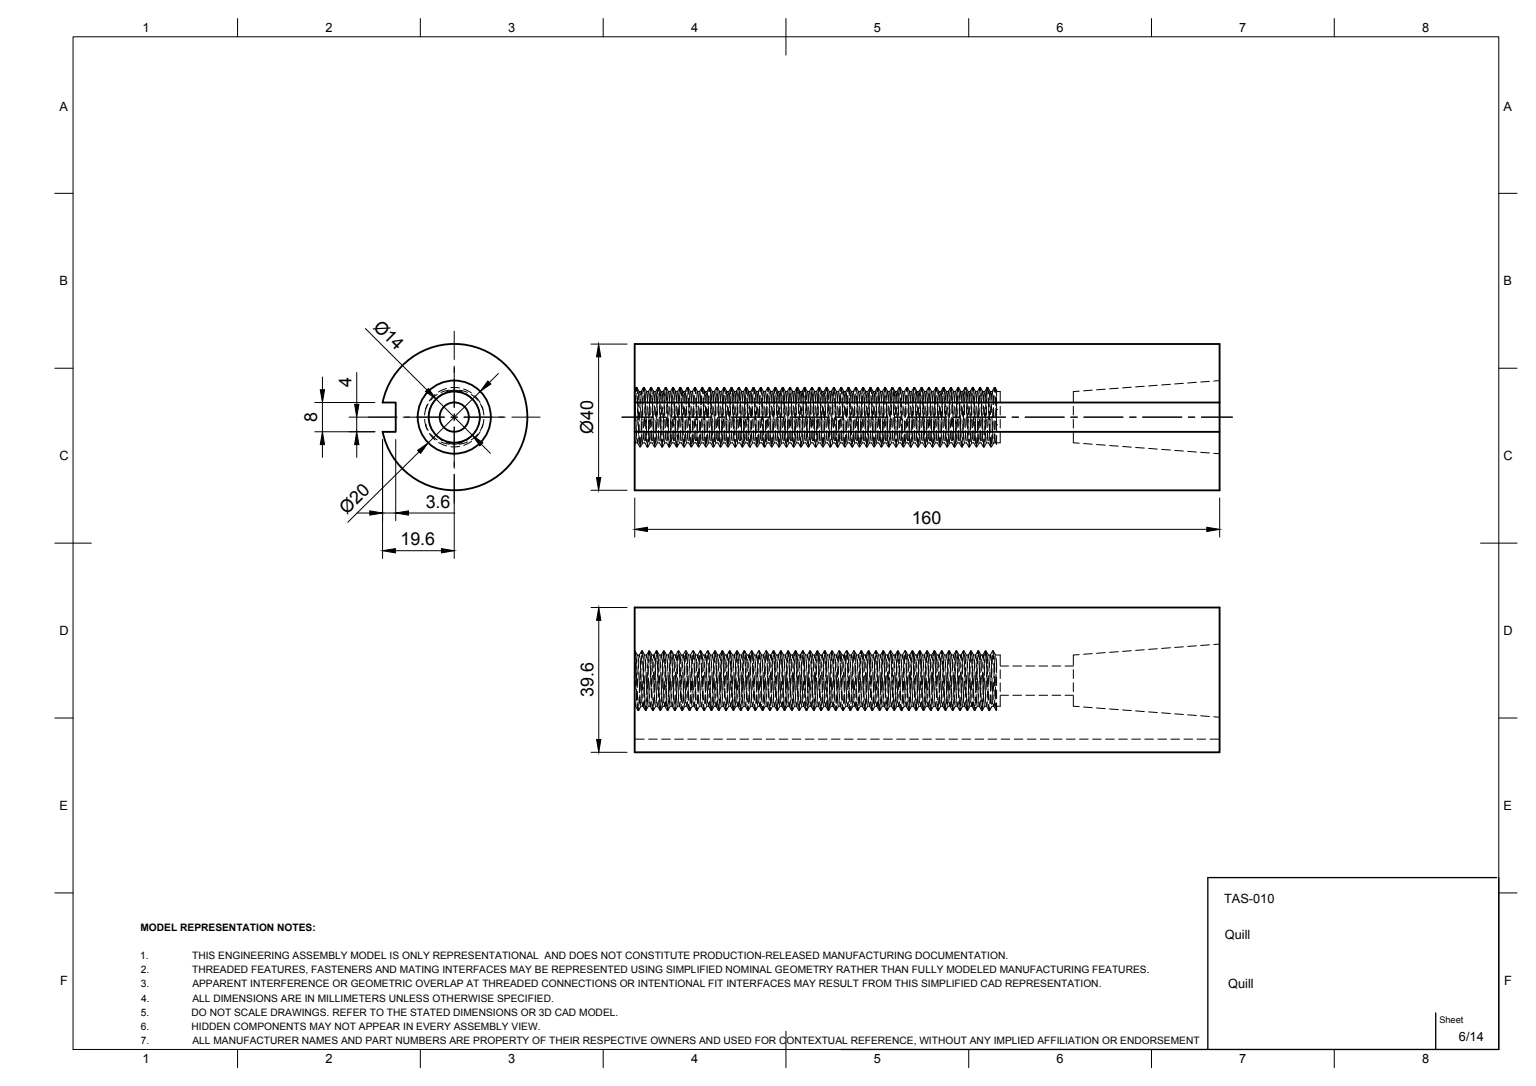
ISO-10303-21;
HEADER;
/* Generated by software containing ST-Developer
 * from STEP Tools, Inc. (www.steptools.com) 
 */

FILE_DESCRIPTION(
/* description */ (
'Independent keyed-quill tailstock, native coupled50mm slider andM16x2
 feed screw, conical dead center, bronze sleeves/thrust washers, cross
-pinned handwheel and bolted guide key. Custom center taper; no standa
rd taper compatibility, machine-bed compatibility or load rating assig
ned.'),
/* implementation_level */ '2;1');

FILE_NAME(
/* name */ 'Quill.step',
/* time_stamp */ '2026-11-14T07:17:36-08:00',
/* author */ (''),
/* organization */ (''),
/* preprocessor_version */ 'ST-DEVELOPER v20.2',
/* originating_system */ 'Autodesk Translation Framework v15.17.0.0',
/* authorisation */ '');

FILE_SCHEMA (('AUTOMOTIVE_DESIGN { 1 0 10303 214 3 1 1 }'));
ENDSEC;

DATA;
#10=MECHANICAL_DESIGN_GEOMETRIC_PRESENTATION_REPRESENTATION('',(#156),#289387);
#111=CONICAL_SURFACE('',#17511,8.5,0.0748598477107669);
#122=SHAPE_REPRESENTATION_RELATIONSHIP('SRR','None',#289457,#139);
#139=ADVANCED_BREP_SHAPE_REPRESENTATION('',(#173),#289373);
#156=STYLED_ITEM('',(#289551),#173);
#173=MANIFOLD_SOLID_BREP('Body1',#16844);
#218=FACE_BOUND('',#1502,.T.);
#219=FACE_BOUND('',#1508,.T.);
#220=FACE_BOUND('',#1513,.T.);
#221=FACE_BOUND('',#1517,.T.);
#293=B_SPLINE_SURFACE_WITH_KNOTS('',3,3,((#180613,#180614,#180615,#180616,
#180617,#180618,#180619,#180620,#180621,#180622,#180623,#180624,#180625,
#180626,#180627,#180628,#180629,#180630,#180631,#180632,#180633,#180634,
#180635,#180636,#180637,#180638,#180639,#180640,#180641,#180642,#180643,
#180644,#180645,#180646,#180647,#180648,#180649,#180650,#180651,#180652,
#180653,#180654,#180655,#180656,#180657,#180658,#180659,#180660,#180661,
#180662,#180663,#180664,#180665,#180666,#180667,#180668,#180669,#180670,
#180671,#180672,#180673,#180674,#180675,#180676,#180677,#180678,#180679,
#180680,#180681,#180682,#180683,#180684,#180685,#180686,#180687,#180688,
#180689,#180690,#180691,#180692,#180693,#180694,#180695,#180696,#180697,
#180698,#180699,#180700,#180701,#180702,#180703,#180704,#180705,#180706,
#180707,#180708,#180709,#180710,#180711,#180712,#180713,#180714,#180715,
#180716,#180717,#180718,#180719,#180720,#180721,#180722,#180723,#180724,
#180725,#180726,#180727,#180728,#180729,#180730,#180731,#180732,#180733,
#180734,#180735,#180736,#180737,#180738,#180739,#180740,#180741,#180742,
#180743,#180744,#180745,#180746,#180747,#180748,#180749,#180750,#180751,
#180752,#180753,#180754,#180755,#180756,#180757,#180758,#180759,#180760,
#180761,#180762,#180763,#180764,#180765,#180766,#180767,#180768,#180769,
#180770,#180771,#180772,#180773,#180774,#180775,#180776,#180777,#180778,
#180779,#180780,#180781,#180782,#180783,#180784,#180785,#180786,#180787,
#180788,#180789,#180790,#180791,#180792,#180793,#180794,#180795,#180796,
#180797,#180798,#180799,#180800,#180801,#180802,#180803,#180804,#180805,
#180806,#180807,#180808,#180809,#180810,#180811,#180812,#180813,#180814,
#180815,#180816,#180817,#180818,#180819,#180820,#180821,#180822,#180823,
#180824,#180825,#180826,#180827,#180828,#180829,#180830,#180831,#180832,
#180833,#180834,#180835,#180836,#180837,#180838,#180839,#180840,#180841,
#180842,#180843,#180844,#180845,#180846,#180847,#180848,#180849,#180850,
#180851,#180852,#180853,#180854,#180855,#180856,#180857,#180858,#180859,
#180860,#180861,#180862,#180863,#180864,#180865,#180866,#180867,#180868,
#180869,#180870,#180871,#180872,#180873,#180874,#180875,#180876,#180877,
#180878,#180879,#180880,#180881,#180882,#180883,#180884,#180885,#180886,
#180887,#180888,#180889,#180890,#180891,#180892,#180893,#180894,#180895,
#180896,#180897,#180898,#180899,#180900,#180901,#180902,#180903,#180904,
#180905,#180906,#180907,#180908,#180909,#180910,#180911,#180912,#180913,
#180914,#180915,#180916,#180917,#180918,#180919,#180920,#180921,#180922,
#180923,#180924,#180925,#180926,#180927,#180928,#180929,#180930,#180931,
#180932,#180933,#180934,#180935,#180936,#180937,#180938,#180939,#180940,
#180941,#180942,#180943,#180944,#180945,#180946,#180947,#180948,#180949,
#180950,#180951,#180952,#180953,#180954,#180955,#180956,#180957,#180958,
#180959,#180960,#180961,#180962,#180963,#180964,#180965,#180966,#180967,
#180968,#180969,#180970,#180971,#180972,#180973,#180974,#180975,#180976,
#180977,#180978,#180979,#180980,#180981,#180982,#180983,#180984,#180985,
#180986,#180987,#180988,#180989,#180990,#180991,#180992,#180993,#180994,
#180995,#180996,#180997,#180998,#180999,#181000,#181001,#181002,#181003,
#181004,#181005,#181006,#181007,#181008,#181009,#181010,#181011,#181012,
#181013,#181014,#181015,#181016,#181017,#181018,#181019,#181020,#181021,
#181022,#181023,#181024,#181025,#181026,#181027,#181028,#181029,#181030,
#181031,#181032,#181033,#181034,#181035,#181036,#181037,#181038,#181039,
#181040,#181041,#181042,#181043,#181044,#181045,#181046,#181047,#181048,
#181049,#181050,#181051,#181052,#181053,#181054,#181055,#181056,#181057,
#181058,#181059,#181060,#181061,#181062,#181063,#181064,#181065,#181066,
#181067,#181068,#181069,#181070,#181071,#181072,#181073,#181074,#181075,
#181076,#181077,#181078,#181079,#181080,#181081,#181082,#181083,#181084,
#181085,#181086,#181087,#181088,#181089,#181090,#181091,#181092,#181093,
#181094,#181095,#181096,#181097,#181098,#181099,#181100,#181101,#181102,
#181103,#181104,#181105,#181106,#181107,#181108,#181109,#181110,#181111,
#181112,#181113,#181114,#181115,#181116,#181117,#181118,#181119,#181120,
#181121,#181122,#181123,#181124,#181125,#181126,#181127,#181128,#181129,
#181130,#181131,#181132,#181133,#181134,#181135,#181136,#181137,#181138,
#181139,#181140,#181141,#181142,#181143,#181144,#181145,#181146,#181147,
#181148,#181149,#181150),(#181151,#181152,#181153,#181154,#181155,#181156,
#181157,#181158,#181159,#181160,#181161,#181162,#181163,#181164,#181165,
#181166,#181167,#181168,#181169,#181170,#181171,#181172,#181173,#181174,
#181175,#181176,#181177,#181178,#181179,#181180,#181181,#181182,#181183,
#181184,#181185,#181186,#181187,#181188,#181189,#181190,#181191,#181192,
#181193,#181194,#181195,#181196,#181197,#181198,#181199,#181200,#181201,
#181202,#181203,#181204,#181205,#181206,#181207,#181208,#181209,#181210,
#181211,#181212,#181213,#181214,#181215,#181216,#181217,#181218,#181219,
#181220,#181221,#181222,#181223,#181224,#181225,#181226,#181227,#181228,
#181229,#181230,#181231,#181232,#181233,#181234,#181235,#181236,#181237,
#181238,#181239,#181240,#181241,#181242,#181243,#181244,#181245,#181246,
#181247,#181248,#181249,#181250,#181251,#181252,#181253,#181254,#181255,
#181256,#181257,#181258,#181259,#181260,#181261,#181262,#181263,#181264,
#181265,#181266,#181267,#181268,#181269,#181270,#181271,#181272,#181273,
#181274,#181275,#181276,#181277,#181278,#181279,#181280,#181281,#181282,
#181283,#181284,#181285,#181286,#181287,#181288,#181289,#181290,#181291,
#181292,#181293,#181294,#181295,#181296,#181297,#181298,#181299,#181300,
#181301,#181302,#181303,#181304,#181305,#181306,#181307,#181308,#181309,
#181310,#181311,#181312,#181313,#181314,#181315,#181316,#181317,#181318,
#181319,#181320,#181321,#181322,#181323,#181324,#181325,#181326,#181327,
#181328,#181329,#181330,#181331,#181332,#181333,#181334,#181335,#181336,
#181337,#181338,#181339,#181340,#181341,#181342,#181343,#181344,#181345,
#181346,#181347,#181348,#181349,#181350,#181351,#181352,#181353,#181354,
#181355,#181356,#181357,#181358,#181359,#181360,#181361,#181362,#181363,
#181364,#181365,#181366,#181367,#181368,#181369,#181370,#181371,#181372,
#181373,#181374,#181375,#181376,#181377,#181378,#181379,#181380,#181381,
#181382,#181383,#181384,#181385,#181386,#181387,#181388,#181389,#181390,
#181391,#181392,#181393,#181394,#181395,#181396,#181397,#181398,#181399,
#181400,#181401,#181402,#181403,#181404,#181405,#181406,#181407,#181408,
#181409,#181410,#181411,#181412,#181413,#181414,#181415,#181416,#181417,
#181418,#181419,#181420,#181421,#181422,#181423,#181424,#181425,#181426,
#181427,#181428,#181429,#181430,#181431,#181432,#181433,#181434,#181435,
#181436,#181437,#181438,#181439,#181440,#181441,#181442,#181443,#181444,
#181445,#181446,#181447,#181448,#181449,#181450,#181451,#181452,#181453,
#181454,#181455,#181456,#181457,#181458,#181459,#181460,#181461,#181462,
#181463,#181464,#181465,#181466,#181467,#181468,#181469,#181470,#181471,
#181472,#181473,#181474,#181475,#181476,#181477,#181478,#181479,#181480,
#181481,#181482,#181483,#181484,#181485,#181486,#181487,#181488,#181489,
#181490,#181491,#181492,#181493,#181494,#181495,#181496,#181497,#181498,
#181499,#181500,#181501,#181502,#181503,#181504,#181505,#181506,#181507,
#181508,#181509,#181510,#181511,#181512,#181513,#181514,#181515,#181516,
#181517,#181518,#181519,#181520,#181521,#181522,#181523,#181524,#181525,
#181526,#181527,#181528,#181529,#181530,#181531,#181532,#181533,#181534,
#181535,#181536,#181537,#181538,#181539,#181540,#181541,#181542,#181543,
#181544,#181545,#181546,#181547,#181548,#181549,#181550,#181551,#181552,
#181553,#181554,#181555,#181556,#181557,#181558,#181559,#181560,#181561,
#181562,#181563,#181564,#181565,#181566,#181567,#181568,#181569,#181570,
#181571,#181572,#181573,#181574,#181575,#181576,#181577,#181578,#181579,
#181580,#181581,#181582,#181583,#181584,#181585,#181586,#181587,#181588,
#181589,#181590,#181591,#181592,#181593,#181594,#181595,#181596,#181597,
#181598,#181599,#181600,#181601,#181602,#181603,#181604,#181605,#181606,
#181607,#181608,#181609,#181610,#181611,#181612,#181613,#181614,#181615,
#181616,#181617,#181618,#181619,#181620,#181621,#181622,#181623,#181624,
#181625,#181626,#181627,#181628,#181629,#181630,#181631,#181632,#181633,
#181634,#181635,#181636,#181637,#181638,#181639,#181640,#181641,#181642,
#181643,#181644,#181645,#181646,#181647,#181648,#181649,#181650,#181651,
#181652,#181653,#181654,#181655,#181656,#181657,#181658,#181659,#181660,
#181661,#181662,#181663,#181664,#181665,#181666,#181667,#181668,#181669,
#181670,#181671,#181672,#181673,#181674,#181675,#181676,#181677,#181678,
#181679,#181680,#181681,#181682,#181683,#181684,#181685,#181686,#181687,
#181688),(#181689,#181690,#181691,#181692,#181693,#181694,#181695,#181696,
#181697,#181698,#181699,#181700,#181701,#181702,#181703,#181704,#181705,
#181706,#181707,#181708,#181709,#181710,#181711,#181712,#181713,#181714,
#181715,#181716,#181717,#181718,#181719,#181720,#181721,#181722,#181723,
#181724,#181725,#181726,#181727,#181728,#181729,#181730,#181731,#181732,
#181733,#181734,#181735,#181736,#181737,#181738,#181739,#181740,#181741,
#181742,#181743,#181744,#181745,#181746,#181747,#181748,#181749,#181750,
#181751,#181752,#181753,#181754,#181755,#181756,#181757,#181758,#181759,
#181760,#181761,#181762,#181763,#181764,#181765,#181766,#181767,#181768,
#181769,#181770,#181771,#181772,#181773,#181774,#181775,#181776,#181777,
#181778,#181779,#181780,#181781,#181782,#181783,#181784,#181785,#181786,
#181787,#181788,#181789,#181790,#181791,#181792,#181793,#181794,#181795,
#181796,#181797,#181798,#181799,#181800,#181801,#181802,#181803,#181804,
#181805,#181806,#181807,#181808,#181809,#181810,#181811,#181812,#181813,
#181814,#181815,#181816,#181817,#181818,#181819,#181820,#181821,#181822,
#181823,#181824,#181825,#181826,#181827,#181828,#181829,#181830,#181831,
#181832,#181833,#181834,#181835,#181836,#181837,#181838,#181839,#181840,
#181841,#181842,#181843,#181844,#181845,#181846,#181847,#181848,#181849,
#181850,#181851,#181852,#181853,#181854,#181855,#181856,#181857,#181858,
#181859,#181860,#181861,#181862,#181863,#181864,#181865,#181866,#181867,
#181868,#181869,#181870,#181871,#181872,#181873,#181874,#181875,#181876,
#181877,#181878,#181879,#181880,#181881,#181882,#181883,#181884,#181885,
#181886,#181887,#181888,#181889,#181890,#181891,#181892,#181893,#181894,
#181895,#181896,#181897,#181898,#181899,#181900,#181901,#181902,#181903,
#181904,#181905,#181906,#181907,#181908,#181909,#181910,#181911,#181912,
#181913,#181914,#181915,#181916,#181917,#181918,#181919,#181920,#181921,
#181922,#181923,#181924,#181925,#181926,#181927,#181928,#181929,#181930,
#181931,#181932,#181933,#181934,#181935,#181936,#181937,#181938,#181939,
#181940,#181941,#181942,#181943,#181944,#181945,#181946,#181947,#181948,
#181949,#181950,#181951,#181952,#181953,#181954,#181955,#181956,#181957,
#181958,#181959,#181960,#181961,#181962,#181963,#181964,#181965,#181966,
#181967,#181968,#181969,#181970,#181971,#181972,#181973,#181974,#181975,
#181976,#181977,#181978,#181979,#181980,#181981,#181982,#181983,#181984,
#181985,#181986,#181987,#181988,#181989,#181990,#181991,#181992,#181993,
#181994,#181995,#181996,#181997,#181998,#181999,#182000,#182001,#182002,
#182003,#182004,#182005,#182006,#182007,#182008,#182009,#182010,#182011,
#182012,#182013,#182014,#182015,#182016,#182017,#182018,#182019,#182020,
#182021,#182022,#182023,#182024,#182025,#182026,#182027,#182028,#182029,
#182030,#182031,#182032,#182033,#182034,#182035,#182036,#182037,#182038,
#182039,#182040,#182041,#182042,#182043,#182044,#182045,#182046,#182047,
#182048,#182049,#182050,#182051,#182052,#182053,#182054,#182055,#182056,
#182057,#182058,#182059,#182060,#182061,#182062,#182063,#182064,#182065,
#182066,#182067,#182068,#182069,#182070,#182071,#182072,#182073,#182074,
#182075,#182076,#182077,#182078,#182079,#182080,#182081,#182082,#182083,
#182084,#182085,#182086,#182087,#182088,#182089,#182090,#182091,#182092,
#182093,#182094,#182095,#182096,#182097,#182098,#182099,#182100,#182101,
#182102,#182103,#182104,#182105,#182106,#182107,#182108,#182109,#182110,
#182111,#182112,#182113,#182114,#182115,#182116,#182117,#182118,#182119,
#182120,#182121,#182122,#182123,#182124,#182125,#182126,#182127,#182128,
#182129,#182130,#182131,#182132,#182133,#182134,#182135,#182136,#182137,
#182138,#182139,#182140,#182141,#182142,#182143,#182144,#182145,#182146,
#182147,#182148,#182149,#182150,#182151,#182152,#182153,#182154,#182155,
#182156,#182157,#182158,#182159,#182160,#182161,#182162,#182163,#182164,
#182165,#182166,#182167,#182168,#182169,#182170,#182171,#182172,#182173,
#182174,#182175,#182176,#182177,#182178,#182179,#182180,#182181,#182182,
#182183,#182184,#182185,#182186,#182187,#182188,#182189,#182190,#182191,
#182192,#182193,#182194,#182195,#182196,#182197,#182198,#182199,#182200,
#182201,#182202,#182203,#182204,#182205,#182206,#182207,#182208,#182209,
#182210,#182211,#182212,#182213,#182214,#182215,#182216,#182217,#182218,
#182219,#182220,#182221,#182222,#182223,#182224,#182225,#182226),(#182227,
#182228,#182229,#182230,#182231,#182232,#182233,#182234,#182235,#182236,
#182237,#182238,#182239,#182240,#182241,#182242,#182243,#182244,#182245,
#182246,#182247,#182248,#182249,#182250,#182251,#182252,#182253,#182254,
#182255,#182256,#182257,#182258,#182259,#182260,#182261,#182262,#182263,
#182264,#182265,#182266,#182267,#182268,#182269,#182270,#182271,#182272,
#182273,#182274,#182275,#182276,#182277,#182278,#182279,#182280,#182281,
#182282,#182283,#182284,#182285,#182286,#182287,#182288,#182289,#182290,
#182291,#182292,#182293,#182294,#182295,#182296,#182297,#182298,#182299,
#182300,#182301,#182302,#182303,#182304,#182305,#182306,#182307,#182308,
#182309,#182310,#182311,#182312,#182313,#182314,#182315,#182316,#182317,
#182318,#182319,#182320,#182321,#182322,#182323,#182324,#182325,#182326,
#182327,#182328,#182329,#182330,#182331,#182332,#182333,#182334,#182335,
#182336,#182337,#182338,#182339,#182340,#182341,#182342,#182343,#182344,
#182345,#182346,#182347,#182348,#182349,#182350,#182351,#182352,#182353,
#182354,#182355,#182356,#182357,#182358,#182359,#182360,#182361,#182362,
#182363,#182364,#182365,#182366,#182367,#182368,#182369,#182370,#182371,
#182372,#182373,#182374,#182375,#182376,#182377,#182378,#182379,#182380,
#182381,#182382,#182383,#182384,#182385,#182386,#182387,#182388,#182389,
#182390,#182391,#182392,#182393,#182394,#182395,#182396,#182397,#182398,
#182399,#182400,#182401,#182402,#182403,#182404,#182405,#182406,#182407,
#182408,#182409,#182410,#182411,#182412,#182413,#182414,#182415,#182416,
#182417,#182418,#182419,#182420,#182421,#182422,#182423,#182424,#182425,
#182426,#182427,#182428,#182429,#182430,#182431,#182432,#182433,#182434,
#182435,#182436,#182437,#182438,#182439,#182440,#182441,#182442,#182443,
#182444,#182445,#182446,#182447,#182448,#182449,#182450,#182451,#182452,
#182453,#182454,#182455,#182456,#182457,#182458,#182459,#182460,#182461,
#182462,#182463,#182464,#182465,#182466,#182467,#182468,#182469,#182470,
#182471,#182472,#182473,#182474,#182475,#182476,#182477,#182478,#182479,
#182480,#182481,#182482,#182483,#182484,#182485,#182486,#182487,#182488,
#182489,#182490,#182491,#182492,#182493,#182494,#182495,#182496,#182497,
#182498,#182499,#182500,#182501,#182502,#182503,#182504,#182505,#182506,
#182507,#182508,#182509,#182510,#182511,#182512,#182513,#182514,#182515,
#182516,#182517,#182518,#182519,#182520,#182521,#182522,#182523,#182524,
#182525,#182526,#182527,#182528,#182529,#182530,#182531,#182532,#182533,
#182534,#182535,#182536,#182537,#182538,#182539,#182540,#182541,#182542,
#182543,#182544,#182545,#182546,#182547,#182548,#182549,#182550,#182551,
#182552,#182553,#182554,#182555,#182556,#182557,#182558,#182559,#182560,
#182561,#182562,#182563,#182564,#182565,#182566,#182567,#182568,#182569,
#182570,#182571,#182572,#182573,#182574,#182575,#182576,#182577,#182578,
#182579,#182580,#182581,#182582,#182583,#182584,#182585,#182586,#182587,
#182588,#182589,#182590,#182591,#182592,#182593,#182594,#182595,#182596,
#182597,#182598,#182599,#182600,#182601,#182602,#182603,#182604,#182605,
#182606,#182607,#182608,#182609,#182610,#182611,#182612,#182613,#182614,
#182615,#182616,#182617,#182618,#182619,#182620,#182621,#182622,#182623,
#182624,#182625,#182626,#182627,#182628,#182629,#182630,#182631,#182632,
#182633,#182634,#182635,#182636,#182637,#182638,#182639,#182640,#182641,
#182642,#182643,#182644,#182645,#182646,#182647,#182648,#182649,#182650,
#182651,#182652,#182653,#182654,#182655,#182656,#182657,#182658,#182659,
#182660,#182661,#182662,#182663,#182664,#182665,#182666,#182667,#182668,
#182669,#182670,#182671,#182672,#182673,#182674,#182675,#182676,#182677,
#182678,#182679,#182680,#182681,#182682,#182683,#182684,#182685,#182686,
#182687,#182688,#182689,#182690,#182691,#182692,#182693,#182694,#182695,
#182696,#182697,#182698,#182699,#182700,#182701,#182702,#182703,#182704,
#182705,#182706,#182707,#182708,#182709,#182710,#182711,#182712,#182713,
#182714,#182715,#182716,#182717,#182718,#182719,#182720,#182721,#182722,
#182723,#182724,#182725,#182726,#182727,#182728,#182729,#182730,#182731,
#182732,#182733,#182734,#182735,#182736,#182737,#182738,#182739,#182740,
#182741,#182742,#182743,#182744,#182745,#182746,#182747,#182748,#182749,
#182750,#182751,#182752,#182753,#182754,#182755,#182756,#182757,#182758,
#182759,#182760,#182761,#182762,#182763,#182764)),.UNSPECIFIED.,.F.,.F.,
 .F.,(4,4),(4,1,1,1,1,1,1,1,1,1,1,1,1,1,1,1,1,1,1,1,1,1,1,1,1,1,1,1,1,1,
1,1,1,1,1,1,1,1,1,1,1,1,1,1,1,1,1,1,1,1,1,1,1,1,1,1,1,1,1,1,1,1,1,1,1,1,
1,1,1,1,1,1,1,1,1,1,1,1,1,1,1,1,1,1,1,1,1,1,1,1,1,1,1,1,1,1,1,1,1,1,1,1,
1,1,1,1,1,1,1,1,1,1,1,1,1,1,1,1,1,1,1,1,1,1,1,1,1,1,1,1,1,1,1,1,1,1,1,1,
1,1,1,1,1,1,1,1,1,1,1,1,1,1,1,1,1,1,1,1,1,1,1,1,1,1,1,1,1,1,1,1,1,1,1,1,
1,1,1,1,1,1,1,1,1,1,1,1,1,1,1,1,1,1,1,1,1,1,1,1,1,1,1,1,1,1,1,1,1,1,1,1,
1,1,1,1,1,1,1,1,1,1,1,1,1,1,1,1,1,1,1,1,1,1,1,1,1,1,1,1,1,1,1,1,1,1,1,1,
1,1,1,1,1,1,1,1,1,1,1,1,1,1,1,1,1,1,1,1,1,1,1,1,1,1,1,1,1,1,1,1,1,1,1,1,
1,1,1,1,1,1,1,1,1,1,1,1,1,1,1,1,1,1,1,1,1,1,1,1,1,1,1,1,1,1,1,1,1,1,1,1,
1,1,1,1,1,1,1,1,1,1,1,1,1,1,1,1,1,1,1,1,1,1,1,1,1,1,1,1,1,1,1,1,1,1,1,1,
1,1,1,1,1,1,1,1,1,1,1,1,1,1,1,1,1,1,1,1,1,1,1,1,1,1,1,1,1,1,1,1,1,1,1,1,
1,1,1,1,1,1,1,1,1,1,1,1,1,1,1,1,1,1,1,1,1,1,1,1,1,1,1,1,1,1,1,1,1,1,1,1,
1,1,1,1,1,1,1,1,1,1,1,1,1,1,1,1,1,1,1,1,1,1,1,1,1,1,1,1,1,1,1,1,1,1,1,1,
1,1,1,1,1,1,1,1,1,1,1,1,1,1,1,1,1,1,1,1,1,1,1,1,1,1,1,1,1,1,1,1,1,1,1,1,
1,1,1,1,1,1,1,1,1,1,1,1,1,1,1,1,1,1,1,1,1,1,1,1,1,1,1,1,1,1,1,1,1,1,1,1,
1,4),(-0.000902833525214243,0.131480103365952),(11.8547611101884,12.3533763570464,
12.851844900354,13.3503134436615,13.8487819869691,14.3472505302766,14.8457190735842,
15.8426561601993,16.8395932468144,17.338061790122,17.8365303334295,18.3349988767371,
18.8334674200446,19.3319359633522,19.8304045066598,20.3288730499673,20.8273415932749,
21.82427867989,22.3227472231976,22.8212157665051,23.8181528531202,24.3166213964278,
24.8150899397353,25.3135584830429,25.8120270263505,26.310495569658,26.8089641129656,
27.3074326562731,27.8059011995807,28.8028382861958,29.3013068295034,29.7997753728109,
30.796712459426,31.2951810027336,31.7936495460412,32.2921180893487,32.7905866326563,
33.2890551759638,33.7875237192714,34.2859922625789,34.7844608058865,35.7813978925016,
36.2798664358092,36.7783349791167,37.7752720657319,38.2737406090394,38.772209152347,
39.2706776956545,39.7691462389621,40.2676147822696,40.7660833255772,41.2645518688848,
41.7630204121923,42.7599574988074,43.258426042115,43.7568945854225,44.7538316720377,
45.2523002153452,45.7507687586528,46.2492373019603,46.7477058452679,47.2461743885754,
47.744642931883,48.2431114751906,48.7415800184981,49.7385171051132,50.2369856484208,
50.7354541917284,51.7323912783435,52.230859821651,52.7293283649586,53.2277969082661,
53.7262654515737,54.2247339948813,54.7232025381888,55.2216710814964,55.7201396248039,
56.7170767114191,57.2155452547266,57.7140137980342,58.7109508846493,59.2094194279568,
59.7078879712644,60.206356514572,60.7048250578795,61.2032936011871,61.7017621444946,
62.2002306878022,62.6986992311097,63.6956363177249,64.1941048610324,64.69257340434,
65.6895104909551,66.1879790342627,66.6864475775702,67.1849161208778,67.6833846641853,
68.1818532074929,68.6803217508004,69.178790294108,69.6772588374156,70.6741959240307,
71.1726644673382,71.6711330106458,72.6680700972609,73.1665386405685,73.665007183876,
74.1634757271836,74.6619442704911,75.1604128137987,75.6588813571063,76.1573499004138,
76.6558184437214,77.6527555303365,78.151224073644,78.6496926169516,79.6466297035667,
80.1450982468743,80.6435667901818,81.1420353334894,81.6405038767969,82.1389724201045,
82.6374409634121,83.1359095067196,83.6343780500272,84.6313151366423,85.1297836799499,
85.6282522232574,86.6251893098725,87.1236578531801,87.6221263964876,88.1205949397952,
88.6190634831028,89.1175320264103,89.6160005697179,90.1144691130254,90.612937656333,
91.6098747429481,92.1083432862557,92.6068118295632,93.6037489161783,94.1022174594859,
94.6006860027935,95.099154546101,95.5976230894086,96.0960916327161,96.5945601760237,
97.0930287193312,97.5914972626388,98.5884343492539,99.0869028925615,99.585371435869,
100.582308522484,101.080777065792,101.579245609099,102.077714152407,102.576182695714,
103.074651239022,103.573119782329,104.071588325637,104.570056868945,105.56699395556,
106.065462498867,106.563931042175,107.56086812879,108.059336672098,108.557805215405,
109.056273758713,109.55474230202,110.053210845328,110.551679388635,111.050147931943,
111.54861647525,112.545553561866,113.044022105173,113.542490648481,114.539427735096,
115.037896278403,115.536364821711,116.034833365018,116.533301908326,117.031770451634,
117.530238994941,118.028707538249,118.527176081556,119.524113168171,120.022581711479,
120.521050254786,121.517987341402,122.016455884709,122.514924428017,123.013392971324,
123.511861514632,124.010330057939,124.508798601247,125.007267144555,125.505735687862,
126.502672774477,127.001141317785,127.499609861092,128.496546947707,128.995015491015,
129.493484034323,129.99195257763,130.490421120938,130.988889664245,131.487358207553,
131.98582675086,132.484295294168,133.481232380783,133.979700924091,134.478169467398,
135.475106554013,135.973575097321,136.472043640628,136.970512183936,137.468980727243,
137.967449270551,138.465917813859,138.964386357166,139.462854900474,140.459791987089,
140.958260530396,141.456729073704,142.453666160319,142.952134703627,143.450603246934,
143.949071790242,144.447540333549,144.946008876857,145.444477420164,145.942945963472,
146.441414506779,147.438351593395,147.936820136702,148.43528868001,149.432225766625,
149.930694309932,150.42916285324,150.927631396547,151.426099939855,151.924568483163,
152.42303702647,152.921505569778,153.419974113085,154.4169111997,154.915379743008,
155.413848286316,156.410785372931,156.909253916238,157.407722459546,157.906191002853,
158.404659546161,158.903128089468,159.401596632776,159.900065176084,160.398533719391,
161.395470806006,161.893939349314,162.392407892621,163.389344979236,163.887813522544,
164.386282065852,164.884750609159,165.383219152467,165.881687695774,166.380156239082,
167.377093325697,168.374030412312,169.370967498927,169.869436042235,170.367904585542,
170.86637312885,171.364841672157,172.361778758772,173.358715845388,174.355652932003,
174.85412147531,175.352590018618,176.349527105233,176.847995648541,177.346464191848,
177.844932735156,178.343401278463,178.841869821771,179.340338365078,179.838806908386,
180.337275451693,181.334212538309,181.832681081616,182.331149624924,183.328086711539,
183.826555254846,184.325023798154,184.823492341461,185.321960884769,185.820429428077,
186.318897971384,186.817366514692,187.315835057999,188.312772144614,188.811240687922,
189.309709231229,190.306646317845,190.805114861152,191.30358340446,191.802051947767,
192.300520491075,192.798989034382,193.29745757769,193.795926120997,194.294394664305,
195.29133175092,195.789800294228,196.288268837535,197.28520592415,197.783674467458,
198.282143010766,198.780611554073,199.279080097381,199.777548640688,200.276017183996,
200.774485727303,201.272954270611,202.269891357226,202.768359900534,203.266828443841,
204.263765530456,204.762234073764,205.260702617071,205.759171160379,206.257639703686,
206.756108246994,207.254576790302,207.753045333609,208.251513876917,209.248450963532,
209.746919506839,210.245388050147,211.242325136762,211.74079368007,212.239262223377,
212.737730766685,213.236199309992,213.7346678533,214.233136396607,214.731604939915,
215.230073483222,216.227010569838,216.725479113145,217.223947656453,218.220884743068,
218.719353286375,219.217821829683,219.71629037299,220.214758916298,220.713227459606,
221.211696002913,221.710164546221,222.208633089528,223.205570176143,223.704038719451,
224.202507262759,225.199444349374,225.697912892681,226.196381435989,226.694849979296,
227.193318522604,227.691787065911,228.190255609219,228.688724152527,229.187192695834,
230.184129782449,230.682598325757,231.181066869064,232.178003955679,232.676472498987,
233.174941042295,233.673409585602,234.17187812891,234.670346672217,235.168815215525,
235.667283758832,236.16575230214,237.162689388755,237.661157932063,238.15962647537,
239.156563561985,239.655032105293,240.1535006486,240.651969191908,241.150437735215,
241.648906278523,242.147374821831,242.645843365138,243.144311908446,244.141248995061,
244.639717538368,245.138186081676,246.135123168291,246.633591711599,247.132060254906,
247.630528798214,248.128997341521,248.627465884829,249.125934428136,249.624402971444,
250.122871514752,251.119808601367,251.618277144674,252.116745687982,253.113682774597,
253.612151317904,254.110619861212,254.60908840452,255.107556947827,255.606025491135,
256.104494034442,256.60296257775,257.101431121057,258.098368207672,258.59683675098,
259.095305294288,260.092242380903,260.59071092421,261.089179467518,261.587648010825,
262.086116554133,262.58458509744,263.083053640748,263.581522184056,264.079990727363,
265.076927813978,265.575396357286,266.073864900593,267.070801987209,267.569270530516,
268.067739073824,268.566207617131,269.064676160439,269.563144703746,270.061613247054,
270.560081790361,271.058550333669,272.055487420284,272.553955963592,273.052424506899,
274.049361593514,274.547830136822,275.046298680129,275.544767223437,276.043235766745,
276.541704310052,277.04017285336,277.538641396667,278.037109939975,279.03404702659,
279.532515569897,280.030984113205,281.02792119982,281.526389743128,282.024858286435,
282.523326829743,283.02179537305,283.520263916358,284.018732459666,284.517201002973,
285.015669546281,286.012606632896,286.511075176203,287.009543719511,288.006480806126,
288.504949349434,289.003417892741,289.501886436049,290.000354979356,290.498823522664,
290.997292065971,291.495760609279,291.994229152586,292.991166239202,293.489634782509,
293.988103325817,294.985040412432,295.483508955739,295.981977499047,296.480446042354,
296.978914585662,297.47738312897,297.975851672277,298.474320215585,298.972788758892,
299.969725845507,300.468194388815,300.966662932122,301.963600018738,302.462068562045,
302.960537105353,303.45900564866,303.957474191968,304.455942735275,304.954411278583,
305.452879821891,305.951348365198,306.948285451813,307.446753995121,307.945222538428,
308.942159625043,309.440628168351,309.939096711659,310.437565254966,310.936033798274,
311.434502341581,311.932970884889,312.431439428196,312.929907971504,313.926845058119,
314.425313601427,314.923782144734,315.920719231349,316.419187774657,316.917656317964,
317.416124861272,317.914593404579,318.413061947887,318.911530491195,319.409999034502,
319.90846757781,320.905404664425,321.90234175104,322.400810294347,322.899278837655,
323.397747380963,323.89621592427,324.394684467578,324.893207835215),
 .UNSPECIFIED.);
#294=B_SPLINE_SURFACE_WITH_KNOTS('',3,3,((#182877,#182878,#182879,#182880,
#182881,#182882,#182883,#182884,#182885,#182886,#182887,#182888,#182889,
#182890,#182891,#182892,#182893,#182894,#182895,#182896,#182897,#182898,
#182899,#182900,#182901,#182902,#182903,#182904,#182905,#182906,#182907,
#182908,#182909,#182910,#182911,#182912,#182913,#182914,#182915,#182916,
#182917,#182918,#182919,#182920,#182921,#182922,#182923,#182924,#182925,
#182926,#182927,#182928,#182929,#182930,#182931,#182932,#182933,#182934,
#182935,#182936,#182937,#182938,#182939,#182940,#182941,#182942,#182943,
#182944,#182945,#182946,#182947,#182948,#182949,#182950,#182951,#182952,
#182953,#182954,#182955,#182956,#182957,#182958,#182959,#182960,#182961,
#182962,#182963,#182964,#182965,#182966,#182967,#182968,#182969,#182970,
#182971,#182972,#182973,#182974,#182975,#182976,#182977,#182978,#182979,
#182980,#182981,#182982,#182983,#182984,#182985,#182986,#182987,#182988,
#182989,#182990,#182991,#182992,#182993,#182994,#182995,#182996,#182997,
#182998,#182999,#183000,#183001,#183002,#183003,#183004,#183005,#183006,
#183007,#183008,#183009,#183010,#183011,#183012,#183013,#183014,#183015,
#183016,#183017,#183018,#183019,#183020,#183021,#183022,#183023,#183024,
#183025,#183026,#183027,#183028,#183029,#183030,#183031,#183032,#183033,
#183034,#183035,#183036,#183037,#183038,#183039,#183040,#183041,#183042,
#183043,#183044,#183045,#183046,#183047,#183048,#183049,#183050,#183051,
#183052,#183053,#183054,#183055,#183056,#183057,#183058,#183059,#183060,
#183061,#183062,#183063,#183064,#183065,#183066,#183067,#183068,#183069,
#183070,#183071,#183072,#183073,#183074,#183075,#183076,#183077,#183078,
#183079,#183080,#183081,#183082,#183083,#183084,#183085,#183086,#183087,
#183088,#183089,#183090,#183091,#183092,#183093,#183094,#183095,#183096,
#183097,#183098,#183099,#183100,#183101,#183102,#183103,#183104,#183105,
#183106,#183107,#183108,#183109,#183110,#183111,#183112,#183113,#183114,
#183115,#183116,#183117,#183118,#183119,#183120,#183121,#183122,#183123,
#183124,#183125,#183126,#183127,#183128,#183129,#183130,#183131,#183132,
#183133,#183134,#183135,#183136,#183137,#183138,#183139,#183140,#183141,
#183142,#183143,#183144,#183145,#183146,#183147,#183148,#183149,#183150,
#183151,#183152,#183153,#183154,#183155,#183156,#183157,#183158,#183159,
#183160,#183161,#183162,#183163,#183164,#183165,#183166,#183167,#183168,
#183169,#183170,#183171,#183172,#183173,#183174,#183175,#183176,#183177,
#183178,#183179,#183180,#183181,#183182,#183183,#183184,#183185,#183186,
#183187,#183188,#183189,#183190,#183191,#183192,#183193,#183194,#183195,
#183196,#183197,#183198,#183199,#183200,#183201,#183202,#183203,#183204,
#183205,#183206,#183207,#183208,#183209,#183210,#183211,#183212,#183213,
#183214,#183215,#183216,#183217,#183218,#183219,#183220,#183221,#183222,
#183223,#183224,#183225,#183226,#183227,#183228,#183229,#183230,#183231,
#183232,#183233,#183234,#183235,#183236,#183237,#183238,#183239,#183240,
#183241,#183242,#183243,#183244,#183245,#183246,#183247,#183248,#183249,
#183250,#183251,#183252,#183253,#183254,#183255,#183256,#183257,#183258,
#183259,#183260,#183261,#183262,#183263,#183264,#183265,#183266,#183267,
#183268,#183269,#183270,#183271,#183272,#183273,#183274,#183275,#183276,
#183277,#183278,#183279,#183280,#183281,#183282,#183283,#183284,#183285,
#183286,#183287,#183288,#183289,#183290,#183291,#183292,#183293,#183294,
#183295,#183296,#183297,#183298,#183299,#183300,#183301,#183302,#183303,
#183304,#183305,#183306,#183307,#183308,#183309,#183310,#183311,#183312,
#183313,#183314,#183315,#183316,#183317,#183318,#183319,#183320,#183321,
#183322,#183323,#183324,#183325,#183326,#183327,#183328,#183329,#183330,
#183331,#183332,#183333,#183334,#183335,#183336,#183337,#183338,#183339,
#183340,#183341,#183342,#183343,#183344,#183345,#183346,#183347,#183348,
#183349,#183350,#183351,#183352,#183353,#183354,#183355,#183356,#183357,
#183358,#183359,#183360,#183361,#183362,#183363,#183364,#183365,#183366,
#183367,#183368,#183369,#183370,#183371,#183372,#183373,#183374,#183375,
#183376,#183377,#183378,#183379,#183380,#183381,#183382,#183383,#183384,
#183385,#183386,#183387,#183388,#183389,#183390,#183391,#183392,#183393,
#183394,#183395,#183396,#183397,#183398,#183399,#183400,#183401,#183402,
#183403,#183404,#183405,#183406,#183407,#183408,#183409,#183410,#183411,
#183412,#183413,#183414),(#183415,#183416,#183417,#183418,#183419,#183420,
#183421,#183422,#183423,#183424,#183425,#183426,#183427,#183428,#183429,
#183430,#183431,#183432,#183433,#183434,#183435,#183436,#183437,#183438,
#183439,#183440,#183441,#183442,#183443,#183444,#183445,#183446,#183447,
#183448,#183449,#183450,#183451,#183452,#183453,#183454,#183455,#183456,
#183457,#183458,#183459,#183460,#183461,#183462,#183463,#183464,#183465,
#183466,#183467,#183468,#183469,#183470,#183471,#183472,#183473,#183474,
#183475,#183476,#183477,#183478,#183479,#183480,#183481,#183482,#183483,
#183484,#183485,#183486,#183487,#183488,#183489,#183490,#183491,#183492,
#183493,#183494,#183495,#183496,#183497,#183498,#183499,#183500,#183501,
#183502,#183503,#183504,#183505,#183506,#183507,#183508,#183509,#183510,
#183511,#183512,#183513,#183514,#183515,#183516,#183517,#183518,#183519,
#183520,#183521,#183522,#183523,#183524,#183525,#183526,#183527,#183528,
#183529,#183530,#183531,#183532,#183533,#183534,#183535,#183536,#183537,
#183538,#183539,#183540,#183541,#183542,#183543,#183544,#183545,#183546,
#183547,#183548,#183549,#183550,#183551,#183552,#183553,#183554,#183555,
#183556,#183557,#183558,#183559,#183560,#183561,#183562,#183563,#183564,
#183565,#183566,#183567,#183568,#183569,#183570,#183571,#183572,#183573,
#183574,#183575,#183576,#183577,#183578,#183579,#183580,#183581,#183582,
#183583,#183584,#183585,#183586,#183587,#183588,#183589,#183590,#183591,
#183592,#183593,#183594,#183595,#183596,#183597,#183598,#183599,#183600,
#183601,#183602,#183603,#183604,#183605,#183606,#183607,#183608,#183609,
#183610,#183611,#183612,#183613,#183614,#183615,#183616,#183617,#183618,
#183619,#183620,#183621,#183622,#183623,#183624,#183625,#183626,#183627,
#183628,#183629,#183630,#183631,#183632,#183633,#183634,#183635,#183636,
#183637,#183638,#183639,#183640,#183641,#183642,#183643,#183644,#183645,
#183646,#183647,#183648,#183649,#183650,#183651,#183652,#183653,#183654,
#183655,#183656,#183657,#183658,#183659,#183660,#183661,#183662,#183663,
#183664,#183665,#183666,#183667,#183668,#183669,#183670,#183671,#183672,
#183673,#183674,#183675,#183676,#183677,#183678,#183679,#183680,#183681,
#183682,#183683,#183684,#183685,#183686,#183687,#183688,#183689,#183690,
#183691,#183692,#183693,#183694,#183695,#183696,#183697,#183698,#183699,
#183700,#183701,#183702,#183703,#183704,#183705,#183706,#183707,#183708,
#183709,#183710,#183711,#183712,#183713,#183714,#183715,#183716,#183717,
#183718,#183719,#183720,#183721,#183722,#183723,#183724,#183725,#183726,
#183727,#183728,#183729,#183730,#183731,#183732,#183733,#183734,#183735,
#183736,#183737,#183738,#183739,#183740,#183741,#183742,#183743,#183744,
#183745,#183746,#183747,#183748,#183749,#183750,#183751,#183752,#183753,
#183754,#183755,#183756,#183757,#183758,#183759,#183760,#183761,#183762,
#183763,#183764,#183765,#183766,#183767,#183768,#183769,#183770,#183771,
#183772,#183773,#183774,#183775,#183776,#183777,#183778,#183779,#183780,
#183781,#183782,#183783,#183784,#183785,#183786,#183787,#183788,#183789,
#183790,#183791,#183792,#183793,#183794,#183795,#183796,#183797,#183798,
#183799,#183800,#183801,#183802,#183803,#183804,#183805,#183806,#183807,
#183808,#183809,#183810,#183811,#183812,#183813,#183814,#183815,#183816,
#183817,#183818,#183819,#183820,#183821,#183822,#183823,#183824,#183825,
#183826,#183827,#183828,#183829,#183830,#183831,#183832,#183833,#183834,
#183835,#183836,#183837,#183838,#183839,#183840,#183841,#183842,#183843,
#183844,#183845,#183846,#183847,#183848,#183849,#183850,#183851,#183852,
#183853,#183854,#183855,#183856,#183857,#183858,#183859,#183860,#183861,
#183862,#183863,#183864,#183865,#183866,#183867,#183868,#183869,#183870,
#183871,#183872,#183873,#183874,#183875,#183876,#183877,#183878,#183879,
#183880,#183881,#183882,#183883,#183884,#183885,#183886,#183887,#183888,
#183889,#183890,#183891,#183892,#183893,#183894,#183895,#183896,#183897,
#183898,#183899,#183900,#183901,#183902,#183903,#183904,#183905,#183906,
#183907,#183908,#183909,#183910,#183911,#183912,#183913,#183914,#183915,
#183916,#183917,#183918,#183919,#183920,#183921,#183922,#183923,#183924,
#183925,#183926,#183927,#183928,#183929,#183930,#183931,#183932,#183933,
#183934,#183935,#183936,#183937,#183938,#183939,#183940,#183941,#183942,
#183943,#183944,#183945,#183946,#183947,#183948,#183949,#183950,#183951,
#183952),(#183953,#183954,#183955,#183956,#183957,#183958,#183959,#183960,
#183961,#183962,#183963,#183964,#183965,#183966,#183967,#183968,#183969,
#183970,#183971,#183972,#183973,#183974,#183975,#183976,#183977,#183978,
#183979,#183980,#183981,#183982,#183983,#183984,#183985,#183986,#183987,
#183988,#183989,#183990,#183991,#183992,#183993,#183994,#183995,#183996,
#183997,#183998,#183999,#184000,#184001,#184002,#184003,#184004,#184005,
#184006,#184007,#184008,#184009,#184010,#184011,#184012,#184013,#184014,
#184015,#184016,#184017,#184018,#184019,#184020,#184021,#184022,#184023,
#184024,#184025,#184026,#184027,#184028,#184029,#184030,#184031,#184032,
#184033,#184034,#184035,#184036,#184037,#184038,#184039,#184040,#184041,
#184042,#184043,#184044,#184045,#184046,#184047,#184048,#184049,#184050,
#184051,#184052,#184053,#184054,#184055,#184056,#184057,#184058,#184059,
#184060,#184061,#184062,#184063,#184064,#184065,#184066,#184067,#184068,
#184069,#184070,#184071,#184072,#184073,#184074,#184075,#184076,#184077,
#184078,#184079,#184080,#184081,#184082,#184083,#184084,#184085,#184086,
#184087,#184088,#184089,#184090,#184091,#184092,#184093,#184094,#184095,
#184096,#184097,#184098,#184099,#184100,#184101,#184102,#184103,#184104,
#184105,#184106,#184107,#184108,#184109,#184110,#184111,#184112,#184113,
#184114,#184115,#184116,#184117,#184118,#184119,#184120,#184121,#184122,
#184123,#184124,#184125,#184126,#184127,#184128,#184129,#184130,#184131,
#184132,#184133,#184134,#184135,#184136,#184137,#184138,#184139,#184140,
#184141,#184142,#184143,#184144,#184145,#184146,#184147,#184148,#184149,
#184150,#184151,#184152,#184153,#184154,#184155,#184156,#184157,#184158,
#184159,#184160,#184161,#184162,#184163,#184164,#184165,#184166,#184167,
#184168,#184169,#184170,#184171,#184172,#184173,#184174,#184175,#184176,
#184177,#184178,#184179,#184180,#184181,#184182,#184183,#184184,#184185,
#184186,#184187,#184188,#184189,#184190,#184191,#184192,#184193,#184194,
#184195,#184196,#184197,#184198,#184199,#184200,#184201,#184202,#184203,
#184204,#184205,#184206,#184207,#184208,#184209,#184210,#184211,#184212,
#184213,#184214,#184215,#184216,#184217,#184218,#184219,#184220,#184221,
#184222,#184223,#184224,#184225,#184226,#184227,#184228,#184229,#184230,
#184231,#184232,#184233,#184234,#184235,#184236,#184237,#184238,#184239,
#184240,#184241,#184242,#184243,#184244,#184245,#184246,#184247,#184248,
#184249,#184250,#184251,#184252,#184253,#184254,#184255,#184256,#184257,
#184258,#184259,#184260,#184261,#184262,#184263,#184264,#184265,#184266,
#184267,#184268,#184269,#184270,#184271,#184272,#184273,#184274,#184275,
#184276,#184277,#184278,#184279,#184280,#184281,#184282,#184283,#184284,
#184285,#184286,#184287,#184288,#184289,#184290,#184291,#184292,#184293,
#184294,#184295,#184296,#184297,#184298,#184299,#184300,#184301,#184302,
#184303,#184304,#184305,#184306,#184307,#184308,#184309,#184310,#184311,
#184312,#184313,#184314,#184315,#184316,#184317,#184318,#184319,#184320,
#184321,#184322,#184323,#184324,#184325,#184326,#184327,#184328,#184329,
#184330,#184331,#184332,#184333,#184334,#184335,#184336,#184337,#184338,
#184339,#184340,#184341,#184342,#184343,#184344,#184345,#184346,#184347,
#184348,#184349,#184350,#184351,#184352,#184353,#184354,#184355,#184356,
#184357,#184358,#184359,#184360,#184361,#184362,#184363,#184364,#184365,
#184366,#184367,#184368,#184369,#184370,#184371,#184372,#184373,#184374,
#184375,#184376,#184377,#184378,#184379,#184380,#184381,#184382,#184383,
#184384,#184385,#184386,#184387,#184388,#184389,#184390,#184391,#184392,
#184393,#184394,#184395,#184396,#184397,#184398,#184399,#184400,#184401,
#184402,#184403,#184404,#184405,#184406,#184407,#184408,#184409,#184410,
#184411,#184412,#184413,#184414,#184415,#184416,#184417,#184418,#184419,
#184420,#184421,#184422,#184423,#184424,#184425,#184426,#184427,#184428,
#184429,#184430,#184431,#184432,#184433,#184434,#184435,#184436,#184437,
#184438,#184439,#184440,#184441,#184442,#184443,#184444,#184445,#184446,
#184447,#184448,#184449,#184450,#184451,#184452,#184453,#184454,#184455,
#184456,#184457,#184458,#184459,#184460,#184461,#184462,#184463,#184464,
#184465,#184466,#184467,#184468,#184469,#184470,#184471,#184472,#184473,
#184474,#184475,#184476,#184477,#184478,#184479,#184480,#184481,#184482,
#184483,#184484,#184485,#184486,#184487,#184488,#184489,#184490),(#184491,
#184492,#184493,#184494,#184495,#184496,#184497,#184498,#184499,#184500,
#184501,#184502,#184503,#184504,#184505,#184506,#184507,#184508,#184509,
#184510,#184511,#184512,#184513,#184514,#184515,#184516,#184517,#184518,
#184519,#184520,#184521,#184522,#184523,#184524,#184525,#184526,#184527,
#184528,#184529,#184530,#184531,#184532,#184533,#184534,#184535,#184536,
#184537,#184538,#184539,#184540,#184541,#184542,#184543,#184544,#184545,
#184546,#184547,#184548,#184549,#184550,#184551,#184552,#184553,#184554,
#184555,#184556,#184557,#184558,#184559,#184560,#184561,#184562,#184563,
#184564,#184565,#184566,#184567,#184568,#184569,#184570,#184571,#184572,
#184573,#184574,#184575,#184576,#184577,#184578,#184579,#184580,#184581,
#184582,#184583,#184584,#184585,#184586,#184587,#184588,#184589,#184590,
#184591,#184592,#184593,#184594,#184595,#184596,#184597,#184598,#184599,
#184600,#184601,#184602,#184603,#184604,#184605,#184606,#184607,#184608,
#184609,#184610,#184611,#184612,#184613,#184614,#184615,#184616,#184617,
#184618,#184619,#184620,#184621,#184622,#184623,#184624,#184625,#184626,
#184627,#184628,#184629,#184630,#184631,#184632,#184633,#184634,#184635,
#184636,#184637,#184638,#184639,#184640,#184641,#184642,#184643,#184644,
#184645,#184646,#184647,#184648,#184649,#184650,#184651,#184652,#184653,
#184654,#184655,#184656,#184657,#184658,#184659,#184660,#184661,#184662,
#184663,#184664,#184665,#184666,#184667,#184668,#184669,#184670,#184671,
#184672,#184673,#184674,#184675,#184676,#184677,#184678,#184679,#184680,
#184681,#184682,#184683,#184684,#184685,#184686,#184687,#184688,#184689,
#184690,#184691,#184692,#184693,#184694,#184695,#184696,#184697,#184698,
#184699,#184700,#184701,#184702,#184703,#184704,#184705,#184706,#184707,
#184708,#184709,#184710,#184711,#184712,#184713,#184714,#184715,#184716,
#184717,#184718,#184719,#184720,#184721,#184722,#184723,#184724,#184725,
#184726,#184727,#184728,#184729,#184730,#184731,#184732,#184733,#184734,
#184735,#184736,#184737,#184738,#184739,#184740,#184741,#184742,#184743,
#184744,#184745,#184746,#184747,#184748,#184749,#184750,#184751,#184752,
#184753,#184754,#184755,#184756,#184757,#184758,#184759,#184760,#184761,
#184762,#184763,#184764,#184765,#184766,#184767,#184768,#184769,#184770,
#184771,#184772,#184773,#184774,#184775,#184776,#184777,#184778,#184779,
#184780,#184781,#184782,#184783,#184784,#184785,#184786,#184787,#184788,
#184789,#184790,#184791,#184792,#184793,#184794,#184795,#184796,#184797,
#184798,#184799,#184800,#184801,#184802,#184803,#184804,#184805,#184806,
#184807,#184808,#184809,#184810,#184811,#184812,#184813,#184814,#184815,
#184816,#184817,#184818,#184819,#184820,#184821,#184822,#184823,#184824,
#184825,#184826,#184827,#184828,#184829,#184830,#184831,#184832,#184833,
#184834,#184835,#184836,#184837,#184838,#184839,#184840,#184841,#184842,
#184843,#184844,#184845,#184846,#184847,#184848,#184849,#184850,#184851,
#184852,#184853,#184854,#184855,#184856,#184857,#184858,#184859,#184860,
#184861,#184862,#184863,#184864,#184865,#184866,#184867,#184868,#184869,
#184870,#184871,#184872,#184873,#184874,#184875,#184876,#184877,#184878,
#184879,#184880,#184881,#184882,#184883,#184884,#184885,#184886,#184887,
#184888,#184889,#184890,#184891,#184892,#184893,#184894,#184895,#184896,
#184897,#184898,#184899,#184900,#184901,#184902,#184903,#184904,#184905,
#184906,#184907,#184908,#184909,#184910,#184911,#184912,#184913,#184914,
#184915,#184916,#184917,#184918,#184919,#184920,#184921,#184922,#184923,
#184924,#184925,#184926,#184927,#184928,#184929,#184930,#184931,#184932,
#184933,#184934,#184935,#184936,#184937,#184938,#184939,#184940,#184941,
#184942,#184943,#184944,#184945,#184946,#184947,#184948,#184949,#184950,
#184951,#184952,#184953,#184954,#184955,#184956,#184957,#184958,#184959,
#184960,#184961,#184962,#184963,#184964,#184965,#184966,#184967,#184968,
#184969,#184970,#184971,#184972,#184973,#184974,#184975,#184976,#184977,
#184978,#184979,#184980,#184981,#184982,#184983,#184984,#184985,#184986,
#184987,#184988,#184989,#184990,#184991,#184992,#184993,#184994,#184995,
#184996,#184997,#184998,#184999,#185000,#185001,#185002,#185003,#185004,
#185005,#185006,#185007,#185008,#185009,#185010,#185011,#185012,#185013,
#185014,#185015,#185016,#185017,#185018,#185019,#185020,#185021,#185022,
#185023,#185024,#185025,#185026,#185027,#185028)),.UNSPECIFIED.,.F.,.F.,
 .F.,(4,4),(4,1,1,1,1,1,1,1,1,1,1,1,1,1,1,1,1,1,1,1,1,1,1,1,1,1,1,1,1,1,
1,1,1,1,1,1,1,1,1,1,1,1,1,1,1,1,1,1,1,1,1,1,1,1,1,1,1,1,1,1,1,1,1,1,1,1,
1,1,1,1,1,1,1,1,1,1,1,1,1,1,1,1,1,1,1,1,1,1,1,1,1,1,1,1,1,1,1,1,1,1,1,1,
1,1,1,1,1,1,1,1,1,1,1,1,1,1,1,1,1,1,1,1,1,1,1,1,1,1,1,1,1,1,1,1,1,1,1,1,
1,1,1,1,1,1,1,1,1,1,1,1,1,1,1,1,1,1,1,1,1,1,1,1,1,1,1,1,1,1,1,1,1,1,1,1,
1,1,1,1,1,1,1,1,1,1,1,1,1,1,1,1,1,1,1,1,1,1,1,1,1,1,1,1,1,1,1,1,1,1,1,1,
1,1,1,1,1,1,1,1,1,1,1,1,1,1,1,1,1,1,1,1,1,1,1,1,1,1,1,1,1,1,1,1,1,1,1,1,
1,1,1,1,1,1,1,1,1,1,1,1,1,1,1,1,1,1,1,1,1,1,1,1,1,1,1,1,1,1,1,1,1,1,1,1,
1,1,1,1,1,1,1,1,1,1,1,1,1,1,1,1,1,1,1,1,1,1,1,1,1,1,1,1,1,1,1,1,1,1,1,1,
1,1,1,1,1,1,1,1,1,1,1,1,1,1,1,1,1,1,1,1,1,1,1,1,1,1,1,1,1,1,1,1,1,1,1,1,
1,1,1,1,1,1,1,1,1,1,1,1,1,1,1,1,1,1,1,1,1,1,1,1,1,1,1,1,1,1,1,1,1,1,1,1,
1,1,1,1,1,1,1,1,1,1,1,1,1,1,1,1,1,1,1,1,1,1,1,1,1,1,1,1,1,1,1,1,1,1,1,1,
1,1,1,1,1,1,1,1,1,1,1,1,1,1,1,1,1,1,1,1,1,1,1,1,1,1,1,1,1,1,1,1,1,1,1,1,
1,1,1,1,1,1,1,1,1,1,1,1,1,1,1,1,1,1,1,1,1,1,1,1,1,1,1,1,1,1,1,1,1,1,1,1,
1,1,1,1,1,1,1,1,1,1,1,1,1,1,1,1,1,1,1,1,1,1,1,1,1,1,1,1,1,1,1,1,1,1,1,1,
1,4),(-0.00284646367232349,0.129536473500696),(14.3987987524829,14.897322120121,
15.3957906634286,15.8942592067361,16.3927277500437,16.8911962933512,17.3896648366588,
18.3866019232739,19.383539009889,19.8820075531966,20.3804760965041,20.8789446398117,
21.3774131831193,21.8758817264268,22.3743502697344,22.8728188130419,23.3712873563495,
24.3682244429646,24.8666929862722,25.3651615295797,26.3620986161948,26.8605671595024,
27.35903570281,27.8575042461175,28.3559727894251,28.8544413327326,29.3529098760402,
29.8513784193477,30.3498469626553,31.3467840492704,31.845252592578,32.3437211358855,
33.3406582225007,33.8391267658082,34.3375953091158,34.8360638524233,35.3345323957309,
35.8330009390384,36.331469482346,36.8299380256536,37.3284065689611,38.3253436555762,
38.8238121988838,39.3222807421914,40.3192178288065,40.817686372114,41.3161549154216,
41.8146234587291,42.3130920020367,42.8115605453443,43.3100290886518,43.8084976319594,
44.3069661752669,45.303903261882,45.8023718051896,46.3008403484972,47.2977774351123,
47.7962459784198,48.2947145217274,48.793183065035,49.2916516083425,49.7901201516501,
50.2885886949576,50.7870572382652,51.2855257815727,52.2824628681879,52.7809314114954,
53.279399954803,54.2763370414181,54.7748055847256,55.2732741280332,55.7717426713408,
56.2702112146483,56.7686797579559,57.2671483012634,57.765616844571,58.2640853878786,
59.2610224744937,59.7594910178012,60.2579595611088,61.2548966477239,61.7533651910315,
62.251833734339,62.7503022776466,63.2487708209541,63.7472393642617,64.2457079075693,
64.7441764508768,65.2426449941844,66.2395820807995,66.738050624107,67.2365191674146,
68.2334562540297,68.7319247973373,69.2303933406448,69.7288618839524,70.22733042726,
70.7257989705675,71.2242675138751,71.7227360571826,72.2212046004902,73.2181416871053,
73.7166102304129,74.2150787737204,75.2120158603355,75.7104844036431,76.2089529469506,
76.7074214902582,77.2058900335658,77.7043585768733,78.2028271201809,78.7012956634885,
79.199764206796,80.1967012934111,80.6951698367187,81.1936383800262,82.1905754666413,
82.6890440099489,83.1875125532565,83.685981096564,84.1844496398716,84.6829181831791,
85.1813867264867,85.6798552697942,86.1783238131018,87.1752608997169,87.6737294430245,
88.1721979863321,89.1691350729472,89.6676036162547,90.1660721595623,90.6645407028698,
91.1630092461774,91.661477789485,92.1599463327925,92.6584148761001,93.1568834194076,
94.1538205060227,94.6522890493303,95.1507575926379,96.147694679253,96.6461632225605,
97.1446317658681,97.6431003091757,98.1415688524832,98.6400373957908,99.1385059390983,
99.6369744824059,100.135443025713,101.132380112329,101.630848655636,102.129317198944,
103.126254285559,103.624722828866,104.123191372174,104.621659915481,105.120128458789,
105.618597002097,106.117065545404,106.615534088712,107.114002632019,108.110939718634,
108.609408261942,109.107876805249,110.104813891865,110.603282435172,111.10175097848,
111.600219521787,112.098688065095,112.597156608402,113.09562515171,113.594093695018,
114.092562238325,115.08949932494,115.587967868248,116.086436411555,117.08337349817,
117.581842041478,118.080310584786,118.578779128093,119.077247671401,119.575716214708,
120.074184758016,120.572653301323,121.071121844631,122.068058931246,122.566527474554,
123.064996017861,124.061933104476,124.560401647784,125.058870191091,125.557338734399,
126.055807277706,126.554275821014,127.052744364322,127.551212907629,128.049681450937,
129.046618537552,129.545087080859,130.043555624167,131.040492710782,131.53896125409,
132.037429797397,132.535898340705,133.034366884012,133.53283542732,134.031303970627,
134.529772513935,135.028241057242,136.025178143858,136.523646687165,137.022115230473,
138.019052317088,138.517520860395,139.015989403703,139.514457947011,140.012926490318,
140.511395033626,141.009863576933,141.508332120241,142.006800663548,143.003737750163,
143.502206293471,144.000674836779,144.997611923394,145.496080466701,145.994549010009,
146.493017553316,146.991486096624,147.489954639931,147.988423183239,148.486891726547,
148.985360269854,149.982297356469,150.480765899777,150.979234443084,151.976171529699,
152.474640073007,152.973108616315,153.471577159622,153.97004570293,154.468514246237,
154.966982789545,155.465451332852,155.96391987616,156.960856962775,157.459325506083,
157.95779404939,158.954731136005,159.453199679313,159.95166822262,160.450136765928,
160.948605309236,161.447073852543,161.945542395851,162.444010939158,162.942479482466,
163.939416569081,164.437885112388,164.936353655696,165.933290742311,166.431759285619,
166.930227828926,167.428696372234,167.927164915541,168.425633458849,168.924102002156,
169.921039088772,170.917976175387,171.914913262002,172.413381805309,172.911850348617,
173.410318891924,173.908787435232,174.905724521847,175.902661608462,176.899598695077,
177.398067238385,177.896535781693,178.893472868308,179.391941411615,179.890409954923,
180.38887849823,180.887347041538,181.385815584845,181.884284128153,182.382752671461,
182.881221214768,183.878158301383,184.376626844691,184.875095387998,185.872032474613,
186.370501017921,186.868969561229,187.367438104536,187.865906647844,188.364375191151,
188.862843734459,189.361312277766,189.859780821074,190.856717907689,191.355186450997,
191.853654994304,192.850592080919,193.349060624227,193.847529167534,194.345997710842,
194.844466254149,195.342934797457,195.841403340765,196.339871884072,196.83834042738,
197.835277513995,198.333746057302,198.83221460061,199.829151687225,200.327620230533,
200.82608877384,201.324557317148,201.823025860455,202.321494403763,202.81996294707,
203.318431490378,203.816900033686,204.813837120301,205.312305663608,205.810774206916,
206.807711293531,207.306179836838,207.804648380146,208.303116923454,208.801585466761,
209.300054010069,209.798522553376,210.296991096684,210.795459639991,211.792396726606,
212.290865269914,212.789333813222,213.786270899837,214.284739443144,214.783207986452,
215.281676529759,215.780145073067,216.278613616374,216.777082159682,217.27555070299,
217.774019246297,218.770956332912,219.26942487622,219.767893419527,220.764830506142,
221.26329904945,221.761767592758,222.260236136065,222.758704679373,223.25717322268,
223.755641765988,224.254110309295,224.752578852603,225.749515939218,226.247984482526,
226.746453025833,227.743390112448,228.241858655756,228.740327199063,229.238795742371,
229.737264285679,230.235732828986,230.734201372294,231.232669915601,231.731138458909,
232.728075545524,233.226544088831,233.725012632139,234.721949718754,235.220418262062,
235.718886805369,236.217355348677,236.715823891984,237.214292435292,237.712760978599,
238.211229521907,238.709698065215,239.70663515183,240.205103695137,240.703572238445,
241.70050932506,242.198977868367,242.697446411675,243.195914954983,243.69438349829,
244.192852041598,244.691320584905,245.189789128213,245.68825767152,246.685194758136,
247.183663301443,247.682131844751,248.679068931366,249.177537474673,249.676006017981,
250.174474561288,250.672943104596,251.171411647904,251.669880191211,252.168348734519,
252.666817277826,253.663754364441,254.162222907749,254.660691451056,255.657628537672,
256.156097080979,256.654565624287,257.153034167594,257.651502710902,258.149971254209,
258.648439797517,259.146908340824,259.645376884132,260.642313970747,261.140782514055,
261.639251057362,262.636188143977,263.134656687285,263.633125230592,264.1315937739,
264.630062317208,265.128530860515,265.626999403823,266.12546794713,266.623936490438,
267.620873577053,268.11934212036,268.617810663668,269.614747750283,270.113216293591,
270.611684836898,271.110153380206,271.608621923513,272.107090466821,272.605559010129,
273.104027553436,273.602496096744,274.599433183359,275.097901726666,275.596370269974,
276.593307356589,277.091775899897,277.590244443204,278.088712986512,278.587181529819,
279.085650073127,279.584118616434,280.082587159742,280.581055703049,281.577992789665,
282.076461332972,282.57492987628,283.571866962895,284.070335506202,284.56880404951,
285.067272592818,285.565741136125,286.064209679433,286.56267822274,287.061146766048,
287.559615309355,288.55655239597,289.055020939278,289.553489482586,290.550426569201,
291.048895112508,291.547363655816,292.045832199123,292.544300742431,293.042769285738,
293.541237829046,294.039706372354,294.538174915661,295.535112002276,296.033580545584,
296.532049088891,297.528986175506,298.027454718814,298.525923262122,299.024391805429,
299.522860348737,300.021328892044,300.519797435352,301.018265978659,301.516734521967,
302.513671608582,303.01214015189,303.510608695197,304.507545781812,305.00601432512,
305.504482868427,306.002951411735,306.501419955042,306.99988849835,307.498357041658,
307.996825584965,308.495294128273,309.492231214888,309.990699758195,310.489168301503,
311.486105388118,311.984573931426,312.483042474733,312.981511018041,313.479979561348,
313.978448104656,314.476916647963,314.975385191271,315.473853734579,316.470790821194,
316.969259364501,317.467727907809,318.464664994424,318.963133537731,319.461602081039,
319.960070624347,320.458539167654,320.957007710962,321.455476254269,321.953944797577,
322.452413340884,323.449350427499,324.446287514115,324.944756057422,325.44322460073,
325.941693144037,326.440161687345,326.938630230652,327.43724547751),
 .UNSPECIFIED.);
#344=PLANE('',#17508);
#345=PLANE('',#17513);
#346=PLANE('',#17514);
#347=PLANE('',#17515);
#348=PLANE('',#17516);
#349=PLANE('',#17518);
#350=PLANE('',#17519);
#351=PLANE('',#17524);
#769=FACE_OUTER_BOUND('',#1450,.T.);
#770=FACE_OUTER_BOUND('',#1451,.T.);
#771=FACE_OUTER_BOUND('',#1452,.T.);
#772=FACE_OUTER_BOUND('',#1453,.T.);
#773=FACE_OUTER_BOUND('',#1454,.T.);
#774=FACE_OUTER_BOUND('',#1455,.T.);
#775=FACE_OUTER_BOUND('',#1456,.T.);
#776=FACE_OUTER_BOUND('',#1457,.T.);
#777=FACE_OUTER_BOUND('',#1458,.T.);
#778=FACE_OUTER_BOUND('',#1459,.T.);
#779=FACE_OUTER_BOUND('',#1460,.T.);
#780=FACE_OUTER_BOUND('',#1461,.T.);
#781=FACE_OUTER_BOUND('',#1462,.T.);
#782=FACE_OUTER_BOUND('',#1463,.T.);
#783=FACE_OUTER_BOUND('',#1464,.T.);
#784=FACE_OUTER_BOUND('',#1465,.T.);
#785=FACE_OUTER_BOUND('',#1466,.T.);
#786=FACE_OUTER_BOUND('',#1467,.T.);
#787=FACE_OUTER_BOUND('',#1468,.T.);
#788=FACE_OUTER_BOUND('',#1469,.T.);
#789=FACE_OUTER_BOUND('',#1470,.T.);
#790=FACE_OUTER_BOUND('',#1471,.T.);
#791=FACE_OUTER_BOUND('',#1472,.T.);
#792=FACE_OUTER_BOUND('',#1473,.T.);
#793=FACE_OUTER_BOUND('',#1474,.T.);
#794=FACE_OUTER_BOUND('',#1475,.T.);
#795=FACE_OUTER_BOUND('',#1476,.T.);
#796=FACE_OUTER_BOUND('',#1477,.T.);
#797=FACE_OUTER_BOUND('',#1478,.T.);
#798=FACE_OUTER_BOUND('',#1479,.T.);
#799=FACE_OUTER_BOUND('',#1480,.T.);
#800=FACE_OUTER_BOUND('',#1481,.T.);
#801=FACE_OUTER_BOUND('',#1482,.T.);
#802=FACE_OUTER_BOUND('',#1483,.T.);
#803=FACE_OUTER_BOUND('',#1484,.T.);
#804=FACE_OUTER_BOUND('',#1485,.T.);
#805=FACE_OUTER_BOUND('',#1486,.T.);
#806=FACE_OUTER_BOUND('',#1487,.T.);
#807=FACE_OUTER_BOUND('',#1488,.T.);
#808=FACE_OUTER_BOUND('',#1489,.T.);
#809=FACE_OUTER_BOUND('',#1490,.T.);
#810=FACE_OUTER_BOUND('',#1491,.T.);
#811=FACE_OUTER_BOUND('',#1492,.T.);
#812=FACE_OUTER_BOUND('',#1493,.T.);
#813=FACE_OUTER_BOUND('',#1494,.T.);
#814=FACE_OUTER_BOUND('',#1495,.T.);
#815=FACE_OUTER_BOUND('',#1496,.T.);
#816=FACE_OUTER_BOUND('',#1497,.T.);
#817=FACE_OUTER_BOUND('',#1498,.T.);
#818=FACE_OUTER_BOUND('',#1499,.T.);
#819=FACE_OUTER_BOUND('',#1500,.T.);
#820=FACE_OUTER_BOUND('',#1501,.T.);
#821=FACE_OUTER_BOUND('',#1503,.T.);
#822=FACE_OUTER_BOUND('',#1504,.T.);
#823=FACE_OUTER_BOUND('',#1505,.T.);
#824=FACE_OUTER_BOUND('',#1506,.T.);
#825=FACE_OUTER_BOUND('',#1507,.T.);
#826=FACE_OUTER_BOUND('',#1509,.T.);
#827=FACE_OUTER_BOUND('',#1510,.T.);
#828=FACE_OUTER_BOUND('',#1511,.T.);
#829=FACE_OUTER_BOUND('',#1512,.T.);
#830=FACE_OUTER_BOUND('',#1514,.T.);
#831=FACE_OUTER_BOUND('',#1515,.T.);
#832=FACE_OUTER_BOUND('',#1516,.T.);
#1450=EDGE_LOOP('',(#12939,#12940,#12941,#12942,#12943,#12944,#12945,#12946));
#1451=EDGE_LOOP('',(#12947,#12948,#12949,#12950,#12951,#12952));
#1452=EDGE_LOOP('',(#12953,#12954,#12955,#12956,#12957,#12958));
#1453=EDGE_LOOP('',(#12959,#12960,#12961,#12962,#12963,#12964));
#1454=EDGE_LOOP('',(#12965,#12966,#12967,#12968,#12969,#12970));
#1455=EDGE_LOOP('',(#12971,#12972,#12973,#12974,#12975,#12976));
#1456=EDGE_LOOP('',(#12977,#12978,#12979,#12980,#12981,#12982));
#1457=EDGE_LOOP('',(#12983,#12984,#12985,#12986,#12987,#12988));
#1458=EDGE_LOOP('',(#12989,#12990,#12991,#12992,#12993,#12994));
#1459=EDGE_LOOP('',(#12995,#12996,#12997,#12998,#12999,#13000));
#1460=EDGE_LOOP('',(#13001,#13002,#13003,#13004,#13005,#13006));
#1461=EDGE_LOOP('',(#13007,#13008,#13009,#13010,#13011,#13012));
#1462=EDGE_LOOP('',(#13013,#13014,#13015,#13016,#13017,#13018));
#1463=EDGE_LOOP('',(#13019,#13020,#13021,#13022,#13023,#13024));
#1464=EDGE_LOOP('',(#13025,#13026,#13027,#13028,#13029,#13030));
#1465=EDGE_LOOP('',(#13031,#13032,#13033,#13034,#13035,#13036));
#1466=EDGE_LOOP('',(#13037,#13038,#13039,#13040,#13041,#13042));
#1467=EDGE_LOOP('',(#13043,#13044,#13045,#13046,#13047,#13048));
#1468=EDGE_LOOP('',(#13049,#13050,#13051,#13052,#13053,#13054));
#1469=EDGE_LOOP('',(#13055,#13056,#13057,#13058,#13059,#13060));
#1470=EDGE_LOOP('',(#13061,#13062,#13063,#13064,#13065,#13066));
#1471=EDGE_LOOP('',(#13067,#13068,#13069,#13070,#13071,#13072));
#1472=EDGE_LOOP('',(#13073,#13074,#13075,#13076,#13077,#13078));
#1473=EDGE_LOOP('',(#13079,#13080,#13081,#13082,#13083,#13084));
#1474=EDGE_LOOP('',(#13085,#13086,#13087,#13088,#13089,#13090));
#1475=EDGE_LOOP('',(#13091,#13092,#13093,#13094,#13095,#13096));
#1476=EDGE_LOOP('',(#13097,#13098,#13099,#13100,#13101,#13102));
#1477=EDGE_LOOP('',(#13103,#13104,#13105,#13106,#13107,#13108));
#1478=EDGE_LOOP('',(#13109,#13110,#13111,#13112,#13113,#13114));
#1479=EDGE_LOOP('',(#13115,#13116,#13117,#13118,#13119,#13120));
#1480=EDGE_LOOP('',(#13121,#13122,#13123,#13124,#13125,#13126));
#1481=EDGE_LOOP('',(#13127,#13128,#13129,#13130,#13131,#13132));
#1482=EDGE_LOOP('',(#13133,#13134,#13135,#13136,#13137,#13138));
#1483=EDGE_LOOP('',(#13139,#13140,#13141,#13142,#13143,#13144));
#1484=EDGE_LOOP('',(#13145,#13146,#13147,#13148,#13149,#13150));
#1485=EDGE_LOOP('',(#13151,#13152,#13153,#13154,#13155,#13156));
#1486=EDGE_LOOP('',(#13157,#13158,#13159,#13160,#13161,#13162));
#1487=EDGE_LOOP('',(#13163,#13164,#13165,#13166,#13167,#13168));
#1488=EDGE_LOOP('',(#13169,#13170,#13171,#13172,#13173,#13174));
#1489=EDGE_LOOP('',(#13175,#13176,#13177,#13178,#13179,#13180));
#1490=EDGE_LOOP('',(#13181,#13182,#13183,#13184,#13185,#13186));
#1491=EDGE_LOOP('',(#13187,#13188,#13189,#13190,#13191,#13192));
#1492=EDGE_LOOP('',(#13193,#13194,#13195,#13196,#13197,#13198));
#1493=EDGE_LOOP('',(#13199,#13200,#13201,#13202,#13203,#13204));
#1494=EDGE_LOOP('',(#13205,#13206,#13207,#13208,#13209,#13210));
#1495=EDGE_LOOP('',(#13211,#13212,#13213,#13214,#13215,#13216));
#1496=EDGE_LOOP('',(#13217,#13218,#13219,#13220,#13221,#13222));
#1497=EDGE_LOOP('',(#13223,#13224,#13225,#13226,#13227,#13228));
#1498=EDGE_LOOP('',(#13229,#13230,#13231,#13232,#13233,#13234));
#1499=EDGE_LOOP('',(#13235,#13236,#13237,#13238,#13239,#13240));
#1500=EDGE_LOOP('',(#13241,#13242,#13243,#13244,#13245,#13246,#13247,#13248,
#13249,#13250,#13251,#13252,#13253,#13254,#13255,#13256,#13257,#13258,#13259,
#13260,#13261,#13262,#13263,#13264,#13265,#13266,#13267,#13268,#13269,#13270,
#13271,#13272,#13273,#13274,#13275,#13276,#13277,#13278,#13279,#13280,#13281,
#13282,#13283,#13284,#13285,#13286,#13287,#13288,#13289,#13290,#13291,#13292,
#13293,#13294,#13295,#13296,#13297,#13298,#13299,#13300,#13301,#13302,#13303,
#13304,#13305,#13306,#13307,#13308,#13309,#13310,#13311,#13312,#13313,#13314,
#13315,#13316,#13317,#13318,#13319,#13320,#13321,#13322,#13323,#13324,#13325,
#13326));
#1501=EDGE_LOOP('',(#13327));
#1502=EDGE_LOOP('',(#13328));
#1503=EDGE_LOOP('',(#13329,#13330,#13331,#13332));
#1504=EDGE_LOOP('',(#13333,#13334,#13335,#13336));
#1505=EDGE_LOOP('',(#13337,#13338,#13339,#13340));
#1506=EDGE_LOOP('',(#13341,#13342,#13343,#13344));
#1507=EDGE_LOOP('',(#13345,#13346,#13347,#13348));
#1508=EDGE_LOOP('',(#13349));
#1509=EDGE_LOOP('',(#13350,#13351,#13352,#13353,#13354));
#1510=EDGE_LOOP('',(#13355,#13356,#13357,#13358,#13359,#13360,#13361,#13362,
#13363,#13364,#13365,#13366,#13367,#13368,#13369,#13370,#13371,#13372,#13373,
#13374,#13375,#13376,#13377,#13378,#13379,#13380,#13381,#13382,#13383,#13384,
#13385,#13386,#13387,#13388,#13389,#13390,#13391,#13392,#13393,#13394,#13395,
#13396,#13397,#13398,#13399,#13400,#13401,#13402,#13403,#13404,#13405,#13406,
#13407,#13408,#13409,#13410,#13411,#13412,#13413,#13414,#13415,#13416,#13417,
#13418,#13419,#13420,#13421,#13422,#13423,#13424,#13425,#13426,#13427,#13428,
#13429,#13430,#13431,#13432,#13433,#13434,#13435,#13436,#13437,#13438,#13439,
#13440,#13441,#13442,#13443,#13444,#13445,#13446,#13447,#13448,#13449,#13450,
#13451,#13452,#13453,#13454,#13455,#13456,#13457,#13458,#13459,#13460,#13461,
#13462,#13463,#13464,#13465,#13466,#13467,#13468,#13469,#13470,#13471,#13472,
#13473,#13474,#13475,#13476,#13477,#13478,#13479,#13480,#13481,#13482,#13483,
#13484,#13485,#13486,#13487,#13488,#13489,#13490,#13491,#13492,#13493,#13494,
#13495,#13496,#13497));
#1511=EDGE_LOOP('',(#13498,#13499,#13500,#13501,#13502,#13503,#13504,#13505,
#13506,#13507,#13508,#13509,#13510,#13511,#13512,#13513,#13514,#13515,#13516,
#13517,#13518,#13519,#13520,#13521,#13522,#13523,#13524,#13525,#13526,#13527,
#13528,#13529,#13530,#13531,#13532,#13533,#13534,#13535,#13536,#13537,#13538,
#13539,#13540,#13541,#13542,#13543,#13544,#13545,#13546,#13547,#13548,#13549,
#13550,#13551,#13552,#13553,#13554,#13555,#13556,#13557,#13558,#13559,#13560,
#13561,#13562,#13563,#13564,#13565,#13566,#13567,#13568,#13569,#13570,#13571,
#13572,#13573,#13574,#13575,#13576,#13577,#13578,#13579,#13580,#13581,#13582,
#13583,#13584,#13585,#13586,#13587,#13588,#13589,#13590,#13591,#13592,#13593,
#13594,#13595,#13596,#13597,#13598,#13599,#13600,#13601,#13602,#13603,#13604,
#13605,#13606,#13607,#13608,#13609,#13610,#13611,#13612,#13613,#13614,#13615,
#13616,#13617,#13618,#13619,#13620,#13621,#13622,#13623,#13624,#13625,#13626,
#13627,#13628,#13629,#13630,#13631,#13632,#13633,#13634,#13635,#13636,#13637,
#13638,#13639,#13640));
#1512=EDGE_LOOP('',(#13641));
#1513=EDGE_LOOP('',(#13642));
#1514=EDGE_LOOP('',(#13643,#13644,#13645,#13646));
#1515=EDGE_LOOP('',(#13647,#13648,#13649,#13650));
#1516=EDGE_LOOP('',(#13651,#13652,#13653,#13654));
#1517=EDGE_LOOP('',(#13655,#13656,#13657,#13658));
#1883=CIRCLE('',#17452,7.01125);
#1884=CIRCLE('',#17453,7.01125);
#1885=CIRCLE('',#17454,7.01125);
#1886=CIRCLE('',#17503,7.01125);
#1887=CIRCLE('',#17506,8.12525);
#1888=CIRCLE('',#17507,8.12524999999999);
#1889=CIRCLE('',#17509,7.);
#1890=CIRCLE('',#17510,4.);
#1891=CIRCLE('',#17512,10.);
#1892=CIRCLE('',#17517,20.);
#1893=CIRCLE('',#17520,4.);
#1894=CIRCLE('',#17523,20.);
#2981=B_SPLINE_CURVE_WITH_KNOTS('',3,(#136545,#136546,#136547,#136548,#136549,
#136550,#136551,#136552,#136553,#136554,#136555,#136556,#136557,#136558,
#136559,#136560,#136561,#136562,#136563,#136564,#136565,#136566,#136567,
#136568,#136569,#136570,#136571,#136572,#136573,#136574,#136575,#136576,
#136577,#136578,#136579,#136580,#136581,#136582,#136583,#136584,#136585,
#136586,#136587,#136588,#136589,#136590,#136591,#136592,#136593,#136594,
#136595,#136596,#136597,#136598,#136599,#136600,#136601,#136602,#136603,
#136604,#136605,#136606,#136607,#136608,#136609,#136610,#136611,#136612,
#136613,#136614,#136615,#136616,#136617,#136618,#136619,#136620,#136621,
#136622,#136623,#136624,#136625,#136626,#136627,#136628,#136629,#136630,
#136631,#136632,#136633,#136634,#136635,#136636,#136637,#136638,#136639,
#136640,#136641,#136642,#136643,#136644,#136645,#136646,#136647,#136648,
#136649,#136650,#136651,#136652,#136653,#136654,#136655,#136656,#136657,
#136658,#136659,#136660,#136661,#136662,#136663,#136664,#136665,#136666,
#136667,#136668,#136669,#136670,#136671,#136672,#136673,#136674,#136675,
#136676,#136677,#136678,#136679,#136680,#136681,#136682,#136683),
 .UNSPECIFIED.,.F.,.F.,(4,3,3,3,3,3,3,3,3,3,3,3,3,3,3,3,3,3,3,3,3,3,3,3,
3,3,3,3,3,3,3,3,3,3,3,3,3,3,3,3,3,3,3,3,3,3,4),(309.542368439887,309.617837246006,
309.693300130921,309.768771534012,309.844299671964,309.919858116417,309.995504346128,
310.047433937301,310.124855595317,310.202216043453,310.279528349287,310.356805768718,
310.434062635597,310.511320314385,310.545902480609,310.632946223822,310.720200992735,
310.807667881397,310.895195896758,310.982729265011,311.044371023916,311.12037421906,
311.196328916559,311.272249437817,311.34816006007,311.424064195079,311.499995258205,
311.542839567224,311.626842158064,311.710897899939,311.795011601748,311.879134544641,
311.963255773904,312.041308110531,312.120017789723,312.198698595032,312.277361399118,
312.356028358848,312.434696723513,312.513392268518,312.539776653839,312.621199463373,
312.702612292933,312.786520518987,312.867924569884,312.953084883516,313.038245197147),
 .UNSPECIFIED.);
#2982=B_SPLINE_CURVE_WITH_KNOTS('',3,(#136691,#136692,#136693,#136694,#136695,
#136696,#136697,#136698,#136699,#136700,#136701,#136702,#136703,#136704,
#136705,#136706,#136707,#136708,#136709,#136710,#136711,#136712,#136713,
#136714,#136715,#136716,#136717,#136718,#136719,#136720,#136721,#136722,
#136723,#136724,#136725,#136726,#136727,#136728,#136729,#136730,#136731,
#136732,#136733,#136734,#136735,#136736,#136737,#136738,#136739,#136740,
#136741,#136742,#136743,#136744,#136745,#136746,#136747,#136748,#136749,
#136750,#136751,#136752,#136753,#136754,#136755,#136756,#136757,#136758,
#136759,#136760,#136761,#136762,#136763,#136764,#136765,#136766,#136767,
#136768,#136769,#136770,#136771,#136772,#136773,#136774,#136775,#136776,
#136777,#136778,#136779,#136780,#136781,#136782,#136783,#136784,#136785,
#136786,#136787,#136788,#136789,#136790,#136791,#136792,#136793,#136794,
#136795,#136796,#136797,#136798,#136799,#136800,#136801,#136802,#136803,
#136804,#136805,#136806,#136807,#136808,#136809,#136810,#136811,#136812,
#136813,#136814,#136815,#136816,#136817,#136818,#136819,#136820,#136821,
#136822,#136823,#136824,#136825,#136826,#136827,#136828,#136829,#136830,
#136831,#136832,#136833,#136834,#136835,#136836,#136837,#136838,#136839,
#136840,#136841,#136842,#136843,#136844,#136845,#136846,#136847,#136848,
#136849,#136850,#136851,#136852,#136853,#136854,#136855,#136856,#136857,
#136858,#136859,#136860,#136861,#136862,#136863,#136864,#136865,#136866,
#136867,#136868,#136869,#136870,#136871,#136872,#136873,#136874,#136875,
#136876,#136877,#136878,#136879,#136880,#136881,#136882,#136883,#136884,
#136885,#136886,#136887,#136888,#136889,#136890,#136891,#136892,#136893,
#136894,#136895,#136896,#136897,#136898),.UNSPECIFIED.,.F.,.F.,(4,3,3,3,
3,3,3,3,3,3,3,3,3,3,3,3,3,3,3,3,3,3,3,3,3,3,3,3,3,3,3,3,3,3,3,3,3,3,3,3,
3,3,3,3,3,3,3,3,3,3,3,3,3,3,3,3,3,3,3,3,3,3,3,3,3,3,3,3,3,4),(-311.017671895807,
-310.930926646246,-310.844202256897,-310.757594142418,-310.671098411025,
-310.584828273228,-310.545902480609,-310.468642660336,-310.391385417305,
-310.31411775789,-310.236797613467,-310.159447861164,-310.082022859537,
-310.047433937301,-309.970550488847,-309.89373679842,-309.816977853812,
-309.740258681202,-309.663564335473,-309.586862252401,-309.510152478292,
-309.433421487568,-309.35665574544,-309.279790647613,-309.202874370491,
-309.125827334062,-309.050496850686,-308.973403311115,-308.896408861735,
-308.81949842116,-308.742656966525,-308.665869522965,-308.589119125357,
-308.512388285924,-308.435663509342,-308.358931306155,-308.282142911163,
-308.205326891268,-308.128419642196,-308.053559764071,-307.976213241289,
-307.898927080985,-307.821688129199,-307.744482426365,-307.667296324788,
-307.590107731801,-307.555091220763,-307.467982168516,-307.38066246706,
-307.293133530895,-307.205545994981,-307.117958806829,-307.056622677456,
-306.980361985978,-306.904149705518,-306.82797170016,-306.75180442684,-306.675644014599,
-306.599458179872,-306.558154134148,-306.475731516247,-306.393279662411,
-306.309881144518,-306.227367701055,-306.143526645948,-306.059685590841,
-305.977675857624,-305.895686555633,-305.813720207621,-305.801967534929),
 .UNSPECIFIED.);
#2983=B_SPLINE_CURVE_WITH_KNOTS('',3,(#136904,#136905,#136906,#136907,#136908,
#136909,#136910,#136911,#136912,#136913,#136914,#136915,#136916,#136917,
#136918,#136919,#136920,#136921,#136922,#136923,#136924,#136925,#136926,
#136927,#136928,#136929,#136930,#136931,#136932,#136933,#136934,#136935,
#136936,#136937,#136938,#136939,#136940,#136941,#136942,#136943,#136944,
#136945,#136946,#136947,#136948,#136949,#136950,#136951,#136952,#136953,
#136954,#136955,#136956,#136957,#136958,#136959,#136960,#136961,#136962,
#136963,#136964,#136965,#136966,#136967,#136968,#136969,#136970,#136971,
#136972,#136973,#136974,#136975,#136976,#136977,#136978,#136979,#136980,
#136981,#136982,#136983,#136984,#136985,#136986,#136987,#136988,#136989,
#136990,#136991,#136992,#136993,#136994,#136995,#136996,#136997,#136998,
#136999,#137000,#137001,#137002,#137003,#137004,#137005,#137006,#137007,
#137008,#137009,#137010,#137011,#137012,#137013,#137014,#137015,#137016,
#137017,#137018,#137019,#137020,#137021,#137022,#137023,#137024,#137025,
#137026,#137027,#137028,#137029,#137030,#137031,#137032,#137033,#137034,
#137035,#137036,#137037,#137038,#137039,#137040,#137041,#137042,#137043,
#137044,#137045,#137046,#137047,#137048,#137049,#137050,#137051,#137052,
#137053,#137054,#137055,#137056,#137057,#137058,#137059,#137060,#137061,
#137062,#137063,#137064,#137065,#137066,#137067,#137068,#137069,#137070,
#137071,#137072,#137073,#137074,#137075,#137076,#137077,#137078,#137079,
#137080,#137081,#137082,#137083,#137084,#137085,#137086,#137087,#137088,
#137089,#137090,#137091,#137092,#137093,#137094,#137095,#137096,#137097,
#137098,#137099,#137100,#137101,#137102,#137103,#137104,#137105,#137106,
#137107,#137108,#137109,#137110,#137111,#137112,#137113,#137114,#137115,
#137116,#137117,#137118,#137119,#137120,#137121,#137122,#137123,#137124,
#137125,#137126,#137127,#137128,#137129,#137130,#137131,#137132,#137133,
#137134,#137135),.UNSPECIFIED.,.F.,.F.,(4,3,3,3,3,3,3,3,3,3,3,3,3,3,3,3,
3,3,3,3,3,3,3,3,3,3,3,3,3,3,3,3,3,3,3,3,3,3,3,3,3,3,3,3,3,3,3,3,3,3,3,3,
3,3,3,3,3,3,3,3,3,3,3,3,3,3,3,3,3,3,3,3,3,3,3,3,3,4),(303.258525738749,
303.337437675126,303.41630459851,303.497492950898,303.576309928053,303.655119327753,
303.73393166642,303.816901604217,303.895777069118,303.974680900916,304.053645652013,
304.06581141761,304.139959257083,304.214049984434,304.288098768055,304.362129722208,
304.436148605976,304.510192013303,304.564279960918,304.655011624552,304.746226212929,
304.837868512921,304.929604166686,305.021232905757,305.062748504226,305.138664739202,
305.214531642008,305.290363594904,305.366184709726,305.441998765712,305.517839199806,
305.561217047533,305.643117176767,305.725038259918,305.808700092649,305.890676262575,
305.975180926708,306.059685590841,306.142226387424,306.224750819407,306.308101648092,
306.390576093353,306.47436511375,306.558154134148,306.634340306684,306.71050467673,
306.786661344806,306.862847287711,306.939049130345,307.015310892414,307.056622677456,
307.144203357248,307.231804230285,307.319316613453,307.406720170908,307.493865126369,
307.555091220763,307.63228178972,307.709468444206,307.786664267124,307.863911006084,
307.941186435182,308.018536116409,308.053559764071,308.130473946048,308.207318862647,
308.284109489602,308.36086076461,308.43758759697,308.514322633225,308.591065641076,
308.667830114684,308.744629557554,308.821528507859,308.898478773299,308.97555968571,
309.050496850686,309.185189742936),.UNSPECIFIED.);
#2984=B_SPLINE_CURVE_WITH_KNOTS('',3,(#137136,#137137,#137138,#137139,#137140,
#137141,#137142,#137143,#137144,#137145,#137146,#137147,#137148,#137149,
#137150,#137151),.UNSPECIFIED.,.F.,.F.,(4,3,3,3,3,4),(309.18518974306,309.260920311614,
309.33654607352,309.412111555631,309.487623538129,309.542368439887),
 .UNSPECIFIED.);
#2985=B_SPLINE_CURVE_WITH_KNOTS('',3,(#137153,#137154,#137155,#137156,#137157,
#137158,#137159,#137160,#137161,#137162,#137163,#137164,#137165,#137166,
#137167,#137168),.UNSPECIFIED.,.F.,.F.,(4,3,3,3,3,4),(-305.801967534929,
-305.720030109092,-305.638119567349,-305.561217047533,-305.48132141018,
-305.44595019883),.UNSPECIFIED.);
#2986=B_SPLINE_CURVE_WITH_KNOTS('',3,(#137169,#137170,#137171,#137172,#137173,
#137174,#137175,#137176,#137177,#137178,#137179,#137180,#137181,#137182,
#137183,#137184,#137185,#137186,#137187,#137188,#137189,#137190,#137191,
#137192,#137193,#137194,#137195,#137196,#137197,#137198,#137199,#137200,
#137201,#137202,#137203,#137204,#137205,#137206,#137207,#137208,#137209,
#137210,#137211,#137212,#137213,#137214,#137215,#137216,#137217,#137218,
#137219,#137220,#137221,#137222,#137223,#137224,#137225,#137226,#137227,
#137228,#137229,#137230,#137231,#137232,#137233,#137234,#137235,#137236,
#137237,#137238,#137239,#137240,#137241,#137242,#137243,#137244,#137245,
#137246,#137247,#137248,#137249,#137250,#137251,#137252,#137253,#137254,
#137255,#137256,#137257,#137258,#137259,#137260,#137261,#137262,#137263,
#137264,#137265,#137266,#137267,#137268,#137269,#137270,#137271,#137272,
#137273,#137274,#137275,#137276,#137277,#137278,#137279,#137280,#137281,
#137282,#137283,#137284,#137285,#137286,#137287,#137288,#137289,#137290,
#137291,#137292,#137293,#137294,#137295,#137296,#137297,#137298,#137299,
#137300,#137301,#137302,#137303,#137304,#137305,#137306,#137307,#137308,
#137309,#137310,#137311,#137312,#137313,#137314,#137315,#137316,#137317,
#137318,#137319,#137320,#137321,#137322,#137323,#137324,#137325,#137326,
#137327,#137328,#137329,#137330,#137331,#137332,#137333,#137334,#137335,
#137336,#137337,#137338,#137339,#137340,#137341,#137342,#137343,#137344,
#137345,#137346,#137347,#137348,#137349,#137350,#137351,#137352,#137353,
#137354,#137355,#137356,#137357,#137358,#137359,#137360,#137361,#137362,
#137363,#137364,#137365,#137366,#137367,#137368,#137369,#137370,#137371,
#137372,#137373,#137374,#137375,#137376,#137377,#137378,#137379,#137380,
#137381,#137382,#137383,#137384,#137385,#137386,#137387,#137388,#137389,
#137390,#137391,#137392,#137393,#137394,#137395,#137396,#137397,#137398,
#137399,#137400,#137401,#137402,#137403,#137404,#137405,#137406),
 .UNSPECIFIED.,.F.,.F.,(4,3,3,3,3,3,3,3,3,3,3,3,3,3,3,3,3,3,3,3,3,3,3,3,
3,3,3,3,3,3,3,3,3,3,3,3,3,3,3,3,3,3,3,3,3,3,3,3,3,3,3,3,3,3,3,3,3,3,3,3,
3,3,3,3,3,3,3,3,3,3,3,3,3,3,3,3,3,3,3,4),(-305.445950198753,-305.370428452089,
-305.293508465123,-305.217956252189,-305.140352378208,-305.062748504226,
-304.971128629841,-304.879391811904,-304.787810304948,-304.696471890485,
-304.605715271465,-304.564279960918,-304.490236908474,-304.416214556437,
-304.342197836222,-304.268143336115,-304.194069814163,-304.119922631049,
-304.06581141761,-303.986854587823,-303.907951856808,-303.829091603746,
-303.750262240707,-303.671452204277,-303.592635952831,-303.513814364812,
-303.434976919948,-303.35611308886,-303.27717612643,-303.198200446288,-303.119134467816,
-303.068874330995,-302.989891304843,-302.911008376975,-302.832214947182,
-302.753523689414,-302.674892927008,-302.596325213187,-302.570405787688,
-302.491812168687,-302.413168932538,-302.334465713034,-302.255644268394,
-302.176755320595,-302.097744603891,-302.07193724438,-301.992866686455,
-301.913869133847,-301.834932901509,-301.756046350948,-301.677197881843,
-301.598371488275,-301.519557236236,-301.440744613705,-301.3619231109,-301.283055184286,
-301.204163620468,-301.125205184055,-301.075000157765,-301.000893610658,
-300.926844006196,-300.85283616429,-300.778845802293,-300.704867345413,
-300.630863971717,-300.576531614458,-300.485533066705,-300.394030439515,
-300.302087508411,-300.210053528992,-300.118144990757,-300.07806307115,
-300.002353717235,-299.926693034302,-299.851066514759,-299.775449141077,
-299.699837964776,-299.624198364613,-299.579594527842,-299.519174510177),
 .UNSPECIFIED.);
#2987=B_SPLINE_CURVE_WITH_KNOTS('',3,(#137412,#137413,#137414,#137415,#137416,
#137417,#137418,#137419,#137420,#137421,#137422,#137423,#137424,#137425,
#137426,#137427,#137428,#137429,#137430,#137431,#137432,#137433,#137434,
#137435,#137436,#137437,#137438,#137439,#137440,#137441,#137442,#137443,
#137444,#137445,#137446,#137447,#137448,#137449,#137450,#137451,#137452,
#137453,#137454,#137455,#137456,#137457,#137458,#137459,#137460,#137461,
#137462,#137463,#137464,#137465,#137466,#137467,#137468,#137469,#137470,
#137471,#137472,#137473,#137474,#137475,#137476,#137477,#137478,#137479,
#137480,#137481,#137482,#137483,#137484,#137485,#137486,#137487,#137488,
#137489,#137490,#137491,#137492,#137493,#137494,#137495,#137496,#137497,
#137498,#137499,#137500,#137501,#137502,#137503,#137504,#137505,#137506,
#137507,#137508,#137509,#137510,#137511,#137512,#137513,#137514,#137515,
#137516,#137517,#137518,#137519,#137520,#137521,#137522,#137523,#137524,
#137525,#137526,#137527,#137528,#137529,#137530,#137531,#137532,#137533,
#137534,#137535,#137536,#137537,#137538,#137539,#137540,#137541,#137542,
#137543,#137544,#137545,#137546,#137547,#137548,#137549,#137550,#137551,
#137552,#137553,#137554,#137555,#137556,#137557,#137558,#137559,#137560,
#137561,#137562,#137563,#137564,#137565,#137566,#137567,#137568,#137569,
#137570,#137571,#137572,#137573,#137574,#137575,#137576,#137577,#137578,
#137579,#137580,#137581,#137582,#137583,#137584,#137585,#137586,#137587,
#137588,#137589,#137590,#137591,#137592,#137593,#137594,#137595,#137596,
#137597,#137598,#137599,#137600,#137601,#137602,#137603,#137604,#137605,
#137606,#137607,#137608,#137609,#137610,#137611,#137612,#137613,#137614,
#137615,#137616,#137617,#137618,#137619,#137620,#137621,#137622,#137623,
#137624,#137625,#137626,#137627,#137628,#137629,#137630,#137631,#137632,
#137633,#137634,#137635,#137636,#137637,#137638,#137639,#137640,#137641,
#137642,#137643,#137644,#137645,#137646,#137647,#137648,#137649),
 .UNSPECIFIED.,.F.,.F.,(4,3,3,3,3,3,3,3,3,3,3,3,3,3,3,3,3,3,3,3,3,3,3,3,
3,3,3,3,3,3,3,3,3,3,3,3,3,3,3,3,3,3,3,3,3,3,3,3,3,3,3,3,3,3,3,3,3,3,3,3,
3,3,3,3,3,3,3,3,3,3,3,3,3,3,3,3,3,3,3,4),(296.975200039958,297.060326286647,
297.087251811305,297.16135726261,297.235405773649,297.309412524818,297.383401802076,
297.457379176772,297.53138147581,297.585720354612,297.676719322946,297.768222397986,
297.860165787089,297.952200215175,298.044109164971,298.08418889792,298.159898714145,
298.235559860927,298.311186845588,298.386804685189,298.462416328099,298.538056394279,
298.582657441227,298.664935798978,298.747237943652,298.830709953873,298.913064491648,
298.997095238091,299.081125984535,299.16350559355,299.245870382945,299.329301419169,
299.411623981629,299.495609254735,299.579594527842,299.655234312579,299.730850091589,
299.806456335517,299.882090677131,299.957739915546,300.033449887924,300.07806307115,
300.169963088292,300.261995467677,300.353874434312,300.445501240997,300.536521816866,
300.576531614458,300.650534617295,300.724516639125,300.798492759581,300.872506336793,
300.946538714768,301.020644576809,301.075000157765,301.153959490174,301.232864811343,
301.311727734892,301.390559841608,301.469372687813,301.548191830672,301.627016356253,
301.705856778677,301.784723621197,301.863663625607,301.942642365685,302.021711404369,
302.07193724438,302.150936727855,302.229836004384,302.3086456406,302.387352824307,
302.465999328936,302.544582465666,302.570405787688,302.645321251716,302.720281133372,
302.795266419379,302.870323713808,302.902004435651),.UNSPECIFIED.);
#2988=B_SPLINE_CURVE_WITH_KNOTS('',3,(#137650,#137651,#137652,#137653,#137654,
#137655,#137656,#137657,#137658,#137659,#137660,#137661,#137662,#137663,
#137664,#137665),.UNSPECIFIED.,.F.,.F.,(4,3,3,3,3,4),(302.902004435756,
302.997785186833,303.068874330995,303.147952562583,303.22694819009,303.258525738749),
 .UNSPECIFIED.);
#2989=B_SPLINE_CURVE_WITH_KNOTS('',3,(#137667,#137668,#137669,#137670,#137671,
#137672,#137673,#137674,#137675,#137676,#137677,#137678,#137679,#137680,
#137681,#137682),.UNSPECIFIED.,.F.,.F.,(4,3,3,3,3,4),(-299.519174510177,
-299.436768573464,-299.354323050957,-299.271865440741,-299.189388037293,
-299.162764891651),.UNSPECIFIED.);
#2990=B_SPLINE_CURVE_WITH_KNOTS('',3,(#137683,#137684,#137685,#137686,#137687,
#137688,#137689,#137690,#137691,#137692,#137693,#137694,#137695,#137696,
#137697,#137698,#137699,#137700,#137701,#137702,#137703,#137704,#137705,
#137706,#137707,#137708,#137709,#137710,#137711,#137712,#137713,#137714,
#137715,#137716,#137717,#137718,#137719,#137720,#137721,#137722,#137723,
#137724,#137725,#137726,#137727,#137728,#137729,#137730,#137731,#137732,
#137733,#137734,#137735,#137736,#137737,#137738,#137739,#137740,#137741,
#137742,#137743,#137744,#137745,#137746,#137747,#137748,#137749,#137750,
#137751,#137752,#137753,#137754,#137755,#137756,#137757,#137758,#137759,
#137760,#137761,#137762,#137763,#137764,#137765,#137766,#137767,#137768,
#137769,#137770,#137771,#137772,#137773,#137774,#137775,#137776,#137777,
#137778,#137779,#137780,#137781,#137782,#137783,#137784,#137785,#137786,
#137787,#137788,#137789,#137790,#137791,#137792,#137793,#137794,#137795,
#137796,#137797,#137798,#137799,#137800,#137801,#137802,#137803,#137804,
#137805,#137806,#137807,#137808,#137809,#137810,#137811,#137812,#137813,
#137814,#137815,#137816,#137817,#137818,#137819,#137820,#137821,#137822,
#137823,#137824,#137825,#137826,#137827,#137828,#137829,#137830,#137831,
#137832,#137833,#137834,#137835,#137836,#137837,#137838,#137839,#137840,
#137841,#137842,#137843,#137844,#137845,#137846,#137847,#137848,#137849,
#137850,#137851,#137852,#137853,#137854,#137855,#137856,#137857,#137858,
#137859,#137860,#137861,#137862,#137863,#137864,#137865,#137866,#137867,
#137868,#137869,#137870,#137871,#137872,#137873,#137874,#137875,#137876,
#137877,#137878,#137879,#137880,#137881,#137882,#137883,#137884,#137885,
#137886,#137887,#137888,#137889,#137890,#137891,#137892,#137893,#137894,
#137895,#137896,#137897,#137898,#137899,#137900,#137901,#137902,#137903,
#137904,#137905,#137906,#137907,#137908,#137909,#137910,#137911,#137912,
#137913,#137914,#137915,#137916,#137917),.UNSPECIFIED.,.F.,.F.,(4,3,3,3,
3,3,3,3,3,3,3,3,3,3,3,3,3,3,3,3,3,3,3,3,3,3,3,3,3,3,3,3,3,3,3,3,3,3,3,3,
3,3,3,3,3,3,3,3,3,3,3,3,3,3,3,3,3,3,3,3,3,3,3,3,3,3,3,3,3,3,3,3,3,3,3,3,
3,3,4),(-299.162764891524,-299.081125984535,-298.99874738162,-298.916383606438,
-298.832952065135,-298.750630510816,-298.666643976022,-298.582657441227,
-298.507017190406,-298.431400944961,-298.355794234514,-298.28015942751,
-298.20450972403,-298.128799289021,-298.08418889792,-297.992288468792,-297.900255646981,
-297.808376225204,-297.716748972121,-297.625727980528,-297.585720354612,
-297.511718426913,-297.437737485504,-297.363762450475,-297.28974996401,
-297.215718680824,-297.141613915406,-297.087251811305,-297.008290393402,
-296.92938296833,-296.850517927347,-296.771683694538,-296.692868718443,
-296.61404745263,-296.535220811344,-296.456378284779,-296.377509353997,
-296.298567300463,-296.21958653277,-296.140515519565,-296.090314724689,
-296.011322839481,-295.9324310649,-295.853628818892,-295.774928827978,-295.69628939192,
-295.617713119395,-295.591846181382,-295.513259452359,-295.434623279105,
-295.355927279677,-295.277113241945,-295.198231807393,-295.119228707778,
-295.093377638074,-295.014305117287,-294.935305563532,-294.856367296706,
-294.777478683235,-294.698628127702,-294.61979962447,-294.54098325164,-294.462168501499,
-294.383344868565,-294.304474822055,-294.225581144014,-294.146620620199,
-294.096440551459,-294.022335113587,-293.948286615963,-293.874279878189,
-293.800290614271,-293.726313252894,-293.652310967098,-293.597972008152,
-293.506788969109,-293.415204127274,-293.323243588072,-293.23580359734),
 .UNSPECIFIED.);
#2991=B_SPLINE_CURVE_WITH_KNOTS('',3,(#137923,#137924,#137925,#137926,#137927,
#137928,#137929,#137930,#137931,#137932,#137933,#137934,#137935,#137936,
#137937,#137938,#137939,#137940,#137941,#137942,#137943,#137944,#137945,
#137946,#137947,#137948,#137949,#137950,#137951,#137952,#137953,#137954,
#137955,#137956,#137957,#137958,#137959,#137960,#137961,#137962,#137963,
#137964,#137965,#137966,#137967,#137968,#137969,#137970,#137971,#137972,
#137973,#137974,#137975,#137976,#137977,#137978,#137979,#137980,#137981,
#137982,#137983,#137984,#137985,#137986,#137987,#137988,#137989,#137990,
#137991,#137992,#137993,#137994,#137995,#137996,#137997,#137998,#137999,
#138000,#138001,#138002,#138003,#138004,#138005,#138006,#138007,#138008,
#138009,#138010,#138011,#138012,#138013,#138014,#138015,#138016,#138017,
#138018,#138019,#138020,#138021,#138022,#138023,#138024,#138025,#138026,
#138027,#138028,#138029,#138030,#138031,#138032,#138033,#138034,#138035,
#138036,#138037,#138038,#138039,#138040,#138041,#138042,#138043,#138044,
#138045,#138046,#138047,#138048,#138049,#138050,#138051,#138052,#138053,
#138054,#138055,#138056,#138057,#138058,#138059,#138060,#138061,#138062,
#138063,#138064,#138065,#138066,#138067,#138068,#138069,#138070,#138071,
#138072,#138073,#138074,#138075,#138076,#138077,#138078,#138079,#138080,
#138081,#138082,#138083,#138084,#138085,#138086,#138087,#138088,#138089,
#138090,#138091,#138092,#138093,#138094,#138095,#138096,#138097,#138098,
#138099,#138100,#138101,#138102,#138103,#138104,#138105,#138106,#138107,
#138108,#138109,#138110,#138111,#138112,#138113,#138114,#138115,#138116,
#138117,#138118,#138119,#138120,#138121,#138122,#138123,#138124,#138125,
#138126,#138127,#138128,#138129,#138130,#138131,#138132,#138133,#138134,
#138135,#138136,#138137,#138138,#138139,#138140,#138141,#138142,#138143,
#138144,#138145,#138146,#138147,#138148,#138149,#138150,#138151,#138152,
#138153,#138154,#138155,#138156,#138157),.UNSPECIFIED.,.F.,.F.,(4,3,3,3,
3,3,3,3,3,3,3,3,3,3,3,3,3,3,3,3,3,3,3,3,3,3,3,3,3,3,3,3,3,3,3,3,3,3,3,3,
3,3,3,3,3,3,3,3,3,3,3,3,3,3,3,3,3,3,3,3,3,3,3,3,3,3,3,3,3,3,3,3,3,3,3,3,
3,3,4),(290.691188989457,290.782659024431,290.874590100086,290.96662251805,
291.058539304055,291.105629291614,291.18133896279,291.256999964875,291.332626805271,
291.408244501611,291.483856001756,291.559495926441,291.604097834922,291.686376606522,
291.768679169128,291.852150971403,291.934505926045,292.018536152137,292.102566378229,
292.184945389364,292.267309579149,292.350740914746,292.433062888566,292.517048905051,
292.601034921537,292.676675030202,292.752291132552,292.827897699049,292.903532361204,
292.979181919227,293.054892208453,293.099503464844,293.191404036096,293.283437007398,
293.375316578752,293.466943976229,293.557965098977,293.597972008152,293.671973922603,
293.745954850711,293.819929872389,293.893942345456,293.967973615205,294.042078367181,
294.096440551459,294.175401966386,294.254309388427,294.333174426327,294.412008656013,
294.49082362895,294.569644891571,294.648471529648,294.727314052994,294.806182980555,
294.885125030883,294.96410579538,295.043176805432,295.093377638074,295.172369539784,
295.251261330761,295.330063593028,295.408763599925,295.487403051785,295.565979339797,
295.591846181382,295.670432894843,295.749069052265,295.82776503562,295.906579057027,
295.985460475111,296.064463558162,296.09031472469,296.171880226951,296.253354390263,
296.334739943628,296.416006787763,296.497198842002,296.578292418501,296.618819128577),
 .UNSPECIFIED.);
#2992=B_SPLINE_CURVE_WITH_KNOTS('',3,(#138158,#138159,#138160,#138161,#138162,
#138163,#138164,#138165,#138166,#138167,#138168,#138169,#138170,#138171,
#138172,#138173),.UNSPECIFIED.,.F.,.F.,(4,3,3,3,3,4),(296.618819128679,
296.703368262176,296.788149274131,296.873040522573,296.958059703437,296.975200039958),
 .UNSPECIFIED.);
#2993=B_SPLINE_CURVE_WITH_KNOTS('',3,(#138175,#138176,#138177,#138178,#138179,
#138180,#138181,#138182,#138183,#138184,#138185,#138186,#138187,#138188,
#138189,#138190),.UNSPECIFIED.,.F.,.F.,(4,3,3,3,3,4),(-293.23580359734,
-293.143889729308,-293.099503464844,-293.022641471914,-292.94584475079,
-292.879579584471),.UNSPECIFIED.);
#2994=B_SPLINE_CURVE_WITH_KNOTS('',3,(#138191,#138192,#138193,#138194,#138195,
#138196,#138197,#138198,#138199,#138200,#138201,#138202,#138203,#138204,
#138205,#138206,#138207,#138208,#138209,#138210,#138211,#138212,#138213,
#138214,#138215,#138216,#138217,#138218,#138219,#138220,#138221,#138222,
#138223,#138224,#138225,#138226,#138227,#138228,#138229,#138230,#138231,
#138232,#138233,#138234,#138235,#138236,#138237,#138238,#138239,#138240,
#138241,#138242,#138243,#138244,#138245,#138246,#138247,#138248,#138249,
#138250,#138251,#138252,#138253,#138254,#138255,#138256,#138257,#138258,
#138259,#138260,#138261,#138262,#138263,#138264,#138265,#138266,#138267,
#138268,#138269,#138270,#138271,#138272,#138273,#138274,#138275,#138276,
#138277,#138278,#138279,#138280,#138281,#138282,#138283,#138284,#138285,
#138286,#138287,#138288,#138289,#138290,#138291,#138292,#138293,#138294,
#138295,#138296,#138297,#138298,#138299,#138300,#138301,#138302,#138303,
#138304,#138305,#138306,#138307,#138308,#138309,#138310,#138311,#138312,
#138313,#138314,#138315,#138316,#138317,#138318,#138319,#138320,#138321,
#138322,#138323,#138324,#138325,#138326,#138327,#138328,#138329,#138330,
#138331,#138332,#138333,#138334,#138335,#138336,#138337,#138338,#138339,
#138340,#138341,#138342,#138343,#138344,#138345,#138346,#138347,#138348,
#138349,#138350,#138351,#138352,#138353,#138354,#138355,#138356,#138357,
#138358,#138359,#138360,#138361,#138362,#138363,#138364,#138365,#138366,
#138367,#138368,#138369,#138370,#138371,#138372,#138373,#138374,#138375,
#138376,#138377,#138378,#138379,#138380,#138381,#138382,#138383,#138384,
#138385,#138386,#138387,#138388,#138389,#138390,#138391,#138392,#138393,
#138394,#138395,#138396,#138397,#138398,#138399,#138400,#138401,#138402,
#138403,#138404,#138405,#138406,#138407,#138408,#138409,#138410),
 .UNSPECIFIED.,.F.,.F.,(4,3,3,3,3,3,3,3,3,3,3,3,3,3,3,3,3,3,3,3,3,3,3,3,
3,3,3,3,3,3,3,3,3,3,3,3,3,3,3,3,3,3,3,3,3,3,3,3,3,3,3,3,3,3,3,3,3,3,3,3,
3,3,3,3,3,3,3,3,3,3,3,3,3,4),(-292.879579584471,-292.797849710705,-292.716119956935,
-292.634390321493,-292.552660802714,-292.47093139893,-292.389202108476,
-292.304255339957,-292.220635864696,-292.138322943735,-292.056584034668,
-291.974845545282,-291.893107468902,-291.811369798854,-291.729632528466,
-291.647895651063,-291.566159159973,-291.484423048523,-291.402687310041,
-291.320951937854,-291.239216925292,-291.157482265683,-291.075747952356,
-290.99401397864,-290.912280337864,-290.830547023359,-290.748814028455,
-290.667081346481,-290.585348970769,-290.50361689465,-290.421885111455,
-290.340153614514,-290.258422397161,-290.176691452726,-290.094960774541,
-290.01323035594,-289.931500190255,-289.849770270818,-289.768040590963,
-289.686311144023,-289.600882949624,-289.5181243863,-289.436385758736,-289.354647954932,
-289.272910948193,-289.191174711825,-289.109439219139,-289.027704443448,
-288.945970358068,-288.864236936315,-288.78250415151,-288.700771976975,
-288.619040386034,-288.537309352013,-288.45557884824,-288.373848848046,
-288.292119324761,-288.208399924667,-288.126661843638,-288.044925348214,
-287.96319033163,-287.881456687141,-287.799724308024,-287.717993087571,
-287.63626291909,-287.55080616961,-287.469069251391,-287.387335242488,-287.305603715969,
-287.223874245041,-287.142139354565,-287.0604092744,-286.978677845338,-286.95260892325),
 .UNSPECIFIED.);
#2995=B_SPLINE_CURVE_WITH_KNOTS('',3,(#138416,#138417,#138418,#138419,#138420,
#138421,#138422,#138423,#138424,#138425,#138426,#138427,#138428,#138429,
#138430,#138431,#138432,#138433,#138434,#138435,#138436,#138437,#138438,
#138439,#138440,#138441,#138442,#138443,#138444,#138445,#138446,#138447,
#138448,#138449,#138450,#138451,#138452,#138453,#138454,#138455,#138456,
#138457,#138458,#138459,#138460,#138461,#138462,#138463,#138464,#138465,
#138466,#138467,#138468,#138469,#138470,#138471,#138472,#138473,#138474,
#138475,#138476,#138477,#138478,#138479,#138480,#138481,#138482,#138483,
#138484,#138485,#138486,#138487,#138488,#138489,#138490,#138491,#138492,
#138493,#138494,#138495,#138496,#138497,#138498,#138499,#138500,#138501,
#138502,#138503,#138504,#138505,#138506,#138507,#138508,#138509,#138510,
#138511,#138512,#138513,#138514,#138515,#138516,#138517,#138518,#138519,
#138520,#138521,#138522,#138523,#138524,#138525,#138526,#138527,#138528,
#138529,#138530,#138531,#138532,#138533,#138534,#138535,#138536,#138537,
#138538,#138539,#138540,#138541,#138542,#138543,#138544,#138545,#138546,
#138547,#138548,#138549,#138550,#138551,#138552,#138553,#138554,#138555,
#138556,#138557,#138558,#138559,#138560,#138561,#138562,#138563,#138564,
#138565,#138566,#138567,#138568,#138569,#138570,#138571,#138572,#138573,
#138574,#138575,#138576,#138577,#138578,#138579,#138580,#138581,#138582,
#138583,#138584,#138585,#138586,#138587,#138588,#138589,#138590,#138591,
#138592,#138593,#138594,#138595,#138596,#138597,#138598,#138599,#138600,
#138601,#138602,#138603,#138604,#138605,#138606,#138607,#138608,#138609,
#138610,#138611,#138612,#138613,#138614,#138615,#138616,#138617,#138618,
#138619,#138620,#138621,#138622,#138623,#138624,#138625,#138626,#138627,
#138628,#138629,#138630,#138631,#138632,#138633,#138634,#138635,#138636,
#138637,#138638,#138639,#138640,#138641,#138642,#138643,#138644,#138645,
#138646,#138647,#138648,#138649,#138650),.UNSPECIFIED.,.F.,.F.,(4,3,3,3,
3,3,3,3,3,3,3,3,3,3,3,3,3,3,3,3,3,3,3,3,3,3,3,3,3,3,3,3,3,3,3,3,3,3,3,3,
3,3,3,3,3,3,3,3,3,3,3,3,3,3,3,3,3,3,3,3,3,3,3,3,3,3,3,3,3,3,3,3,3,3,3,3,
3,3,4),(284.408859837487,284.484471751109,284.56011303113,284.625538228616,
284.707817000464,284.790119563321,284.873591365472,284.955946320364,285.039976546144,
285.124006771923,285.206385782528,285.28874997178,285.372181307643,285.454503280938,
285.538489298085,285.622475315231,285.698115424451,285.773731527356,285.849338094408,
285.924972757117,286.000622315693,286.076332605469,286.120943858538,286.212844428244,
286.304877397962,286.396756967787,286.488384363818,286.579405485302,286.619412401846,
286.693414316533,286.767395244875,286.841370266786,286.915382740085,286.989414010064,
287.063518762268,287.117880945153,287.1968423611,287.27574978417,287.354614823107,
287.433449053833,287.512264027813,287.591085291473,287.669911930586,287.748754454962,
287.827623383545,287.906565434877,287.985546200366,288.064617211384,288.114818031769,
288.193809927111,288.272701711788,288.351503967835,288.430203968659,288.508843414541,
288.587419696728,288.613286575076,288.691873298233,288.770509465491,288.849205458802,
288.928019490279,289.006900918497,289.085904011706,289.111755118384,289.190827640138,
289.269827194878,289.348765462706,289.427654077192,289.506504633753,289.585333138023,
289.664149511897,289.742964263085,289.821787897067,289.90065794462,289.9795516237,
290.058512148541,290.108692204999,290.190292057889,290.271695048658,290.335633821397),
 .UNSPECIFIED.);
#2996=B_SPLINE_CURVE_WITH_KNOTS('',3,(#138651,#138652,#138653,#138654,#138655,
#138656,#138657,#138658,#138659,#138660,#138661,#138662,#138663,#138664,
#138665,#138666),.UNSPECIFIED.,.F.,.F.,(4,3,3,3,3,4),(290.335633821483,
290.406514795855,290.477380699428,290.548271359671,290.607160748306,290.691188989457),
 .UNSPECIFIED.);
#2997=B_SPLINE_CURVE_WITH_KNOTS('',3,(#138668,#138669,#138670,#138671,#138672,
#138673,#138674,#138675,#138676,#138677,#138678,#138679,#138680,#138681,
#138682,#138683),.UNSPECIFIED.,.F.,.F.,(4,3,3,3,3,4),(-286.95260892325,
-286.870879379414,-286.789144264495,-286.707414027146,-286.625682238195,
-286.596394277292),.UNSPECIFIED.);
#2998=B_SPLINE_CURVE_WITH_KNOTS('',3,(#138684,#138685,#138686,#138687,#138688,
#138689,#138690,#138691,#138692,#138693,#138694,#138695,#138696,#138697,
#138698,#138699,#138700,#138701,#138702,#138703,#138704,#138705,#138706,
#138707,#138708,#138709,#138710,#138711,#138712,#138713,#138714,#138715,
#138716,#138717,#138718,#138719,#138720,#138721,#138722,#138723,#138724,
#138725,#138726,#138727,#138728,#138729,#138730,#138731,#138732,#138733,
#138734,#138735,#138736,#138737,#138738,#138739,#138740,#138741,#138742,
#138743,#138744,#138745,#138746,#138747,#138748,#138749,#138750,#138751,
#138752,#138753,#138754,#138755,#138756,#138757,#138758,#138759,#138760,
#138761,#138762,#138763,#138764,#138765,#138766,#138767,#138768,#138769,
#138770,#138771,#138772,#138773,#138774,#138775,#138776,#138777,#138778,
#138779,#138780,#138781,#138782,#138783,#138784,#138785,#138786,#138787,
#138788,#138789,#138790,#138791,#138792,#138793,#138794,#138795,#138796,
#138797,#138798,#138799,#138800,#138801,#138802,#138803,#138804,#138805,
#138806,#138807,#138808,#138809,#138810,#138811,#138812,#138813,#138814,
#138815,#138816,#138817,#138818,#138819,#138820,#138821,#138822,#138823,
#138824,#138825,#138826,#138827,#138828,#138829,#138830,#138831,#138832,
#138833,#138834,#138835,#138836,#138837,#138838,#138839,#138840,#138841,
#138842,#138843,#138844,#138845,#138846,#138847,#138848,#138849,#138850,
#138851,#138852,#138853,#138854,#138855,#138856,#138857,#138858,#138859,
#138860,#138861,#138862,#138863,#138864,#138865,#138866,#138867,#138868,
#138869,#138870,#138871,#138872,#138873,#138874,#138875,#138876,#138877,
#138878,#138879,#138880,#138881,#138882,#138883,#138884,#138885,#138886,
#138887,#138888,#138889,#138890,#138891,#138892,#138893,#138894,#138895,
#138896,#138897,#138898,#138899,#138900,#138901,#138902,#138903,#138904,
#138905,#138906,#138907,#138908,#138909,#138910,#138911,#138912,#138913,
#138914,#138915,#138916,#138917,#138918),.UNSPECIFIED.,.F.,.F.,(4,3,3,3,
3,3,3,3,3,3,3,3,3,3,3,3,3,3,3,3,3,3,3,3,3,3,3,3,3,3,3,3,3,3,3,3,3,3,3,3,
3,3,3,3,3,3,3,3,3,3,3,3,3,3,3,3,3,3,3,3,3,3,3,3,3,3,3,3,3,3,3,3,3,3,3,3,
3,3,4),(-286.596394277292,-286.505074083817,-286.409041527497,-286.316842690878,
-286.22459197147,-286.132509475947,-286.120943858538,-286.045234187422,
-285.969573185398,-285.893946345062,-285.818328648781,-285.742717148696,
-285.66707722407,-285.622475315231,-285.540196543376,-285.457893980512,
-285.374422178365,-285.292067223465,-285.208036997694,-285.124006771923,
-285.041627761322,-284.959263572073,-284.875832236209,-284.793510262917,
-284.709524245767,-284.625538228616,-284.549898119394,-284.474282016488,
-284.398675449434,-284.323040786724,-284.247391228145,-284.171680938368,
-284.127069685308,-284.035169115606,-283.943136145893,-283.851256576072,
-283.759629180044,-283.668608058564,-283.628601142001,-283.554599227313,
-283.480618298969,-283.406643277056,-283.332630803756,-283.258599533774,
-283.184494781569,-283.130132598693,-283.051171182746,-282.972263759677,
-282.89339872074,-282.814564490015,-282.735749516036,-282.656928252376,
-282.578101613264,-282.499259088887,-282.420390160305,-282.341448108973,
-282.262467343485,-282.183396332467,-282.133195512078,-282.054203616739,
-281.975311832064,-281.896509576019,-281.817809575197,-281.739170129318,
-281.660593847132,-281.63472696877,-281.556140245607,-281.477504078345,
-281.398808085029,-281.319994053547,-281.241112625324,-281.162109532109,
-281.136258425463,-281.05855966127,-280.980933020594,-280.90304644441,-280.825531995737,
-280.747459355796,-280.669386715856),.UNSPECIFIED.);
#2999=B_SPLINE_CURVE_WITH_KNOTS('',3,(#138924,#138925,#138926,#138927,#138928,
#138929,#138930,#138931,#138932,#138933,#138934,#138935,#138936,#138937,
#138938,#138939,#138940,#138941,#138942,#138943,#138944,#138945,#138946,
#138947,#138948,#138949,#138950,#138951,#138952,#138953,#138954,#138955,
#138956,#138957,#138958,#138959,#138960,#138961,#138962,#138963,#138964,
#138965,#138966,#138967,#138968,#138969,#138970,#138971,#138972,#138973,
#138974,#138975,#138976,#138977,#138978,#138979,#138980,#138981,#138982,
#138983,#138984,#138985,#138986,#138987,#138988,#138989,#138990,#138991,
#138992,#138993,#138994,#138995,#138996,#138997,#138998,#138999,#139000,
#139001,#139002,#139003,#139004,#139005,#139006,#139007,#139008,#139009,
#139010,#139011,#139012,#139013,#139014,#139015,#139016,#139017,#139018,
#139019,#139020,#139021,#139022,#139023,#139024,#139025,#139026,#139027,
#139028,#139029,#139030,#139031,#139032,#139033,#139034,#139035,#139036,
#139037,#139038,#139039,#139040,#139041,#139042,#139043,#139044,#139045,
#139046,#139047,#139048,#139049,#139050,#139051,#139052,#139053,#139054,
#139055,#139056,#139057,#139058,#139059,#139060,#139061,#139062,#139063,
#139064,#139065,#139066,#139067,#139068,#139069,#139070,#139071,#139072,
#139073,#139074,#139075,#139076,#139077,#139078,#139079,#139080,#139081,
#139082,#139083,#139084,#139085,#139086,#139087,#139088,#139089,#139090,
#139091,#139092,#139093,#139094,#139095,#139096,#139097,#139098,#139099,
#139100,#139101,#139102,#139103,#139104,#139105,#139106,#139107,#139108,
#139109,#139110,#139111,#139112,#139113,#139114,#139115,#139116,#139117,
#139118,#139119,#139120,#139121,#139122,#139123,#139124,#139125,#139126,
#139127,#139128,#139129,#139130,#139131,#139132,#139133,#139134,#139135,
#139136,#139137,#139138,#139139,#139140,#139141,#139142,#139143,#139144,
#139145,#139146,#139147,#139148,#139149,#139150,#139151,#139152,#139153,
#139154,#139155,#139156,#139157,#139158,#139159,#139160,#139161),
 .UNSPECIFIED.,.F.,.F.,(4,3,3,3,3,3,3,3,3,3,3,3,3,3,3,3,3,3,3,3,3,3,3,3,
3,3,3,3,3,3,3,3,3,3,3,3,3,3,3,3,3,3,3,3,3,3,3,3,3,3,3,3,3,3,3,3,3,3,3,3,
3,3,3,3,3,3,3,3,3,3,3,3,3,3,3,3,3,3,3,4),(278.125459419588,278.145447165617,
278.227826176221,278.310190365473,278.393621701336,278.475943674631,278.559929691778,
278.643915708925,278.719555818145,278.79517192105,278.870778488103,278.946413150811,
279.022062709388,279.097772999164,279.142384252232,279.234284821936,279.32631779165,
279.418197361473,279.509824757503,279.600845878986,279.64085279554,279.714854710229,
279.788835638572,279.862810660485,279.936823133786,280.010854403768,280.084959155973,
280.139321338848,280.218282754795,280.297190177864,280.3760552168,280.454889447526,
280.533704421505,280.612525685165,280.691352324277,280.770194848653,280.849063777236,
280.928005828567,281.006986594055,281.086057605073,281.136258425463,281.215250320801,
281.294142105475,281.372944361519,281.45164436234,281.530283808218,281.608860090403,
281.63472696877,281.713313691934,281.791949859198,281.870645852514,281.949459883998,
282.028341312222,282.107344405438,282.133195512078,282.212268033827,282.291267588562,
282.370205856386,282.449094470868,282.527945027424,282.60677353169,282.685589905558,
282.764404656742,282.843228290719,282.922098338268,283.000992017343,283.07995254218,
283.130132598693,283.204238036795,283.27828653465,283.352293272657,283.426282536809,
283.500259898421,283.574262184455,283.628601142001,283.717952507213,283.807870450816,
283.898002918138,283.988285085807,284.052448514116),.UNSPECIFIED.);
#3000=B_SPLINE_CURVE_WITH_KNOTS('',3,(#139162,#139163,#139164,#139165,#139166,
#139167,#139168,#139169,#139170,#139171,#139172,#139173,#139174,#139175,
#139176,#139177),.UNSPECIFIED.,.F.,.F.,(4,3,3,3,3,4),(284.052448514218,
284.127069685308,284.202777478049,284.278438680736,284.354067936897,284.408859837487),
 .UNSPECIFIED.);
#3001=B_SPLINE_CURVE_WITH_KNOTS('',3,(#139179,#139180,#139181,#139182,#139183,
#139184,#139185,#139186,#139187,#139188,#139189,#139190,#139191,#139192,
#139193,#139194),.UNSPECIFIED.,.F.,.F.,(4,3,3,3,3,4),(-280.669386715856,
-280.591919617408,-280.514418752512,-280.436900105981,-280.359320140393,
-280.313208970232),.UNSPECIFIED.);
#3002=B_SPLINE_CURVE_WITH_KNOTS('',3,(#139195,#139196,#139197,#139198,#139199,
#139200,#139201,#139202,#139203,#139204,#139205,#139206,#139207,#139208,
#139209,#139210,#139211,#139212,#139213,#139214,#139215,#139216,#139217,
#139218,#139219,#139220,#139221,#139222,#139223,#139224,#139225,#139226,
#139227,#139228,#139229,#139230,#139231,#139232,#139233,#139234,#139235,
#139236,#139237,#139238,#139239,#139240,#139241,#139242,#139243,#139244,
#139245,#139246,#139247,#139248,#139249,#139250,#139251,#139252,#139253,
#139254,#139255,#139256,#139257,#139258,#139259,#139260,#139261,#139262,
#139263,#139264,#139265,#139266,#139267,#139268,#139269,#139270,#139271,
#139272,#139273,#139274,#139275,#139276,#139277,#139278,#139279,#139280,
#139281,#139282,#139283,#139284,#139285,#139286,#139287,#139288,#139289,
#139290,#139291,#139292,#139293,#139294,#139295,#139296,#139297,#139298,
#139299,#139300,#139301,#139302,#139303,#139304,#139305,#139306,#139307,
#139308,#139309,#139310,#139311,#139312,#139313,#139314,#139315,#139316,
#139317,#139318,#139319,#139320,#139321,#139322,#139323,#139324,#139325,
#139326,#139327,#139328,#139329,#139330,#139331,#139332,#139333,#139334,
#139335,#139336,#139337,#139338,#139339,#139340,#139341,#139342,#139343,
#139344,#139345,#139346,#139347,#139348,#139349,#139350,#139351,#139352,
#139353,#139354,#139355,#139356,#139357,#139358,#139359,#139360,#139361,
#139362,#139363,#139364,#139365,#139366,#139367,#139368,#139369,#139370,
#139371,#139372,#139373,#139374,#139375,#139376,#139377,#139378,#139379,
#139380,#139381,#139382,#139383,#139384,#139385,#139386,#139387,#139388,
#139389,#139390,#139391,#139392,#139393,#139394,#139395,#139396,#139397,
#139398,#139399,#139400,#139401,#139402,#139403,#139404,#139405,#139406,
#139407,#139408,#139409,#139410,#139411,#139412,#139413,#139414,#139415,
#139416,#139417,#139418,#139419,#139420,#139421,#139422,#139423,#139424,
#139425,#139426,#139427,#139428,#139429),.UNSPECIFIED.,.F.,.F.,(4,3,3,3,
3,3,3,3,3,3,3,3,3,3,3,3,3,3,3,3,3,3,3,3,3,3,3,3,3,3,3,3,3,3,3,3,3,3,3,3,
3,3,3,3,3,3,3,3,3,3,3,3,3,3,3,3,3,3,3,3,3,3,3,3,3,3,3,3,3,3,3,3,3,3,3,3,
3,3,4),(-280.313208970112,-280.171571993323,-280.139321338848,-280.065215900744,
-279.991167402887,-279.917160664878,-279.843171400723,-279.769194039109,
-279.695191753074,-279.64085279554,-279.549853695804,-279.458350478127,
-279.366406939197,-279.274372362018,-279.182463271897,-279.142384252232,
-279.066674581115,-278.99101357909,-278.915386738754,-278.839769042472,
-278.764157542387,-278.68851761776,-278.643915708925,-278.56163693707,-278.479334374206,
-278.395862572059,-278.31350761716,-278.229477391388,-278.145447165617,
-278.063068155016,-277.980703965768,-277.897272629903,-277.814950656611,
-277.730964639461,-277.64697862231,-277.571338513088,-277.495722410181,
-277.420115843127,-277.344481180417,-277.268831621838,-277.193121332061,
-277.148510079002,-277.056609509301,-276.964576539589,-276.872696969768,
-276.781069573741,-276.690048452261,-276.650041535695,-276.576039621006,
-276.502058692663,-276.42808367075,-276.354071197449,-276.280039927468,
-276.205935175262,-276.151572992387,-276.07261157644,-275.99370415337,-275.914839114434,
-275.836004883708,-275.757189909729,-275.678368646069,-275.599542006956,
-275.52069948258,-275.441830553997,-275.362888502666,-275.283907737177,
-275.204836726159,-275.154635905772,-275.075644010434,-274.99675222576,
-274.917949969717,-274.839249968896,-274.760610523018,-274.682034240834,
-274.656167362465,-274.577575184507,-274.498944533264,-274.420231322113,
-274.38703094937),.UNSPECIFIED.);
#3003=B_SPLINE_CURVE_WITH_KNOTS('',3,(#139435,#139436,#139437,#139438,#139439,
#139440,#139441,#139442,#139443,#139444,#139445,#139446,#139447,#139448,
#139449,#139450,#139451,#139452,#139453,#139454,#139455,#139456,#139457,
#139458,#139459,#139460,#139461,#139462,#139463,#139464,#139465,#139466,
#139467,#139468,#139469,#139470,#139471,#139472,#139473,#139474,#139475,
#139476,#139477,#139478,#139479,#139480,#139481,#139482,#139483,#139484,
#139485,#139486,#139487,#139488,#139489,#139490,#139491,#139492,#139493,
#139494,#139495,#139496,#139497,#139498,#139499,#139500,#139501,#139502,
#139503,#139504,#139505,#139506,#139507,#139508,#139509,#139510,#139511,
#139512,#139513,#139514,#139515,#139516,#139517,#139518,#139519,#139520,
#139521,#139522,#139523,#139524,#139525,#139526,#139527,#139528,#139529,
#139530,#139531,#139532,#139533,#139534,#139535,#139536,#139537,#139538,
#139539,#139540,#139541,#139542,#139543,#139544,#139545,#139546,#139547,
#139548,#139549,#139550,#139551,#139552,#139553,#139554,#139555,#139556,
#139557,#139558,#139559,#139560,#139561,#139562,#139563,#139564,#139565,
#139566,#139567,#139568,#139569,#139570,#139571,#139572,#139573,#139574,
#139575,#139576,#139577,#139578,#139579,#139580,#139581,#139582,#139583,
#139584,#139585,#139586,#139587,#139588,#139589,#139590,#139591,#139592,
#139593,#139594,#139595,#139596,#139597,#139598,#139599,#139600,#139601,
#139602,#139603,#139604,#139605,#139606,#139607,#139608,#139609,#139610,
#139611,#139612,#139613,#139614,#139615,#139616,#139617,#139618,#139619,
#139620,#139621,#139622,#139623,#139624,#139625,#139626,#139627,#139628,
#139629,#139630,#139631,#139632,#139633,#139634,#139635,#139636,#139637,
#139638,#139639,#139640,#139641,#139642,#139643,#139644,#139645,#139646,
#139647,#139648,#139649,#139650,#139651,#139652,#139653,#139654,#139655,
#139656,#139657,#139658,#139659,#139660,#139661,#139662,#139663,#139664,
#139665,#139666,#139667,#139668,#139669,#139670,#139671,#139672,#139673,
#139674,#139675),.UNSPECIFIED.,.F.,.F.,(4,3,3,3,3,3,3,3,3,3,3,3,3,3,3,3,
3,3,3,3,3,3,3,3,3,3,3,3,3,3,3,3,3,3,3,3,3,3,3,3,3,3,3,3,3,3,3,3,3,3,3,3,
3,3,3,3,3,3,3,3,3,3,3,3,3,3,3,3,3,3,3,3,3,3,3,3,3,3,3,3,4),(271.842181774342,
271.917788389078,271.993426636706,272.069084165035,272.144799202209,272.163824645927,
272.255725215627,272.347758185338,272.439637755158,272.531265151185,272.622286272665,
272.662293189234,272.736295103923,272.810276032267,272.88425105418,272.958263527481,
273.032294797463,273.106399549668,273.160761732542,273.239723148489,273.318630571558,
273.397495610495,273.47632984122,273.555144815198,273.633966078858,273.712792717971,
273.791635242347,273.87050417093,273.949446222261,274.028426987749,274.107497998767,
274.157698819157,274.236690714496,274.315582499171,274.394384755216,274.473084756038,
274.551724201916,274.630300484102,274.656167362465,274.734754085628,274.813390252891,
274.892086246207,274.970900277689,275.049781705912,275.128784799127,275.154635905772,
275.233708427521,275.312707982256,275.39164625008,275.470534864562,275.549385421118,
275.628213925384,275.707030299253,275.785845050437,275.864668684414,275.943538731962,
276.022432411038,276.101392935875,276.151572992387,276.22567843049,276.299726928345,
276.373733666352,276.447722930505,276.521700292117,276.595702578151,276.650041535695,
276.741040635428,276.832543853103,276.924487392031,277.016521969207,277.108431059326,
277.148510079002,277.22421975012,277.299880752146,277.375507592485,277.451125288767,
277.526736788854,277.602376713482,277.64697862231,277.736638973094,277.769263207038),
 .UNSPECIFIED.);
#3004=B_SPLINE_CURVE_WITH_KNOTS('',3,(#139676,#139677,#139678,#139679,#139680,
#139681,#139682,#139683,#139684,#139685,#139686,#139687,#139688,#139689,
#139690,#139691),.UNSPECIFIED.,.F.,.F.,(4,3,3,3,3,4),(277.769263207152,
277.850658313745,277.932074100619,278.013494947125,278.094934709019,278.125459419588),
 .UNSPECIFIED.);
#3005=B_SPLINE_CURVE_WITH_KNOTS('',3,(#139693,#139694,#139695,#139696,#139697,
#139698,#139699,#139700,#139701,#139702,#139703,#139704,#139705),
 .UNSPECIFIED.,.F.,.F.,(4,3,3,3,4),(-274.38703094937,-274.308189681096,
-274.229211245105,-274.157698819157,-274.030023662932),.UNSPECIFIED.);
#3006=B_SPLINE_CURVE_WITH_KNOTS('',3,(#139706,#139707,#139708,#139709,#139710,
#139711,#139712,#139713,#139714,#139715,#139716,#139717,#139718,#139719,
#139720,#139721,#139722,#139723,#139724,#139725,#139726,#139727,#139728,
#139729,#139730,#139731,#139732,#139733,#139734,#139735,#139736,#139737,
#139738,#139739,#139740,#139741,#139742,#139743,#139744,#139745,#139746,
#139747,#139748,#139749,#139750,#139751,#139752,#139753,#139754,#139755,
#139756,#139757,#139758,#139759,#139760,#139761,#139762,#139763,#139764,
#139765,#139766,#139767,#139768,#139769,#139770,#139771,#139772,#139773,
#139774,#139775,#139776,#139777,#139778,#139779,#139780,#139781,#139782,
#139783,#139784,#139785,#139786,#139787,#139788,#139789,#139790,#139791,
#139792,#139793,#139794,#139795,#139796,#139797,#139798,#139799,#139800,
#139801,#139802,#139803,#139804,#139805,#139806,#139807,#139808,#139809,
#139810,#139811,#139812,#139813,#139814,#139815,#139816,#139817,#139818,
#139819,#139820,#139821,#139822,#139823,#139824,#139825,#139826,#139827,
#139828,#139829,#139830,#139831,#139832,#139833,#139834,#139835,#139836,
#139837,#139838,#139839,#139840,#139841,#139842,#139843,#139844,#139845,
#139846,#139847,#139848,#139849,#139850,#139851,#139852,#139853,#139854,
#139855,#139856,#139857,#139858,#139859,#139860,#139861,#139862,#139863,
#139864,#139865,#139866,#139867,#139868,#139869,#139870,#139871,#139872,
#139873,#139874,#139875,#139876,#139877,#139878,#139879,#139880,#139881,
#139882,#139883,#139884,#139885,#139886,#139887,#139888,#139889,#139890,
#139891,#139892,#139893,#139894,#139895,#139896,#139897,#139898,#139899,
#139900,#139901,#139902,#139903,#139904,#139905,#139906,#139907,#139908,
#139909,#139910,#139911,#139912,#139913,#139914,#139915,#139916,#139917,
#139918,#139919,#139920,#139921,#139922,#139923,#139924,#139925,#139926,
#139927,#139928,#139929,#139930,#139931,#139932,#139933,#139934,#139935,
#139936,#139937),.UNSPECIFIED.,.F.,.F.,(4,3,3,3,3,3,3,3,3,3,3,3,3,3,3,3,
3,3,3,3,3,3,3,3,3,3,3,3,3,3,3,3,3,3,3,3,3,3,3,3,3,3,3,3,3,3,3,3,3,3,3,3,
3,3,3,3,3,3,3,3,3,3,3,3,3,3,3,3,3,3,3,3,3,3,3,3,3,4),(-274.030023662853,
-273.951996221985,-273.874039086137,-273.796138642435,-273.716716528698,
-273.63888579274,-273.561067507186,-273.483249412772,-273.402627492714,
-273.324746987742,-273.242754360142,-273.160761732542,-273.08665629444,
-273.012607796585,-272.938601058577,-272.864611794424,-272.790634432811,
-272.716632146778,-272.662293189234,-272.571294089501,-272.479790871824,
-272.387847332896,-272.295812755718,-272.203903665599,-272.163824645927,
-272.088114974809,-272.012453972782,-271.936827132444,-271.861209436161,
-271.785597936074,-271.709958011445,-271.665356102619,-271.583077330767,
-271.500774767905,-271.417302965757,-271.33494801086,-271.250917785086,
-271.166887559312,-271.08450854871,-271.00214435946,-270.918713023596,-270.836391050303,
-270.752405033154,-270.668419016004,-270.592778906782,-270.517162803874,
-270.44155623682,-270.36592157411,-270.290272015531,-270.214561725753,-270.169950472696,
-270.078049902996,-269.986016933286,-269.894137363467,-269.80250996744,
-269.711488845961,-269.671481929389,-269.5974800147,-269.523499086356,-269.449524064443,
-269.375511591142,-269.30148032116,-269.227375568955,-269.173013386081,
-269.094051970134,-269.015144547065,-268.936279508129,-268.857445277403,
-268.778630303423,-268.699809039763,-268.620982400651,-268.542139876274,
-268.463270947691,-268.38432889636,-268.305348130871,-268.226277119853,
-268.176076299466,-268.102429383984),.UNSPECIFIED.);
#3007=B_SPLINE_CURVE_WITH_KNOTS('',3,(#139943,#139944,#139945,#139946,#139947,
#139948,#139949,#139950,#139951,#139952,#139953,#139954,#139955,#139956,
#139957,#139958,#139959,#139960,#139961,#139962,#139963,#139964,#139965,
#139966,#139967,#139968,#139969,#139970,#139971,#139972,#139973,#139974,
#139975,#139976,#139977,#139978,#139979,#139980,#139981,#139982,#139983,
#139984,#139985,#139986,#139987,#139988,#139989,#139990,#139991,#139992,
#139993,#139994,#139995,#139996,#139997,#139998,#139999,#140000,#140001,
#140002,#140003,#140004,#140005,#140006,#140007,#140008,#140009,#140010,
#140011,#140012,#140013,#140014,#140015,#140016,#140017,#140018,#140019,
#140020,#140021,#140022,#140023,#140024,#140025,#140026,#140027,#140028,
#140029,#140030,#140031,#140032,#140033,#140034,#140035,#140036,#140037,
#140038,#140039,#140040,#140041,#140042,#140043,#140044,#140045,#140046,
#140047,#140048,#140049,#140050,#140051,#140052,#140053,#140054,#140055,
#140056,#140057,#140058,#140059,#140060,#140061,#140062,#140063,#140064,
#140065,#140066,#140067,#140068,#140069,#140070,#140071,#140072,#140073,
#140074,#140075,#140076,#140077,#140078,#140079,#140080,#140081,#140082,
#140083,#140084,#140085,#140086,#140087,#140088,#140089,#140090,#140091,
#140092,#140093,#140094,#140095,#140096,#140097,#140098,#140099,#140100,
#140101,#140102,#140103,#140104,#140105,#140106,#140107,#140108,#140109,
#140110,#140111,#140112,#140113,#140114,#140115,#140116,#140117,#140118,
#140119,#140120,#140121,#140122,#140123,#140124,#140125,#140126,#140127,
#140128,#140129,#140130,#140131,#140132,#140133,#140134,#140135,#140136,
#140137,#140138,#140139,#140140,#140141,#140142,#140143,#140144,#140145,
#140146,#140147,#140148,#140149,#140150,#140151,#140152,#140153,#140154,
#140155,#140156,#140157,#140158,#140159,#140160,#140161,#140162,#140163,
#140164,#140165,#140166,#140167,#140168,#140169,#140170,#140171,#140172,
#140173,#140174,#140175,#140176,#140177,#140178,#140179,#140180),
 .UNSPECIFIED.,.F.,.F.,(4,3,3,3,3,3,3,3,3,3,3,3,3,3,3,3,3,3,3,3,3,3,3,3,
3,3,3,3,3,3,3,3,3,3,3,3,3,3,3,3,3,3,3,3,3,3,3,3,3,3,3,3,3,3,3,3,3,3,3,3,
3,3,3,3,3,3,3,3,3,3,3,3,3,3,3,3,3,3,3,4),(265.559741333664,265.650294523403,
265.683733582928,265.757735497617,265.831716425961,265.905691447874,265.979703921175,
266.053735191157,266.127839943363,266.182202126236,266.261163542183,266.340070965252,
266.418936004189,266.497770234914,266.576585208893,266.655406472553,266.734233111665,
266.813075636041,266.891944564624,266.970886615955,267.049867381444,267.128938392461,
267.179139212851,267.25813110819,267.337022892865,267.41582514891,267.494525149732,
267.57316459561,267.651740877796,267.677607756159,267.756194479322,267.834830646585,
267.9135266399,267.992340671383,268.071222099606,268.150225192821,268.176076299466,
268.255148821215,268.33414837595,268.413086643774,268.491975258256,268.570825814812,
268.649654319077,268.728470692946,268.80728544413,268.886109078107,268.964979125656,
269.043872804731,269.122833329568,269.173013386081,269.247118824183,269.321167322038,
269.395174060045,269.469163324198,269.54314068581,269.617142971843,269.671481929389,
269.762481029126,269.853984246805,269.945927785737,270.037962362917,270.12987145304,
270.169950472697,270.245660143813,270.321321145838,270.396947986175,270.472565682456,
270.548177182542,270.623817107169,270.668419016004,270.750697787859,270.833000350723,
270.91647215287,270.99882710777,271.082857333541,271.166887559312,271.248393466682,
271.329881157949,271.411356799843,271.486077899858),.UNSPECIFIED.);
#3008=B_SPLINE_CURVE_WITH_KNOTS('',3,(#140181,#140182,#140183,#140184,#140185,
#140186,#140187,#140188,#140189,#140190,#140191,#140192,#140193,#140194,
#140195,#140196),.UNSPECIFIED.,.F.,.F.,(4,3,3,3,3,4),(271.486077899858,
271.575717001239,271.665356102619,271.740996288,271.816611901616,271.842181774342),
 .UNSPECIFIED.);
#3009=B_SPLINE_CURVE_WITH_KNOTS('',3,(#140198,#140199,#140200,#140201,#140202,
#140203,#140204,#140205,#140206,#140207,#140208,#140209,#140210,#140211,
#140212,#140213),.UNSPECIFIED.,.F.,.F.,(4,3,3,3,3,4),(-268.102429383984,
-268.022019545821,-267.941766207012,-267.861606921436,-267.781567544259,
-267.74683835584),.UNSPECIFIED.);
#3010=B_SPLINE_CURVE_WITH_KNOTS('',3,(#140214,#140215,#140216,#140217,#140218,
#140219,#140220,#140221,#140222,#140223,#140224,#140225,#140226,#140227,
#140228,#140229,#140230,#140231,#140232,#140233,#140234,#140235,#140236,
#140237,#140238,#140239,#140240,#140241,#140242,#140243,#140244,#140245,
#140246,#140247,#140248,#140249,#140250,#140251,#140252,#140253,#140254,
#140255,#140256,#140257,#140258,#140259,#140260,#140261,#140262,#140263,
#140264,#140265,#140266,#140267,#140268,#140269,#140270,#140271,#140272,
#140273,#140274,#140275,#140276,#140277,#140278,#140279,#140280,#140281,
#140282,#140283,#140284,#140285,#140286,#140287,#140288,#140289,#140290,
#140291,#140292,#140293,#140294,#140295,#140296,#140297,#140298,#140299,
#140300,#140301,#140302,#140303,#140304,#140305,#140306,#140307,#140308,
#140309,#140310,#140311,#140312,#140313,#140314,#140315,#140316,#140317,
#140318,#140319,#140320,#140321,#140322,#140323,#140324,#140325,#140326,
#140327,#140328,#140329,#140330,#140331,#140332,#140333,#140334,#140335,
#140336,#140337,#140338,#140339,#140340,#140341,#140342,#140343,#140344,
#140345,#140346,#140347,#140348,#140349,#140350,#140351,#140352,#140353,
#140354,#140355,#140356,#140357,#140358,#140359,#140360,#140361,#140362,
#140363,#140364,#140365,#140366,#140367,#140368,#140369,#140370,#140371,
#140372,#140373,#140374,#140375,#140376,#140377,#140378,#140379,#140380,
#140381,#140382,#140383,#140384,#140385,#140386,#140387,#140388,#140389,
#140390,#140391,#140392,#140393,#140394,#140395,#140396,#140397,#140398,
#140399,#140400,#140401,#140402,#140403,#140404,#140405,#140406,#140407,
#140408,#140409,#140410,#140411,#140412,#140413,#140414,#140415,#140416,
#140417,#140418,#140419,#140420,#140421,#140422,#140423,#140424,#140425,
#140426,#140427,#140428,#140429,#140430,#140431,#140432,#140433,#140434,
#140435,#140436,#140437,#140438,#140439,#140440,#140441,#140442,#140443,
#140444,#140445,#140446,#140447,#140448),.UNSPECIFIED.,.F.,.F.,(4,3,3,3,
3,3,3,3,3,3,3,3,3,3,3,3,3,3,3,3,3,3,3,3,3,3,3,3,3,3,3,3,3,3,3,3,3,3,3,3,
3,3,3,3,3,3,3,3,3,3,3,3,3,3,3,3,3,3,3,3,3,3,3,3,3,3,3,3,3,3,3,3,3,3,3,3,
3,3,4),(-267.746838355753,-267.677607756159,-267.59902103299,-267.520384865722,
-267.441688872401,-267.362874840913,-267.283993412684,-267.204990319463,
-267.179139212851,-267.100066691102,-267.021067136368,-266.942128868545,
-266.863240254064,-266.784389697509,-266.705561193244,-266.626744819376,
-266.547930068193,-266.469106434217,-266.390236386669,-266.311342707595,
-266.232382182759,-266.182202126236,-266.108096688134,-266.034048190279,
-265.960041452272,-265.886052188119,-265.812074826506,-265.738072540473,
-265.683733582928,-265.592734483193,-265.501231265519,-265.40928772659,
-265.317253149413,-265.225344059293,-265.185265039621,-265.109555368503,
-265.033894366476,-264.958267526138,-264.882649829855,-264.807038329767,
-264.731398405139,-264.686796496313,-264.604517724461,-264.522215161599,
-264.438743359451,-264.356388404554,-264.27235817878,-264.188327953006,
-264.105948942403,-264.023584753153,-263.940153417289,-263.857831443995,
-263.773845426847,-263.689859409698,-263.614219300477,-263.538603197572,
-263.462996630519,-263.38736196781,-263.311712409233,-263.236002119457,
-263.191390866391,-263.099490296686,-263.007457326971,-262.915577757147,
-262.823950361117,-262.732929239634,-262.692922323083,-262.618920408396,
-262.544939480053,-262.470964458141,-262.396951984841,-262.322920714861,
-262.248815962657,-262.194453779776,-262.115994960713,-262.037605868093,
-261.959258290357,-261.880941468947,-261.82024085972),.UNSPECIFIED.);
#3011=B_SPLINE_CURVE_WITH_KNOTS('',3,(#140454,#140455,#140456,#140457,#140458,
#140459,#140460,#140461,#140462,#140463,#140464,#140465,#140466,#140467,
#140468,#140469,#140470,#140471,#140472,#140473,#140474,#140475,#140476,
#140477,#140478,#140479,#140480,#140481,#140482,#140483,#140484,#140485,
#140486,#140487,#140488,#140489,#140490,#140491,#140492,#140493,#140494,
#140495,#140496,#140497,#140498,#140499,#140500,#140501,#140502,#140503,
#140504,#140505,#140506,#140507,#140508,#140509,#140510,#140511,#140512,
#140513,#140514,#140515,#140516,#140517,#140518,#140519,#140520,#140521,
#140522,#140523,#140524,#140525,#140526,#140527,#140528,#140529,#140530,
#140531,#140532,#140533,#140534,#140535,#140536,#140537,#140538,#140539,
#140540,#140541,#140542,#140543,#140544,#140545,#140546,#140547,#140548,
#140549,#140550,#140551,#140552,#140553,#140554,#140555,#140556,#140557,
#140558,#140559,#140560,#140561,#140562,#140563,#140564,#140565,#140566,
#140567,#140568,#140569,#140570,#140571,#140572,#140573,#140574,#140575,
#140576,#140577,#140578,#140579,#140580,#140581,#140582,#140583,#140584,
#140585,#140586,#140587,#140588,#140589,#140590,#140591,#140592,#140593,
#140594,#140595,#140596,#140597,#140598,#140599,#140600,#140601,#140602,
#140603,#140604,#140605,#140606,#140607,#140608,#140609,#140610,#140611,
#140612,#140613,#140614,#140615,#140616,#140617,#140618,#140619,#140620,
#140621,#140622,#140623,#140624,#140625,#140626,#140627,#140628,#140629,
#140630,#140631,#140632,#140633,#140634,#140635,#140636,#140637,#140638,
#140639,#140640,#140641,#140642,#140643,#140644,#140645,#140646,#140647,
#140648,#140649,#140650,#140651,#140652,#140653,#140654,#140655,#140656,
#140657,#140658,#140659,#140660,#140661,#140662,#140663,#140664,#140665,
#140666,#140667,#140668,#140669,#140670,#140671,#140672,#140673,#140674,
#140675,#140676,#140677,#140678,#140679,#140680,#140681,#140682,#140683,
#140684,#140685,#140686,#140687,#140688,#140689,#140690,#140691),
 .UNSPECIFIED.,.F.,.F.,(4,3,3,3,3,3,3,3,3,3,3,3,3,3,3,3,3,3,3,3,3,3,3,3,
3,3,3,3,3,3,3,3,3,3,3,3,3,3,3,3,3,3,3,3,3,3,3,3,3,3,3,3,3,3,3,3,3,3,3,3,
3,3,3,3,3,3,3,3,3,3,3,3,3,3,3,3,3,3,3,4),(259.275636793971,259.354548515047,
259.433416828795,259.512253313696,259.591069523036,259.669890816851,259.74871655884,
259.827557258332,259.906423433194,259.985362535655,260.064339495741,260.143408327936,
260.200579606545,260.279571501884,260.358463286559,260.437265542604,260.515965543426,
260.594604989306,260.673181271491,260.699048149853,260.777634873016,260.856271040278,
260.934967033593,261.013781065075,261.092662493298,261.171665586513,261.19751669316,
261.27658921491,261.355588769645,261.43452703747,261.513415651951,261.592266208508,
261.671094712774,261.749911086643,261.828725837828,261.907549471805,261.986419519354,
262.06531319843,262.144273723268,262.194453779776,262.268559217878,262.342607715732,
262.416614453739,262.490603717892,262.564581079503,262.638583365536,262.692922323083,
262.783921422819,262.875424640497,262.967368179428,263.059402756607,263.151311846729,
263.191390866391,263.267100537508,263.342761539533,263.418388379871,263.494006076152,
263.569617576239,263.645257500866,263.689859409698,263.772138181552,263.854440744416,
263.937912546563,264.020267501462,264.104297727234,264.188327953006,264.270706963607,
264.353071152856,264.43650248872,264.518824462012,264.602810479163,264.686796496313,
264.762436605534,264.83805270844,264.913659275494,264.989293938203,265.064943496781,
265.140653786557,265.185265039621,265.202892592679),.UNSPECIFIED.);
#3012=B_SPLINE_CURVE_WITH_KNOTS('',3,(#140692,#140693,#140694,#140695,#140696,
#140697,#140698,#140699,#140700,#140701,#140702,#140703,#140704),
 .UNSPECIFIED.,.F.,.F.,(4,3,3,3,4),(265.202892592755,265.294397540302,265.385932105706,
265.477236696826,265.559741333664),.UNSPECIFIED.);
#3013=B_SPLINE_CURVE_WITH_KNOTS('',3,(#140706,#140707,#140708,#140709,#140710,
#140711,#140712,#140713,#140714,#140715,#140716,#140717,#140718,#140719,
#140720,#140721),.UNSPECIFIED.,.F.,.F.,(4,3,3,3,3,4),(-261.82024085972,
-261.741950618838,-261.663641105925,-261.585322321214,-261.506958996887,
-261.463653048573),.UNSPECIFIED.);
#3014=B_SPLINE_CURVE_WITH_KNOTS('',3,(#140722,#140723,#140724,#140725,#140726,
#140727,#140728,#140729,#140730,#140731,#140732,#140733,#140734,#140735,
#140736,#140737,#140738,#140739,#140740,#140741,#140742,#140743,#140744,
#140745,#140746,#140747,#140748,#140749,#140750,#140751,#140752,#140753,
#140754,#140755,#140756,#140757,#140758,#140759,#140760,#140761,#140762,
#140763,#140764,#140765,#140766,#140767,#140768,#140769,#140770,#140771,
#140772,#140773,#140774,#140775,#140776,#140777,#140778,#140779,#140780,
#140781,#140782,#140783,#140784,#140785,#140786,#140787,#140788,#140789,
#140790,#140791,#140792,#140793,#140794,#140795,#140796,#140797,#140798,
#140799,#140800,#140801,#140802,#140803,#140804,#140805,#140806,#140807,
#140808,#140809,#140810,#140811,#140812,#140813,#140814,#140815,#140816,
#140817,#140818,#140819,#140820,#140821,#140822,#140823,#140824,#140825,
#140826,#140827,#140828,#140829,#140830,#140831,#140832,#140833,#140834,
#140835,#140836,#140837,#140838,#140839,#140840,#140841,#140842,#140843,
#140844,#140845,#140846,#140847,#140848,#140849,#140850,#140851,#140852,
#140853,#140854,#140855,#140856,#140857,#140858,#140859,#140860,#140861,
#140862,#140863,#140864,#140865,#140866,#140867,#140868,#140869,#140870,
#140871,#140872,#140873,#140874,#140875,#140876,#140877,#140878,#140879,
#140880,#140881,#140882,#140883,#140884,#140885,#140886,#140887,#140888,
#140889,#140890,#140891,#140892,#140893,#140894,#140895,#140896,#140897,
#140898,#140899,#140900,#140901,#140902,#140903,#140904,#140905,#140906,
#140907,#140908,#140909,#140910,#140911,#140912,#140913,#140914,#140915,
#140916,#140917,#140918,#140919,#140920,#140921,#140922,#140923,#140924,
#140925,#140926,#140927,#140928,#140929,#140930,#140931,#140932,#140933,
#140934,#140935,#140936,#140937,#140938,#140939,#140940,#140941,#140942,
#140943,#140944,#140945,#140946,#140947,#140948,#140949,#140950,#140951,
#140952,#140953,#140954,#140955,#140956),.UNSPECIFIED.,.F.,.F.,(4,3,3,3,
3,3,3,3,3,3,3,3,3,3,3,3,3,3,3,3,3,3,3,3,3,3,3,3,3,3,3,3,3,3,3,3,3,3,3,3,
3,3,3,3,3,3,3,3,3,3,3,3,3,3,3,3,3,3,3,3,3,3,3,3,3,3,3,3,3,3,3,3,3,3,3,3,
3,3,4),(-261.463653048459,-261.365739326353,-261.266508210912,-261.19751669316,
-261.118524797823,-261.03963301315,-260.960830757107,-260.882130756287,
-260.80349131041,-260.724915028226,-260.699048149853,-260.620461426688,
-260.541825259424,-260.463129266106,-260.384315234622,-260.305433806398,
-260.22643071318,-260.200579606545,-260.121507084795,-260.04250753006,-259.963569262236,
-259.884680647755,-259.805830091199,-259.727001586933,-259.648185213064,
-259.569370461881,-259.490546827903,-259.411676780355,-259.332783101279,
-259.253822576442,-259.20364251993,-259.129537081829,-259.055488583975,
-258.981481845968,-258.907492581816,-258.833515220205,-258.759512934173,
-258.705173976623,-258.614174876885,-258.522671659206,-258.430728120274,
-258.338693543093,-258.246784452969,-258.206705433315,-258.130995762198,
-258.055334760173,-257.979707919836,-257.904090223555,-257.828478723469,
-257.752838798842,-257.708236890008,-257.625958118154,-257.543655555291,
-257.460183753144,-257.377828798245,-257.293798572473,-257.2097683467,-257.127389336097,
-257.045025146846,-256.961593810982,-256.879271837688,-256.79528582054,
-256.711299803392,-256.635659694172,-256.560043591267,-256.484437024215,
-256.408802361507,-256.33315280293,-256.257442513154,-256.212831260085,
-256.12093069038,-256.028897720663,-255.937018150839,-255.845390754807,
-255.754369633324,-255.714362716777,-255.640362204278,-255.566381661442,
-255.536653192137),.UNSPECIFIED.);
#3015=B_SPLINE_CURVE_WITH_KNOTS('',3,(#140962,#140963,#140964,#140965,#140966,
#140967,#140968,#140969,#140970,#140971,#140972,#140973,#140974,#140975,
#140976,#140977,#140978,#140979,#140980,#140981,#140982,#140983,#140984,
#140985,#140986,#140987,#140988,#140989,#140990,#140991,#140992,#140993,
#140994,#140995,#140996,#140997,#140998,#140999,#141000,#141001,#141002,
#141003,#141004,#141005,#141006,#141007,#141008,#141009,#141010,#141011,
#141012,#141013,#141014,#141015,#141016,#141017,#141018,#141019,#141020,
#141021,#141022,#141023,#141024,#141025,#141026,#141027,#141028,#141029,
#141030,#141031,#141032,#141033,#141034,#141035,#141036,#141037,#141038,
#141039,#141040,#141041,#141042,#141043,#141044,#141045,#141046,#141047,
#141048,#141049,#141050,#141051,#141052,#141053,#141054,#141055,#141056,
#141057,#141058,#141059,#141060,#141061,#141062,#141063,#141064,#141065,
#141066,#141067,#141068,#141069,#141070,#141071,#141072,#141073,#141074,
#141075,#141076,#141077,#141078,#141079,#141080,#141081,#141082,#141083,
#141084,#141085,#141086,#141087,#141088,#141089,#141090,#141091,#141092,
#141093,#141094,#141095,#141096,#141097,#141098,#141099,#141100,#141101,
#141102,#141103,#141104,#141105,#141106,#141107,#141108,#141109,#141110,
#141111,#141112,#141113,#141114,#141115,#141116,#141117,#141118,#141119,
#141120,#141121,#141122,#141123,#141124,#141125,#141126,#141127,#141128,
#141129,#141130,#141131,#141132,#141133,#141134,#141135,#141136,#141137,
#141138,#141139,#141140,#141141,#141142,#141143,#141144,#141145,#141146,
#141147,#141148,#141149,#141150,#141151,#141152,#141153,#141154,#141155,
#141156,#141157,#141158,#141159,#141160,#141161,#141162,#141163,#141164,
#141165,#141166,#141167,#141168,#141169,#141170,#141171,#141172,#141173,
#141174,#141175,#141176,#141177,#141178,#141179,#141180,#141181,#141182,
#141183,#141184,#141185,#141186,#141187,#141188,#141189,#141190,#141191,
#141192,#141193,#141194,#141195,#141196),.UNSPECIFIED.,.F.,.F.,(4,3,3,3,
3,3,3,3,3,3,3,3,3,3,3,3,3,3,3,3,3,3,3,3,3,3,3,3,3,3,3,3,3,3,3,3,3,3,3,3,
3,3,3,3,3,3,3,3,3,3,3,3,3,3,3,3,3,3,3,3,3,3,3,3,3,3,3,3,3,3,3,3,3,3,3,3,
3,3,4),(252.992365321722,253.072326619286,253.152399003248,253.222020000239,
253.301011895578,253.379903680253,253.458705936298,253.53740593712,253.616045382999,
253.694621665185,253.720488543547,253.799075266711,253.877711433975,253.956407427292,
254.035221458775,254.114102887,254.193105980216,254.218957086855,254.298029608604,
254.377029163339,254.455967431163,254.534856045644,254.6137066022,254.692535106466,
254.771351480335,254.850166231518,254.928989865496,255.007859913044,255.086753592119,
255.165714116956,255.21589417347,255.289999611571,255.364048109426,255.438054847432,
255.512044111584,255.586021473196,255.660023759229,255.714362716777,255.805361816515,
255.896865034194,255.988808573126,256.080843150307,256.17275224043,256.212831260085,
256.288540931202,256.364201933227,256.439828773564,256.515446469845,256.591057969931,
256.666697894558,256.711299803392,256.793578575246,256.875881138109,256.959352940256,
257.041707895155,257.125738120927,257.2097683467,257.292147357303,257.374511546554,
257.457942882418,257.540264855712,257.62425087286,257.708236890008,257.783876999228,
257.859493102133,257.935099669185,258.010734331894,258.08638389047,258.162094180246,
258.206705433315,258.298606003021,258.390638972737,258.482518542562,258.574145938593,
258.665167060077,258.705173976623,258.775894354609,258.847800819991,258.919707285374),
 .UNSPECIFIED.);
#3016=B_SPLINE_CURVE_WITH_KNOTS('',3,(#141197,#141198,#141199,#141200,#141201,
#141202,#141203,#141204,#141205,#141206,#141207,#141208,#141209,#141210,
#141211,#141212),.UNSPECIFIED.,.F.,.F.,(4,3,3,3,3,4),(258.919707285499,
258.998551910999,259.077463224529,259.156505125832,259.20364251993,259.275636793971),
 .UNSPECIFIED.);
#3017=B_SPLINE_CURVE_WITH_KNOTS('',3,(#141214,#141215,#141216,#141217,#141218,
#141219,#141220,#141221,#141222,#141223,#141224,#141225,#141226,#141227,
#141228,#141229,#141230,#141231,#141232),.UNSPECIFIED.,.F.,.F.,(4,3,3,3,
3,3,4),(-255.536653192137,-255.462676298287,-255.388657906524,-255.3146152606,
-255.240504027705,-255.21589417347,-255.180467741394),.UNSPECIFIED.);
#3018=B_SPLINE_CURVE_WITH_KNOTS('',3,(#141233,#141234,#141235,#141236,#141237,
#141238,#141239,#141240,#141241,#141242,#141243,#141244,#141245,#141246,
#141247,#141248,#141249,#141250,#141251,#141252,#141253,#141254,#141255,
#141256,#141257,#141258,#141259,#141260,#141261,#141262,#141263,#141264,
#141265,#141266,#141267,#141268,#141269,#141270,#141271,#141272,#141273,
#141274,#141275,#141276,#141277,#141278,#141279,#141280,#141281,#141282,
#141283,#141284,#141285,#141286,#141287,#141288,#141289,#141290,#141291,
#141292,#141293,#141294,#141295,#141296,#141297,#141298,#141299,#141300,
#141301,#141302,#141303,#141304,#141305,#141306,#141307,#141308,#141309,
#141310,#141311,#141312,#141313,#141314,#141315,#141316,#141317,#141318,
#141319,#141320,#141321,#141322,#141323,#141324,#141325,#141326,#141327,
#141328,#141329,#141330,#141331,#141332,#141333,#141334,#141335,#141336,
#141337,#141338,#141339,#141340,#141341,#141342,#141343,#141344,#141345,
#141346,#141347,#141348,#141349,#141350,#141351,#141352,#141353,#141354,
#141355,#141356,#141357,#141358,#141359,#141360,#141361,#141362,#141363,
#141364,#141365,#141366,#141367,#141368,#141369,#141370,#141371,#141372,
#141373,#141374,#141375,#141376,#141377,#141378,#141379,#141380,#141381,
#141382,#141383,#141384,#141385,#141386,#141387,#141388,#141389,#141390,
#141391,#141392,#141393,#141394,#141395,#141396,#141397,#141398,#141399,
#141400,#141401,#141402,#141403,#141404,#141405,#141406,#141407,#141408,
#141409,#141410,#141411,#141412,#141413,#141414,#141415,#141416,#141417,
#141418,#141419,#141420,#141421,#141422,#141423,#141424,#141425,#141426,
#141427,#141428,#141429,#141430,#141431,#141432,#141433,#141434,#141435,
#141436,#141437,#141438,#141439,#141440,#141441,#141442,#141443,#141444,
#141445,#141446,#141447,#141448,#141449,#141450,#141451,#141452,#141453,
#141454,#141455,#141456,#141457,#141458,#141459,#141460,#141461,#141462,
#141463,#141464,#141465,#141466,#141467,#141468,#141469,#141470),
 .UNSPECIFIED.,.F.,.F.,(4,3,3,3,3,3,3,3,3,3,3,3,3,3,3,3,3,3,3,3,3,3,3,3,
3,3,3,3,3,3,3,3,3,3,3,3,3,3,3,3,3,3,3,3,3,3,3,3,3,3,3,3,3,3,3,3,3,3,3,3,
3,3,3,3,3,3,3,3,3,3,3,3,3,3,3,3,3,3,3,4),(-255.180467741312,-255.101973116499,
-255.023538197481,-254.9451503052,-254.866796796049,-254.7858168324,-254.707481506871,
-254.6291405407,-254.550782482535,-254.472395872106,-254.393936405803,-254.315434389609,
-254.236847990182,-254.218957086855,-254.139965191516,-254.061073406842,
-253.982271150797,-253.903571149976,-253.824931704097,-253.746355421912,
-253.720488543547,-253.641901820383,-253.563265653119,-253.484569659802,
-253.405755628319,-253.326874200094,-253.247871106878,-253.222020000239,
-253.14294747849,-253.063947923755,-252.985009655931,-252.90612104145,-252.827270484893,
-252.748441980628,-252.669625606759,-252.590810855576,-252.511987221598,
-252.43311717405,-252.354223494975,-252.275262970138,-252.225082913624,
-252.150977475523,-252.076928977668,-252.002922239662,-251.92893297551,
-251.854955613898,-251.780953327865,-251.726614370317,-251.63561527058,
-251.544112052901,-251.452168513969,-251.360133936788,-251.268224846665,
-251.228145827009,-251.152436155892,-251.076775153867,-251.00114831353,
-250.925530617249,-250.849919117163,-250.774279192536,-250.729677283702,
-250.647398511848,-250.565095948984,-250.481624146836,-250.399269191937,
-250.315238966166,-250.231208740394,-250.148829729793,-250.066465540544,
-249.98303420468,-249.900712231388,-249.816726214238,-249.732740197087,
-249.657100291293,-249.581484716781,-249.50587900288,-249.43024848262,-249.35460320045,
-249.278904741001,-249.253903437549),.UNSPECIFIED.);
#3019=B_SPLINE_CURVE_WITH_KNOTS('',3,(#141476,#141477,#141478,#141479,#141480,
#141481,#141482,#141483,#141484,#141485,#141486,#141487,#141488,#141489,
#141490,#141491,#141492,#141493,#141494,#141495,#141496,#141497,#141498,
#141499,#141500,#141501,#141502,#141503,#141504,#141505,#141506,#141507,
#141508,#141509,#141510,#141511,#141512,#141513,#141514,#141515,#141516,
#141517,#141518,#141519,#141520,#141521,#141522,#141523,#141524,#141525,
#141526,#141527,#141528,#141529,#141530,#141531,#141532,#141533,#141534,
#141535,#141536,#141537,#141538,#141539,#141540,#141541,#141542,#141543,
#141544,#141545,#141546,#141547,#141548,#141549,#141550,#141551,#141552,
#141553,#141554,#141555,#141556,#141557,#141558,#141559,#141560,#141561,
#141562,#141563,#141564,#141565,#141566,#141567,#141568,#141569,#141570,
#141571,#141572,#141573,#141574,#141575,#141576,#141577,#141578,#141579,
#141580,#141581,#141582,#141583,#141584,#141585,#141586,#141587,#141588,
#141589,#141590,#141591,#141592,#141593,#141594,#141595,#141596,#141597,
#141598,#141599,#141600,#141601,#141602,#141603,#141604,#141605,#141606,
#141607,#141608,#141609,#141610,#141611,#141612,#141613,#141614,#141615,
#141616,#141617,#141618,#141619,#141620,#141621,#141622,#141623,#141624,
#141625,#141626,#141627,#141628,#141629,#141630,#141631,#141632,#141633,
#141634,#141635,#141636,#141637,#141638,#141639,#141640,#141641,#141642,
#141643,#141644,#141645,#141646,#141647,#141648,#141649,#141650,#141651,
#141652,#141653,#141654,#141655,#141656,#141657,#141658,#141659,#141660,
#141661,#141662,#141663,#141664,#141665,#141666,#141667,#141668,#141669,
#141670,#141671,#141672,#141673,#141674,#141675,#141676,#141677,#141678,
#141679,#141680,#141681,#141682,#141683,#141684,#141685,#141686,#141687,
#141688,#141689,#141690,#141691,#141692,#141693,#141694,#141695,#141696,
#141697,#141698,#141699,#141700,#141701,#141702,#141703,#141704,#141705,
#141706,#141707,#141708,#141709,#141710),.UNSPECIFIED.,.F.,.F.,(4,3,3,3,
3,3,3,3,3,3,3,3,3,3,3,3,3,3,3,3,3,3,3,3,3,3,3,3,3,3,3,3,3,3,3,3,3,3,3,3,
3,3,3,3,3,3,3,3,3,3,3,3,3,3,3,3,3,3,3,3,3,3,3,3,3,3,3,3,3,3,3,3,3,3,3,3,
3,3,4),(246.709703796838,246.741928937241,246.820515660405,246.899151827669,
246.977847820986,247.05666185247,247.135543280694,247.214546373911,247.240397480549,
247.319470002299,247.398469557034,247.477407824858,247.556296439339,247.635146995895,
247.71397550016,247.792791874029,247.871606625213,247.95043025919,248.029300306738,
248.108193985814,248.187154510651,248.237334567164,248.311440005265,248.385488503119,
248.459495241126,248.533484505278,248.60746186689,248.681464152923,248.735803110471,
248.826802210207,248.918305427884,249.010248966815,249.102283543994,249.194192634116,
249.234271653779,249.309981324897,249.385642326925,249.461269167263,249.536886863547,
249.612498363634,249.688138288263,249.732740197087,249.815018968939,249.897321531799,
249.980793333948,250.063148288844,250.147178514619,250.231208740394,250.313587750997,
250.395951940248,250.479383276112,250.561705249406,250.645691266554,250.729677283702,
250.805317392922,250.880933495828,250.95654006288,251.032174725589,251.107824284166,
251.183534573942,251.228145827009,251.320046396713,251.412079366429,251.503958936253,
251.595586332285,251.686607453767,251.726614370317,251.800616285004,251.874597213347,
251.948572235259,252.022584708558,252.096615978538,252.170720730742,252.225082913624,
252.31338252294,252.401525174677,252.489509903532,252.577143865673,252.636521978204),
 .UNSPECIFIED.);
#3020=B_SPLINE_CURVE_WITH_KNOTS('',3,(#141711,#141712,#141713,#141714,#141715,
#141716,#141717,#141718,#141719,#141720,#141721,#141722,#141723,#141724,
#141725,#141726),.UNSPECIFIED.,.F.,.F.,(4,3,3,3,3,4),(252.63652197832,252.716213408794,
252.795966776382,252.875752384699,252.955608181191,252.992365321722),
 .UNSPECIFIED.);
#3021=B_SPLINE_CURVE_WITH_KNOTS('',3,(#141728,#141729,#141730,#141731,#141732,
#141733,#141734,#141735,#141736,#141737,#141738,#141739,#141740,#141741,
#141742,#141743),.UNSPECIFIED.,.F.,.F.,(4,3,3,3,3,4),(-249.253903437549,
-249.234271653779,-249.139112369578,-249.043810942917,-248.94881027079,
-248.897282434214),.UNSPECIFIED.);
#3022=B_SPLINE_CURVE_WITH_KNOTS('',3,(#141744,#141745,#141746,#141747,#141748,
#141749,#141750,#141751,#141752,#141753,#141754,#141755,#141756,#141757,
#141758,#141759,#141760,#141761,#141762,#141763,#141764,#141765,#141766,
#141767,#141768,#141769,#141770,#141771,#141772,#141773,#141774,#141775,
#141776,#141777,#141778,#141779,#141780,#141781,#141782,#141783,#141784,
#141785,#141786,#141787,#141788,#141789,#141790,#141791,#141792,#141793,
#141794,#141795,#141796,#141797,#141798,#141799,#141800,#141801,#141802,
#141803,#141804,#141805,#141806,#141807,#141808,#141809,#141810,#141811,
#141812,#141813,#141814,#141815,#141816,#141817,#141818,#141819,#141820,
#141821,#141822,#141823,#141824,#141825,#141826,#141827,#141828,#141829,
#141830,#141831,#141832,#141833,#141834,#141835,#141836,#141837,#141838,
#141839,#141840,#141841,#141842,#141843,#141844,#141845,#141846,#141847,
#141848,#141849,#141850,#141851,#141852,#141853,#141854,#141855,#141856,
#141857,#141858,#141859,#141860,#141861,#141862,#141863,#141864,#141865,
#141866,#141867,#141868,#141869,#141870,#141871,#141872,#141873,#141874,
#141875,#141876,#141877,#141878,#141879,#141880,#141881,#141882,#141883,
#141884,#141885,#141886,#141887,#141888,#141889,#141890,#141891,#141892,
#141893,#141894,#141895,#141896,#141897,#141898,#141899,#141900,#141901,
#141902,#141903,#141904,#141905,#141906,#141907,#141908,#141909,#141910,
#141911,#141912,#141913,#141914,#141915,#141916,#141917,#141918,#141919,
#141920,#141921,#141922,#141923,#141924,#141925,#141926,#141927,#141928,
#141929,#141930,#141931,#141932,#141933,#141934,#141935,#141936,#141937,
#141938,#141939,#141940,#141941,#141942,#141943,#141944,#141945,#141946,
#141947,#141948,#141949,#141950,#141951,#141952,#141953,#141954,#141955,
#141956,#141957,#141958,#141959,#141960,#141961,#141962,#141963),
 .UNSPECIFIED.,.F.,.F.,(4,3,3,3,3,3,3,3,3,3,3,3,3,3,3,3,3,3,3,3,3,3,3,3,
3,3,3,3,3,3,3,3,3,3,3,3,3,3,3,3,3,3,3,3,3,3,3,3,3,3,3,3,3,3,3,3,3,3,3,3,
3,3,3,3,3,3,3,3,3,3,3,3,3,4),(-248.897282434214,-248.815552560448,-248.733822806678,
-248.652093171236,-248.570363652457,-248.488634248674,-248.406904958219,
-248.3219581897,-248.238338714439,-248.156025793479,-248.074286884412,-247.992548395025,
-247.910810318645,-247.829072648598,-247.747335378209,-247.665598500806,
-247.583862009716,-247.502125898266,-247.420390159784,-247.338654787598,
-247.256919775036,-247.175185115427,-247.093450802099,-247.011716828383,
-246.929983187607,-246.848249873102,-246.766516878198,-246.684784196225,
-246.603051820513,-246.521319744394,-246.439587961198,-246.357856464257,
-246.276125246904,-246.194394302469,-246.112663624285,-246.030933205684,
-245.949203039999,-245.867473120562,-245.785743440707,-245.704013993766,
-245.618585799367,-245.535827236043,-245.45408860848,-245.372350804676,
-245.290613797936,-245.208877561568,-245.127142068883,-245.045407293192,
-244.963673207811,-244.881939786059,-244.800207001254,-244.718474826718,
-244.636743235777,-244.555012201756,-244.473281697984,-244.391551697789,
-244.309822174504,-244.22610277441,-244.144364693382,-244.062628197957,
-243.980893181373,-243.899159536884,-243.817427157767,-243.735695937314,
-243.653965768834,-243.568509019354,-243.486772101135,-243.405038092231,
-243.323306565712,-243.241577094784,-243.159842204308,-243.078112124143,
-242.996380695082,-242.970311772993),.UNSPECIFIED.);
#3023=B_SPLINE_CURVE_WITH_KNOTS('',3,(#141969,#141970,#141971,#141972,#141973,
#141974,#141975,#141976,#141977,#141978,#141979,#141980,#141981,#141982,
#141983,#141984,#141985,#141986,#141987,#141988,#141989,#141990,#141991,
#141992,#141993,#141994,#141995,#141996,#141997,#141998,#141999,#142000,
#142001,#142002,#142003,#142004,#142005,#142006,#142007,#142008,#142009,
#142010,#142011,#142012,#142013,#142014,#142015,#142016,#142017,#142018,
#142019,#142020,#142021,#142022,#142023,#142024,#142025,#142026,#142027,
#142028,#142029,#142030,#142031,#142032,#142033,#142034,#142035,#142036,
#142037,#142038,#142039,#142040,#142041,#142042,#142043,#142044,#142045,
#142046,#142047,#142048,#142049,#142050,#142051,#142052,#142053,#142054,
#142055,#142056,#142057,#142058,#142059,#142060,#142061,#142062,#142063,
#142064,#142065,#142066,#142067,#142068,#142069,#142070,#142071,#142072,
#142073,#142074,#142075,#142076,#142077,#142078,#142079,#142080,#142081,
#142082,#142083,#142084,#142085,#142086,#142087,#142088,#142089,#142090,
#142091,#142092,#142093,#142094,#142095,#142096,#142097,#142098,#142099,
#142100,#142101,#142102,#142103,#142104,#142105,#142106,#142107,#142108,
#142109,#142110,#142111,#142112,#142113,#142114,#142115,#142116,#142117,
#142118,#142119,#142120,#142121,#142122,#142123,#142124,#142125,#142126,
#142127,#142128,#142129,#142130,#142131,#142132,#142133,#142134,#142135,
#142136,#142137,#142138,#142139,#142140,#142141,#142142,#142143,#142144,
#142145,#142146,#142147,#142148,#142149,#142150,#142151,#142152,#142153,
#142154,#142155,#142156,#142157,#142158,#142159,#142160,#142161,#142162,
#142163,#142164,#142165,#142166,#142167,#142168,#142169,#142170,#142171,
#142172,#142173,#142174,#142175,#142176,#142177,#142178,#142179,#142180,
#142181,#142182,#142183,#142184,#142185,#142186,#142187,#142188,#142189,
#142190,#142191,#142192,#142193,#142194,#142195,#142196,#142197,#142198,
#142199,#142200),.UNSPECIFIED.,.F.,.F.,(4,3,3,3,3,3,3,3,3,3,3,3,3,3,3,3,
3,3,3,3,3,3,3,3,3,3,3,3,3,3,3,3,3,3,3,3,3,3,3,3,3,3,3,3,3,3,3,3,3,3,3,3,
3,3,3,3,3,3,3,3,3,3,3,3,3,3,3,3,3,3,3,3,3,3,3,3,3,4),(240.426626170505,
240.505559763057,240.584444689868,240.663292543497,240.742119607048,240.820935434143,
240.899750532045,240.97857540635,241.057447086753,241.136343221325,241.215305082781,
241.258774960858,241.33288039896,241.406928896815,241.480935634822,241.554924898975,
241.628902260588,241.702904546621,241.757243504166,241.8482426039,241.939745821575,
242.031689360503,242.12372393768,242.215633027799,242.255712047473,242.331421718591,
242.407082720618,242.482709560957,242.55832725724,242.633938757327,242.709578681956,
242.754180590781,242.836459362633,242.918761925495,243.002233727643,243.08458868254,
243.168618908314,243.252649134088,243.335028144691,243.417392333942,243.500823669805,
243.583145643099,243.667131660248,243.751117677396,243.826757786617,243.902373889522,
243.977980456575,244.053615119284,244.129264677861,244.204974967637,244.249586220703,
244.341486790406,244.433519760121,244.525399329943,244.617026725973,244.708047847455,
244.748054764011,244.8220566787,244.896037607043,244.970012628957,245.044025102257,
245.118056372239,245.192161124444,245.246523307319,245.325484723266,245.404392146335,
245.483257185272,245.562091415997,245.640906389976,245.719727653636,245.798554292748,
245.877396817124,245.956265745707,246.035207797038,246.114188562527,246.193259573544,
246.243460393934,246.35333667114),.UNSPECIFIED.);
#3024=B_SPLINE_CURVE_WITH_KNOTS('',3,(#142201,#142202,#142203,#142204,#142205,
#142206,#142207,#142208,#142209,#142210,#142211,#142212,#142213,#142214,
#142215,#142216),.UNSPECIFIED.,.F.,.F.,(4,3,3,3,3,4),(246.353336671251,
246.429405639111,246.505380470581,246.581301005019,246.657176301325,246.709703796838),
 .UNSPECIFIED.);
#3025=B_SPLINE_CURVE_WITH_KNOTS('',3,(#142218,#142219,#142220,#142221,#142222,
#142223,#142224,#142225,#142226,#142227,#142228,#142229,#142230,#142231,
#142232,#142233),.UNSPECIFIED.,.F.,.F.,(4,3,3,3,3,4),(-242.970311772993,
-242.888582229157,-242.806847114238,-242.725116876889,-242.643385087938,
-242.614097127035),.UNSPECIFIED.);
#3026=B_SPLINE_CURVE_WITH_KNOTS('',3,(#142234,#142235,#142236,#142237,#142238,
#142239,#142240,#142241,#142242,#142243,#142244,#142245,#142246,#142247,
#142248,#142249,#142250,#142251,#142252,#142253,#142254,#142255,#142256,
#142257,#142258,#142259,#142260,#142261,#142262,#142263,#142264,#142265,
#142266,#142267,#142268,#142269,#142270,#142271,#142272,#142273,#142274,
#142275,#142276,#142277,#142278,#142279,#142280,#142281,#142282,#142283,
#142284,#142285,#142286,#142287,#142288,#142289,#142290,#142291,#142292,
#142293,#142294,#142295,#142296,#142297,#142298,#142299,#142300,#142301,
#142302,#142303,#142304,#142305,#142306,#142307,#142308,#142309,#142310,
#142311,#142312,#142313,#142314,#142315,#142316,#142317,#142318,#142319,
#142320,#142321,#142322,#142323,#142324,#142325,#142326,#142327,#142328,
#142329,#142330,#142331,#142332,#142333,#142334,#142335,#142336,#142337,
#142338,#142339,#142340,#142341,#142342,#142343,#142344,#142345,#142346,
#142347,#142348,#142349,#142350,#142351,#142352,#142353,#142354,#142355,
#142356,#142357,#142358,#142359,#142360,#142361,#142362,#142363,#142364,
#142365,#142366,#142367,#142368,#142369,#142370,#142371,#142372,#142373,
#142374,#142375,#142376,#142377,#142378,#142379,#142380,#142381,#142382,
#142383,#142384,#142385,#142386,#142387,#142388,#142389,#142390,#142391,
#142392,#142393,#142394,#142395,#142396,#142397,#142398,#142399,#142400,
#142401,#142402,#142403,#142404,#142405,#142406,#142407,#142408,#142409,
#142410,#142411,#142412,#142413,#142414,#142415,#142416,#142417,#142418,
#142419,#142420,#142421,#142422,#142423,#142424,#142425,#142426,#142427,
#142428,#142429,#142430,#142431,#142432,#142433,#142434,#142435,#142436,
#142437,#142438,#142439,#142440,#142441,#142442,#142443,#142444,#142445,
#142446,#142447,#142448,#142449,#142450,#142451,#142452,#142453,#142454,
#142455,#142456,#142457,#142458,#142459,#142460,#142461,#142462,#142463,
#142464,#142465,#142466,#142467,#142468,#142469,#142470,#142471),
 .UNSPECIFIED.,.F.,.F.,(4,3,3,3,3,3,3,3,3,3,3,3,3,3,3,3,3,3,3,3,3,3,3,3,
3,3,3,3,3,3,3,3,3,3,3,3,3,3,3,3,3,3,3,3,3,3,3,3,3,3,3,3,3,3,3,3,3,3,3,3,
3,3,3,3,3,3,3,3,3,3,3,3,3,3,3,3,3,3,3,4),(-242.614097127035,-242.53872344443,
-242.463324904272,-242.387914432477,-242.3124425137,-242.255712047473,-242.163811477774,
-242.071778508064,-241.979898938246,-241.88827154222,-241.797250420742,
-241.757243504166,-241.683241589477,-241.609260661133,-241.53528563922,
-241.461273165919,-241.387241895937,-241.313137143731,-241.258774960858,
-241.179813544911,-241.100906121842,-241.022041082906,-240.94320685218,
-240.864391878201,-240.785570614541,-240.706743975429,-240.627901451053,
-240.54903252247,-240.470090471139,-240.391109705651,-240.312038694633,
-240.261837874243,-240.182845978904,-240.103954194229,-240.025151938184,
-239.946451937363,-239.867812491484,-239.789236209298,-239.763369330935,
-239.684782607772,-239.606146440509,-239.527450447193,-239.448636415711,
-239.369754987488,-239.290751894272,-239.264900787628,-239.185828265879,
-239.106828711144,-239.02789044332,-238.949001828839,-238.870151272282,
-238.791322768017,-238.712506394148,-238.633691642964,-238.554868008987,
-238.475997961439,-238.397104282363,-238.318143757526,-238.267963701013,
-238.19385826291,-238.119809765055,-238.045803027048,-237.971813762894,
-237.897836401282,-237.823834115248,-237.769495157705,-237.678496057971,
-237.586992840297,-237.495049301369,-237.403014724192,-237.311105634074,
-237.271026614398,-237.19531694328,-237.119655941254,-237.044029100915,
-236.968411404632,-236.892799904545,-236.817159979917,-236.77255807109,
-236.687327340016),.UNSPECIFIED.);
#3027=B_SPLINE_CURVE_WITH_KNOTS('',3,(#142477,#142478,#142479,#142480,#142481,
#142482,#142483,#142484,#142485,#142486,#142487,#142488,#142489,#142490,
#142491,#142492,#142493,#142494,#142495,#142496,#142497,#142498,#142499,
#142500,#142501,#142502,#142503,#142504,#142505,#142506,#142507,#142508,
#142509,#142510,#142511,#142512,#142513,#142514,#142515,#142516,#142517,
#142518,#142519,#142520,#142521,#142522,#142523,#142524,#142525,#142526,
#142527,#142528,#142529,#142530,#142531,#142532,#142533,#142534,#142535,
#142536,#142537,#142538,#142539,#142540,#142541,#142542,#142543,#142544,
#142545,#142546,#142547,#142548,#142549,#142550,#142551,#142552,#142553,
#142554,#142555,#142556,#142557,#142558,#142559,#142560,#142561,#142562,
#142563,#142564,#142565,#142566,#142567,#142568,#142569,#142570,#142571,
#142572,#142573,#142574,#142575,#142576,#142577,#142578,#142579,#142580,
#142581,#142582,#142583,#142584,#142585,#142586,#142587,#142588,#142589,
#142590,#142591,#142592,#142593,#142594,#142595,#142596,#142597,#142598,
#142599,#142600,#142601,#142602,#142603,#142604,#142605,#142606,#142607,
#142608,#142609,#142610,#142611,#142612,#142613,#142614,#142615,#142616,
#142617,#142618,#142619,#142620,#142621,#142622,#142623,#142624,#142625,
#142626,#142627,#142628,#142629,#142630,#142631,#142632,#142633,#142634,
#142635,#142636,#142637,#142638,#142639,#142640,#142641,#142642,#142643,
#142644,#142645,#142646,#142647,#142648,#142649,#142650,#142651,#142652,
#142653,#142654,#142655,#142656,#142657,#142658,#142659,#142660,#142661,
#142662,#142663,#142664,#142665,#142666,#142667,#142668,#142669,#142670,
#142671,#142672,#142673,#142674,#142675,#142676,#142677,#142678,#142679,
#142680,#142681,#142682,#142683,#142684,#142685,#142686,#142687,#142688,
#142689,#142690,#142691,#142692,#142693,#142694,#142695,#142696,#142697,
#142698,#142699,#142700,#142701,#142702,#142703,#142704,#142705,#142706,
#142707,#142708,#142709,#142710,#142711),.UNSPECIFIED.,.F.,.F.,(4,3,3,3,
3,3,3,3,3,3,3,3,3,3,3,3,3,3,3,3,3,3,3,3,3,3,3,3,3,3,3,3,3,3,3,3,3,3,3,3,
3,3,3,3,3,3,3,3,3,3,3,3,3,3,3,3,3,3,3,3,3,3,3,3,3,3,3,3,3,3,3,3,3,3,3,3,
3,3,4),(234.143309340879,234.227320887716,234.280215354552,234.354320792655,
234.42836929051,234.502376028518,234.576365292671,234.650342654284,234.724344940318,
234.77868389786,234.869682997594,234.961186215269,235.053129754197,235.145164331373,
235.237073421492,235.277152441167,235.352862112285,235.428523114311,235.504149954649,
235.579767650931,235.655379151018,235.731019075646,235.775620984475,235.857899756329,
235.940202319193,236.023674121341,236.10602907624,236.190059302011,236.274089527783,
236.356468538383,236.438832727631,236.522264063496,236.604586036787,236.688572053938,
236.77255807109,236.848198180312,236.923814283219,236.999420850274,237.075055512984,
237.150705071563,237.226415361341,237.271026614398,237.362927184098,237.45496015381,
237.54683972363,237.638467119658,237.729488241138,237.769495157705,237.843497072394,
237.917478000738,237.991453022651,238.065465495951,238.139496765933,238.213601518138,
238.267963701013,238.34692511696,238.42583254003,238.504697578966,238.583531809693,
238.662346783672,238.741168047332,238.819994686445,238.898837210821,238.977706139405,
239.056648190736,239.135628956225,239.214699967243,239.264900787628,239.343892682965,
239.422784467639,239.501586723681,239.580286724501,239.658926170379,239.737502452563,
239.763369330935,239.84006483917,239.914714461518,239.992432912695,240.070151363873),
 .UNSPECIFIED.);
#3028=B_SPLINE_CURVE_WITH_KNOTS('',3,(#142712,#142713,#142714,#142715,#142716,
#142717,#142718,#142719,#142720,#142721,#142722,#142723,#142724),
 .UNSPECIFIED.,.F.,.F.,(4,3,3,3,4),(240.070151363961,240.165994619102,240.261837874243,
240.344232022374,240.426626170505),.UNSPECIFIED.);
#3029=B_SPLINE_CURVE_WITH_KNOTS('',3,(#142726,#142727,#142728,#142729,#142730,
#142731,#142732,#142733,#142734,#142735,#142736,#142737,#142738,#142739,
#142740,#142741),.UNSPECIFIED.,.F.,.F.,(4,3,3,3,3,4),(-236.687327340016,
-236.605018875511,-236.522672705988,-236.440315080971,-236.35793754469,
-236.330911819855),.UNSPECIFIED.);
#3030=B_SPLINE_CURVE_WITH_KNOTS('',3,(#142742,#142743,#142744,#142745,#142746,
#142747,#142748,#142749,#142750,#142751,#142752,#142753,#142754,#142755,
#142756,#142757,#142758,#142759,#142760,#142761,#142762,#142763,#142764,
#142765,#142766,#142767,#142768,#142769,#142770,#142771,#142772,#142773,
#142774,#142775,#142776,#142777,#142778,#142779,#142780,#142781,#142782,
#142783,#142784,#142785,#142786,#142787,#142788,#142789,#142790,#142791,
#142792,#142793,#142794,#142795,#142796,#142797,#142798,#142799,#142800,
#142801,#142802,#142803,#142804,#142805,#142806,#142807,#142808,#142809,
#142810,#142811,#142812,#142813,#142814,#142815,#142816,#142817,#142818,
#142819,#142820,#142821,#142822,#142823,#142824,#142825,#142826,#142827,
#142828,#142829,#142830,#142831,#142832,#142833,#142834,#142835,#142836,
#142837,#142838,#142839,#142840,#142841,#142842,#142843,#142844,#142845,
#142846,#142847,#142848,#142849,#142850,#142851,#142852,#142853,#142854,
#142855,#142856,#142857,#142858,#142859,#142860,#142861,#142862,#142863,
#142864,#142865,#142866,#142867,#142868,#142869,#142870,#142871,#142872,
#142873,#142874,#142875,#142876,#142877,#142878,#142879,#142880,#142881,
#142882,#142883,#142884,#142885,#142886,#142887,#142888,#142889,#142890,
#142891,#142892,#142893,#142894,#142895,#142896,#142897,#142898,#142899,
#142900,#142901,#142902,#142903,#142904,#142905,#142906,#142907,#142908,
#142909,#142910,#142911,#142912,#142913,#142914,#142915,#142916,#142917,
#142918,#142919,#142920,#142921,#142922,#142923,#142924,#142925,#142926,
#142927,#142928,#142929,#142930,#142931,#142932,#142933,#142934,#142935,
#142936,#142937,#142938,#142939,#142940,#142941,#142942,#142943,#142944,
#142945,#142946,#142947,#142948,#142949,#142950,#142951,#142952,#142953,
#142954,#142955,#142956,#142957,#142958,#142959,#142960,#142961,#142962,
#142963,#142964,#142965,#142966,#142967,#142968,#142969,#142970,#142971,
#142972,#142973,#142974,#142975,#142976,#142977,#142978,#142979),
 .UNSPECIFIED.,.F.,.F.,(4,3,3,3,3,3,3,3,3,3,3,3,3,3,3,3,3,3,3,3,3,3,3,3,
3,3,3,3,3,3,3,3,3,3,3,3,3,3,3,3,3,3,3,3,3,3,3,3,3,3,3,3,3,3,3,3,3,3,3,3,
3,3,3,3,3,3,3,3,3,3,3,3,3,3,3,3,3,3,3,4),(-236.330911819752,-236.274089527782,
-236.191710517193,-236.109346327957,-236.025914992087,-235.943593018808,
-235.859607001641,-235.775620984475,-235.69998087525,-235.62436477234,-235.548758205282,
-235.473123542569,-235.397473983987,-235.321763694207,-235.277152441167,
-235.185251871468,-235.093218901759,-235.001339331941,-234.909711935916,
-234.818690814438,-234.77868389786,-234.704681983171,-234.630701054827,
-234.556726032914,-234.482713559614,-234.408682289632,-234.334577537427,
-234.280215354552,-234.201253938605,-234.122346515535,-234.043481476598,
-233.964647245872,-233.885832271893,-233.807011008233,-233.728184369121,
-233.649341844744,-233.570472916161,-233.491530864829,-233.412550099341,
-233.333479088322,-233.283278267937,-233.2042863726,-233.125394587926,-233.046592331883,
-232.967892331062,-232.889252885185,-232.810676603001,-232.78480972463,
-232.706223001466,-232.627586834202,-232.548890840884,-232.470076809401,
-232.391195381176,-232.312192287959,-232.286341181322,-232.207268659573,
-232.128269104838,-232.049330837014,-231.970442222533,-231.891591665977,
-231.812763161711,-231.733946787842,-231.655132036659,-231.576308402681,
-231.497438355133,-231.418544676057,-231.339584151221,-231.289404094707,
-231.215298656605,-231.14125015875,-231.067243420743,-230.99325415659,-230.919276794977,
-230.845274508944,-230.790935551399,-230.700035430836,-230.608423997618,
-230.516541195554,-230.424506658068,-230.403871264419),.UNSPECIFIED.);
#3031=B_SPLINE_CURVE_WITH_KNOTS('',3,(#142985,#142986,#142987,#142988,#142989,
#142990,#142991,#142992,#142993,#142994,#142995,#142996,#142997,#142998,
#142999,#143000,#143001,#143002,#143003,#143004,#143005,#143006,#143007,
#143008,#143009,#143010,#143011,#143012,#143013,#143014,#143015,#143016,
#143017,#143018,#143019,#143020,#143021,#143022,#143023,#143024,#143025,
#143026,#143027,#143028,#143029,#143030,#143031,#143032,#143033,#143034,
#143035,#143036,#143037,#143038,#143039,#143040,#143041,#143042,#143043,
#143044,#143045,#143046,#143047,#143048,#143049,#143050,#143051,#143052,
#143053,#143054,#143055,#143056,#143057,#143058,#143059,#143060,#143061,
#143062,#143063,#143064,#143065,#143066,#143067,#143068,#143069,#143070,
#143071,#143072,#143073,#143074,#143075,#143076,#143077,#143078,#143079,
#143080,#143081,#143082,#143083,#143084,#143085,#143086,#143087,#143088,
#143089,#143090,#143091,#143092,#143093,#143094,#143095,#143096,#143097,
#143098,#143099,#143100,#143101,#143102,#143103,#143104,#143105,#143106,
#143107,#143108,#143109,#143110,#143111,#143112,#143113,#143114,#143115,
#143116,#143117,#143118,#143119,#143120,#143121,#143122,#143123,#143124,
#143125,#143126,#143127,#143128,#143129,#143130,#143131,#143132,#143133,
#143134,#143135,#143136,#143137,#143138,#143139,#143140,#143141,#143142,
#143143,#143144,#143145,#143146,#143147,#143148,#143149,#143150,#143151,
#143152,#143153,#143154,#143155,#143156,#143157,#143158,#143159,#143160,
#143161,#143162,#143163,#143164,#143165,#143166,#143167,#143168,#143169,
#143170,#143171,#143172,#143173,#143174,#143175,#143176,#143177,#143178,
#143179,#143180,#143181,#143182,#143183,#143184,#143185,#143186,#143187,
#143188,#143189,#143190,#143191,#143192,#143193,#143194,#143195,#143196,
#143197,#143198,#143199,#143200,#143201,#143202,#143203,#143204,#143205,
#143206,#143207,#143208,#143209,#143210,#143211,#143212,#143213,#143214,
#143215,#143216,#143217,#143218,#143219),.UNSPECIFIED.,.F.,.F.,(4,3,3,3,
3,3,3,3,3,3,3,3,3,3,3,3,3,3,3,3,3,3,3,3,3,3,3,3,3,3,3,3,3,3,3,3,3,3,3,3,
3,3,3,3,3,3,3,3,3,3,3,3,3,3,3,3,3,3,3,3,3,3,3,3,3,3,3,3,3,3,3,3,3,3,3,3,
3,3,4),(227.859336579383,227.950680999062,228.042561426182,228.134579702056,
228.226520588781,228.298592834862,228.374302505979,228.449963508003,228.52559034834,
228.601208044621,228.676819544707,228.752459469334,228.797061378169,228.879340150024,
228.961642712888,229.045114515035,229.127469469934,229.211499695706,229.295529921477,
229.377908932078,229.460273121326,229.543704457191,229.626026430483,229.710012447633,
229.793998464784,229.869638574006,229.945254676912,230.020861243967,230.096495906677,
230.172145465256,230.247855755033,230.292467008092,230.384367577794,230.476400547506,
230.568280117326,230.659907513352,230.750928634833,230.790935551399,230.864937466087,
230.938918394431,231.012893416344,231.086905889644,231.160937159626,231.235041911832,
231.289404094707,231.368365510654,231.447272933724,231.52613797266,231.604972203387,
231.683787177365,231.762608441025,231.841435080137,231.920277604514,231.999146533096,
232.078088584428,232.157069349917,232.236140360935,232.286341181322,232.365333076661,
232.444224861336,232.523027117381,232.601727118202,232.68036656408,232.758942846266,
232.78480972463,232.863396447793,232.942032615055,233.02072860837,233.099542639852,
233.178424068074,233.257427161289,233.283278267937,233.365646306409,233.447916375147,
233.532678795556,233.614707660166,233.700836858474,233.782651577588,233.786966056781),
 .UNSPECIFIED.);
#3032=B_SPLINE_CURVE_WITH_KNOTS('',3,(#143220,#143221,#143222,#143223,#143224,
#143225,#143226,#143227,#143228,#143229,#143230,#143231,#143232,#143233,
#143234,#143235),.UNSPECIFIED.,.F.,.F.,(4,3,3,3,3,4),(233.786966674316,
233.870479334874,233.954172167115,234.0379522201,234.121843783026,234.143309340879),
 .UNSPECIFIED.);
#3033=B_SPLINE_CURVE_WITH_KNOTS('',3,(#143237,#143238,#143239,#143240,#143241,
#143242,#143243,#143244,#143245,#143246,#143247,#143248,#143249,#143250,
#143251,#143252,#143253,#143254,#143255),.UNSPECIFIED.,.F.,.F.,(4,3,3,3,
3,3,4),(-230.403871264419,-230.311987089053,-230.292467008092,-230.215986240579,
-230.139557082451,-230.063172142902,-230.047726512675),.UNSPECIFIED.);
#3034=B_SPLINE_CURVE_WITH_KNOTS('',3,(#143256,#143257,#143258,#143259,#143260,
#143261,#143262,#143263,#143264,#143265,#143266,#143267,#143268,#143269,
#143270,#143271,#143272,#143273,#143274,#143275,#143276,#143277,#143278,
#143279,#143280,#143281,#143282,#143283,#143284,#143285,#143286,#143287,
#143288,#143289,#143290,#143291,#143292,#143293,#143294,#143295,#143296,
#143297,#143298,#143299,#143300,#143301,#143302,#143303,#143304,#143305,
#143306,#143307,#143308,#143309,#143310,#143311,#143312,#143313,#143314,
#143315,#143316,#143317,#143318,#143319,#143320,#143321,#143322,#143323,
#143324,#143325,#143326,#143327,#143328,#143329,#143330,#143331,#143332,
#143333,#143334,#143335,#143336,#143337,#143338,#143339,#143340,#143341,
#143342,#143343,#143344,#143345,#143346,#143347,#143348,#143349,#143350,
#143351,#143352,#143353,#143354,#143355,#143356,#143357,#143358,#143359,
#143360,#143361,#143362,#143363,#143364,#143365,#143366,#143367,#143368,
#143369,#143370,#143371,#143372,#143373,#143374,#143375,#143376,#143377,
#143378,#143379,#143380,#143381,#143382,#143383,#143384,#143385,#143386,
#143387,#143388,#143389,#143390,#143391,#143392,#143393,#143394,#143395,
#143396,#143397,#143398,#143399,#143400,#143401,#143402,#143403,#143404,
#143405,#143406,#143407,#143408,#143409,#143410,#143411,#143412,#143413,
#143414,#143415,#143416,#143417,#143418,#143419,#143420,#143421,#143422,
#143423,#143424,#143425,#143426,#143427,#143428,#143429,#143430,#143431,
#143432,#143433,#143434,#143435,#143436,#143437,#143438,#143439,#143440,
#143441,#143442,#143443,#143444,#143445,#143446,#143447,#143448,#143449,
#143450,#143451,#143452,#143453,#143454,#143455,#143456,#143457,#143458,
#143459,#143460,#143461,#143462,#143463,#143464,#143465,#143466,#143467,
#143468,#143469,#143470,#143471,#143472,#143473,#143474,#143475),
 .UNSPECIFIED.,.F.,.F.,(4,3,3,3,3,3,3,3,3,3,3,3,3,3,3,3,3,3,3,3,3,3,3,3,
3,3,3,3,3,3,3,3,3,3,3,3,3,3,3,3,3,3,3,3,3,3,3,3,3,3,3,3,3,3,3,3,3,3,3,3,
3,3,3,3,3,3,3,3,3,3,3,3,3,4),(-230.047726512675,-229.965996638909,-229.884266885139,
-229.802537249697,-229.720807730918,-229.639078327135,-229.557349036681,
-229.472402268161,-229.3887827929,-229.30646987194,-229.224730962873,-229.142992473487,
-229.061254397107,-228.979516727059,-228.897779456671,-228.816042579268,
-228.734306088178,-228.652569976728,-228.570834238246,-228.489098866059,
-228.407363853497,-228.325629193888,-228.243894880561,-228.162160906845,
-228.080427266069,-227.998693951564,-227.91696095666,-227.835228274686,
-227.753495898974,-227.671763822855,-227.59003203966,-227.508300542719,
-227.426569325366,-227.344838380931,-227.263107702746,-227.181377284145,
-227.09964711846,-227.017917199024,-226.936187519169,-226.854458072228,
-226.769029877829,-226.686271314505,-226.604532686942,-226.522794883138,
-226.441057876398,-226.35932164003,-226.277586147345,-226.195851371654,
-226.114117286273,-226.032383864521,-225.950651079716,-225.86891890518,
-225.787187314239,-225.705456280218,-225.623725776446,-225.541995776251,
-225.460266252966,-225.376546852872,-225.294808771843,-225.213072276419,
-225.131337259834,-225.049603615346,-224.967871236229,-224.886140015776,
-224.804409847296,-224.718953097815,-224.637216179596,-224.555482170693,
-224.473750644174,-224.392021173245,-224.310286282769,-224.228556202604,
-224.146824773543,-224.120755851454),.UNSPECIFIED.);
#3035=B_SPLINE_CURVE_WITH_KNOTS('',3,(#143481,#143482,#143483,#143484,#143485,
#143486,#143487,#143488,#143489,#143490,#143491,#143492,#143493,#143494,
#143495,#143496,#143497,#143498,#143499,#143500,#143501,#143502,#143503,
#143504,#143505,#143506,#143507,#143508,#143509,#143510,#143511,#143512,
#143513,#143514,#143515,#143516,#143517,#143518,#143519,#143520,#143521,
#143522,#143523,#143524,#143525,#143526,#143527,#143528,#143529,#143530,
#143531,#143532,#143533,#143534,#143535,#143536,#143537,#143538,#143539,
#143540,#143541,#143542,#143543,#143544,#143545,#143546,#143547,#143548,
#143549,#143550,#143551,#143552,#143553,#143554,#143555,#143556,#143557,
#143558,#143559,#143560,#143561,#143562,#143563,#143564,#143565,#143566,
#143567,#143568,#143569,#143570,#143571,#143572,#143573,#143574,#143575,
#143576,#143577,#143578,#143579,#143580,#143581,#143582,#143583,#143584,
#143585,#143586,#143587,#143588,#143589,#143590,#143591,#143592,#143593,
#143594,#143595,#143596,#143597,#143598,#143599,#143600,#143601,#143602,
#143603,#143604,#143605,#143606,#143607,#143608,#143609,#143610,#143611,
#143612,#143613,#143614,#143615,#143616,#143617,#143618,#143619,#143620,
#143621,#143622,#143623,#143624,#143625,#143626,#143627,#143628,#143629,
#143630,#143631,#143632,#143633,#143634,#143635,#143636,#143637,#143638,
#143639,#143640,#143641,#143642,#143643,#143644,#143645,#143646,#143647,
#143648,#143649,#143650,#143651,#143652,#143653,#143654,#143655,#143656,
#143657,#143658,#143659,#143660,#143661,#143662,#143663,#143664,#143665,
#143666,#143667,#143668,#143669,#143670,#143671,#143672,#143673,#143674,
#143675,#143676,#143677,#143678,#143679,#143680,#143681,#143682,#143683,
#143684,#143685,#143686,#143687,#143688,#143689,#143690,#143691,#143692,
#143693,#143694,#143695,#143696,#143697,#143698,#143699,#143700,#143701,
#143702,#143703,#143704,#143705,#143706,#143707,#143708,#143709,#143710,
#143711,#143712,#143713,#143714,#143715,#143716,#143717,#143718),
 .UNSPECIFIED.,.F.,.F.,(4,3,3,3,3,3,3,3,3,3,3,3,3,3,3,3,3,3,3,3,3,3,3,3,
3,3,3,3,3,3,3,3,3,3,3,3,3,3,3,3,3,3,3,3,3,3,3,3,3,3,3,3,3,3,3,3,3,3,3,3,
3,3,3,3,3,3,3,3,3,3,3,3,3,3,3,3,3,3,3,4),(221.577058603984,221.652672288649,
221.728284922499,221.80392501773,221.818501771863,221.900780543719,221.983083106584,
222.066554908731,222.148909863632,222.232940089401,222.316970315171,222.399349325771,
222.481713515019,222.565144850884,222.647466824175,222.731452841327,222.815438858478,
222.891078967699,222.966695070606,223.04230163766,223.117936300369,223.193585858948,
223.269296148725,223.313907401786,223.405807971491,223.497840941208,223.589720511032,
223.681347907064,223.772369028547,223.812375945094,223.886377859781,223.960358788123,
224.034333810035,224.108346283333,224.182377553314,224.256482305518,224.310844488401,
224.389805904348,224.468713327418,224.547578366354,224.62641259708,224.705227571059,
224.78404883472,224.862875473832,224.941717998208,225.020586926792,225.099528978123,
225.178509743612,225.25758075463,225.307781575016,225.386773470355,225.46566525503,
225.544467511075,225.623167511897,225.701806957777,225.780383239963,225.806250118324,
225.884836841487,225.963473008749,226.042169002064,226.120983033547,226.199864461769,
226.278867554984,226.304718661631,226.383791183381,226.462790738116,226.54172900594,
226.620617620421,226.699468176978,226.778296681244,226.857113055113,226.935927806296,
227.014751440274,227.093621487822,227.172515166897,227.251475691734,227.301655748246,
227.384641264441,227.467394863404,227.503780749601),.UNSPECIFIED.);
#3036=B_SPLINE_CURVE_WITH_KNOTS('',3,(#143719,#143720,#143721,#143722,#143723,
#143724,#143725,#143726,#143727,#143728,#143729,#143730,#143731,#143732,
#143733,#143734,#143735,#143736,#143737),.UNSPECIFIED.,.F.,.F.,(4,3,3,3,
3,3,4),(227.503780749711,227.577866635172,227.648878133573,227.719884644627,
227.790914707643,227.800124291554,227.859336579383),.UNSPECIFIED.);
#3037=B_SPLINE_CURVE_WITH_KNOTS('',3,(#143739,#143740,#143741,#143742,#143743,
#143744,#143745,#143746,#143747,#143748,#143749,#143750,#143751,#143752,
#143753,#143754),.UNSPECIFIED.,.F.,.F.,(4,3,3,3,3,4),(-224.120755851454,
-224.039026307618,-223.957291192699,-223.87556095535,-223.793829166399,
-223.764541205496),.UNSPECIFIED.);
#3038=B_SPLINE_CURVE_WITH_KNOTS('',3,(#143755,#143756,#143757,#143758,#143759,
#143760,#143761,#143762,#143763,#143764,#143765,#143766,#143767,#143768,
#143769,#143770,#143771,#143772,#143773,#143774,#143775,#143776,#143777,
#143778,#143779,#143780,#143781,#143782,#143783,#143784,#143785,#143786,
#143787,#143788,#143789,#143790,#143791,#143792,#143793,#143794,#143795,
#143796,#143797,#143798,#143799,#143800,#143801,#143802,#143803,#143804,
#143805,#143806,#143807,#143808,#143809,#143810,#143811,#143812,#143813,
#143814,#143815,#143816,#143817,#143818,#143819,#143820,#143821,#143822,
#143823,#143824,#143825,#143826,#143827,#143828,#143829,#143830,#143831,
#143832,#143833,#143834,#143835,#143836,#143837,#143838,#143839,#143840,
#143841,#143842,#143843,#143844,#143845,#143846,#143847,#143848,#143849,
#143850,#143851,#143852,#143853,#143854,#143855,#143856,#143857,#143858,
#143859,#143860,#143861,#143862,#143863,#143864,#143865,#143866,#143867,
#143868,#143869,#143870,#143871,#143872,#143873,#143874,#143875,#143876,
#143877,#143878,#143879,#143880,#143881,#143882,#143883,#143884,#143885,
#143886,#143887,#143888,#143889,#143890,#143891,#143892,#143893,#143894,
#143895,#143896,#143897,#143898,#143899,#143900,#143901,#143902,#143903,
#143904,#143905,#143906,#143907,#143908,#143909,#143910,#143911,#143912,
#143913,#143914,#143915,#143916,#143917,#143918,#143919,#143920,#143921,
#143922,#143923,#143924,#143925,#143926,#143927,#143928,#143929,#143930,
#143931,#143932,#143933,#143934,#143935,#143936,#143937,#143938,#143939,
#143940,#143941,#143942,#143943,#143944,#143945,#143946,#143947,#143948,
#143949,#143950,#143951,#143952,#143953,#143954,#143955,#143956,#143957,
#143958,#143959,#143960,#143961,#143962,#143963,#143964,#143965,#143966,
#143967,#143968,#143969,#143970,#143971,#143972,#143973,#143974,#143975,
#143976,#143977,#143978,#143979,#143980,#143981,#143982,#143983,#143984,
#143985,#143986,#143987,#143988,#143989),.UNSPECIFIED.,.F.,.F.,(4,3,3,3,
3,3,3,3,3,3,3,3,3,3,3,3,3,3,3,3,3,3,3,3,3,3,3,3,3,3,3,3,3,3,3,3,3,3,3,3,
3,3,3,3,3,3,3,3,3,3,3,3,3,3,3,3,3,3,3,3,3,3,3,3,3,3,3,3,3,3,3,3,3,3,3,3,
3,3,4),(-223.764541205496,-223.672803714405,-223.580435572842,-223.487896573484,
-223.395424020174,-223.313907401786,-223.238197730668,-223.162536728641,
-223.086909888302,-223.011292192019,-222.935680691932,-222.860040767303,
-222.815438858478,-222.733160086626,-222.650857523765,-222.567385721616,
-222.48503076672,-222.401000540945,-222.316970315171,-222.234591304568,
-222.152227115317,-222.068795779453,-221.986473806159,-221.902487789011,
-221.818501771863,-221.742861662642,-221.667245559737,-221.591638992684,
-221.516004329975,-221.440354771398,-221.364644481622,-221.320033228556,
-221.228132658852,-221.136099689136,-221.044220119313,-220.952592723282,
-220.861571601799,-220.821564685248,-220.74756277056,-220.673581842218,
-220.599606820306,-220.525594347006,-220.451563077025,-220.377458324821,
-220.323096141941,-220.244134725994,-220.165227302924,-220.086362263987,
-220.007528033261,-219.928713059282,-219.849891795622,-219.771065156509,
-219.692222632132,-219.613353703549,-219.534411652218,-219.455430886729,
-219.37635987571,-219.326159055325,-219.247167159987,-219.168275375312,
-219.089473119268,-219.010773118447,-218.932133672568,-218.853557390383,
-218.827690512018,-218.749103788854,-218.670467621591,-218.591771628275,
-218.512957596792,-218.434076168568,-218.355073075352,-218.32922196871,
-218.251485982939,-218.173821811482,-218.096216627412,-218.018663395878,
-217.941140397265,-217.863632607374,-217.837561537579),.UNSPECIFIED.);
#3039=B_SPLINE_CURVE_WITH_KNOTS('',3,(#143995,#143996,#143997,#143998,#143999,
#144000,#144001,#144002,#144003,#144004,#144005,#144006,#144007,#144008,
#144009,#144010,#144011,#144012,#144013,#144014,#144015,#144016,#144017,
#144018,#144019,#144020,#144021,#144022,#144023,#144024,#144025,#144026,
#144027,#144028,#144029,#144030,#144031,#144032,#144033,#144034,#144035,
#144036,#144037,#144038,#144039,#144040,#144041,#144042,#144043,#144044,
#144045,#144046,#144047,#144048,#144049,#144050,#144051,#144052,#144053,
#144054,#144055,#144056,#144057,#144058,#144059,#144060,#144061,#144062,
#144063,#144064,#144065,#144066,#144067,#144068,#144069,#144070,#144071,
#144072,#144073,#144074,#144075,#144076,#144077,#144078,#144079,#144080,
#144081,#144082,#144083,#144084,#144085,#144086,#144087,#144088,#144089,
#144090,#144091,#144092,#144093,#144094,#144095,#144096,#144097,#144098,
#144099,#144100,#144101,#144102,#144103,#144104,#144105,#144106,#144107,
#144108,#144109,#144110,#144111,#144112,#144113,#144114,#144115,#144116,
#144117,#144118,#144119,#144120,#144121,#144122,#144123,#144124,#144125,
#144126,#144127,#144128,#144129,#144130,#144131,#144132,#144133,#144134,
#144135,#144136,#144137,#144138,#144139,#144140,#144141,#144142,#144143,
#144144,#144145,#144146,#144147,#144148,#144149,#144150,#144151,#144152,
#144153,#144154,#144155,#144156,#144157,#144158,#144159,#144160,#144161,
#144162,#144163,#144164,#144165,#144166,#144167,#144168,#144169,#144170,
#144171,#144172,#144173,#144174,#144175,#144176,#144177,#144178,#144179,
#144180,#144181,#144182,#144183,#144184,#144185,#144186,#144187,#144188,
#144189,#144190,#144191,#144192,#144193,#144194,#144195,#144196,#144197,
#144198,#144199,#144200,#144201,#144202,#144203,#144204,#144205,#144206,
#144207,#144208,#144209,#144210,#144211,#144212,#144213,#144214,#144215,
#144216,#144217,#144218,#144219,#144220,#144221,#144222,#144223,#144224,
#144225,#144226,#144227,#144228,#144229,#144230,#144231,#144232),
 .UNSPECIFIED.,.F.,.F.,(4,3,3,3,3,3,3,3,3,3,3,3,3,3,3,3,3,3,3,3,3,3,3,3,
3,3,3,3,3,3,3,3,3,3,3,3,3,3,3,3,3,3,3,3,3,3,3,3,3,3,3,3,3,3,3,3,3,3,3,3,
3,3,3,3,3,3,3,3,3,3,3,3,3,3,3,3,3,3,3,4),(215.293584957643,215.338410708865,
215.420789719468,215.503153908718,215.586585244582,215.668907217876,215.752893235024,
215.836879252173,215.912519361393,215.988135464298,216.063742031351,216.13937669406,
216.215026252636,216.290736542412,216.33534779548,216.427248365185,216.519281334901,
216.611160904726,216.702788300757,216.793809422241,216.833816338788,216.907818253476,
216.981799181818,217.05577420373,217.12978667703,217.20381794701,217.277922699215,
217.332284882095,217.411246298042,217.490153721111,217.569018760048,217.647852990774,
217.726667964752,217.805489228412,217.884315867525,217.963158391901,218.042027320484,
218.120969371815,218.199950137304,218.279021148322,218.32922196871,218.408213864049,
218.487105648724,218.565907904768,218.64460790559,218.723247351469,218.801823633655,
218.827690512018,218.906277235182,218.984913402445,219.063609395762,219.142423427246,
219.22130485547,219.300307948686,219.326159055326,219.405231577075,219.48423113181,
219.563169399634,219.642058014116,219.720908570672,219.799737074937,219.878553448806,
219.95736819999,220.036191833967,220.115061881515,220.193955560591,220.272916085428,
220.323096141941,220.397201580042,220.471250077897,220.545256815903,220.619246080055,
220.693223441667,220.767225727699,220.821564685248,220.910526452492,221.000020868658,
221.08972837351,221.179600242886,221.220595442298),.UNSPECIFIED.);
#3040=B_SPLINE_CURVE_WITH_KNOTS('',3,(#144233,#144234,#144235,#144236,#144237,
#144238,#144239,#144240,#144241,#144242,#144243,#144244,#144245,#144246,
#144247,#144248),.UNSPECIFIED.,.F.,.F.,(4,3,3,3,3,4),(221.220595442422,
221.320033228556,221.395742383023,221.47140477704,221.547032011141,221.577058603984),
 .UNSPECIFIED.);
#3041=B_SPLINE_CURVE_WITH_KNOTS('',3,(#144250,#144251,#144252,#144253,#144254,
#144255,#144256,#144257,#144258,#144259,#144260,#144261,#144262,#144263,
#144264,#144265),.UNSPECIFIED.,.F.,.F.,(4,3,3,3,3,4),(-217.837561537579,
-217.760053293282,-217.682505293837,-217.604936121589,-217.527300607496,
-217.481355898413),.UNSPECIFIED.);
#3042=B_SPLINE_CURVE_WITH_KNOTS('',3,(#144266,#144267,#144268,#144269,#144270,
#144271,#144272,#144273,#144274,#144275,#144276,#144277,#144278,#144279,
#144280,#144281,#144282,#144283,#144284,#144285,#144286,#144287,#144288,
#144289,#144290,#144291,#144292,#144293,#144294,#144295,#144296,#144297,
#144298,#144299,#144300,#144301,#144302,#144303,#144304,#144305,#144306,
#144307,#144308,#144309,#144310,#144311,#144312,#144313,#144314,#144315,
#144316,#144317,#144318,#144319,#144320,#144321,#144322,#144323,#144324,
#144325,#144326,#144327,#144328,#144329,#144330,#144331,#144332,#144333,
#144334,#144335,#144336,#144337,#144338,#144339,#144340,#144341,#144342,
#144343,#144344,#144345,#144346,#144347,#144348,#144349,#144350,#144351,
#144352,#144353,#144354,#144355,#144356,#144357,#144358,#144359,#144360,
#144361,#144362,#144363,#144364,#144365,#144366,#144367,#144368,#144369,
#144370,#144371,#144372,#144373,#144374,#144375,#144376,#144377,#144378,
#144379,#144380,#144381,#144382,#144383,#144384,#144385,#144386,#144387,
#144388,#144389,#144390,#144391,#144392,#144393,#144394,#144395,#144396,
#144397,#144398,#144399,#144400,#144401,#144402,#144403,#144404,#144405,
#144406,#144407,#144408,#144409,#144410,#144411,#144412,#144413,#144414,
#144415,#144416,#144417,#144418,#144419,#144420,#144421,#144422,#144423,
#144424,#144425,#144426,#144427,#144428,#144429,#144430,#144431,#144432,
#144433,#144434,#144435,#144436,#144437,#144438,#144439,#144440,#144441,
#144442,#144443,#144444,#144445,#144446,#144447,#144448,#144449,#144450,
#144451,#144452,#144453,#144454,#144455,#144456,#144457,#144458,#144459,
#144460,#144461,#144462,#144463,#144464,#144465,#144466,#144467,#144468,
#144469,#144470,#144471,#144472,#144473,#144474,#144475,#144476,#144477,
#144478,#144479,#144480,#144481,#144482,#144483,#144484,#144485,#144486,
#144487,#144488,#144489,#144490,#144491,#144492,#144493,#144494,#144495,
#144496,#144497),.UNSPECIFIED.,.F.,.F.,(4,3,3,3,3,3,3,3,3,3,3,3,3,3,3,3,
3,3,3,3,3,3,3,3,3,3,3,3,3,3,3,3,3,3,3,3,3,3,3,3,3,3,3,3,3,3,3,3,3,3,3,3,
3,3,3,3,3,3,3,3,3,3,3,3,3,3,3,3,3,3,3,3,3,3,3,3,3,4),(-217.481355898316,
-217.332284882095,-217.258179443994,-217.18413094614,-217.110124208134,
-217.036134943982,-216.96215758237,-216.888155296338,-216.833816338788,
-216.74281723905,-216.651314021371,-216.559370482438,-216.467335905257,
-216.375426815133,-216.33534779548,-216.259638124363,-216.183977122338,
-216.108350282001,-216.03273258572,-215.957121085634,-215.881481161007,
-215.836879252173,-215.754600480319,-215.672297917456,-215.588826115309,
-215.50647116041,-215.422440934638,-215.338410708865,-215.256031698262,
-215.173667509011,-215.090236173147,-215.007914199853,-214.923928182705,
-214.839942165557,-214.764302056337,-214.688685953432,-214.613079386379,
-214.537444723671,-214.461795165095,-214.386084875319,-214.34147362225,
-214.249573052545,-214.157540082829,-214.065660513004,-213.974033116973,
-213.88301199549,-213.843005078942,-213.769003164254,-213.695022235912,
-213.621047214,-213.5470347407,-213.473003470719,-213.398898718515,-213.344536535635,
-213.265575119688,-213.186667696619,-213.107802657682,-213.028968426957,
-212.950153452978,-212.871332189318,-212.792505550206,-212.713663025829,
-212.634794097247,-212.555852045915,-212.476871280426,-212.397800269408,
-212.34759944902,-212.268607553681,-212.189715769005,-212.11091351296,-212.032213512137,
-211.953574066258,-211.874997784072,-211.849130905712,-211.770531646682,
-211.69189389683,-211.613163329234,-211.555186956847),.UNSPECIFIED.);
#3043=B_SPLINE_CURVE_WITH_KNOTS('',3,(#144503,#144504,#144505,#144506,#144507,
#144508,#144509,#144510,#144511,#144512,#144513,#144514,#144515,#144516,
#144517,#144518,#144519,#144520,#144521,#144522,#144523,#144524,#144525,
#144526,#144527,#144528,#144529,#144530,#144531,#144532,#144533,#144534,
#144535,#144536,#144537,#144538,#144539,#144540,#144541,#144542,#144543,
#144544,#144545,#144546,#144547,#144548,#144549,#144550,#144551,#144552,
#144553,#144554,#144555,#144556,#144557,#144558,#144559,#144560,#144561,
#144562,#144563,#144564,#144565,#144566,#144567,#144568,#144569,#144570,
#144571,#144572,#144573,#144574,#144575,#144576,#144577,#144578,#144579,
#144580,#144581,#144582,#144583,#144584,#144585,#144586,#144587,#144588,
#144589,#144590,#144591,#144592,#144593,#144594,#144595,#144596,#144597,
#144598,#144599,#144600,#144601,#144602,#144603,#144604,#144605,#144606,
#144607,#144608,#144609,#144610,#144611,#144612,#144613,#144614,#144615,
#144616,#144617,#144618,#144619,#144620,#144621,#144622,#144623,#144624,
#144625,#144626,#144627,#144628,#144629,#144630,#144631,#144632,#144633,
#144634,#144635,#144636,#144637,#144638,#144639,#144640,#144641,#144642,
#144643,#144644,#144645,#144646,#144647,#144648,#144649,#144650,#144651,
#144652,#144653,#144654,#144655,#144656,#144657,#144658,#144659,#144660,
#144661,#144662,#144663,#144664,#144665,#144666,#144667,#144668,#144669,
#144670,#144671,#144672,#144673,#144674,#144675,#144676,#144677,#144678,
#144679,#144680,#144681,#144682,#144683,#144684,#144685,#144686,#144687,
#144688,#144689,#144690,#144691,#144692,#144693,#144694,#144695,#144696,
#144697,#144698,#144699,#144700,#144701,#144702,#144703,#144704,#144705,
#144706,#144707,#144708,#144709,#144710,#144711,#144712,#144713,#144714,
#144715,#144716,#144717,#144718,#144719,#144720,#144721,#144722,#144723,
#144724,#144725,#144726,#144727,#144728,#144729,#144730,#144731,#144732,
#144733,#144734,#144735,#144736,#144737,#144738,#144739,#144740,#144741,
#144742,#144743),.UNSPECIFIED.,.F.,.F.,(4,3,3,3,3,3,3,3,3,3,3,3,3,3,3,3,
3,3,3,3,3,3,3,3,3,3,3,3,3,3,3,3,3,3,3,3,3,3,3,3,3,3,3,3,3,3,3,3,3,3,3,3,
3,3,3,3,3,3,3,3,3,3,3,3,3,3,3,3,3,3,3,3,3,3,3,3,3,3,3,3,4),(209.010381503964,
209.085988047285,209.161622800332,209.237272587392,209.312982998961,209.356788189174,
209.448688758878,209.540721728594,209.632601298418,209.724228694449,209.815249815932,
209.855256732482,209.92925864717,210.003239575514,210.077214597427,210.151227070727,
210.225258340709,210.299363092915,210.35372527579,210.432686691737,210.511594114806,
210.590459153743,210.669293384468,210.748108358447,210.826929622107,210.905756261219,
210.984598785595,211.063467714177,211.142409765509,211.221390530997,211.300461542015,
211.350662362405,211.429654257743,211.508546042417,211.587348298461,211.666048299282,
211.74468774516,211.823264027345,211.849130905712,211.927717628876,212.00635379614,
212.085049789458,212.163863820941,212.242745249165,212.321748342382,212.34759944902,
212.42667197077,212.505671525505,212.584609793329,212.66349840781,212.742348964366,
212.821177468632,212.8999938425,212.978808593684,213.057632227662,213.13650227521,
213.215395954286,213.294356479123,213.344536535635,213.418641973736,213.49269047159,
213.566697209596,213.640686473748,213.71466383536,213.788666121392,213.843005078942,
213.93400417868,214.025507396355,214.117450935285,214.209485512466,214.301394602588,
214.34147362225,214.417183293369,214.492844295396,214.568471135735,214.644088832019,
214.719700332106,214.795340256735,214.839942165558,214.930975113248,214.937410135242),
 .UNSPECIFIED.);
#3044=B_SPLINE_CURVE_WITH_KNOTS('',3,(#144744,#144745,#144746,#144747,#144748,
#144749,#144750,#144751,#144752,#144753,#144754,#144755,#144756,#144757,
#144758,#144759),.UNSPECIFIED.,.F.,.F.,(4,3,3,3,3,4),(214.937410135318,
215.018871014483,215.100353018709,215.181840116616,215.263345603113,215.293584957643),
 .UNSPECIFIED.);
#3045=B_SPLINE_CURVE_WITH_KNOTS('',3,(#144761,#144762,#144763,#144764,#144765,
#144766,#144767,#144768,#144769,#144770,#144771,#144772,#144773,#144774,
#144775,#144776),.UNSPECIFIED.,.F.,.F.,(4,3,3,3,3,4),(-211.555186956847,
-211.476324236877,-211.39733291139,-211.350662362405,-211.217629850047,
-211.198170591137),.UNSPECIFIED.);
#3046=B_SPLINE_CURVE_WITH_KNOTS('',3,(#144777,#144778,#144779,#144780,#144781,
#144782,#144783,#144784,#144785,#144786,#144787,#144788,#144789,#144790,
#144791,#144792,#144793,#144794,#144795,#144796,#144797,#144798,#144799,
#144800,#144801,#144802,#144803,#144804,#144805,#144806,#144807,#144808,
#144809,#144810,#144811,#144812,#144813,#144814,#144815,#144816,#144817,
#144818,#144819,#144820,#144821,#144822,#144823,#144824,#144825,#144826,
#144827,#144828,#144829,#144830,#144831,#144832,#144833,#144834,#144835,
#144836,#144837,#144838,#144839,#144840,#144841,#144842,#144843,#144844,
#144845,#144846,#144847,#144848,#144849,#144850,#144851,#144852,#144853,
#144854,#144855,#144856,#144857,#144858,#144859,#144860,#144861,#144862,
#144863,#144864,#144865,#144866,#144867,#144868,#144869,#144870,#144871,
#144872,#144873,#144874,#144875,#144876,#144877,#144878,#144879,#144880,
#144881,#144882,#144883,#144884,#144885,#144886,#144887,#144888,#144889,
#144890,#144891,#144892,#144893,#144894,#144895,#144896,#144897,#144898,
#144899,#144900,#144901,#144902,#144903,#144904,#144905,#144906,#144907,
#144908,#144909,#144910,#144911,#144912,#144913,#144914,#144915,#144916,
#144917,#144918,#144919,#144920,#144921,#144922,#144923,#144924,#144925,
#144926,#144927,#144928,#144929,#144930,#144931,#144932,#144933,#144934,
#144935,#144936,#144937,#144938,#144939,#144940,#144941,#144942,#144943,
#144944,#144945,#144946,#144947,#144948,#144949,#144950,#144951,#144952,
#144953,#144954,#144955,#144956,#144957,#144958,#144959,#144960,#144961,
#144962,#144963,#144964,#144965,#144966,#144967,#144968,#144969,#144970,
#144971,#144972,#144973,#144974,#144975,#144976,#144977,#144978,#144979,
#144980,#144981,#144982,#144983,#144984,#144985,#144986,#144987,#144988,
#144989,#144990,#144991,#144992,#144993,#144994,#144995,#144996,#144997,
#144998,#144999,#145000,#145001,#145002,#145003,#145004,#145005,#145006,
#145007,#145008,#145009,#145010,#145011),.UNSPECIFIED.,.F.,.F.,(4,3,3,3,
3,3,3,3,3,3,3,3,3,3,3,3,3,3,3,3,3,3,3,3,3,3,3,3,3,3,3,3,3,3,3,3,3,3,3,3,
3,3,3,3,3,3,3,3,3,3,3,3,3,3,3,3,3,3,3,3,3,3,3,3,3,3,3,3,3,3,3,3,3,3,3,3,
3,3,4),(-211.198170591051,-211.120197743593,-211.042291363753,-210.96443779742,
-210.886623209151,-210.8088299744,-210.731045779471,-210.653258318129,-210.575426098554,
-210.497571869303,-210.419643103381,-210.353725275789,-210.279619837687,
-210.205571339833,-210.131564601827,-210.057575337674,-209.983597976063,
-209.90959569003,-209.855256732482,-209.764257632745,-209.672754415067,
-209.580810876135,-209.488776298956,-209.396867208834,-209.356788189174,
-209.281078518057,-209.205417516032,-209.129790675694,-209.054172979413,
-208.978561479327,-208.9029215547,-208.858319645867,-208.776040874013,-208.693738311149,
-208.610266509002,-208.527911554103,-208.443881328331,-208.359851102559,
-208.277472091958,-208.195107902709,-208.111676566845,-208.029354593553,
-207.945368576402,-207.861382559252,-207.78574245003,-207.710126347124,
-207.63451978007,-207.55888511736,-207.483235558781,-207.407525269004,-207.362914015944,
-207.271013446243,-207.17898047653,-207.087100906709,-206.995473510682,
-206.904452389201,-206.864445472637,-206.790443557949,-206.716462629605,
-206.642487607692,-206.568475134392,-206.49444386441,-206.420339112205,
-206.365976929329,-206.287015513382,-206.208108090313,-206.129243051376,
-206.05040882065,-205.971593846672,-205.892772583012,-205.813945943899,
-205.735103419523,-205.65623449094,-205.577292439608,-205.49831167412,-205.419240663102,
-205.369039842714,-205.289130625658,-205.27050831412),.UNSPECIFIED.);
#3047=B_SPLINE_CURVE_WITH_KNOTS('',3,(#145017,#145018,#145019,#145020,#145021,
#145022,#145023,#145024,#145025,#145026,#145027,#145028,#145029,#145030,
#145031,#145032,#145033,#145034,#145035,#145036,#145037,#145038,#145039,
#145040,#145041,#145042,#145043,#145044,#145045,#145046,#145047,#145048,
#145049,#145050,#145051,#145052,#145053,#145054,#145055,#145056,#145057,
#145058,#145059,#145060,#145061,#145062,#145063,#145064,#145065,#145066,
#145067,#145068,#145069,#145070,#145071,#145072,#145073,#145074,#145075,
#145076,#145077,#145078,#145079,#145080,#145081,#145082,#145083,#145084,
#145085,#145086,#145087,#145088,#145089,#145090,#145091,#145092,#145093,
#145094,#145095,#145096,#145097,#145098,#145099,#145100,#145101,#145102,
#145103,#145104,#145105,#145106,#145107,#145108,#145109,#145110,#145111,
#145112,#145113,#145114,#145115,#145116,#145117,#145118,#145119,#145120,
#145121,#145122,#145123,#145124,#145125,#145126,#145127,#145128,#145129,
#145130,#145131,#145132,#145133,#145134,#145135,#145136,#145137,#145138,
#145139,#145140,#145141,#145142,#145143,#145144,#145145,#145146,#145147,
#145148,#145149,#145150,#145151,#145152,#145153,#145154,#145155,#145156,
#145157,#145158,#145159,#145160,#145161,#145162,#145163,#145164,#145165,
#145166,#145167,#145168,#145169,#145170,#145171,#145172,#145173,#145174,
#145175,#145176,#145177,#145178,#145179,#145180,#145181,#145182,#145183,
#145184,#145185,#145186,#145187,#145188,#145189,#145190,#145191,#145192,
#145193,#145194,#145195,#145196,#145197,#145198,#145199,#145200,#145201,
#145202,#145203,#145204,#145205,#145206,#145207,#145208,#145209,#145210,
#145211,#145212,#145213,#145214,#145215,#145216,#145217,#145218,#145219,
#145220,#145221,#145222,#145223,#145224,#145225,#145226,#145227,#145228,
#145229,#145230,#145231,#145232,#145233,#145234,#145235,#145236,#145237,
#145238,#145239,#145240,#145241,#145242,#145243,#145244,#145245,#145246,
#145247,#145248,#145249,#145250,#145251,#145252,#145253,#145254),
 .UNSPECIFIED.,.F.,.F.,(4,3,3,3,3,3,3,3,3,3,3,3,3,3,3,3,3,3,3,3,3,3,3,3,
3,3,3,3,3,3,3,3,3,3,3,3,3,3,3,3,3,3,3,3,3,3,3,3,3,3,3,3,3,3,3,3,3,3,3,3,
3,3,3,3,3,3,3,3,3,3,3,3,3,3,3,3,3,3,3,4),(202.727851097702,202.818931905915,
202.876697126176,202.950699040865,203.024679969209,203.098654991122,203.172667464423,
203.246698734404,203.32080348661,203.375165669484,203.454127085431,203.5330345085,
203.611899547437,203.690733778163,203.769548752142,203.848370015802,203.927196654914,
204.00603917929,204.084908107873,204.163850159204,204.242830924693,204.321901935711,
204.372102756099,204.451094651437,204.529986436111,204.608788692154,204.687488692975,
204.766128138853,204.844704421037,204.870571299406,204.94915802257,205.027794189834,
205.106490183151,205.185304214635,205.264185642859,205.343188736076,205.369039842714,
205.448112364463,205.527111919198,205.606050187022,205.684938801503,205.76378935806,
205.842617862325,205.921434236194,206.000248987378,206.079072621355,206.157942668903,
206.236836347979,206.315796872816,206.365976929329,206.440082367431,206.514130865286,
206.588137603294,206.662126867447,206.736104229059,206.810106515092,206.864445472637,
206.955444572371,207.046947790046,207.138891328975,207.230925906152,207.322834996271,
207.362914015944,207.438623687062,207.514284689089,207.589911529427,207.66552922571,
207.741140725798,207.816780650426,207.861382559252,207.943661331104,208.025963893966,
208.109435696114,208.191790651011,208.275820876785,208.359851102559,208.441480017848,
208.523091015779,208.604687165193,208.654224828063),.UNSPECIFIED.);
#3048=B_SPLINE_CURVE_WITH_KNOTS('',3,(#145255,#145256,#145257,#145258,#145259,
#145260,#145261,#145262,#145263,#145264,#145265,#145266,#145267,#145268,
#145269,#145270),.UNSPECIFIED.,.F.,.F.,(4,3,3,3,3,4),(208.654224828187,
208.740497929717,208.826719004093,208.858319645867,208.934350574915,209.010381503964),
 .UNSPECIFIED.);
#3049=B_SPLINE_CURVE_WITH_KNOTS('',3,(#145272,#145273,#145274,#145275,#145276,
#145277,#145278,#145279,#145280,#145281,#145282,#145283,#145284,#145285,
#145286,#145287),.UNSPECIFIED.,.F.,.F.,(4,3,3,3,3,4),(-205.27050831412,
-205.190744529819,-205.11111727546,-205.031571299999,-204.952123552818,
-204.914985284074),.UNSPECIFIED.);
#3050=B_SPLINE_CURVE_WITH_KNOTS('',3,(#145288,#145289,#145290,#145291,#145292,
#145293,#145294,#145295,#145296,#145297,#145298,#145299,#145300,#145301,
#145302,#145303,#145304,#145305,#145306,#145307,#145308,#145309,#145310,
#145311,#145312,#145313,#145314,#145315,#145316,#145317,#145318,#145319,
#145320,#145321,#145322,#145323,#145324,#145325,#145326,#145327,#145328,
#145329,#145330,#145331,#145332,#145333,#145334,#145335,#145336,#145337,
#145338,#145339,#145340,#145341,#145342,#145343,#145344,#145345,#145346,
#145347,#145348,#145349,#145350,#145351,#145352,#145353,#145354,#145355,
#145356,#145357,#145358,#145359,#145360,#145361,#145362,#145363,#145364,
#145365,#145366,#145367,#145368,#145369,#145370,#145371,#145372,#145373,
#145374,#145375,#145376,#145377,#145378,#145379,#145380,#145381,#145382,
#145383,#145384,#145385,#145386,#145387,#145388,#145389,#145390,#145391,
#145392,#145393,#145394,#145395,#145396,#145397,#145398,#145399,#145400,
#145401,#145402,#145403,#145404,#145405,#145406,#145407,#145408,#145409,
#145410,#145411,#145412,#145413,#145414,#145415,#145416,#145417,#145418,
#145419,#145420,#145421,#145422,#145423,#145424,#145425,#145426,#145427,
#145428,#145429,#145430,#145431,#145432,#145433,#145434,#145435,#145436,
#145437,#145438,#145439,#145440,#145441,#145442,#145443,#145444,#145445,
#145446,#145447,#145448,#145449,#145450,#145451,#145452,#145453,#145454,
#145455,#145456,#145457,#145458,#145459,#145460,#145461,#145462,#145463,
#145464,#145465,#145466,#145467,#145468,#145469,#145470,#145471,#145472,
#145473,#145474,#145475,#145476,#145477,#145478,#145479,#145480,#145481,
#145482,#145483,#145484,#145485,#145486,#145487,#145488,#145489,#145490,
#145491,#145492,#145493,#145494,#145495,#145496,#145497,#145498,#145499,
#145500,#145501,#145502,#145503,#145504,#145505,#145506,#145507,#145508,
#145509,#145510,#145511,#145512,#145513,#145514,#145515,#145516,#145517,
#145518,#145519,#145520,#145521,#145522),.UNSPECIFIED.,.F.,.F.,(4,3,3,3,
3,3,3,3,3,3,3,3,3,3,3,3,3,3,3,3,3,3,3,3,3,3,3,3,3,3,3,3,3,3,3,3,3,3,3,3,
3,3,3,3,3,3,3,3,3,3,3,3,3,3,3,3,3,3,3,3,3,3,3,3,3,3,3,3,3,3,3,3,3,3,3,3,
3,3,4),(-204.914985283957,-204.870571299406,-204.791984576244,-204.713348408983,
-204.634652415668,-204.555838384187,-204.476956955965,-204.397953862751,
-204.372102756099,-204.293030234349,-204.214030679614,-204.13509241179,
-204.056203797308,-203.977353240752,-203.898524736486,-203.819708362616,
-203.740893611432,-203.662069977454,-203.583199929906,-203.50430625083,
-203.425345725992,-203.375165669484,-203.301060231382,-203.227011733527,
-203.153004995519,-203.079015731366,-203.005038369754,-202.93103608372,
-202.876697126176,-202.785698026443,-202.694194808769,-202.602251269841,
-202.510216692664,-202.418307602545,-202.378228582869,-202.302518911751,
-202.226857909725,-202.151231069388,-202.075613373105,-202.000001873018,
-201.92436194839,-201.879760039561,-201.797481267707,-201.715178704842,
-201.631706902695,-201.549351947796,-201.465321722024,-201.381291496253,
-201.298912485652,-201.216548296405,-201.13311696054,-201.050794987249,
-200.966808970097,-200.882822952946,-200.807182843724,-200.731566740817,
-200.655960173762,-200.580325511052,-200.504675952473,-200.428965662696,
-200.384354409638,-200.292453839936,-200.200420870225,-200.108541300405,
-200.016913904378,-199.925892782898,-199.885885866331,-199.811883951642,
-199.737903023298,-199.663928001386,-199.589915528085,-199.515884258103,
-199.441779505898,-199.387417323023,-199.309170163293,-199.22899001696,
-199.15085344188,-199.069651509919,-198.988449577959),.UNSPECIFIED.);
#3051=B_SPLINE_CURVE_WITH_KNOTS('',3,(#145528,#145529,#145530,#145531,#145532,
#145533,#145534,#145535,#145536,#145537,#145538,#145539,#145540,#145541,
#145542,#145543,#145544,#145545,#145546,#145547,#145548,#145549,#145550,
#145551,#145552,#145553,#145554,#145555,#145556,#145557,#145558,#145559,
#145560,#145561,#145562,#145563,#145564,#145565,#145566,#145567,#145568,
#145569,#145570,#145571,#145572,#145573,#145574,#145575,#145576,#145577,
#145578,#145579,#145580,#145581,#145582,#145583,#145584,#145585,#145586,
#145587,#145588,#145589,#145590,#145591,#145592,#145593,#145594,#145595,
#145596,#145597,#145598,#145599,#145600,#145601,#145602,#145603,#145604,
#145605,#145606,#145607,#145608,#145609,#145610,#145611,#145612,#145613,
#145614,#145615,#145616,#145617,#145618,#145619,#145620,#145621,#145622,
#145623,#145624,#145625,#145626,#145627,#145628,#145629,#145630,#145631,
#145632,#145633,#145634,#145635,#145636,#145637,#145638,#145639,#145640,
#145641,#145642,#145643,#145644,#145645,#145646,#145647,#145648,#145649,
#145650,#145651,#145652,#145653,#145654,#145655,#145656,#145657,#145658,
#145659,#145660,#145661,#145662,#145663,#145664,#145665,#145666,#145667,
#145668,#145669,#145670,#145671,#145672,#145673,#145674,#145675,#145676,
#145677,#145678,#145679,#145680,#145681,#145682,#145683,#145684,#145685,
#145686,#145687,#145688,#145689,#145690,#145691,#145692,#145693,#145694,
#145695,#145696,#145697,#145698,#145699,#145700,#145701,#145702,#145703,
#145704,#145705,#145706,#145707,#145708,#145709,#145710,#145711,#145712,
#145713,#145714,#145715,#145716,#145717,#145718,#145719,#145720,#145721,
#145722,#145723,#145724,#145725,#145726,#145727,#145728,#145729,#145730,
#145731,#145732,#145733,#145734,#145735,#145736,#145737,#145738,#145739,
#145740,#145741,#145742,#145743,#145744,#145745,#145746,#145747,#145748,
#145749,#145750,#145751,#145752,#145753,#145754,#145755,#145756,#145757,
#145758,#145759,#145760,#145761,#145762),.UNSPECIFIED.,.F.,.F.,(4,3,3,3,
3,3,3,3,3,3,3,3,3,3,3,3,3,3,3,3,3,3,3,3,3,3,3,3,3,3,3,3,3,3,3,3,3,3,3,3,
3,3,3,3,3,3,3,3,3,3,3,3,3,3,3,3,3,3,3,3,3,3,3,3,3,3,3,3,3,3,3,3,3,3,3,3,
3,3,4),(196.443737963822,196.522665757598,196.601546491101,196.680391752479,
196.759213102051,196.838504358019,196.917327604243,196.996162560754,197.07501974207,
197.154650594001,197.233615182068,197.313579165931,197.393543149793,197.472535045132,
197.551426829808,197.630229085853,197.708929086675,197.787568532554,197.86614481474,
197.892011693101,197.970598416264,198.049234583526,198.127930576842,198.206744608324,
198.285626036547,198.364629129762,198.390480236408,198.469552758158,198.548552312893,
198.627490580717,198.706379195198,198.785229751754,198.86405825602,198.942874629889,
199.021689381072,199.10051301505,199.179383062598,199.258276741674,199.337237266511,
199.387417323023,199.461522761125,199.535571258981,199.609577996988,199.683567261141,
199.757544622754,199.831546908788,199.885885866331,199.976884966065,200.06838818374,
200.160331722668,200.252366299845,200.344275389964,200.384354409638,200.460064080756,
200.535725082783,200.611351923121,200.686969619404,200.762581119492,200.83822104412,
200.882822952946,200.965101724798,201.04740428766,201.130876089808,201.213231044705,
201.297261270479,201.381291496253,201.463670506856,201.546034696106,201.62946603197,
201.711788005263,201.795774022412,201.879760039561,201.955357754018,202.030931327645,
202.106495255714,202.182086177459,202.257691990731,202.333355910857,202.371039520793),
 .UNSPECIFIED.);
#3052=B_SPLINE_CURVE_WITH_KNOTS('',3,(#145763,#145764,#145765,#145766,#145767,
#145768,#145769,#145770,#145771,#145772,#145773,#145774,#145775,#145776,
#145777,#145778),.UNSPECIFIED.,.F.,.F.,(4,3,3,3,3,4),(202.371039520883,
202.378228582869,202.470178269923,202.562210817129,202.654076209428,202.727851097702),
 .UNSPECIFIED.);
#3053=B_SPLINE_CURVE_WITH_KNOTS('',3,(#145780,#145781,#145782,#145783,#145784,
#145785,#145786,#145787,#145788,#145789,#145790,#145791,#145792,#145793,
#145794,#145795),.UNSPECIFIED.,.F.,.F.,(4,3,3,3,3,4),(-198.988449577959,
-198.910364452514,-198.832250522121,-198.754121808537,-198.675939145095,
-198.631799976778),.UNSPECIFIED.);
#3054=B_SPLINE_CURVE_WITH_KNOTS('',3,(#145796,#145797,#145798,#145799,#145800,
#145801,#145802,#145803,#145804,#145805,#145806,#145807,#145808,#145809,
#145810,#145811,#145812,#145813,#145814,#145815,#145816,#145817,#145818,
#145819,#145820,#145821,#145822,#145823,#145824,#145825,#145826,#145827,
#145828,#145829,#145830,#145831,#145832,#145833,#145834,#145835,#145836,
#145837,#145838,#145839,#145840,#145841,#145842,#145843,#145844,#145845,
#145846,#145847,#145848,#145849,#145850,#145851,#145852,#145853,#145854,
#145855,#145856,#145857,#145858,#145859,#145860,#145861,#145862,#145863,
#145864,#145865,#145866,#145867,#145868,#145869,#145870,#145871,#145872,
#145873,#145874,#145875,#145876,#145877,#145878,#145879,#145880,#145881,
#145882,#145883,#145884,#145885,#145886,#145887,#145888,#145889,#145890,
#145891,#145892,#145893,#145894,#145895,#145896,#145897,#145898,#145899,
#145900,#145901,#145902,#145903,#145904,#145905,#145906,#145907,#145908,
#145909,#145910,#145911,#145912,#145913,#145914,#145915,#145916,#145917,
#145918,#145919,#145920,#145921,#145922,#145923,#145924,#145925,#145926,
#145927,#145928,#145929,#145930,#145931,#145932,#145933,#145934,#145935,
#145936,#145937,#145938,#145939,#145940,#145941,#145942,#145943,#145944,
#145945,#145946,#145947,#145948,#145949,#145950,#145951,#145952,#145953,
#145954,#145955,#145956,#145957,#145958,#145959,#145960,#145961,#145962,
#145963,#145964,#145965,#145966,#145967,#145968,#145969,#145970,#145971,
#145972,#145973,#145974,#145975,#145976,#145977,#145978,#145979,#145980,
#145981,#145982,#145983,#145984,#145985,#145986,#145987,#145988,#145989,
#145990,#145991,#145992,#145993,#145994,#145995,#145996,#145997,#145998,
#145999,#146000,#146001,#146002,#146003,#146004,#146005,#146006,#146007,
#146008,#146009,#146010,#146011,#146012,#146013,#146014,#146015,#146016,
#146017,#146018,#146019,#146020,#146021,#146022,#146023,#146024,#146025,
#146026,#146027,#146028,#146029,#146030),.UNSPECIFIED.,.F.,.F.,(4,3,3,3,
3,3,3,3,3,3,3,3,3,3,3,3,3,3,3,3,3,3,3,3,3,3,3,3,3,3,3,3,3,3,3,3,3,3,3,3,
3,3,3,3,3,3,3,3,3,3,3,3,3,3,3,3,3,3,3,3,3,3,3,3,3,3,3,3,3,3,3,3,3,3,3,3,
3,3,4),(-198.631799976686,-198.530223734246,-198.42689683786,-198.390480236408,
-198.311488341069,-198.232596556394,-198.15379430035,-198.075094299528,
-197.996454853649,-197.917878571464,-197.8920116931,-197.813424969937,-197.734788802675,
-197.656092809359,-197.577278777877,-197.498397349654,-197.419394256439,
-197.393543149793,-197.314470628043,-197.235471073308,-197.156532805484,
-197.077644191003,-196.998793634447,-196.919965130181,-196.841148756312,
-196.762334005128,-196.683510371151,-196.604640323602,-196.525746644527,
-196.44678611969,-196.396606063178,-196.322500625076,-196.24845212722,-196.174445389213,
-196.10045612506,-196.026478763447,-195.952476477413,-195.89813751987,-195.807138420136,
-195.715635202461,-195.623691663533,-195.531657086357,-195.439747996238,
-195.399668976563,-195.323959305445,-195.248298303418,-195.17267146308,
-195.097053766797,-195.021442266709,-194.945802342081,-194.901200433255,
-194.818921661403,-194.736619098541,-194.653147296393,-194.570792341496,
-194.486762115722,-194.402731889948,-194.320352879346,-194.237988690096,
-194.154557354232,-194.072235380939,-193.988249363789,-193.90426334664,
-193.828623237418,-193.753007134511,-193.677400567456,-193.601765904746,
-193.526116346167,-193.450406056389,-193.405794803332,-193.313894233632,
-193.221861263921,-193.129981694102,-193.038354298076,-192.947333176598,
-192.907326260025,-192.833325706021,-192.759340356795,-192.704890585279),
 .UNSPECIFIED.);
#3055=B_SPLINE_CURVE_WITH_KNOTS('',3,(#146036,#146037,#146038,#146039,#146040,
#146041,#146042,#146043,#146044,#146045,#146046,#146047,#146048,#146049,
#146050,#146051,#146052,#146053,#146054,#146055,#146056,#146057,#146058,
#146059,#146060,#146061,#146062,#146063,#146064,#146065,#146066,#146067,
#146068,#146069,#146070,#146071,#146072,#146073,#146074,#146075,#146076,
#146077,#146078,#146079,#146080,#146081,#146082,#146083,#146084,#146085,
#146086,#146087,#146088,#146089,#146090,#146091,#146092,#146093,#146094,
#146095,#146096,#146097,#146098,#146099,#146100,#146101,#146102,#146103,
#146104,#146105,#146106,#146107,#146108,#146109,#146110,#146111,#146112,
#146113,#146114,#146115,#146116,#146117,#146118,#146119,#146120,#146121,
#146122,#146123,#146124,#146125,#146126,#146127,#146128,#146129,#146130,
#146131,#146132,#146133,#146134,#146135,#146136,#146137,#146138,#146139,
#146140,#146141,#146142,#146143,#146144,#146145,#146146,#146147,#146148,
#146149,#146150,#146151,#146152,#146153,#146154,#146155,#146156,#146157,
#146158,#146159,#146160,#146161,#146162,#146163,#146164,#146165,#146166,
#146167,#146168,#146169,#146170,#146171,#146172,#146173,#146174,#146175,
#146176,#146177,#146178,#146179,#146180,#146181,#146182,#146183,#146184,
#146185,#146186,#146187,#146188,#146189,#146190,#146191,#146192,#146193,
#146194,#146195,#146196,#146197,#146198,#146199,#146200,#146201,#146202,
#146203,#146204,#146205,#146206,#146207,#146208,#146209,#146210,#146211,
#146212,#146213,#146214,#146215,#146216,#146217,#146218,#146219,#146220,
#146221,#146222,#146223,#146224,#146225,#146226,#146227,#146228,#146229,
#146230,#146231,#146232,#146233,#146234,#146235,#146236,#146237,#146238,
#146239,#146240,#146241,#146242,#146243,#146244,#146245,#146246,#146247,
#146248,#146249,#146250,#146251,#146252,#146253,#146254,#146255,#146256,
#146257,#146258,#146259,#146260,#146261,#146262,#146263,#146264,#146265,
#146266,#146267,#146268,#146269,#146270,#146271,#146272,#146273),
 .UNSPECIFIED.,.F.,.F.,(4,3,3,3,3,3,3,3,3,3,3,3,3,3,3,3,3,3,3,3,3,3,3,3,
3,3,3,3,3,3,3,3,3,3,3,3,3,3,3,3,3,3,3,3,3,3,3,3,3,3,3,3,3,3,3,3,3,3,3,3,
3,3,3,3,3,3,3,3,3,3,3,3,3,3,3,3,3,3,3,4),(190.160514847461,190.239950536493,
190.319437569548,190.399017127351,190.414983543487,190.493975438826,190.572867223502,
190.651669479548,190.73036948037,190.809008926249,190.887585208435,190.913452086795,
190.992038809958,191.07067497722,191.149370970535,191.228185002017,191.30706643024,
191.386069523455,191.411920630102,191.490993151852,191.569992706587,191.648930974411,
191.727819588892,191.806670145448,191.885498649714,191.964315023583,192.043129774766,
192.121953408744,192.200823456292,192.279717135367,192.358677660204,192.408857716717,
192.482963154819,192.557011652674,192.631018390681,192.705007654834,192.778985016446,
192.85298730248,192.907326260025,192.998325359763,193.089828577442,193.181772116374,
193.273806693554,193.365715783677,193.405794803333,193.481504474449,193.557165476474,
193.63279231681,193.708410013091,193.784021513177,193.859661437804,193.90426334664,
193.986542118494,194.068844681359,194.152316483506,194.234671438406,194.318701664177,
194.402731889948,194.485110900549,194.567475089797,194.650906425662,194.733228398954,
194.817214416104,194.901200433255,194.976840542477,195.052456645383,195.128063212437,
195.203697875147,195.279347433726,195.355057723503,195.399668976563,195.491569546264,
195.583602515976,195.675482085796,195.767109481821,195.8581306033,195.89813751987,
195.968852952326,196.039554024148,196.087854213605),.UNSPECIFIED.);
#3056=B_SPLINE_CURVE_WITH_KNOTS('',3,(#146274,#146275,#146276,#146277,#146278,
#146279,#146280,#146281,#146282,#146283,#146284,#146285,#146286,#146287,
#146288,#146289),.UNSPECIFIED.,.F.,.F.,(4,3,3,3,3,4),(196.087854213704,
196.16581340922,196.243822506616,196.321954292725,196.396606063178,196.443737963822),
 .UNSPECIFIED.);
#3057=B_SPLINE_CURVE_WITH_KNOTS('',3,(#146291,#146292,#146293,#146294,#146295,
#146296,#146297,#146298,#146299,#146300,#146301,#146302,#146303,#146304,
#146305,#146306),.UNSPECIFIED.,.F.,.F.,(4,3,3,3,3,4),(-192.704890585279,
-192.630880807372,-192.556855814682,-192.482753841835,-192.408857716717,
-192.348614669598),.UNSPECIFIED.);
#3058=B_SPLINE_CURVE_WITH_KNOTS('',3,(#146307,#146308,#146309,#146310,#146311,
#146312,#146313,#146314,#146315,#146316,#146317,#146318,#146319,#146320,
#146321,#146322,#146323,#146324,#146325,#146326,#146327,#146328,#146329,
#146330,#146331,#146332,#146333,#146334,#146335,#146336,#146337,#146338,
#146339,#146340,#146341,#146342,#146343,#146344,#146345,#146346,#146347,
#146348,#146349,#146350,#146351,#146352,#146353,#146354,#146355,#146356,
#146357,#146358,#146359,#146360,#146361,#146362,#146363,#146364,#146365,
#146366,#146367,#146368,#146369,#146370,#146371,#146372,#146373,#146374,
#146375,#146376,#146377,#146378,#146379,#146380,#146381,#146382,#146383,
#146384,#146385,#146386,#146387,#146388,#146389,#146390,#146391,#146392,
#146393,#146394,#146395,#146396,#146397,#146398,#146399,#146400,#146401,
#146402,#146403,#146404,#146405,#146406,#146407,#146408,#146409,#146410,
#146411,#146412,#146413,#146414,#146415,#146416,#146417,#146418,#146419,
#146420,#146421,#146422,#146423,#146424,#146425,#146426,#146427,#146428,
#146429,#146430,#146431,#146432,#146433,#146434,#146435,#146436,#146437,
#146438,#146439,#146440,#146441,#146442,#146443,#146444,#146445,#146446,
#146447,#146448,#146449,#146450,#146451,#146452,#146453,#146454,#146455,
#146456,#146457,#146458,#146459,#146460,#146461,#146462,#146463,#146464,
#146465,#146466,#146467,#146468,#146469,#146470,#146471,#146472,#146473,
#146474,#146475,#146476,#146477,#146478,#146479,#146480,#146481,#146482,
#146483,#146484,#146485,#146486,#146487,#146488,#146489,#146490,#146491,
#146492,#146493,#146494,#146495,#146496,#146497,#146498,#146499,#146500,
#146501,#146502,#146503,#146504,#146505,#146506,#146507,#146508,#146509,
#146510,#146511,#146512,#146513,#146514,#146515,#146516,#146517,#146518,
#146519,#146520,#146521,#146522,#146523,#146524,#146525,#146526,#146527,
#146528,#146529,#146530,#146531,#146532,#146533,#146534,#146535,#146536,
#146537,#146538,#146539,#146540,#146541,#146542,#146543,#146544),
 .UNSPECIFIED.,.F.,.F.,(4,3,3,3,3,3,3,3,3,3,3,3,3,3,3,3,3,3,3,3,3,3,3,3,
3,3,3,3,3,3,3,3,3,3,3,3,3,3,3,3,3,3,3,3,3,3,3,3,3,3,3,3,3,3,3,3,3,3,3,3,
3,3,3,3,3,3,3,3,3,3,3,3,3,3,3,3,3,3,3,4),(-192.348614669501,-192.270390617134,
-192.192227777621,-192.11411295072,-192.036032971698,-191.957965294289,
-191.879903180881,-191.801834718374,-191.723747991729,-191.645592249413,
-191.567402408137,-191.489114269976,-191.411920630102,-191.332928734764,
-191.25403695009,-191.175234694046,-191.096534693225,-191.017895247347,
-190.939318965163,-190.913452086795,-190.834865363631,-190.756229196367,
-190.67753320305,-190.598719171567,-190.519837743343,-190.440834650126,
-190.414983543487,-190.335911021738,-190.256911467003,-190.177973199179,
-190.099084584697,-190.020234028141,-189.941405523876,-189.862589150007,
-189.783774398823,-189.704950764846,-189.626080717298,-189.547187038222,
-189.468226513385,-189.418046456872,-189.34394101877,-189.269892520915,
-189.195885782908,-189.121896518755,-189.047919157142,-188.973916871109,
-188.919577913564,-188.82857881383,-188.737075596154,-188.645132057226,
-188.553097480049,-188.461188389929,-188.421109370257,-188.345399699139,
-188.269738697112,-188.194111856774,-188.118494160491,-188.042882660403,
-187.967242735775,-187.922640826949,-187.840362055097,-187.758059492235,
-187.674587690087,-187.59223273519,-187.508202509416,-187.424172283642,
-187.341793273039,-187.259429083788,-187.175997747925,-187.093675774631,
-187.009689757482,-186.925703740334,-186.850063631113,-186.774447528207,
-186.698840961154,-186.623206298445,-186.547556739867,-186.471846450091,
-186.427235197027,-186.42200373843),.UNSPECIFIED.);
#3059=B_SPLINE_CURVE_WITH_KNOTS('',3,(#146550,#146551,#146552,#146553,#146554,
#146555,#146556,#146557,#146558,#146559,#146560,#146561,#146562,#146563,
#146564,#146565,#146566,#146567,#146568,#146569,#146570,#146571,#146572,
#146573,#146574,#146575,#146576,#146577,#146578,#146579,#146580,#146581,
#146582,#146583,#146584,#146585,#146586,#146587,#146588,#146589,#146590,
#146591,#146592,#146593,#146594,#146595,#146596,#146597,#146598,#146599,
#146600,#146601,#146602,#146603,#146604,#146605,#146606,#146607,#146608,
#146609,#146610,#146611,#146612,#146613,#146614,#146615,#146616,#146617,
#146618,#146619,#146620,#146621,#146622,#146623,#146624,#146625,#146626,
#146627,#146628,#146629,#146630,#146631,#146632,#146633,#146634,#146635,
#146636,#146637,#146638,#146639,#146640,#146641,#146642,#146643,#146644,
#146645,#146646,#146647,#146648,#146649,#146650,#146651,#146652,#146653,
#146654,#146655,#146656,#146657,#146658,#146659,#146660,#146661,#146662,
#146663,#146664,#146665,#146666,#146667,#146668,#146669,#146670,#146671,
#146672,#146673,#146674,#146675,#146676,#146677,#146678,#146679,#146680,
#146681,#146682,#146683,#146684,#146685,#146686,#146687,#146688,#146689,
#146690,#146691,#146692,#146693,#146694,#146695,#146696,#146697,#146698,
#146699,#146700,#146701,#146702,#146703,#146704,#146705,#146706,#146707,
#146708,#146709,#146710,#146711,#146712,#146713,#146714,#146715,#146716,
#146717,#146718,#146719,#146720,#146721,#146722,#146723,#146724,#146725,
#146726,#146727,#146728,#146729,#146730,#146731,#146732,#146733,#146734,
#146735,#146736,#146737,#146738,#146739,#146740,#146741,#146742,#146743,
#146744,#146745,#146746,#146747,#146748,#146749,#146750,#146751,#146752,
#146753,#146754,#146755,#146756,#146757,#146758,#146759,#146760,#146761,
#146762,#146763,#146764,#146765,#146766,#146767,#146768,#146769,#146770,
#146771,#146772,#146773,#146774,#146775,#146776,#146777,#146778,#146779,
#146780,#146781,#146782,#146783,#146784),.UNSPECIFIED.,.F.,.F.,(4,3,3,3,
3,3,3,3,3,3,3,3,3,3,3,3,3,3,3,3,3,3,3,3,3,3,3,3,3,3,3,3,3,3,3,3,3,3,3,3,
3,3,3,3,3,3,3,3,3,3,3,3,3,3,3,3,3,3,3,3,3,3,3,3,3,3,3,3,3,3,3,3,3,3,3,3,
3,3,4),(183.87796157873,183.934892480489,184.013479203651,184.092115370914,
184.170811364229,184.249625395711,184.328506823934,184.407509917149,184.433361023796,
184.512433545546,184.591433100282,184.670371368106,184.749259982587,184.828110539145,
184.906939043411,184.98575541728,185.064570168464,185.143393802442,185.222263849991,
185.301157529067,185.380118053904,185.430298110412,185.504403548514,185.578452046368,
185.652458784375,185.726448048528,185.80042541014,185.874427696173,185.928766653719,
186.019765753455,186.111268971133,186.203212510064,186.295247087243,186.387156177364,
186.427235197027,186.502944868144,186.578605870169,186.654232710506,186.729850406788,
186.805461906874,186.881101831501,186.925703740334,187.007982512188,187.090285075052,
187.173756877199,187.256111832098,187.34014205787,187.424172283642,187.506551294243,
187.588915483491,187.672346819356,187.754668792648,187.838654809798,187.922640826949,
187.99828093617,188.073897039077,188.14950360613,188.225138268839,188.300787827417,
188.376498117194,188.421109370257,188.513009939962,188.605042909677,188.696922479502,
188.788549875532,188.879570997015,188.919577913565,188.993579828252,189.067560756595,
189.141535778506,189.215548251805,189.289579521785,189.363684273989,189.418046456872,
189.508079469988,189.597935928296,189.687584901263,189.776793207838,189.804668906392),
 .UNSPECIFIED.);
#3060=B_SPLINE_CURVE_WITH_KNOTS('',3,(#146785,#146786,#146787,#146788,#146789,
#146790,#146791,#146792,#146793,#146794,#146795,#146796,#146797,#146798,
#146799,#146800),.UNSPECIFIED.,.F.,.F.,(4,3,3,3,3,4),(189.804668906524,
189.883885148564,189.963143028557,190.042422162795,190.121758264539,190.160514847461),
 .UNSPECIFIED.);
#3061=B_SPLINE_CURVE_WITH_KNOTS('',3,(#146802,#146803,#146804,#146805,#146806,
#146807,#146808,#146809,#146810,#146811,#146812,#146813,#146814),
 .UNSPECIFIED.,.F.,.F.,(4,3,3,3,4),(-186.42200373843,-186.32760531351,-186.233107414807,
-186.138937815505,-186.065429362419),.UNSPECIFIED.);
#3062=B_SPLINE_CURVE_WITH_KNOTS('',3,(#146815,#146816,#146817,#146818,#146819,
#146820,#146821,#146822,#146823,#146824,#146825,#146826,#146827,#146828,
#146829,#146830,#146831,#146832,#146833,#146834,#146835,#146836,#146837,
#146838,#146839,#146840,#146841,#146842,#146843,#146844,#146845,#146846,
#146847,#146848,#146849,#146850,#146851,#146852,#146853,#146854,#146855,
#146856,#146857,#146858,#146859,#146860,#146861,#146862,#146863,#146864,
#146865,#146866,#146867,#146868,#146869,#146870,#146871,#146872,#146873,
#146874,#146875,#146876,#146877,#146878,#146879,#146880,#146881,#146882,
#146883,#146884,#146885,#146886,#146887,#146888,#146889,#146890,#146891,
#146892,#146893,#146894,#146895,#146896,#146897,#146898,#146899,#146900,
#146901,#146902,#146903,#146904,#146905,#146906,#146907,#146908,#146909,
#146910,#146911,#146912,#146913,#146914,#146915,#146916,#146917,#146918,
#146919,#146920,#146921,#146922,#146923,#146924,#146925,#146926,#146927,
#146928,#146929,#146930,#146931,#146932,#146933,#146934,#146935,#146936,
#146937,#146938,#146939,#146940,#146941,#146942,#146943,#146944,#146945,
#146946,#146947,#146948,#146949,#146950,#146951,#146952,#146953,#146954,
#146955,#146956,#146957,#146958,#146959,#146960,#146961,#146962,#146963,
#146964,#146965,#146966,#146967,#146968,#146969,#146970,#146971,#146972,
#146973,#146974,#146975,#146976,#146977,#146978,#146979,#146980,#146981,
#146982,#146983,#146984,#146985,#146986,#146987,#146988,#146989,#146990,
#146991,#146992,#146993,#146994,#146995,#146996,#146997,#146998,#146999,
#147000,#147001,#147002,#147003,#147004,#147005,#147006,#147007,#147008,
#147009,#147010,#147011,#147012,#147013,#147014,#147015,#147016,#147017,
#147018,#147019,#147020,#147021,#147022,#147023,#147024,#147025,#147026,
#147027,#147028,#147029,#147030,#147031,#147032,#147033,#147034),
 .UNSPECIFIED.,.F.,.F.,(4,3,3,3,3,3,3,3,3,3,3,3,3,3,3,3,3,3,3,3,3,3,3,3,
3,3,3,3,3,3,3,3,3,3,3,3,3,3,3,3,3,3,3,3,3,3,3,3,3,3,3,3,3,3,3,3,3,3,3,3,
3,3,3,3,3,3,3,3,3,3,3,3,3,4),(-186.065429362419,-185.983699488653,-185.901969734882,
-185.820240099441,-185.738510580662,-185.656781176878,-185.575051886423,
-185.490105117904,-185.406485642643,-185.324172721683,-185.242433812616,
-185.16069532323,-185.07895724685,-184.997219576802,-184.915482306414,-184.833745429011,
-184.75200893792,-184.67027282647,-184.588537087988,-184.506801715802,-184.42506670324,
-184.343332043631,-184.261597730303,-184.179863756587,-184.098130115812,
-184.016396801307,-183.934663806402,-183.852931124429,-183.771198748717,
-183.689466672597,-183.607734889402,-183.526003392461,-183.444272175108,
-183.362541230673,-183.280810552488,-183.199080133888,-183.117349968202,
-183.035620048765,-182.95389036891,-182.87216092197,-182.786732727571,-182.703974164247,
-182.622235536683,-182.540497732879,-182.45876072614,-182.377024489772,
-182.295288997086,-182.213554221395,-182.131820136015,-182.050086714262,
-181.968353929457,-181.886621754922,-181.80489016398,-181.72315912996,-181.641428626187,
-181.559698625992,-181.477969102708,-181.394249702613,-181.312511621585,
-181.23077512616,-181.149040109576,-181.067306465087,-180.98557408597,-180.903842865517,
-180.822112697037,-180.736655947557,-180.654919029338,-180.573185020435,
-180.491453493915,-180.409724022987,-180.327989132511,-180.246259052346,
-180.164527623284,-180.138458701197),.UNSPECIFIED.);
#3063=B_SPLINE_CURVE_WITH_KNOTS('',3,(#147040,#147041,#147042,#147043,#147044,
#147045,#147046,#147047,#147048,#147049,#147050,#147051,#147052,#147053,
#147054,#147055,#147056,#147057,#147058,#147059,#147060,#147061,#147062,
#147063,#147064,#147065,#147066,#147067,#147068,#147069,#147070,#147071,
#147072,#147073,#147074,#147075,#147076,#147077,#147078,#147079,#147080,
#147081,#147082,#147083,#147084,#147085,#147086,#147087,#147088,#147089,
#147090,#147091,#147092,#147093,#147094,#147095,#147096,#147097,#147098,
#147099,#147100,#147101,#147102,#147103,#147104,#147105,#147106,#147107,
#147108,#147109,#147110,#147111,#147112,#147113,#147114,#147115,#147116,
#147117,#147118,#147119,#147120,#147121,#147122,#147123,#147124,#147125,
#147126,#147127,#147128,#147129,#147130,#147131,#147132,#147133,#147134,
#147135,#147136,#147137,#147138,#147139,#147140,#147141,#147142,#147143,
#147144,#147145,#147146,#147147,#147148,#147149,#147150,#147151,#147152,
#147153,#147154,#147155,#147156,#147157,#147158,#147159,#147160,#147161,
#147162,#147163,#147164,#147165,#147166,#147167,#147168,#147169,#147170,
#147171,#147172,#147173,#147174,#147175,#147176,#147177,#147178,#147179,
#147180,#147181,#147182,#147183,#147184,#147185,#147186,#147187,#147188,
#147189,#147190,#147191,#147192,#147193,#147194,#147195,#147196,#147197,
#147198,#147199,#147200,#147201,#147202,#147203,#147204,#147205,#147206,
#147207,#147208,#147209,#147210,#147211,#147212,#147213,#147214,#147215,
#147216,#147217,#147218,#147219,#147220,#147221,#147222,#147223,#147224,
#147225,#147226,#147227,#147228,#147229,#147230,#147231,#147232,#147233,
#147234,#147235,#147236,#147237,#147238,#147239,#147240,#147241,#147242,
#147243,#147244,#147245,#147246,#147247,#147248,#147249,#147250,#147251,
#147252,#147253,#147254,#147255,#147256,#147257,#147258,#147259,#147260,
#147261,#147262,#147263,#147264,#147265,#147266,#147267,#147268,#147269,
#147270,#147271),.UNSPECIFIED.,.F.,.F.,(4,3,3,3,3,3,3,3,3,3,3,3,3,3,3,3,
3,3,3,3,3,3,3,3,3,3,3,3,3,3,3,3,3,3,3,3,3,3,3,3,3,3,3,3,3,3,3,3,3,3,3,3,
3,3,3,3,3,3,3,3,3,3,3,3,3,3,3,3,3,3,3,3,3,3,3,3,3,4),(177.594716365316,
177.673667692144,177.752566694605,177.831424976149,177.910257755466,177.989075987583,
178.06789018167,178.146710843128,178.225576826486,178.304464218069,178.38342159048,
178.451738504106,178.525843942414,178.599892440475,178.673899178688,178.747888443046,
178.821865804863,178.8958680911,178.950207047413,179.041206146889,179.13270936428,
179.224652902903,179.316687479773,179.408596569598,179.448675590721,179.524385261863,
179.600046263912,179.675673104274,179.75129080058,179.826902300691,179.902542225342,
179.947144134028,180.029422905902,180.111725468786,180.195197270924,180.277552225844,
180.36158245159,180.445612677336,180.527991687909,180.610355877129,180.693787213008,
180.776109186271,180.860095203457,180.944081220644,181.019721329879,181.095337432798,
181.170943999866,181.246578662589,181.32222822118,181.397938510971,181.442549763951,
181.534450333637,181.626483303333,181.718362873137,181.809990269148,181.901011390613,
181.941018307259,182.015020221949,182.089001150295,182.162976172209,182.236988645512,
182.311019915495,182.385124667702,182.439486850566,182.518448266513,182.597355689582,
182.676220728518,182.755054959244,182.833869933222,182.912691196882,182.991517835994,
183.070360360371,183.149229288953,183.228171340284,183.307152105773,183.38622311679,
183.436423937181,183.521483599344),.UNSPECIFIED.);
#3064=B_SPLINE_CURVE_WITH_KNOTS('',3,(#147272,#147273,#147274,#147275,#147276,
#147277,#147278,#147279,#147280,#147281,#147282,#147283,#147284,#147285,
#147286,#147287),.UNSPECIFIED.,.F.,.F.,(4,3,3,3,3,4),(183.521483599436,
183.598089530995,183.674591230521,183.751032931773,183.827419279678,183.87796157873),
 .UNSPECIFIED.);
#3065=B_SPLINE_CURVE_WITH_KNOTS('',3,(#147289,#147290,#147291,#147292,#147293,
#147294,#147295,#147296,#147297,#147298,#147299,#147300,#147301,#147302,
#147303,#147304),.UNSPECIFIED.,.F.,.F.,(4,3,3,3,3,4),(-180.138458701197,
-180.056729157361,-179.974994042442,-179.893263805093,-179.811532016142,
-179.782244055239),.UNSPECIFIED.);
#3066=B_SPLINE_CURVE_WITH_KNOTS('',3,(#147305,#147306,#147307,#147308,#147309,
#147310,#147311,#147312,#147313,#147314,#147315,#147316,#147317,#147318,
#147319,#147320,#147321,#147322,#147323,#147324,#147325,#147326,#147327,
#147328,#147329,#147330,#147331,#147332,#147333,#147334,#147335,#147336,
#147337,#147338,#147339,#147340,#147341,#147342,#147343,#147344,#147345,
#147346,#147347,#147348,#147349,#147350,#147351,#147352,#147353,#147354,
#147355,#147356,#147357,#147358,#147359,#147360,#147361,#147362,#147363,
#147364,#147365,#147366,#147367,#147368,#147369,#147370,#147371,#147372,
#147373,#147374,#147375,#147376,#147377,#147378,#147379,#147380,#147381,
#147382,#147383,#147384,#147385,#147386,#147387,#147388,#147389,#147390,
#147391,#147392,#147393,#147394,#147395,#147396,#147397,#147398,#147399,
#147400,#147401,#147402,#147403,#147404,#147405,#147406,#147407,#147408,
#147409,#147410,#147411,#147412,#147413,#147414,#147415,#147416,#147417,
#147418,#147419,#147420,#147421,#147422,#147423,#147424,#147425,#147426,
#147427,#147428,#147429,#147430,#147431,#147432,#147433,#147434,#147435,
#147436,#147437,#147438,#147439,#147440,#147441,#147442,#147443,#147444,
#147445,#147446,#147447,#147448,#147449,#147450,#147451,#147452,#147453,
#147454,#147455,#147456,#147457,#147458,#147459,#147460,#147461,#147462,
#147463,#147464,#147465,#147466,#147467,#147468,#147469,#147470,#147471,
#147472,#147473,#147474,#147475,#147476,#147477,#147478,#147479,#147480,
#147481,#147482,#147483,#147484,#147485,#147486,#147487,#147488,#147489,
#147490,#147491,#147492,#147493,#147494,#147495,#147496,#147497,#147498,
#147499,#147500,#147501,#147502,#147503,#147504,#147505,#147506,#147507,
#147508,#147509,#147510,#147511,#147512,#147513,#147514,#147515,#147516,
#147517,#147518,#147519,#147520,#147521,#147522,#147523,#147524,#147525,
#147526,#147527,#147528,#147529,#147530,#147531,#147532,#147533,#147534,
#147535,#147536,#147537,#147538,#147539,#147540,#147541,#147542,#147543,
#147544,#147545),.UNSPECIFIED.,.F.,.F.,(4,3,3,3,3,3,3,3,3,3,3,3,3,3,3,3,
3,3,3,3,3,3,3,3,3,3,3,3,3,3,3,3,3,3,3,3,3,3,3,3,3,3,3,3,3,3,3,3,3,3,3,3,
3,3,3,3,3,3,3,3,3,3,3,3,3,3,3,3,3,3,3,3,3,3,3,3,3,3,3,3,4),(-179.782244055239,
-179.70674937923,-179.631225012669,-179.555683642121,-179.480083302716,
-179.448675590721,-179.356775021314,-179.264742051907,-179.172862482386,
-179.081235086644,-178.990213965419,-178.950207047413,-178.876205132521,
-178.802224203973,-178.728249181856,-178.65423670835,-178.580205438163,
-178.506100685752,-178.451738504106,-178.37277708835,-178.293869665473,
-178.21500462673,-178.136170396199,-178.057355422415,-177.978534158949,
-177.89970752003,-177.820864995846,-177.741996067454,-177.66305401631,-177.584073251007,
-177.505002240169,-177.454801417491,-177.375809521819,-177.296917736817,
-177.218115480452,-177.13941547932,-177.060776033139,-176.982199750662,
-176.956332874183,-176.87774615106,-176.799109983836,-176.720413990555,
-176.641599959103,-176.562718530908,-176.483715437716,-176.457864330876,
-176.378791810217,-176.299792256578,-176.220853989855,-176.141965376475,
-176.063114821019,-175.984286317844,-175.90546994506,-175.826655194952,
-175.747831562039,-175.668961515531,-175.590067837481,-175.511107313639,
-175.46092724426,-175.386821801255,-175.312773298522,-175.238766555663,
-175.164777286706,-175.090799920313,-175.016797629551,-174.962458700953,
-174.871459625913,-174.779956434837,-174.688012923564,-174.595978373746,
-174.504069309141,-174.463990157645,-174.388280473823,-174.312619459148,
-174.236992606224,-174.161374897479,-174.085763384994,-174.010123448111,
-173.965521614338,-173.883281692548,-173.855477722695),.UNSPECIFIED.);
#3067=B_SPLINE_CURVE_WITH_KNOTS('',3,(#147551,#147552,#147553,#147554,#147555,
#147556,#147557,#147558,#147559,#147560,#147561,#147562,#147563,#147564,
#147565,#147566,#147567,#147568,#147569,#147570,#147571,#147572,#147573,
#147574,#147575,#147576,#147577,#147578,#147579,#147580,#147581,#147582,
#147583,#147584,#147585,#147586,#147587,#147588,#147589,#147590,#147591,
#147592,#147593,#147594,#147595,#147596,#147597,#147598,#147599,#147600,
#147601,#147602,#147603,#147604,#147605,#147606,#147607,#147608,#147609,
#147610,#147611,#147612,#147613,#147614,#147615,#147616,#147617,#147618,
#147619,#147620,#147621,#147622,#147623,#147624,#147625,#147626,#147627,
#147628,#147629,#147630,#147631,#147632,#147633,#147634,#147635,#147636,
#147637,#147638,#147639,#147640,#147641,#147642,#147643,#147644,#147645,
#147646,#147647,#147648,#147649,#147650,#147651,#147652,#147653,#147654,
#147655,#147656,#147657,#147658,#147659,#147660,#147661,#147662,#147663,
#147664,#147665,#147666,#147667,#147668,#147669,#147670,#147671,#147672,
#147673,#147674,#147675,#147676,#147677,#147678,#147679,#147680,#147681,
#147682,#147683,#147684,#147685,#147686,#147687,#147688,#147689,#147690,
#147691,#147692,#147693,#147694,#147695,#147696,#147697,#147698,#147699,
#147700,#147701,#147702,#147703,#147704,#147705,#147706,#147707,#147708,
#147709,#147710,#147711,#147712,#147713,#147714,#147715,#147716,#147717,
#147718,#147719,#147720,#147721,#147722,#147723,#147724,#147725,#147726,
#147727,#147728,#147729,#147730,#147731,#147732,#147733,#147734,#147735,
#147736,#147737,#147738,#147739,#147740,#147741,#147742,#147743,#147744,
#147745,#147746,#147747,#147748,#147749,#147750,#147751,#147752,#147753,
#147754,#147755,#147756,#147757,#147758,#147759,#147760,#147761,#147762,
#147763,#147764,#147765,#147766,#147767,#147768,#147769,#147770,#147771,
#147772,#147773,#147774,#147775,#147776,#147777,#147778,#147779,#147780,
#147781,#147782,#147783,#147784,#147785),.UNSPECIFIED.,.F.,.F.,(4,3,3,3,
3,3,3,3,3,3,3,3,3,3,3,3,3,3,3,3,3,3,3,3,3,3,3,3,3,3,3,3,3,3,3,3,3,3,3,3,
3,3,3,3,3,3,3,3,3,3,3,3,3,3,3,3,3,3,3,3,3,3,3,3,3,3,3,3,3,3,3,3,3,3,3,3,
3,3,4),(171.311431343321,171.394462023174,171.4731788978,171.547284682488,
171.621333526952,171.695340611491,171.769330221457,171.843307928735,171.917310559088,
171.971647441108,172.062645935509,172.154148482996,172.246091299276,172.338125146677,
172.430033533839,172.470115984415,172.545825784847,172.621486916478,172.697113886636,
172.772731712749,172.848343342738,172.923983396916,172.968584527723,173.050863244669,
173.133165751679,173.216637581517,173.298992479751,173.383022775391,173.46705307103,
173.549432078143,173.631796263722,173.715227601376,173.79754957065,173.881535592494,
173.965521614338,174.04116173582,174.116777851093,174.192384430612,174.268019105903,
174.343668677136,174.419378979628,174.463990157645,174.555890701794,174.647923644425,
174.739803186861,174.831430556288,174.92245165336,174.962458700953,175.036460620371,
175.110441553481,175.184416580198,175.258429058346,175.332460333206,175.406565090317,
175.46092724426,175.539888659215,175.618796081269,175.697661119169,175.776495348841,
175.855310321749,175.934131584323,176.01295822234,176.091800745614,176.170669673091,
176.249611723317,176.3285924877,176.407663497624,176.457864330876,176.536856226191,
176.615748010839,176.694550266853,176.773250267641,176.851889713482,176.930465995628,
176.956332874183,177.030702036272,177.105081017374,177.17952040767,177.238298292035),
 .UNSPECIFIED.);
#3068=B_SPLINE_CURVE_WITH_KNOTS('',3,(#147786,#147787,#147788,#147789,#147790,
#147791,#147792,#147793,#147794,#147795,#147796,#147797,#147798,#147799,
#147800,#147801),.UNSPECIFIED.,.F.,.F.,(4,3,3,3,3,4),(177.238298292165,
177.328651471841,177.419665567986,177.454801417491,177.533869140457,177.594716365316),
 .UNSPECIFIED.);
#3069=B_SPLINE_CURVE_WITH_KNOTS('',3,(#147803,#147804,#147805,#147806,#147807,
#147808,#147809,#147810,#147811,#147812,#147813,#147814,#147815,#147816,
#147817,#147818),.UNSPECIFIED.,.F.,.F.,(4,3,3,3,3,4),(-173.855477722695,
-173.773204617602,-173.690895316582,-173.608575252747,-173.526235864634,
-173.499058748059),.UNSPECIFIED.);
#3070=B_SPLINE_CURVE_WITH_KNOTS('',3,(#147819,#147820,#147821,#147822,#147823,
#147824,#147825,#147826,#147827,#147828,#147829,#147830,#147831,#147832,
#147833,#147834,#147835,#147836,#147837,#147838,#147839,#147840,#147841,
#147842,#147843,#147844,#147845,#147846,#147847,#147848,#147849,#147850,
#147851,#147852,#147853,#147854,#147855,#147856,#147857,#147858,#147859,
#147860,#147861,#147862,#147863,#147864,#147865,#147866,#147867,#147868,
#147869,#147870,#147871,#147872,#147873,#147874,#147875,#147876,#147877,
#147878,#147879,#147880,#147881,#147882,#147883,#147884,#147885,#147886,
#147887,#147888,#147889,#147890,#147891,#147892,#147893,#147894,#147895,
#147896,#147897,#147898,#147899,#147900,#147901,#147902,#147903,#147904,
#147905,#147906,#147907,#147908,#147909,#147910,#147911,#147912,#147913,
#147914,#147915,#147916,#147917,#147918,#147919,#147920,#147921,#147922,
#147923,#147924,#147925,#147926,#147927,#147928,#147929,#147930,#147931,
#147932,#147933,#147934,#147935,#147936,#147937,#147938,#147939,#147940,
#147941,#147942,#147943,#147944,#147945,#147946,#147947,#147948,#147949,
#147950,#147951,#147952,#147953,#147954,#147955,#147956,#147957,#147958,
#147959,#147960,#147961,#147962,#147963,#147964,#147965,#147966,#147967,
#147968,#147969,#147970,#147971,#147972,#147973,#147974,#147975,#147976,
#147977,#147978,#147979,#147980,#147981,#147982,#147983,#147984,#147985,
#147986,#147987,#147988,#147989,#147990,#147991,#147992,#147993,#147994,
#147995,#147996,#147997,#147998,#147999,#148000,#148001,#148002,#148003,
#148004,#148005,#148006,#148007,#148008,#148009,#148010,#148011,#148012,
#148013,#148014,#148015,#148016,#148017,#148018,#148019,#148020,#148021,
#148022,#148023,#148024,#148025,#148026,#148027,#148028,#148029,#148030,
#148031,#148032,#148033,#148034,#148035,#148036,#148037,#148038,#148039,
#148040,#148041,#148042,#148043,#148044,#148045,#148046,#148047,#148048,
#148049,#148050,#148051,#148052,#148053,#148054,#148055,#148056),
 .UNSPECIFIED.,.F.,.F.,(4,3,3,3,3,3,3,3,3,3,3,3,3,3,3,3,3,3,3,3,3,3,3,3,
3,3,3,3,3,3,3,3,3,3,3,3,3,3,3,3,3,3,3,3,3,3,3,3,3,3,3,3,3,3,3,3,3,3,3,3,
3,3,3,3,3,3,3,3,3,3,3,3,3,3,3,3,3,3,3,4),(-173.499058747929,-173.46705307103,
-173.384674116491,-173.302309983779,-173.218878619765,-173.13655670272,
-173.052570615222,-172.968584527723,-172.892944288927,-172.817328056207,
-172.741721359174,-172.666086566588,-172.590436878105,-172.514726458919,
-172.470115984415,-172.378216119382,-172.28618387761,-172.194305017949,
-172.102678297202,-172.011657774091,-171.971647441108,-171.897645181924,
-171.823663908182,-171.749688540053,-171.675675720032,-171.60164410271,
-171.527539003634,-171.4731788978,-171.394217594986,-171.315310285976,-171.236445361765,
-171.157611246176,-171.078796387488,-170.99997523868,-170.921148713993,
-170.842306303387,-170.763437487691,-170.684495547107,-170.605514891192,
-170.526443986869,-170.476241811185,-170.397250490465,-170.318359277892,
-170.239557590234,-170.160858149801,-170.082219258926,-170.003643522044,
-169.977773267877,-169.899184973782,-169.820547207909,-169.741849591751,
-169.663033911633,-169.584150820255,-169.505146053935,-169.47930472457,
-169.400234194684,-169.321236642535,-169.242300383456,-169.163413779317,
-169.084565230139,-169.005738717276,-168.9269243219,-168.848111532234,-168.76928983873,
-168.690421686318,-168.611529876873,-168.532571165133,-168.482367637955,
-168.408257109661,-168.334203555212,-168.260191795563,-168.18619757205,
-168.112215282172,-168.038208133164,-167.983899094647,-167.892990978227,
-167.801368859447,-167.70948624669,-167.617471027762,-167.571942423577),
 .UNSPECIFIED.);
#3071=B_SPLINE_CURVE_WITH_KNOTS('',3,(#148062,#148063,#148064,#148065,#148066,
#148067,#148068,#148069,#148070,#148071,#148072,#148073,#148074,#148075,
#148076,#148077,#148078,#148079,#148080,#148081,#148082,#148083,#148084,
#148085,#148086,#148087,#148088,#148089,#148090,#148091,#148092,#148093,
#148094,#148095,#148096,#148097,#148098,#148099,#148100,#148101,#148102,
#148103,#148104,#148105,#148106,#148107,#148108,#148109,#148110,#148111,
#148112,#148113,#148114,#148115,#148116,#148117,#148118,#148119,#148120,
#148121,#148122,#148123,#148124,#148125,#148126,#148127,#148128,#148129,
#148130,#148131,#148132,#148133,#148134,#148135,#148136,#148137,#148138,
#148139,#148140,#148141,#148142,#148143,#148144,#148145,#148146,#148147,
#148148,#148149,#148150,#148151,#148152,#148153,#148154,#148155,#148156,
#148157,#148158,#148159,#148160,#148161,#148162,#148163,#148164,#148165,
#148166,#148167,#148168,#148169,#148170,#148171,#148172,#148173,#148174,
#148175,#148176,#148177,#148178,#148179,#148180,#148181,#148182,#148183,
#148184,#148185,#148186,#148187,#148188,#148189,#148190,#148191,#148192,
#148193,#148194,#148195,#148196,#148197,#148198,#148199,#148200,#148201,
#148202,#148203,#148204,#148205,#148206,#148207,#148208,#148209,#148210,
#148211,#148212,#148213,#148214,#148215,#148216,#148217,#148218,#148219,
#148220,#148221,#148222,#148223,#148224,#148225,#148226,#148227,#148228,
#148229,#148230,#148231,#148232,#148233,#148234,#148235,#148236,#148237,
#148238,#148239,#148240,#148241,#148242,#148243,#148244,#148245,#148246,
#148247,#148248,#148249,#148250,#148251,#148252,#148253,#148254,#148255,
#148256,#148257,#148258,#148259,#148260,#148261,#148262,#148263,#148264,
#148265,#148266,#148267,#148268,#148269,#148270,#148271,#148272,#148273,
#148274,#148275,#148276,#148277,#148278,#148279,#148280,#148281,#148282,
#148283,#148284,#148285,#148286,#148287,#148288,#148289,#148290,#148291,
#148292,#148293),.UNSPECIFIED.,.F.,.F.,(4,3,3,3,3,3,3,3,3,3,3,3,3,3,3,3,
3,3,3,3,3,3,3,3,3,3,3,3,3,3,3,3,3,3,3,3,3,3,3,3,3,3,3,3,3,3,3,3,3,3,3,3,
3,3,3,3,3,3,3,3,3,3,3,3,3,3,3,3,3,3,3,3,3,3,3,3,3,4),(165.02754145477,165.117918435358,
165.211327921046,165.302367295196,165.396961836652,165.491556378109,165.567514022134,
165.643423783486,165.719300013385,165.795167433697,165.871028965888,165.946918501106,
165.990024921417,166.072127026197,166.15424939746,166.237810414276,166.319981292175,
166.404237378449,166.488493464724,166.570935886981,166.653364296468,166.736763724359,
166.819150225261,166.903056116646,166.986962008032,167.062596601454,167.138207188958,
167.21380824425,167.289437415811,167.365081491186,167.440786333058,167.48543055134,
167.57731665728,167.669334116649,167.761197748819,167.852809518232,167.943816086182,
167.983899094647,168.057905873878,168.131891713771,168.205871692892,168.279889182454,
168.353925506678,168.428035352154,168.482367637955,168.561327246203,168.64023281893,
168.719095969567,168.797928278697,168.876741302422,168.955560584526,169.034385225545,
169.113225739348,169.192092648921,169.271032682423,169.350011430197,169.429080442211,
169.47930472457,169.558298286639,169.637191727285,169.71599562514,169.794697239726,
169.873338280972,169.951916126491,169.977773267877,170.056359443274,170.13499505431,
170.21369048415,170.292503944947,170.371384798467,170.450387315026,170.476241811185,
170.559521333102,170.642694489389,170.725698825545,170.808594331111,170.891316876558,
170.955112984985),.UNSPECIFIED.);
#3072=B_SPLINE_CURVE_WITH_KNOTS('',3,(#148294,#148295,#148296,#148297,#148298,
#148299,#148300,#148301,#148302,#148303,#148304,#148305,#148306,#148307,
#148308,#148309),.UNSPECIFIED.,.F.,.F.,(4,3,3,3,3,4),(170.95511468872,171.037715426029,
171.120454088486,171.203260261769,171.286161630498,171.311431343321),
 .UNSPECIFIED.);
#3073=B_SPLINE_CURVE_WITH_KNOTS('',3,(#148311,#148312,#148313,#148314,#148315,
#148316,#148317,#148318,#148319,#148320,#148321,#148322,#148323,#148324,
#148325,#148326),.UNSPECIFIED.,.F.,.F.,(4,3,3,3,3,4),(-167.571942423577,
-167.485430551339,-167.409258995797,-167.333137055842,-167.257054247403,
-167.21587344088),.UNSPECIFIED.);
#3074=B_SPLINE_CURVE_WITH_KNOTS('',3,(#148327,#148328,#148329,#148330,#148331,
#148332,#148333,#148334,#148335,#148336,#148337,#148338,#148339,#148340,
#148341,#148342,#148343,#148344,#148345,#148346,#148347,#148348,#148349,
#148350,#148351,#148352,#148353,#148354,#148355,#148356,#148357,#148358,
#148359,#148360,#148361,#148362,#148363,#148364,#148365,#148366,#148367,
#148368,#148369,#148370,#148371,#148372,#148373,#148374,#148375,#148376,
#148377,#148378,#148379,#148380,#148381,#148382,#148383,#148384,#148385,
#148386,#148387,#148388,#148389,#148390,#148391,#148392,#148393,#148394,
#148395,#148396,#148397,#148398,#148399,#148400,#148401,#148402,#148403,
#148404,#148405,#148406,#148407,#148408,#148409,#148410,#148411,#148412,
#148413,#148414,#148415,#148416,#148417,#148418,#148419,#148420,#148421,
#148422,#148423,#148424,#148425,#148426,#148427,#148428,#148429,#148430,
#148431,#148432,#148433,#148434,#148435,#148436,#148437,#148438,#148439,
#148440,#148441,#148442,#148443,#148444,#148445,#148446,#148447,#148448,
#148449,#148450,#148451,#148452,#148453,#148454,#148455,#148456,#148457,
#148458,#148459,#148460,#148461,#148462,#148463,#148464,#148465,#148466,
#148467,#148468,#148469,#148470,#148471,#148472,#148473,#148474,#148475,
#148476,#148477,#148478,#148479,#148480,#148481,#148482,#148483,#148484,
#148485,#148486,#148487,#148488,#148489,#148490,#148491,#148492,#148493,
#148494,#148495,#148496,#148497,#148498,#148499,#148500,#148501,#148502,
#148503,#148504,#148505,#148506,#148507,#148508,#148509,#148510,#148511,
#148512,#148513,#148514,#148515,#148516,#148517,#148518,#148519,#148520,
#148521,#148522,#148523,#148524,#148525,#148526,#148527,#148528,#148529,
#148530,#148531,#148532,#148533,#148534,#148535,#148536,#148537,#148538,
#148539,#148540,#148541,#148542,#148543,#148544,#148545,#148546),
 .UNSPECIFIED.,.F.,.F.,(4,3,3,3,3,3,3,3,3,3,3,3,3,3,3,3,3,3,3,3,3,3,3,3,
3,3,3,3,3,3,3,3,3,3,3,3,3,3,3,3,3,3,3,3,3,3,3,3,3,3,3,3,3,3,3,3,3,3,3,3,
3,3,3,3,3,3,3,3,3,3,3,3,3,4),(-167.21587344088,-167.134143567114,-167.052413813343,
-166.970684177902,-166.888954659123,-166.807225255339,-166.725495964884,
-166.640549196365,-166.556929721104,-166.474616800144,-166.392877891077,
-166.31113940169,-166.229401325311,-166.147663655263,-166.065926384875,
-165.984189507472,-165.902453016381,-165.820716904931,-165.738981166449,
-165.657245794263,-165.575510781701,-165.493776122092,-165.412041808764,
-165.330307835048,-165.248574194272,-165.166840879767,-165.085107884863,
-165.003375202889,-164.921642827178,-164.839910751058,-164.758178967863,
-164.676447470922,-164.594716253569,-164.512985309134,-164.431254630949,
-164.349524212349,-164.267794046663,-164.186064127227,-164.104334447371,
-164.022605000431,-163.937176806032,-163.854418242708,-163.772679615145,
-163.690941811341,-163.609204804601,-163.527468568233,-163.445733075548,
-163.363998299857,-163.282264214476,-163.200530792723,-163.118798007918,
-163.037065833383,-162.955334242442,-162.873603208421,-162.791872704648,
-162.710142704454,-162.628413181169,-162.544693781075,-162.462955700046,
-162.381219204622,-162.299484188037,-162.217750543549,-162.136018164432,
-162.054286943979,-161.972556775498,-161.887100026018,-161.805363107799,
-161.723629098896,-161.641897572377,-161.560168101449,-161.478433210973,
-161.396703130808,-161.314971701746,-161.288902779658),.UNSPECIFIED.);
#3075=B_SPLINE_CURVE_WITH_KNOTS('',3,(#148552,#148553,#148554,#148555,#148556,
#148557,#148558,#148559,#148560,#148561,#148562,#148563,#148564,#148565,
#148566,#148567,#148568,#148569,#148570,#148571,#148572,#148573,#148574,
#148575,#148576,#148577,#148578,#148579,#148580,#148581,#148582,#148583,
#148584,#148585,#148586,#148587,#148588,#148589,#148590,#148591,#148592,
#148593,#148594,#148595,#148596,#148597,#148598,#148599,#148600,#148601,
#148602,#148603,#148604,#148605,#148606,#148607,#148608,#148609,#148610,
#148611,#148612,#148613,#148614,#148615,#148616,#148617,#148618,#148619,
#148620,#148621,#148622,#148623,#148624,#148625,#148626,#148627,#148628,
#148629,#148630,#148631,#148632,#148633,#148634,#148635,#148636,#148637,
#148638,#148639,#148640,#148641,#148642,#148643,#148644,#148645,#148646,
#148647,#148648,#148649,#148650,#148651,#148652,#148653,#148654,#148655,
#148656,#148657,#148658,#148659,#148660,#148661,#148662,#148663,#148664,
#148665,#148666,#148667,#148668,#148669,#148670,#148671,#148672,#148673,
#148674,#148675,#148676,#148677,#148678,#148679,#148680,#148681,#148682,
#148683,#148684,#148685,#148686,#148687,#148688,#148689,#148690,#148691,
#148692,#148693,#148694,#148695,#148696,#148697,#148698,#148699,#148700,
#148701,#148702,#148703,#148704,#148705,#148706,#148707,#148708,#148709,
#148710,#148711,#148712,#148713,#148714,#148715,#148716,#148717,#148718,
#148719,#148720,#148721,#148722,#148723,#148724,#148725,#148726,#148727,
#148728,#148729,#148730,#148731,#148732,#148733,#148734,#148735,#148736,
#148737,#148738,#148739,#148740,#148741,#148742,#148743,#148744,#148745,
#148746,#148747,#148748,#148749,#148750,#148751,#148752,#148753,#148754,
#148755,#148756,#148757,#148758,#148759,#148760,#148761,#148762,#148763,
#148764,#148765,#148766,#148767,#148768,#148769,#148770,#148771),
 .UNSPECIFIED.,.F.,.F.,(4,3,3,3,3,3,3,3,3,3,3,3,3,3,3,3,3,3,3,3,3,3,3,3,
3,3,3,3,3,3,3,3,3,3,3,3,3,3,3,3,3,3,3,3,3,3,3,3,3,3,3,3,3,3,3,3,3,3,3,3,
3,3,3,3,3,3,3,3,3,3,3,3,3,4),(158.744957016583,158.82668689035,158.90841664412,
158.990146279561,159.07187579834,159.153605202124,159.235334492578,159.320281261098,
159.403900736359,159.486213657319,159.567952566386,159.649691055772,159.731429132152,
159.8131668022,159.894904072588,159.976640949991,160.058377441081,160.140113552531,
160.221849291013,160.3035846632,160.385319675762,160.467054335371,160.548788648698,
160.630522622414,160.71225626319,160.793989577695,160.8757225726,160.957455254573,
161.039187630285,161.120919706404,161.2026514896,161.28438298654,161.366114203894,
161.447845148329,161.529575826513,161.611306245114,161.693036410799,161.774766330236,
161.856496010091,161.938225457032,162.023653651431,162.106412214755,162.188150842318,
162.269888646122,162.351625652862,162.43336188923,162.515097381915,162.596832157606,
162.678566242987,162.76029966474,162.842032449545,162.92376462408,163.005496215021,
163.087227249042,163.168957752814,163.250687753009,163.332417276294,163.416136676388,
163.497874757417,163.579611252841,163.661346269426,163.743079913914,163.824812293031,
163.906543513484,163.988273681965,164.073730431445,164.155467349664,164.237201358567,
164.318932885086,164.400662356015,164.48239724649,164.564127326655,164.645858755717,
164.671927677806),.UNSPECIFIED.);
#3076=B_SPLINE_CURVE_WITH_KNOTS('',3,(#148772,#148773,#148774,#148775,#148776,
#148777,#148778,#148779,#148780,#148781,#148782,#148783,#148784,#148785,
#148786,#148787,#148788,#148789,#148790),.UNSPECIFIED.,.F.,.F.,(4,3,3,3,
3,3,4),(164.672427783019,164.744041659808,164.8156404277,164.88722929276,
164.958841893886,164.993087834802,165.02754145477),.UNSPECIFIED.);
#3077=B_SPLINE_CURVE_WITH_KNOTS('',3,(#148792,#148793,#148794,#148795,#148796,
#148797,#148798,#148799,#148800,#148801,#148802,#148803,#148804,#148805,
#148806,#148807),.UNSPECIFIED.,.F.,.F.,(4,3,3,3,3,4),(-161.288902779658,
-161.207173235822,-161.125438120903,-161.043707883554,-160.961976094603,
-160.9326881337),.UNSPECIFIED.);
#3078=B_SPLINE_CURVE_WITH_KNOTS('',3,(#148808,#148809,#148810,#148811,#148812,
#148813,#148814,#148815,#148816,#148817,#148818,#148819,#148820,#148821,
#148822,#148823,#148824,#148825,#148826,#148827,#148828,#148829,#148830,
#148831,#148832,#148833,#148834,#148835,#148836,#148837,#148838,#148839,
#148840,#148841,#148842,#148843,#148844,#148845,#148846,#148847,#148848,
#148849,#148850,#148851,#148852,#148853,#148854,#148855,#148856,#148857,
#148858,#148859,#148860,#148861,#148862,#148863,#148864,#148865,#148866,
#148867,#148868,#148869,#148870,#148871,#148872,#148873,#148874,#148875,
#148876,#148877,#148878,#148879,#148880,#148881,#148882,#148883,#148884,
#148885,#148886,#148887,#148888,#148889,#148890,#148891,#148892,#148893,
#148894,#148895,#148896,#148897,#148898,#148899,#148900,#148901,#148902,
#148903,#148904,#148905,#148906,#148907,#148908,#148909,#148910,#148911,
#148912,#148913,#148914,#148915,#148916,#148917,#148918,#148919,#148920,
#148921,#148922,#148923,#148924,#148925,#148926,#148927,#148928,#148929,
#148930,#148931,#148932,#148933,#148934,#148935,#148936,#148937,#148938,
#148939,#148940,#148941,#148942,#148943,#148944,#148945,#148946,#148947,
#148948,#148949,#148950,#148951,#148952,#148953,#148954,#148955,#148956,
#148957,#148958,#148959,#148960,#148961,#148962,#148963,#148964,#148965,
#148966,#148967,#148968,#148969,#148970,#148971,#148972,#148973,#148974,
#148975,#148976,#148977,#148978,#148979,#148980,#148981,#148982,#148983,
#148984,#148985,#148986,#148987,#148988,#148989,#148990,#148991,#148992,
#148993,#148994,#148995,#148996,#148997,#148998,#148999,#149000,#149001,
#149002,#149003,#149004,#149005,#149006,#149007,#149008,#149009,#149010,
#149011,#149012,#149013,#149014,#149015,#149016,#149017,#149018,#149019,
#149020,#149021,#149022,#149023,#149024,#149025,#149026,#149027,#149028,
#149029,#149030,#149031,#149032,#149033,#149034,#149035,#149036,#149037,
#149038,#149039,#149040,#149041,#149042,#149043,#149044,#149045),
 .UNSPECIFIED.,.F.,.F.,(4,3,3,3,3,3,3,3,3,3,3,3,3,3,3,3,3,3,3,3,3,3,3,3,
3,3,3,3,3,3,3,3,3,3,3,3,3,3,3,3,3,3,3,3,3,3,3,3,3,3,3,3,3,3,3,3,3,3,3,3,
3,3,3,3,3,3,3,3,3,3,3,3,3,3,3,3,3,3,3,4),(-160.9326881337,-160.851753714582,
-160.770640585143,-160.689254829997,-160.607715595427,-160.525950020712,
-160.506870945034,-160.429026496388,-160.351272650518,-160.273595290889,
-160.195980354179,-160.118413820932,-160.040878611182,-159.963359829769,
-159.885844826791,-159.808320956824,-159.730742760459,-159.653137126767,
-159.575447421521,-159.509933858419,-159.431228794851,-159.352592103808,
-159.274012702095,-159.195486763226,-159.116992780832,-159.038519564958,
-159.011465315111,-158.929812605011,-158.848093681957,-158.764319454419,
-158.682430650419,-158.597713711111,-158.512996771803,-158.431594055443,
-158.350260504194,-158.266327435269,-158.185145307839,-158.099836768167,
-158.014528228496,-157.935506745639,-157.856463939296,-157.777390015581,
-157.698242168605,-157.619052686286,-157.53978064037,-157.516059685188,
-157.438550009036,-157.361107114613,-157.283716716122,-157.206364564723,
-157.129036439365,-157.051701752493,-156.974360228904,-156.896998990283,
-156.819605149562,-156.74211896366,-156.664584530957,-156.586930454071,
-156.519122598573,-156.443888371344,-156.368748377998,-156.293686181249,
-156.218685427187,-156.143729825913,-156.066036786669,-155.991108027357,
-155.916172470055,-155.841215430626,-155.76622220858,-155.691136858506,
-155.615996739876,-155.54074829231,-155.522185511958,-155.444955082429,
-155.367811457943,-155.290741127077,-155.213741865405,-155.13678410832,
-155.059853433246,-155.005663677983),.UNSPECIFIED.);
#3079=B_SPLINE_CURVE_WITH_KNOTS('',3,(#149051,#149052,#149053,#149054,#149055,
#149056,#149057,#149058,#149059,#149060,#149061,#149062,#149063,#149064,
#149065,#149066,#149067,#149068,#149069,#149070,#149071,#149072,#149073,
#149074,#149075,#149076,#149077,#149078,#149079,#149080,#149081,#149082,
#149083,#149084,#149085,#149086,#149087,#149088,#149089,#149090,#149091,
#149092,#149093,#149094,#149095,#149096,#149097,#149098,#149099,#149100,
#149101,#149102,#149103,#149104,#149105,#149106,#149107,#149108,#149109,
#149110,#149111,#149112,#149113,#149114,#149115,#149116,#149117,#149118,
#149119,#149120,#149121,#149122,#149123,#149124,#149125,#149126,#149127,
#149128,#149129,#149130,#149131,#149132,#149133,#149134,#149135,#149136,
#149137,#149138,#149139,#149140,#149141,#149142,#149143,#149144,#149145,
#149146,#149147,#149148,#149149,#149150,#149151,#149152,#149153,#149154,
#149155,#149156,#149157,#149158,#149159,#149160,#149161,#149162,#149163,
#149164,#149165,#149166,#149167,#149168,#149169,#149170,#149171,#149172,
#149173,#149174,#149175,#149176,#149177,#149178,#149179,#149180,#149181,
#149182,#149183,#149184,#149185,#149186,#149187,#149188,#149189,#149190,
#149191,#149192,#149193,#149194,#149195,#149196,#149197,#149198,#149199,
#149200,#149201,#149202,#149203,#149204,#149205,#149206,#149207,#149208,
#149209,#149210,#149211,#149212,#149213,#149214,#149215,#149216,#149217,
#149218,#149219,#149220,#149221,#149222,#149223,#149224,#149225,#149226,
#149227,#149228,#149229,#149230,#149231,#149232,#149233,#149234,#149235,
#149236,#149237,#149238,#149239,#149240,#149241,#149242,#149243,#149244,
#149245,#149246,#149247,#149248,#149249,#149250,#149251,#149252,#149253,
#149254,#149255,#149256,#149257,#149258,#149259,#149260,#149261,#149262,
#149263,#149264,#149265,#149266,#149267,#149268,#149269,#149270,#149271,
#149272,#149273,#149274,#149275,#149276,#149277,#149278,#149279,#149280,
#149281,#149282,#149283,#149284,#149285,#149286,#149287,#149288,#149289,
#149290,#149291),.UNSPECIFIED.,.F.,.F.,(4,3,3,3,3,3,3,3,3,3,3,3,3,3,3,3,
3,3,3,3,3,3,3,3,3,3,3,3,3,3,3,3,3,3,3,3,3,3,3,3,3,3,3,3,3,3,3,3,3,3,3,3,
3,3,3,3,3,3,3,3,3,3,3,3,3,3,3,3,3,3,3,3,3,3,3,3,3,3,3,3,4),(152.461872548045,
152.531374252113,152.608905049108,152.686380993047,152.76381497896,152.841222846017,
152.918615169387,152.996015244036,153.02984279542,153.108966009833,153.188092851743,
153.267233018585,153.346420626813,153.425634399544,153.50490824031,153.528311338728,
153.613266920936,153.698202335754,153.783065063921,153.867859507684,153.952513587944,
154.026779882035,154.104294440241,154.181804546132,154.259322876478,154.336889387948,
154.414483072056,154.492147142944,154.525248425343,154.603042406765,154.680774851418,
154.758459588496,154.836110412816,154.913741093835,154.991382886643,155.069034149677,
155.146707365294,155.224415026398,155.302215990995,155.380066106682,155.458034270177,
155.522185511958,155.597418690668,155.672557806474,155.747619295678,155.822619511427,
155.897574743044,155.975268224986,156.050197038596,156.125132807108,156.200090214791,
156.275083962399,156.350170069209,156.425311080461,156.50056061365,156.519122598573,
156.596785594421,156.674356120084,156.751848550961,156.829277208533,156.906656369881,
156.984003284394,157.061333319959,157.138659355257,157.215994264305,157.293384539171,
157.37080265027,157.448307120662,157.516059685188,157.595324306327,157.674520101997,
157.753656985933,157.83273536786,157.911778254531,157.990793017878,158.014528228496,
158.093583812149,158.172704056942,158.251857104928,158.331092251217,158.388376241259),
 .UNSPECIFIED.);
#3080=B_SPLINE_CURVE_WITH_KNOTS('',3,(#149292,#149293,#149294,#149295,#149296,
#149297,#149298,#149299,#149300,#149301,#149302,#149303,#149304,#149305,
#149306,#149307),.UNSPECIFIED.,.F.,.F.,(4,3,3,3,3,4),(158.388742370626,
158.470471914462,158.552207029381,158.63393726673,158.715669055681,158.744957016583),
 .UNSPECIFIED.);
#3081=B_SPLINE_CURVE_WITH_KNOTS('',3,(#149309,#149310,#149311,#149312,#149313,
#149314,#149315,#149316,#149317,#149318,#149319,#149320,#149321,#149322,
#149323,#149324),.UNSPECIFIED.,.F.,.F.,(4,3,3,3,3,4),(-155.005663677983,
-154.928750365625,-154.851804570041,-154.77484175986,-154.697816546421,
-154.649502826602),.UNSPECIFIED.);
#3082=B_SPLINE_CURVE_WITH_KNOTS('',3,(#149325,#149326,#149327,#149328,#149329,
#149330,#149331,#149332,#149333,#149334,#149335,#149336,#149337,#149338,
#149339,#149340,#149341,#149342,#149343,#149344,#149345,#149346,#149347,
#149348,#149349,#149350,#149351,#149352,#149353,#149354,#149355,#149356,
#149357,#149358,#149359,#149360,#149361,#149362,#149363,#149364,#149365,
#149366,#149367,#149368,#149369,#149370,#149371,#149372,#149373,#149374,
#149375,#149376,#149377,#149378,#149379,#149380,#149381,#149382,#149383,
#149384,#149385,#149386,#149387,#149388,#149389,#149390,#149391,#149392,
#149393,#149394,#149395,#149396,#149397,#149398,#149399,#149400,#149401,
#149402,#149403,#149404,#149405,#149406,#149407,#149408,#149409,#149410,
#149411,#149412,#149413,#149414,#149415,#149416,#149417,#149418,#149419,
#149420,#149421,#149422,#149423,#149424,#149425,#149426,#149427,#149428,
#149429,#149430,#149431,#149432,#149433,#149434,#149435,#149436,#149437,
#149438,#149439,#149440,#149441,#149442,#149443,#149444,#149445,#149446,
#149447,#149448,#149449,#149450,#149451,#149452,#149453,#149454,#149455,
#149456,#149457,#149458,#149459,#149460,#149461,#149462,#149463,#149464,
#149465,#149466,#149467,#149468,#149469,#149470,#149471,#149472,#149473,
#149474,#149475,#149476,#149477,#149478,#149479,#149480,#149481,#149482,
#149483,#149484,#149485,#149486,#149487,#149488,#149489,#149490,#149491,
#149492,#149493,#149494,#149495,#149496,#149497,#149498,#149499,#149500,
#149501,#149502,#149503,#149504,#149505,#149506,#149507,#149508,#149509,
#149510,#149511,#149512,#149513,#149514,#149515,#149516,#149517,#149518,
#149519,#149520,#149521,#149522,#149523,#149524,#149525,#149526,#149527,
#149528,#149529,#149530,#149531,#149532,#149533,#149534,#149535,#149536,
#149537,#149538,#149539,#149540,#149541,#149542,#149543,#149544,#149545,
#149546,#149547,#149548,#149549,#149550,#149551,#149552,#149553,#149554,
#149555,#149556,#149557,#149558,#149559,#149560,#149561,#149562),
 .UNSPECIFIED.,.F.,.F.,(4,3,3,3,3,3,3,3,3,3,3,3,3,3,3,3,3,3,3,3,3,3,3,3,
3,3,3,3,3,3,3,3,3,3,3,3,3,3,3,3,3,3,3,3,3,3,3,3,3,3,3,3,3,3,3,3,3,3,3,3,
3,3,3,3,3,3,3,3,3,3,3,3,3,3,3,3,3,3,3,4),(-154.649502826521,-154.525248425343,
-154.447587709264,-154.369984567194,-154.29242625479,-154.214898763173,
-154.137389544905,-154.059877070554,-154.026779882035,-153.942155713893,
-153.857420741895,-153.772553364838,-153.687641000974,-153.602685811278,
-153.528311338728,-153.449042151582,-153.369823495967,-153.290645602546,
-153.211499792603,-153.132374156501,-153.053254885006,-153.02984279542,
-152.952441049764,-152.875047326639,-152.797648790269,-152.720206658767,
-152.642740007134,-152.565206289548,-152.531374252113,-152.441611266669,
-152.351813698248,-152.262177425072,-152.172732395101,-152.083727450608,
-152.032905708805,-151.958589664459,-151.884292438208,-151.809999042985,
-151.735665740119,-151.661311952551,-151.586883380113,-151.534437165498,
-151.455503202959,-151.376623859828,-151.297787454988,-151.218982340526,
-151.140196893334,-151.061405591473,-150.982609139477,-150.903796964785,
-150.824958485864,-150.746046820653,-150.667096413218,-150.588055433093,
-150.537500078883,-150.458590748963,-150.379781364379,-150.301061176057,
-150.222442401086,-150.143883589462,-150.065386817239,-150.039031535575,
-149.960384680215,-149.881686893022,-149.802927930414,-149.724049334714,
-149.645102435641,-149.566032998171,-149.540562992267,-149.461498149583,
-149.382507986401,-149.29998865198,-149.221122885299,-149.142291855357,
-149.063484993942,-148.984691749771,-148.905888638323,-148.827080945834,
-148.748242150062,-148.722353311028),.UNSPECIFIED.);
#3083=B_SPLINE_CURVE_WITH_KNOTS('',3,(#149568,#149569,#149570,#149571,#149572,
#149573,#149574,#149575,#149576,#149577,#149578,#149579,#149580,#149581,
#149582,#149583,#149584,#149585,#149586,#149587,#149588,#149589,#149590,
#149591,#149592,#149593,#149594,#149595,#149596,#149597,#149598,#149599,
#149600,#149601,#149602,#149603,#149604,#149605,#149606,#149607,#149608,
#149609,#149610,#149611,#149612,#149613,#149614,#149615,#149616,#149617,
#149618,#149619,#149620,#149621,#149622,#149623,#149624,#149625,#149626,
#149627,#149628,#149629,#149630,#149631,#149632,#149633,#149634,#149635,
#149636,#149637,#149638,#149639,#149640,#149641,#149642,#149643,#149644,
#149645,#149646,#149647,#149648,#149649,#149650,#149651,#149652,#149653,
#149654,#149655,#149656,#149657,#149658,#149659,#149660,#149661,#149662,
#149663,#149664,#149665,#149666,#149667,#149668,#149669,#149670,#149671,
#149672,#149673,#149674,#149675,#149676,#149677,#149678,#149679,#149680,
#149681,#149682,#149683,#149684,#149685,#149686,#149687,#149688,#149689,
#149690,#149691,#149692,#149693,#149694,#149695,#149696,#149697,#149698,
#149699,#149700,#149701,#149702,#149703,#149704,#149705,#149706,#149707,
#149708,#149709,#149710,#149711,#149712,#149713,#149714,#149715,#149716,
#149717,#149718,#149719,#149720,#149721,#149722,#149723,#149724,#149725,
#149726,#149727,#149728,#149729,#149730,#149731,#149732,#149733,#149734,
#149735,#149736,#149737,#149738,#149739,#149740,#149741,#149742,#149743,
#149744,#149745,#149746,#149747,#149748,#149749,#149750,#149751,#149752,
#149753,#149754,#149755,#149756,#149757,#149758,#149759,#149760,#149761,
#149762,#149763,#149764,#149765,#149766,#149767,#149768,#149769,#149770,
#149771,#149772,#149773,#149774,#149775,#149776,#149777,#149778,#149779,
#149780,#149781,#149782,#149783,#149784,#149785,#149786,#149787),
 .UNSPECIFIED.,.F.,.F.,(4,3,3,3,3,3,3,3,3,3,3,3,3,3,3,3,3,3,3,3,3,3,3,3,
3,3,3,3,3,3,3,3,3,3,3,3,3,3,3,3,3,3,3,3,3,3,3,3,3,3,3,3,3,3,3,3,3,3,3,3,
3,3,3,3,3,3,3,3,3,3,3,3,3,4),(146.178586402224,146.260316275991,146.342046029761,
146.423775665203,146.505505183982,146.587234587766,146.66896387822,146.753910646739,
146.837530122,146.91984304296,147.001581952028,147.083320441414,147.165058517794,
147.246796187842,147.32853345823,147.410270335633,147.492006826723,147.573742938173,
147.655478676655,147.737214048842,147.818949061404,147.900683721013,147.98241803434,
148.064152008057,148.145885648832,148.227618963337,148.309351958242,148.391084640215,
148.472817015927,148.554549092046,148.636280875242,148.718012372182,148.799743589536,
148.881474533971,148.963205212155,149.044935630756,149.126665796441,149.208395715878,
149.290125395733,149.371854842673,149.457283037073,149.540041600397,149.62178022796,
149.703518031764,149.785255038504,149.866991274872,149.948726767557,150.030461543248,
150.112195628629,150.193929050381,150.275661835186,150.357394009722,150.439125600663,
150.520856634684,150.602587138456,150.684317138651,150.766046661936,150.84976606203,
150.931504143059,151.013240638483,151.094975655068,151.176709299556,151.258441678673,
151.340172899126,151.421903067606,151.507359817086,151.589096735305,151.670830744209,
151.752562270728,151.834291741656,151.916026632132,151.997756712297,152.079488141359,
152.105557063447),.UNSPECIFIED.);
#3084=B_SPLINE_CURVE_WITH_KNOTS('',3,(#149788,#149789,#149790,#149791,#149792,
#149793,#149794,#149795,#149796,#149797,#149798,#149799,#149800),
 .UNSPECIFIED.,.F.,.F.,(4,3,3,3,4),(152.105557063447,152.195632841689,152.285955846226,
152.37647093208,152.461872548045),.UNSPECIFIED.);
#3085=B_SPLINE_CURVE_WITH_KNOTS('',3,(#149802,#149803,#149804,#149805,#149806,
#149807,#149808,#149809,#149810,#149811,#149812,#149813,#149814,#149815,
#149816,#149817),.UNSPECIFIED.,.F.,.F.,(4,3,3,3,3,4),(-148.722353311028,
-148.643465082527,-148.564514557937,-148.543625905652,-148.454971712497,
-148.366317519341),.UNSPECIFIED.);
#3086=B_SPLINE_CURVE_WITH_KNOTS('',3,(#149818,#149819,#149820,#149821,#149822,
#149823,#149824,#149825,#149826,#149827,#149828,#149829,#149830,#149831,
#149832,#149833,#149834,#149835,#149836,#149837,#149838,#149839,#149840,
#149841,#149842,#149843,#149844,#149845,#149846,#149847,#149848,#149849,
#149850,#149851,#149852,#149853,#149854,#149855,#149856,#149857,#149858,
#149859,#149860,#149861,#149862,#149863,#149864,#149865,#149866,#149867,
#149868,#149869,#149870,#149871,#149872,#149873,#149874,#149875,#149876,
#149877,#149878,#149879,#149880,#149881,#149882,#149883,#149884,#149885,
#149886,#149887,#149888,#149889,#149890,#149891,#149892,#149893,#149894,
#149895,#149896,#149897,#149898,#149899,#149900,#149901,#149902,#149903,
#149904,#149905,#149906,#149907,#149908,#149909,#149910,#149911,#149912,
#149913,#149914,#149915,#149916,#149917,#149918,#149919,#149920,#149921,
#149922,#149923,#149924,#149925,#149926,#149927,#149928,#149929,#149930,
#149931,#149932,#149933,#149934,#149935,#149936,#149937,#149938,#149939,
#149940,#149941,#149942,#149943,#149944,#149945,#149946,#149947,#149948,
#149949,#149950,#149951,#149952,#149953,#149954,#149955,#149956,#149957,
#149958,#149959,#149960,#149961,#149962,#149963,#149964,#149965,#149966,
#149967,#149968,#149969,#149970,#149971,#149972,#149973,#149974,#149975,
#149976,#149977,#149978,#149979,#149980,#149981,#149982,#149983,#149984,
#149985,#149986,#149987,#149988,#149989,#149990,#149991,#149992,#149993,
#149994,#149995,#149996,#149997,#149998,#149999,#150000,#150001,#150002,
#150003,#150004,#150005,#150006,#150007,#150008,#150009,#150010,#150011,
#150012,#150013,#150014,#150015,#150016,#150017,#150018,#150019,#150020,
#150021,#150022,#150023,#150024,#150025,#150026,#150027,#150028,#150029,
#150030,#150031,#150032,#150033,#150034,#150035,#150036,#150037,#150038,
#150039,#150040,#150041,#150042,#150043,#150044,#150045,#150046,#150047,
#150048,#150049,#150050,#150051,#150052,#150053,#150054,#150055),
 .UNSPECIFIED.,.F.,.F.,(4,3,3,3,3,3,3,3,3,3,3,3,3,3,3,3,3,3,3,3,3,3,3,3,
3,3,3,3,3,3,3,3,3,3,3,3,3,3,3,3,3,3,3,3,3,3,3,3,3,3,3,3,3,3,3,3,3,3,3,3,
3,3,3,3,3,3,3,3,3,3,3,3,3,3,3,3,3,3,3,4),(-148.36631751921,-148.295097778499,
-148.223893167673,-148.152698698807,-148.081479920567,-148.045157362345,
-147.954159342607,-147.862657150356,-147.770714478799,-147.678680645011,
-147.586772073684,-147.546688819037,-147.470982507544,-147.395324882409,
-147.319701434226,-147.244087145053,-147.168479062259,-147.092842558515,
-147.04822027573,-146.965936488568,-146.883628796585,-146.800159530544,
-146.717799306148,-146.633775519285,-146.549751732422,-146.467376065816,
-146.385015272141,-146.301582251385,-146.219263712141,-146.135273450628,
-146.051283189114,-145.97564198174,-145.90002477354,-145.824417094708,-145.748781313446,
-145.673130631722,-145.597419216424,-145.552814645807,-145.46091508944,
-145.368883184751,-145.277004679384,-145.185378310241,-145.094358120478,
-145.054346102499,-144.980344107589,-144.906363098792,-144.832387996217,
-144.758375442111,-144.684344091165,-144.610239258084,-144.555877559192,
-144.476916121412,-144.398008675984,-144.319143614219,-144.240309360249,
-144.161494362667,-144.082673075002,-144.00384641167,-143.925003862908,
-143.846134909821,-143.767192833972,-143.688212043952,-143.609141008602,
-143.558940472577,-143.479948660699,-143.401056959162,-143.322254785764,
-143.243554866504,-143.16491550145,-143.086339298753,-143.060471929269,
-142.981885159439,-142.903248944468,-142.824552902507,-142.745738821302,
-142.666857342744,-142.587854198644,-142.562003385962,-142.478726056179,
-142.439142960337),.UNSPECIFIED.);
#3087=B_SPLINE_CURVE_WITH_KNOTS('',3,(#150061,#150062,#150063,#150064,#150065,
#150066,#150067,#150068,#150069,#150070,#150071,#150072,#150073,#150074,
#150075,#150076,#150077,#150078,#150079,#150080,#150081,#150082,#150083,
#150084,#150085,#150086,#150087,#150088,#150089,#150090,#150091,#150092,
#150093,#150094,#150095,#150096,#150097,#150098,#150099,#150100,#150101,
#150102,#150103,#150104,#150105,#150106,#150107,#150108,#150109,#150110,
#150111,#150112,#150113,#150114,#150115,#150116,#150117,#150118,#150119,
#150120,#150121,#150122,#150123,#150124,#150125,#150126,#150127,#150128,
#150129,#150130,#150131,#150132,#150133,#150134,#150135,#150136,#150137,
#150138,#150139,#150140,#150141,#150142,#150143,#150144,#150145,#150146,
#150147,#150148,#150149,#150150,#150151,#150152,#150153,#150154,#150155,
#150156,#150157,#150158,#150159,#150160,#150161,#150162,#150163,#150164,
#150165,#150166,#150167,#150168,#150169,#150170,#150171,#150172,#150173,
#150174,#150175,#150176,#150177,#150178,#150179,#150180,#150181,#150182,
#150183,#150184,#150185,#150186,#150187,#150188,#150189,#150190,#150191,
#150192,#150193,#150194,#150195,#150196,#150197,#150198,#150199,#150200,
#150201,#150202,#150203,#150204,#150205,#150206,#150207,#150208,#150209,
#150210,#150211,#150212,#150213,#150214,#150215,#150216,#150217,#150218,
#150219,#150220,#150221,#150222,#150223,#150224,#150225,#150226,#150227,
#150228,#150229,#150230,#150231,#150232,#150233,#150234,#150235,#150236,
#150237,#150238,#150239,#150240,#150241,#150242,#150243,#150244,#150245,
#150246,#150247,#150248,#150249,#150250,#150251,#150252,#150253,#150254,
#150255,#150256,#150257,#150258,#150259,#150260,#150261,#150262,#150263,
#150264,#150265,#150266,#150267,#150268,#150269,#150270,#150271,#150272,
#150273,#150274,#150275,#150276,#150277,#150278,#150279,#150280,#150281,
#150282,#150283,#150284,#150285,#150286,#150287,#150288,#150289,#150290,
#150291,#150292,#150293,#150294,#150295,#150296,#150297,#150298,#150299,
#150300,#150301),.UNSPECIFIED.,.F.,.F.,(4,3,3,3,3,3,3,3,3,3,3,3,3,3,3,3,
3,3,3,3,3,3,3,3,3,3,3,3,3,3,3,3,3,3,3,3,3,3,3,3,3,3,3,3,3,3,3,3,3,3,3,3,
3,3,3,3,3,3,3,3,3,3,3,3,3,3,3,3,3,3,3,3,3,3,3,3,3,3,3,3,4),(139.895602067557,
139.977901874986,140.060171044567,140.069660669424,140.145300773922,140.220916872101,
140.296523434427,140.372158092422,140.447807646289,140.52351793138,140.568129212731,
140.660029796919,140.752062781502,140.843942365698,140.935569775318,141.02659090873,
141.066597756039,141.140599667601,141.214580592822,141.288555611617,141.362568081812,
141.436599348694,141.51070409782,141.565066299346,141.644027707974,141.722935123658,
141.80180015516,141.88063437842,141.959449344918,142.038270601121,142.117097232801,
142.195939749784,142.27480867103,142.353750715161,142.432731473525,142.511802477606,
142.562003385962,142.640995331965,142.719887166777,142.79868947233,142.877389521512,
142.95602901502,143.034605343613,143.060471929269,143.139058572594,143.217694658848,
143.296390570157,143.37520451866,143.454085863362,143.533088872827,143.558940472577,
143.638013018572,143.717012597661,143.795950889894,143.874839528783,143.953690109694,
144.032518638095,144.11133503593,144.19014981086,144.268973468316,144.347843538777,
144.426737240448,144.505697787184,144.555877559192,144.629983078104,144.704031656759,
144.778038475533,144.852027820258,144.926005262392,145.000007628607,145.054346102499,
145.145344259658,145.236846452989,145.328788914312,145.420822418235,145.512730496857,
145.552814645807,145.628975917023,145.705087664326,145.781160440953,145.822371756267),
 .UNSPECIFIED.);
#3088=B_SPLINE_CURVE_WITH_KNOTS('',3,(#150302,#150303,#150304,#150305,#150306,
#150307,#150308,#150309,#150310,#150311,#150312,#150313,#150314,#150315,
#150316,#150317),.UNSPECIFIED.,.F.,.F.,(4,3,3,3,3,4),(145.822371756267,
145.904101300103,145.985836415022,146.067566652371,146.149298441322,146.178586402224),
 .UNSPECIFIED.);
#3089=B_SPLINE_CURVE_WITH_KNOTS('',3,(#150319,#150320,#150321,#150322,#150323,
#150324,#150325,#150326,#150327,#150328,#150329,#150330,#150331,#150332,
#150333,#150334),.UNSPECIFIED.,.F.,.F.,(4,3,3,3,3,4),(-142.439142960337,
-142.356023082934,-142.273070385938,-142.190228256313,-142.107546608186,
-142.083132212162),.UNSPECIFIED.);
#3090=B_SPLINE_CURVE_WITH_KNOTS('',3,(#150335,#150336,#150337,#150338,#150339,
#150340,#150341,#150342,#150343,#150344,#150345,#150346,#150347,#150348,
#150349,#150350,#150351,#150352,#150353,#150354,#150355,#150356,#150357,
#150358,#150359,#150360,#150361,#150362,#150363,#150364,#150365,#150366,
#150367,#150368,#150369,#150370,#150371,#150372,#150373,#150374,#150375,
#150376,#150377,#150378,#150379,#150380,#150381,#150382,#150383,#150384,
#150385,#150386,#150387,#150388,#150389,#150390,#150391,#150392,#150393,
#150394,#150395,#150396,#150397,#150398,#150399,#150400,#150401,#150402,
#150403,#150404,#150405,#150406,#150407,#150408,#150409,#150410,#150411,
#150412,#150413,#150414,#150415,#150416,#150417,#150418,#150419,#150420,
#150421,#150422,#150423,#150424,#150425,#150426,#150427,#150428,#150429,
#150430,#150431,#150432,#150433,#150434,#150435,#150436,#150437,#150438,
#150439,#150440,#150441,#150442,#150443,#150444,#150445,#150446,#150447,
#150448,#150449,#150450,#150451,#150452,#150453,#150454,#150455,#150456,
#150457,#150458,#150459,#150460,#150461,#150462,#150463,#150464,#150465,
#150466,#150467,#150468,#150469,#150470,#150471,#150472,#150473,#150474,
#150475,#150476,#150477,#150478,#150479,#150480,#150481,#150482,#150483,
#150484,#150485,#150486,#150487,#150488,#150489,#150490,#150491,#150492,
#150493,#150494,#150495,#150496,#150497,#150498,#150499,#150500,#150501,
#150502,#150503,#150504,#150505,#150506,#150507,#150508,#150509,#150510,
#150511,#150512,#150513,#150514,#150515,#150516,#150517,#150518,#150519,
#150520,#150521,#150522,#150523,#150524,#150525,#150526,#150527,#150528,
#150529,#150530,#150531,#150532,#150533,#150534,#150535,#150536,#150537,
#150538,#150539,#150540,#150541,#150542,#150543,#150544,#150545,#150546,
#150547,#150548,#150549,#150550,#150551,#150552,#150553,#150554,#150555,
#150556,#150557,#150558,#150559,#150560,#150561,#150562,#150563,#150564,
#150565,#150566,#150567,#150568,#150569),.UNSPECIFIED.,.F.,.F.,(4,3,3,3,
3,3,3,3,3,3,3,3,3,3,3,3,3,3,3,3,3,3,3,3,3,3,3,3,3,3,3,3,3,3,3,3,3,3,3,3,
3,3,3,3,3,3,3,3,3,3,3,3,3,3,3,3,3,3,3,3,3,3,3,3,3,3,3,3,3,3,3,3,3,3,3,3,
3,3,4),(-142.083130505234,-142.000499302849,-141.917779667378,-141.834977613084,
-141.752059853652,-141.66908716499,-141.586038721683,-141.565066299346,
-141.490960864321,-141.416912369555,-141.342905634648,-141.268916373607,
-141.194939015116,-141.120936732207,-141.066597756039,-140.975598644234,
-140.884095413094,-140.792151859509,-140.700117267453,-140.608208162886,
-140.568129212731,-140.492419546296,-140.416758548968,-140.341131713343,
-140.265514021781,-140.189902526422,-140.114262606517,-140.069660669424,
-139.98738189348,-139.90507932644,-139.821607526359,-139.739252567185,-139.65522234665,
-139.571192126116,-139.488813117401,-139.406448930065,-139.323017593251,
-139.240695621887,-139.156709602348,-139.072723582809,-138.997083473201,
-138.921467369906,-138.845860802462,-138.770226139361,-138.69457658039,
-138.61886629022,-138.574255039501,-138.482354469857,-138.390321500201,
-138.298441930429,-138.206814534445,-138.115793412998,-138.075786496194,
-138.001784581558,-137.927803653267,-137.853828631407,-137.779816158162,
-137.705784888235,-137.631680136085,-137.577317952886,-137.498356536905,
-137.419449113802,-137.34058407483,-137.261749844069,-137.182934870054,
-137.104113606357,-137.025286967207,-136.946444442794,-136.867575514174,
-136.788633462805,-136.709652697279,-136.630581686223,-136.580380866271,
-136.501378523423,-136.422477075346,-136.343694796591,-136.264982735704,
-136.186348045329,-136.155837210071),.UNSPECIFIED.);
#3091=B_SPLINE_CURVE_WITH_KNOTS('',3,(#150575,#150576,#150577,#150578,#150579,
#150580,#150581,#150582,#150583,#150584,#150585,#150586,#150587,#150588,
#150589,#150590,#150591,#150592,#150593,#150594,#150595,#150596,#150597,
#150598,#150599,#150600,#150601,#150602,#150603,#150604,#150605,#150606,
#150607,#150608,#150609,#150610,#150611,#150612,#150613,#150614,#150615,
#150616,#150617,#150618,#150619,#150620,#150621,#150622,#150623,#150624,
#150625,#150626,#150627,#150628,#150629,#150630,#150631,#150632,#150633,
#150634,#150635,#150636,#150637,#150638,#150639,#150640,#150641,#150642,
#150643,#150644,#150645,#150646,#150647,#150648,#150649,#150650,#150651,
#150652,#150653,#150654,#150655,#150656,#150657,#150658,#150659,#150660,
#150661,#150662,#150663,#150664,#150665,#150666,#150667,#150668,#150669,
#150670,#150671,#150672,#150673,#150674,#150675,#150676,#150677,#150678,
#150679,#150680,#150681,#150682,#150683,#150684,#150685,#150686,#150687,
#150688,#150689,#150690,#150691,#150692,#150693,#150694,#150695,#150696,
#150697,#150698,#150699,#150700,#150701,#150702,#150703,#150704,#150705,
#150706,#150707,#150708,#150709,#150710,#150711,#150712,#150713,#150714,
#150715,#150716,#150717,#150718,#150719,#150720,#150721,#150722,#150723,
#150724,#150725,#150726,#150727,#150728,#150729,#150730,#150731,#150732,
#150733,#150734,#150735,#150736,#150737,#150738,#150739,#150740,#150741,
#150742,#150743,#150744,#150745,#150746,#150747,#150748,#150749,#150750,
#150751,#150752,#150753,#150754,#150755,#150756,#150757,#150758,#150759,
#150760,#150761,#150762,#150763,#150764,#150765,#150766,#150767,#150768,
#150769,#150770,#150771,#150772,#150773,#150774,#150775,#150776,#150777,
#150778,#150779,#150780,#150781,#150782,#150783,#150784,#150785,#150786,
#150787,#150788,#150789,#150790,#150791,#150792,#150793,#150794,#150795,
#150796,#150797,#150798,#150799,#150800,#150801,#150802,#150803,#150804,
#150805,#150806,#150807,#150808,#150809,#150810,#150811,#150812),
 .UNSPECIFIED.,.F.,.F.,(4,3,3,3,3,3,3,3,3,3,3,3,3,3,3,3,3,3,3,3,3,3,3,3,
3,3,3,3,3,3,3,3,3,3,3,3,3,3,3,3,3,3,3,3,3,3,3,3,3,3,3,3,3,3,3,3,3,3,3,3,
3,3,3,3,3,3,3,3,3,3,3,3,3,3,3,3,3,3,3,4),(133.611894774878,133.703844055645,
133.799892579167,133.891713018518,133.983244652198,134.074173849049,134.088038149733,
134.162040064416,134.236020992754,134.309996014661,134.384008487955,134.458039757931,
134.532144510131,134.586506693041,134.665468108988,134.744375532057,134.823240570993,
134.902074801719,134.980889775697,135.059711039357,135.138537678469,135.217380202845,
135.296249131428,135.375191182759,135.454171948247,135.533242959265,135.583443779656,
135.662435675016,135.741327459713,135.820129715778,135.898829716621,135.97746916252,
136.056045444726,136.081912322963,136.160499046081,136.239135213299,136.317831206568,
136.396645238004,136.47552666618,136.554529759348,136.580380866271,136.659453388058,
136.73845294283,136.817391210691,136.89627982521,136.975130381803,137.053958886106,
137.132775260011,137.211590011231,137.290413645245,137.369283692828,137.448177371938,
137.527137896809,137.577317952886,137.651423390933,137.725471888733,137.799478626685,
137.873467890785,137.947445252344,138.021447538325,138.075786496194,138.166785595894,
138.258288813528,138.350232352405,138.442266929528,138.53417601959,138.574255039501,
138.649964711011,138.725625713429,138.801252554159,138.876870250831,138.952481751307,
139.028121676321,139.072723582809,139.154965444528,139.237231094181,139.319536624453,
139.401853127536,139.484193158093,139.539186449088),.UNSPECIFIED.);
#3092=B_SPLINE_CURVE_WITH_KNOTS('',3,(#150813,#150814,#150815,#150816,#150817,
#150818,#150819,#150820,#150821,#150822,#150823,#150824,#150825,#150826,
#150827,#150828),.UNSPECIFIED.,.F.,.F.,(4,3,3,3,3,4),(139.539186449218,
139.571192126116,139.653573056315,139.735937288415,139.818282645486,139.895602067557),
 .UNSPECIFIED.);
#3093=B_SPLINE_CURVE_WITH_KNOTS('',3,(#150830,#150831,#150832,#150833,#150834,
#150835,#150836,#150837,#150838,#150839,#150840,#150841,#150842,#150843,
#150844,#150845),.UNSPECIFIED.,.F.,.F.,(4,3,3,3,3,4),(-136.155837210071,
-136.081912322963,-136.007543160793,-135.933164179611,-135.85872478924,
-135.799946905112),.UNSPECIFIED.);
#3094=B_SPLINE_CURVE_WITH_KNOTS('',3,(#150846,#150847,#150848,#150849,#150850,
#150851,#150852,#150853,#150854,#150855,#150856,#150857,#150858,#150859,
#150860,#150861,#150862,#150863,#150864,#150865,#150866,#150867,#150868,
#150869,#150870,#150871,#150872,#150873,#150874,#150875,#150876,#150877,
#150878,#150879,#150880,#150881,#150882,#150883,#150884,#150885,#150886,
#150887,#150888,#150889,#150890,#150891,#150892,#150893,#150894,#150895,
#150896,#150897,#150898,#150899,#150900,#150901,#150902,#150903,#150904,
#150905,#150906,#150907,#150908,#150909,#150910,#150911,#150912,#150913,
#150914,#150915,#150916,#150917,#150918,#150919,#150920,#150921,#150922,
#150923,#150924,#150925,#150926,#150927,#150928,#150929,#150930,#150931,
#150932,#150933,#150934,#150935,#150936,#150937,#150938,#150939,#150940,
#150941,#150942,#150943,#150944,#150945,#150946,#150947,#150948,#150949,
#150950,#150951,#150952,#150953,#150954,#150955,#150956,#150957,#150958,
#150959,#150960,#150961,#150962,#150963,#150964,#150965,#150966,#150967,
#150968,#150969,#150970,#150971,#150972,#150973,#150974,#150975,#150976,
#150977,#150978,#150979,#150980,#150981,#150982,#150983,#150984,#150985,
#150986,#150987,#150988,#150989,#150990,#150991,#150992,#150993,#150994,
#150995,#150996,#150997,#150998,#150999,#151000,#151001,#151002,#151003,
#151004,#151005,#151006,#151007,#151008,#151009,#151010,#151011,#151012,
#151013,#151014,#151015,#151016,#151017,#151018,#151019,#151020,#151021,
#151022,#151023,#151024,#151025,#151026,#151027,#151028,#151029,#151030,
#151031,#151032,#151033,#151034,#151035,#151036,#151037,#151038,#151039,
#151040,#151041,#151042,#151043,#151044,#151045,#151046,#151047,#151048,
#151049,#151050,#151051,#151052,#151053,#151054,#151055,#151056,#151057,
#151058,#151059,#151060,#151061,#151062,#151063,#151064,#151065,#151066,
#151067,#151068,#151069,#151070,#151071,#151072,#151073,#151074,#151075,
#151076,#151077,#151078,#151079,#151080),.UNSPECIFIED.,.F.,.F.,(4,3,3,3,
3,3,3,3,3,3,3,3,3,3,3,3,3,3,3,3,3,3,3,3,3,3,3,3,3,3,3,3,3,3,3,3,3,3,3,3,
3,3,3,3,3,3,3,3,3,3,3,3,3,3,3,3,3,3,3,3,3,3,3,3,3,3,3,3,3,3,3,3,3,3,3,3,
3,3,4),(-135.799946904982,-135.709593726747,-135.618579632177,-135.583443779656,
-135.504371257906,-135.425371703171,-135.346433435348,-135.267544820866,
-135.18869426431,-135.109865760044,-135.031049386175,-134.952234634992,
-134.873411001014,-134.794540953466,-134.71564727439,-134.636686749553,
-134.586506693041,-134.512401254945,-134.438352757096,-134.364346019095,
-134.290356754948,-134.216379393341,-134.142377107314,-134.088038149733,
-133.997039049987,-133.905535832298,-133.813592293355,-133.721557716163,
-133.629648626029,-133.589569606426,-133.513859935311,-133.438198933289,
-133.362572092954,-133.286954396674,-133.211342896591,-133.135702971966,
-133.091101063118,-133.008822291261,-132.926519728395,-132.843047926249,
-132.760692971348,-132.676662745579,-132.59263251981,-132.51025350921,-132.427889319963,
-132.344457984098,-132.262136010807,-132.178149993655,-132.094163976503,
-132.018523867281,-131.942907764374,-131.867301197319,-131.791666534609,
-131.716016976031,-131.640306686253,-131.595695433195,-131.503794863493,
-131.411761893781,-131.31988232396,-131.228254927932,-131.137233806452,
-131.097226889888,-131.0232249752,-130.949244046856,-130.875269024943,-130.801256551643,
-130.727225281661,-130.653120529456,-130.59875834658,-130.519788908694,
-130.438987933081,-130.360125171892,-130.281291165063,-130.202475388716,
-130.120201817486,-130.041376296381,-129.962540678799,-129.883669978161,
-129.873381103796),.UNSPECIFIED.);
#3095=B_SPLINE_CURVE_WITH_KNOTS('',3,(#151086,#151087,#151088,#151089,#151090,
#151091,#151092,#151093,#151094,#151095,#151096,#151097,#151098,#151099,
#151100,#151101,#151102,#151103,#151104,#151105,#151106,#151107,#151108,
#151109,#151110,#151111,#151112,#151113,#151114,#151115,#151116,#151117,
#151118,#151119,#151120,#151121,#151122,#151123,#151124,#151125,#151126,
#151127,#151128,#151129,#151130,#151131,#151132,#151133,#151134,#151135,
#151136,#151137,#151138,#151139,#151140,#151141,#151142,#151143,#151144,
#151145,#151146,#151147,#151148,#151149,#151150,#151151,#151152,#151153,
#151154,#151155,#151156,#151157,#151158,#151159,#151160,#151161,#151162,
#151163,#151164,#151165,#151166,#151167,#151168,#151169,#151170,#151171,
#151172,#151173,#151174,#151175,#151176,#151177,#151178,#151179,#151180,
#151181,#151182,#151183,#151184,#151185,#151186,#151187,#151188,#151189,
#151190,#151191,#151192,#151193,#151194,#151195,#151196,#151197,#151198,
#151199,#151200,#151201,#151202,#151203,#151204,#151205,#151206,#151207,
#151208,#151209,#151210,#151211,#151212,#151213,#151214,#151215,#151216,
#151217,#151218,#151219,#151220,#151221,#151222,#151223,#151224,#151225,
#151226,#151227,#151228,#151229,#151230,#151231,#151232,#151233,#151234,
#151235,#151236,#151237,#151238,#151239,#151240,#151241,#151242,#151243,
#151244,#151245,#151246,#151247,#151248,#151249,#151250,#151251,#151252,
#151253,#151254,#151255,#151256,#151257,#151258,#151259,#151260,#151261,
#151262,#151263,#151264,#151265,#151266,#151267,#151268,#151269,#151270,
#151271,#151272,#151273,#151274,#151275,#151276,#151277,#151278,#151279,
#151280,#151281,#151282,#151283,#151284,#151285,#151286,#151287,#151288,
#151289,#151290,#151291,#151292,#151293,#151294,#151295,#151296,#151297,
#151298,#151299,#151300,#151301,#151302,#151303,#151304,#151305),
 .UNSPECIFIED.,.F.,.F.,(4,3,3,3,3,3,3,3,3,3,3,3,3,3,3,3,3,3,3,3,3,3,3,3,
3,3,3,3,3,3,3,3,3,3,3,3,3,3,3,3,3,3,3,3,3,3,3,3,3,3,3,3,3,3,3,3,3,3,3,3,
3,3,3,3,3,3,3,3,3,3,3,3,3,4),(127.329030480685,127.410760354451,127.492490108222,
127.574219743663,127.655949262443,127.737678666226,127.819407956681,127.9043547252,
127.987974200461,128.070287121421,128.152026030488,128.233764519875,128.315502596255,
128.397240266302,128.47897753669,128.560714414093,128.642450905183,128.724187016634,
128.805922755116,128.887658127302,128.969393139864,129.051127799473,129.132862112801,
129.214596086517,129.296329727292,129.378063041797,129.459796036702,129.541528718675,
129.623261094387,129.704993170506,129.786724953702,129.868456450642,129.950187667996,
130.031918612431,130.113649290615,130.195379709216,130.277109874901,130.358839794338,
130.440569474193,130.522298921133,130.607727115532,130.690485678857,130.77222430642,
130.853962110224,130.935699116964,131.017435353331,131.099170846017,131.180905621708,
131.262639707089,131.344373128841,131.426105913646,131.507838088182,131.589569679123,
131.671300713144,131.753031216916,131.834761217111,131.916490740395,132.00021014049,
132.081948221518,132.163684716943,132.245419733527,132.327153378016,132.408885757133,
132.490616977586,132.572347146066,132.657803895546,132.739540813765,132.821274822668,
132.903006349188,132.984735820116,133.066470710592,133.148200790757,133.229932219818,
133.256001141908),.UNSPECIFIED.);
#3096=B_SPLINE_CURVE_WITH_KNOTS('',3,(#151306,#151307,#151308,#151309,#151310,
#151311,#151312,#151313,#151314,#151315,#151316,#151317,#151318,#151319,
#151320,#151321,#151322,#151323,#151324),.UNSPECIFIED.,.F.,.F.,(4,3,3,3,
3,3,4),(133.256001141908,133.331495817858,133.407020184361,133.482561554849,
133.558161894196,133.589569606426,133.611894774878),.UNSPECIFIED.);
#3097=B_SPLINE_CURVE_WITH_KNOTS('',3,(#151326,#151327,#151328,#151329,#151330,
#151331,#151332,#151333,#151334,#151335,#151336,#151337,#151338,#151339,
#151340,#151341),.UNSPECIFIED.,.F.,.F.,(4,3,3,3,3,4),(-129.873381103796,
-129.794432154857,-129.715442567629,-129.636366301135,-129.601821259965,
-129.516761597802),.UNSPECIFIED.);
#3098=B_SPLINE_CURVE_WITH_KNOTS('',3,(#151342,#151343,#151344,#151345,#151346,
#151347,#151348,#151349,#151350,#151351,#151352,#151353,#151354,#151355,
#151356,#151357,#151358,#151359,#151360,#151361,#151362,#151363,#151364,
#151365,#151366,#151367,#151368,#151369,#151370,#151371,#151372,#151373,
#151374,#151375,#151376,#151377,#151378,#151379,#151380,#151381,#151382,
#151383,#151384,#151385,#151386,#151387,#151388,#151389,#151390,#151391,
#151392,#151393,#151394,#151395,#151396,#151397,#151398,#151399,#151400,
#151401,#151402,#151403,#151404,#151405,#151406,#151407,#151408,#151409,
#151410,#151411,#151412,#151413,#151414,#151415,#151416,#151417,#151418,
#151419,#151420,#151421,#151422,#151423,#151424,#151425,#151426,#151427,
#151428,#151429,#151430,#151431,#151432,#151433,#151434,#151435,#151436,
#151437,#151438,#151439,#151440,#151441,#151442,#151443,#151444,#151445,
#151446,#151447,#151448,#151449,#151450,#151451,#151452,#151453,#151454,
#151455,#151456,#151457,#151458,#151459,#151460,#151461,#151462,#151463,
#151464,#151465,#151466,#151467,#151468,#151469,#151470,#151471,#151472,
#151473,#151474,#151475,#151476,#151477,#151478,#151479,#151480,#151481,
#151482,#151483,#151484,#151485,#151486,#151487,#151488,#151489,#151490,
#151491,#151492,#151493,#151494,#151495,#151496,#151497,#151498,#151499,
#151500,#151501,#151502,#151503,#151504,#151505,#151506,#151507,#151508,
#151509,#151510,#151511,#151512,#151513,#151514,#151515,#151516,#151517,
#151518,#151519,#151520,#151521,#151522,#151523,#151524,#151525,#151526,
#151527,#151528,#151529,#151530,#151531,#151532,#151533,#151534,#151535,
#151536,#151537,#151538,#151539,#151540,#151541,#151542,#151543,#151544,
#151545,#151546,#151547,#151548,#151549,#151550,#151551,#151552,#151553,
#151554,#151555,#151556,#151557,#151558,#151559,#151560,#151561,#151562,
#151563,#151564,#151565,#151566,#151567,#151568,#151569,#151570,#151571,
#151572,#151573,#151574,#151575,#151576,#151577,#151578,#151579),
 .UNSPECIFIED.,.F.,.F.,(4,3,3,3,3,3,3,3,3,3,3,3,3,3,3,3,3,3,3,3,3,3,3,3,
3,3,3,3,3,3,3,3,3,3,3,3,3,3,3,3,3,3,3,3,3,3,3,3,3,3,3,3,3,3,3,3,3,3,3,3,
3,3,3,3,3,3,3,3,3,3,3,3,3,3,3,3,3,3,3,4),(-129.51676159771,-129.440162129166,
-129.3636436382,-129.287207051255,-129.210817745977,-129.134465961583,-129.103352716657,
-129.024765993494,-128.946129826232,-128.867433832917,-128.788619801435,
-128.709738373212,-128.630735279997,-128.60488417335,-128.5258116516,-128.446812096865,
-128.367873829041,-128.28898521456,-128.210134658003,-128.131306153737,
-128.052489779869,-127.973675028685,-127.894851394707,-127.815981347159,
-127.737087668083,-127.658127143246,-127.607947086735,-127.533841648633,
-127.459793150777,-127.38578641277,-127.311797148617,-127.237819787004,
-127.16381750097,-127.109478543427,-127.018479443693,-126.926976226018,
-126.83503268709,-126.742998109913,-126.651089019794,-126.61101000012,-126.535300329002,
-126.459639326975,-126.384012486637,-126.308394790354,-126.232783290266,
-126.157143365638,-126.112541456812,-126.03026268496,-125.947960122098,
-125.86448831995,-125.782133365053,-125.698103139279,-125.614072913505,
-125.531693902902,-125.449329713651,-125.365898377787,-125.283576404493,
-125.199590387345,-125.115604370197,-125.039964260976,-124.964348158071,
-124.888741591018,-124.813106928309,-124.737457369732,-124.661747079956,
-124.61713582689,-124.525235257187,-124.433202287472,-124.34132271765,-124.24969532162,
-124.158674200137,-124.118667283582,-124.044665368893,-123.970684440549,
-123.896709418635,-123.822696945334,-123.748665675352,-123.674560923147,
-123.620198740274,-123.590150617738),.UNSPECIFIED.);
#3099=B_SPLINE_CURVE_WITH_KNOTS('',3,(#151585,#151586,#151587,#151588,#151589,
#151590,#151591,#151592,#151593,#151594,#151595,#151596,#151597,#151598,
#151599,#151600,#151601,#151602,#151603,#151604,#151605,#151606,#151607,
#151608,#151609,#151610,#151611,#151612,#151613,#151614,#151615,#151616,
#151617,#151618,#151619,#151620,#151621,#151622,#151623,#151624,#151625,
#151626,#151627,#151628,#151629,#151630,#151631,#151632,#151633,#151634,
#151635,#151636,#151637,#151638,#151639,#151640,#151641,#151642,#151643,
#151644,#151645,#151646,#151647,#151648,#151649,#151650,#151651,#151652,
#151653,#151654,#151655,#151656,#151657,#151658,#151659,#151660,#151661,
#151662,#151663,#151664,#151665,#151666,#151667,#151668,#151669,#151670,
#151671,#151672,#151673,#151674,#151675,#151676,#151677,#151678,#151679,
#151680,#151681,#151682,#151683,#151684,#151685,#151686,#151687,#151688,
#151689,#151690,#151691,#151692,#151693,#151694,#151695,#151696,#151697,
#151698,#151699,#151700,#151701,#151702,#151703,#151704,#151705,#151706,
#151707,#151708,#151709,#151710,#151711,#151712,#151713,#151714,#151715,
#151716,#151717,#151718,#151719,#151720,#151721,#151722,#151723,#151724,
#151725,#151726,#151727,#151728,#151729,#151730,#151731,#151732,#151733,
#151734,#151735,#151736,#151737,#151738,#151739,#151740,#151741,#151742,
#151743,#151744,#151745,#151746,#151747,#151748,#151749,#151750,#151751,
#151752,#151753,#151754,#151755,#151756,#151757,#151758,#151759,#151760,
#151761,#151762,#151763,#151764,#151765,#151766,#151767,#151768,#151769,
#151770,#151771,#151772,#151773,#151774,#151775,#151776,#151777,#151778,
#151779,#151780,#151781,#151782,#151783,#151784,#151785,#151786,#151787,
#151788,#151789,#151790,#151791,#151792,#151793,#151794,#151795,#151796,
#151797,#151798,#151799,#151800,#151801,#151802,#151803,#151804,#151805,
#151806,#151807,#151808,#151809,#151810,#151811,#151812,#151813,#151814,
#151815,#151816,#151817,#151818,#151819),.UNSPECIFIED.,.F.,.F.,(4,3,3,3,
3,3,3,3,3,3,3,3,3,3,3,3,3,3,3,3,3,3,3,3,3,3,3,3,3,3,3,3,3,3,3,3,3,3,3,3,
3,3,3,3,3,3,3,3,3,3,3,3,3,3,3,3,3,3,3,3,3,3,3,3,3,3,3,3,3,3,3,3,3,3,3,3,
3,3,4),(121.04580412481,121.123867226472,121.20193141621,121.280008607331,
121.35811071905,121.436284155121,121.51449773961,121.59279954696,121.626324567044,
121.705316462383,121.784208247058,121.863010503103,121.941710503926,122.020349949805,
122.098926231991,122.124793110352,122.203379833515,122.282016000777,122.360711994093,
122.439526025575,122.518407453798,122.597410547013,122.623261653659,122.702334175409,
122.781333730144,122.860271997968,122.939160612449,123.018011169005,123.096839673271,
123.17565604714,123.254470798323,123.333294432301,123.412164479849,123.491058158925,
123.570018683762,123.620198740274,123.694304178376,123.768352676231,123.842359414238,
123.916348678391,123.990326040003,124.064328326036,124.118667283582,124.209666383319,
124.301169600998,124.39311313993,124.48514771711,124.577056807233,124.61713582689,
124.692845498007,124.768506500031,124.844133340368,124.919751036649,124.995362536735,
125.071002461362,125.115604370197,125.197883142052,125.280185704916,125.363657507063,
125.446012461962,125.530042687734,125.614072913505,125.696451924106,125.778816113354,
125.862247449219,125.94456942251,126.028555439661,126.112541456812,126.188181566034,
126.263797668941,126.339404235995,126.415038898706,126.490688457284,126.566398747061,
126.61101000012,126.705396416608,126.799894665305,126.894075848052,126.972815834728),
 .UNSPECIFIED.);
#3100=B_SPLINE_CURVE_WITH_KNOTS('',3,(#151820,#151821,#151822,#151823,#151824,
#151825,#151826,#151827,#151828,#151829,#151830,#151831,#151832,#151833,
#151834,#151835),.UNSPECIFIED.,.F.,.F.,(4,3,3,3,3,4),(126.972815834728,
127.054545378564,127.136280493483,127.218010730832,127.299742519783,127.329030480685),
 .UNSPECIFIED.);
#3101=B_SPLINE_CURVE_WITH_KNOTS('',3,(#151837,#151838,#151839,#151840,#151841,
#151842,#151843,#151844,#151845,#151846,#151847,#151848,#151849),
 .UNSPECIFIED.,.F.,.F.,(4,3,3,3,4),(-123.590150617738,-123.500202190511,
-123.410405737001,-123.321051447307,-123.233576290755),.UNSPECIFIED.);
#3102=B_SPLINE_CURVE_WITH_KNOTS('',3,(#151850,#151851,#151852,#151853,#151854,
#151855,#151856,#151857,#151858,#151859,#151860,#151861,#151862,#151863,
#151864,#151865,#151866,#151867,#151868,#151869,#151870,#151871,#151872,
#151873,#151874,#151875,#151876,#151877,#151878,#151879,#151880,#151881,
#151882,#151883,#151884,#151885,#151886,#151887,#151888,#151889,#151890,
#151891,#151892,#151893,#151894,#151895,#151896,#151897,#151898,#151899,
#151900,#151901,#151902,#151903,#151904,#151905,#151906,#151907,#151908,
#151909,#151910,#151911,#151912,#151913,#151914,#151915,#151916,#151917,
#151918,#151919,#151920,#151921,#151922,#151923,#151924,#151925,#151926,
#151927,#151928,#151929,#151930,#151931,#151932,#151933,#151934,#151935,
#151936,#151937,#151938,#151939,#151940,#151941,#151942,#151943,#151944,
#151945,#151946,#151947,#151948,#151949,#151950,#151951,#151952,#151953,
#151954,#151955,#151956,#151957,#151958,#151959,#151960,#151961,#151962,
#151963,#151964,#151965,#151966,#151967,#151968,#151969,#151970,#151971,
#151972,#151973,#151974,#151975,#151976,#151977,#151978,#151979,#151980,
#151981,#151982,#151983,#151984,#151985,#151986,#151987,#151988,#151989,
#151990,#151991,#151992,#151993,#151994,#151995,#151996,#151997,#151998,
#151999,#152000,#152001,#152002,#152003,#152004,#152005,#152006,#152007,
#152008,#152009,#152010,#152011,#152012,#152013,#152014,#152015,#152016,
#152017,#152018,#152019,#152020,#152021,#152022,#152023,#152024,#152025,
#152026,#152027,#152028,#152029,#152030,#152031,#152032,#152033,#152034,
#152035,#152036,#152037,#152038,#152039,#152040,#152041,#152042,#152043,
#152044,#152045,#152046,#152047,#152048,#152049,#152050,#152051,#152052,
#152053,#152054,#152055,#152056,#152057,#152058,#152059,#152060,#152061,
#152062,#152063,#152064,#152065,#152066,#152067,#152068,#152069,#152070,
#152071,#152072,#152073,#152074,#152075,#152076,#152077,#152078,#152079,
#152080,#152081,#152082,#152083,#152084),.UNSPECIFIED.,.F.,.F.,(4,3,3,3,
3,3,3,3,3,3,3,3,3,3,3,3,3,3,3,3,3,3,3,3,3,3,3,3,3,3,3,3,3,3,3,3,3,3,3,3,
3,3,3,3,3,3,3,3,3,3,3,3,3,3,3,3,3,3,3,3,3,3,3,3,3,3,3,3,3,3,3,3,3,3,3,3,
3,3,4),(-123.233576290623,-123.154340788253,-123.075085132784,-122.99580002089,
-122.916476130551,-122.837062311739,-122.757601429428,-122.678037844198,
-122.623261653659,-122.544269758321,-122.465377973647,-122.386575717604,
-122.307875716783,-122.229236270906,-122.150659988722,-122.124793110352,
-122.046206387188,-121.967570219925,-121.888874226607,-121.810060195124,
-121.731178766899,-121.652175673683,-121.626324567044,-121.547252045294,
-121.46825249056,-121.389314222736,-121.310425608255,-121.231575051698,
-121.152746547433,-121.073930173564,-120.99511542238,-120.916291788403,
-120.837421740854,-120.758528061779,-120.679567536942,-120.629387480429,
-120.555282042327,-120.481233544472,-120.407226806465,-120.333237542312,
-120.259260180699,-120.185257894666,-120.130918937121,-120.039919837387,
-119.948416619712,-119.856473080783,-119.764438503607,-119.672529413488,
-119.632450393814,-119.556740722696,-119.481079720669,-119.40545288033,
-119.329835184047,-119.25422368396,-119.178583759332,-119.133981850506,
-119.051703078654,-118.969400515792,-118.885928713644,-118.803573758747,
-118.719543532973,-118.635513307199,-118.553134296596,-118.470770107346,
-118.387338771482,-118.305016798188,-118.22103078104,-118.137044763891,
-118.06140465467,-117.985788551765,-117.910181984712,-117.834547322003,
-117.758897763426,-117.68318747365,-117.638576220584,-117.54663341521,-117.454600059247,
-117.362706616229,-117.306038383074),.UNSPECIFIED.);
#3103=B_SPLINE_CURVE_WITH_KNOTS('',3,(#152090,#152091,#152092,#152093,#152094,
#152095,#152096,#152097,#152098,#152099,#152100,#152101,#152102,#152103,
#152104,#152105,#152106,#152107,#152108,#152109,#152110,#152111,#152112,
#152113,#152114,#152115,#152116,#152117,#152118,#152119,#152120,#152121,
#152122,#152123,#152124,#152125,#152126,#152127,#152128,#152129,#152130,
#152131,#152132,#152133,#152134,#152135,#152136,#152137,#152138,#152139,
#152140,#152141,#152142,#152143,#152144,#152145,#152146,#152147,#152148,
#152149,#152150,#152151,#152152,#152153,#152154,#152155,#152156,#152157,
#152158,#152159,#152160,#152161,#152162,#152163,#152164,#152165,#152166,
#152167,#152168,#152169,#152170,#152171,#152172,#152173,#152174,#152175,
#152176,#152177,#152178,#152179,#152180,#152181,#152182,#152183,#152184,
#152185,#152186,#152187,#152188,#152189,#152190,#152191,#152192,#152193,
#152194,#152195,#152196,#152197,#152198,#152199,#152200,#152201,#152202,
#152203,#152204,#152205,#152206,#152207,#152208,#152209,#152210,#152211,
#152212,#152213,#152214,#152215,#152216,#152217,#152218,#152219,#152220,
#152221,#152222,#152223,#152224,#152225,#152226,#152227,#152228,#152229,
#152230,#152231,#152232,#152233,#152234,#152235,#152236,#152237,#152238,
#152239,#152240,#152241,#152242,#152243,#152244,#152245,#152246,#152247,
#152248,#152249,#152250,#152251,#152252,#152253,#152254,#152255,#152256,
#152257,#152258,#152259,#152260,#152261,#152262,#152263,#152264,#152265,
#152266,#152267,#152268,#152269,#152270,#152271,#152272,#152273,#152274,
#152275,#152276,#152277,#152278,#152279,#152280,#152281,#152282,#152283,
#152284,#152285,#152286,#152287,#152288,#152289,#152290,#152291,#152292,
#152293,#152294,#152295,#152296,#152297,#152298,#152299,#152300,#152301,
#152302,#152303,#152304,#152305,#152306,#152307,#152308,#152309,#152310,
#152311,#152312,#152313,#152314,#152315,#152316,#152317,#152318,#152319,
#152320,#152321,#152322,#152323,#152324),.UNSPECIFIED.,.F.,.F.,(4,3,3,3,
3,3,3,3,3,3,3,3,3,3,3,3,3,3,3,3,3,3,3,3,3,3,3,3,3,3,3,3,3,3,3,3,3,3,3,3,
3,3,3,3,3,3,3,3,3,3,3,3,3,3,3,3,3,3,3,3,3,3,3,3,3,3,3,3,3,3,3,3,3,3,3,3,
3,3,4),(114.763381035136,114.842229958887,114.920966376191,114.999637094917,
115.078236134955,115.146233504046,115.224820227208,115.30345639447,115.382152387785,
115.460966419266,115.539847847488,115.618850940703,115.644702047353,115.723774569103,
115.802774123839,115.881712391663,115.960601006145,116.039451562701,116.118280066968,
116.197096440837,116.275911192021,116.354734825999,116.433604873548,116.512498552624,
116.591459077462,116.641639133969,116.715744572071,116.789793069925,116.863799807932,
116.937789072085,117.011766433696,117.08576871973,117.140107677276,117.231106777012,
117.32260999469,117.414553533621,117.5065881108,117.598497200922,117.638576220584,
117.714285891701,117.789946893726,117.865573734064,117.941191430345,118.016802930432,
118.092442855059,118.137044763891,118.219323535745,118.301626098609,118.385097900756,
118.467452855655,118.551483081427,118.635513307199,118.7178923178,118.800256507049,
118.883687842913,118.966009816205,119.049995833355,119.133981850506,119.209621959727,
119.285238062634,119.360844629687,119.436479292397,119.512128850974,119.587839140751,
119.632450393814,119.724350963519,119.816383933236,119.90826350306,119.999890899091,
120.090912020574,120.130918937122,120.204920851809,120.278901780151,120.352876802063,
120.426889275362,120.500920545342,120.575025297546,120.629387480429,120.689630527549),
 .UNSPECIFIED.);
#3104=B_SPLINE_CURVE_WITH_KNOTS('',3,(#152325,#152326,#152327,#152328,#152329,
#152330,#152331,#152332,#152333,#152334,#152335,#152336,#152337,#152338,
#152339,#152340),.UNSPECIFIED.,.F.,.F.,(4,3,3,3,3,4),(120.689630527646,
120.767862687141,120.846020793888,120.924135361203,121.002215288158,121.04580412481),
 .UNSPECIFIED.);
#3105=B_SPLINE_CURVE_WITH_KNOTS('',3,(#152342,#152343,#152344,#152345,#152346,
#152347,#152348,#152349,#152350,#152351,#152352,#152353,#152354,#152355,
#152356,#152357),.UNSPECIFIED.,.F.,.F.,(4,3,3,3,3,4),(-117.306038383074,
-117.21490246554,-117.140107677276,-117.069392244814,-116.998691172987,
-116.950390983542),.UNSPECIFIED.);
#3106=B_SPLINE_CURVE_WITH_KNOTS('',3,(#152358,#152359,#152360,#152361,#152362,
#152363,#152364,#152365,#152366,#152367,#152368,#152369,#152370,#152371,
#152372,#152373,#152374,#152375,#152376,#152377,#152378,#152379,#152380,
#152381,#152382,#152383,#152384,#152385,#152386,#152387,#152388,#152389,
#152390,#152391,#152392,#152393,#152394,#152395,#152396,#152397,#152398,
#152399,#152400,#152401,#152402,#152403,#152404,#152405,#152406,#152407,
#152408,#152409,#152410,#152411,#152412,#152413,#152414,#152415,#152416,
#152417,#152418,#152419,#152420,#152421,#152422,#152423,#152424,#152425,
#152426,#152427,#152428,#152429,#152430,#152431,#152432,#152433,#152434,
#152435,#152436,#152437,#152438,#152439,#152440,#152441,#152442,#152443,
#152444,#152445,#152446,#152447,#152448,#152449,#152450,#152451,#152452,
#152453,#152454,#152455,#152456,#152457,#152458,#152459,#152460,#152461,
#152462,#152463,#152464,#152465,#152466,#152467,#152468,#152469,#152470,
#152471,#152472,#152473,#152474,#152475,#152476,#152477,#152478,#152479,
#152480,#152481,#152482,#152483,#152484,#152485,#152486,#152487,#152488,
#152489,#152490,#152491,#152492,#152493,#152494,#152495,#152496,#152497,
#152498,#152499,#152500,#152501,#152502,#152503,#152504,#152505,#152506,
#152507,#152508,#152509,#152510,#152511,#152512,#152513,#152514,#152515,
#152516,#152517,#152518,#152519,#152520,#152521,#152522,#152523,#152524,
#152525,#152526,#152527,#152528,#152529,#152530,#152531,#152532,#152533,
#152534,#152535,#152536,#152537,#152538,#152539,#152540,#152541,#152542,
#152543,#152544,#152545,#152546,#152547,#152548,#152549,#152550,#152551,
#152552,#152553,#152554,#152555,#152556,#152557,#152558,#152559,#152560,
#152561,#152562,#152563,#152564,#152565,#152566,#152567,#152568,#152569,
#152570,#152571,#152572,#152573,#152574,#152575,#152576,#152577,#152578,
#152579,#152580,#152581,#152582,#152583,#152584,#152585,#152586,#152587,
#152588,#152589,#152590,#152591,#152592),.UNSPECIFIED.,.F.,.F.,(4,3,3,3,
3,3,3,3,3,3,3,3,3,3,3,3,3,3,3,3,3,3,3,3,3,3,3,3,3,3,3,3,3,3,3,3,3,3,3,3,
3,3,3,3,3,3,3,3,3,3,3,3,3,3,3,3,3,3,3,3,3,3,3,3,3,3,3,3,3,3,3,3,3,3,3,3,
3,3,4),(-116.950390983443,-116.872431787928,-116.794422690535,-116.716290904427,
-116.641639133969,-116.562677718021,-116.483770294951,-116.404905256013,
-116.326071025286,-116.247256051307,-116.168434787645,-116.089608148532,
-116.010765624155,-115.931896695571,-115.852954644239,-115.773973878749,
-115.69490286773,-115.644702047353,-115.565710152015,-115.486818367341,
-115.408016111297,-115.329316110476,-115.250676664598,-115.172100382413,
-115.146233504046,-115.067646780882,-114.989010613619,-114.910314620303,
-114.831500588819,-114.752619160596,-114.67361606738,-114.647764960738,
-114.568692438988,-114.489692884253,-114.410754616429,-114.331866001947,
-114.253015445391,-114.174186941125,-114.095370567256,-114.016555816072,
-113.937732182094,-113.858862134546,-113.77996845547,-113.701007930633,
-113.650827874123,-113.576722436022,-113.502673938168,-113.428667200161,
-113.354677936009,-113.280700574398,-113.206698288365,-113.152359330816,
-113.061360231079,-112.9698570134,-112.877913474468,-112.785878897287,-112.693969807164,
-112.653890787508,-112.578181116391,-112.502520114366,-112.426893274029,
-112.351275577748,-112.275664077662,-112.200024153035,-112.155422244201,
-112.073143472347,-111.990840909484,-111.907369107336,-111.825014152438,
-111.740983926666,-111.656953700893,-111.57457469029,-111.492210501039,
-111.408779165175,-111.326457191881,-111.242471174733,-111.158485157585,
-111.082886699848,-111.023443944257),.UNSPECIFIED.);
#3107=B_SPLINE_CURVE_WITH_KNOTS('',3,(#152598,#152599,#152600,#152601,#152602,
#152603,#152604,#152605,#152606,#152607,#152608,#152609,#152610,#152611,
#152612,#152613,#152614,#152615,#152616,#152617,#152618,#152619,#152620,
#152621,#152622,#152623,#152624,#152625,#152626,#152627,#152628,#152629,
#152630,#152631,#152632,#152633,#152634,#152635,#152636,#152637,#152638,
#152639,#152640,#152641,#152642,#152643,#152644,#152645,#152646,#152647,
#152648,#152649,#152650,#152651,#152652,#152653,#152654,#152655,#152656,
#152657,#152658,#152659,#152660,#152661,#152662,#152663,#152664,#152665,
#152666,#152667,#152668,#152669,#152670,#152671,#152672,#152673,#152674,
#152675,#152676,#152677,#152678,#152679,#152680,#152681,#152682,#152683,
#152684,#152685,#152686,#152687,#152688,#152689,#152690,#152691,#152692,
#152693,#152694,#152695,#152696,#152697,#152698,#152699,#152700,#152701,
#152702,#152703,#152704,#152705,#152706,#152707,#152708,#152709,#152710,
#152711,#152712,#152713,#152714,#152715,#152716,#152717,#152718,#152719,
#152720,#152721,#152722,#152723,#152724,#152725,#152726,#152727,#152728,
#152729,#152730,#152731,#152732,#152733,#152734,#152735,#152736,#152737,
#152738,#152739,#152740,#152741,#152742,#152743,#152744,#152745,#152746,
#152747,#152748,#152749,#152750,#152751,#152752,#152753,#152754,#152755,
#152756,#152757,#152758,#152759,#152760,#152761,#152762,#152763,#152764,
#152765,#152766,#152767,#152768,#152769,#152770,#152771,#152772,#152773,
#152774,#152775,#152776,#152777,#152778,#152779,#152780,#152781,#152782,
#152783,#152784,#152785,#152786,#152787,#152788,#152789,#152790,#152791,
#152792,#152793,#152794,#152795,#152796,#152797,#152798,#152799,#152800,
#152801,#152802,#152803,#152804,#152805,#152806,#152807,#152808,#152809,
#152810,#152811,#152812,#152813,#152814,#152815,#152816,#152817,#152818,
#152819,#152820,#152821,#152822,#152823,#152824,#152825,#152826,#152827,
#152828,#152829,#152830,#152831,#152832),.UNSPECIFIED.,.F.,.F.,(4,3,3,3,
3,3,3,3,3,3,3,3,3,3,3,3,3,3,3,3,3,3,3,3,3,3,3,3,3,3,3,3,3,3,3,3,3,3,3,3,
3,3,3,3,3,3,3,3,3,3,3,3,3,3,3,3,3,3,3,3,3,3,3,3,3,3,3,3,3,3,3,3,3,3,3,3,
3,3,4),(108.478674260886,108.557552281005,108.636553196501,108.666142441048,
108.745214962797,108.824214517533,108.903152785357,108.982041399838,109.060891956394,
109.13972046066,109.218536834529,109.297351585712,109.376175219689,109.455045267237,
109.533938946313,109.61289947115,109.663079527663,109.737184965764,109.811233463619,
109.885240201625,109.959229465777,110.033206827389,110.107209113421,110.16154807097,
110.252547170709,110.344050388387,110.43599392732,110.5280285045,110.619937594623,
110.660016614278,110.735726285395,110.81138728742,110.887014127756,110.962631824038,
111.038243324123,111.11388324875,111.158485157585,111.240763929439,111.323066492301,
111.406538294449,111.488893249347,111.57292347512,111.656953700893,111.739332711496,
111.821696900748,111.905128236611,111.987450209905,112.071436227053,112.155422244201,
112.231062353421,112.306678456326,112.382285023379,112.457919686087,112.533569244663,
112.609279534439,112.653890787508,112.745791357214,112.837824326931,112.929703896756,
113.021331292787,113.112352414271,113.152359330816,113.226361245503,113.300342173846,
113.374317195758,113.448329669058,113.522360939038,113.596465691242,113.650827874123,
113.72907653155,113.80726520934,113.885402422488,113.96351040033,114.041600985793,
114.119686009305,114.197799010695,114.275925669416,114.354107310553,114.406445220369),
 .UNSPECIFIED.);
#3108=B_SPLINE_CURVE_WITH_KNOTS('',3,(#152833,#152834,#152835,#152836,#152837,
#152838,#152839,#152840,#152841,#152842,#152843,#152844,#152845,#152846,
#152847,#152848),.UNSPECIFIED.,.F.,.F.,(4,3,3,3,3,4),(114.406445220461,
114.508021462892,114.611348359269,114.647764960738,114.726761857662,114.763381035136),
 .UNSPECIFIED.);
#3109=B_SPLINE_CURVE_WITH_KNOTS('',3,(#152850,#152851,#152852,#152853,#152854,
#152855,#152856,#152857,#152858,#152859,#152860,#152861,#152862,#152863,
#152864,#152865),.UNSPECIFIED.,.F.,.F.,(4,3,3,3,3,4),(-111.023443944257,
-110.947879173554,-110.872289747824,-110.796688202473,-110.721026482249,
-110.667205676354),.UNSPECIFIED.);
#3110=B_SPLINE_CURVE_WITH_KNOTS('',3,(#152866,#152867,#152868,#152869,#152870,
#152871,#152872,#152873,#152874,#152875,#152876,#152877,#152878,#152879,
#152880,#152881,#152882,#152883,#152884,#152885,#152886,#152887,#152888,
#152889,#152890,#152891,#152892,#152893,#152894,#152895,#152896,#152897,
#152898,#152899,#152900,#152901,#152902,#152903,#152904,#152905,#152906,
#152907,#152908,#152909,#152910,#152911,#152912,#152913,#152914,#152915,
#152916,#152917,#152918,#152919,#152920,#152921,#152922,#152923,#152924,
#152925,#152926,#152927,#152928,#152929,#152930,#152931,#152932,#152933,
#152934,#152935,#152936,#152937,#152938,#152939,#152940,#152941,#152942,
#152943,#152944,#152945,#152946,#152947,#152948,#152949,#152950,#152951,
#152952,#152953,#152954,#152955,#152956,#152957,#152958,#152959,#152960,
#152961,#152962,#152963,#152964,#152965,#152966,#152967,#152968,#152969,
#152970,#152971,#152972,#152973,#152974,#152975,#152976,#152977,#152978,
#152979,#152980,#152981,#152982,#152983,#152984,#152985,#152986,#152987,
#152988,#152989,#152990,#152991,#152992,#152993,#152994,#152995,#152996,
#152997,#152998,#152999,#153000,#153001,#153002,#153003,#153004,#153005,
#153006,#153007,#153008,#153009,#153010,#153011,#153012,#153013,#153014,
#153015,#153016,#153017,#153018,#153019,#153020,#153021,#153022,#153023,
#153024,#153025,#153026,#153027,#153028,#153029,#153030,#153031,#153032,
#153033,#153034,#153035,#153036,#153037,#153038,#153039,#153040,#153041,
#153042,#153043,#153044,#153045,#153046,#153047,#153048,#153049,#153050,
#153051,#153052,#153053,#153054,#153055,#153056,#153057,#153058,#153059,
#153060,#153061,#153062,#153063,#153064,#153065,#153066,#153067,#153068,
#153069,#153070,#153071,#153072,#153073,#153074,#153075,#153076,#153077,
#153078,#153079,#153080,#153081,#153082,#153083,#153084,#153085,#153086,
#153087,#153088,#153089,#153090,#153091,#153092,#153093,#153094,#153095,
#153096,#153097,#153098,#153099,#153100,#153101,#153102,#153103,#153104,
#153105,#153106),.UNSPECIFIED.,.F.,.F.,(4,3,3,3,3,3,3,3,3,3,3,3,3,3,3,3,
3,3,3,3,3,3,3,3,3,3,3,3,3,3,3,3,3,3,3,3,3,3,3,3,3,3,3,3,3,3,3,3,3,3,3,3,
3,3,3,3,3,3,3,3,3,3,3,3,3,3,3,3,3,3,3,3,3,3,3,3,3,3,3,3,4),(-110.667205676264,
-110.660016614278,-110.568116044574,-110.476083074859,-110.384203505036,
-110.292576109006,-110.201554987524,-110.16154807097,-110.087546156283,
-110.01356522794,-109.939590206028,-109.865577732729,-109.791546462748,
-109.717441710544,-109.663079527663,-109.584118111716,-109.505210688647,
-109.42634564971,-109.347511418984,-109.268696445006,-109.189875181345,
-109.111048542233,-109.032206017857,-108.953337089274,-108.874395037942,
-108.795414272454,-108.716343261435,-108.666142441048,-108.587150545709,
-108.508258761033,-108.429456504988,-108.350756504166,-108.272117058286,
-108.1935407761,-108.16767389774,-108.089087174578,-108.010451007316,-107.931755014,
-107.852940982519,-107.774059554296,-107.695056461082,-107.669205354433,
-107.590132832683,-107.511133277947,-107.432195010123,-107.353306395641,
-107.274455839085,-107.195627334818,-107.116810960949,-107.037996209765,
-106.959172575787,-106.880302528238,-106.801408849162,-106.722448324325,
-106.672268267817,-106.598162829715,-106.524114331861,-106.450107593854,
-106.376118329702,-106.30214096809,-106.228138682057,-106.17379972451,-106.082800624774,
-105.991297407096,-105.899353868165,-105.807319290985,-105.715410200864,
-105.675331181202,-105.599621510085,-105.523960508059,-105.448333667722,
-105.37271597144,-105.297104471354,-105.221464546727,-105.176862637895,
-105.094588492349,-105.012289926871,-104.929953560671,-104.847605501347,
-104.765237375343,-104.740291169727),.UNSPECIFIED.);
#3111=B_SPLINE_CURVE_WITH_KNOTS('',3,(#153112,#153113,#153114,#153115,#153116,
#153117,#153118,#153119,#153120,#153121,#153122,#153123,#153124,#153125,
#153126,#153127,#153128,#153129,#153130,#153131,#153132,#153133,#153134,
#153135,#153136,#153137,#153138,#153139,#153140,#153141,#153142,#153143,
#153144,#153145,#153146,#153147,#153148,#153149,#153150,#153151,#153152,
#153153,#153154,#153155,#153156,#153157,#153158,#153159,#153160,#153161,
#153162,#153163,#153164,#153165,#153166,#153167,#153168,#153169,#153170,
#153171,#153172,#153173,#153174,#153175,#153176,#153177,#153178,#153179,
#153180,#153181,#153182,#153183,#153184,#153185,#153186,#153187,#153188,
#153189,#153190,#153191,#153192,#153193,#153194,#153195,#153196,#153197,
#153198,#153199,#153200,#153201,#153202,#153203,#153204,#153205,#153206,
#153207,#153208,#153209,#153210,#153211,#153212,#153213,#153214,#153215,
#153216,#153217,#153218,#153219,#153220,#153221,#153222,#153223,#153224,
#153225,#153226,#153227,#153228,#153229,#153230,#153231,#153232,#153233,
#153234,#153235,#153236,#153237,#153238,#153239,#153240,#153241,#153242,
#153243,#153244,#153245,#153246,#153247,#153248,#153249,#153250,#153251,
#153252,#153253,#153254,#153255,#153256,#153257,#153258,#153259,#153260,
#153261,#153262,#153263,#153264,#153265,#153266,#153267,#153268,#153269,
#153270,#153271,#153272,#153273,#153274,#153275,#153276,#153277,#153278,
#153279,#153280,#153281,#153282,#153283,#153284,#153285,#153286,#153287,
#153288,#153289,#153290,#153291,#153292,#153293,#153294,#153295,#153296,
#153297,#153298,#153299,#153300,#153301,#153302,#153303,#153304,#153305,
#153306,#153307,#153308,#153309,#153310,#153311,#153312,#153313,#153314,
#153315,#153316,#153317,#153318,#153319,#153320,#153321,#153322,#153323,
#153324,#153325,#153326,#153327,#153328,#153329,#153330,#153331,#153332,
#153333,#153334,#153335,#153336,#153337,#153338,#153339,#153340,#153341,
#153342,#153343,#153344,#153345,#153346),.UNSPECIFIED.,.F.,.F.,(4,3,3,3,
3,3,3,3,3,3,3,3,3,3,3,3,3,3,3,3,3,3,3,3,3,3,3,3,3,3,3,3,3,3,3,3,3,3,3,3,
3,3,3,3,3,3,3,3,3,3,3,3,3,3,3,3,3,3,3,3,3,3,3,3,3,3,3,3,3,3,3,3,3,3,3,3,
3,3,4),(102.196903430706,102.274689906697,102.352474506175,102.430269534311,
102.508113205017,102.585985365738,102.663924460471,102.684519921357,102.758625359459,
102.832673857315,102.906680595322,102.980669859475,103.054647221088,103.128649507121,
103.182988464665,103.273987564398,103.365490782074,103.457434321002,103.549468898179,
103.641377988298,103.681457007972,103.75716667909,103.832827681117,103.908454521455,
103.984072217738,104.059683717825,104.135323642454,104.17992555128,104.262204323132,
104.344506885994,104.427978688142,104.510333643039,104.594363868813,104.678394094587,
104.76077310519,104.84313729444,104.926568630304,105.008890603598,105.092876620746,
105.176862637895,105.252502747116,105.328118850021,105.403725417074,105.479360079783,
105.55500963836,105.630719928136,105.675331181202,105.767231750907,105.859264720624,
105.951144290448,106.042771686478,106.133792807961,106.17379972451,106.247801639198,
106.32178256754,106.395757589452,106.469770062751,106.543801332732,106.617906084937,
106.672268267817,106.751229683765,106.830137106834,106.909002145771,106.987836376498,
107.066651350477,107.145472614138,107.224299253251,107.303141777627,107.382010706211,
107.460952757542,107.539933523032,107.61900453405,107.669205354433,107.749104703786,
107.82889315808,107.908540526475,107.988104779652,108.06756570541,108.123259913073),
 .UNSPECIFIED.);
#3112=B_SPLINE_CURVE_WITH_KNOTS('',3,(#153347,#153348,#153349,#153350,#153351,
#153352,#153353,#153354,#153355,#153356,#153357,#153358,#153359,#153360,
#153361,#153362),.UNSPECIFIED.,.F.,.F.,(4,3,3,3,3,4),(108.12325991319,108.16767389774,
108.24627820679,108.324921018778,108.403664244961,108.478674260886),
 .UNSPECIFIED.);
#3113=B_SPLINE_CURVE_WITH_KNOTS('',3,(#153364,#153365,#153366,#153367,#153368,
#153369,#153370,#153371,#153372,#153373,#153374,#153375,#153376,#153377,
#153378,#153379),.UNSPECIFIED.,.F.,.F.,(4,3,3,3,3,4),(-104.740291169727,
-104.678394094587,-104.596765179296,-104.515154181363,-104.433558031947,
-104.384020369084),.UNSPECIFIED.);
#3114=B_SPLINE_CURVE_WITH_KNOTS('',3,(#153380,#153381,#153382,#153383,#153384,
#153385,#153386,#153387,#153388,#153389,#153390,#153391,#153392,#153393,
#153394,#153395,#153396,#153397,#153398,#153399,#153400,#153401,#153402,
#153403,#153404,#153405,#153406,#153407,#153408,#153409,#153410,#153411,
#153412,#153413,#153414,#153415,#153416,#153417,#153418,#153419,#153420,
#153421,#153422,#153423,#153424,#153425,#153426,#153427,#153428,#153429,
#153430,#153431,#153432,#153433,#153434,#153435,#153436,#153437,#153438,
#153439,#153440,#153441,#153442,#153443,#153444,#153445,#153446,#153447,
#153448,#153449,#153450,#153451,#153452,#153453,#153454,#153455,#153456,
#153457,#153458,#153459,#153460,#153461,#153462,#153463,#153464,#153465,
#153466,#153467,#153468,#153469,#153470,#153471,#153472,#153473,#153474,
#153475,#153476,#153477,#153478,#153479,#153480,#153481,#153482,#153483,
#153484,#153485,#153486,#153487,#153488,#153489,#153490,#153491,#153492,
#153493,#153494,#153495,#153496,#153497,#153498,#153499,#153500,#153501,
#153502,#153503,#153504,#153505,#153506,#153507,#153508,#153509,#153510,
#153511,#153512,#153513,#153514,#153515,#153516,#153517,#153518,#153519,
#153520,#153521,#153522,#153523,#153524,#153525,#153526,#153527,#153528,
#153529,#153530,#153531,#153532,#153533,#153534,#153535,#153536,#153537,
#153538,#153539,#153540,#153541,#153542,#153543,#153544,#153545,#153546,
#153547,#153548,#153549,#153550,#153551,#153552,#153553,#153554,#153555,
#153556,#153557,#153558,#153559,#153560,#153561,#153562,#153563,#153564,
#153565,#153566,#153567,#153568,#153569,#153570,#153571,#153572,#153573,
#153574,#153575,#153576,#153577,#153578,#153579,#153580,#153581,#153582,
#153583,#153584,#153585,#153586,#153587,#153588,#153589,#153590,#153591,
#153592,#153593,#153594,#153595,#153596,#153597,#153598,#153599,#153600,
#153601,#153602,#153603,#153604,#153605,#153606,#153607,#153608,#153609,
#153610,#153611,#153612,#153613,#153614,#153615,#153616,#153617,#153618,
#153619,#153620),.UNSPECIFIED.,.F.,.F.,(4,3,3,3,3,3,3,3,3,3,3,3,3,3,3,3,
3,3,3,3,3,3,3,3,3,3,3,3,3,3,3,3,3,3,3,3,3,3,3,3,3,3,3,3,3,3,3,3,3,3,3,3,
3,3,3,3,3,3,3,3,3,3,3,3,3,3,3,3,3,3,3,3,3,3,3,3,3,3,3,3,4),(-104.38402036896,
-104.297747267439,-104.211526193072,-104.17992555128,-104.104285442056,
-104.028669339147,-103.953062772091,-103.877428109379,-103.801778550799,
-103.72606826102,-103.681457007972,-103.589556438273,-103.497523468563,
-103.405643898744,-103.314016502719,-103.222995381241,-103.182988464665,
-103.108986549976,-103.035005621632,-102.961030599719,-102.887018126419,
-102.812986856437,-102.738882104231,-102.684519921357,-102.60555850541,
-102.526651082341,-102.447786043404,-102.368951812678,-102.290136838699,
-102.211315575039,-102.132488935927,-102.05364641155,-101.974777482967,
-101.895835431636,-101.816854666147,-101.737783655129,-101.687582834742,
-101.608590939403,-101.529699154728,-101.450896898683,-101.372196897862,
-101.293557451984,-101.214981169798,-101.189114291434,-101.110527568271,
-101.031891401009,-100.953195407692,-100.87438137621,-100.795499947987,
-100.716496854772,-100.690645748127,-100.611573226377,-100.532573671642,
-100.453635403818,-100.374746789337,-100.29589623278,-100.217067728515,
-100.138251354646,-100.059436603462,-99.9806129694843,-99.9017429219359,
-99.8228492428599,-99.7438887180229,-99.6937086615116,-99.6196032234094,
-99.5455547255546,-99.4715479875472,-99.3975587233941,-99.323581361782,
-99.2495790757487,-99.195240118204,-99.1042410184677,-99.0127378007954,
-98.9207942618662,-98.8287596846874,-98.7368505945678,-98.6967715748965,
-98.6210612370815,-98.5453977770355,-98.469770943029,-98.4567671119247),
 .UNSPECIFIED.);
#3115=B_SPLINE_CURVE_WITH_KNOTS('',3,(#153626,#153627,#153628,#153629,#153630,
#153631,#153632,#153633,#153634,#153635,#153636,#153637,#153638,#153639,
#153640,#153641,#153642,#153643,#153644,#153645,#153646,#153647,#153648,
#153649,#153650,#153651,#153652,#153653,#153654,#153655,#153656,#153657,
#153658,#153659,#153660,#153661,#153662,#153663,#153664,#153665,#153666,
#153667,#153668,#153669,#153670,#153671,#153672,#153673,#153674,#153675,
#153676,#153677,#153678,#153679,#153680,#153681,#153682,#153683,#153684,
#153685,#153686,#153687,#153688,#153689,#153690,#153691,#153692,#153693,
#153694,#153695,#153696,#153697,#153698,#153699,#153700,#153701,#153702,
#153703,#153704,#153705,#153706,#153707,#153708,#153709,#153710,#153711,
#153712,#153713,#153714,#153715,#153716,#153717,#153718,#153719,#153720,
#153721,#153722,#153723,#153724,#153725,#153726,#153727,#153728,#153729,
#153730,#153731,#153732,#153733,#153734,#153735,#153736,#153737,#153738,
#153739,#153740,#153741,#153742,#153743,#153744,#153745,#153746,#153747,
#153748,#153749,#153750,#153751,#153752,#153753,#153754,#153755,#153756,
#153757,#153758,#153759,#153760,#153761,#153762,#153763,#153764,#153765,
#153766,#153767,#153768,#153769,#153770,#153771,#153772,#153773,#153774,
#153775,#153776,#153777,#153778,#153779,#153780,#153781,#153782,#153783,
#153784,#153785,#153786,#153787,#153788,#153789,#153790,#153791,#153792,
#153793,#153794,#153795,#153796,#153797,#153798,#153799,#153800,#153801,
#153802,#153803,#153804,#153805,#153806,#153807,#153808,#153809,#153810,
#153811,#153812,#153813,#153814,#153815,#153816,#153817,#153818,#153819,
#153820,#153821,#153822,#153823,#153824,#153825,#153826,#153827,#153828,
#153829,#153830,#153831,#153832,#153833,#153834,#153835,#153836,#153837,
#153838,#153839,#153840,#153841,#153842,#153843,#153844,#153845,#153846,
#153847,#153848,#153849,#153850,#153851,#153852,#153853,#153854,#153855,
#153856,#153857,#153858,#153859,#153860),.UNSPECIFIED.,.F.,.F.,(4,3,3,3,
3,3,3,3,3,3,3,3,3,3,3,3,3,3,3,3,3,3,3,3,3,3,3,3,3,3,3,3,3,3,3,3,3,3,3,3,
3,3,3,3,3,3,3,3,3,3,3,3,3,3,3,3,3,3,3,3,3,3,3,3,3,3,3,3,3,3,3,3,3,3,3,3,
3,3,4),(95.9134562041998,95.9874494352425,96.0614280794984,96.1354322403172,
96.2044288583587,96.2954279580946,96.3869311757722,96.4788747147027,96.5709092918821,
96.6628183820036,96.7028974016663,96.7786070727838,96.8542680748096,96.9298949151471,
97.0055126114294,97.0811241115159,97.1567640361435,97.2013659449738,97.2836447168271,
97.3659472796899,97.4494190818378,97.5317740367358,97.6158042625086,97.6998344882814,
97.7822134988835,97.8645776881333,97.9480090239972,98.0303309972902,98.1143170144396,
98.198303031589,98.2739431408102,98.3495592437161,98.4251658107696,98.5008004734788,
98.5764500320564,98.6521603218331,98.6967715748965,98.7886721445999,98.8807051143141,
98.9725846841366,99.0642120801662,99.1552332016479,99.1952401182041,99.269242032892,
99.3432229612353,99.4171979831476,99.4912104564474,99.5652417264285,99.6393464786333,
99.6937086615116,99.772670077459,99.8515775005284,99.9304425394651,100.009276770191,
100.08809174417,100.16691300783,100.245739646943,100.324582171319,100.403451099902,
100.482393151234,100.561373916723,100.640444927741,100.690645748127,100.769637643465,
100.848529428139,100.927331684183,101.006031685004,101.084671130883,101.163247413067,
101.189114291434,101.267701014598,101.346337181861,101.425033175179,101.503847206662,
101.582728634886,101.661731728102,101.687582834742,101.820615347273,101.84007460601),
 .UNSPECIFIED.);
#3116=B_SPLINE_CURVE_WITH_KNOTS('',3,(#153861,#153862,#153863,#153864,#153865,
#153866,#153867,#153868,#153869,#153870,#153871,#153872,#153873,#153874,
#153875,#153876),.UNSPECIFIED.,.F.,.F.,(4,3,3,3,3,4),(101.840074606096,
101.918052868575,101.995951121691,102.073802611243,102.151615518596,102.196903430706),
 .UNSPECIFIED.);
#3117=B_SPLINE_CURVE_WITH_KNOTS('',3,(#153878,#153879,#153880,#153881,#153882,
#153883,#153884,#153885,#153886,#153887,#153888,#153889,#153890,#153891,
#153892,#153893,#153894,#153895,#153896),.UNSPECIFIED.,.F.,.F.,(4,3,3,3,
3,3,4),(-98.4567671119247,-98.3811514041528,-98.3055396637728,-98.2298999732549,
-98.1983030315889,-98.1072700840541,-98.1008350619045),.UNSPECIFIED.);
#3118=B_SPLINE_CURVE_WITH_KNOTS('',3,(#153897,#153898,#153899,#153900,#153901,
#153902,#153903,#153904,#153905,#153906,#153907,#153908,#153909,#153910,
#153911,#153912,#153913,#153914,#153915,#153916,#153917,#153918,#153919,
#153920,#153921,#153922,#153923,#153924,#153925,#153926,#153927,#153928,
#153929,#153930,#153931,#153932,#153933,#153934,#153935,#153936,#153937,
#153938,#153939,#153940,#153941,#153942,#153943,#153944,#153945,#153946,
#153947,#153948,#153949,#153950,#153951,#153952,#153953,#153954,#153955,
#153956,#153957,#153958,#153959,#153960,#153961,#153962,#153963,#153964,
#153965,#153966,#153967,#153968,#153969,#153970,#153971,#153972,#153973,
#153974,#153975,#153976,#153977,#153978,#153979,#153980,#153981,#153982,
#153983,#153984,#153985,#153986,#153987,#153988,#153989,#153990,#153991,
#153992,#153993,#153994,#153995,#153996,#153997,#153998,#153999,#154000,
#154001,#154002,#154003,#154004,#154005,#154006,#154007,#154008,#154009,
#154010,#154011,#154012,#154013,#154014,#154015,#154016,#154017,#154018,
#154019,#154020,#154021,#154022,#154023,#154024,#154025,#154026,#154027,
#154028,#154029,#154030,#154031,#154032,#154033,#154034,#154035,#154036,
#154037,#154038,#154039,#154040,#154041,#154042,#154043,#154044,#154045,
#154046,#154047,#154048,#154049,#154050,#154051,#154052,#154053,#154054,
#154055,#154056,#154057,#154058,#154059,#154060,#154061,#154062,#154063,
#154064,#154065,#154066,#154067,#154068,#154069,#154070,#154071,#154072,
#154073,#154074,#154075,#154076,#154077,#154078,#154079,#154080,#154081,
#154082,#154083,#154084,#154085,#154086,#154087,#154088,#154089,#154090,
#154091,#154092,#154093,#154094,#154095,#154096,#154097,#154098,#154099,
#154100,#154101,#154102,#154103,#154104,#154105,#154106,#154107,#154108,
#154109,#154110,#154111,#154112,#154113,#154114,#154115,#154116,#154117,
#154118,#154119,#154120,#154121,#154122,#154123,#154124,#154125,#154126,
#154127,#154128,#154129,#154130,#154131,#154132,#154133,#154134),
 .UNSPECIFIED.,.F.,.F.,(4,3,3,3,3,3,3,3,3,3,3,3,3,3,3,3,3,3,3,3,3,3,3,3,
3,3,3,3,3,3,3,3,3,3,3,3,3,3,3,3,3,3,3,3,3,3,3,3,3,3,3,3,3,3,3,3,3,3,3,3,
3,3,3,3,3,3,3,3,3,3,3,3,3,3,3,3,3,3,3,4),(-98.1008350618282,-98.0193723107643,
-97.9378849353233,-97.8563932604577,-97.7748767781644,-97.6998344882814,
-97.6174554776792,-97.5350912884297,-97.4516599525657,-97.3693379792726,
-97.2853519621232,-97.2013659449738,-97.1257258357525,-97.0501097328464,
-96.9745031657927,-96.8988685030833,-96.8232189445056,-96.7475086547288,
-96.7028974016662,-96.6109968319633,-96.5189638622495,-96.4270842924274,
-96.3354568963981,-96.2444357749168,-96.2044288583587,-96.1304269436705,
-96.0564460153271,-95.9824709934147,-95.9084585201146,-95.8344272501333,
-95.7603224979283,-95.7059603150511,-95.6269988991039,-95.5480914760347,
-95.4692264370982,-95.3903922063724,-95.3115772323937,-95.2327559687335,
-95.1539293296212,-95.0750868052449,-94.9962178766622,-94.9172758253308,
-94.838295059842,-94.7592240488239,-94.709023228436,-94.6300313330974,-94.5511395484225,
-94.4723372923782,-94.3936372915567,-94.314997845678,-94.2364215634927,
-94.2105546851284,-94.1319679619649,-94.053331794702,-93.9746358013858,
-93.895821769903,-93.8169403416795,-93.7379372484637,-93.7120861418209,
-93.6330136200713,-93.5540140653362,-93.4750757975122,-93.3961871830309,
-93.3173366264747,-93.238508122209,-93.1596917483401,-93.0808769971564,
-93.0020533631788,-92.9231833156305,-92.8442896365547,-92.7653291117177,
-92.7151490552058,-92.6410436171038,-92.5669951192492,-92.4929883812423,
-92.4189991170896,-92.3450217554775,-92.2710194694443,-92.2166805118982,
-92.1745156025595),.UNSPECIFIED.);
#3119=B_SPLINE_CURVE_WITH_KNOTS('',3,(#154140,#154141,#154142,#154143,#154144,
#154145,#154146,#154147,#154148,#154149,#154150,#154151,#154152,#154153,
#154154,#154155,#154156,#154157,#154158,#154159,#154160,#154161,#154162,
#154163,#154164,#154165,#154166,#154167,#154168,#154169,#154170,#154171,
#154172,#154173,#154174,#154175,#154176,#154177,#154178,#154179,#154180,
#154181,#154182,#154183,#154184,#154185,#154186,#154187,#154188,#154189,
#154190,#154191,#154192,#154193,#154194,#154195,#154196,#154197,#154198,
#154199,#154200,#154201,#154202,#154203,#154204,#154205,#154206,#154207,
#154208,#154209,#154210,#154211,#154212,#154213,#154214,#154215,#154216,
#154217,#154218,#154219,#154220,#154221,#154222,#154223,#154224,#154225,
#154226,#154227,#154228,#154229,#154230,#154231,#154232,#154233,#154234,
#154235,#154236,#154237,#154238,#154239,#154240,#154241,#154242,#154243,
#154244,#154245,#154246,#154247,#154248,#154249,#154250,#154251,#154252,
#154253,#154254,#154255,#154256,#154257,#154258,#154259,#154260,#154261,
#154262,#154263,#154264,#154265,#154266,#154267,#154268,#154269,#154270,
#154271,#154272,#154273,#154274,#154275,#154276,#154277,#154278,#154279,
#154280,#154281,#154282,#154283,#154284,#154285,#154286,#154287,#154288,
#154289,#154290,#154291,#154292,#154293,#154294,#154295,#154296,#154297,
#154298,#154299,#154300,#154301,#154302,#154303,#154304,#154305,#154306,
#154307,#154308,#154309,#154310,#154311,#154312,#154313,#154314,#154315,
#154316,#154317,#154318,#154319,#154320,#154321,#154322,#154323,#154324,
#154325,#154326,#154327,#154328,#154329,#154330,#154331,#154332,#154333,
#154334,#154335,#154336,#154337,#154338,#154339,#154340,#154341,#154342,
#154343,#154344,#154345,#154346,#154347,#154348,#154349,#154350,#154351,
#154352,#154353,#154354,#154355,#154356,#154357,#154358,#154359,#154360,
#154361,#154362,#154363,#154364,#154365,#154366,#154367,#154368,#154369,
#154370,#154371,#154372,#154373,#154374),.UNSPECIFIED.,.F.,.F.,(4,3,3,3,
3,3,3,3,3,3,3,3,3,3,3,3,3,3,3,3,3,3,3,3,3,3,3,3,3,3,3,3,3,3,3,3,3,3,3,3,
3,3,3,3,3,3,3,3,3,3,3,3,3,3,3,3,3,3,3,3,3,3,3,3,3,3,3,3,3,3,3,3,3,3,3,3,
3,3,4),(89.6300395101817,89.7243377953605,89.8000474664779,89.8757084685036,
89.9513353088409,90.0269530051231,90.1025645052098,90.1782044298374,90.222806338668,
90.3050851105214,90.3873876733842,90.4708594755321,90.5532144304302,90.6372446562029,
90.7212748819756,90.8036538925775,90.8860180818271,90.9694494176911,91.0517713909838,
91.1357574081335,91.2197434252831,91.2953835345044,91.3709996374104,91.4466062044641,
91.5222408671736,91.5978904257513,91.6736007155281,91.7182119685907,91.8101125382937,
91.9021455080077,91.9940250778299,92.0856524738591,92.1766735953405,92.2166805118982,
92.2906824265863,92.3646633549297,92.4386383768422,92.5126508501422,92.5866821201235,
92.6607868723284,92.7151490552058,92.794110471153,92.8730178942222,92.9518829331587,
93.0307171638846,93.1095321378633,93.1883534015235,93.2671800406358,93.3460225650122,
93.424891493595,93.5038335449265,93.5828143104152,93.6618853214333,93.7120861418209,
93.7910780371595,93.8699698218343,93.9487720778786,94.0274720787001,94.1061115245789,
94.1846878067641,94.2105546851285,94.289141408292,94.3677775755548,94.4464735688713,
94.525287600354,94.6041690285776,94.6831721217933,94.709023228436,94.786765196696,
94.8644314260667,94.9420360592962,95.0195897015247,95.0971148667966,95.1746242892932,
95.2521306918767,95.3296741511598,95.4072349269498,95.4848662150954,95.5568892987335),
 .UNSPECIFIED.);
#3120=B_SPLINE_CURVE_WITH_KNOTS('',3,(#154375,#154376,#154377,#154378,#154379,
#154380,#154381,#154382,#154383,#154384,#154385,#154386,#154387),
 .UNSPECIFIED.,.F.,.F.,(4,3,3,3,4),(95.5568892988304,95.7059603150512,95.7800702622623,
95.8541168037861,95.9134562041998),.UNSPECIFIED.);
#3121=B_SPLINE_CURVE_WITH_KNOTS('',3,(#154389,#154390,#154391,#154392,#154393,
#154394,#154395,#154396,#154397,#154398,#154399,#154400,#154401),
 .UNSPECIFIED.,.F.,.F.,(4,3,3,3,4),(-92.1745156025595,-92.0851629640592,
-91.9955575606049,-91.9057144617474,-91.817649754849),.UNSPECIFIED.);
#3122=B_SPLINE_CURVE_WITH_KNOTS('',3,(#154402,#154403,#154404,#154405,#154406,
#154407,#154408,#154409,#154410,#154411,#154412,#154413,#154414,#154415,
#154416,#154417,#154418,#154419,#154420,#154421,#154422,#154423,#154424,
#154425,#154426,#154427,#154428,#154429,#154430,#154431,#154432,#154433,
#154434,#154435,#154436,#154437,#154438,#154439,#154440,#154441,#154442,
#154443,#154444,#154445,#154446,#154447,#154448,#154449,#154450,#154451,
#154452,#154453,#154454,#154455,#154456,#154457,#154458,#154459,#154460,
#154461,#154462,#154463,#154464,#154465,#154466,#154467,#154468,#154469,
#154470,#154471,#154472,#154473,#154474,#154475,#154476,#154477,#154478,
#154479,#154480,#154481,#154482,#154483,#154484,#154485,#154486,#154487,
#154488,#154489,#154490,#154491,#154492,#154493,#154494,#154495,#154496,
#154497,#154498,#154499,#154500,#154501,#154502,#154503,#154504,#154505,
#154506,#154507,#154508,#154509,#154510,#154511,#154512,#154513,#154514,
#154515,#154516,#154517,#154518,#154519,#154520,#154521,#154522,#154523,
#154524,#154525,#154526,#154527,#154528,#154529,#154530,#154531,#154532,
#154533,#154534,#154535,#154536,#154537,#154538,#154539,#154540,#154541,
#154542,#154543,#154544,#154545,#154546,#154547,#154548,#154549,#154550,
#154551,#154552,#154553,#154554,#154555,#154556,#154557,#154558,#154559,
#154560,#154561,#154562,#154563,#154564,#154565,#154566,#154567,#154568,
#154569,#154570,#154571,#154572,#154573,#154574,#154575,#154576,#154577,
#154578,#154579,#154580,#154581,#154582,#154583,#154584,#154585,#154586,
#154587,#154588,#154589,#154590,#154591,#154592,#154593,#154594,#154595,
#154596,#154597,#154598,#154599,#154600,#154601,#154602,#154603,#154604,
#154605,#154606,#154607,#154608,#154609,#154610,#154611,#154612,#154613,
#154614,#154615,#154616,#154617,#154618,#154619,#154620,#154621,#154622,
#154623,#154624,#154625,#154626,#154627,#154628,#154629,#154630,#154631,
#154632,#154633,#154634,#154635,#154636),.UNSPECIFIED.,.F.,.F.,(4,3,3,3,
3,3,3,3,3,3,3,3,3,3,3,3,3,3,3,3,3,3,3,3,3,3,3,3,3,3,3,3,3,3,3,3,3,3,3,3,
3,3,3,3,3,3,3,3,3,3,3,3,3,3,3,3,3,3,3,3,3,3,3,3,3,3,3,3,3,3,3,3,3,3,3,3,
3,3,4),(-91.8176497547249,-91.7182119685907,-91.6425022974724,-91.5668412954458,
-91.4912144551078,-91.4155967588247,-91.3399852587375,-91.2643453341091,
-91.2197434252831,-91.1374646534299,-91.0551620905675,-90.9716902884195,
-90.889335333522,-90.8053051077488,-90.7212748819755,-90.6388958713735,
-90.5565316821242,-90.4731003462601,-90.3907783729674,-90.3067923558177,
-90.222806338668,-90.1471662294466,-90.0715501265406,-89.995943559487,-89.9203088967776,
-89.8446593381999,-89.7689490484231,-89.7243377953604,-89.6324372256577,
-89.5404042559442,-89.4485246861222,-89.3568972900923,-89.2658761686112,
-89.2258692520529,-89.1518673373648,-89.0778864090216,-89.0039113871093,
-88.9298989138093,-88.8558676438278,-88.7817628916227,-88.7274007087453,
-88.6484392927982,-88.569531869729,-88.4906668307924,-88.4118326000669,
-88.3330176260878,-88.2541963624276,-88.1753697233152,-88.0965271989387,
-88.0176582703557,-87.9387162190243,-87.8597354535355,-87.7806644425174,
-87.7304636221302,-87.6514717267914,-87.5725799421166,-87.4937776860723,
-87.4150776852505,-87.3364382393722,-87.2578619571867,-87.2319950788226,
-87.1534083556589,-87.0747721883961,-86.9960761950799,-86.9172621635974,
-86.8383807353739,-86.7593776421582,-86.7335265355151,-86.6544473002854,
-86.5754422403857,-86.4964996701987,-86.4176158351969,-86.3387667922288,
-86.2599420069206,-86.1811309618265,-86.1023075062359,-86.0234798687421,
-85.9446144097895,-85.8904867273958),.UNSPECIFIED.);
#3123=B_SPLINE_CURVE_WITH_KNOTS('',3,(#154642,#154643,#154644,#154645,#154646,
#154647,#154648,#154649,#154650,#154651,#154652,#154653,#154654,#154655,
#154656,#154657,#154658,#154659,#154660,#154661,#154662,#154663,#154664,
#154665,#154666,#154667,#154668,#154669,#154670,#154671,#154672,#154673,
#154674,#154675,#154676,#154677,#154678,#154679,#154680,#154681,#154682,
#154683,#154684,#154685,#154686,#154687,#154688,#154689,#154690,#154691,
#154692,#154693,#154694,#154695,#154696,#154697,#154698,#154699,#154700,
#154701,#154702,#154703,#154704,#154705,#154706,#154707,#154708,#154709,
#154710,#154711,#154712,#154713,#154714,#154715,#154716,#154717,#154718,
#154719,#154720,#154721,#154722,#154723,#154724,#154725,#154726,#154727,
#154728,#154729,#154730,#154731,#154732,#154733,#154734,#154735,#154736,
#154737,#154738,#154739,#154740,#154741,#154742,#154743,#154744,#154745,
#154746,#154747,#154748,#154749,#154750,#154751,#154752,#154753,#154754,
#154755,#154756,#154757,#154758,#154759,#154760,#154761,#154762,#154763,
#154764,#154765,#154766,#154767,#154768,#154769,#154770,#154771,#154772,
#154773,#154774,#154775,#154776,#154777,#154778,#154779,#154780,#154781,
#154782,#154783,#154784,#154785,#154786,#154787,#154788,#154789,#154790,
#154791,#154792,#154793,#154794,#154795,#154796,#154797,#154798,#154799,
#154800,#154801,#154802,#154803,#154804,#154805,#154806,#154807,#154808,
#154809,#154810,#154811,#154812,#154813,#154814,#154815,#154816,#154817,
#154818,#154819,#154820,#154821,#154822,#154823,#154824,#154825,#154826,
#154827,#154828,#154829,#154830,#154831,#154832,#154833,#154834,#154835,
#154836,#154837,#154838,#154839,#154840,#154841,#154842,#154843,#154844,
#154845,#154846,#154847,#154848,#154849,#154850,#154851,#154852,#154853,
#154854,#154855,#154856,#154857,#154858,#154859,#154860,#154861),
 .UNSPECIFIED.,.F.,.F.,(4,3,3,3,3,3,3,3,3,3,3,3,3,3,3,3,3,3,3,3,3,3,3,3,
3,3,3,3,3,3,3,3,3,3,3,3,3,3,3,3,3,3,3,3,3,3,3,3,3,3,3,3,3,3,3,3,3,3,3,3,
3,3,3,3,3,3,3,3,3,3,3,3,3,4),(83.3467333304285,83.4284632041948,83.5101929579649,
83.5919225934066,83.6736521121857,83.7553815159691,83.8371108064235,83.9220575749427,
84.0056770502037,84.0879899711638,84.1697288802311,84.2514673696174,84.3332054459974,
84.4149431160448,84.4966803864333,84.5784172638362,84.6601537549263,84.7418898663764,
84.8236256048585,84.9053609770448,84.9870959896069,85.0688306492161,85.1505649625434,
85.2322989362597,85.3140325770352,85.3957658915402,85.4774988864446,85.5592315684181,
85.6409639441299,85.7226960202491,85.8044278034446,85.8861593003851,85.9678905177387,
86.0496214621738,86.1313521403579,86.2130825589589,86.2948127246442,86.3765426440807,
86.4582723239359,86.5400017708761,86.6254299652753,86.7081885285996,86.7899271561628,
86.8716649599667,86.9534019667064,87.0351382030743,87.11687369576,87.1986084714508,
87.2803425568315,87.3620759785842,87.4438087633892,87.5255409379243,87.6072725288654,
87.6890035628865,87.7707340666591,87.8524640668536,87.9341935901381,88.0179129902326,
88.099651071261,88.1813875666854,88.2631225832699,88.3448562277583,88.4265886068752,
88.5083198273283,88.5900499958087,88.6755067452889,88.7572436635079,88.8389776724112,
88.9207091989303,89.0024386698586,89.0841735603345,89.1659036404995,89.247635069561,
89.2737039916508),.UNSPECIFIED.);
#3124=B_SPLINE_CURVE_WITH_KNOTS('',3,(#154862,#154863,#154864,#154865,#154866,
#154867,#154868,#154869,#154870,#154871,#154872,#154873,#154874),
 .UNSPECIFIED.,.F.,.F.,(4,3,3,3,4),(89.2737039916508,89.3656387825245,89.4579312834165,
89.5504795579867,89.6300395101817),.UNSPECIFIED.);
#3125=B_SPLINE_CURVE_WITH_KNOTS('',3,(#154876,#154877,#154878,#154879,#154880,
#154881,#154882,#154883,#154884,#154885,#154886,#154887,#154888,#154889,
#154890,#154891),.UNSPECIFIED.,.F.,.F.,(4,3,3,3,3,4),(-85.8904867273958,
-85.8115303384309,-85.7365894489,-85.6536039327013,-85.5708503337389,-85.5344644475453),
 .UNSPECIFIED.);
#3126=B_SPLINE_CURVE_WITH_KNOTS('',3,(#154892,#154893,#154894,#154895,#154896,
#154897,#154898,#154899,#154900,#154901,#154902,#154903,#154904,#154905,
#154906,#154907,#154908,#154909,#154910,#154911,#154912,#154913,#154914,
#154915,#154916,#154917,#154918,#154919,#154920,#154921,#154922,#154923,
#154924,#154925,#154926,#154927,#154928,#154929,#154930,#154931,#154932,
#154933,#154934,#154935,#154936,#154937,#154938,#154939,#154940,#154941,
#154942,#154943,#154944,#154945,#154946,#154947,#154948,#154949,#154950,
#154951,#154952,#154953,#154954,#154955,#154956,#154957,#154958,#154959,
#154960,#154961,#154962,#154963,#154964,#154965,#154966,#154967,#154968,
#154969,#154970,#154971,#154972,#154973,#154974,#154975,#154976,#154977,
#154978,#154979,#154980,#154981,#154982,#154983,#154984,#154985,#154986,
#154987,#154988,#154989,#154990,#154991,#154992,#154993,#154994,#154995,
#154996,#154997,#154998,#154999,#155000,#155001,#155002,#155003,#155004,
#155005,#155006,#155007,#155008,#155009,#155010,#155011,#155012,#155013,
#155014,#155015,#155016,#155017,#155018,#155019,#155020,#155021,#155022,
#155023,#155024,#155025,#155026,#155027,#155028,#155029,#155030,#155031,
#155032,#155033,#155034,#155035,#155036,#155037,#155038,#155039,#155040,
#155041,#155042,#155043,#155044,#155045,#155046,#155047,#155048,#155049,
#155050,#155051,#155052,#155053,#155054,#155055,#155056,#155057,#155058,
#155059,#155060,#155061,#155062,#155063,#155064,#155065,#155066,#155067,
#155068,#155069,#155070,#155071,#155072,#155073,#155074,#155075,#155076,
#155077,#155078,#155079,#155080,#155081,#155082,#155083,#155084,#155085,
#155086,#155087,#155088,#155089,#155090,#155091,#155092,#155093,#155094,
#155095,#155096,#155097,#155098,#155099,#155100,#155101,#155102,#155103,
#155104,#155105,#155106,#155107,#155108,#155109,#155110,#155111,#155112,
#155113,#155114,#155115,#155116,#155117,#155118,#155119,#155120,#155121,
#155122,#155123,#155124,#155125,#155126,#155127,#155128,#155129),
 .UNSPECIFIED.,.F.,.F.,(4,3,3,3,3,3,3,3,3,3,3,3,3,3,3,3,3,3,3,3,3,3,3,3,
3,3,3,3,3,3,3,3,3,3,3,3,3,3,3,3,3,3,3,3,3,3,3,3,3,3,3,3,3,3,3,3,3,3,3,3,
3,3,3,3,3,3,3,3,3,3,3,3,3,3,3,3,3,3,3,4),(-85.534464447435,-85.4603785619744,
-85.389367063574,-85.3183605525203,-85.2473304895041,-85.2381209055924,
-85.1471218058569,-85.0556185881807,-84.9636750492508,-84.8716404720719,
-84.7797313819514,-84.7396523622849,-84.6639426911673,-84.5882816891414,
-84.5126548488037,-84.4370371525214,-84.3614256524346,-84.2857857278067,
-84.2411838189773,-84.1589050471238,-84.0766024842607,-83.993130682113,
-83.910775727215,-83.8267455014424,-83.7427152756697,-83.6603362650678,
-83.5779720758183,-83.4945407399542,-83.4122187666616,-83.3282327495119,
-83.2442467323622,-83.1686066231408,-83.0929905202347,-83.0173839531808,
-82.9417492904714,-82.8660997318935,-82.7903894421167,-82.7457781890546,
-82.6538776193516,-82.561844649637,-82.469965079815,-82.3783376837873,-82.2873165623051,
-82.2473096457471,-82.1733077310589,-82.0993268027156,-82.0253517808033,
-81.9513393075032,-81.8773080375218,-81.8032032853168,-81.7488411024395,
-81.6698796864922,-81.5909722634228,-81.5121072244858,-81.4332729937596,
-81.3544580197812,-81.2756367561211,-81.1968101170086,-81.1179675926322,
-81.0390986640493,-80.9601566127179,-80.8811758472291,-80.802104836211,
-80.7519040158244,-80.6729121204856,-80.5940203358109,-80.5152180797672,
-80.4365180789458,-80.3578786330677,-80.2793023508825,-80.2534354725168,
-80.1748487493532,-80.0962125820902,-80.0175165887737,-79.9387025572909,
-79.8598211290667,-79.7808180358505,-79.7549669292093,-79.67261042862,-79.6072239344785),
 .UNSPECIFIED.);
#3127=B_SPLINE_CURVE_WITH_KNOTS('',3,(#155135,#155136,#155137,#155138,#155139,
#155140,#155141,#155142,#155143,#155144,#155145,#155146,#155147,#155148,
#155149,#155150,#155151,#155152,#155153,#155154,#155155,#155156,#155157,
#155158,#155159,#155160,#155161,#155162,#155163,#155164,#155165,#155166,
#155167,#155168,#155169,#155170,#155171,#155172,#155173,#155174,#155175,
#155176,#155177,#155178,#155179,#155180,#155181,#155182,#155183,#155184,
#155185,#155186,#155187,#155188,#155189,#155190,#155191,#155192,#155193,
#155194,#155195,#155196,#155197,#155198,#155199,#155200,#155201,#155202,
#155203,#155204,#155205,#155206,#155207,#155208,#155209,#155210,#155211,
#155212,#155213,#155214,#155215,#155216,#155217,#155218,#155219,#155220,
#155221,#155222,#155223,#155224,#155225,#155226,#155227,#155228,#155229,
#155230,#155231,#155232,#155233,#155234,#155235,#155236,#155237,#155238,
#155239,#155240,#155241,#155242,#155243,#155244,#155245,#155246,#155247,
#155248,#155249,#155250,#155251,#155252,#155253,#155254,#155255,#155256,
#155257,#155258,#155259,#155260,#155261,#155262,#155263,#155264,#155265,
#155266,#155267,#155268,#155269,#155270,#155271,#155272,#155273,#155274,
#155275,#155276,#155277,#155278,#155279,#155280,#155281,#155282,#155283,
#155284,#155285,#155286,#155287,#155288,#155289,#155290,#155291,#155292,
#155293,#155294,#155295,#155296,#155297,#155298,#155299,#155300,#155301,
#155302,#155303,#155304,#155305,#155306,#155307,#155308,#155309,#155310,
#155311,#155312,#155313,#155314,#155315,#155316,#155317,#155318,#155319,
#155320,#155321,#155322,#155323,#155324,#155325,#155326,#155327,#155328,
#155329,#155330,#155331,#155332,#155333,#155334,#155335,#155336,#155337,
#155338,#155339,#155340,#155341,#155342,#155343,#155344,#155345,#155346,
#155347,#155348,#155349,#155350,#155351,#155352,#155353,#155354,#155355,
#155356,#155357,#155358,#155359,#155360,#155361,#155362,#155363,#155364,
#155365,#155366,#155367,#155368,#155369,#155370,#155371,#155372,#155373,
#155374,#155375),.UNSPECIFIED.,.F.,.F.,(4,3,3,3,3,3,3,3,3,3,3,3,3,3,3,3,
3,3,3,3,3,3,3,3,3,3,3,3,3,3,3,3,3,3,3,3,3,3,3,3,3,3,3,3,3,3,3,3,3,3,3,3,
3,3,3,3,3,3,3,3,3,3,3,3,3,3,3,3,3,3,3,3,3,3,3,3,3,3,3,3,4),(77.0637438066728,
77.1460509018794,77.2283272461551,77.2626242126715,77.3382643218935,77.4138804248002,
77.4894869918545,77.5651216545645,77.640771213143,77.7164815029205,77.7610927559791,
77.8529933256816,77.9450262953949,78.0369058652165,78.128533261245,78.2195543827259,
78.2595612992866,78.3335632139748,78.4075441423182,78.4815191642309,78.5555316375308,
78.6295629075121,78.7036676597172,78.7580298425942,78.8369912585414,78.9158986816107,
78.9947637205473,79.0735979512731,79.1524129252519,79.2312341889121,79.3100608280245,
79.3889033524008,79.4677722809837,79.5467143323151,79.625695097804,79.7047661088221,
79.7549669292093,79.8339588245478,79.9128506092226,79.9916528652669,80.0703528660884,
80.1489923119669,80.2275685941521,80.2534354725169,80.3320221956804,80.4106583629434,
80.4893543562597,80.5681683877424,80.647049815966,80.7260529091818,80.7519040158244,
80.830976537574,80.9099760923091,80.9889143601331,81.0678029746144,81.1466535311706,
81.2254820354363,81.3042984093052,81.3831131604889,81.4619367944664,81.5408068420147,
81.6197005210906,81.6986610459276,81.7488411024395,81.8229465405415,81.896995038396,
81.9710017764029,82.0449910405556,82.1189684021677,82.1929706882008,82.2473096457471,
82.338308745483,82.4298119631601,82.5217555020904,82.6137900792692,82.7056991693903,
82.7457781890547,82.8222589565696,82.8986881147001,82.9750730542511,82.9905186844712),
 .UNSPECIFIED.);
#3128=B_SPLINE_CURVE_WITH_KNOTS('',3,(#155376,#155377,#155378,#155379,#155380,
#155381,#155382,#155383,#155384,#155385,#155386,#155387,#155388,#155389,
#155390,#155391),.UNSPECIFIED.,.F.,.F.,(4,3,3,3,3,4),(82.9905186844712,
83.0722482283072,83.1539833432262,83.2357135805754,83.3174453695265,83.3467333304285),
 .UNSPECIFIED.);
#3129=B_SPLINE_CURVE_WITH_KNOTS('',3,(#155393,#155394,#155395,#155396,#155397,
#155398,#155399,#155400,#155401,#155402,#155403,#155404,#155405,#155406,
#155407,#155408),.UNSPECIFIED.,.F.,.F.,(4,3,3,3,3,4),(-79.6072239344785,
-79.5250325657862,-79.4429820957931,-79.3610225518867,-79.2791885693329,
-79.2512791403658),.UNSPECIFIED.);
#3130=B_SPLINE_CURVE_WITH_KNOTS('',3,(#155409,#155410,#155411,#155412,#155413,
#155414,#155415,#155416,#155417,#155418,#155419,#155420,#155421,#155422,
#155423,#155424,#155425,#155426,#155427,#155428,#155429,#155430,#155431,
#155432,#155433,#155434,#155435,#155436,#155437,#155438,#155439,#155440,
#155441,#155442,#155443,#155444,#155445,#155446,#155447,#155448,#155449,
#155450,#155451,#155452,#155453,#155454,#155455,#155456,#155457,#155458,
#155459,#155460,#155461,#155462,#155463,#155464,#155465,#155466,#155467,
#155468,#155469,#155470,#155471,#155472,#155473,#155474,#155475,#155476,
#155477,#155478,#155479,#155480,#155481,#155482,#155483,#155484,#155485,
#155486,#155487,#155488,#155489,#155490,#155491,#155492,#155493,#155494,
#155495,#155496,#155497,#155498,#155499,#155500,#155501,#155502,#155503,
#155504,#155505,#155506,#155507,#155508,#155509,#155510,#155511,#155512,
#155513,#155514,#155515,#155516,#155517,#155518,#155519,#155520,#155521,
#155522,#155523,#155524,#155525,#155526,#155527,#155528,#155529,#155530,
#155531,#155532,#155533,#155534,#155535,#155536,#155537,#155538,#155539,
#155540,#155541,#155542,#155543,#155544,#155545,#155546,#155547,#155548,
#155549,#155550,#155551,#155552,#155553,#155554,#155555,#155556,#155557,
#155558,#155559,#155560,#155561,#155562,#155563,#155564,#155565,#155566,
#155567,#155568,#155569,#155570,#155571,#155572,#155573,#155574,#155575,
#155576,#155577,#155578,#155579,#155580,#155581,#155582,#155583,#155584,
#155585,#155586,#155587,#155588,#155589,#155590,#155591,#155592,#155593,
#155594,#155595,#155596,#155597,#155598,#155599,#155600,#155601,#155602,
#155603,#155604,#155605,#155606,#155607,#155608,#155609,#155610,#155611,
#155612,#155613,#155614,#155615,#155616,#155617,#155618,#155619,#155620,
#155621,#155622,#155623,#155624,#155625,#155626,#155627,#155628,#155629,
#155630,#155631,#155632,#155633,#155634,#155635,#155636,#155637,#155638,
#155639,#155640),.UNSPECIFIED.,.F.,.F.,(4,3,3,3,3,3,3,3,3,3,3,3,3,3,3,3,
3,3,3,3,3,3,3,3,3,3,3,3,3,3,3,3,3,3,3,3,3,3,3,3,3,3,3,3,3,3,3,3,3,3,3,3,
3,3,3,3,3,3,3,3,3,3,3,3,3,3,3,3,3,3,3,3,3,3,3,3,3,4),(-79.2512785228306,
-79.1677334496107,-79.0840691932055,-79.0002387934004,-78.9163372798076,
-78.8323326741379,-78.7580298425942,-78.6839244044922,-78.6098759066377,
-78.5358691686304,-78.4618799044777,-78.3879025428657,-78.3139002568326,
-78.2595612992866,-78.1685621995506,-78.0770589818738,-77.9851154429436,
-77.8930808657643,-77.8011717756431,-77.761092755979,-77.6853830848615,
-77.6097220828355,-77.5340952424979,-77.4584775462156,-77.382866046129,
-77.3072261215013,-77.2626242126715,-77.180345440818,-77.0980428779547,
-77.014571075807,-76.9322161209089,-76.8481858951364,-76.7641556693639,
-76.681776658762,-76.5994124695124,-76.5159811336484,-76.4336591603557,
-76.349673143206,-76.2656871260564,-76.1900470168349,-76.1144309139291,
-76.0388243468752,-75.9631896841656,-75.8875401255878,-75.8118298358109,
-75.7672185827488,-75.6753180130453,-75.5832850433304,-75.4914054735083,
-75.3997780774793,-75.3087569559981,-75.2687500394412,-75.1947481247532,
-75.1207671964098,-75.0467921744976,-74.9727797011978,-74.8987484312166,
-74.8246436790119,-74.7702814961337,-74.6913200801863,-74.6124126571173,
-74.5335476181811,-74.4547133874553,-74.3758984134772,-74.2970771498171,
-74.2182505107048,-74.1394079863288,-74.0605390577459,-73.9815970064143,
-73.9026162409256,-73.8235452299075,-73.7733444095186,-73.6943456368794,
-73.6154474967274,-73.5366695691337,-73.4579618401987,-73.3793327385231,
-73.3240852745455),.UNSPECIFIED.);
#3131=B_SPLINE_CURVE_WITH_KNOTS('',3,(#155646,#155647,#155648,#155649,#155650,
#155651,#155652,#155653,#155654,#155655,#155656,#155657,#155658,#155659,
#155660,#155661,#155662,#155663,#155664,#155665,#155666,#155667,#155668,
#155669,#155670,#155671,#155672,#155673,#155674,#155675,#155676,#155677,
#155678,#155679,#155680,#155681,#155682,#155683,#155684,#155685,#155686,
#155687,#155688,#155689,#155690,#155691,#155692,#155693,#155694,#155695,
#155696,#155697,#155698,#155699,#155700,#155701,#155702,#155703,#155704,
#155705,#155706,#155707,#155708,#155709,#155710,#155711,#155712,#155713,
#155714,#155715,#155716,#155717,#155718,#155719,#155720,#155721,#155722,
#155723,#155724,#155725,#155726,#155727,#155728,#155729,#155730,#155731,
#155732,#155733,#155734,#155735,#155736,#155737,#155738,#155739,#155740,
#155741,#155742,#155743,#155744,#155745,#155746,#155747,#155748,#155749,
#155750,#155751,#155752,#155753,#155754,#155755,#155756,#155757,#155758,
#155759,#155760,#155761,#155762,#155763,#155764,#155765,#155766,#155767,
#155768,#155769,#155770,#155771,#155772,#155773,#155774,#155775,#155776,
#155777,#155778,#155779,#155780,#155781,#155782,#155783,#155784,#155785,
#155786,#155787,#155788,#155789,#155790,#155791,#155792,#155793,#155794,
#155795,#155796,#155797,#155798,#155799,#155800,#155801,#155802,#155803,
#155804,#155805,#155806,#155807,#155808,#155809,#155810,#155811,#155812,
#155813,#155814,#155815,#155816,#155817,#155818,#155819,#155820,#155821,
#155822,#155823,#155824,#155825,#155826,#155827,#155828,#155829,#155830,
#155831,#155832,#155833,#155834,#155835,#155836,#155837,#155838,#155839,
#155840,#155841,#155842,#155843,#155844,#155845,#155846,#155847,#155848,
#155849,#155850,#155851,#155852,#155853,#155854,#155855,#155856,#155857,
#155858,#155859,#155860,#155861,#155862,#155863,#155864,#155865,#155866,
#155867,#155868,#155869,#155870,#155871,#155872,#155873,#155874,#155875,
#155876,#155877,#155878,#155879,#155880,#155881,#155882,#155883,#155884,
#155885,#155886),.UNSPECIFIED.,.F.,.F.,(4,3,3,3,3,3,3,3,3,3,3,3,3,3,3,3,
3,3,3,3,3,3,3,3,3,3,3,3,3,3,3,3,3,3,3,3,3,3,3,3,3,3,3,3,3,3,3,3,3,3,3,3,
3,3,3,3,3,3,3,3,3,3,3,3,3,3,3,3,3,3,3,3,3,3,3,3,3,3,3,3,4),(70.7799867132232,
70.7825331496733,70.8744337193759,70.9664666890899,71.058346258912,71.1499736549409,
71.2409947764223,71.2810016929808,71.355003607669,71.4289845360125,71.5029595579251,
71.5769720312251,71.6510033012064,71.7251080534115,71.7794702362884,71.8584316522356,
71.9373390753048,72.0162041142414,72.0950383449674,72.1738533189461,72.2526745826062,
72.3315012217186,72.4103437460949,72.4892126746776,72.568154726009,72.6471354914978,
72.726206502516,72.7764073229035,72.855399218242,72.9342910029167,73.0130932589609,
73.0917932597823,73.1704327056608,73.249008987846,73.274875866211,73.3534625893746,
73.4320987566377,73.5107947499542,73.5896087814371,73.6684902096608,73.7474933028768,
73.7733444095186,73.8524169312682,73.9314164860032,74.0103547538272,74.0892433683085,
74.1680939248648,74.2469224291305,74.3257388029993,74.4045535541831,74.4833771881605,
74.5622472357088,74.6411409147846,74.7201014396216,74.7702814961337,74.8443869342357,
74.9184354320902,74.9924421700973,75.06643143425,75.1404087958621,75.2144110818953,
75.2687500394413,75.359749139177,75.4512523568538,75.5431958957836,75.6352304729624,
75.7271395630831,75.7672185827488,75.8429282538665,75.9185892558926,75.9942160962305,
76.0698337925129,76.1454452925997,76.2210852172276,76.2656871260564,76.3479703571948,
76.4302779995685,76.5126237436815,76.5949809727244,76.6773585381553,76.7073333772916),
 .UNSPECIFIED.);
#3132=B_SPLINE_CURVE_WITH_KNOTS('',3,(#155887,#155888,#155889,#155890,#155891,
#155892,#155893,#155894,#155895,#155896,#155897,#155898,#155899,#155900,
#155901,#155902),.UNSPECIFIED.,.F.,.F.,(4,3,3,3,3,4),(76.7073333773951,
76.764155669364,76.8465358442871,76.9289000222271,77.0112452878717,77.0637438066728),
 .UNSPECIFIED.);
#3133=B_SPLINE_CURVE_WITH_KNOTS('',3,(#155904,#155905,#155906,#155907,#155908,
#155909,#155910,#155911,#155912,#155913,#155914,#155915,#155916,#155917,
#155918,#155919),.UNSPECIFIED.,.F.,.F.,(4,3,3,3,3,4),(-73.3240852745455,
-73.274875866211,-73.1981803579767,-73.1235307356291,-73.0458122844514,
-72.9680938332738),.UNSPECIFIED.);
#3134=B_SPLINE_CURVE_WITH_KNOTS('',3,(#155920,#155921,#155922,#155923,#155924,
#155925,#155926,#155927,#155928,#155929,#155930,#155931,#155932,#155933,
#155934,#155935,#155936,#155937,#155938,#155939,#155940,#155941,#155942,
#155943,#155944,#155945,#155946,#155947,#155948,#155949,#155950,#155951,
#155952,#155953,#155954,#155955,#155956,#155957,#155958,#155959,#155960,
#155961,#155962,#155963,#155964,#155965,#155966,#155967,#155968,#155969,
#155970,#155971,#155972,#155973,#155974,#155975,#155976,#155977,#155978,
#155979,#155980,#155981,#155982,#155983,#155984,#155985,#155986,#155987,
#155988,#155989,#155990,#155991,#155992,#155993,#155994,#155995,#155996,
#155997,#155998,#155999,#156000,#156001,#156002,#156003,#156004,#156005,
#156006,#156007,#156008,#156009,#156010,#156011,#156012,#156013,#156014,
#156015,#156016,#156017,#156018,#156019,#156020,#156021,#156022,#156023,
#156024,#156025,#156026,#156027,#156028,#156029,#156030,#156031,#156032,
#156033,#156034,#156035,#156036,#156037,#156038,#156039,#156040,#156041,
#156042,#156043,#156044,#156045,#156046,#156047,#156048,#156049,#156050,
#156051,#156052,#156053,#156054,#156055,#156056,#156057,#156058,#156059,
#156060,#156061,#156062,#156063,#156064,#156065,#156066,#156067,#156068,
#156069,#156070,#156071,#156072,#156073,#156074,#156075,#156076,#156077,
#156078,#156079,#156080,#156081,#156082,#156083,#156084,#156085,#156086,
#156087,#156088,#156089,#156090,#156091,#156092,#156093,#156094,#156095,
#156096,#156097,#156098,#156099,#156100,#156101,#156102,#156103,#156104,
#156105,#156106,#156107,#156108,#156109,#156110,#156111,#156112,#156113,
#156114,#156115,#156116,#156117,#156118,#156119,#156120,#156121,#156122,
#156123,#156124,#156125,#156126,#156127,#156128,#156129,#156130,#156131,
#156132,#156133,#156134,#156135,#156136,#156137,#156138,#156139,#156140,
#156141,#156142,#156143,#156144,#156145,#156146,#156147,#156148,#156149,
#156150,#156151),.UNSPECIFIED.,.F.,.F.,(4,3,3,3,3,3,3,3,3,3,3,3,3,3,3,3,
3,3,3,3,3,3,3,3,3,3,3,3,3,3,3,3,3,3,3,3,3,3,3,3,3,3,3,3,3,3,3,3,3,3,3,3,
3,3,3,3,3,3,3,3,3,3,3,3,3,3,3,3,3,3,3,3,3,3,3,3,3,4),(-72.9680938331862,
-72.8722505780449,-72.7764073229035,-72.6973348011539,-72.6183352464187,
-72.5393969785947,-72.4605083641133,-72.3816578075571,-72.3028293032914,
-72.2240129294225,-72.1451981782387,-72.0663745442612,-71.9875044967129,
-71.908610817637,-71.8296502928,-71.7794702362883,-71.7053647981864,-71.6313163003318,
-71.5573095623247,-71.4833202981721,-71.4093429365601,-71.3353406505269,
-71.2810016929808,-71.1900025932449,-71.0984993755676,-71.0065558366373,
-70.9145212594584,-70.8226121693373,-70.7825331496732,-70.7068234785557,
-70.6311624765299,-70.5555356361924,-70.4799179399102,-70.4043064398236,
-70.3286665151959,-70.2840646063657,-70.2017858345122,-70.1194832716494,
-70.0360114695015,-69.9536565146034,-69.8696262888308,-69.7855960630581,
-69.7032170524562,-69.6208528632067,-69.5374215273427,-69.4550995540499,
-69.3711135369003,-69.2871275197506,-69.2114874105292,-69.1358713076231,
-69.0602647405694,-68.98463007786,-68.9089805192822,-68.8332702295053,-68.788658976443,
-68.69675840674,-68.6047254370263,-68.5128458672042,-68.4212184711754,-68.3301973496942,
-68.2901904331355,-68.2161885184473,-68.1422075901039,-68.0682325681916,
-67.9942200948916,-67.9201888249102,-67.8460840727052,-67.7917218898279,
-67.7127532835095,-67.6338405959854,-67.5549769868227,-67.4761421238226,
-67.3973254830067,-67.3185165534304,-67.2396875472761,-67.160849079403,
-67.0819685455894,-67.0415072947074),.UNSPECIFIED.);
#3135=B_SPLINE_CURVE_WITH_KNOTS('',3,(#156157,#156158,#156159,#156160,#156161,
#156162,#156163,#156164,#156165,#156166,#156167,#156168,#156169,#156170,
#156171,#156172,#156173,#156174,#156175,#156176,#156177,#156178,#156179,
#156180,#156181,#156182,#156183,#156184,#156185,#156186,#156187,#156188,
#156189,#156190,#156191,#156192,#156193,#156194,#156195,#156196,#156197,
#156198,#156199,#156200,#156201,#156202,#156203,#156204,#156205,#156206,
#156207,#156208,#156209,#156210,#156211,#156212,#156213,#156214,#156215,
#156216,#156217,#156218,#156219,#156220,#156221,#156222,#156223,#156224,
#156225,#156226,#156227,#156228,#156229,#156230,#156231,#156232,#156233,
#156234,#156235,#156236,#156237,#156238,#156239,#156240,#156241,#156242,
#156243,#156244,#156245,#156246,#156247,#156248,#156249,#156250,#156251,
#156252,#156253,#156254,#156255,#156256,#156257,#156258,#156259,#156260,
#156261,#156262,#156263,#156264,#156265,#156266,#156267,#156268,#156269,
#156270,#156271,#156272,#156273,#156274,#156275,#156276,#156277,#156278,
#156279,#156280,#156281,#156282,#156283,#156284,#156285,#156286,#156287,
#156288,#156289,#156290,#156291,#156292,#156293,#156294,#156295,#156296,
#156297,#156298,#156299,#156300,#156301,#156302,#156303,#156304,#156305,
#156306,#156307,#156308,#156309,#156310,#156311,#156312,#156313,#156314,
#156315,#156316,#156317,#156318,#156319,#156320,#156321,#156322,#156323,
#156324,#156325,#156326,#156327,#156328,#156329,#156330,#156331,#156332,
#156333,#156334,#156335,#156336,#156337,#156338,#156339,#156340,#156341,
#156342,#156343,#156344,#156345,#156346,#156347,#156348,#156349,#156350,
#156351,#156352,#156353,#156354,#156355,#156356,#156357,#156358,#156359,
#156360,#156361,#156362,#156363,#156364,#156365,#156366,#156367,#156368,
#156369,#156370,#156371,#156372,#156373,#156374,#156375,#156376),
 .UNSPECIFIED.,.F.,.F.,(4,3,3,3,3,3,3,3,3,3,3,3,3,3,3,3,3,3,3,3,3,3,3,3,
3,3,3,3,3,3,3,3,3,3,3,3,3,3,3,3,3,3,3,3,3,3,3,3,3,3,3,3,3,3,3,3,3,3,3,3,
3,3,3,3,3,3,3,3,3,3,3,3,3,4),(64.4971774088899,64.5789072826559,64.6606370364263,
64.7423666718676,64.8240961906468,64.9058255944302,64.9875548848845,65.0725016534037,
65.1561211286648,65.2384340496249,65.3201729586921,65.4019114480785,65.4836495244585,
65.5653871945059,65.6471244648944,65.7288613422973,65.8105978333875,65.8923339448375,
65.9740696833197,66.055805055506,66.1375400680681,66.2192747276772,66.3010090410045,
66.3827430147207,66.4644766554963,66.5462099700013,66.6279429649057,66.7096756468792,
66.7914080225911,66.8731400987103,66.9548718819059,67.0366033788464,67.1183345962,
67.200065540635,67.2817962188191,67.3635266374201,67.4452568031052,67.5269867225418,
67.6087164023969,67.6904458493373,67.7758740437365,67.8586326070607,67.940371234624,
68.0221090384279,68.1038460451676,68.1855822815355,68.2673177742213,68.3490525499121,
68.4307866352927,68.5125200570455,68.5942528418505,68.6759850163858,68.757716607327,
68.839447641348,68.9211781451206,69.0029081453151,69.0846376685999,69.1683570686944,
69.2500951497228,69.3318316451472,69.4135666617318,69.4953003062201,69.5770326853371,
69.6587639057902,69.7404940742708,69.8259508237509,69.9076877419699,69.9894217508731,
70.0711532773924,70.1528827483207,70.2346176387967,70.3163477189616,70.3980791480231,
70.4241480701121),.UNSPECIFIED.);
#3136=B_SPLINE_CURVE_WITH_KNOTS('',3,(#156377,#156378,#156379,#156380,#156381,
#156382,#156383,#156384,#156385,#156386,#156387,#156388,#156389,#156390,
#156391,#156392),.UNSPECIFIED.,.F.,.F.,(4,3,3,3,3,4),(70.4241480701121,
70.4995216491135,70.5749196434235,70.6503295519316,70.7257998391169,70.7799867132232),
 .UNSPECIFIED.);
#3137=B_SPLINE_CURVE_WITH_KNOTS('',3,(#156394,#156395,#156396,#156397,#156398,
#156399,#156400,#156401,#156402,#156403,#156404,#156405,#156406,#156407,
#156408,#156409),.UNSPECIFIED.,.F.,.F.,(4,3,3,3,3,4),(-67.0415072947074,
-66.9625466064109,-66.8835422217944,-66.8044565762651,-66.7947848032128,
-66.6849085260066),.UNSPECIFIED.);
#3138=B_SPLINE_CURVE_WITH_KNOTS('',3,(#156410,#156411,#156412,#156413,#156414,
#156415,#156416,#156417,#156418,#156419,#156420,#156421,#156422,#156423,
#156424,#156425,#156426,#156427,#156428,#156429,#156430,#156431,#156432,
#156433,#156434,#156435,#156436,#156437,#156438,#156439,#156440,#156441,
#156442,#156443,#156444,#156445,#156446,#156447,#156448,#156449,#156450,
#156451,#156452,#156453,#156454,#156455,#156456,#156457,#156458,#156459,
#156460,#156461,#156462,#156463,#156464,#156465,#156466,#156467,#156468,
#156469,#156470,#156471,#156472,#156473,#156474,#156475,#156476,#156477,
#156478,#156479,#156480,#156481,#156482,#156483,#156484,#156485,#156486,
#156487,#156488,#156489,#156490,#156491,#156492,#156493,#156494,#156495,
#156496,#156497,#156498,#156499,#156500,#156501,#156502,#156503,#156504,
#156505,#156506,#156507,#156508,#156509,#156510,#156511,#156512,#156513,
#156514,#156515,#156516,#156517,#156518,#156519,#156520,#156521,#156522,
#156523,#156524,#156525,#156526,#156527,#156528,#156529,#156530,#156531,
#156532,#156533,#156534,#156535,#156536,#156537,#156538,#156539,#156540,
#156541,#156542,#156543,#156544,#156545,#156546,#156547,#156548,#156549,
#156550,#156551,#156552,#156553,#156554,#156555,#156556,#156557,#156558,
#156559,#156560,#156561,#156562,#156563,#156564,#156565,#156566,#156567,
#156568,#156569,#156570,#156571,#156572,#156573,#156574,#156575,#156576,
#156577,#156578,#156579,#156580,#156581,#156582,#156583,#156584,#156585,
#156586,#156587,#156588,#156589,#156590,#156591,#156592,#156593,#156594,
#156595,#156596,#156597,#156598,#156599,#156600,#156601,#156602,#156603,
#156604,#156605,#156606,#156607,#156608,#156609,#156610,#156611,#156612,
#156613,#156614,#156615,#156616,#156617,#156618,#156619,#156620,#156621,
#156622,#156623,#156624,#156625,#156626,#156627,#156628,#156629,#156630,
#156631,#156632,#156633,#156634,#156635,#156636,#156637,#156638,#156639,
#156640,#156641,#156642,#156643,#156644),.UNSPECIFIED.,.F.,.F.,(4,3,3,3,
3,3,3,3,3,3,3,3,3,3,3,3,3,3,3,3,3,3,3,3,3,3,3,3,3,3,3,3,3,3,3,3,3,3,3,3,
3,3,3,3,3,3,3,3,3,3,3,3,3,3,3,3,3,3,3,3,3,3,3,3,3,3,3,3,3,3,3,3,3,3,3,3,
3,3,4),(-66.6849085258952,-66.6088428877483,-66.5307112307875,-66.454794221533,
-66.3755552407191,-66.2963162599052,-66.217729536742,-66.1390933694789,
-66.0603973761627,-65.98158334468,-65.9027019164564,-65.8236988232405,-65.7978477165977,
-65.718775194848,-65.639775640113,-65.5608373722887,-65.4819487578074,-65.4030982012506,
-65.3242696969848,-65.2454533231158,-65.1666385719322,-65.0878149379551,
-65.0089448904068,-64.9300512113308,-64.8510906864937,-64.8009106299825,
-64.7268051918805,-64.6527566940262,-64.5787499560192,-64.5047606918665,
-64.4307833302543,-64.3567810442212,-64.302442086675,-64.2114429869394,
-64.1199397692619,-64.0279962303319,-63.9359616531531,-63.8440525630324,
-63.8039735433674,-63.7282638722498,-63.6526028702242,-63.5769760298864,
-63.501358333604,-63.4257468335173,-63.3501069088897,-63.3055050000599,
-63.2232262282068,-63.1409236653438,-63.0574518631959,-62.975096908298,
-62.8910666825251,-62.8070364567523,-62.7246574461501,-62.6422932569008,
-62.5588619210368,-62.4765399477438,-62.3925539305943,-62.3085679134447,
-62.2329278042234,-62.1573117013175,-62.081705134264,-62.0060704715546,
-61.9304209129773,-61.8547106232006,-61.8100993701372,-61.7181988004331,
-61.6261658307195,-61.534286260897,-61.4426588648701,-61.3516377433887,
-61.3116308268296,-61.2376289121415,-61.1636479837985,-61.0896729618857,
-61.0156604885858,-60.9416292186042,-60.8675244663993,-60.8131622835221,
-60.7582306085734),.UNSPECIFIED.);
#3139=B_SPLINE_CURVE_WITH_KNOTS('',3,(#156650,#156651,#156652,#156653,#156654,
#156655,#156656,#156657,#156658,#156659,#156660,#156661,#156662,#156663,
#156664,#156665,#156666,#156667,#156668,#156669,#156670,#156671,#156672,
#156673,#156674,#156675,#156676,#156677,#156678,#156679,#156680,#156681,
#156682,#156683,#156684,#156685,#156686,#156687,#156688,#156689,#156690,
#156691,#156692,#156693,#156694,#156695,#156696,#156697,#156698,#156699,
#156700,#156701,#156702,#156703,#156704,#156705,#156706,#156707,#156708,
#156709,#156710,#156711,#156712,#156713,#156714,#156715,#156716,#156717,
#156718,#156719,#156720,#156721,#156722,#156723,#156724,#156725,#156726,
#156727,#156728,#156729,#156730,#156731,#156732,#156733,#156734,#156735,
#156736,#156737,#156738,#156739,#156740,#156741,#156742,#156743,#156744,
#156745,#156746,#156747,#156748,#156749,#156750,#156751,#156752,#156753,
#156754,#156755,#156756,#156757,#156758,#156759,#156760,#156761,#156762,
#156763,#156764,#156765,#156766,#156767,#156768,#156769,#156770,#156771,
#156772,#156773,#156774,#156775,#156776,#156777,#156778,#156779,#156780,
#156781,#156782,#156783,#156784,#156785,#156786,#156787,#156788,#156789,
#156790,#156791,#156792,#156793,#156794,#156795,#156796,#156797,#156798,
#156799,#156800,#156801,#156802,#156803,#156804,#156805,#156806,#156807,
#156808,#156809,#156810,#156811,#156812,#156813,#156814,#156815,#156816,
#156817,#156818,#156819,#156820,#156821,#156822,#156823,#156824,#156825,
#156826,#156827,#156828,#156829,#156830,#156831,#156832,#156833,#156834,
#156835,#156836,#156837,#156838,#156839,#156840,#156841,#156842,#156843,
#156844,#156845,#156846,#156847,#156848,#156849,#156850,#156851,#156852,
#156853,#156854,#156855,#156856,#156857,#156858,#156859,#156860,#156861,
#156862,#156863,#156864,#156865,#156866,#156867,#156868,#156869,#156870,
#156871,#156872,#156873,#156874,#156875,#156876,#156877,#156878,#156879,
#156880,#156881,#156882,#156883,#156884),.UNSPECIFIED.,.F.,.F.,(4,3,3,3,
3,3,3,3,3,3,3,3,3,3,3,3,3,3,3,3,3,3,3,3,3,3,3,3,3,3,3,3,3,3,3,3,3,3,3,3,
3,3,3,3,3,3,3,3,3,3,3,3,3,3,3,3,3,3,3,3,3,3,3,3,3,3,3,3,3,3,3,3,3,3,3,3,
3,3,4),(58.2138923057233,58.2922290577518,58.3705658184217,58.4489140372679,
58.5272851692979,58.6057275535383,58.6842073400998,58.7627801355672,58.8192881102919,
58.8982800056304,58.9771717903052,59.0559740463494,59.1346740471708,59.2133134930495,
59.2918897752347,59.3177566535994,59.3963433767629,59.474979544026,59.5536755373422,
59.6324895688251,59.7113709970488,59.7903740902648,59.816225196907,59.8952977186566,
59.9742972733916,60.0532355412157,60.132124155697,60.2109747122533,60.289803216519,
60.3686195903879,60.4474343415717,60.5262579755491,60.6051280230974,60.6840217021733,
60.7629822270103,60.8131622835221,60.887267721624,60.9613162194785,61.0353229574855,
61.1093122216381,61.1832895832501,61.2572918692832,61.3116308268296,61.4026299265654,
61.4941331442422,61.5860766831724,61.6781112603513,61.7700203504723,61.8100993701372,
61.8858090412549,61.9614700432808,62.0370968836184,62.1127145799009,62.1883260799876,
62.2639660046154,62.3085679134448,62.390846685298,62.4731492481605,62.5566210503085,
62.6389760052064,62.7230062309794,62.8070364567523,62.8894154673545,62.9717796566043,
63.0552109924682,63.1375329657612,63.2215189829106,63.3055050000599,63.3811451092811,
63.4567612121871,63.5323677792406,63.6080024419499,63.6836520005274,63.7593622903041,
63.8039735433674,63.8991328275661,63.9944342542252,64.0894349263504,64.1409627629325),
 .UNSPECIFIED.);
#3140=B_SPLINE_CURVE_WITH_KNOTS('',3,(#156885,#156886,#156887,#156888,#156889,
#156890,#156891,#156892,#156893,#156894,#156895,#156896,#156897,#156898,
#156899,#156900),.UNSPECIFIED.,.F.,.F.,(4,3,3,3,3,4),(64.1409627629325,
64.2226923067685,64.3044274216875,64.3861576590365,64.4678894479876,64.4971774088899),
 .UNSPECIFIED.);
#3141=B_SPLINE_CURVE_WITH_KNOTS('',3,(#156902,#156903,#156904,#156905,#156906,
#156907,#156908,#156909,#156910,#156911,#156912,#156913,#156914),
 .UNSPECIFIED.,.F.,.F.,(4,3,3,3,4),(-60.7582306085734,-60.6691037611657,
-60.5810548876563,-60.4913890532995,-60.4017232189426),.UNSPECIFIED.);
#3142=B_SPLINE_CURVE_WITH_KNOTS('',3,(#156915,#156916,#156917,#156918,#156919,
#156920,#156921,#156922,#156923,#156924,#156925,#156926,#156927,#156928,
#156929,#156930,#156931,#156932,#156933,#156934,#156935,#156936,#156937,
#156938,#156939,#156940,#156941,#156942,#156943,#156944,#156945,#156946,
#156947,#156948,#156949,#156950,#156951,#156952,#156953,#156954,#156955,
#156956,#156957,#156958,#156959,#156960,#156961,#156962,#156963,#156964,
#156965,#156966,#156967,#156968,#156969,#156970,#156971,#156972,#156973,
#156974,#156975,#156976,#156977,#156978,#156979,#156980,#156981,#156982,
#156983,#156984,#156985,#156986,#156987,#156988,#156989,#156990,#156991,
#156992,#156993,#156994,#156995,#156996,#156997,#156998,#156999,#157000,
#157001,#157002,#157003,#157004,#157005,#157006,#157007,#157008,#157009,
#157010,#157011,#157012,#157013,#157014,#157015,#157016,#157017,#157018,
#157019,#157020,#157021,#157022,#157023,#157024,#157025,#157026,#157027,
#157028,#157029,#157030,#157031,#157032,#157033,#157034,#157035,#157036,
#157037,#157038,#157039,#157040,#157041,#157042,#157043,#157044,#157045,
#157046,#157047,#157048,#157049,#157050,#157051,#157052,#157053,#157054,
#157055,#157056,#157057,#157058,#157059,#157060,#157061,#157062,#157063,
#157064,#157065,#157066,#157067,#157068,#157069,#157070,#157071,#157072,
#157073,#157074,#157075,#157076,#157077,#157078,#157079,#157080,#157081,
#157082,#157083,#157084,#157085,#157086,#157087,#157088,#157089,#157090,
#157091,#157092,#157093,#157094,#157095,#157096,#157097,#157098,#157099,
#157100,#157101,#157102,#157103,#157104,#157105,#157106,#157107,#157108,
#157109,#157110,#157111,#157112,#157113,#157114,#157115,#157116,#157117,
#157118,#157119,#157120,#157121,#157122,#157123,#157124,#157125,#157126,
#157127,#157128,#157129,#157130,#157131,#157132,#157133,#157134,#157135,
#157136,#157137,#157138,#157139,#157140,#157141,#157142,#157143,#157144,
#157145,#157146,#157147,#157148,#157149),.UNSPECIFIED.,.F.,.F.,(4,3,3,3,
3,3,3,3,3,3,3,3,3,3,3,3,3,3,3,3,3,3,3,3,3,3,3,3,3,3,3,3,3,3,3,3,3,3,3,3,
3,3,3,3,3,3,3,3,3,3,3,3,3,3,3,3,3,3,3,3,3,3,3,3,3,3,3,3,3,3,3,3,3,3,3,3,
3,3,4),(-60.401723218827,-60.3220092933395,-60.2422614639156,-60.1624718065184,
-60.0826323710433,-60.002695033114,-59.9227035170359,-59.8426133993631,
-59.816225196907,-59.7372333015685,-59.6583415168936,-59.5795392608493,
-59.5008392600278,-59.4221998141494,-59.3436235319641,-59.3177566535994,
-59.2391699304359,-59.1605337631728,-59.0818377698565,-59.0030237383736,
-58.9241423101499,-58.845139216934,-58.8192881102918,-58.7402155885422,
-58.6612160338072,-58.5822777659832,-58.5033891515018,-58.4245385949456,
-58.3457100906799,-58.2668937168111,-58.1880789656273,-58.1092553316499,
-58.0303852841016,-57.9514916050257,-57.8725310801887,-57.8223510236767,
-57.7482455855748,-57.6741970877203,-57.6001903497133,-57.5262010855606,
-57.4522237239486,-57.3782214379155,-57.3238824803692,-57.2328833806335,
-57.1413801629565,-57.0494366240264,-56.9574020468475,-56.8654929567266,
-56.8254139370616,-56.7497042659439,-56.674043263918,-56.5984164235803,
-56.5227987272979,-56.4471872272111,-56.3715473025833,-56.326945393754,
-56.2446666219008,-56.1623640590383,-56.0788922568903,-55.9965373019925,
-55.9125070762195,-55.8284768504465,-55.7460978398443,-55.6637336505946,
-55.5803023147307,-55.4979803414377,-55.4139943242883,-55.3300083071389,
-55.2543681979176,-55.1787520950117,-55.103145527958,-55.0275108652487,
-54.9518613066711,-54.8761510168944,-54.8315397638314,-54.7395871468826,
-54.6475551712311,-54.5557033213318,-54.4741437745622),.UNSPECIFIED.);
#3143=B_SPLINE_CURVE_WITH_KNOTS('',3,(#157155,#157156,#157157,#157158,#157159,
#157160,#157161,#157162,#157163,#157164,#157165,#157166,#157167,#157168,
#157169,#157170,#157171,#157172,#157173,#157174,#157175,#157176,#157177,
#157178,#157179,#157180,#157181,#157182,#157183,#157184,#157185,#157186,
#157187,#157188,#157189,#157190,#157191,#157192,#157193,#157194,#157195,
#157196,#157197,#157198,#157199,#157200,#157201,#157202,#157203,#157204,
#157205,#157206,#157207,#157208,#157209,#157210,#157211,#157212,#157213,
#157214,#157215,#157216,#157217,#157218,#157219,#157220,#157221,#157222,
#157223,#157224,#157225,#157226,#157227,#157228,#157229,#157230,#157231,
#157232,#157233,#157234,#157235,#157236,#157237,#157238,#157239,#157240,
#157241,#157242,#157243,#157244,#157245,#157246,#157247,#157248,#157249,
#157250,#157251,#157252,#157253,#157254,#157255,#157256,#157257,#157258,
#157259,#157260,#157261,#157262,#157263,#157264,#157265,#157266,#157267,
#157268,#157269,#157270,#157271,#157272,#157273,#157274,#157275,#157276,
#157277,#157278,#157279,#157280,#157281,#157282,#157283,#157284,#157285,
#157286,#157287,#157288,#157289,#157290,#157291,#157292,#157293,#157294,
#157295,#157296,#157297,#157298,#157299,#157300,#157301,#157302,#157303,
#157304,#157305,#157306,#157307,#157308,#157309,#157310,#157311,#157312,
#157313,#157314,#157315,#157316,#157317,#157318,#157319,#157320,#157321,
#157322,#157323,#157324,#157325,#157326,#157327,#157328,#157329,#157330,
#157331,#157332,#157333,#157334,#157335,#157336,#157337,#157338,#157339,
#157340,#157341,#157342,#157343,#157344,#157345,#157346,#157347,#157348,
#157349,#157350,#157351,#157352,#157353,#157354,#157355,#157356,#157357,
#157358,#157359,#157360,#157361,#157362,#157363,#157364,#157365,#157366,
#157367,#157368,#157369,#157370,#157371,#157372,#157373,#157374,#157375,
#157376,#157377,#157378,#157379,#157380,#157381,#157382,#157383,#157384,
#157385,#157386,#157387,#157388,#157389,#157390,#157391,#157392),
 .UNSPECIFIED.,.F.,.F.,(4,3,3,3,3,3,3,3,3,3,3,3,3,3,3,3,3,3,3,3,3,3,3,3,
3,3,3,3,3,3,3,3,3,3,3,3,3,3,3,3,3,3,3,3,3,3,3,3,3,3,3,3,3,3,3,3,3,3,3,3,
3,3,3,3,3,3,3,3,3,3,3,3,3,3,3,3,3,3,3,4),(51.9314713010136,52.010349088432,
52.0925610781474,52.1712486835971,52.2498775775425,52.3284465749947,52.3391970472936,
52.4177837704572,52.4964199377203,52.575115931037,52.6539299625199,52.7328113907437,
52.8118144839596,52.8376655906012,52.9167381123508,52.9957376670859,53.0746759349099,
53.1535645493913,53.2324151059476,53.3112436102133,53.3900599840822,53.4688747352658,
53.5476983692433,53.6265684167916,53.7054620958675,53.7844226207045,53.8346026772163,
53.9087081153182,53.9827566131727,54.0567633511797,54.1307526153323,54.2047299769443,
54.2787322629774,54.3330712205238,54.4240703202597,54.5155735379368,54.6075170768671,
54.6995516540461,54.7914607441672,54.8315397638314,54.9072494349489,54.9829104369747,
55.0585372773123,55.1341549735946,55.2097664736812,55.2854063983089,55.3300083071389,
55.4122870789922,55.494589641855,55.5780614440028,55.6604163989009,55.7444466246737,
55.8284768504465,55.9108558610486,55.9932200502983,56.0766513861622,56.1589733594553,
56.2429593766047,56.3269453937541,56.4025855029753,56.4782016058812,56.5538081729345,
56.6294428356438,56.7050923942214,56.780802683998,56.8254139370616,56.9173145067649,
57.009347476479,57.1012270463014,57.1928544423309,57.2838755638127,57.3238824803692,
57.3978843950572,57.4718653234005,57.5458403453128,57.6198528186127,57.6938840885939,
57.7679888407988,57.8223510236767,57.8577774557529),.UNSPECIFIED.);
#3144=B_SPLINE_CURVE_WITH_KNOTS('',3,(#157393,#157394,#157395,#157396,#157397,
#157398,#157399,#157400,#157401,#157402,#157403,#157404,#157405,#157406,
#157407,#157408),.UNSPECIFIED.,.F.,.F.,(4,3,3,3,3,4),(57.8577774558344,
57.9362807382,58.014711565424,58.0930995598951,58.17145295758,58.2138923057233),
 .UNSPECIFIED.);
#3145=B_SPLINE_CURVE_WITH_KNOTS('',3,(#157410,#157411,#157412,#157413,#157414,
#157415,#157416,#157417,#157418,#157419,#157420,#157421,#157422,#157423,
#157424,#157425),.UNSPECIFIED.,.F.,.F.,(4,3,3,3,3,4),(-54.4741437745622,
-54.3830887300197,-54.3330712205238,-54.2623508425394,-54.1904443771559,
-54.1185379117723),.UNSPECIFIED.);
#3146=B_SPLINE_CURVE_WITH_KNOTS('',3,(#157426,#157427,#157428,#157429,#157430,
#157431,#157432,#157433,#157434,#157435,#157436,#157437,#157438,#157439,
#157440,#157441,#157442,#157443,#157444,#157445,#157446,#157447,#157448,
#157449,#157450,#157451,#157452,#157453,#157454,#157455,#157456,#157457,
#157458,#157459,#157460,#157461,#157462,#157463,#157464,#157465,#157466,
#157467,#157468,#157469,#157470,#157471,#157472,#157473,#157474,#157475,
#157476,#157477,#157478,#157479,#157480,#157481,#157482,#157483,#157484,
#157485,#157486,#157487,#157488,#157489,#157490,#157491,#157492,#157493,
#157494,#157495,#157496,#157497,#157498,#157499,#157500,#157501,#157502,
#157503,#157504,#157505,#157506,#157507,#157508,#157509,#157510,#157511,
#157512,#157513,#157514,#157515,#157516,#157517,#157518,#157519,#157520,
#157521,#157522,#157523,#157524,#157525,#157526,#157527,#157528,#157529,
#157530,#157531,#157532,#157533,#157534,#157535,#157536,#157537,#157538,
#157539,#157540,#157541,#157542,#157543,#157544,#157545,#157546,#157547,
#157548,#157549,#157550,#157551,#157552,#157553,#157554,#157555,#157556,
#157557,#157558,#157559,#157560,#157561,#157562,#157563,#157564,#157565,
#157566,#157567,#157568,#157569,#157570,#157571,#157572,#157573,#157574,
#157575,#157576,#157577,#157578,#157579,#157580,#157581,#157582,#157583,
#157584,#157585,#157586,#157587,#157588,#157589,#157590,#157591,#157592,
#157593,#157594,#157595,#157596,#157597,#157598,#157599,#157600,#157601,
#157602,#157603,#157604,#157605,#157606,#157607,#157608,#157609,#157610,
#157611,#157612,#157613,#157614,#157615,#157616,#157617,#157618,#157619,
#157620,#157621,#157622,#157623,#157624,#157625,#157626,#157627,#157628,
#157629,#157630,#157631,#157632,#157633,#157634,#157635,#157636,#157637,
#157638,#157639,#157640,#157641,#157642,#157643,#157644,#157645,#157646,
#157647,#157648,#157649,#157650,#157651,#157652,#157653,#157654,#157655,
#157656,#157657,#157658,#157659,#157660,#157661,#157662,#157663),
 .UNSPECIFIED.,.F.,.F.,(4,3,3,3,3,3,3,3,3,3,3,3,3,3,3,3,3,3,3,3,3,3,3,3,
3,3,3,3,3,3,3,3,3,3,3,3,3,3,3,3,3,3,3,3,3,3,3,3,3,3,3,3,3,3,3,3,3,3,3,3,
3,3,3,3,3,3,3,3,3,3,3,3,3,3,3,3,3,3,3,4),(-54.1185379116474,-54.0396932861478,
-53.9607819726184,-53.881740071316,-53.8346026772163,-53.755641261269,-53.6767338381998,
-53.5978687992631,-53.5190345685371,-53.4402195945583,-53.3613983308981,
-53.2825716917857,-53.2037291674094,-53.1248602388266,-53.0459181874951,
-52.9669374220063,-52.8878664109882,-52.8376655906011,-52.7586736952626,
-52.6797819105877,-52.6009796545436,-52.5222796537221,-52.4436402078436,
-52.3650639256585,-52.3391970472936,-52.2606103241301,-52.1819741568671,
-52.1032781635508,-52.024464132068,-51.9455827038444,-51.8665796106285,
-51.840728503986,-51.7616559822364,-51.6826564275014,-51.6037181596773,
-51.524829545196,-51.4459789886397,-51.367150484374,-51.2883341105051,-51.2095193593214,
-51.1306957253439,-51.0518256777956,-50.9729319987198,-50.8939714738828,
-50.8437914173709,-50.7696859792689,-50.6956374814144,-50.6216307434073,
-50.5476414792546,-50.4736641176425,-50.3996618316093,-50.3453228740633,
-50.2543237743278,-50.162820556651,-50.0708770177211,-49.9788424405425,
-49.8869333504217,-49.8468543307558,-49.7711446596381,-49.6954836576122,
-49.6198568172745,-49.544239120992,-49.4686276209053,-49.3929876962775,
-49.3483857874482,-49.266107015595,-49.1838044527324,-49.1003326505845,
-49.0179776956867,-48.9339474699137,-48.8499172441407,-48.7675382335386,
-48.685174044289,-48.601742708425,-48.519420735132,-48.4354347179826,-48.3514487008331,
-48.2758079681556,-48.2001936861576,-48.1916415759627),.UNSPECIFIED.);
#3147=B_SPLINE_CURVE_WITH_KNOTS('',3,(#157669,#157670,#157671,#157672,#157673,
#157674,#157675,#157676,#157677,#157678,#157679,#157680,#157681,#157682,
#157683,#157684,#157685,#157686,#157687,#157688,#157689,#157690,#157691,
#157692,#157693,#157694,#157695,#157696,#157697,#157698,#157699,#157700,
#157701,#157702,#157703,#157704,#157705,#157706,#157707,#157708,#157709,
#157710,#157711,#157712,#157713,#157714,#157715,#157716,#157717,#157718,
#157719,#157720,#157721,#157722,#157723,#157724,#157725,#157726,#157727,
#157728,#157729,#157730,#157731,#157732,#157733,#157734,#157735,#157736,
#157737,#157738,#157739,#157740,#157741,#157742,#157743,#157744,#157745,
#157746,#157747,#157748,#157749,#157750,#157751,#157752,#157753,#157754,
#157755,#157756,#157757,#157758,#157759,#157760,#157761,#157762,#157763,
#157764,#157765,#157766,#157767,#157768,#157769,#157770,#157771,#157772,
#157773,#157774,#157775,#157776,#157777,#157778,#157779,#157780,#157781,
#157782,#157783,#157784,#157785,#157786,#157787,#157788,#157789,#157790,
#157791,#157792,#157793,#157794,#157795,#157796,#157797,#157798,#157799,
#157800,#157801,#157802,#157803,#157804,#157805,#157806,#157807,#157808,
#157809,#157810,#157811,#157812,#157813,#157814,#157815,#157816,#157817,
#157818,#157819,#157820,#157821,#157822,#157823,#157824,#157825,#157826,
#157827,#157828,#157829,#157830,#157831,#157832,#157833,#157834,#157835,
#157836,#157837,#157838,#157839,#157840,#157841,#157842,#157843,#157844,
#157845,#157846,#157847,#157848,#157849,#157850,#157851,#157852,#157853,
#157854,#157855,#157856,#157857,#157858,#157859,#157860,#157861,#157862,
#157863,#157864,#157865,#157866,#157867,#157868,#157869,#157870,#157871,
#157872,#157873,#157874,#157875,#157876,#157877,#157878,#157879,#157880,
#157881,#157882,#157883,#157884,#157885,#157886,#157887,#157888,#157889,
#157890,#157891,#157892,#157893,#157894,#157895,#157896,#157897,#157898,
#157899,#157900,#157901,#157902,#157903),.UNSPECIFIED.,.F.,.F.,(4,3,3,3,
3,3,3,3,3,3,3,3,3,3,3,3,3,3,3,3,3,3,3,3,3,3,3,3,3,3,3,3,3,3,3,3,3,3,3,3,
3,3,3,3,3,3,3,3,3,3,3,3,3,3,3,3,3,3,3,3,3,3,3,3,3,3,3,3,3,3,3,3,3,3,3,3,
3,3,4),(45.6468212085296,45.7256771159923,45.8046642745895,45.8591059842953,
45.938178506045,46.0171780607802,46.0961163286042,46.1750049430857,46.2538554996418,
46.3326840039076,46.4115003777766,46.4903151289606,46.5691387629384,46.6480088104868,
46.7269024895627,46.8058630143996,46.8560430709105,46.9301485090125,47.004197006867,
47.0782037448741,47.1521930090267,47.2261703706386,47.3001726566718,47.354511614218,
47.4455107139543,47.5370139316309,47.6289574705612,47.7209920477399,47.8129011378603,
47.8529801575256,47.9286898286431,48.0043508306691,48.0799776710068,48.1555953672892,
48.2312068673758,48.3068467920036,48.3514487008331,48.4337274726864,48.5160300355491,
48.599501837697,48.681856792595,48.7658870183678,48.8499172441407,48.9322962547427,
49.0146604439924,49.0980917798564,49.1804137531494,49.2643997702988,49.3483857874483,
49.4240258966695,49.4996419995754,49.5752485666291,49.6508832293383,49.726532787916,
49.8022430776929,49.8468543307558,49.9387549004592,50.030787870172,50.1226674399944,
50.2142948360256,50.3053159575074,50.3453228740634,50.4193247887513,50.4933057170947,
50.5672807390074,50.6412932123071,50.7153244822882,50.789429234493,50.8437914173709,
50.9222508834037,51.0037935415499,51.0821383235146,51.1604532036749,51.2387496665986,
51.3170391836195,51.3953501369081,51.4736731259674,51.552038685281,51.5745921485733),
 .UNSPECIFIED.);
#3148=B_SPLINE_CURVE_WITH_KNOTS('',3,(#157904,#157905,#157906,#157907,#157908,
#157909,#157910,#157911,#157912,#157913,#157914,#157915,#157916,#157917,
#157918,#157919),.UNSPECIFIED.,.F.,.F.,(4,3,3,3,3,4),(51.5745921486873,
51.6725058707897,51.7717369862272,51.8407285039861,51.9197400789197,51.9314713010136),
 .UNSPECIFIED.);
#3149=B_SPLINE_CURVE_WITH_KNOTS('',3,(#157921,#157922,#157923,#157924,#157925,
#157926,#157927,#157928,#157929,#157930,#157931,#157932,#157933,#157934,
#157935,#157936,#157937,#157938,#157939),.UNSPECIFIED.,.F.,.F.,(4,3,3,3,
3,3,4),(-48.1916415759627,-48.1160351770241,-48.0403994804095,-47.964747421664,
-47.8890357469598,-47.8529801575256,-47.8353526044678),.UNSPECIFIED.);
#3150=B_SPLINE_CURVE_WITH_KNOTS('',3,(#157940,#157941,#157942,#157943,#157944,
#157945,#157946,#157947,#157948,#157949,#157950,#157951,#157952,#157953,
#157954,#157955,#157956,#157957,#157958,#157959,#157960,#157961,#157962,
#157963,#157964,#157965,#157966,#157967,#157968,#157969,#157970,#157971,
#157972,#157973,#157974,#157975,#157976,#157977,#157978,#157979,#157980,
#157981,#157982,#157983,#157984,#157985,#157986,#157987,#157988,#157989,
#157990,#157991,#157992,#157993,#157994,#157995,#157996,#157997,#157998,
#157999,#158000,#158001,#158002,#158003,#158004,#158005,#158006,#158007,
#158008,#158009,#158010,#158011,#158012,#158013,#158014,#158015,#158016,
#158017,#158018,#158019,#158020,#158021,#158022,#158023,#158024,#158025,
#158026,#158027,#158028,#158029,#158030,#158031,#158032,#158033,#158034,
#158035,#158036,#158037,#158038,#158039,#158040,#158041,#158042,#158043,
#158044,#158045,#158046,#158047,#158048,#158049,#158050,#158051,#158052,
#158053,#158054,#158055,#158056,#158057,#158058,#158059,#158060,#158061,
#158062,#158063,#158064,#158065,#158066,#158067,#158068,#158069,#158070,
#158071,#158072,#158073,#158074,#158075,#158076,#158077,#158078,#158079,
#158080,#158081,#158082,#158083,#158084,#158085,#158086,#158087,#158088,
#158089,#158090,#158091,#158092,#158093,#158094,#158095,#158096,#158097,
#158098,#158099,#158100,#158101,#158102,#158103,#158104,#158105,#158106,
#158107,#158108,#158109,#158110,#158111,#158112,#158113,#158114,#158115,
#158116,#158117,#158118,#158119,#158120,#158121,#158122,#158123,#158124,
#158125,#158126,#158127,#158128,#158129,#158130,#158131,#158132,#158133,
#158134,#158135,#158136,#158137,#158138,#158139,#158140,#158141,#158142,
#158143,#158144,#158145,#158146,#158147,#158148,#158149,#158150,#158151,
#158152,#158153,#158154,#158155,#158156,#158157,#158158,#158159,#158160,
#158161,#158162,#158163,#158164,#158165,#158166,#158167,#158168,#158169,
#158170,#158171,#158172,#158173,#158174,#158175,#158176,#158177),
 .UNSPECIFIED.,.F.,.F.,(4,3,3,3,3,3,3,3,3,3,3,3,3,3,3,3,3,3,3,3,3,3,3,3,
3,3,3,3,3,3,3,3,3,3,3,3,3,3,3,3,3,3,3,3,3,3,3,3,3,3,3,3,3,3,3,3,3,3,3,3,
3,3,3,3,3,3,3,3,3,3,3,3,3,3,3,3,3,3,3,4),(-47.8353526043918,-47.7438818493918,
-47.6523361208125,-47.5609865054093,-47.4698969508807,-47.3793718635444,
-47.354511614218,-47.2805096995299,-47.2065287711865,-47.132553749274,-47.0585412759741,
-46.9845100059928,-46.9104052537878,-46.8560430709104,-46.7770816549632,
-46.698174231894,-46.6193091929574,-46.5404749622316,-46.4616599882529,
-46.3828387245927,-46.3040120854804,-46.225169561104,-46.1463006325212,
-46.0673585811898,-45.9883778157009,-45.9093068046828,-45.8591059842953,
-45.7801140889568,-45.7012223042821,-45.622420048238,-45.5437200474165,
-45.4650806015379,-45.3865043193528,-45.3606374409878,-45.2820507178242,
-45.2034145505611,-45.1247185572446,-45.0459045257617,-44.967023097538,
-44.888020004322,-44.8621688976802,-44.7830963759306,-44.7040968211956,
-44.6251585533716,-44.5462699388903,-44.467419382334,-44.3885908780683,
-44.3097745041995,-44.2309597530157,-44.1521361190383,-44.07326607149,-43.9943723924142,
-43.9154118675772,-43.8652318110651,-43.7911263729631,-43.7170778751086,
-43.6430711371015,-43.5690818729488,-43.4951045113367,-43.4211022253034,
-43.3667632677575,-43.2757641680218,-43.184260950345,-43.0923174114152,
-43.0002828342366,-42.9083737441158,-42.86829472445,-42.7925850533323,-42.7169240513064,
-42.6412972109688,-42.5656795146863,-42.4900680145996,-42.4144280899718,
-42.3698261811424,-42.2875502010023,-42.2052500532836,-42.1229103589057,
-42.0405596721461,-41.9581865681693,-41.9084162677792),.UNSPECIFIED.);
#3151=B_SPLINE_CURVE_WITH_KNOTS('',3,(#158183,#158184,#158185,#158186,#158187,
#158188,#158189,#158190,#158191,#158192,#158193,#158194,#158195,#158196,
#158197,#158198,#158199,#158200,#158201,#158202,#158203,#158204,#158205,
#158206,#158207,#158208,#158209,#158210,#158211,#158212,#158213,#158214,
#158215,#158216,#158217,#158218,#158219,#158220,#158221,#158222,#158223,
#158224,#158225,#158226,#158227,#158228,#158229,#158230,#158231,#158232,
#158233,#158234,#158235,#158236,#158237,#158238,#158239,#158240,#158241,
#158242,#158243,#158244,#158245,#158246,#158247,#158248,#158249,#158250,
#158251,#158252,#158253,#158254,#158255,#158256,#158257,#158258,#158259,
#158260,#158261,#158262,#158263,#158264,#158265,#158266,#158267,#158268,
#158269,#158270,#158271,#158272,#158273,#158274,#158275,#158276,#158277,
#158278,#158279,#158280,#158281,#158282,#158283,#158284,#158285,#158286,
#158287,#158288,#158289,#158290,#158291,#158292,#158293,#158294,#158295,
#158296,#158297,#158298,#158299,#158300,#158301,#158302,#158303,#158304,
#158305,#158306,#158307,#158308,#158309,#158310,#158311,#158312,#158313,
#158314,#158315,#158316,#158317,#158318,#158319,#158320,#158321,#158322,
#158323,#158324,#158325,#158326,#158327,#158328,#158329,#158330,#158331,
#158332,#158333,#158334,#158335,#158336,#158337,#158338,#158339,#158340,
#158341,#158342,#158343,#158344,#158345,#158346,#158347,#158348,#158349,
#158350,#158351,#158352,#158353,#158354,#158355,#158356,#158357,#158358,
#158359,#158360,#158361,#158362,#158363,#158364,#158365,#158366,#158367,
#158368,#158369,#158370,#158371,#158372,#158373,#158374,#158375,#158376,
#158377,#158378,#158379,#158380,#158381,#158382,#158383,#158384,#158385,
#158386,#158387,#158388,#158389,#158390,#158391,#158392,#158393,#158394,
#158395,#158396,#158397,#158398,#158399,#158400,#158401,#158402,#158403,
#158404,#158405,#158406,#158407,#158408,#158409,#158410,#158411,#158412,
#158413,#158414,#158415,#158416,#158417),.UNSPECIFIED.,.F.,.F.,(4,3,3,3,
3,3,3,3,3,3,3,3,3,3,3,3,3,3,3,3,3,3,3,3,3,3,3,3,3,3,3,3,3,3,3,3,3,3,3,3,
3,3,3,3,3,3,3,3,3,3,3,3,3,3,3,3,3,3,3,3,3,3,3,3,3,3,3,3,3,3,3,3,3,3,3,3,
3,3,4),(39.3650750661798,39.4428973253601,39.520713993561,39.5985373278778,
39.6764073153725,39.7543022948959,39.8322681440181,39.8774834646046,39.9515889027065,
40.025637400561,40.0996441385683,40.173633402721,40.247610764333,40.3216130503661,
40.3759520079122,40.4669511076482,40.5584543253243,40.6503978642546,40.7424324414336,
40.8343415315547,40.8744205512198,40.9501302223373,41.025791224363,41.1014180647006,
41.1770357609829,41.2526472610696,41.3282871856971,41.3728890945273,41.4551678663805,
41.5374704292436,41.6209422313914,41.7032971862895,41.7873274120622,41.8713576378349,
41.9537366484368,42.0361008376866,42.1195321735505,42.2018541468433,42.2858401639928,
42.3698261811424,42.4454662903638,42.5210823932697,42.5966889603235,42.672323623033,
42.7479731816105,42.8236834713872,42.86829472445,42.9601952941527,43.0522282638671,
43.1441078336892,43.2357352297184,43.3267563511995,43.3667632677576,43.4407651824456,
43.5147461107889,43.5887211327014,43.6627336060013,43.7367648759821,43.810869628187,
43.8652318110651,43.9441932270122,44.0231006500812,44.1019656890176,44.1807999197432,
44.2596148937224,44.3384361573826,44.4172627964949,44.4961053208715,44.5749742494545,
44.653916300786,44.732897066275,44.8119680772932,44.8621688976802,44.9426880221432,
45.0230879351252,45.1033329860329,45.183484530017,45.2635184145895,45.2914068413062),
 .UNSPECIFIED.);
#3152=B_SPLINE_CURVE_WITH_KNOTS('',3,(#158418,#158419,#158420,#158421,#158422,
#158423,#158424,#158425,#158426,#158427,#158428,#158429,#158430,#158431,
#158432,#158433),.UNSPECIFIED.,.F.,.F.,(4,3,3,3,3,4),(45.2914068413937,
45.3606374409878,45.4392344513366,45.5178699470115,45.5965949508927,45.6468212085296),
 .UNSPECIFIED.);
#3153=B_SPLINE_CURVE_WITH_KNOTS('',3,(#158435,#158436,#158437,#158438,#158439,
#158440,#158441,#158442,#158443,#158444,#158445,#158446,#158447,#158448,
#158449,#158450),.UNSPECIFIED.,.F.,.F.,(4,3,3,3,3,4),(-41.9084162677792,
-41.8713576378349,-41.7898517304649,-41.7083640391987,-41.6268883973049,
-41.5521672972882),.UNSPECIFIED.);
#3154=B_SPLINE_CURVE_WITH_KNOTS('',3,(#158451,#158452,#158453,#158454,#158455,
#158456,#158457,#158458,#158459,#158460,#158461,#158462,#158463,#158464,
#158465,#158466,#158467,#158468,#158469,#158470,#158471,#158472,#158473,
#158474,#158475,#158476,#158477,#158478,#158479,#158480,#158481,#158482,
#158483,#158484,#158485,#158486,#158487,#158488,#158489,#158490,#158491,
#158492,#158493,#158494,#158495,#158496,#158497,#158498,#158499,#158500,
#158501,#158502,#158503,#158504,#158505,#158506,#158507,#158508,#158509,
#158510,#158511,#158512,#158513,#158514,#158515,#158516,#158517,#158518,
#158519,#158520,#158521,#158522,#158523,#158524,#158525,#158526,#158527,
#158528,#158529,#158530,#158531,#158532,#158533,#158534,#158535,#158536,
#158537,#158538,#158539,#158540,#158541,#158542,#158543,#158544,#158545,
#158546,#158547,#158548,#158549,#158550,#158551,#158552,#158553,#158554,
#158555,#158556,#158557,#158558,#158559,#158560,#158561,#158562,#158563,
#158564,#158565,#158566,#158567,#158568,#158569,#158570,#158571,#158572,
#158573,#158574,#158575,#158576,#158577,#158578,#158579,#158580,#158581,
#158582,#158583,#158584,#158585,#158586,#158587,#158588,#158589,#158590,
#158591,#158592,#158593,#158594,#158595,#158596,#158597,#158598,#158599,
#158600,#158601,#158602,#158603,#158604,#158605,#158606,#158607,#158608,
#158609,#158610,#158611,#158612,#158613,#158614,#158615,#158616,#158617,
#158618,#158619,#158620,#158621,#158622,#158623,#158624,#158625,#158626,
#158627,#158628,#158629,#158630,#158631,#158632,#158633,#158634,#158635,
#158636,#158637,#158638,#158639,#158640,#158641,#158642,#158643,#158644,
#158645,#158646,#158647,#158648,#158649,#158650,#158651,#158652,#158653,
#158654,#158655,#158656,#158657,#158658,#158659,#158660,#158661,#158662,
#158663,#158664,#158665,#158666,#158667,#158668,#158669,#158670,#158671,
#158672,#158673,#158674,#158675,#158676,#158677,#158678,#158679,#158680,
#158681,#158682,#158683,#158684,#158685,#158686,#158687,#158688),
 .UNSPECIFIED.,.F.,.F.,(4,3,3,3,3,3,3,3,3,3,3,3,3,3,3,3,3,3,3,3,3,3,3,3,
3,3,3,3,3,3,3,3,3,3,3,3,3,3,3,3,3,3,3,3,3,3,3,3,3,3,3,3,3,3,3,3,3,3,3,3,
3,3,3,3,3,3,3,3,3,3,3,3,3,3,3,3,3,3,3,4),(-41.5521672972882,-41.4625281959078,
-41.3728890945273,-41.2972489853062,-41.2216328824004,-41.1460263153471,
-41.0703916526379,-40.9947420940603,-40.9190318042837,-40.8744205512198,
-40.7825199815166,-40.6904870118016,-40.5986074419793,-40.5069800459494,
-40.4159589244676,-40.3759520079122,-40.3019500932241,-40.2279691648807,
-40.1539941429681,-40.0799816696681,-40.0059503996867,-39.9318456474817,
-39.8774834646046,-39.7985220486573,-39.7196146255882,-39.6407495866517,
-39.5619153559262,-39.4831003819476,-39.4042791182875,-39.3254524791752,
-39.2466099547988,-39.1677410262161,-39.0887989748847,-39.0098182093957,
-38.9307471983775,-38.8805463779895,-38.801554482651,-38.7226626979764,
-38.6438604419319,-38.5651604411105,-38.4865209952314,-38.4079447130463,
-38.382077834682,-38.3034911115186,-38.2248549442554,-38.1461589509396,
-38.0673449194569,-37.9884634912329,-37.9094603980172,-37.8836092913744,
-37.8045367696248,-37.7255372148899,-37.6465989470658,-37.5677103325842,
-37.4888597760277,-37.410031271762,-37.3312148978932,-37.2524001467095,
-37.1735765127321,-37.0947064651839,-37.0158127861082,-36.9368522612713,
-36.8866722047593,-36.8125667666573,-36.7385182688028,-36.6645115307967,
-36.590522266644,-36.5165449050318,-36.4425426189986,-36.3882036614517,
-36.2972045617156,-36.2057013440403,-36.1137578051107,-36.0217232279321,
-35.9298141378113,-35.8897351181442,-35.814026435445,-35.7383644598627,
-35.6627367767685,-35.6249640953535),.UNSPECIFIED.);
#3155=B_SPLINE_CURVE_WITH_KNOTS('',3,(#158694,#158695,#158696,#158697,#158698,
#158699,#158700,#158701,#158702,#158703,#158704,#158705,#158706,#158707,
#158708,#158709,#158710,#158711,#158712,#158713,#158714,#158715,#158716,
#158717,#158718,#158719,#158720,#158721,#158722,#158723,#158724,#158725,
#158726,#158727,#158728,#158729,#158730,#158731,#158732,#158733,#158734,
#158735,#158736,#158737,#158738,#158739,#158740,#158741,#158742,#158743,
#158744,#158745,#158746,#158747,#158748,#158749,#158750,#158751,#158752,
#158753,#158754,#158755,#158756,#158757,#158758,#158759,#158760,#158761,
#158762,#158763,#158764,#158765,#158766,#158767,#158768,#158769,#158770,
#158771,#158772,#158773,#158774,#158775,#158776,#158777,#158778,#158779,
#158780,#158781,#158782,#158783,#158784,#158785,#158786,#158787,#158788,
#158789,#158790,#158791,#158792,#158793,#158794,#158795,#158796,#158797,
#158798,#158799,#158800,#158801,#158802,#158803,#158804,#158805,#158806,
#158807,#158808,#158809,#158810,#158811,#158812,#158813,#158814,#158815,
#158816,#158817,#158818,#158819,#158820,#158821,#158822,#158823,#158824,
#158825,#158826,#158827,#158828,#158829,#158830,#158831,#158832,#158833,
#158834,#158835,#158836,#158837,#158838,#158839,#158840,#158841,#158842,
#158843,#158844,#158845,#158846,#158847,#158848,#158849,#158850,#158851,
#158852,#158853,#158854,#158855,#158856,#158857,#158858,#158859,#158860,
#158861,#158862,#158863,#158864,#158865,#158866,#158867,#158868,#158869,
#158870,#158871,#158872,#158873,#158874,#158875,#158876,#158877,#158878,
#158879,#158880,#158881,#158882,#158883,#158884,#158885,#158886,#158887,
#158888,#158889,#158890,#158891,#158892,#158893,#158894,#158895,#158896,
#158897,#158898,#158899,#158900,#158901,#158902,#158903,#158904,#158905,
#158906,#158907,#158908,#158909,#158910,#158911,#158912,#158913,#158914,
#158915,#158916,#158917,#158918,#158919,#158920,#158921,#158922,#158923,
#158924,#158925,#158926,#158927,#158928),.UNSPECIFIED.,.F.,.F.,(4,3,3,3,
3,3,3,3,3,3,3,3,3,3,3,3,3,3,3,3,3,3,3,3,3,3,3,3,3,3,3,3,3,3,3,3,3,3,3,3,
3,3,3,3,3,3,3,3,3,3,3,3,3,3,3,3,3,3,3,3,3,3,3,3,3,3,3,3,3,3,3,3,3,3,3,3,
3,3,4),(33.0816676322956,33.1556600429916,33.2296420595945,33.3036185021859,
33.3776189751015,33.3973924016064,33.4883915013423,33.5798947190199,33.6718382579498,
33.7638728351289,33.8557819252498,33.895860944914,33.9715706160315,34.0472316180573,
34.1228584583949,34.1984761546772,34.2740876547638,34.3497275793915,34.3943294882215,
34.4766082600749,34.5589108229377,34.6423826250856,34.7247375799837,34.8087678057564,
34.8927980315291,34.975177042131,35.0575412313805,35.1409725672445,35.2232945405373,
35.3072805576869,35.3912665748366,35.466906684058,35.5425227869641,35.6181293540178,
35.6937640167273,35.769413575305,35.8451238650819,35.8897351181442,35.981635687847,
36.0736686575608,36.1655482273828,36.2571756234118,36.3481967448931,36.3882036614517,
36.4622055761398,36.5361865044833,36.6101615263958,36.6841739996958,36.7582052696771,
36.8323100218821,36.8866722047593,36.9656336207065,37.0445410437757,37.1234060827122,
37.2022403134381,37.2810552874168,37.359876551077,37.4387031901894,37.5175457145658,
37.5964146431485,37.6753566944799,37.7543374599686,37.8334084709867,37.8836092913744,
37.962601186713,38.0414929713878,38.120295227432,38.1989952282536,38.2776346741321,
38.3562109563174,38.382077834682,38.4606645578453,38.5393007251084,38.6179967184244,
38.696810749907,38.7756921781308,38.8546952713465,38.8805463779895,39.0082215342141),
 .UNSPECIFIED.);
#3156=B_SPLINE_CURVE_WITH_KNOTS('',3,(#158929,#158930,#158931,#158932,#158933,
#158934,#158935,#158936,#158937,#158938,#158939,#158940,#158941,#158942,
#158943,#158944),.UNSPECIFIED.,.F.,.F.,(4,3,3,3,3,4),(39.0082215342936,
39.0862558873874,39.1642044673432,39.2421030021683,39.3199578461465,39.3650750661798),
 .UNSPECIFIED.);
#3157=B_SPLINE_CURVE_WITH_KNOTS('',3,(#158946,#158947,#158948,#158949,#158950,
#158951,#158952,#158953,#158954,#158955,#158956,#158957,#158958,#158959,
#158960,#158961),.UNSPECIFIED.,.F.,.F.,(4,3,3,3,3,4),(-35.6249640953535,
-35.5493511139821,-35.4703088444094,-35.3912665748366,-35.3016062240681,
-35.2689819901086),.UNSPECIFIED.);
#3158=B_SPLINE_CURVE_WITH_KNOTS('',3,(#158962,#158963,#158964,#158965,#158966,
#158967,#158968,#158969,#158970,#158971,#158972,#158973,#158974,#158975,
#158976,#158977,#158978,#158979,#158980,#158981,#158982,#158983,#158984,
#158985,#158986,#158987,#158988,#158989,#158990,#158991,#158992,#158993,
#158994,#158995,#158996,#158997,#158998,#158999,#159000,#159001,#159002,
#159003,#159004,#159005,#159006,#159007,#159008,#159009,#159010,#159011,
#159012,#159013,#159014,#159015,#159016,#159017,#159018,#159019,#159020,
#159021,#159022,#159023,#159024,#159025,#159026,#159027,#159028,#159029,
#159030,#159031,#159032,#159033,#159034,#159035,#159036,#159037,#159038,
#159039,#159040,#159041,#159042,#159043,#159044,#159045,#159046,#159047,
#159048,#159049,#159050,#159051,#159052,#159053,#159054,#159055,#159056,
#159057,#159058,#159059,#159060,#159061,#159062,#159063,#159064,#159065,
#159066,#159067,#159068,#159069,#159070,#159071,#159072,#159073,#159074,
#159075,#159076,#159077,#159078,#159079,#159080,#159081,#159082,#159083,
#159084,#159085,#159086,#159087,#159088,#159089,#159090,#159091,#159092,
#159093,#159094,#159095,#159096,#159097,#159098,#159099,#159100,#159101,
#159102,#159103,#159104,#159105,#159106,#159107,#159108,#159109,#159110,
#159111,#159112,#159113,#159114,#159115,#159116,#159117,#159118,#159119,
#159120,#159121,#159122,#159123,#159124,#159125,#159126,#159127,#159128,
#159129,#159130,#159131,#159132,#159133,#159134,#159135,#159136,#159137,
#159138,#159139,#159140,#159141,#159142,#159143,#159144,#159145,#159146,
#159147,#159148,#159149,#159150,#159151,#159152,#159153,#159154,#159155,
#159156,#159157,#159158,#159159,#159160,#159161,#159162,#159163,#159164,
#159165,#159166,#159167,#159168,#159169,#159170,#159171,#159172,#159173,
#159174,#159175,#159176,#159177,#159178,#159179,#159180,#159181,#159182,
#159183,#159184,#159185,#159186,#159187,#159188,#159189,#159190,#159191,
#159192,#159193,#159194,#159195,#159196,#159197,#159198,#159199),
 .UNSPECIFIED.,.F.,.F.,(4,3,3,3,3,3,3,3,3,3,3,3,3,3,3,3,3,3,3,3,3,3,3,3,
3,3,3,3,3,3,3,3,3,3,3,3,3,3,3,3,3,3,3,3,3,3,3,3,3,3,3,3,3,3,3,3,3,3,3,3,
3,3,3,3,3,3,3,3,3,3,3,3,3,3,3,3,3,3,3,4),(-35.2689819899945,-35.1875860810853,
-35.1061679575443,-35.0247451134917,-34.9433006085595,-34.8927980315291,
-34.8104190209271,-34.7280548316773,-34.6446234958133,-34.5623015225204,
-34.4783155053709,-34.3943294882215,-34.3186893790001,-34.243073276094,
-34.1674667090403,-34.0918320463309,-34.0161824877531,-33.9404721979762,
-33.8958609449139,-33.803960375211,-33.7119274054973,-33.6200478356754,
-33.5284204396465,-33.4373993181653,-33.3973924016064,-33.3233904869182,
-33.2494095585748,-33.1754345366622,-33.1014220633622,-33.0273907933808,
-32.9532860411758,-32.8989238582988,-32.8199624423516,-32.7410550192824,
-32.6621899803458,-32.5833557496199,-32.5045407756412,-32.425719511981,
-32.3468928728687,-32.2680503484923,-32.1891814199096,-32.1102393685781,
-32.0312586030894,-31.9521875920712,-31.9019867716837,-31.8229948763452,
-31.7441030916705,-31.6653008356263,-31.5866008348049,-31.5079613889263,
-31.4293851067412,-31.4035182283762,-31.3249315052126,-31.2462953379495,
-31.1675993446332,-31.0887853131503,-31.0099038849267,-30.9309007917107,
-30.9050496850686,-30.825977163319,-30.746977608584,-30.66803934076,-30.5891507262786,
-30.5103001697224,-30.4314716654567,-30.3526552915878,-30.2738405404041,
-30.1950169064267,-30.1161468588784,-30.0372531798026,-29.9582926549656,
-29.9081125984535,-29.8340071603516,-29.7599586624969,-29.6859519244899,
-29.6119626603372,-29.5379852987251,-29.463983012692,-29.4096440551459,
-29.3426756889445),.UNSPECIFIED.);
#3159=B_SPLINE_CURVE_WITH_KNOTS('',3,(#159205,#159206,#159207,#159208,#159209,
#159210,#159211,#159212,#159213,#159214,#159215,#159216,#159217,#159218,
#159219,#159220,#159221,#159222,#159223,#159224,#159225,#159226,#159227,
#159228,#159229,#159230,#159231,#159232,#159233,#159234,#159235,#159236,
#159237,#159238,#159239,#159240,#159241,#159242,#159243,#159244,#159245,
#159246,#159247,#159248,#159249,#159250,#159251,#159252,#159253,#159254,
#159255,#159256,#159257,#159258,#159259,#159260,#159261,#159262,#159263,
#159264,#159265,#159266,#159267,#159268,#159269,#159270,#159271,#159272,
#159273,#159274,#159275,#159276,#159277,#159278,#159279,#159280,#159281,
#159282,#159283,#159284,#159285,#159286,#159287,#159288,#159289,#159290,
#159291,#159292,#159293,#159294,#159295,#159296,#159297,#159298,#159299,
#159300,#159301,#159302,#159303,#159304,#159305,#159306,#159307,#159308,
#159309,#159310,#159311,#159312,#159313,#159314,#159315,#159316,#159317,
#159318,#159319,#159320,#159321,#159322,#159323,#159324,#159325,#159326,
#159327,#159328,#159329,#159330,#159331,#159332,#159333,#159334,#159335,
#159336,#159337,#159338,#159339,#159340,#159341,#159342,#159343,#159344,
#159345,#159346,#159347,#159348,#159349,#159350,#159351,#159352,#159353,
#159354,#159355,#159356,#159357,#159358,#159359,#159360,#159361,#159362,
#159363,#159364,#159365,#159366,#159367,#159368,#159369,#159370,#159371,
#159372,#159373,#159374,#159375,#159376,#159377,#159378,#159379,#159380,
#159381,#159382,#159383,#159384,#159385,#159386,#159387,#159388,#159389,
#159390,#159391,#159392,#159393,#159394,#159395,#159396,#159397,#159398,
#159399,#159400,#159401,#159402,#159403,#159404,#159405,#159406,#159407,
#159408,#159409,#159410,#159411,#159412,#159413,#159414,#159415,#159416,
#159417,#159418,#159419,#159420,#159421,#159422,#159423,#159424,#159425,
#159426,#159427,#159428,#159429,#159430,#159431,#159432,#159433,#159434,
#159435,#159436,#159437,#159438,#159439,#159440,#159441,#159442),
 .UNSPECIFIED.,.F.,.F.,(4,3,3,3,3,3,3,3,3,3,3,3,3,3,3,3,3,3,3,3,3,3,3,3,
3,3,3,3,3,3,3,3,3,3,3,3,3,3,3,3,3,3,3,3,3,3,3,3,3,3,3,3,3,3,3,3,3,3,3,3,
3,3,3,3,3,3,3,3,3,3,3,3,3,3,3,3,3,3,3,4),(26.7981096470418,26.8902131063854,
26.9173013386081,26.9930110097253,27.0686720117508,27.1442988520881,27.2199165483701,
27.2955280484565,27.3711679730839,27.4157698819157,27.4980486537694,27.5803512166326,
27.6638230187803,27.7461779736786,27.830208199451,27.9142384252233,27.9966174358251,
28.0789816250744,28.1624129609385,28.2447349342312,28.328720951381,28.4127069685308,
28.4883470777522,28.5639631806583,28.6395697477119,28.7152044104214,28.7908539689992,
28.866564258776,28.9111755118384,29.0030760815413,29.0951090512552,29.1869886210773,
29.2786160171064,29.3696371385877,29.4096440551459,29.483645969834,29.5576268981774,
29.6316019200899,29.7056143933899,29.7796456633712,29.8537504155762,29.9081125984535,
29.9870740144007,30.0659814374699,30.1448464764065,30.2236807071324,30.302495681111,
30.3813169447712,30.4601435838836,30.5389861082599,30.6178550368427,30.6967970881741,
30.7757778536629,30.8548488646811,30.9050496850686,30.9840415804072,31.062933365082,
31.1417356211263,31.2204356219479,31.2990750678265,31.3776513500118,31.4035182283762,
31.4821049515397,31.5607411188028,31.6394371121192,31.7182511436019,31.7971325718255,
31.8761356650413,31.9019867716837,31.9796905707252,32.0573184284515,32.1348845444677,
32.2123990485688,32.289884947382,32.3673550257151,32.4448220569819,32.5223226907332,
32.5998408827482,32.6774206041791,32.7250362269146),.UNSPECIFIED.);
#3160=B_SPLINE_CURVE_WITH_KNOTS('',3,(#159443,#159444,#159445,#159446,#159447,
#159448,#159449,#159450,#159451,#159452,#159453,#159454,#159455,#159456,
#159457,#159458),.UNSPECIFIED.,.F.,.F.,(4,3,3,3,3,4),(32.7250362270345,
32.8666732039272,32.8989238582988,32.9730371102414,33.0470853245701,33.0816676322956),
 .UNSPECIFIED.);
#3161=B_SPLINE_CURVE_WITH_KNOTS('',3,(#159460,#159461,#159462,#159463,#159464,
#159465,#159466,#159467,#159468,#159469,#159470,#159471,#159472),
 .UNSPECIFIED.,.F.,.F.,(4,3,3,3,4),(-29.3426756889445,-29.252824355409,
-29.1627373608491,-29.0724643622336,-28.9857966830313),.UNSPECIFIED.);
#3162=B_SPLINE_CURVE_WITH_KNOTS('',3,(#159473,#159474,#159475,#159476,#159477,
#159478,#159479,#159480,#159481,#159482,#159483,#159484,#159485,#159486,
#159487,#159488,#159489,#159490,#159491,#159492,#159493,#159494,#159495,
#159496,#159497,#159498,#159499,#159500,#159501,#159502,#159503,#159504,
#159505,#159506,#159507,#159508,#159509,#159510,#159511,#159512,#159513,
#159514,#159515,#159516,#159517,#159518,#159519,#159520,#159521,#159522,
#159523,#159524,#159525,#159526,#159527,#159528,#159529,#159530,#159531,
#159532,#159533,#159534,#159535,#159536,#159537,#159538,#159539,#159540,
#159541,#159542,#159543,#159544,#159545,#159546,#159547,#159548,#159549,
#159550,#159551,#159552,#159553,#159554,#159555,#159556,#159557,#159558,
#159559,#159560,#159561,#159562,#159563,#159564,#159565,#159566,#159567,
#159568,#159569,#159570,#159571,#159572,#159573,#159574,#159575,#159576,
#159577,#159578,#159579,#159580,#159581,#159582,#159583,#159584,#159585,
#159586,#159587,#159588,#159589,#159590,#159591,#159592,#159593,#159594,
#159595,#159596,#159597,#159598,#159599,#159600,#159601,#159602,#159603,
#159604,#159605,#159606,#159607,#159608,#159609,#159610,#159611,#159612,
#159613,#159614,#159615,#159616,#159617,#159618,#159619,#159620,#159621,
#159622,#159623,#159624,#159625,#159626,#159627,#159628,#159629,#159630,
#159631,#159632,#159633,#159634,#159635,#159636,#159637,#159638,#159639,
#159640,#159641,#159642,#159643,#159644,#159645,#159646,#159647,#159648,
#159649,#159650,#159651,#159652,#159653,#159654,#159655,#159656,#159657,
#159658,#159659,#159660,#159661,#159662,#159663,#159664,#159665,#159666,
#159667,#159668,#159669,#159670,#159671,#159672,#159673,#159674,#159675,
#159676,#159677,#159678,#159679,#159680,#159681,#159682,#159683,#159684,
#159685,#159686,#159687,#159688,#159689,#159690,#159691,#159692,#159693,
#159694,#159695,#159696,#159697,#159698,#159699,#159700,#159701,#159702,
#159703,#159704,#159705,#159706,#159707),.UNSPECIFIED.,.F.,.F.,(4,3,3,3,
3,3,3,3,3,3,3,3,3,3,3,3,3,3,3,3,3,3,3,3,3,3,3,3,3,3,3,3,3,3,3,3,3,3,3,3,
3,3,3,3,3,3,3,3,3,3,3,3,3,3,3,3,3,3,3,3,3,3,3,3,3,3,3,3,3,3,3,3,3,3,3,3,
3,3,4),(-28.985796682929,-28.9111755118384,-28.8354658407202,-28.7598048386937,
-28.6841779983556,-28.6085603020726,-28.5329488019854,-28.4573088773571,
-28.4127069685308,-28.3304281966777,-28.2481256338155,-28.1646538316674,
-28.0822988767698,-27.9982686509965,-27.9142384252232,-27.8318594146209,
-27.7494952253709,-27.6660638895071,-27.583741916214,-27.4997558990649,
-27.4157698819157,-27.3401297726947,-27.2645136697891,-27.1889071027363,
-27.1132724400273,-27.0376228814498,-26.9619125916734,-26.9173013386081,
-26.8254007689034,-26.7333677991868,-26.641488229363,-26.5498608333321,
-26.458839711849,-26.4188327953006,-26.3448308806132,-26.2708499522705,
-26.1968749303587,-26.1228624570593,-26.0488311870786,-25.9747264348744,
-25.920364251993,-25.8414028360458,-25.7624954129767,-25.6836303740406,
-25.6047961433149,-25.5259811693365,-25.4471599056764,-25.3683332665642,
-25.289490742188,-25.2106218136058,-25.1316797622744,-25.0526989967857,
-24.9736279857675,-24.9234271653779,-24.8444352700362,-24.7655434853584,
-24.6867412293113,-24.6080412284866,-24.5294017826055,-24.4508255004176,
-24.4249586220703,-24.3463718989129,-24.2677357316562,-24.1890397383471,
-24.1102257068707,-24.0313442786536,-23.9523411854441,-23.9264900787628,
-23.8474119781529,-23.7684078578114,-23.6894660330283,-23.610582322527,
-23.5317331437529,-23.4529079627478,-23.3740962622646,-23.295225741387,
-23.216394325695,-23.1375042522246,-23.0586141787543),.UNSPECIFIED.);
#3163=B_SPLINE_CURVE_WITH_KNOTS('',3,(#159713,#159714,#159715,#159716,#159717,
#159718,#159719,#159720,#159721,#159722,#159723,#159724,#159725,#159726,
#159727,#159728,#159729,#159730,#159731,#159732,#159733,#159734,#159735,
#159736,#159737,#159738,#159739,#159740,#159741,#159742,#159743,#159744,
#159745,#159746,#159747,#159748,#159749,#159750,#159751,#159752,#159753,
#159754,#159755,#159756,#159757,#159758,#159759,#159760,#159761,#159762,
#159763,#159764,#159765,#159766,#159767,#159768,#159769,#159770,#159771,
#159772,#159773,#159774,#159775,#159776,#159777,#159778,#159779,#159780,
#159781,#159782,#159783,#159784,#159785,#159786,#159787,#159788,#159789,
#159790,#159791,#159792,#159793,#159794,#159795,#159796,#159797,#159798,
#159799,#159800,#159801,#159802,#159803,#159804,#159805,#159806,#159807,
#159808,#159809,#159810,#159811,#159812,#159813,#159814,#159815,#159816,
#159817,#159818,#159819,#159820,#159821,#159822,#159823,#159824,#159825,
#159826,#159827,#159828,#159829,#159830,#159831,#159832,#159833,#159834,
#159835,#159836,#159837,#159838,#159839,#159840,#159841,#159842,#159843,
#159844,#159845,#159846,#159847,#159848,#159849,#159850,#159851,#159852,
#159853,#159854,#159855,#159856,#159857,#159858,#159859,#159860,#159861,
#159862,#159863,#159864,#159865,#159866,#159867,#159868,#159869,#159870,
#159871,#159872,#159873,#159874,#159875,#159876,#159877,#159878,#159879,
#159880,#159881,#159882,#159883,#159884,#159885,#159886,#159887,#159888,
#159889,#159890,#159891,#159892,#159893,#159894,#159895,#159896,#159897,
#159898,#159899,#159900,#159901,#159902,#159903,#159904,#159905,#159906,
#159907,#159908,#159909,#159910,#159911,#159912,#159913,#159914,#159915,
#159916,#159917,#159918,#159919,#159920,#159921,#159922,#159923,#159924,
#159925,#159926,#159927,#159928,#159929,#159930,#159931,#159932),
 .UNSPECIFIED.,.F.,.F.,(4,3,3,3,3,3,3,3,3,3,3,3,3,3,3,3,3,3,3,3,3,3,3,3,
3,3,3,3,3,3,3,3,3,3,3,3,3,3,3,3,3,3,3,3,3,3,3,3,3,3,3,3,3,3,3,3,3,3,3,3,
3,3,3,3,3,3,3,3,3,3,3,3,3,4),(20.5148802586327,20.5966101323988,20.6783398861692,
20.7600695216108,20.8417990403898,20.9235284441734,21.0052577346279,21.0902045031471,
21.1738239784081,21.2561368993682,21.3378758084354,21.4196142978218,21.5013523742017,
21.5830900442492,21.6648273146377,21.7465641920405,21.8283006831307,21.9100367945807,
21.9917725330629,22.0735079052492,22.1552429178113,22.2369775774205,22.3187118907478,
22.400445864464,22.4821795052395,22.5639128197445,22.645645814649,22.7273784966224,
22.8091108723342,22.8908429484535,22.972574731649,23.0543062285894,23.136037445943,
23.217768390378,23.2994990685622,23.3812294871632,23.4629596528485,23.5446895722853,
23.6264192521404,23.7081486990807,23.7935768934799,23.8763354568041,23.9580740843673,
24.0398118881713,24.121548894911,24.2032851312789,24.2850206239646,24.3667553996553,
24.4484894850359,24.5302229067887,24.6119556915937,24.6936878661289,24.7754194570701,
24.8571504910911,24.9388809948637,25.0206109950583,25.1023405183429,25.1860599184374,
25.2677979994658,25.3495344948902,25.4312695114747,25.513003155963,25.5947355350801,
25.6764667555333,25.7581969240138,25.8436536734939,25.9253905917129,26.0071246006162,
26.0888561271355,26.1705855980639,26.2523204885399,26.334050568705,26.4157819977665,
26.4418509198549),.UNSPECIFIED.);
#3164=B_SPLINE_CURVE_WITH_KNOTS('',3,(#159933,#159934,#159935,#159936,#159937,
#159938,#159939,#159940,#159941,#159942,#159943,#159944,#159945),
 .UNSPECIFIED.,.F.,.F.,(4,3,3,3,4),(26.4418509198549,26.5333568795253,26.6252438530259,
26.7174516395712,26.7981096470418),.UNSPECIFIED.);
#3165=B_SPLINE_CURVE_WITH_KNOTS('',3,(#159947,#159948,#159949,#159950,#159951,
#159952,#159953,#159954,#159955,#159956,#159957,#159958,#159959,#159960,
#159961,#159962),.UNSPECIFIED.,.F.,.F.,(4,3,3,3,3,4),(-23.0586141787543,
-22.9796536386338,-22.9295529921477,-22.8479531392553,-22.7665501484863,
-22.7026113757494),.UNSPECIFIED.);
#3166=B_SPLINE_CURVE_WITH_KNOTS('',3,(#159963,#159964,#159965,#159966,#159967,
#159968,#159969,#159970,#159971,#159972,#159973,#159974,#159975,#159976,
#159977,#159978,#159979,#159980,#159981,#159982,#159983,#159984,#159985,
#159986,#159987,#159988,#159989,#159990,#159991,#159992,#159993,#159994,
#159995,#159996,#159997,#159998,#159999,#160000,#160001,#160002,#160003,
#160004,#160005,#160006,#160007,#160008,#160009,#160010,#160011,#160012,
#160013,#160014,#160015,#160016,#160017,#160018,#160019,#160020,#160021,
#160022,#160023,#160024,#160025,#160026,#160027,#160028,#160029,#160030,
#160031,#160032,#160033,#160034,#160035,#160036,#160037,#160038,#160039,
#160040,#160041,#160042,#160043,#160044,#160045,#160046,#160047,#160048,
#160049,#160050,#160051,#160052,#160053,#160054,#160055,#160056,#160057,
#160058,#160059,#160060,#160061,#160062,#160063,#160064,#160065,#160066,
#160067,#160068,#160069,#160070,#160071,#160072,#160073,#160074,#160075,
#160076,#160077,#160078,#160079,#160080,#160081,#160082,#160083,#160084,
#160085,#160086,#160087,#160088,#160089,#160090,#160091,#160092,#160093,
#160094,#160095,#160096,#160097,#160098,#160099,#160100,#160101,#160102,
#160103,#160104,#160105,#160106,#160107,#160108,#160109,#160110,#160111,
#160112,#160113,#160114,#160115,#160116,#160117,#160118,#160119,#160120,
#160121,#160122,#160123,#160124,#160125,#160126,#160127,#160128,#160129,
#160130,#160131,#160132,#160133,#160134,#160135,#160136,#160137,#160138,
#160139,#160140,#160141,#160142,#160143,#160144,#160145,#160146,#160147,
#160148,#160149,#160150,#160151,#160152,#160153,#160154,#160155,#160156,
#160157,#160158,#160159,#160160,#160161,#160162,#160163,#160164,#160165,
#160166,#160167,#160168,#160169,#160170,#160171,#160172,#160173,#160174,
#160175,#160176,#160177,#160178,#160179,#160180,#160181,#160182,#160183,
#160184,#160185,#160186,#160187,#160188,#160189,#160190,#160191,#160192,
#160193,#160194,#160195,#160196,#160197,#160198,#160199,#160200),
 .UNSPECIFIED.,.F.,.F.,(4,3,3,3,3,3,3,3,3,3,3,3,3,3,3,3,3,3,3,3,3,3,3,3,
3,3,3,3,3,3,3,3,3,3,3,3,3,3,3,3,3,3,3,3,3,3,3,3,3,3,3,3,3,3,3,3,3,3,3,3,
3,3,3,3,3,3,3,3,3,3,3,3,3,3,3,3,3,3,3,4),(-22.7026113756635,-22.63173040129,
-22.5608644977156,-22.4899738374718,-22.4310844488401,-22.3400853491217,
-22.2485821314641,-22.156638592555,-22.0646040153979,-21.9726949252976,
-21.9326159055326,-21.8569062343569,-21.7812452322732,-21.7056183918778,
-21.6300006955379,-21.5543891953937,-21.4787492707089,-21.434147362225,
-21.3518685906234,-21.2695660280155,-21.1860942257409,-21.103739271098,
-21.0197090450077,-20.9356788189174,-20.853299807784,-20.7709356180008,
-20.6875042824031,-20.6051823085844,-20.5211962920972,-20.4372102756099,
-20.3615701669439,-20.2859540645933,-20.2103474980945,-20.134712835939,
-20.0590632779147,-19.9833529886882,-19.9387417323023,-19.8468411610517,
-19.754808189751,-19.662928618399,-19.5713012209253,-19.4802800981782,-19.4402731889948,
-19.3662712745431,-19.2922903464352,-19.218315324757,-19.1443028516895,
-19.0702715819395,-18.9961668299636,-18.9418046456872,-18.8628432307598,
-18.7839358087192,-18.7050707708183,-18.6262365411328,-18.5474215681963,
-18.468600305575,-18.3897736674978,-18.3109311441513,-18.2320622165907,
-18.1531201662622,-18.0741394017655,-17.9950683917138,-17.9448675590721,
-17.8658756573626,-17.7869838663843,-17.7081816041176,-17.6294815972208,
-17.5508421453608,-17.4722658573496,-17.4463990157645,-17.3678123023036,
-17.2891761448826,-17.2104801615263,-17.1316661401196,-17.0527847220363,
-16.9737816389859,-16.947930472457,-16.866341548056,-16.7848569941609,-16.7753213308628),
 .UNSPECIFIED.);
#3167=B_SPLINE_CURVE_WITH_KNOTS('',3,(#160206,#160207,#160208,#160209,#160210,
#160211,#160212,#160213,#160214,#160215,#160216,#160217,#160218,#160219,
#160220,#160221,#160222,#160223,#160224,#160225,#160226,#160227,#160228,
#160229,#160230,#160231,#160232,#160233,#160234,#160235,#160236,#160237,
#160238,#160239,#160240,#160241,#160242,#160243,#160244,#160245,#160246,
#160247,#160248,#160249,#160250,#160251,#160252,#160253,#160254,#160255,
#160256,#160257,#160258,#160259,#160260,#160261,#160262,#160263,#160264,
#160265,#160266,#160267,#160268,#160269,#160270,#160271,#160272,#160273,
#160274,#160275,#160276,#160277,#160278,#160279,#160280,#160281,#160282,
#160283,#160284,#160285,#160286,#160287,#160288,#160289,#160290,#160291,
#160292,#160293,#160294,#160295,#160296,#160297,#160298,#160299,#160300,
#160301,#160302,#160303,#160304,#160305,#160306,#160307,#160308,#160309,
#160310,#160311,#160312,#160313,#160314,#160315,#160316,#160317,#160318,
#160319,#160320,#160321,#160322,#160323,#160324,#160325,#160326,#160327,
#160328,#160329,#160330,#160331,#160332,#160333,#160334,#160335,#160336,
#160337,#160338,#160339,#160340,#160341,#160342,#160343,#160344,#160345,
#160346,#160347,#160348,#160349,#160350,#160351,#160352,#160353,#160354,
#160355,#160356,#160357,#160358,#160359,#160360,#160361,#160362,#160363,
#160364,#160365,#160366,#160367,#160368,#160369,#160370,#160371,#160372,
#160373,#160374,#160375,#160376,#160377,#160378,#160379,#160380,#160381,
#160382,#160383,#160384,#160385,#160386,#160387,#160388,#160389,#160390,
#160391,#160392,#160393,#160394,#160395,#160396,#160397,#160398,#160399,
#160400,#160401,#160402,#160403,#160404,#160405,#160406,#160407,#160408,
#160409,#160410,#160411,#160412,#160413,#160414,#160415,#160416,#160417,
#160418,#160419,#160420,#160421,#160422,#160423,#160424,#160425,#160426,
#160427,#160428,#160429,#160430,#160431,#160432,#160433,#160434,#160435,
#160436,#160437,#160438,#160439,#160440,#160441,#160442,#160443),
 .UNSPECIFIED.,.F.,.F.,(4,3,3,3,3,3,3,3,3,3,3,3,3,3,3,3,3,3,3,3,3,3,3,3,
3,3,3,3,3,3,3,3,3,3,3,3,3,3,3,3,3,3,3,3,3,3,3,3,3,3,3,3,3,3,3,3,3,3,3,3,
3,3,3,3,3,3,3,3,3,3,3,3,3,3,3,3,3,3,3,4),(14.231883480232,14.3141973780922,
14.3964809558168,14.4555877559192,14.5312280067413,14.6068442521871,14.6824509626349,
14.7580857696397,14.8337354731209,14.9094459081311,14.9540562992267,15.0459567283529,
15.1379895501617,15.2298689719367,15.3214962250171,15.4125172166086,15.4525248425343,
15.5265267702345,15.6005077116442,15.6744827466736,15.7484952331392,15.8225265163264,
15.8966312817451,15.9509933858419,16.0299548037444,16.1088622288164,16.1877272697983,
16.2665615026073,16.345376478702,16.424197744515,16.5030243858,16.5818669123645,
16.6607358431467,16.7396778966799,16.8186586643724,16.8977296775774,16.947930472457,
17.0269223576651,17.1058141322463,17.1846163782545,17.2633163691684,17.3419558052269,
17.4205320777516,17.4463990157645,17.5249857447869,17.6036219180417,17.6823179174691,
17.7611319552012,17.8400133897525,17.9190164893673,17.9448675590721,18.0239400798595,
18.1029396336136,18.1818779004403,18.2607665139104,18.3396170694441,18.4184455726759,
18.4972619455054,18.5760766956466,18.6549003285804,18.7337703750903,18.8126640531305,
18.8916245769453,18.9418046456872,19.0159100835603,19.0899585811844,19.1639653189595,
19.2379545828783,19.3119319442551,19.385934230052,19.4402731889948,19.5312722900101,
19.6227755091177,19.7147190496085,19.8067536283734,19.8986627200372,19.9387417323023,
20.0156037252305,20.0924004463538,20.1586656126753),.UNSPECIFIED.);
#3168=B_SPLINE_CURVE_WITH_KNOTS('',3,(#160444,#160445,#160446,#160447,#160448,
#160449,#160450,#160451,#160452,#160453,#160454,#160455,#160456,#160457,
#160458,#160459),.UNSPECIFIED.,.F.,.F.,(4,3,3,3,3,4),(20.1586656126753,
20.2403951565113,20.3221302714303,20.4038605087794,20.4855922977304,20.5148802586327),
 .UNSPECIFIED.);
#3169=B_SPLINE_CURVE_WITH_KNOTS('',3,(#160461,#160462,#160463,#160464,#160465,
#160466,#160467,#160468,#160469,#160470,#160471,#160472,#160473,#160474,
#160475,#160476),.UNSPECIFIED.,.F.,.F.,(4,3,3,3,3,4),(-16.7753213308628,
-16.6939460132947,-16.6126881417199,-16.5315046550008,-16.4504174865027,
-16.4194260685698),.UNSPECIFIED.);
#3170=B_SPLINE_CURVE_WITH_KNOTS('',3,(#160477,#160478,#160479,#160480,#160481,
#160482,#160483,#160484,#160485,#160486,#160487,#160488,#160489,#160490,
#160491,#160492,#160493,#160494,#160495,#160496,#160497,#160498,#160499,
#160500,#160501,#160502,#160503,#160504,#160505,#160506,#160507,#160508,
#160509,#160510,#160511,#160512,#160513,#160514,#160515,#160516,#160517,
#160518,#160519,#160520,#160521,#160522,#160523,#160524,#160525,#160526,
#160527,#160528,#160529,#160530,#160531,#160532,#160533,#160534,#160535,
#160536,#160537,#160538,#160539,#160540,#160541,#160542,#160543,#160544,
#160545,#160546,#160547,#160548,#160549,#160550,#160551,#160552,#160553,
#160554,#160555,#160556,#160557,#160558,#160559,#160560,#160561,#160562,
#160563,#160564,#160565,#160566,#160567,#160568,#160569,#160570,#160571,
#160572,#160573,#160574,#160575,#160576,#160577,#160578,#160579,#160580,
#160581,#160582,#160583,#160584,#160585,#160586,#160587,#160588,#160589,
#160590,#160591,#160592,#160593,#160594,#160595,#160596,#160597,#160598,
#160599,#160600,#160601,#160602,#160603,#160604,#160605,#160606,#160607,
#160608,#160609,#160610,#160611,#160612,#160613,#160614,#160615,#160616,
#160617,#160618,#160619,#160620,#160621,#160622,#160623,#160624,#160625,
#160626,#160627,#160628,#160629,#160630,#160631,#160632,#160633,#160634,
#160635,#160636,#160637,#160638,#160639,#160640,#160641,#160642,#160643,
#160644,#160645,#160646,#160647,#160648,#160649,#160650,#160651,#160652,
#160653,#160654,#160655,#160656,#160657,#160658,#160659,#160660,#160661,
#160662,#160663,#160664,#160665,#160666,#160667,#160668,#160669,#160670,
#160671,#160672,#160673,#160674,#160675,#160676,#160677,#160678,#160679,
#160680,#160681,#160682,#160683,#160684,#160685,#160686,#160687,#160688,
#160689,#160690,#160691,#160692,#160693,#160694,#160695,#160696,#160697,
#160698,#160699,#160700,#160701,#160702,#160703,#160704,#160705,#160706,
#160707,#160708),.UNSPECIFIED.,.F.,.F.,(4,3,3,3,3,3,3,3,3,3,3,3,3,3,3,3,
3,3,3,3,3,3,3,3,3,3,3,3,3,3,3,3,3,3,3,3,3,3,3,3,3,3,3,3,3,3,3,3,3,3,3,3,
3,3,3,3,3,3,3,3,3,3,3,3,3,3,3,3,3,3,3,3,3,3,3,3,3,4),(-16.4194260684678,
-16.3348432118268,-16.2501027335155,-16.1651650733611,-16.0801426234198,
-15.9950222397046,-15.9509933858419,-15.8768879345363,-15.8028394234964,
-15.728832672326,-15.6548433950672,-15.5808660203712,-15.506863721332,-15.4525248425343,
-15.3615258742025,-15.270022799166,-15.1780794100646,-15.0860449819812,
-14.9941360321871,-14.9540562992267,-14.8783464830015,-14.8026853362177,
-14.7270583515563,-14.6514405119547,-14.5758288690443,-14.5001888028641,
-14.4555877559192,-14.3733093981691,-14.2910072534959,-14.2075352432749,
-14.1251807055008,-14.0411499590562,-13.9571192126116,-13.8747396035953,
-13.7923748141998,-13.7089437779758,-13.6266212155157,-13.5426359424099,
-13.4586506693041,-13.3830108845675,-13.3073951055576,-13.2317888616295,
-13.1561545200157,-13.0805052816012,-13.0047953092234,-12.9601821259965,
-12.868282108857,-12.7762497294734,-12.6843707628409,-12.5927439561573,
-12.5017233802903,-12.4617135826889,-12.3877105798512,-12.3137285580205,
-12.2397524375635,-12.1657388603515,-12.0917064823757,-12.0176006203337,
-11.9632450393814,-11.8842857069725,-11.8053803858034,-11.7265174622548,
-11.6476853555399,-11.5688725093352,-11.4900533664762,-11.4112288408948,
-11.3323884184719,-11.2535215759515,-11.1745815715412,-11.0956028314634,
-11.0165337927795,-10.9663079527663,-10.8873050792045,-10.8084026717488,
-10.72938700255,-10.6506762921222,-10.5715081435379,-10.4923399949537),
 .UNSPECIFIED.);
#3171=B_SPLINE_CURVE_WITH_KNOTS('',3,(#160714,#160715,#160716,#160717,#160718,
#160719,#160720,#160721,#160722,#160723,#160724,#160725,#160726),
 .UNSPECIFIED.,.F.,.F.,(4,3,3,3,4),(-4.2102189925341,-4.13326383456533,
-4.05618009768139,-3.98774834646046,-3.85305545421067),.UNSPECIFIED.);
#3172=B_SPLINE_CURVE_WITH_KNOTS('',3,(#160728,#160729,#160730,#160731,#160732,
#160733,#160734,#160735,#160736,#160737,#160738,#160739,#160740,#160741,
#160742,#160743,#160744,#160745,#160746,#160747,#160748,#160749,#160750,
#160751,#160752,#160753,#160754,#160755,#160756,#160757,#160758,#160759,
#160760,#160761,#160762,#160763,#160764,#160765,#160766,#160767,#160768,
#160769,#160770,#160771,#160772,#160773,#160774,#160775,#160776,#160777,
#160778,#160779,#160780,#160781,#160782,#160783,#160784,#160785,#160786,
#160787,#160788,#160789,#160790,#160791,#160792,#160793,#160794,#160795,
#160796,#160797,#160798,#160799,#160800,#160801,#160802,#160803,#160804,
#160805,#160806,#160807,#160808,#160809,#160810,#160811,#160812,#160813,
#160814,#160815,#160816,#160817,#160818,#160819,#160820,#160821,#160822,
#160823,#160824,#160825,#160826,#160827,#160828,#160829,#160830,#160831,
#160832,#160833,#160834,#160835,#160836,#160837,#160838,#160839,#160840,
#160841,#160842,#160843,#160844,#160845,#160846,#160847,#160848,#160849,
#160850,#160851,#160852,#160853,#160854,#160855,#160856,#160857,#160858,
#160859,#160860,#160861,#160862,#160863,#160864,#160865,#160866,#160867,
#160868,#160869,#160870,#160871,#160872,#160873,#160874,#160875,#160876,
#160877,#160878,#160879,#160880,#160881),.UNSPECIFIED.,.F.,.F.,(4,3,3,3,
3,3,3,3,3,3,3,3,3,3,3,3,3,3,3,3,3,3,3,3,3,3,3,3,3,3,3,3,3,3,3,3,3,3,3,3,
3,3,3,3,3,3,3,3,3,3,3,4),(-3.85305545408635,-3.77733322152493,-3.70169587286144,
-3.62612730711408,-3.54671280120549,-3.47123186819023,-3.39576658341081,
-3.32030250466635,-3.24482519243858,-3.16928858882332,-3.09371744426421,
-3.01806353171231,-2.99081125984535,-2.91338960182974,-2.83602915369424,
-2.75871684786117,-2.68143942843154,-2.604182561553,-2.52692488276581,-2.49234271653779,
-2.40529897332284,-2.31804420440917,-2.23057731574574,-2.14304930038302,
-2.05551593212837,-1.99387417323023,-1.91787097808727,-1.84191628058941,
-1.76599575933275,-1.69008513708016,-1.61418100207181,-1.53824993894703,
-1.49540562992267,-1.41140303908181,-1.32734729720491,-1.24323359539477,
-1.15911065250105,-1.07498942323625,-0.996937086615118,-0.918227407423238,
-0.839546602114508,-0.760883798027845,-0.682216838298316,-0.60354847363303,
-0.524852928628286,-0.498468543307558,-0.417045733774206,-0.335632904215115,
-0.251724678161337,-0.170320627264329,-0.0851603136321654,-1.82627892504507E-15),
 .UNSPECIFIED.);
#3173=B_SPLINE_CURVE_WITH_KNOTS('',3,(#160885,#160886,#160887,#160888,#160889,
#160890,#160891,#160892,#160893,#160894,#160895,#160896,#160897,#160898,
#160899,#160900,#160901,#160902,#160903,#160904,#160905,#160906,#160907,
#160908,#160909,#160910,#160911,#160912,#160913,#160914,#160915,#160916,
#160917,#160918,#160919,#160920,#160921,#160922,#160923,#160924,#160925,
#160926,#160927,#160928,#160929,#160930,#160931,#160932,#160933,#160934,
#160935,#160936,#160937,#160938,#160939,#160940,#160941,#160942,#160943,
#160944,#160945,#160946,#160947,#160948,#160949,#160950,#160951,#160952,
#160953,#160954,#160955,#160956,#160957,#160958,#160959,#160960,#160961,
#160962,#160963,#160964,#160965,#160966,#160967,#160968,#160969,#160970,
#160971,#160972,#160973,#160974,#160975,#160976,#160977,#160978,#160979,
#160980,#160981,#160982,#160983,#160984,#160985,#160986,#160987,#160988,
#160989,#160990,#160991,#160992,#160993,#160994,#160995,#160996,#160997,
#160998,#160999,#161000,#161001,#161002,#161003,#161004,#161005,#161006,
#161007,#161008,#161009,#161010,#161011,#161012,#161013,#161014,#161015,
#161016,#161017,#161018,#161019,#161020,#161021,#161022,#161023,#161024,
#161025,#161026,#161027,#161028,#161029,#161030,#161031,#161032,#161033,
#161034,#161035,#161036,#161037,#161038,#161039,#161040,#161041,#161042,
#161043,#161044,#161045,#161046,#161047,#161048,#161049,#161050,#161051,
#161052,#161053,#161054,#161055,#161056,#161057,#161058,#161059,#161060,
#161061,#161062,#161063,#161064,#161065,#161066,#161067,#161068,#161069,
#161070,#161071,#161072,#161073,#161074,#161075,#161076,#161077,#161078,
#161079,#161080,#161081,#161082,#161083,#161084,#161085,#161086,#161087,
#161088,#161089,#161090,#161091,#161092,#161093,#161094,#161095,#161096,
#161097,#161098,#161099,#161100,#161101,#161102,#161103,#161104),
 .UNSPECIFIED.,.F.,.F.,(4,3,3,3,3,3,3,3,3,3,3,3,3,3,3,3,3,3,3,3,3,3,3,3,
3,3,3,3,3,3,3,3,3,3,3,3,3,3,3,3,3,3,3,3,3,3,3,3,3,3,3,3,3,3,3,3,3,3,3,3,
3,3,3,3,3,3,3,3,3,3,3,3,3,4),(2.02057330133861,2.10731855090179,2.19404294025265,
2.28065105473334,2.36714678612864,2.45341692392646,2.49234271653779,2.56960253681016,
2.64685977983922,2.72412743925298,2.80144758367556,2.87879733597736,2.95622233760274,
2.99081125984535,3.06769470829953,3.14450839872675,3.22126734333478,3.29798651594428,
3.37468086167416,3.45138294474633,3.5280927188547,3.60482370957874,3.68158945170787,
3.75845454953412,3.83537082665699,3.91241786308591,3.98774834646046,4.0648418860315,
4.14183633541153,4.21874677598679,4.29558823062224,4.37237567418249,4.44912607179099,
4.52585691122378,4.602581687806,4.6793138909937,4.7561022859856,4.83291830588097,
4.90982555495308,4.98468543307558,5.06203195585688,5.13931811616054,5.21655706794557,
5.29376277077859,5.37094887235525,5.44813746534129,5.48315397638314,5.57026302863232,
5.65758273008965,5.74511166625669,5.8326992021723,5.92028639032618,5.9816225196907,
6.05788321116819,6.13409549162699,6.21027349698447,6.28644077030324,6.36260118254298,
6.4387870172689,6.48009106299825,6.5625136809008,6.64496553473764,6.72836405262968,
6.81087749609412,6.89471855119997,6.97855960630581,7.06056935141231,7.14255800395656,
7.22617554037076,7.30811590022636,7.39257202491986,7.47702814961337,7.55692378696674,
7.59229499831615),.UNSPECIFIED.);
#3174=B_SPLINE_CURVE_WITH_KNOTS('',3,(#161105,#161106,#161107,#161108,#161109,
#161110,#161111,#161112,#161113,#161114,#161115,#161116,#161117,#161118,
#161119,#161120),.UNSPECIFIED.,.F.,.F.,(4,3,3,3,3,4),(7.59229499839287,
7.66781581452666,7.74335395647864,7.81890012251005,7.89450003993217,7.94810021833352),
 .UNSPECIFIED.);
#3175=B_SPLINE_CURVE_WITH_KNOTS('',3,(#161123,#161124,#161125,#161126,#161127,
#161128,#161129,#161130,#161131,#161132,#161133,#161134,#161135,#161136,
#161137,#161138,#161139,#161140,#161141,#161142,#161143,#161144,#161145,
#161146,#161147,#161148,#161149,#161150,#161151,#161152,#161153,#161154,
#161155,#161156,#161157,#161158,#161159,#161160,#161161,#161162,#161163,
#161164,#161165,#161166,#161167,#161168,#161169,#161170,#161171,#161172,
#161173,#161174,#161175,#161176,#161177,#161178,#161179,#161180,#161181,
#161182,#161183,#161184,#161185,#161186,#161187,#161188,#161189,#161190,
#161191,#161192,#161193,#161194,#161195,#161196,#161197,#161198,#161199,
#161200,#161201,#161202,#161203,#161204,#161205,#161206,#161207,#161208,
#161209,#161210,#161211,#161212,#161213,#161214,#161215,#161216,#161217,
#161218,#161219,#161220,#161221,#161222,#161223,#161224,#161225,#161226,
#161227,#161228,#161229,#161230,#161231,#161232,#161233,#161234,#161235,
#161236,#161237,#161238,#161239,#161240,#161241,#161242,#161243,#161244,
#161245,#161246,#161247,#161248,#161249,#161250,#161251,#161252,#161253,
#161254,#161255,#161256,#161257,#161258,#161259,#161260,#161261,#161262,
#161263,#161264,#161265,#161266,#161267,#161268,#161269,#161270,#161271,
#161272,#161273,#161274,#161275,#161276,#161277,#161278,#161279,#161280,
#161281,#161282,#161283,#161284,#161285,#161286,#161287,#161288,#161289,
#161290,#161291,#161292,#161293,#161294,#161295,#161296,#161297,#161298,
#161299,#161300,#161301,#161302,#161303,#161304,#161305,#161306,#161307,
#161308,#161309,#161310,#161311,#161312,#161313,#161314,#161315,#161316,
#161317,#161318,#161319,#161320,#161321,#161322,#161323,#161324,#161325,
#161326,#161327,#161328,#161329,#161330,#161331,#161332,#161333,#161334,
#161335,#161336,#161337,#161338,#161339,#161340,#161341,#161342,#161343,
#161344,#161345,#161346,#161347,#161348,#161349,#161350,#161351,#161352,
#161353,#161354,#161355,#161356,#161357,#161358,#161359,#161360),
 .UNSPECIFIED.,.F.,.F.,(4,3,3,3,3,3,3,3,3,3,3,3,3,3,3,3,3,3,3,3,3,3,3,3,
3,3,3,3,3,3,3,3,3,3,3,3,3,3,3,3,3,3,3,3,3,3,3,3,3,3,3,3,3,3,3,3,3,3,3,3,
3,3,3,3,3,3,3,3,3,3,3,3,3,3,3,3,3,3,3,4),(7.94810021833352,7.97549669292093,
8.06711656730402,8.15885338523794,8.25043489219158,8.34177330665132,8.43252992566801,
8.47396523622849,8.54800828867236,8.62203064070959,8.69604736092453,8.77010186103058,
8.84417538298251,8.91832256609645,8.97243377953604,9.05139060932345,9.13029334033861,
9.20915359340074,9.28798295643997,9.36679299287031,9.44560924431697,9.52443083233563,
9.60326827720018,9.68213210828826,9.76106907071863,9.84004475086048,9.91911072933346,
9.96937086615116,10.048353892304,10.1272368201723,10.206030249966,10.2847215077339,
10.3633522701407,10.4419199839626,10.4678394094587,10.5464330284591,10.6250762646076,
10.7037794841114,10.7826009287505,10.8614898765492,10.9405005932523,10.9663079527663,
11.0453785106916,11.1243760632993,11.2033122956374,11.2821988461979,11.3610473153034,
11.4398737088712,11.5186879609097,11.5975005834405,11.6763220862447,11.7551900128592,
11.8340815766776,11.9130400130903,11.9632450393814,12.0373515864893,12.1114011909516,
12.1854090328583,12.2593993948568,12.333377851737,12.4073812254331,12.461713582689,
12.5527121304417,12.6442147576327,12.7361576887354,12.8281916681528,12.9201002063867,
12.9601821259965,13.0358914799109,13.1115521628426,13.1871786823854,13.2627960560663,
13.3384072323673,13.4140468325296,13.4586506693041,13.5410375115435,13.6246482100316,
13.7070972633513,13.7912887844235,13.8754803054957),.UNSPECIFIED.);
#3176=B_SPLINE_CURVE_WITH_KNOTS('',3,(#161361,#161362,#161363,#161364,#161365,
#161366,#161367,#161368,#161369,#161370,#161371,#161372,#161373,#161374,
#161375,#161376),.UNSPECIFIED.,.F.,.F.,(4,3,3,3,3,4),(13.8754803056222,
13.9571192126116,14.0394983452062,14.1218621763033,14.2042074048479,14.231883480232),
 .UNSPECIFIED.);
#3177=B_SPLINE_CURVE_WITH_KNOTS('',3,(#161378,#161379,#161380,#161381,#161382,
#161383,#161384,#161385,#161386,#161387,#161388,#161389,#161390,#161391,
#161392,#161393,#161394,#161395,#161396),.UNSPECIFIED.,.F.,.F.,(4,3,3,3,
3,3,4),(-10.4923399949537,-10.4678394094587,-10.3929239454309,-10.3179640637741,
-10.2429787777672,-10.1679214833374,-10.1362407614956),.UNSPECIFIED.);
#3178=B_SPLINE_CURVE_WITH_KNOTS('',3,(#161397,#161398,#161399,#161400,#161401,
#161402,#161403,#161404,#161405,#161406,#161407,#161408,#161409,#161410,
#161411,#161412,#161413,#161414,#161415,#161416,#161417,#161418,#161419,
#161420,#161421,#161422,#161423,#161424,#161425,#161426,#161427,#161428,
#161429,#161430,#161431,#161432,#161433,#161434,#161435,#161436,#161437,
#161438,#161439,#161440,#161441,#161442,#161443,#161444,#161445,#161446,
#161447,#161448,#161449,#161450,#161451,#161452,#161453,#161454,#161455,
#161456,#161457,#161458,#161459,#161460,#161461,#161462,#161463,#161464,
#161465,#161466,#161467,#161468,#161469,#161470,#161471,#161472,#161473,
#161474,#161475,#161476,#161477,#161478,#161479,#161480,#161481,#161482,
#161483,#161484,#161485,#161486,#161487,#161488,#161489,#161490,#161491,
#161492,#161493,#161494,#161495,#161496,#161497,#161498,#161499,#161500,
#161501,#161502,#161503,#161504,#161505,#161506,#161507,#161508,#161509,
#161510,#161511,#161512,#161513,#161514,#161515,#161516,#161517,#161518,
#161519,#161520,#161521,#161522,#161523,#161524,#161525,#161526,#161527,
#161528,#161529,#161530,#161531,#161532,#161533,#161534,#161535,#161536,
#161537,#161538,#161539,#161540,#161541,#161542,#161543,#161544,#161545,
#161546,#161547,#161548,#161549,#161550,#161551,#161552,#161553,#161554,
#161555,#161556,#161557,#161558,#161559,#161560,#161561,#161562,#161563,
#161564,#161565,#161566,#161567,#161568,#161569,#161570,#161571,#161572,
#161573,#161574,#161575,#161576,#161577,#161578,#161579,#161580,#161581,
#161582,#161583,#161584,#161585,#161586,#161587,#161588,#161589,#161590,
#161591,#161592,#161593,#161594,#161595,#161596,#161597,#161598,#161599,
#161600,#161601,#161602,#161603,#161604,#161605,#161606,#161607,#161608,
#161609,#161610,#161611,#161612,#161613,#161614,#161615,#161616,#161617,
#161618,#161619,#161620,#161621,#161622,#161623,#161624,#161625,#161626,
#161627,#161628),.UNSPECIFIED.,.F.,.F.,(4,3,3,3,3,3,3,3,3,3,3,3,3,3,3,3,
3,3,3,3,3,3,3,3,3,3,3,3,3,3,3,3,3,3,3,3,3,3,3,3,3,3,3,3,3,3,3,3,3,3,3,3,
3,3,3,3,3,3,3,3,3,3,3,3,3,3,3,3,3,3,3,3,3,3,3,3,3,4),(-10.1362407613902,
-10.0404600103124,-9.96937086615116,-9.8903033587492,-9.81130884994392,
-9.73237564784757,-9.6534921071148,-9.57464662055245,-9.49582315096894,
-9.41701178211171,-9.33820199578966,-9.25938327602393,-9.18051803145294,
-9.10162909268758,-9.02267316761131,-8.97243377953605,-8.89828594006323,
-8.82419521271217,-8.75014642909095,-8.67611547493831,-8.60209659116966,
-8.5280531838428,-8.47396523622849,-8.38323357259632,-8.29201898422131,
-8.20037668423165,-8.10864103046863,-8.01701229140009,-7.97549669292093,
-7.89958045794402,-7.8237135551364,-7.7478816022398,-7.67206048741651,-7.59624643142938,
-7.52040599733432,-7.47702814961337,-7.39512802038051,-7.31320693723104,
-7.22954510449973,-7.14756893457477,-7.06306427044029,-6.97855960630581,
-6.89601880972164,-6.8134943777379,-6.73014354905299,-6.64766910379144,
-6.56388008339485,-6.48009106299825,-6.40390489046263,-6.32774052041723,
-6.25158385234168,-6.17539790943762,-6.09919606680476,-6.02293430473634,
-5.9816225196907,-5.89404183989763,-5.80644096685919,-5.71892858368981,
-5.63152502623376,-5.54438007077154,-5.48315397638314,-5.40596340742709,
-5.32877675294137,-5.25158093002387,-5.17433419106375,-5.09705876196652,
-5.01970908073965,-4.98468543307558,-4.90776221233483,-4.83091062748332,
-4.75332417311467,-4.67657256393022,-4.59984318628236,-4.52312254376973,
-4.44489665596082,-4.36812994750742,-4.28917447002076,-4.2102189925341),
 .UNSPECIFIED.);
#3179=B_SPLINE_CURVE_WITH_KNOTS('',3,(#161632,#161633,#161634,#161635,#161636,
#161637,#161638,#161639,#161640,#161641,#161642,#161643,#161644,#161645,
#161646,#161647,#161648,#161649,#161650,#161651,#161652,#161653,#161654,
#161655,#161656,#161657,#161658,#161659,#161660,#161661,#161662,#161663,
#161664,#161665,#161666,#161667,#161668,#161669,#161670,#161671,#161672,
#161673,#161674,#161675,#161676,#161677,#161678,#161679,#161680,#161681,
#161682,#161683,#161684,#161685,#161686),.UNSPECIFIED.,.F.,.F.,(4,3,3,3,
3,3,3,3,3,3,3,3,3,3,3,3,3,3,4),(14.3988535768134,14.4773090887871,14.5557627497234,
14.6342164121779,14.7126808485184,14.7911453674607,14.8696199926236,14.897322120121,
14.9731691685373,15.0489941245849,15.1248067164951,15.2006302452213,15.2764581123458,
15.3523191565515,15.3957906634286,15.4769611354302,15.5581346632558,15.639296551796,
15.7079632679496),.UNSPECIFIED.);
#3180=B_SPLINE_CURVE_WITH_KNOTS('',3,(#161690,#161691,#161692,#161693,#161694,
#161695,#161696,#161697),.UNSPECIFIED.,.F.,.F.,(4,2,2,4),(13.8754803054958,
14.7048380819337,15.5341958583716,15.7079632679496),.UNSPECIFIED.);
#3181=B_SPLINE_CURVE_WITH_KNOTS('',3,(#161699,#161700,#161701,#161702,#161703,
#161704,#161705,#161706,#161707,#161708,#161709,#161710,#161711,#161712,
#161713),.UNSPECIFIED.,.F.,.F.,(4,1,1,1,1,1,1,1,1,1,1,1,4),(15.7079632679496,
15.8426561601993,16.8395932468144,17.338061790122,17.8365303334295,18.3349988767371,
18.8334674200446,19.3319359633522,19.8304045066598,20.3288730499673,20.8273415932749,
21.82427867989,21.9911485751291),.UNSPECIFIED.);
#3182=B_SPLINE_CURVE_WITH_KNOTS('',3,(#161715,#161716,#161717,#161718,#161719,
#161720,#161721,#161722,#161723,#161724,#161725,#161726,#161727,#161728,
#161729,#161730,#161731,#161732,#161733,#161734,#161735,#161736,#161737,
#161738,#161739,#161740,#161741,#161742,#161743,#161744,#161745,#161746,
#161747,#161748,#161749,#161750,#161751,#161752,#161753,#161754,#161755,
#161756,#161757,#161758,#161759,#161760,#161761,#161762,#161763,#161764,
#161765,#161766,#161767,#161768,#161769,#161770,#161771,#161772,#161773,
#161774,#161775,#161776,#161777,#161778,#161779,#161780,#161781,#161782,
#161783,#161784,#161785,#161786,#161787,#161788,#161789,#161790,#161791,
#161792,#161793,#161794,#161795,#161796,#161797,#161798,#161799,#161800,
#161801,#161802,#161803,#161804,#161805,#161806,#161807,#161808,#161809,
#161810,#161811,#161812,#161813,#161814,#161815,#161816,#161817,#161818,
#161819,#161820,#161821,#161822,#161823,#161824,#161825,#161826,#161827,
#161828,#161829,#161830,#161831,#161832,#161833,#161834,#161835,#161836,
#161837,#161838,#161839,#161840,#161841,#161842,#161843,#161844,#161845,
#161846,#161847,#161848,#161849,#161850,#161851,#161852,#161853,#161854,
#161855,#161856,#161857,#161858,#161859,#161860,#161861,#161862,#161863,
#161864,#161865,#161866,#161867,#161868,#161869,#161870,#161871,#161872,
#161873,#161874,#161875,#161876,#161877,#161878,#161879,#161880,#161881,
#161882,#161883,#161884,#161885,#161886,#161887,#161888,#161889,#161890,
#161891,#161892,#161893,#161894,#161895,#161896,#161897,#161898,#161899,
#161900,#161901,#161902,#161903,#161904,#161905,#161906,#161907,#161908,
#161909,#161910,#161911,#161912,#161913,#161914,#161915,#161916,#161917,
#161918,#161919,#161920,#161921,#161922,#161923,#161924,#161925,#161926,
#161927,#161928,#161929,#161930,#161931,#161932,#161933,#161934,#161935,
#161936,#161937,#161938,#161939,#161940,#161941,#161942,#161943,#161944,
#161945,#161946,#161947,#161948,#161949,#161950,#161951,#161952,#161953,
#161954,#161955,#161956,#161957,#161958,#161959,#161960,#161961,#161962,
#161963,#161964,#161965,#161966,#161967,#161968,#161969,#161970),
 .UNSPECIFIED.,.F.,.F.,(4,3,3,3,3,3,3,3,3,3,3,3,3,3,3,3,3,3,3,3,3,3,3,3,
3,3,3,3,3,3,3,3,3,3,3,3,3,3,3,3,3,3,3,3,3,3,3,3,3,3,3,3,3,3,3,3,3,3,3,3,
3,3,3,3,3,3,3,3,3,3,3,3,3,3,3,3,3,3,3,3,3,3,3,3,3,4),(21.9911485751291,
22.063496052357,22.1357752717274,22.2080149164767,22.28022855992,22.3227472231976,
22.3984962342701,22.4742911622871,22.5501412873131,22.6261033785794,22.702127044247,
22.7782701758204,22.8212157665051,22.8974244542329,22.9735651300765,23.0496482567728,
23.1256842565747,23.2016835182255,23.2787421850874,23.3547054036644,23.4306649451627,
23.5066302188929,23.5845108774497,23.6605386368451,23.7393457449827,23.8181528531202,
23.8895771968369,23.9609483903943,24.0322800260588,24.1035944219084,24.1748961647337,
24.2462226946391,24.3166213964278,24.4043263537643,24.4925021480966,24.5811059728463,
24.669805701723,24.7584014261205,24.8150899397353,24.8880590784629,24.9609827620746,
25.0338739797433,25.1067558678726,25.1796304740047,25.2525331111681,25.3135584830429,
25.3928598158705,25.4721833074765,25.5515264797574,25.6309001340357,25.7102823939454,
25.7896797474913,25.8120270263505,25.8914240280869,25.9708073030149,26.0501743520023,
26.1295191321404,26.2088417487659,26.2881355804246,26.310495569658,26.3833981064024,
26.4562781007974,26.5291485083777,26.6020449917875,26.6749537871511,26.7479222399894,
26.8089641129656,26.8975383090898,26.9862385321724,27.0748052013842,27.1631484764552,
27.2509180668742,27.3074326562731,27.3787561671641,27.4500599299111,27.5213574458225,
27.5926899541536,27.6640383256156,27.7354589933113,27.8059011995807,27.8879447479105,
27.9699232619414,28.0517634418163,28.1335007431438,28.2150493567445,28.2743338822451),
 .UNSPECIFIED.);
#3183=B_SPLINE_CURVE_WITH_KNOTS('',3,(#161972,#161973,#161974,#161975,#161976,
#161977,#161978,#161979,#161980,#161981,#161982,#161983,#161984,#161985,
#161986,#161987,#161988,#161989,#161990,#161991,#161992,#161993,#161994,
#161995,#161996,#161997,#161998,#161999,#162000,#162001,#162002,#162003,
#162004,#162005,#162006,#162007,#162008,#162009,#162010,#162011,#162012,
#162013,#162014,#162015,#162016,#162017,#162018,#162019,#162020,#162021,
#162022,#162023,#162024,#162025,#162026,#162027,#162028,#162029,#162030,
#162031,#162032,#162033,#162034,#162035,#162036,#162037,#162038,#162039,
#162040,#162041,#162042,#162043,#162044,#162045,#162046,#162047,#162048,
#162049,#162050,#162051,#162052,#162053,#162054,#162055,#162056,#162057,
#162058,#162059,#162060,#162061,#162062,#162063,#162064,#162065,#162066,
#162067,#162068,#162069,#162070,#162071,#162072,#162073,#162074,#162075,
#162076,#162077,#162078,#162079,#162080,#162081,#162082,#162083,#162084,
#162085,#162086,#162087,#162088,#162089,#162090,#162091,#162092,#162093,
#162094,#162095,#162096,#162097,#162098,#162099,#162100,#162101,#162102,
#162103,#162104,#162105,#162106,#162107,#162108,#162109,#162110,#162111,
#162112,#162113,#162114,#162115,#162116,#162117,#162118,#162119,#162120,
#162121,#162122,#162123,#162124,#162125,#162126,#162127,#162128,#162129,
#162130,#162131,#162132,#162133,#162134,#162135,#162136,#162137,#162138,
#162139,#162140,#162141,#162142,#162143,#162144,#162145,#162146,#162147,
#162148,#162149,#162150,#162151,#162152,#162153,#162154,#162155,#162156,
#162157,#162158,#162159,#162160,#162161,#162162,#162163,#162164,#162165,
#162166,#162167,#162168,#162169,#162170,#162171,#162172,#162173,#162174,
#162175,#162176,#162177,#162178,#162179,#162180,#162181,#162182,#162183,
#162184,#162185,#162186,#162187,#162188,#162189,#162190,#162191,#162192,
#162193,#162194,#162195,#162196,#162197,#162198,#162199,#162200,#162201,
#162202,#162203,#162204,#162205,#162206,#162207,#162208,#162209,#162210,
#162211,#162212,#162213,#162214,#162215,#162216,#162217,#162218,#162219,
#162220,#162221,#162222,#162223,#162224,#162225,#162226,#162227),
 .UNSPECIFIED.,.F.,.F.,(4,3,3,3,3,3,3,3,3,3,3,3,3,3,3,3,3,3,3,3,3,3,3,3,
3,3,3,3,3,3,3,3,3,3,3,3,3,3,3,3,3,3,3,3,3,3,3,3,3,3,3,3,3,3,3,3,3,3,3,3,
3,3,3,3,3,3,3,3,3,3,3,3,3,3,3,3,3,3,3,3,3,3,3,3,3,4),(28.2743338823087,
28.3524992901552,28.4307348821981,28.5090430266781,28.5874765565581,28.6659730322945,
28.7445841671321,28.8028382861958,28.8789711486772,28.9550108400185,29.030966835712,
29.1068252686922,29.1826263227681,29.2583656341798,29.3013068295034,29.3770491999729,
29.452837326493,29.5286805032169,29.604635467491,29.6806519059134,29.7567877075728,
29.7997753728109,29.8759859523571,29.9521285556643,30.0282136410446,30.1042516263436,
30.1802528959144,30.2573103413534,30.3332756024773,30.4092371933377,30.4852045193935,
30.5630815044016,30.6391113008366,30.7179118801313,30.796712459426,30.8681357340553,
30.9395058607466,31.0108364320444,31.0821497693047,31.1534504559005,31.2247759371654,
31.2951810027336,31.3828864933078,31.4710628571004,31.5596672692188,31.6483675776298,
31.7369638390569,31.7936495460412,31.8666189899611,31.9395429805229,32.0124345067303,
32.0853167051164,32.1581916226244,32.2310945717994,32.2921180893487,32.3714188737895,
32.4507418047674,32.530084407287,32.6094574849733,32.6888391664853,32.7682359441056,
32.7905866326563,32.8699840270845,32.9493677006684,33.0287351520635,33.1080803356296,
33.1874033546504,33.2666975840301,33.2890551759638,33.3619575762874,33.4348374333879,
33.5077077028764,33.5806040473371,33.6535127031778,33.7264810161821,33.7875237192714,
33.8760980508646,33.9647984163178,34.053365228401,34.141708641946,34.2294783585552,
34.2859922625789,34.3543180996439,34.4226219070607,34.4909372077778,34.5575191894883),
 .UNSPECIFIED.);
#3184=B_SPLINE_CURVE_WITH_KNOTS('',3,(#162229,#162230,#162231,#162232,#162233,
#162234,#162235,#162236,#162237,#162238,#162239,#162240,#162241,#162242,
#162243,#162244,#162245,#162246,#162247,#162248,#162249,#162250,#162251,
#162252,#162253,#162254,#162255,#162256,#162257,#162258,#162259,#162260,
#162261,#162262,#162263,#162264,#162265,#162266,#162267,#162268,#162269,
#162270,#162271,#162272,#162273,#162274,#162275,#162276,#162277,#162278,
#162279,#162280,#162281,#162282,#162283,#162284,#162285,#162286,#162287,
#162288,#162289,#162290,#162291,#162292,#162293,#162294,#162295,#162296,
#162297,#162298,#162299,#162300,#162301,#162302,#162303,#162304,#162305,
#162306,#162307,#162308,#162309,#162310,#162311,#162312,#162313,#162314,
#162315,#162316,#162317,#162318,#162319,#162320,#162321,#162322,#162323,
#162324,#162325,#162326,#162327,#162328,#162329,#162330,#162331,#162332,
#162333,#162334,#162335,#162336,#162337,#162338,#162339,#162340,#162341,
#162342,#162343,#162344,#162345,#162346,#162347,#162348,#162349,#162350,
#162351,#162352,#162353,#162354,#162355,#162356,#162357,#162358,#162359,
#162360,#162361,#162362,#162363,#162364,#162365,#162366,#162367,#162368,
#162369,#162370,#162371,#162372,#162373,#162374,#162375,#162376,#162377,
#162378,#162379,#162380,#162381,#162382,#162383,#162384,#162385,#162386,
#162387,#162388,#162389,#162390,#162391,#162392,#162393,#162394,#162395,
#162396,#162397,#162398,#162399,#162400,#162401,#162402,#162403,#162404,
#162405,#162406,#162407,#162408,#162409,#162410,#162411,#162412,#162413,
#162414,#162415,#162416,#162417,#162418,#162419,#162420,#162421,#162422,
#162423,#162424,#162425,#162426,#162427,#162428,#162429,#162430,#162431,
#162432,#162433,#162434,#162435,#162436,#162437,#162438,#162439,#162440,
#162441,#162442,#162443,#162444,#162445,#162446,#162447,#162448,#162449,
#162450,#162451,#162452,#162453,#162454,#162455,#162456,#162457,#162458,
#162459,#162460,#162461,#162462,#162463,#162464,#162465,#162466,#162467,
#162468,#162469,#162470,#162471,#162472,#162473,#162474,#162475,#162476,
#162477,#162478,#162479,#162480,#162481,#162482,#162483,#162484,#162485,
#162486,#162487,#162488,#162489,#162490,#162491,#162492,#162493,#162494,
#162495,#162496,#162497,#162498,#162499,#162500,#162501,#162502,#162503,
#162504,#162505,#162506,#162507,#162508,#162509,#162510,#162511,#162512,
#162513,#162514,#162515,#162516,#162517,#162518,#162519,#162520,#162521,
#162522,#162523,#162524,#162525,#162526,#162527,#162528,#162529,#162530,
#162531,#162532,#162533,#162534,#162535,#162536,#162537,#162538,#162539,
#162540,#162541,#162542,#162543,#162544,#162545,#162546,#162547,#162548,
#162549,#162550,#162551,#162552,#162553,#162554,#162555,#162556,#162557,
#162558,#162559,#162560,#162561,#162562,#162563,#162564,#162565,#162566,
#162567,#162568,#162569,#162570,#162571,#162572,#162573,#162574,#162575,
#162576,#162577,#162578,#162579,#162580,#162581,#162582,#162583,#162584,
#162585,#162586,#162587,#162588,#162589,#162590,#162591,#162592,#162593,
#162594,#162595,#162596,#162597,#162598,#162599,#162600,#162601,#162602,
#162603,#162604,#162605,#162606,#162607,#162608,#162609,#162610,#162611,
#162612,#162613,#162614,#162615,#162616,#162617,#162618,#162619,#162620,
#162621,#162622,#162623,#162624,#162625,#162626,#162627,#162628,#162629,
#162630,#162631,#162632,#162633,#162634,#162635,#162636,#162637,#162638,
#162639,#162640,#162641,#162642,#162643,#162644,#162645,#162646,#162647,
#162648,#162649,#162650,#162651,#162652,#162653,#162654,#162655,#162656,
#162657,#162658,#162659,#162660,#162661,#162662,#162663,#162664,#162665,
#162666,#162667,#162668,#162669,#162670,#162671,#162672,#162673,#162674,
#162675,#162676,#162677,#162678,#162679,#162680,#162681,#162682,#162683,
#162684,#162685,#162686,#162687,#162688,#162689,#162690,#162691,#162692,
#162693,#162694,#162695,#162696,#162697,#162698,#162699,#162700,#162701,
#162702,#162703,#162704,#162705,#162706,#162707,#162708,#162709,#162710,
#162711,#162712,#162713,#162714,#162715,#162716,#162717,#162718,#162719,
#162720,#162721,#162722,#162723,#162724,#162725,#162726,#162727,#162728,
#162729,#162730,#162731,#162732,#162733,#162734,#162735,#162736,#162737,
#162738,#162739,#162740,#162741,#162742,#162743,#162744,#162745,#162746,
#162747,#162748,#162749,#162750,#162751,#162752,#162753,#162754,#162755,
#162756,#162757,#162758,#162759,#162760,#162761,#162762,#162763,#162764,
#162765,#162766,#162767,#162768,#162769,#162770,#162771,#162772,#162773,
#162774,#162775,#162776,#162777,#162778,#162779,#162780,#162781,#162782,
#162783,#162784,#162785,#162786,#162787,#162788,#162789,#162790,#162791,
#162792,#162793,#162794,#162795,#162796,#162797,#162798,#162799,#162800,
#162801,#162802,#162803,#162804,#162805,#162806,#162807,#162808,#162809,
#162810,#162811,#162812,#162813,#162814,#162815,#162816,#162817,#162818,
#162819,#162820,#162821,#162822,#162823,#162824,#162825,#162826,#162827,
#162828,#162829,#162830,#162831,#162832,#162833,#162834,#162835,#162836,
#162837,#162838,#162839,#162840,#162841,#162842,#162843,#162844,#162845,
#162846,#162847,#162848,#162849,#162850,#162851,#162852,#162853,#162854,
#162855,#162856,#162857,#162858,#162859,#162860,#162861,#162862,#162863,
#162864,#162865,#162866,#162867,#162868,#162869,#162870,#162871,#162872,
#162873,#162874,#162875,#162876,#162877,#162878,#162879,#162880,#162881,
#162882,#162883,#162884,#162885,#162886,#162887,#162888,#162889,#162890,
#162891,#162892,#162893,#162894,#162895,#162896,#162897,#162898,#162899,
#162900,#162901,#162902,#162903,#162904,#162905,#162906,#162907,#162908,
#162909,#162910,#162911,#162912,#162913,#162914,#162915,#162916,#162917,
#162918,#162919,#162920,#162921,#162922,#162923,#162924,#162925,#162926,
#162927,#162928,#162929,#162930,#162931,#162932,#162933,#162934),
 .UNSPECIFIED.,.F.,.F.,(4,2,2,2,2,2,2,2,2,2,2,2,2,2,2,2,2,2,2,2,2,2,2,2,
2,2,2,2,2,2,2,2,2,2,2,2,2,2,2,2,2,2,2,2,2,2,2,2,2,2,2,2,2,2,2,2,2,2,2,2,
2,2,2,2,2,2,2,2,2,2,2,2,2,2,2,2,2,2,2,2,2,2,2,2,2,2,2,2,2,2,2,2,2,2,2,2,
2,2,2,2,2,2,2,2,2,2,2,2,2,2,2,2,2,2,2,2,2,2,2,2,2,2,2,2,2,2,2,2,2,2,2,2,
2,2,2,2,2,2,2,2,2,2,2,2,2,2,2,2,2,2,2,2,2,2,2,2,2,2,2,2,2,2,2,2,2,2,2,2,
2,2,2,2,2,2,2,2,2,2,2,2,2,2,2,2,2,2,2,2,2,2,2,2,2,2,2,2,2,2,2,2,2,2,2,2,
2,2,2,2,2,2,2,2,2,2,2,2,2,2,2,2,2,2,2,2,2,2,2,2,2,2,2,2,2,2,2,2,2,2,2,2,
2,2,2,2,2,2,2,2,2,2,2,2,2,2,2,2,2,2,2,2,2,2,2,2,2,2,2,2,2,2,2,2,2,2,2,2,
2,2,2,2,2,2,2,2,2,2,2,2,2,2,2,2,2,2,2,2,2,2,2,2,2,2,2,2,2,2,2,2,2,2,2,2,
2,2,2,2,2,2,2,2,2,2,2,2,2,2,2,2,2,2,2,2,2,2,2,2,2,2,2,2,2,2,2,2,2,2,2,2,
2,2,2,2,4),(0.0017515687772967,0.138325053356595,0.151276780243772,0.155417338248591,
0.159555236496333,0.162228688491512,0.164324512341607,0.166279619726446,
0.168343676188257,0.171236107367478,0.178859989943288,0.286447337701843,
0.306422960151675,0.337450622805883,0.381798567778655,0.483543771061002,
0.552589452192858,0.587426297663754,0.593869037401524,0.597335588765897,
0.599930739551836,0.602778066778233,0.6078501347858,0.62299837233455,0.88925622396032,
0.966227315679684,0.996167927523107,1.01353649868113,1.01789582511869,1.0200448176947,
1.02229467168772,1.02488615663501,1.02926826985985,1.0450887399084,1.16611709033031,
1.3093237217122,1.36123288072709,1.38592794762347,1.39573370032208,1.40257220206871,
1.40924126413931,1.41795089558398,1.43266333782643,1.55754294091557,1.71762008710786,
1.76930642454278,1.77894991119294,1.78246797805769,1.78458335780597,1.78685804959934,
1.78979118646403,1.79608054282211,1.85896281509135,2.06879091335953,2.19079911093772,
2.20049647818805,2.20459181449844,2.20754914304387,2.21024052938154,2.21383347180757,
2.22257891539509,2.30606328763443,2.40162405827975,2.51628376135754,2.61951894546772,
2.63366657267915,2.63762610262992,2.640028241587,2.64218952728719,2.6449398560019,
2.64929451210425,2.6711444683841,2.76498742292603,2.93502751766293,3.05473296397257,
3.0834464034837,3.09752924238869,3.10880083224543,3.1216989272624,3.14370797869731,
3.26255241531138,3.38249007778415,3.40709068860276,3.42416763503091,3.43135831811938,
3.43636855510755,3.44193711502854,3.45221546534293,3.5018559733613,3.54515239928105,
3.58332661591931,3.61042988000154,3.62352680689319,3.6330475862313,3.64488421775403,
3.66524744499144,3.758830697354,3.80476408814399,3.82956825981784,3.83778725084525,
3.84371036254889,3.85037319087125,3.86168670320928,3.91027566677167,3.9129985584667,
3.91368009540159,3.91779784471794,4.01435332239539,4.06897923977882,4.09050616813681,
4.10696608988951,4.12612287126621,4.19034722147345,4.22948196296821,4.24279877693456,
4.2561098056066,4.28990075193618,4.33635578632061,4.35846208144909,4.37794013402896,
4.39436665437786,4.41509029525811,4.46205924034342,4.487048611373,4.58626846791351,
4.6128945658258,4.63105975539313,4.63905473275387,4.64504281643948,4.65160163012007,
4.66452176213023,4.7205301054893,4.79074110597474,4.81028622731075,4.83668892242472,
4.84969338544162,4.86021928284336,4.87249061078675,4.89446875201819,4.98252906666981,
5.01724332579486,5.03807694217747,5.04612645537648,5.05184511077815,5.05786608123225,
5.0685289742,5.11472989385464,5.23691881353043,5.27772913550408,5.3461004621232,
5.36611083947209,5.37845710219832,5.38984318575178,5.40493041891499,5.43943120713386,
5.62925048650287,5.75652278427547,5.83353688349086,5.83952285080448,5.84242323059355,
5.84449009585872,5.84666379680256,5.84950935941345,5.85557763469844,5.95740276971331,
6.02263446905738,6.10472251589366,6.26147037625291,6.27125445803611,6.27505948910482,
6.27780537262738,6.2807243592377,6.2845956769982,6.29304455380973,6.44850059962419,
6.68156938000003,6.69379067055946,6.69780794539533,6.70004380724059,6.70229680535922,
6.70509137168914,6.71052801700793,6.74742507824072,6.8482799829783,7.03844185882802,
7.06470219409981,7.07492136391038,7.08114810646387,7.08772294922664,7.09591661711547,
7.11211867733351,7.2921261147837,7.34270829555601,7.45286986577465,7.45987475668961,
7.46266516599736,7.46497423176599,7.46732637697601,7.47073288629693,7.47957714845698,
7.51965030796423,7.54473192479103,7.69220648587477,7.86843571804428,7.87949254280103,
7.88350069772908,7.88630163968428,7.88890837742962,7.89247223464457,7.89936987780593,
7.94439721742122,8.05083804224671,8.19808001189696,8.30788654712594,8.31529884038834,
8.31815775804147,8.320213434276,8.32239191784763,8.32526866233631,8.33137560922606,
8.38385747816661,8.44272943600845,8.53370538440831,8.72343406498634,8.75905557155854,
8.77320749174054,8.78477657451478,8.79531839325679,8.81059912094329,8.84893515011331,
8.90440066059995,8.98993905574617,9.02152384109188,9.06993198504814,9.09958347649567,
9.10888413783582,9.11408272678337,9.11876512707595,9.11878073989593,9.11879631953773,
9.11881186501636,9.1188273767727,9.11884285512973,9.11885830041947,9.11887371297768,
9.11888909317892,9.11890444133229,9.11891975775977,9.11893504289695,9.11895029703402,
9.11896552050978,9.11898071368812,9.1189958768656,9.119011010385,9.11902611459777,
9.11904118976973,9.11905623627824,9.11907125448075,9.11908624461243,9.11910120699744,
9.11911614193394,9.11913104967132,9.11914593063062,9.11916078510116,9.11917561337012,
9.11919041571846,9.11920519247744,9.11921994397121,9.11923467049878,9.11924937232786,
9.11926404973785,9.11927870301223,9.11929333243354,9.11930793832082,9.11932252092869,
9.11933708044505,9.11935161719383,9.11936613150718,9.11938062365889,9.11939509398288,
9.11940954269116,9.1194239700672,9.11943837637845,9.11945276187849,9.11946712679392,
9.1194814714212,9.11949579605101,9.11951010091221,9.11952438627004,9.11953865241671,
9.12513615870805,9.13307319168024,9.14667555097134,9.17821235740199,9.26435424754514,
9.290813057662,9.3037988742816,9.31360821167378,9.31384830845949,9.314072301997,
9.31428127100334,9.3144762254085,9.3146581096178,9.31482780594748,9.31498613808514,
9.3151338745275,9.31527173195236,9.31540037847771,9.31552043679201,9.31563248713119,
9.31573707011319,9.31583468940297,9.31592581422803,9.3160108817309,9.31609029918427,
9.31616444604063,9.31628967332175,9.31641312126722,9.31653482283826,9.31665481348598,
9.31677312663185,9.32844945619472,9.35354311887971,9.38726251861441,9.44199029596007,
9.44931792646235,9.50578435580815,9.51596452740012,9.52148073677252,9.52707785530135,
9.53481458275568,9.55287949424507,9.57963179856445,9.68000740471447,9.74617233089887,
9.76659357125358,9.78173234185024,9.79750085548905,9.8152918680815,9.82367586210791,
9.84619224069513,9.90827042514558,9.91839595744867,9.92930854127623,9.94149638644303,
9.96101002456414,10.0154532726687,10.0460807300154,10.0618751072877,10.0772264137265,
10.0932476479946,10.1148962593431,10.2289668597367),.UNSPECIFIED.);
#3185=B_SPLINE_CURVE_WITH_KNOTS('',3,(#162936,#162937,#162938,#162939,#162940,
#162941,#162942,#162943,#162944,#162945,#162946,#162947,#162948,#162949,
#162950,#162951,#162952,#162953,#162954,#162955,#162956,#162957,#162958,
#162959,#162960,#162961,#162962,#162963,#162964,#162965,#162966,#162967,
#162968,#162969,#162970,#162971,#162972,#162973,#162974,#162975,#162976,
#162977,#162978,#162979,#162980,#162981,#162982,#162983,#162984,#162985,
#162986,#162987,#162988,#162989,#162990,#162991,#162992,#162993,#162994,
#162995,#162996,#162997,#162998,#162999,#163000,#163001,#163002,#163003,
#163004,#163005,#163006,#163007,#163008,#163009,#163010,#163011,#163012,
#163013,#163014,#163015,#163016,#163017,#163018,#163019,#163020,#163021,
#163022,#163023,#163024,#163025,#163026,#163027,#163028,#163029,#163030,
#163031,#163032,#163033,#163034,#163035,#163036,#163037,#163038,#163039,
#163040,#163041,#163042,#163043,#163044,#163045,#163046,#163047,#163048,
#163049,#163050,#163051,#163052,#163053,#163054,#163055,#163056,#163057,
#163058,#163059,#163060,#163061,#163062,#163063,#163064,#163065,#163066,
#163067,#163068,#163069,#163070,#163071,#163072,#163073,#163074,#163075,
#163076,#163077,#163078,#163079,#163080,#163081,#163082,#163083,#163084,
#163085,#163086,#163087,#163088,#163089,#163090,#163091,#163092,#163093,
#163094,#163095,#163096,#163097,#163098,#163099,#163100,#163101,#163102,
#163103,#163104,#163105,#163106,#163107,#163108,#163109,#163110,#163111,
#163112,#163113,#163114,#163115,#163116,#163117,#163118,#163119,#163120,
#163121,#163122,#163123,#163124,#163125,#163126,#163127,#163128,#163129,
#163130,#163131,#163132,#163133,#163134,#163135,#163136,#163137,#163138,
#163139,#163140,#163141,#163142,#163143,#163144,#163145,#163146,#163147,
#163148,#163149,#163150,#163151,#163152,#163153,#163154,#163155,#163156,
#163157,#163158,#163159,#163160,#163161,#163162,#163163,#163164,#163165,
#163166,#163167,#163168,#163169,#163170,#163171,#163172,#163173,#163174,
#163175,#163176,#163177,#163178,#163179,#163180,#163181,#163182,#163183,
#163184,#163185,#163186,#163187,#163188,#163189,#163190,#163191,#163192,
#163193,#163194,#163195,#163196,#163197,#163198,#163199,#163200,#163201,
#163202,#163203,#163204,#163205,#163206,#163207,#163208,#163209,#163210,
#163211,#163212,#163213,#163214,#163215,#163216,#163217,#163218,#163219,
#163220,#163221,#163222,#163223,#163224,#163225,#163226,#163227,#163228,
#163229,#163230,#163231,#163232,#163233,#163234,#163235,#163236,#163237,
#163238,#163239,#163240,#163241,#163242,#163243,#163244,#163245,#163246,
#163247,#163248,#163249,#163250,#163251,#163252,#163253,#163254,#163255,
#163256,#163257,#163258,#163259,#163260,#163261,#163262,#163263,#163264,
#163265,#163266,#163267,#163268,#163269,#163270,#163271,#163272,#163273,
#163274,#163275,#163276,#163277,#163278,#163279,#163280,#163281,#163282,
#163283,#163284,#163285,#163286,#163287,#163288,#163289,#163290,#163291,
#163292,#163293,#163294,#163295,#163296,#163297,#163298,#163299,#163300,
#163301,#163302,#163303,#163304,#163305,#163306,#163307,#163308,#163309,
#163310,#163311,#163312,#163313,#163314,#163315,#163316,#163317,#163318,
#163319,#163320,#163321,#163322,#163323,#163324,#163325,#163326,#163327,
#163328,#163329,#163330,#163331,#163332,#163333,#163334,#163335,#163336,
#163337,#163338,#163339,#163340,#163341,#163342,#163343,#163344,#163345,
#163346,#163347,#163348,#163349,#163350,#163351,#163352,#163353,#163354,
#163355,#163356,#163357,#163358,#163359,#163360,#163361,#163362,#163363,
#163364,#163365,#163366,#163367,#163368,#163369,#163370,#163371,#163372,
#163373,#163374,#163375,#163376,#163377,#163378,#163379,#163380,#163381,
#163382,#163383,#163384,#163385,#163386,#163387,#163388,#163389,#163390,
#163391,#163392,#163393,#163394,#163395,#163396,#163397,#163398,#163399,
#163400,#163401,#163402,#163403,#163404,#163405,#163406,#163407,#163408,
#163409,#163410,#163411,#163412,#163413,#163414,#163415,#163416,#163417,
#163418,#163419,#163420,#163421,#163422,#163423,#163424,#163425,#163426,
#163427,#163428,#163429,#163430,#163431,#163432,#163433,#163434,#163435,
#163436,#163437,#163438,#163439,#163440,#163441,#163442,#163443,#163444,
#163445,#163446,#163447,#163448,#163449,#163450,#163451,#163452,#163453,
#163454,#163455,#163456,#163457,#163458,#163459,#163460,#163461,#163462,
#163463,#163464,#163465,#163466,#163467),.UNSPECIFIED.,.F.,.F.,(4,2,2,2,
2,2,2,2,2,2,2,2,2,2,2,2,2,2,2,2,2,2,2,2,2,2,2,2,2,2,2,2,2,2,2,2,2,2,2,2,
2,2,2,2,2,2,2,2,2,2,2,2,2,2,2,2,2,2,2,2,2,2,2,2,2,2,2,2,2,2,2,2,2,2,2,2,
2,2,2,2,2,2,2,2,2,2,2,2,2,2,2,2,2,2,2,2,2,2,2,2,2,2,2,2,2,2,2,2,2,2,2,2,
2,2,2,2,2,2,2,2,2,2,2,2,2,2,2,2,2,2,2,2,2,2,2,2,2,2,2,2,2,2,2,2,2,2,2,2,
2,2,2,2,2,2,2,2,2,2,2,2,2,2,2,2,2,2,2,2,2,2,2,2,2,2,2,2,2,2,2,2,2,2,2,2,
2,2,2,2,2,2,2,2,2,2,2,2,2,2,2,2,2,2,2,2,2,2,2,2,2,2,2,2,2,2,2,2,2,2,2,2,
2,2,2,2,2,2,2,2,2,2,2,2,2,2,2,2,2,2,2,2,2,2,2,2,2,2,2,2,2,2,2,2,2,2,2,2,
2,2,2,2,2,2,2,2,2,4),(0.00102620743934878,0.0700209818904994,0.0806719562036417,
0.0876625602166402,0.0933455982497069,0.0987635694929107,0.10602105163566,
0.118954101730982,0.140940519298676,0.209927368824877,0.268278680050802,
0.290788123848363,0.2919857074657,0.293116341985048,0.29419909489967,0.295251736500306,
0.305095991739884,0.315213759000764,0.328817503760316,0.358985729663482,
0.453055377360456,0.476259475550913,0.487476149288899,0.496530106114982,
0.502362935886591,0.507952479037652,0.514967017977698,0.53441096837326,
0.663378493294355,0.774388809782231,0.808040657082333,0.820068145035925,
0.830549616056012,0.841938577459714,0.856814654914812,0.889668268399421,
1.01781338348057,1.19311357534889,1.25965708118509,1.27850067970099,1.28634410385851,
1.29211690711147,1.2950063661145,1.29718598972696,1.29923650175584,1.30207830880631,
1.30939161247657,1.4341398828131,1.54173678797794,1.71526985075659,1.72379199624076,
1.72767606657096,1.73059608260202,1.73333669055125,1.73712453524325,1.74681126620348,
1.898363775872,1.97547626769385,2.13789994777,2.14630839788965,2.14967966470455,
2.15203770884844,2.15433929067944,2.15710462687996,2.16396246266373,2.23778839586647,
2.48337361210746,2.50425612762181,2.5207052170681,2.52891807390989,2.53551225970664,
2.54167570172066,2.5515628889052,2.57578129448143,2.82408548684629,2.89769158901368,
2.90948589066238,2.9132945898873,2.91573226843855,2.91801364819259,2.92099323901915,
2.92598222351163,2.9596933461137,3.165804822578,3.31929548950605,3.33073917196909,
3.33511641802254,3.33812842403486,3.34107658092285,3.34462635678182,3.35347659320394,
3.43665628113804,3.47789038546963,3.65816755393568,3.75935762839008,3.76648180533531,
3.7695192772212,3.77172386934463,3.77373887638085,3.77644219370254,3.78308977881575,
3.87773376043939,3.99967004399163,4.17758947343506,4.21147312485926,4.22645416308629,
4.23781998571136,4.25020225283901,4.27040312051728,4.34103645665924,4.47438213190967,
4.52334182318996,4.54212774238508,4.55603631215657,4.56266520027506,4.56823060131556,
4.57527433558988,4.58662504521373,4.66167321453443,4.69769899208694,4.73617727699897,
4.75095049247094,4.76168106237837,4.77165913967037,4.78835947139651,4.84062578258731,
4.92440623133414,4.94156425673843,4.96119170028082,4.96876520393286,4.9740885556359,
4.98083171383756,4.99253057159583,5.05847221417962,5.0606767050835,5.11330849752744,
5.15365353057435,5.20049130544304,5.22120477625719,5.23762195018358,5.25708729763257,
5.27917829186422,5.32559172290031,5.35937866830028,5.37268531287157,5.38599123315558,
5.42502051697027,5.48935159506218,5.50848090263054,5.52493354984753,5.54647271440661,
5.60127777609871,5.69860381934907,5.69978175859626,5.75323504073444,5.76473709065591,
5.77143805049514,5.77676619526878,5.78442657528527,5.80469744512164,5.83799372064855,
5.95032276254109,5.97045843955424,5.98224423502657,5.99176770424688,6.00492814241617,
6.03242686949473,6.0714412386122,6.11453656211721,6.16299771366623,6.17319076156436,
6.17874083826709,6.18375076520503,6.1909769334548,6.20828153075202,6.23332523994474,
6.35370862854993,6.47125471359405,6.49319723231978,6.50607591877961,6.51734239045168,
6.53143448628335,6.56022510285602,6.68058966593425,6.8528966158712,6.96245257734062,
6.96914099139685,6.97180617002718,6.97401190368873,6.97625912026927,6.97951427689822,
6.98796906763584,6.99968093921829,7.03286204984243,7.06304267189232,7.2265002485369,
7.39008670450619,7.39998130684094,7.40380293181339,7.40655192432134,7.40946603371027,
7.41331704609155,7.42166713793362,7.55863755388565,7.74705828798871,7.81797439460717,
7.82438517814879,7.827340224763,7.82961719733814,7.8320642948198,7.83552560643319,
7.84588866273015,7.95965297673849,8.03807689306549,8.09222294330772,8.1826611921389,
8.19655832434229,8.2050279646888,8.21165495037634,8.21855984671554,8.22837613678482,
8.23955667813622,8.25950737175954,8.47155694349294,8.58044036235954,8.58744562595582,
8.5902348076198,8.5925423212446,8.59489234334112,8.59796594661942,8.60546728409272,
8.68905625519971,8.776979042251,8.96796635367108,9.0022192860846,9.00838741969961,
9.01213313976895,9.01504124778092,9.0181883553364,9.02318866121053,9.03933031646316,
9.13334434742648,9.2361744062263,9.30498849781451,9.43334371731024,9.44177802167838,
9.44479619338025,9.44689434784662,9.44883783825147,9.4514814362744,9.45655114230102,
9.4879687260255,9.59953843124879,9.69148493559475,9.82745307051558,9.88016251002461,
9.8981974190565,9.90892889271097,9.92035674372422,9.93152864887158,9.94633440437264,
9.97022941381108,10.0186624710519,10.1113075789678,10.1997473077657,10.2233318581722),
 .UNSPECIFIED.);
#3186=B_SPLINE_CURVE_WITH_KNOTS('',3,(#163469,#163470,#163471,#163472,#163473,
#163474,#163475,#163476,#163477,#163478,#163479,#163480,#163481,#163482,
#163483),.UNSPECIFIED.,.F.,.F.,(4,1,1,1,1,1,1,1,1,1,1,1,4),(59.6902604182067,
59.7078879712644,60.206356514572,60.7048250578795,61.2032936011871,61.7017621444946,
62.2002306878022,62.6986992311097,63.6956363177249,64.1941048610324,64.69257340434,
65.6895104909551,65.9734457253863),.UNSPECIFIED.);
#3187=B_SPLINE_CURVE_WITH_KNOTS('',3,(#163485,#163486,#163487,#163488,#163489,
#163490,#163491,#163492,#163493,#163494,#163495,#163496,#163497,#163498,
#163499,#163500,#163501,#163502,#163503,#163504,#163505,#163506,#163507,
#163508,#163509,#163510,#163511,#163512,#163513,#163514,#163515,#163516,
#163517,#163518,#163519,#163520,#163521,#163522,#163523,#163524,#163525,
#163526,#163527,#163528,#163529,#163530,#163531,#163532,#163533,#163534,
#163535,#163536,#163537,#163538,#163539,#163540,#163541,#163542,#163543,
#163544,#163545,#163546,#163547,#163548,#163549,#163550,#163551,#163552,
#163553,#163554,#163555,#163556,#163557,#163558,#163559,#163560,#163561,
#163562,#163563,#163564,#163565,#163566,#163567,#163568,#163569,#163570,
#163571,#163572,#163573,#163574,#163575,#163576,#163577,#163578,#163579,
#163580,#163581,#163582,#163583,#163584,#163585,#163586,#163587,#163588,
#163589,#163590,#163591,#163592,#163593,#163594,#163595,#163596,#163597,
#163598,#163599,#163600,#163601,#163602,#163603,#163604,#163605,#163606,
#163607,#163608,#163609,#163610,#163611,#163612,#163613,#163614,#163615,
#163616,#163617,#163618,#163619,#163620,#163621,#163622,#163623,#163624,
#163625,#163626,#163627,#163628,#163629,#163630,#163631,#163632,#163633,
#163634,#163635,#163636,#163637,#163638,#163639,#163640,#163641,#163642,
#163643,#163644,#163645,#163646,#163647,#163648,#163649,#163650,#163651,
#163652,#163653,#163654,#163655,#163656,#163657,#163658,#163659,#163660,
#163661,#163662,#163663,#163664,#163665,#163666,#163667,#163668,#163669,
#163670,#163671,#163672,#163673,#163674,#163675,#163676,#163677,#163678,
#163679,#163680,#163681,#163682,#163683,#163684,#163685,#163686,#163687,
#163688,#163689,#163690,#163691,#163692,#163693,#163694,#163695,#163696,
#163697,#163698,#163699,#163700,#163701,#163702,#163703,#163704,#163705,
#163706,#163707,#163708,#163709,#163710,#163711,#163712,#163713,#163714,
#163715,#163716,#163717,#163718,#163719,#163720,#163721,#163722,#163723,
#163724,#163725,#163726,#163727,#163728,#163729,#163730,#163731,#163732,
#163733,#163734,#163735,#163736,#163737,#163738,#163739,#163740,#163741,
#163742,#163743),.UNSPECIFIED.,.F.,.F.,(4,3,3,3,3,3,3,3,3,3,3,3,3,3,3,3,
3,3,3,3,3,3,3,3,3,3,3,3,3,3,3,3,3,3,3,3,3,3,3,3,3,3,3,3,3,3,3,3,3,3,3,3,
3,3,3,3,3,3,3,3,3,3,3,3,3,3,3,3,3,3,3,3,3,3,3,3,3,3,3,3,3,3,3,3,3,3,4),
(65.9734457253863,66.0415874873975,66.1097252065017,66.1778850487403,66.1879790342627,
66.2756845236033,66.3638608860217,66.4524652966393,66.541165603522,66.6297618634573,
66.6864475775702,66.7594170220203,66.8323410131141,66.9052325398549,66.9781147387756,
67.0509896568192,67.1238926065293,67.1849161208778,67.2642169048273,67.3435398353038,
67.4228824373142,67.5022555144866,67.581637195484,67.6610339725923,67.6833846641853,
67.7627820588542,67.8421657326823,67.9215331843232,68.0008783681353,68.0802013874019,
68.1594956170233,68.1818532074929,68.2547556077617,68.327635464807,68.4005057342406,
68.4734020786457,68.5463107344307,68.6192790473791,68.6803217508004,68.7688960824135,
68.8575964478861,68.9461632599889,69.0345066735528,69.122276390178,69.178790294108,
69.250113792458,69.3214175426133,69.3927150458857,69.4640475415319,69.5353959002714,
69.6068165552382,69.6772588374156,69.7533623334367,69.8294154795072,69.9054286697423,
69.981412269623,70.0573766229516,70.1344790355865,70.210450763625,70.2864350908839,
70.3624414325567,70.4403800554252,70.5164890948532,70.5953425094419,70.6741959240307,
70.750328796276,70.8263684973471,70.9023245027181,70.9781829452555,71.0539840088092,
71.1297233295435,71.1726644673382,71.248406832161,71.324194952911,71.4000381237537,
71.4759930820135,71.5520095143471,71.6281453098475,71.6711330106458,71.7483084662108,
71.8254087694881,71.902441172545,71.9794128876601,72.0563165758884,72.1331783316029,
72.20999778443,72.2566310325659),.UNSPECIFIED.);
#3188=B_SPLINE_CURVE_WITH_KNOTS('',3,(#163745,#163746,#163747,#163748,#163749,
#163750,#163751,#163752,#163753,#163754,#163755,#163756,#163757,#163758,
#163759,#163760,#163761,#163762,#163763,#163764,#163765,#163766,#163767,
#163768,#163769,#163770,#163771,#163772,#163773,#163774,#163775,#163776,
#163777,#163778,#163779,#163780,#163781,#163782,#163783,#163784,#163785,
#163786,#163787,#163788,#163789,#163790,#163791,#163792,#163793,#163794,
#163795,#163796,#163797,#163798,#163799,#163800,#163801,#163802,#163803,
#163804,#163805,#163806,#163807,#163808,#163809,#163810,#163811,#163812,
#163813,#163814,#163815,#163816,#163817,#163818,#163819,#163820,#163821,
#163822,#163823,#163824,#163825,#163826,#163827,#163828,#163829,#163830,
#163831,#163832,#163833,#163834,#163835,#163836,#163837,#163838,#163839,
#163840,#163841,#163842,#163843,#163844,#163845,#163846,#163847,#163848,
#163849,#163850,#163851,#163852,#163853,#163854,#163855,#163856,#163857,
#163858,#163859,#163860,#163861,#163862,#163863,#163864,#163865,#163866,
#163867,#163868,#163869,#163870,#163871,#163872,#163873,#163874,#163875,
#163876,#163877,#163878,#163879,#163880,#163881,#163882,#163883,#163884,
#163885,#163886,#163887,#163888,#163889,#163890,#163891,#163892,#163893,
#163894,#163895,#163896,#163897,#163898,#163899,#163900,#163901,#163902,
#163903,#163904,#163905,#163906,#163907,#163908,#163909,#163910,#163911,
#163912,#163913,#163914,#163915,#163916,#163917,#163918,#163919,#163920,
#163921,#163922,#163923,#163924,#163925,#163926,#163927,#163928,#163929,
#163930,#163931,#163932,#163933,#163934,#163935,#163936,#163937,#163938,
#163939,#163940,#163941,#163942,#163943,#163944,#163945,#163946,#163947,
#163948,#163949,#163950,#163951,#163952,#163953,#163954,#163955,#163956,
#163957,#163958,#163959,#163960,#163961,#163962,#163963,#163964,#163965,
#163966,#163967,#163968,#163969,#163970,#163971,#163972,#163973,#163974,
#163975,#163976,#163977,#163978,#163979,#163980,#163981,#163982,#163983,
#163984,#163985,#163986,#163987,#163988,#163989,#163990,#163991,#163992,
#163993,#163994,#163995,#163996,#163997,#163998,#163999,#164000),
 .UNSPECIFIED.,.F.,.F.,(4,3,3,3,3,3,3,3,3,3,3,3,3,3,3,3,3,3,3,3,3,3,3,3,
3,3,3,3,3,3,3,3,3,3,3,3,3,3,3,3,3,3,3,3,3,3,3,3,3,3,3,3,3,3,3,3,3,3,3,3,
3,3,3,3,3,3,3,3,3,3,3,3,3,3,3,3,3,3,3,3,3,3,3,3,3,4),(72.2566310326343,
72.341007590014,72.4257777283301,72.510706500726,72.59578785161,72.6680700972609,
72.7394933721108,72.810863499024,72.8821940705451,72.9535074080307,73.024808094853,
73.0961335763454,73.1665386405685,73.2542441299096,73.342420492328,73.4310249029457,
73.5197252098287,73.6083214697641,73.665007183876,73.7379766283261,73.8109006194199,
73.8837921461609,73.9566743450818,74.0295492631251,74.1024522128351,74.1634757271836,
74.242776511133,74.3220994416096,74.4014420436201,74.4808151207924,74.5601968017891,
74.6395935788977,74.6619442704911,74.74134166516,74.8207253389878,74.9000927906292,
74.9794379744413,75.0587609937076,75.1380552233294,75.1604128137987,75.2333152140674,
75.3061950711126,75.3790653405456,75.4519616849508,75.5248703407358,75.5978386536842,
75.6588813571063,75.7474556887191,75.8361560541932,75.924722866296,76.0130662798609,
76.1008359964866,76.1573499004138,76.2286733987638,76.2999771489191,76.371274652191,
76.4426071478373,76.5139555065764,76.5853761615433,76.6558184437214,76.7319219397426,
76.8079750858132,76.8839882760484,76.9599718759296,77.0359362292584,77.1130386418931,
77.1890103699317,77.2649946971906,77.3410010388627,77.4189396617312,77.4950487011589,
77.5739021157477,77.6527555303365,77.7288884025816,77.8049281036525,77.8808841090234,
77.9567425515606,78.0325436151146,78.108282935849,78.151224073644,78.2243297162825,
78.2974563861152,78.3706483030038,78.4438786071505,78.517191606161,78.5398163397455),
 .UNSPECIFIED.);
#3189=B_SPLINE_CURVE_WITH_KNOTS('',3,(#164002,#164003,#164004,#164005,#164006,
#164007,#164008,#164009,#164010,#164011,#164012,#164013,#164014,#164015,
#164016),.UNSPECIFIED.,.F.,.F.,(4,1,1,1,1,1,1,1,1,1,1,1,4),(78.5398163397455,
78.6496926169516,79.6466297035667,80.1450982468743,80.6435667901818,81.1420353334894,
81.6405038767969,82.1389724201045,82.6374409634121,83.1359095067196,83.6343780500272,
84.6313151366423,84.8230016469251),.UNSPECIFIED.);
#3190=B_SPLINE_CURVE_WITH_KNOTS('',3,(#164018,#164019,#164020,#164021,#164022,
#164023,#164024,#164025,#164026,#164027,#164028,#164029,#164030,#164031,
#164032,#164033,#164034,#164035,#164036,#164037,#164038,#164039,#164040,
#164041,#164042,#164043,#164044,#164045,#164046,#164047,#164048,#164049,
#164050,#164051,#164052,#164053,#164054,#164055,#164056,#164057,#164058,
#164059,#164060,#164061,#164062,#164063,#164064,#164065,#164066,#164067,
#164068,#164069,#164070,#164071,#164072,#164073,#164074,#164075,#164076,
#164077,#164078,#164079,#164080,#164081,#164082,#164083,#164084,#164085,
#164086,#164087,#164088,#164089,#164090,#164091,#164092,#164093,#164094,
#164095,#164096,#164097,#164098,#164099,#164100,#164101,#164102,#164103,
#164104,#164105,#164106,#164107,#164108,#164109,#164110,#164111,#164112,
#164113,#164114,#164115,#164116,#164117,#164118,#164119,#164120,#164121,
#164122,#164123,#164124,#164125,#164126,#164127,#164128,#164129,#164130,
#164131,#164132,#164133,#164134,#164135,#164136,#164137,#164138,#164139,
#164140,#164141,#164142,#164143,#164144,#164145,#164146,#164147,#164148,
#164149,#164150,#164151,#164152,#164153,#164154,#164155,#164156,#164157,
#164158,#164159,#164160,#164161,#164162,#164163,#164164,#164165,#164166,
#164167,#164168,#164169,#164170,#164171,#164172,#164173,#164174,#164175,
#164176,#164177,#164178,#164179,#164180,#164181,#164182,#164183,#164184,
#164185,#164186,#164187,#164188,#164189,#164190,#164191,#164192,#164193,
#164194,#164195,#164196,#164197,#164198,#164199,#164200,#164201,#164202,
#164203,#164204,#164205,#164206,#164207,#164208,#164209,#164210,#164211,
#164212,#164213,#164214,#164215,#164216,#164217,#164218,#164219,#164220,
#164221,#164222,#164223,#164224,#164225,#164226,#164227,#164228,#164229,
#164230,#164231,#164232,#164233,#164234,#164235,#164236,#164237,#164238,
#164239,#164240,#164241,#164242,#164243,#164244,#164245,#164246,#164247,
#164248,#164249,#164250,#164251,#164252,#164253,#164254,#164255,#164256,
#164257,#164258,#164259,#164260,#164261,#164262,#164263,#164264,#164265,
#164266,#164267,#164268,#164269,#164270,#164271,#164272,#164273),
 .UNSPECIFIED.,.F.,.F.,(4,3,3,3,3,3,3,3,3,3,3,3,3,3,3,3,3,3,3,3,3,3,3,3,
3,3,3,3,3,3,3,3,3,3,3,3,3,3,3,3,3,3,3,3,3,3,3,3,3,3,3,3,3,3,3,3,3,3,3,3,
3,3,3,3,3,3,3,3,3,3,3,3,3,3,3,3,3,3,3,3,3,3,3,3,3,4),(84.8230016469251,
84.8950329886772,84.9670035295852,85.0389391630576,85.1108531641058,85.1297836799499,
85.2055260447726,85.2813141655222,85.3571573363646,85.4331122946245,85.5091287269584,
85.5852645224588,85.6282522232574,85.7044628037309,85.780605407983,85.8566904943232,
85.9327284805954,86.0087297511505,86.0857871959908,86.1617524581157,86.2377140499803,
86.3136813770418,86.3915583602494,86.467588157682,86.5463887337772,86.6251893098725,
86.6966125847225,86.7679827116359,86.8393132831573,86.9106266206429,86.9819273074649,
87.0532527889575,87.1236578531801,87.2113633425206,87.2995397049393,87.3881441155568,
87.4768444224396,87.5654406823742,87.6221263964876,87.6950958409377,87.7680198320316,
87.8409113587729,87.9137935576939,87.9866684757374,88.0595714254476,88.1205949397952,
88.1998957237444,88.2792186542207,88.3585612562308,88.4379343334031,88.5173160144004,
88.5967127915087,88.6190634831028,88.6984608777717,88.7778445516,88.8572120032418,
88.936557187054,89.0158802063202,89.0951744359419,89.1175320264103,89.190434426679,
89.2633142837243,89.3361845531575,89.4090808975625,89.4819895533475,89.554957866296,
89.6160005697179,89.7045749013317,89.793275266806,89.8818420789087,89.9701854924737,
90.0579552090997,90.1144691130254,90.1857926113755,90.257096361531,90.3283938648039,
90.3997263604502,90.4710747191896,90.5424953741565,90.612937656333,90.6939127385888,
90.7748258176601,90.8576659473002,90.9383778712841,91.0222821037523,91.1061863362205),
 .UNSPECIFIED.);
#3191=B_SPLINE_CURVE_WITH_KNOTS('',3,(#164275,#164276,#164277,#164278,#164279,
#164280,#164281,#164282,#164283,#164284,#164285,#164286,#164287,#164288,
#164289,#164290,#164291,#164292,#164293,#164294,#164295,#164296,#164297,
#164298,#164299,#164300,#164301,#164302,#164303,#164304,#164305,#164306,
#164307,#164308,#164309,#164310,#164311,#164312,#164313,#164314,#164315,
#164316,#164317,#164318,#164319,#164320,#164321,#164322,#164323,#164324,
#164325,#164326,#164327,#164328,#164329,#164330,#164331,#164332,#164333,
#164334,#164335,#164336,#164337,#164338,#164339,#164340,#164341,#164342,
#164343,#164344,#164345,#164346,#164347,#164348,#164349,#164350,#164351,
#164352,#164353,#164354,#164355,#164356,#164357,#164358,#164359,#164360,
#164361,#164362,#164363,#164364,#164365,#164366,#164367,#164368,#164369,
#164370,#164371,#164372,#164373,#164374,#164375,#164376,#164377,#164378,
#164379,#164380,#164381,#164382,#164383,#164384,#164385,#164386,#164387,
#164388,#164389,#164390,#164391,#164392,#164393,#164394,#164395,#164396,
#164397,#164398,#164399,#164400,#164401,#164402,#164403,#164404,#164405,
#164406,#164407,#164408,#164409,#164410,#164411,#164412,#164413,#164414,
#164415,#164416,#164417,#164418,#164419,#164420,#164421,#164422,#164423,
#164424,#164425,#164426,#164427,#164428,#164429,#164430,#164431,#164432,
#164433,#164434,#164435,#164436,#164437,#164438,#164439,#164440,#164441,
#164442,#164443,#164444,#164445,#164446,#164447,#164448,#164449,#164450,
#164451,#164452,#164453,#164454,#164455,#164456,#164457,#164458,#164459,
#164460,#164461,#164462,#164463,#164464,#164465,#164466,#164467,#164468,
#164469,#164470,#164471,#164472,#164473,#164474,#164475,#164476,#164477,
#164478,#164479,#164480,#164481,#164482,#164483,#164484,#164485,#164486,
#164487,#164488,#164489,#164490,#164491,#164492,#164493,#164494,#164495,
#164496,#164497,#164498,#164499,#164500,#164501,#164502,#164503,#164504,
#164505,#164506,#164507,#164508,#164509,#164510,#164511,#164512,#164513,
#164514,#164515,#164516,#164517,#164518,#164519,#164520,#164521,#164522,
#164523,#164524,#164525,#164526,#164527,#164528,#164529,#164530,#164531,
#164532,#164533),.UNSPECIFIED.,.F.,.F.,(4,3,3,3,3,3,3,3,3,3,3,3,3,3,3,3,
3,3,3,3,3,3,3,3,3,3,3,3,3,3,3,3,3,3,3,3,3,3,3,3,3,3,3,3,3,3,3,3,3,3,3,3,
3,3,3,3,3,3,3,3,3,3,3,3,3,3,3,3,3,3,3,3,3,3,3,3,3,3,3,3,3,3,3,3,3,3,4),
(91.1061869541046,91.185072039433,91.2640500284989,91.3431199147297,91.4223307290269,
91.501614799976,91.5810109127831,91.6098747429481,91.6860076151932,91.7620473162646,
91.8380033216353,91.9138617641726,91.9896628277263,92.0654021484602,92.1083432862557,
92.1840856510784,92.2598737718279,92.3357169426699,92.4116719009298,92.487688333264,
92.5638241287644,92.6068118295632,92.6830224100368,92.7591650142889,92.8352501006293,
92.9112880869015,92.9872893574565,93.0643468022967,93.1403120644216,93.2162736562862,
93.2922409833475,93.3701179665552,93.4461477639878,93.5249483400831,93.6037489161783,
93.6751721910282,93.7465423179415,93.8178728894628,93.8891862269484,93.9604869137707,
94.0318123952632,94.1022174594859,94.1899229488263,94.2780993112448,94.3667037218623,
94.455404028745,94.5440002886799,94.6006860027935,94.6736554472436,94.7465794383374,
94.8194709650783,94.8923531639992,94.9652280820427,95.0381310317529,95.099154546101,
95.1784553300503,95.2577782605266,95.3371208625367,95.416493939709,95.495875620706,
95.5752723978145,95.5976230894086,95.6770204840775,95.7564041579055,95.8357716095462,
95.9151167933585,95.9944398126247,96.0737340422464,96.0960916327161,96.1689940329847,
96.24187389003,96.3147441594632,96.3876405038683,96.4605491596532,96.5335174726015,
96.5945601760237,96.6831345076366,96.7718348731101,96.8604016852129,96.9487450987768,
97.0365148154024,97.0930287193312,97.1614881029375,97.229931937027,97.2983663514909,
97.3668185260313,97.3893722612842),.UNSPECIFIED.);
#3192=B_SPLINE_CURVE_WITH_KNOTS('',3,(#164535,#164536,#164537,#164538,#164539,
#164540,#164541,#164542,#164543,#164544,#164545,#164546,#164547,#164548,
#164549,#164550,#164551,#164552,#164553,#164554,#164555,#164556,#164557,
#164558,#164559,#164560,#164561,#164562,#164563,#164564,#164565,#164566,
#164567,#164568,#164569,#164570,#164571,#164572,#164573,#164574,#164575,
#164576,#164577,#164578,#164579,#164580,#164581,#164582,#164583,#164584,
#164585,#164586,#164587,#164588,#164589,#164590,#164591,#164592,#164593,
#164594,#164595,#164596,#164597,#164598,#164599,#164600,#164601,#164602,
#164603,#164604,#164605,#164606,#164607,#164608,#164609,#164610,#164611,
#164612,#164613,#164614,#164615,#164616,#164617,#164618,#164619,#164620,
#164621,#164622,#164623,#164624,#164625,#164626,#164627,#164628,#164629,
#164630,#164631,#164632,#164633,#164634,#164635,#164636,#164637,#164638,
#164639,#164640,#164641,#164642,#164643,#164644,#164645,#164646,#164647,
#164648,#164649,#164650,#164651,#164652,#164653,#164654,#164655,#164656,
#164657,#164658,#164659,#164660,#164661,#164662,#164663,#164664,#164665,
#164666,#164667,#164668,#164669,#164670,#164671,#164672,#164673,#164674,
#164675,#164676,#164677,#164678,#164679,#164680,#164681,#164682,#164683,
#164684,#164685,#164686,#164687,#164688,#164689,#164690,#164691,#164692,
#164693,#164694,#164695,#164696,#164697,#164698,#164699,#164700,#164701,
#164702,#164703,#164704,#164705,#164706,#164707,#164708,#164709,#164710,
#164711,#164712,#164713,#164714,#164715,#164716,#164717,#164718,#164719,
#164720,#164721,#164722,#164723,#164724,#164725,#164726,#164727,#164728,
#164729,#164730,#164731,#164732,#164733,#164734,#164735,#164736,#164737,
#164738,#164739,#164740,#164741,#164742,#164743,#164744,#164745,#164746,
#164747,#164748,#164749,#164750,#164751,#164752,#164753,#164754,#164755,
#164756,#164757,#164758,#164759,#164760,#164761,#164762,#164763,#164764,
#164765,#164766,#164767,#164768,#164769,#164770,#164771,#164772,#164773,
#164774,#164775,#164776,#164777,#164778,#164779,#164780,#164781,#164782,
#164783,#164784,#164785,#164786,#164787,#164788,#164789,#164790,#164791,
#164792,#164793,#164794,#164795,#164796,#164797,#164798,#164799,#164800,
#164801,#164802,#164803,#164804,#164805,#164806,#164807,#164808,#164809,
#164810,#164811,#164812,#164813,#164814,#164815,#164816,#164817,#164818,
#164819,#164820,#164821,#164822,#164823,#164824,#164825,#164826,#164827,
#164828,#164829,#164830,#164831,#164832,#164833,#164834,#164835,#164836,
#164837,#164838,#164839,#164840,#164841,#164842,#164843,#164844,#164845,
#164846,#164847,#164848,#164849,#164850,#164851,#164852,#164853,#164854,
#164855,#164856,#164857,#164858,#164859,#164860,#164861,#164862,#164863,
#164864,#164865,#164866,#164867,#164868,#164869,#164870,#164871,#164872,
#164873,#164874,#164875,#164876,#164877,#164878,#164879,#164880,#164881,
#164882,#164883,#164884,#164885,#164886,#164887,#164888,#164889,#164890,
#164891,#164892,#164893,#164894,#164895,#164896,#164897,#164898,#164899,
#164900,#164901,#164902,#164903,#164904,#164905,#164906,#164907,#164908,
#164909,#164910,#164911,#164912,#164913,#164914,#164915,#164916,#164917,
#164918,#164919,#164920,#164921,#164922,#164923,#164924,#164925,#164926,
#164927,#164928,#164929,#164930,#164931,#164932,#164933,#164934,#164935,
#164936,#164937,#164938,#164939,#164940,#164941,#164942,#164943,#164944,
#164945,#164946,#164947,#164948,#164949,#164950,#164951,#164952,#164953,
#164954,#164955,#164956,#164957,#164958,#164959,#164960,#164961,#164962,
#164963,#164964,#164965,#164966,#164967,#164968,#164969,#164970,#164971,
#164972,#164973,#164974,#164975,#164976,#164977,#164978,#164979,#164980,
#164981,#164982,#164983,#164984,#164985,#164986,#164987,#164988,#164989,
#164990,#164991,#164992,#164993,#164994,#164995,#164996,#164997,#164998,
#164999,#165000,#165001,#165002,#165003,#165004,#165005,#165006,#165007,
#165008,#165009,#165010,#165011,#165012,#165013,#165014,#165015,#165016,
#165017,#165018,#165019,#165020,#165021,#165022,#165023,#165024,#165025,
#165026,#165027,#165028,#165029,#165030,#165031,#165032,#165033,#165034,
#165035,#165036,#165037,#165038,#165039,#165040,#165041,#165042,#165043,
#165044,#165045,#165046,#165047,#165048,#165049,#165050,#165051,#165052,
#165053,#165054,#165055,#165056,#165057,#165058,#165059,#165060,#165061,
#165062,#165063,#165064,#165065,#165066,#165067,#165068,#165069,#165070,
#165071,#165072,#165073,#165074,#165075,#165076,#165077,#165078,#165079,
#165080,#165081,#165082,#165083,#165084,#165085,#165086,#165087,#165088,
#165089,#165090,#165091,#165092,#165093,#165094,#165095,#165096,#165097,
#165098,#165099,#165100,#165101,#165102,#165103,#165104,#165105,#165106,
#165107,#165108,#165109,#165110,#165111,#165112,#165113,#165114,#165115,
#165116,#165117,#165118,#165119,#165120,#165121,#165122,#165123,#165124,
#165125,#165126,#165127,#165128,#165129,#165130,#165131,#165132,#165133,
#165134,#165135,#165136,#165137,#165138,#165139,#165140,#165141,#165142,
#165143,#165144,#165145,#165146,#165147,#165148,#165149,#165150,#165151,
#165152,#165153,#165154,#165155,#165156,#165157,#165158,#165159,#165160,
#165161,#165162,#165163,#165164,#165165,#165166,#165167,#165168,#165169,
#165170,#165171,#165172,#165173,#165174,#165175,#165176,#165177,#165178,
#165179,#165180,#165181,#165182,#165183,#165184,#165185,#165186,#165187,
#165188,#165189,#165190,#165191,#165192,#165193,#165194,#165195,#165196,
#165197,#165198,#165199,#165200,#165201,#165202,#165203,#165204,#165205,
#165206,#165207,#165208,#165209,#165210,#165211,#165212,#165213,#165214,
#165215,#165216,#165217,#165218,#165219,#165220,#165221,#165222,#165223,
#165224,#165225,#165226,#165227,#165228,#165229,#165230,#165231,#165232,
#165233,#165234,#165235,#165236,#165237,#165238,#165239,#165240,#165241,
#165242,#165243,#165244,#165245,#165246,#165247,#165248,#165249,#165250,
#165251,#165252,#165253,#165254,#165255,#165256,#165257,#165258),
 .UNSPECIFIED.,.F.,.F.,(4,2,2,2,2,2,2,2,2,2,2,2,2,2,2,2,2,2,2,2,2,2,2,2,
2,2,2,2,2,2,2,2,2,2,2,2,2,2,2,2,2,2,2,2,2,2,2,2,2,2,2,2,2,2,2,2,2,2,2,2,
2,2,2,2,2,2,2,2,2,2,2,2,2,2,2,2,2,2,2,2,2,2,2,2,2,2,2,2,2,2,2,2,2,2,2,2,
2,2,2,2,2,2,2,2,2,2,2,2,2,2,2,2,2,2,2,2,2,2,2,2,2,2,2,2,2,2,2,2,2,2,2,2,
2,2,2,2,2,2,2,2,2,2,2,2,2,2,2,2,2,2,2,2,2,2,2,2,2,2,2,2,2,2,2,2,2,2,2,2,
2,2,2,2,2,2,2,2,2,2,2,2,2,2,2,2,2,2,2,2,2,2,2,2,2,2,2,2,2,2,2,2,2,2,2,2,
2,2,2,2,2,2,2,2,2,2,2,2,2,2,2,2,2,2,2,2,2,2,2,2,2,2,2,2,2,2,2,2,2,2,2,2,
2,2,2,2,2,2,2,2,2,2,2,2,2,2,2,2,2,2,2,2,2,2,2,2,2,2,2,2,2,2,2,2,2,2,2,2,
2,2,2,2,2,2,2,2,2,2,2,2,2,2,2,2,2,2,2,2,2,2,2,2,2,2,2,2,2,2,2,2,2,2,2,2,
2,2,2,2,2,2,2,2,2,2,2,2,2,2,2,2,2,2,2,2,2,2,2,2,2,2,2,2,2,2,2,2,2,2,2,2,
2,2,2,2,2,2,2,2,2,2,2,2,2,4),(0.00175068145111175,0.134011030493767,0.138634978208069,
0.141510891536465,0.143675177905201,0.145865861977993,0.147898128219227,
0.150670147329979,0.156128791954469,0.218904577978021,0.253373337729684,
0.271399628962356,0.297726024991574,0.334632242767568,0.409083717063428,
0.520385324309226,0.566345440885185,0.573275583049934,0.576845253459886,
0.579699806871459,0.58255545909305,0.587669036857107,0.603126833170253,
0.870804313282468,0.927422269494703,0.970581617958302,0.984891875418743,
0.994813470394621,0.998399463628681,1.00049902275691,1.00276556583873,1.00569105443112,
1.01177742507548,1.05391356569697,1.18009633810029,1.28059991335028,1.33131231686721,
1.36347352356323,1.37424075320674,1.38127739511405,1.38786128432668,1.39614134393183,
1.4090925899202,1.47859786697299,1.49115523764654,1.55871838182118,1.6400507016171,
1.74326408493459,1.75266721674397,1.75746543472939,1.76146386785603,1.76392991606873,
1.76618948797032,1.76905778140773,1.77485609804717,1.8161320534101,1.82162002368309,
2.04722862911486,2.1596758369333,2.17763716594957,2.18283861950859,2.18603146184098,
2.18892818775009,2.19264720187391,2.19859053660356,2.22922431720825,2.44839371798544,
2.60656799284768,2.61498176304512,2.61823132686803,2.62047799114371,2.62268579227223,
2.62535664959904,2.63207631729564,2.73650099359328,2.91260834049862,3.03413896399209,
3.06308463758117,3.07720865049273,3.08848150615735,3.10134686954032,3.12321606461796,
3.23928404073321,3.36047347272984,3.38606706105148,3.40365638652497,3.41093121471606,
3.41647669150467,3.42301926965352,3.43471750094256,3.50662769021987,3.58033457861406,
3.5974510175504,3.60861788776679,3.61933499877933,3.63222294110174,3.66402302370758,
3.71871540548264,3.77935003739452,3.79899838570045,3.81301678758811,3.81975196395409,
3.82569940995075,3.83341569211323,3.8461781803915,3.95715492100013,4.00589566204327,
4.05167656332163,4.07205957561714,4.08830035182536,4.10831338891101,4.15752195595253,
4.19208659720518,4.20272163769428,4.2186851683656,4.23070700122613,4.24812676325788,
4.304461625542,4.32279881912596,4.34879086999873,4.36569829043325,4.38118536310892,
4.408006893285,4.54680592976487,4.58521538376171,4.60130133424854,4.61380268457729,
4.62071771357805,4.62661544059658,4.63413770759333,4.651631668965,4.72859306163979,
4.7794707745708,4.81290323013672,4.82706741833238,4.83771048242841,4.84786367479352,
4.86553244870683,4.96137711464545,4.99648683212428,5.01746876894224,5.02553781623566,
5.03125923032708,5.03651959628616,5.04622401050655,5.07989689879688,5.1142738476073,
5.25314698952696,5.25623071551449,5.32536953398259,5.34544566715934,5.35780433808763,
5.3691832859131,5.38423334506416,5.41851704874251,5.60387741343003,5.73060722271663,
5.81277345713204,5.81945616133057,5.82212094555868,5.82432708718931,5.82657546245093,
5.82983364060598,5.83830374223236,5.87559417485033,5.91338366008016,6.0012139475115,
6.08349114031398,6.240631152834,6.2504149007525,6.25421925360012,6.25696445981735,
6.25988255228077,6.26375238830769,6.27219685741442,6.42713990792728,6.6605772612252,
6.67282472533302,6.67684477474014,6.67908078752245,6.68133302228001,6.68412526920551,
6.68955304243106,6.72623012148463,6.82397060594503,6.89647081849563,7.03199979411896,
7.0482913028952,7.05661375056243,7.06320297248004,7.07022130004281,7.08090257149064,
7.11293058485085,7.35812291436516,7.43204235528481,7.43890392114801,7.44167055307541,
7.44397312791639,7.44633210338918,7.44977302276103,7.45884511930544,7.50066991308049,
7.52835637967532,7.672750589987,7.84764417394031,7.85846618543644,7.86243744503269,
7.86522796872251,7.86783721604346,7.871423425317,7.87843012943556,7.92648394749109,
7.98435140079447,8.17240102025664,8.28706847158256,8.2942807017657,8.29710619189759,
8.29915282949482,8.30133570215935,8.30424206064701,8.31050513071682,8.36196508622292,
8.42013957513948,8.51054999994118,8.61358515036602,8.71226959267471,8.74173865690321,
8.75595991399811,8.76724262799249,8.77777254733366,8.79268411751894,8.83872658224809,
8.91210064491931,8.98107778509443,9.03942084606236,9.07690281967958,9.086896578827,
9.09220420910962,9.09722913784367,9.09724523595471,9.09726129654262,9.09727732001483,
9.09729330669885,9.09730925702172,9.09732517135649,9.09734105008431,9.09735689363703,
9.09737270235281,9.09738847657413,9.09740421675583,9.09741992323606,9.09743559638129,
9.09745123648668,9.09746684401147,9.09748241923962,9.09749796253769,9.09751347432227,
9.09752895492289,9.09754440468476,9.09755982394042,9.09757521304138,9.0975905722994,
9.09760590207696,9.0976212027568,9.09763647458273,9.09765171789646,9.09766693304972,
9.09768212034341,9.09769728004803,9.09771241261139,9.09772751835617,9.0977425975128,
9.09775765037659,9.09777267726359,9.09778767853363,9.09780265453569,9.09781760558654,
9.0978325319059,9.09784743384839,9.09786231166902,9.09787716567843,9.09789199612518,
9.0979068033323,9.0979215876016,9.09793634923074,9.09795108847808,9.09796580564063,
9.09798050103171,9.09799517490246,9.09800982753272,9.09802445926074,9.09803907028262,
9.09805366090144,9.09806823138489,9.09808278196589,9.0980973129296,9.09811182454834,
9.098126317194,9.09814079107453,9.09815524636716,9.09816968342256,9.10376770015621,
9.11170544754015,9.12531173155767,9.15686879604102,9.254550635845,9.27408438484564,
9.28574103015298,9.29592948071053,9.29603839081233,9.29614580743692,9.29625175834067,
9.29635627070302,9.29645937111086,9.29656108559078,9.29666143961484,9.29676045811431,
9.29685816547961,9.29695458558435,9.31092411781765,9.34412631179128,9.39483863365628,
9.47158465277903,9.48944448302903,9.49702740511677,9.50260413151457,9.50891371067642,
9.50895489382347,9.50899621336665,9.50903767187097,9.50907927213511,9.50912101701083,
9.50916290933531,9.50920495196572,9.50924714778553,9.50928949974651,9.50933201081573,
9.50937468394175,9.52063607473001,9.53505424093766,9.56737159552485,9.63207094206619,
9.67801527753326,9.71864187171298,9.74401598578509,9.75928174231616,9.77510754230476,
9.79264076242029,9.80201134648943,9.82507503155774,9.88661125776569,9.89686058377307,
9.90774692212002,9.91994448989332,9.93949531280475,9.99424684689922,10.0246091225099,
10.0403705671353,10.0557025297082,10.0717420470211,10.0934521740875,10.2275071693496),
 .UNSPECIFIED.);
#3193=B_SPLINE_CURVE_WITH_KNOTS('',3,(#165260,#165261,#165262,#165263,#165264,
#165265,#165266,#165267,#165268,#165269,#165270,#165271,#165272,#165273,
#165274,#165275,#165276,#165277,#165278,#165279,#165280,#165281,#165282,
#165283,#165284,#165285,#165286,#165287,#165288,#165289,#165290,#165291,
#165292,#165293,#165294,#165295,#165296,#165297,#165298,#165299,#165300,
#165301,#165302,#165303,#165304,#165305,#165306,#165307,#165308,#165309,
#165310,#165311,#165312,#165313,#165314,#165315,#165316,#165317,#165318,
#165319,#165320,#165321,#165322,#165323,#165324,#165325,#165326,#165327,
#165328,#165329,#165330,#165331,#165332,#165333,#165334,#165335,#165336,
#165337,#165338,#165339,#165340,#165341,#165342,#165343,#165344,#165345,
#165346,#165347,#165348,#165349,#165350,#165351,#165352,#165353,#165354,
#165355,#165356,#165357,#165358,#165359,#165360,#165361,#165362,#165363,
#165364,#165365,#165366,#165367,#165368,#165369,#165370,#165371,#165372,
#165373,#165374,#165375,#165376,#165377,#165378,#165379,#165380,#165381,
#165382,#165383,#165384,#165385,#165386,#165387,#165388,#165389,#165390,
#165391,#165392,#165393,#165394,#165395,#165396,#165397,#165398,#165399,
#165400,#165401,#165402,#165403,#165404,#165405,#165406,#165407,#165408,
#165409,#165410,#165411,#165412,#165413,#165414,#165415,#165416,#165417,
#165418,#165419,#165420,#165421,#165422,#165423,#165424,#165425,#165426,
#165427,#165428,#165429,#165430,#165431,#165432,#165433,#165434,#165435,
#165436,#165437,#165438,#165439,#165440,#165441,#165442,#165443,#165444,
#165445,#165446,#165447,#165448,#165449,#165450,#165451,#165452,#165453,
#165454,#165455,#165456,#165457,#165458,#165459,#165460,#165461,#165462,
#165463,#165464,#165465,#165466,#165467,#165468,#165469,#165470,#165471,
#165472,#165473,#165474,#165475,#165476,#165477,#165478,#165479,#165480,
#165481,#165482,#165483,#165484,#165485,#165486,#165487,#165488,#165489,
#165490,#165491,#165492,#165493,#165494,#165495,#165496,#165497,#165498,
#165499,#165500,#165501,#165502,#165503,#165504,#165505,#165506,#165507,
#165508,#165509,#165510,#165511,#165512,#165513,#165514,#165515,#165516,
#165517,#165518,#165519,#165520,#165521,#165522,#165523,#165524,#165525,
#165526,#165527,#165528,#165529,#165530,#165531,#165532,#165533,#165534,
#165535,#165536,#165537,#165538,#165539,#165540,#165541,#165542,#165543,
#165544,#165545,#165546,#165547,#165548,#165549,#165550,#165551,#165552,
#165553,#165554,#165555,#165556,#165557,#165558,#165559,#165560,#165561,
#165562,#165563,#165564,#165565,#165566,#165567,#165568,#165569,#165570,
#165571,#165572,#165573,#165574,#165575,#165576,#165577,#165578,#165579,
#165580,#165581,#165582,#165583,#165584,#165585,#165586,#165587,#165588,
#165589,#165590,#165591,#165592,#165593,#165594,#165595,#165596,#165597,
#165598,#165599,#165600,#165601,#165602,#165603,#165604,#165605,#165606,
#165607,#165608,#165609,#165610,#165611,#165612,#165613,#165614,#165615,
#165616,#165617,#165618,#165619,#165620,#165621,#165622,#165623,#165624,
#165625,#165626,#165627,#165628,#165629,#165630,#165631,#165632,#165633,
#165634,#165635,#165636,#165637,#165638,#165639,#165640,#165641,#165642,
#165643,#165644,#165645,#165646,#165647,#165648,#165649,#165650,#165651,
#165652,#165653,#165654,#165655,#165656,#165657,#165658,#165659,#165660,
#165661,#165662,#165663,#165664,#165665,#165666,#165667,#165668,#165669,
#165670,#165671,#165672,#165673,#165674,#165675,#165676,#165677,#165678,
#165679,#165680,#165681,#165682,#165683,#165684,#165685,#165686,#165687,
#165688,#165689,#165690,#165691,#165692,#165693,#165694,#165695,#165696,
#165697,#165698,#165699,#165700,#165701,#165702,#165703,#165704,#165705,
#165706,#165707,#165708,#165709,#165710,#165711,#165712,#165713,#165714,
#165715,#165716,#165717,#165718,#165719,#165720,#165721,#165722,#165723,
#165724,#165725,#165726,#165727,#165728,#165729,#165730,#165731,#165732,
#165733,#165734,#165735,#165736,#165737,#165738,#165739,#165740,#165741,
#165742,#165743,#165744,#165745,#165746,#165747,#165748,#165749,#165750,
#165751,#165752,#165753,#165754,#165755,#165756,#165757,#165758,#165759,
#165760,#165761,#165762,#165763,#165764,#165765,#165766,#165767,#165768,
#165769,#165770,#165771,#165772,#165773,#165774,#165775,#165776,#165777,
#165778,#165779,#165780,#165781,#165782,#165783,#165784,#165785,#165786,
#165787,#165788,#165789,#165790,#165791,#165792,#165793,#165794,#165795,
#165796,#165797,#165798,#165799,#165800,#165801),.UNSPECIFIED.,.F.,.F.,
(4,2,2,2,2,2,2,2,2,2,2,2,2,2,2,2,2,2,2,2,2,2,2,2,2,2,2,2,2,2,2,2,2,2,2,
2,2,2,2,2,2,2,2,2,2,2,2,2,2,2,2,2,2,2,2,2,2,2,2,2,2,2,2,2,2,2,2,2,2,2,2,
2,2,2,2,2,2,2,2,2,2,2,2,2,2,2,2,2,2,2,2,2,2,2,2,2,2,2,2,2,2,2,2,2,2,2,2,
2,2,2,2,2,2,2,2,2,2,2,2,2,2,2,2,2,2,2,2,2,2,2,2,2,2,2,2,2,2,2,2,2,2,2,2,
2,2,2,2,2,2,2,2,2,2,2,2,2,2,2,2,2,2,2,2,2,2,2,2,2,2,2,2,2,2,2,2,2,2,2,2,
2,2,2,2,2,2,2,2,2,2,2,2,2,2,2,2,2,2,2,2,2,2,2,2,2,2,2,2,2,2,2,2,2,2,2,2,
2,2,2,2,2,2,2,2,2,2,2,2,2,2,2,2,2,2,2,2,2,2,2,2,2,2,2,2,2,2,2,2,2,2,2,2,
2,2,2,2,2,2,2,2,2,2,2,2,2,2,2,2,2,2,2,4),(0.00186199683268441,0.0535642282285645,
0.0630877328723694,0.0696351131693898,0.0752500213517179,0.0811989772806776,
0.088362912300289,0.10908685004617,0.119623293193971,0.201548095287269,
0.244189440712299,0.269675950580021,0.280137626972409,0.290169430701876,
0.300137816356626,0.31678381431195,0.369057831022039,0.37083408155873,0.431445777403261,
0.455973952503189,0.467595688565333,0.476972384577673,0.482457599612003,
0.487927247505554,0.494527592164464,0.510720097351574,0.617630405419689,
0.65911088494058,0.767015788711514,0.792505078442363,0.803780297652384,
0.81526496408748,0.825913352571771,0.840603391281476,0.880582300677057,
1.00281431820652,1.161471926301,1.23740230070852,1.25803714022971,1.26641154476457,
1.27265338125613,1.27554861976409,1.27772911668787,1.27977789660999,1.28261325563633,
1.28988797049119,1.41277504561787,1.52102929598508,1.69581005597633,1.70433583150545,
1.70822053462579,1.71114060620604,1.71388095931465,1.71766796647744,1.72734995544263,
1.87813929223131,1.95513954672685,2.11856549384494,2.12424496224557,2.12876929239171,
2.13146616057173,2.1334936688928,2.13605295738736,2.14040659402505,2.1554872883031,
2.15745647869779,2.17614527331743,2.21387900683578,2.32340512223105,2.46810413041667,
2.48678589322234,2.50179402274962,2.50962019097846,2.51618420073926,2.52242896408552,
2.53275891623459,2.55971100605392,2.74839199957644,2.8730923394382,2.88868062295377,
2.89289618240161,2.89542468657957,2.89768135341565,2.90052826897125,2.90603885331675,
2.94067875320462,3.14960715613848,3.30358274056309,3.31202051377418,3.31588838086973,
3.31880544491032,3.32155002035642,3.32535403434762,3.33513980875609,3.49314022624314,
3.57604723511976,3.67666450751218,3.69982988544085,3.72793708234981,3.744115649835,
3.74825858110122,3.75070109352932,3.75285471351248,3.75553693169349,3.75967247259297,
3.77851407675741,4.00151591376745,4.09062969189725,4.17487210723701,4.19787459767563,
4.21083142662629,4.22209059252564,4.23607106785952,4.26312676595551,4.45153254464311,
4.50264690832833,4.52196238343777,4.53617166594015,4.54285600582181,4.5484163993348,
4.55540384444795,4.56655767443692,4.6321874210292,4.68495437240109,4.71824348253228,
4.73232118112925,4.74294826238949,4.75456667003629,4.77388306384699,4.87683237556472,
4.93132912088735,4.94439015254172,4.95096941616951,4.95694800077712,4.96476356588773,
4.97817805183452,5.04853713350459,5.11382318120744,5.1757174525467,5.19637450479622,
5.21155273698212,5.22881143792393,5.25754612351168,5.30027725845294,5.33874981194839,
5.35242214148458,5.36540416933083,5.39841500532554,5.47211467157039,5.49055122316089,
5.507139283974,5.52991417199247,5.59700422966766,5.65839282004497,5.72751564801281,
5.74244898033661,5.749950073129,5.7558709698339,5.76277644098215,5.77787389000309,
5.79963225545946,5.87487674202028,5.93619073628499,5.95347487049008,5.96355822923337,
5.97422741436862,5.98860245227584,6.0240060522236,6.09301632905145,6.14320146832196,
6.1534827616281,6.1590500169829,6.16405738516219,6.17124025073293,6.18828403224541,
6.21282485305556,6.3326432396067,6.45153966852532,6.4735396407168,6.48643156207287,
6.49769724050674,6.51177200729218,6.54046636723328,6.66008290580623,6.82994401051037,
6.92489536519698,6.94587361642104,6.95016677254978,6.95289750564723,6.95505564666766,
6.95746704872175,6.96147148843887,6.97609737426708,7.08992812678715,7.23761359847736,
7.37090196039549,7.38047786746523,7.38424648066357,7.38698156305497,7.38990353148128,
7.39380358869357,7.40241497286651,7.52229387398696,7.72419730999893,7.79829781366815,
7.80476052531121,7.8077254300926,7.81000408578516,7.81244719036203,7.81495136837684,
7.82229806306039,7.83263610775129,7.95753542443239,8.14578033661352,8.17281096784043,
8.18314786432988,8.18939302260039,8.19595516725053,8.2033268272341,8.21723703484199,
8.23453167456104,8.35927511476581,8.52759722226799,8.55247731645695,8.56565555726439,
8.56978660265598,8.57204571919405,8.57429402342049,8.57704422684477,8.58163166081751,
8.60599943034831,8.65445800415061,8.75341181582875,8.82966261761597,8.97796569438977,
8.98762867651646,8.99141172282758,8.99415041113987,8.99706982851656,9.00095557332558,
9.00949131344891,9.18872204606232,9.28193523226186,9.41272295691981,9.42190792789857,
9.42538573198735,9.42744977026146,9.42940392715672,9.43212876400306,9.43507507126447,
9.44681506989839,9.47586682520955,9.56539509660465,9.66959759990051,9.67324628813472,
9.69476972276663,9.83257384078495,9.86658710463717,9.88047385728483,9.89196937718491,
9.90248245502818,9.91403223559125,9.92986860774804,10.0393653359466,10.0773539343858,
10.1300511129673,10.2018099159825,10.2132832248525,10.2192571617898,10.2224066646963,
10.2237944604769),.UNSPECIFIED.);
#3194=B_SPLINE_CURVE_WITH_KNOTS('',3,(#165803,#165804,#165805,#165806,#165807,
#165808,#165809,#165810,#165811,#165812,#165813,#165814,#165815,#165816,
#165817,#165818,#165819,#165820,#165821,#165822,#165823,#165824,#165825,
#165826,#165827,#165828,#165829,#165830,#165831,#165832,#165833,#165834,
#165835,#165836,#165837,#165838,#165839,#165840,#165841,#165842,#165843,
#165844,#165845,#165846,#165847,#165848,#165849,#165850,#165851,#165852,
#165853,#165854,#165855,#165856,#165857,#165858,#165859,#165860,#165861,
#165862,#165863,#165864,#165865,#165866,#165867,#165868,#165869,#165870,
#165871,#165872,#165873,#165874,#165875,#165876,#165877,#165878,#165879,
#165880,#165881,#165882,#165883,#165884,#165885,#165886,#165887,#165888,
#165889,#165890,#165891,#165892,#165893,#165894,#165895,#165896,#165897,
#165898,#165899,#165900,#165901,#165902,#165903,#165904,#165905,#165906,
#165907,#165908,#165909,#165910,#165911,#165912,#165913,#165914,#165915,
#165916,#165917,#165918,#165919,#165920,#165921,#165922,#165923,#165924,
#165925,#165926,#165927,#165928,#165929,#165930,#165931,#165932,#165933,
#165934,#165935,#165936,#165937,#165938,#165939,#165940,#165941,#165942,
#165943,#165944,#165945,#165946,#165947,#165948,#165949,#165950,#165951,
#165952,#165953,#165954,#165955,#165956,#165957,#165958,#165959,#165960,
#165961,#165962,#165963,#165964,#165965,#165966,#165967,#165968,#165969,
#165970,#165971,#165972,#165973,#165974,#165975,#165976,#165977,#165978,
#165979,#165980,#165981,#165982,#165983,#165984,#165985,#165986,#165987,
#165988,#165989,#165990,#165991,#165992,#165993,#165994,#165995,#165996,
#165997,#165998,#165999,#166000,#166001,#166002,#166003,#166004,#166005,
#166006,#166007,#166008,#166009,#166010,#166011,#166012,#166013,#166014,
#166015,#166016,#166017,#166018,#166019,#166020,#166021,#166022,#166023,
#166024,#166025,#166026,#166027,#166028,#166029,#166030,#166031,#166032,
#166033,#166034,#166035,#166036,#166037,#166038,#166039,#166040,#166041,
#166042,#166043,#166044,#166045,#166046,#166047,#166048,#166049,#166050,
#166051,#166052,#166053,#166054,#166055,#166056,#166057,#166058,#166059,
#166060,#166061,#166062,#166063,#166064,#166065,#166066,#166067,#166068,
#166069,#166070,#166071,#166072,#166073,#166074,#166075,#166076,#166077,
#166078,#166079,#166080,#166081,#166082,#166083,#166084,#166085,#166086,
#166087,#166088,#166089,#166090,#166091,#166092,#166093,#166094,#166095,
#166096,#166097,#166098,#166099,#166100,#166101,#166102,#166103,#166104,
#166105,#166106,#166107,#166108,#166109,#166110,#166111,#166112,#166113,
#166114,#166115,#166116,#166117,#166118,#166119,#166120,#166121,#166122,
#166123,#166124,#166125,#166126,#166127,#166128,#166129,#166130,#166131,
#166132,#166133,#166134,#166135,#166136,#166137,#166138,#166139,#166140,
#166141,#166142,#166143,#166144,#166145,#166146,#166147,#166148,#166149,
#166150,#166151,#166152,#166153,#166154,#166155,#166156,#166157,#166158,
#166159,#166160,#166161,#166162,#166163,#166164,#166165,#166166,#166167,
#166168,#166169,#166170,#166171,#166172,#166173,#166174,#166175,#166176,
#166177,#166178,#166179,#166180,#166181,#166182,#166183,#166184,#166185,
#166186,#166187,#166188,#166189,#166190,#166191,#166192,#166193,#166194,
#166195,#166196,#166197,#166198,#166199,#166200,#166201,#166202,#166203,
#166204,#166205,#166206,#166207,#166208,#166209,#166210,#166211,#166212,
#166213,#166214,#166215,#166216,#166217,#166218,#166219,#166220,#166221,
#166222,#166223,#166224,#166225,#166226,#166227,#166228,#166229,#166230,
#166231,#166232,#166233,#166234,#166235,#166236,#166237,#166238,#166239,
#166240,#166241,#166242,#166243,#166244,#166245,#166246,#166247,#166248,
#166249,#166250,#166251,#166252,#166253,#166254,#166255,#166256,#166257,
#166258,#166259,#166260,#166261,#166262,#166263,#166264,#166265,#166266,
#166267,#166268,#166269,#166270,#166271,#166272,#166273,#166274,#166275,
#166276,#166277,#166278,#166279,#166280,#166281,#166282,#166283,#166284,
#166285,#166286,#166287,#166288,#166289,#166290,#166291,#166292,#166293,
#166294,#166295,#166296,#166297,#166298,#166299,#166300,#166301,#166302,
#166303,#166304,#166305,#166306,#166307,#166308,#166309,#166310,#166311,
#166312,#166313,#166314,#166315,#166316,#166317,#166318,#166319,#166320,
#166321,#166322,#166323,#166324,#166325,#166326,#166327,#166328,#166329,
#166330,#166331,#166332,#166333,#166334,#166335,#166336,#166337,#166338,
#166339,#166340,#166341,#166342,#166343,#166344,#166345,#166346,#166347,
#166348,#166349,#166350,#166351,#166352,#166353,#166354,#166355,#166356,
#166357,#166358,#166359,#166360,#166361,#166362,#166363,#166364,#166365,
#166366,#166367,#166368,#166369,#166370,#166371,#166372,#166373,#166374,
#166375,#166376,#166377,#166378,#166379,#166380,#166381,#166382,#166383,
#166384,#166385,#166386,#166387,#166388,#166389,#166390,#166391,#166392,
#166393,#166394),.UNSPECIFIED.,.F.,.F.,(4,2,2,2,2,2,2,2,2,2,2,2,2,2,2,2,
2,2,2,2,2,2,2,2,2,2,2,2,2,2,2,2,2,2,2,2,2,2,2,2,2,2,2,2,2,2,2,2,2,2,2,2,
2,2,2,2,2,2,2,2,2,2,2,2,2,2,2,2,2,2,2,2,2,2,2,2,2,2,2,2,2,2,2,2,2,2,2,2,
2,2,2,2,2,2,2,2,2,2,2,2,2,2,2,2,2,2,2,2,2,2,2,2,2,2,2,2,2,2,2,2,2,2,2,2,
2,2,2,2,2,2,2,2,2,2,2,2,2,2,2,2,2,2,2,2,2,2,2,2,2,2,2,2,2,2,2,2,2,2,2,2,
2,2,2,2,2,2,2,2,2,2,2,2,2,2,2,2,2,2,2,2,2,2,2,2,2,2,2,2,2,2,2,2,2,2,2,2,
2,2,2,2,2,2,2,2,2,2,2,2,2,2,2,2,2,2,2,2,2,2,2,2,2,2,2,2,2,2,2,2,2,2,2,2,
2,2,2,2,2,2,2,2,2,2,2,2,2,2,2,2,2,2,2,2,2,2,2,2,2,2,2,2,2,2,2,2,2,2,2,2,
2,2,2,2,2,2,2,2,2,2,2,2,2,2,2,2,2,2,2,2,2,2,2,2,2,2,2,4),(0.00188190208457017,
0.00399627713341498,0.00873346078420522,0.0196781469812297,0.0856369599480584,
0.161869882608815,0.175737014961344,0.186182018023973,0.196303179196513,
0.206344975829605,0.223395483122565,0.280569084600253,0.341429096207342,
0.374922414610643,0.388925204464006,0.396843424988868,0.402465300888644,
0.40817524846264,0.414838693706063,0.42616349746827,0.474906685334838,0.576981540011668,
0.627361376000328,0.630159019113763,0.631722892788452,0.632567972685891,
0.633016321902011,0.634982791062869,0.636534990113496,0.637744550736026,
0.638677280703863,0.639390520969028,0.639932318775882,0.640341765382074,
0.640649963956381,0.641574755610088,0.656940208644136,0.673167247567888,
0.693227522909643,0.738030196848381,0.775390350516043,0.798232859895037,
0.80954310109032,0.821989926849744,0.827826911121362,0.858601163433563,
0.918035570875503,0.935076074699258,0.951101962048288,0.968945151418558,
0.999212564962949,1.14454667873245,1.17469868185873,1.18848310579882,1.19670465538289,
1.20276285105365,1.20844387698576,1.21396960848659,1.22424468494723,1.28766561062729,
1.34152699585792,1.37574915565574,1.40104465114948,1.41148520739628,1.42153158100933,
1.43152337018159,1.44830202563702,1.50589792573087,1.57219325631432,1.59129402420728,
1.60512352989554,1.6107715416142,1.61616820931015,1.62216505797161,1.63264728587892,
1.68087548643409,1.78837934048518,1.86671182185378,1.89944189697937,1.92464929704944,
1.93577431579996,1.9471793023478,1.95796026479062,1.97625411815051,2.0301224455804,
2.24383548879379,2.36171191159315,2.39754176563455,2.40389933322904,2.40684862651801,
2.40903795723456,2.41107214203255,2.41385167968018,2.4193397805965,2.48385531213702,
2.51635324883219,2.70798411436433,2.8270133535038,2.83567077444962,2.83957986274691,
2.84250378776175,2.84523725015434,2.84899822616757,2.85852621101432,2.99096102885002,
3.14520869896789,3.19736879721844,3.24271933681024,3.25679728248856,3.26086488725105,
3.26336042126369,3.26562394671381,3.26852964835857,3.27318066824222,3.29796765457727,
3.33579943223096,3.4113810060932,3.54794764449462,3.62043879645794,3.63425973820241,
3.64195743614027,3.64848779316595,3.65587102728352,3.66823900904374,3.71147090873089,
3.76230070591415,3.92459900760316,3.98989280945017,4.01837214484894,4.0234600944039,
4.02618030125787,4.02820895394901,4.03042741944535,4.03436168120946,4.04597543793212,
4.04691811385669,4.29182271975965,4.39365336085305,4.43747543095095,4.4443233437924,
4.44787568433054,4.45047984560055,4.45368350128684,4.45893505367947,4.47544724711454,
4.7874602434939,4.86468783702226,4.87708779838307,4.88086238931171,4.8832230103228,
4.88539441458556,4.88817814711441,4.89408376138162,4.936766886737,5.114669525566,
5.28650197513703,5.32213065495992,5.3362819177911,5.34784898100086,5.35962994739869,
5.37693645312297,5.426208416691,5.54801068839648,5.59446180885821,5.60142787624911,
5.65902934921753,5.67031119029756,5.67644769639869,5.68211753646609,5.68989507527497,
5.708860805591,5.72499754754483,5.80228082916276,5.81388619575106,5.84916595000714,
5.86238407825231,5.8731785196803,5.88424187843515,5.90080664840088,5.95571664728315,
6.03507302572295,6.07003480130233,6.07948728764132,6.08491457861945,6.09110945593149,
6.10023215772556,6.12608762339023,6.15027767645197,6.28751983695318,6.32130515314122,
6.33977899967134,6.35466082524932,6.37649860877436,6.40297669314087,6.47177880842746,
6.48533865175689,6.49842213323086,6.53292344288207,6.6044893659996,6.62304051502869,
6.63960728147354,6.66216839586275,6.72677357419958,6.79092377531655,6.86064898836049,
6.87415034180332,6.8819914004204,6.88797582782014,6.89454414028451,6.9075268602895,
6.91709340421134,6.9342523150848,7.01800187584957,7.07035517995359,7.0870663139455,
7.09704934855207,7.10778414978548,7.12256113904019,7.16103441391893,7.19703950833263,
7.27199204172726,7.28345682786914,7.29053475450935,7.29610567296989,7.30270846818865,
7.31646627749367,7.32659124670002,7.35893639309173,7.48872860506365,7.51790696745331,
7.58852944976054,7.60873548413547,7.62112236694546,7.63249337448912,7.64748264309209,
7.68139131372957,7.85957857108816,7.98353725714297,8.07611339840757,8.08276340023158,
8.08546781040463,8.08748367171114,8.08968923712917,8.09272812182832,8.09985593466942,
8.20111400639101,8.24558059665294,8.47132399001199,8.50873758336276,8.51508830173201,
8.51888909708128,8.52180683926192,8.52486900330743,8.52960175168872,8.53511851340148,
8.54540669291271,8.63395034576474,8.87508719385648,8.93278321007588,8.93897836069356,
8.94189347840398,8.94416546258657,8.94663301765988,8.95057352872476,8.96348488003056,
9.0503347083963,9.19328516283191,9.29668033899776,9.3123037639036,9.32036894188253,
9.32695700208053,9.33398004758763,9.34468285234216,9.37688562016362,9.42524405614271,
9.45075560818347,9.57144882521517,9.69540937830716,9.70228079273981,9.70504896937153,
9.70735186806826,9.70971019284281,9.71314836479771,9.72220295897674,9.76389393225265,
10.0273273265981,10.0435888611411,10.1149195263784,10.1225790603345,10.1263770390947,
10.1291206067928,10.1318877839019,10.1347204895935,10.1383950572546,10.1441483691459,
10.2281508016451),.UNSPECIFIED.);
#3195=B_SPLINE_CURVE_WITH_KNOTS('',3,(#166396,#166397,#166398,#166399,#166400,
#166401,#166402,#166403,#166404,#166405,#166406,#166407,#166408,#166409,
#166410,#166411,#166412,#166413,#166414,#166415,#166416,#166417,#166418,
#166419,#166420,#166421,#166422,#166423,#166424,#166425,#166426,#166427,
#166428,#166429,#166430,#166431,#166432,#166433,#166434,#166435,#166436,
#166437,#166438,#166439,#166440,#166441,#166442,#166443,#166444,#166445,
#166446,#166447,#166448,#166449,#166450,#166451,#166452,#166453,#166454,
#166455,#166456,#166457,#166458,#166459,#166460,#166461,#166462,#166463,
#166464,#166465,#166466,#166467,#166468,#166469,#166470,#166471,#166472,
#166473,#166474,#166475,#166476,#166477,#166478,#166479,#166480,#166481,
#166482,#166483,#166484,#166485,#166486,#166487,#166488,#166489,#166490,
#166491,#166492,#166493,#166494,#166495,#166496,#166497,#166498,#166499,
#166500,#166501,#166502,#166503,#166504,#166505,#166506,#166507,#166508,
#166509,#166510,#166511,#166512,#166513,#166514,#166515,#166516,#166517,
#166518,#166519,#166520,#166521,#166522,#166523,#166524,#166525,#166526,
#166527,#166528,#166529,#166530,#166531,#166532,#166533,#166534,#166535,
#166536,#166537,#166538,#166539,#166540,#166541,#166542,#166543,#166544,
#166545,#166546,#166547,#166548,#166549,#166550,#166551,#166552,#166553,
#166554,#166555,#166556,#166557,#166558,#166559,#166560,#166561,#166562,
#166563,#166564,#166565,#166566,#166567,#166568,#166569,#166570,#166571,
#166572,#166573,#166574,#166575,#166576,#166577,#166578,#166579,#166580,
#166581,#166582,#166583,#166584,#166585,#166586,#166587,#166588,#166589,
#166590,#166591,#166592,#166593,#166594,#166595,#166596,#166597,#166598,
#166599,#166600,#166601,#166602,#166603,#166604,#166605,#166606,#166607,
#166608,#166609,#166610,#166611,#166612,#166613,#166614,#166615,#166616,
#166617,#166618,#166619,#166620,#166621,#166622,#166623,#166624,#166625,
#166626,#166627,#166628,#166629,#166630,#166631,#166632,#166633,#166634,
#166635,#166636,#166637,#166638,#166639,#166640,#166641,#166642,#166643,
#166644,#166645,#166646,#166647,#166648,#166649,#166650,#166651),
 .UNSPECIFIED.,.F.,.F.,(4,3,3,3,3,3,3,3,3,3,3,3,3,3,3,3,3,3,3,3,3,3,3,3,
3,3,3,3,3,3,3,3,3,3,3,3,3,3,3,3,3,3,3,3,3,3,3,3,3,3,3,3,3,3,3,3,3,3,3,3,
3,3,3,3,3,3,3,3,3,3,3,3,3,3,3,3,3,3,3,3,3,3,3,3,3,4),(135.088484268768,
135.174411881758,135.260833130134,135.347449824148,135.434213236371,135.475106554013,
135.546529828863,135.617899955776,135.689230527297,135.760543864782,135.831844551604,
135.903170033097,135.973575097321,136.061280586662,136.149456949081,136.238061359699,
136.326761666583,136.415357926518,136.472043640628,136.545013085078,136.617937076171,
136.690828602912,136.763710801833,136.836585719876,136.909488669586,136.970512183936,
137.049812967885,137.129135898362,137.208478500372,137.287851577545,137.367233258542,
137.446630035651,137.468980727243,137.548378121912,137.62776179574,137.707129247381,
137.786474431193,137.865797450459,137.945091680081,137.967449270551,138.04035167082,
138.113231527865,138.186101797298,138.258998141703,138.331906797488,138.404875110437,
138.465917813859,138.554492145472,138.643192510946,138.731759323049,138.820102736613,
138.907872453238,138.964386357166,139.035709855516,139.107013605671,139.178311108943,
139.24964360459,139.320991963329,139.392412618296,139.462854900474,139.538958396495,
139.615011542566,139.691024732801,139.767008332682,139.84297268601,139.920075098645,
139.996046826684,140.072031153943,140.148037495615,140.225976118484,140.302085157912,
140.3809385725,140.459791987089,140.535924859334,140.611964560405,140.687920565776,
140.763779008313,140.839580071867,140.915319392601,140.958260530396,141.031847365433,
141.10545872087,141.179143713537,141.252869320595,141.326690169256,141.371669411541),
 .UNSPECIFIED.);
#3196=B_SPLINE_CURVE_WITH_KNOTS('',3,(#166653,#166654,#166655,#166656,#166657,
#166658,#166659,#166660,#166661,#166662,#166663,#166664,#166665,#166666,
#166667),.UNSPECIFIED.,.F.,.F.,(4,1,1,1,1,1,1,1,1,1,1,1,4),(141.371669411541,
141.456729073704,142.453666160319,142.952134703627,143.450603246934,143.949071790242,
144.447540333549,144.946008876857,145.444477420164,145.942945963472,146.441414506779,
147.438351593395,147.654854718721),.UNSPECIFIED.);
#3197=B_SPLINE_CURVE_WITH_KNOTS('',3,(#166669,#166670,#166671,#166672,#166673,
#166674,#166675,#166676,#166677,#166678,#166679,#166680,#166681,#166682,
#166683,#166684,#166685,#166686,#166687,#166688,#166689,#166690,#166691,
#166692,#166693,#166694,#166695,#166696,#166697,#166698,#166699,#166700,
#166701,#166702,#166703,#166704,#166705,#166706,#166707,#166708,#166709,
#166710,#166711,#166712,#166713,#166714,#166715,#166716,#166717,#166718,
#166719,#166720,#166721,#166722,#166723,#166724,#166725,#166726,#166727,
#166728,#166729,#166730,#166731,#166732,#166733,#166734,#166735,#166736,
#166737,#166738,#166739,#166740,#166741,#166742,#166743,#166744,#166745,
#166746,#166747,#166748,#166749,#166750,#166751,#166752,#166753,#166754,
#166755,#166756,#166757,#166758,#166759,#166760,#166761,#166762,#166763,
#166764,#166765,#166766,#166767,#166768,#166769,#166770,#166771,#166772,
#166773,#166774,#166775,#166776,#166777,#166778,#166779,#166780,#166781,
#166782,#166783,#166784,#166785,#166786,#166787,#166788,#166789,#166790,
#166791,#166792,#166793,#166794,#166795,#166796,#166797,#166798,#166799,
#166800,#166801,#166802,#166803,#166804,#166805,#166806,#166807,#166808,
#166809,#166810,#166811,#166812,#166813,#166814,#166815,#166816,#166817,
#166818,#166819,#166820,#166821,#166822,#166823,#166824,#166825,#166826,
#166827,#166828,#166829,#166830,#166831,#166832,#166833,#166834,#166835,
#166836,#166837,#166838,#166839,#166840,#166841,#166842,#166843,#166844,
#166845,#166846,#166847,#166848,#166849,#166850,#166851,#166852,#166853,
#166854,#166855,#166856,#166857,#166858,#166859,#166860,#166861,#166862,
#166863,#166864,#166865,#166866,#166867,#166868,#166869,#166870,#166871,
#166872,#166873,#166874,#166875,#166876,#166877,#166878,#166879,#166880,
#166881,#166882,#166883,#166884,#166885,#166886,#166887,#166888,#166889,
#166890,#166891,#166892,#166893,#166894,#166895,#166896,#166897,#166898,
#166899,#166900,#166901,#166902,#166903,#166904,#166905,#166906,#166907,
#166908,#166909,#166910,#166911,#166912,#166913,#166914,#166915,#166916,
#166917,#166918,#166919,#166920,#166921,#166922,#166923,#166924),
 .UNSPECIFIED.,.F.,.F.,(4,3,3,3,3,3,3,3,3,3,3,3,3,3,3,3,3,3,3,3,3,3,3,3,
3,3,3,3,3,3,3,3,3,3,3,3,3,3,3,3,3,3,3,3,3,3,3,3,3,3,3,3,3,3,3,3,3,3,3,3,
3,3,3,3,3,3,3,3,3,3,3,3,3,3,3,3,3,3,3,3,3,3,3,3,3,4),(147.654854718721,
147.72659930312,147.798301556539,147.869977993175,147.936820136702,148.01256250148,
148.088350622185,148.164193792981,148.240148751194,148.316165183482,148.392300978936,
148.43528868001,148.511499260519,148.587641864807,148.663726951184,148.739764937492,
148.815766208083,148.892823652901,148.968788915062,149.044750506961,149.120717834058,
149.198594817199,149.274624614666,149.353425190645,149.432225766625,149.503649041421,
149.575019168282,149.64634973975,149.717663077184,149.788963763955,149.860289245397,
149.930694309932,150.018399799239,150.106576161617,150.195180572185,150.283880879014,
150.372477138894,150.42916285324,150.502132298068,150.57505628954,150.647947816658,
150.720830015955,150.793704934373,150.866607884455,150.927631396547,151.006932178665,
151.08625510729,151.165597707437,151.244970782754,151.324352461906,151.403749237202,
151.426099939855,151.505497338627,151.584881016578,151.664248472337,151.743593660218,
151.822916683505,151.90221091705,151.924568483163,151.99747087888,152.070350731371,
152.143220996249,152.216117336111,152.289025987356,152.361994295789,152.42303702647,
152.511611372041,152.600311751838,152.688878577832,152.777222004591,152.864991732835,
152.921505569778,152.992829065116,153.064132812262,153.13543031253,153.206762805185,
153.278111160937,153.349531812937,153.419974113085,153.500009163612,153.57998474546,
153.659895229108,153.739703944664,153.819442361188,153.899074932354,153.938038318046),
 .UNSPECIFIED.);
#3198=B_SPLINE_CURVE_WITH_KNOTS('',3,(#166926,#166927,#166928,#166929,#166930,
#166931,#166932,#166933,#166934,#166935,#166936,#166937,#166938,#166939,
#166940,#166941,#166942,#166943,#166944,#166945,#166946,#166947,#166948,
#166949,#166950,#166951,#166952,#166953,#166954,#166955,#166956,#166957,
#166958,#166959,#166960,#166961,#166962,#166963,#166964,#166965,#166966,
#166967,#166968,#166969,#166970,#166971,#166972,#166973,#166974,#166975,
#166976,#166977,#166978,#166979,#166980,#166981,#166982,#166983,#166984,
#166985,#166986,#166987,#166988,#166989,#166990,#166991,#166992,#166993,
#166994,#166995,#166996,#166997,#166998,#166999,#167000,#167001,#167002,
#167003,#167004,#167005,#167006,#167007,#167008,#167009,#167010,#167011,
#167012,#167013,#167014,#167015,#167016,#167017,#167018,#167019,#167020,
#167021,#167022,#167023,#167024,#167025,#167026,#167027,#167028,#167029,
#167030,#167031,#167032,#167033,#167034,#167035,#167036,#167037,#167038,
#167039,#167040,#167041,#167042,#167043,#167044,#167045,#167046,#167047,
#167048,#167049,#167050,#167051,#167052,#167053,#167054,#167055,#167056,
#167057,#167058,#167059,#167060,#167061,#167062,#167063,#167064,#167065,
#167066,#167067,#167068,#167069,#167070,#167071,#167072,#167073,#167074,
#167075,#167076,#167077,#167078,#167079,#167080,#167081,#167082,#167083,
#167084,#167085,#167086,#167087,#167088,#167089,#167090,#167091,#167092,
#167093,#167094,#167095,#167096,#167097,#167098,#167099,#167100,#167101,
#167102,#167103,#167104,#167105,#167106,#167107,#167108,#167109,#167110,
#167111,#167112,#167113,#167114,#167115,#167116,#167117,#167118,#167119,
#167120,#167121,#167122,#167123,#167124,#167125,#167126,#167127,#167128,
#167129,#167130,#167131,#167132,#167133,#167134,#167135,#167136,#167137,
#167138,#167139,#167140,#167141,#167142,#167143,#167144,#167145,#167146,
#167147,#167148,#167149,#167150,#167151,#167152,#167153,#167154,#167155,
#167156,#167157,#167158,#167159,#167160,#167161,#167162,#167163,#167164,
#167165,#167166,#167167,#167168,#167169,#167170,#167171,#167172,#167173,
#167174,#167175,#167176,#167177,#167178,#167179,#167180,#167181),
 .UNSPECIFIED.,.F.,.F.,(4,3,3,3,3,3,3,3,3,3,3,3,3,3,3,3,3,3,3,3,3,3,3,3,
3,3,3,3,3,3,3,3,3,3,3,3,3,3,3,3,3,3,3,3,3,3,3,3,3,3,3,3,3,3,3,3,3,3,3,3,
3,3,3,3,3,3,3,3,3,3,3,3,3,3,3,3,3,3,3,3,3,3,3,3,3,4),(153.9380400259,154.01774156604,
154.097563789192,154.177571946043,154.257667774446,154.337910276897,154.4169111997,
154.493044120776,154.569083870191,154.645039923326,154.720898412545,154.796699522112,
154.872438887665,154.915379743008,154.991122030882,155.066910073592,155.142753165459,
155.218708043807,155.294724395709,155.370860110543,155.413848286316,155.490058890158,
155.566201517879,155.642286627742,155.718324637542,155.79432593158,155.871383361749,
155.947348647013,156.023310261818,156.099277611579,156.177154551917,156.253184371199,
156.331984872065,156.410785372931,156.482208725666,156.553578930457,156.624909579826,
156.696222994972,156.767523759411,156.838849318175,156.909253916238,156.996958497115,
157.085133874579,157.173737247445,157.262436517993,157.351031797816,157.407722459546,
157.480692987845,157.553618060411,157.62651066566,157.699393935898,157.772269921869,
157.845173929934,157.906191002853,157.985488516737,158.064808145032,158.144147430725,
158.223517208898,158.302895613596,158.382289175932,158.404659546161,158.484062011193,
158.563450771727,158.642823298686,158.722173484869,158.801501443599,158.880800482891,
158.903128089468,158.976027192385,159.048903755277,159.121770735486,159.194663807133,
159.267569196936,159.340534269289,159.401596632776,159.49017046845,159.578870172144,
159.667436123138,159.755778593328,159.843547284668,159.900065176084,159.968705563624,
160.03733317896,160.105951360206,160.174594356136,160.220901167348),
 .UNSPECIFIED.);
#3199=B_SPLINE_CURVE_WITH_KNOTS('',3,(#167183,#167184,#167185,#167186,#167187,
#167188,#167189,#167190,#167191,#167192,#167193,#167194,#167195,#167196,
#167197,#167198,#167199,#167200),.UNSPECIFIED.,.F.,.F.,(4,2,2,2,2,2,2,2,
4),(160.221433754171,161.050583109518,161.879940885956,162.709298662394,
163.538656438832,164.36801421527,165.197371991708,166.026729768145,166.504401885182),
 .UNSPECIFIED.);
#3200=B_SPLINE_CURVE_WITH_KNOTS('',3,(#167202,#167203,#167204,#167205,#167206,
#167207,#167208,#167209,#167210,#167211,#167212,#167213),.UNSPECIFIED.,
 .F.,.F.,(4,1,1,1,1,1,1,1,1,4),(166.504733301143,167.377093325697,168.374030412312,
169.370967498927,169.869436042235,170.367904585542,170.86637312885,171.364841672157,
172.361778758772,172.787595947439),.UNSPECIFIED.);
#3201=B_SPLINE_CURVE_WITH_KNOTS('',3,(#167215,#167216,#167217,#167218,#167219,
#167220,#167221,#167222,#167223,#167224,#167225,#167226,#167227,#167228,
#167229,#167230,#167231,#167232),.UNSPECIFIED.,.F.,.F.,(4,2,2,2,2,2,2,2,
4),(172.787595947439,173.616953723877,174.446311500315,175.275669276753,
176.105027053191,176.934384829629,177.763742606067,178.593100382505,179.070781254619),
 .UNSPECIFIED.);
#3202=B_SPLINE_CURVE_WITH_KNOTS('',3,(#167234,#167235,#167236,#167237,#167238,
#167239,#167240,#167241,#167242,#167243,#167244,#167245,#167246,#167247,
#167248,#167249,#167250,#167251,#167252,#167253,#167254,#167255,#167256,
#167257,#167258,#167259,#167260,#167261,#167262,#167263,#167264,#167265,
#167266,#167267,#167268,#167269,#167270,#167271,#167272,#167273,#167274,
#167275,#167276,#167277,#167278,#167279,#167280,#167281,#167282,#167283,
#167284,#167285,#167286,#167287,#167288,#167289,#167290,#167291,#167292,
#167293,#167294,#167295,#167296,#167297,#167298,#167299,#167300,#167301,
#167302,#167303,#167304,#167305,#167306,#167307,#167308,#167309,#167310,
#167311,#167312,#167313,#167314,#167315,#167316,#167317,#167318,#167319,
#167320,#167321,#167322,#167323,#167324,#167325,#167326,#167327,#167328,
#167329,#167330,#167331,#167332,#167333,#167334,#167335,#167336,#167337,
#167338,#167339,#167340,#167341,#167342,#167343,#167344,#167345,#167346,
#167347,#167348,#167349,#167350,#167351,#167352,#167353,#167354,#167355,
#167356,#167357,#167358,#167359,#167360,#167361,#167362,#167363,#167364,
#167365,#167366,#167367,#167368,#167369,#167370,#167371,#167372,#167373,
#167374,#167375,#167376,#167377,#167378,#167379,#167380,#167381,#167382,
#167383,#167384,#167385,#167386,#167387,#167388,#167389,#167390,#167391,
#167392,#167393,#167394,#167395,#167396,#167397,#167398,#167399,#167400,
#167401,#167402,#167403,#167404,#167405,#167406,#167407,#167408,#167409,
#167410,#167411,#167412,#167413,#167414,#167415,#167416,#167417,#167418,
#167419,#167420,#167421,#167422,#167423,#167424,#167425,#167426,#167427,
#167428,#167429,#167430,#167431,#167432,#167433,#167434,#167435,#167436,
#167437,#167438,#167439,#167440,#167441,#167442,#167443,#167444,#167445,
#167446,#167447,#167448,#167449,#167450,#167451,#167452,#167453,#167454,
#167455,#167456,#167457,#167458,#167459,#167460,#167461,#167462,#167463,
#167464,#167465,#167466,#167467,#167468,#167469,#167470,#167471,#167472,
#167473,#167474,#167475,#167476,#167477,#167478,#167479,#167480,#167481,
#167482,#167483,#167484,#167485,#167486,#167487,#167488,#167489,#167490,
#167491,#167492,#167493,#167494,#167495,#167496,#167497,#167498,#167499,
#167500,#167501,#167502,#167503,#167504,#167505,#167506,#167507,#167508,
#167509,#167510,#167511,#167512,#167513,#167514,#167515,#167516,#167517,
#167518,#167519,#167520,#167521,#167522,#167523,#167524,#167525,#167526,
#167527,#167528,#167529,#167530,#167531,#167532,#167533,#167534,#167535,
#167536,#167537,#167538,#167539,#167540,#167541,#167542,#167543,#167544,
#167545,#167546,#167547,#167548,#167549,#167550,#167551,#167552,#167553,
#167554,#167555,#167556,#167557,#167558,#167559,#167560,#167561,#167562,
#167563,#167564,#167565,#167566,#167567,#167568,#167569,#167570,#167571,
#167572,#167573,#167574,#167575,#167576,#167577,#167578,#167579,#167580,
#167581,#167582,#167583,#167584,#167585,#167586,#167587,#167588,#167589,
#167590,#167591,#167592,#167593,#167594,#167595,#167596,#167597,#167598,
#167599,#167600,#167601,#167602,#167603,#167604,#167605,#167606,#167607,
#167608,#167609,#167610,#167611,#167612,#167613,#167614,#167615,#167616,
#167617,#167618,#167619,#167620,#167621,#167622,#167623,#167624,#167625,
#167626,#167627,#167628,#167629,#167630,#167631,#167632,#167633,#167634,
#167635,#167636,#167637,#167638,#167639,#167640,#167641,#167642,#167643,
#167644,#167645,#167646,#167647,#167648,#167649,#167650,#167651,#167652,
#167653,#167654,#167655,#167656,#167657,#167658,#167659,#167660,#167661,
#167662,#167663,#167664,#167665,#167666,#167667,#167668,#167669,#167670,
#167671,#167672,#167673,#167674,#167675,#167676,#167677,#167678,#167679,
#167680,#167681,#167682,#167683,#167684,#167685,#167686,#167687,#167688,
#167689,#167690,#167691,#167692,#167693,#167694,#167695,#167696,#167697,
#167698,#167699,#167700,#167701,#167702,#167703,#167704,#167705,#167706,
#167707,#167708,#167709,#167710,#167711,#167712,#167713,#167714,#167715,
#167716,#167717,#167718,#167719,#167720,#167721,#167722,#167723,#167724,
#167725,#167726,#167727,#167728,#167729,#167730,#167731,#167732,#167733,
#167734,#167735,#167736,#167737,#167738,#167739,#167740,#167741,#167742,
#167743,#167744,#167745,#167746,#167747,#167748,#167749,#167750,#167751,
#167752,#167753,#167754,#167755,#167756,#167757,#167758,#167759,#167760,
#167761,#167762,#167763,#167764,#167765,#167766,#167767,#167768,#167769,
#167770,#167771,#167772,#167773,#167774,#167775,#167776,#167777,#167778,
#167779,#167780,#167781,#167782,#167783,#167784,#167785,#167786,#167787,
#167788,#167789,#167790,#167791,#167792,#167793,#167794,#167795,#167796,
#167797,#167798,#167799,#167800,#167801,#167802,#167803,#167804,#167805,
#167806,#167807,#167808,#167809,#167810,#167811,#167812,#167813),
 .UNSPECIFIED.,.F.,.F.,(4,2,2,2,2,2,2,2,2,2,2,2,2,2,2,2,2,2,2,2,2,2,2,2,
2,2,2,2,2,2,2,2,2,2,2,2,2,2,2,2,2,2,2,2,2,2,2,2,2,2,2,2,2,2,2,2,2,2,2,2,
2,2,2,2,2,2,2,2,2,2,2,2,2,2,2,2,2,2,2,2,2,2,2,2,2,2,2,2,2,2,2,2,2,2,2,2,
2,2,2,2,2,2,2,2,2,2,2,2,2,2,2,2,2,2,2,2,2,2,2,2,2,2,2,2,2,2,2,2,2,2,2,2,
2,2,2,2,2,2,2,2,2,2,2,2,2,2,2,2,2,2,2,2,2,2,2,2,2,2,2,2,2,2,2,2,2,2,2,2,
2,2,2,2,2,2,2,2,2,2,2,2,2,2,2,2,2,2,2,2,2,2,2,2,2,2,2,2,2,2,2,2,2,2,2,2,
2,2,2,2,2,2,2,2,2,2,2,2,2,2,2,2,2,2,2,2,2,2,2,2,2,2,2,2,2,2,2,2,2,2,2,2,
2,2,2,2,2,2,2,2,2,2,2,2,2,2,2,2,2,2,2,2,2,2,2,2,2,2,2,2,2,2,2,2,2,2,2,2,
2,2,2,2,2,2,2,2,2,2,2,2,2,4),(0.00175473219377527,0.0102639915195822,0.0198551234661248,
0.0302624690351261,0.0442639585826937,0.0762429488247187,0.110239649230437,
0.141167562458834,0.199412869610709,0.207414357874238,0.213183952960719,
0.218465970450596,0.223602668039412,0.232650938987427,0.255783539160852,
0.285481548946414,0.289429207702587,0.387495333935431,0.469927022923076,
0.502691690386715,0.520987016661417,0.533502844462343,0.544021574055287,
0.555281059642907,0.569419391193581,0.59850935210662,0.694552126930168,
0.811921268581424,0.880576941442497,0.962237397992056,1.00024304425663,
1.00665281604221,1.0095615408409,1.0117437427584,1.01378796825245,1.01716291012073,
1.02571567642927,1.15936661647529,1.23081736289662,1.33873084442956,1.43058111604604,
1.43852973544966,1.44230426895295,1.44520768326752,1.44798223725234,1.45269045860845,
1.46532649307236,1.66881119872638,1.78561912740571,1.83270908311646,1.85792111085327,
1.86254606258551,1.86530647538949,1.86755602336931,1.86981043098472,1.87391598249238,
1.88688176234183,2.07146869941756,2.20405899312687,2.22191526164143,2.2322523882598,
2.23945424949218,2.24646731437987,2.24648779918434,2.24650846143184,2.24652930160323,
2.24655032020409,2.24657151770201,2.2465928944687,2.24661445089594,2.24663617867777,
2.24665806969917,2.24668014241987,2.24670240458843,2.24672878287883,2.2467560505632,
2.24678422992943,2.2468133433831,2.24684341329753,2.24687446205743,2.24690651202037,
2.24693958543641,2.24697370441048,2.2470088909034,2.24704516665339,2.25363205660697,
2.26196122984078,2.27829941173527,2.42277900501808,2.50239711969813,2.60865122694243,
2.62302258262459,2.62711867329848,2.62962041614353,2.63188228856662,2.63477573781953,
2.63937301690103,2.66372676850353,2.83675971454541,2.95093174102913,3.02940881452137,
3.04380590509473,3.04859521224104,3.05169582858694,3.05462253382368,3.05848104175936,
3.06709423594561,3.14172326738905,3.31349454649346,3.47163136632539,3.48003623722723,
3.48328387300885,3.4855296942585,3.48773705371138,3.49040784876959,3.49712988682739,
3.60041100660568,3.77728778908965,3.89902308387369,3.92798960650723,3.94211463379963,
3.95338430996426,3.96624174476683,3.98808691089097,4.10360942433689,4.22502169338295,
4.25077288853278,4.26844156627594,4.27572797744257,4.28074259414517,4.28627095258433,
4.29634956798692,4.33861879763701,4.41080859296117,4.43757189899509,4.45864029675713,
4.47060258147791,4.48115569481206,4.49458495611188,4.52343382075178,4.58024363676307,
4.64333646649951,4.67285838548971,4.68155635514232,4.68751173879338,4.69321943481464,
4.7013640159026,4.72475739058829,4.85117107257798,4.91158601336947,4.93373620098741,
4.95024994073748,4.96900584347225,5.01033944071091,5.04715643646294,5.06749076981571,
5.08336672650831,5.09540066083849,5.11293414767461,5.16450425872884,5.20523099201403,
5.22388156243171,5.24041785976391,5.26276410868403,5.32515061251997,5.39082874106249,
5.39833906223304,5.40214996477169,5.46712424776639,5.47882920950683,5.48557401439953,
5.49089767759533,5.49846957464732,5.51808263661487,5.53522140029342,5.61878935055442,
5.67127506498819,5.68799340436212,5.69797518539345,5.70870451942961,5.72346636505519,
5.76184645233346,5.79770679465068,5.8721853988259,5.88402367110536,5.89120586463471,
5.89678650209857,5.90329424901015,5.91654913550917,5.93419862424077,6.06223755129916,
6.18529951441336,6.20739172807289,6.2203043684978,6.23156810301128,6.24561405996954,
6.27415203952366,6.39257553874006,6.48898460078045,6.65681224782744,6.67958074887322,
6.68399482209428,6.68676263693873,6.6889251373689,6.69131580485672,6.69522722337943,
6.70890884844539,6.80389264846716,6.97328335917045,7.10492468536199,7.11448183264075,
7.11824741278404,7.12098181151917,7.12390447185036,7.12780790026219,7.13643667647576,
7.25628636913056,7.45913210414344,7.53235043294122,7.53879543894682,7.54175713943717,
7.54403540023546,7.54648011053504,7.55032142064125,7.56238820330349,7.63912570255235,
7.88504274321496,7.90841725196076,7.91717885079275,7.92346022498246,7.92935939418366,
7.93695347219224,7.95044890555484,7.96685431206167,8.0796301237949,8.28267026853171,
8.28719827583329,8.300086867302,8.30418217661532,8.30643417327188,8.30868338328819,
8.31144642315177,8.31649931281682,8.34749806235849,8.37808690709208,8.50176356742623,
8.70798840858865,8.72096628124147,8.72572628919026,8.72851063790588,8.7311195772564,
8.73471389008161,8.74176641706399,8.7912658949537,8.88288436049876,9.00857158721545,
9.14724117327041,9.15640766933732,9.15988259505161,9.16194610852591,9.16390054970121,
9.16662703393643,9.17209866878485,9.21035819211417,9.29338820192485,9.44452207735449,
9.56902893193325,9.60247371703836,9.61722186940431,9.62858925684194,9.63906982278748,
9.65114910945188,9.68554096969399,9.73451548259927,9.9019120522969,9.93949848342984,
9.94948066519615,9.95478401210923,9.96016128914257,9.96583709243551,9.9687285708481,
9.98881023100644,10.0306775926922,10.1157874817235,10.1359746972935,10.1477584569336,
10.1580074895441,10.1682341579043,10.1814573680671,10.2240413365649),
 .UNSPECIFIED.);
#3203=B_SPLINE_CURVE_WITH_KNOTS('',3,(#167815,#167816,#167817,#167818,#167819,
#167820,#167821,#167822,#167823,#167824,#167825,#167826,#167827,#167828,
#167829,#167830,#167831,#167832),.UNSPECIFIED.,.F.,.F.,(4,2,2,2,2,2,2,2,
4),(191.637151868978,192.466509645416,193.295867421854,194.125225198292,
194.95458297473,195.783940751168,196.613298527606,197.442656304043,197.920337176157),
 .UNSPECIFIED.);
#3204=B_SPLINE_CURVE_WITH_KNOTS('',3,(#167834,#167835,#167836,#167837,#167838,
#167839,#167840,#167841,#167842,#167843,#167844,#167845,#167846,#167847,
#167848,#167849,#167850,#167851,#167852,#167853,#167854,#167855,#167856,
#167857,#167858,#167859,#167860,#167861,#167862,#167863,#167864,#167865,
#167866,#167867,#167868,#167869,#167870,#167871,#167872,#167873,#167874,
#167875,#167876,#167877,#167878,#167879,#167880,#167881,#167882,#167883,
#167884,#167885,#167886,#167887,#167888,#167889,#167890,#167891,#167892,
#167893,#167894,#167895,#167896,#167897,#167898,#167899,#167900,#167901,
#167902,#167903,#167904,#167905,#167906,#167907,#167908,#167909,#167910,
#167911,#167912,#167913,#167914,#167915,#167916,#167917,#167918,#167919,
#167920,#167921,#167922,#167923,#167924,#167925,#167926,#167927,#167928,
#167929,#167930,#167931,#167932,#167933,#167934,#167935,#167936,#167937,
#167938,#167939,#167940,#167941,#167942,#167943,#167944,#167945,#167946,
#167947,#167948,#167949,#167950,#167951,#167952,#167953,#167954,#167955,
#167956,#167957,#167958,#167959,#167960,#167961,#167962,#167963,#167964,
#167965,#167966,#167967,#167968,#167969,#167970,#167971,#167972,#167973,
#167974,#167975,#167976,#167977,#167978,#167979,#167980,#167981,#167982,
#167983,#167984,#167985,#167986,#167987,#167988,#167989,#167990,#167991,
#167992,#167993,#167994,#167995,#167996,#167997,#167998,#167999,#168000,
#168001,#168002,#168003,#168004,#168005,#168006,#168007,#168008,#168009,
#168010,#168011,#168012,#168013,#168014,#168015,#168016,#168017,#168018,
#168019,#168020,#168021,#168022,#168023,#168024,#168025,#168026,#168027,
#168028,#168029,#168030,#168031,#168032,#168033,#168034,#168035,#168036,
#168037,#168038,#168039,#168040,#168041,#168042,#168043,#168044,#168045,
#168046,#168047,#168048,#168049,#168050,#168051,#168052,#168053,#168054,
#168055,#168056,#168057,#168058,#168059,#168060,#168061,#168062,#168063,
#168064,#168065,#168066,#168067,#168068,#168069,#168070,#168071,#168072,
#168073,#168074,#168075,#168076,#168077,#168078,#168079,#168080,#168081,
#168082,#168083,#168084,#168085,#168086,#168087,#168088,#168089,#168090,
#168091,#168092,#168093,#168094,#168095,#168096,#168097,#168098,#168099,
#168100,#168101,#168102,#168103,#168104,#168105,#168106,#168107,#168108,
#168109,#168110,#168111,#168112,#168113,#168114,#168115,#168116,#168117,
#168118,#168119,#168120,#168121,#168122,#168123,#168124,#168125,#168126,
#168127,#168128,#168129,#168130,#168131,#168132,#168133,#168134,#168135,
#168136,#168137,#168138,#168139,#168140,#168141,#168142,#168143,#168144,
#168145,#168146,#168147,#168148,#168149,#168150,#168151,#168152,#168153,
#168154,#168155,#168156,#168157,#168158,#168159,#168160,#168161,#168162,
#168163,#168164,#168165,#168166,#168167,#168168,#168169,#168170,#168171,
#168172,#168173,#168174,#168175,#168176,#168177,#168178,#168179,#168180,
#168181,#168182,#168183,#168184,#168185,#168186,#168187,#168188,#168189,
#168190,#168191,#168192,#168193,#168194,#168195,#168196,#168197,#168198,
#168199,#168200,#168201,#168202,#168203,#168204,#168205,#168206,#168207,
#168208,#168209,#168210,#168211,#168212,#168213,#168214,#168215,#168216,
#168217,#168218,#168219,#168220,#168221,#168222,#168223,#168224,#168225,
#168226,#168227,#168228,#168229,#168230,#168231,#168232,#168233,#168234,
#168235,#168236,#168237,#168238,#168239,#168240,#168241,#168242,#168243,
#168244,#168245,#168246,#168247,#168248,#168249,#168250,#168251,#168252,
#168253,#168254,#168255,#168256,#168257,#168258,#168259,#168260,#168261,
#168262,#168263,#168264,#168265,#168266,#168267,#168268,#168269,#168270,
#168271,#168272,#168273,#168274,#168275,#168276,#168277,#168278,#168279,
#168280,#168281,#168282,#168283,#168284,#168285,#168286,#168287,#168288,
#168289,#168290,#168291,#168292,#168293,#168294,#168295,#168296,#168297,
#168298,#168299,#168300,#168301,#168302,#168303,#168304,#168305,#168306,
#168307,#168308,#168309,#168310,#168311,#168312,#168313,#168314,#168315,
#168316,#168317,#168318,#168319,#168320,#168321,#168322,#168323,#168324,
#168325,#168326,#168327,#168328,#168329,#168330,#168331,#168332,#168333,
#168334,#168335,#168336,#168337,#168338,#168339,#168340,#168341,#168342,
#168343,#168344,#168345,#168346,#168347,#168348,#168349,#168350,#168351,
#168352,#168353,#168354,#168355,#168356,#168357,#168358,#168359,#168360,
#168361,#168362,#168363,#168364,#168365,#168366,#168367,#168368,#168369,
#168370,#168371,#168372,#168373,#168374,#168375,#168376,#168377,#168378,
#168379,#168380,#168381,#168382,#168383,#168384,#168385,#168386,#168387,
#168388,#168389,#168390,#168391,#168392,#168393,#168394,#168395,#168396,
#168397,#168398,#168399,#168400,#168401,#168402,#168403,#168404,#168405,
#168406,#168407,#168408,#168409,#168410,#168411,#168412,#168413,#168414,
#168415,#168416,#168417,#168418,#168419,#168420,#168421,#168422,#168423,
#168424,#168425,#168426,#168427,#168428,#168429,#168430,#168431,#168432,
#168433,#168434,#168435),.UNSPECIFIED.,.F.,.F.,(4,2,2,2,2,2,2,2,2,2,2,2,
2,2,2,2,2,2,2,2,2,2,2,2,2,2,2,2,2,2,2,2,2,2,2,2,2,2,2,2,2,2,2,2,2,2,2,2,
2,2,2,2,2,2,2,2,2,2,2,2,2,2,2,2,2,2,2,2,2,2,2,2,2,2,2,2,2,2,2,2,2,2,2,2,
2,2,2,2,2,2,2,2,2,2,2,2,2,2,2,2,2,2,2,2,2,2,2,2,2,2,2,2,2,2,2,2,2,2,2,2,
2,2,2,2,2,2,2,2,2,2,2,2,2,2,2,2,2,2,2,2,2,2,2,2,2,2,2,2,2,2,2,2,2,2,2,2,
2,2,2,2,2,2,2,2,2,2,2,2,2,2,2,2,2,2,2,2,2,2,2,2,2,2,2,2,2,2,2,2,2,2,2,2,
2,2,2,2,2,2,2,2,2,2,2,2,2,2,2,2,2,2,2,2,2,2,2,2,2,2,2,2,2,2,2,2,2,2,2,2,
2,2,2,2,2,2,2,2,2,2,2,2,2,2,2,2,2,2,2,2,2,2,2,2,2,2,2,2,2,2,2,2,2,2,2,2,
2,2,2,2,2,2,2,2,2,2,2,2,2,2,2,2,2,2,2,2,2,2,2,2,2,2,2,2,2,2,2,2,2,2,2,2,
4),(0.00175495097563408,0.0352625399406719,0.197360108617795,0.253608699459729,
0.274137831421876,0.284540307816254,0.291090370885871,0.296216182098079,
0.301785480521977,0.308860599834827,0.320319216837973,0.371350304294198,
0.436674209203219,0.471058084799032,0.485293161062722,0.495397622816899,
0.506513777457236,0.523788811408338,0.593857050788224,0.645243823011645,
0.675776901551024,0.688989513769135,0.696610806006971,0.702172600756485,
0.707502347824358,0.714198211852011,0.725673491290616,0.778350542453821,
0.782644126998547,0.882418987187402,0.933655256832732,0.954764872212928,
0.970598314027118,0.988147877967994,1.02602581308313,1.0712697490232,1.08942473941662,
1.08982884048817,1.09023277301792,1.09063663129866,1.09104051294525,1.09144451882367,
1.09157517239452,1.09171715794843,1.09187136545249,1.09203874037196,1.09222028517601,
1.09241706072286,1.09263018747407,1.09286084657252,1.09311028083545,1.09337979568197,
1.09367076006785,1.09398460752515,1.09432283737211,1.09468701623391,1.09507877994561,
1.09549983595649,1.09595196631501,1.09643703122404,1.0969569731285,1.10801517055347,
1.1223962736298,1.20753471703579,1.23311876062243,1.24910045041635,1.25707286181742,
1.25968093241407,1.28124030461214,1.33602465638445,1.44760942221458,1.47544015371053,
1.48852304799468,1.49647212012827,1.50243551124633,1.50842090095045,1.51497755266692,
1.52789598185376,1.5839778386596,1.63204744207204,1.67109965763502,1.69912000847182,
1.71240757755335,1.7225174825199,1.73410848898233,1.75361627552157,1.8181894524433,
1.8725488350463,1.89102387475517,1.90070279013383,1.9081864858002,1.91408237897576,
1.91917605973781,1.92628729049803,1.94633080341079,1.95083214455481,2.07858476422359,
2.20518474348015,2.22116889423628,2.23277651738855,2.24425943024408,2.25553366701155,
2.26970958505557,2.30551636427595,2.49938912017426,2.65901711994682,2.69853463434638,
2.70386637554691,2.70656479820441,2.70851570434621,2.71059091729695,2.71352458133718,
2.72140834618246,2.83658764567174,3.00040939141186,3.1246582500748,3.13440830470489,
3.13851197617747,3.14147020754299,3.14415895465361,3.14774327053315,3.15680295804168,
3.24890927194457,3.43790246844447,3.49385049845787,3.5232874633109,3.55416366803585,
3.55929913921458,3.5620297101123,3.56406071201076,3.56659589152047,3.57084018130091,
3.5849646110978,3.60917850321082,3.62918076345487,3.75799623904513,3.84812567182715,
3.91983489106167,3.93361836881346,3.9413085110774,3.94783915022913,3.95522986102456,
3.967630035295,4.01118304502898,4.05140509298979,4.12020746605273,4.20109216079533,
4.28369738842697,4.31726063527399,4.32257183516267,4.32533945489747,4.327589568565,
4.32983820038647,4.33392208256509,4.3466634704121,4.58536769347246,4.69172273248207,
4.73666401108837,4.7435554222001,4.74711699813715,4.7499972939198,4.75286392617472,
4.75803223062875,4.77390391493287,5.05627709492252,5.11325855885042,5.17229405399529,
5.17769174262378,5.18044835212201,5.18247690613933,5.18467086704538,5.1876452745471,
5.19441022531098,5.30168709418233,5.4964913320072,5.59555220571743,5.62506448040751,
5.6392917567656,5.65057292509323,5.66336876815058,5.68549874640199,5.81110591610013,
5.94204548835099,5.96390036591449,5.97126094232207,5.97640205841875,5.98223293598735,
5.99086700088689,6.01638172990783,6.04212509726058,6.12901010287418,6.1534241991619,
6.1661829252739,6.17669678700075,6.18917163010758,6.21275339876847,6.22944691034306,
6.28371868699829,6.36456173047886,6.3765056194844,6.38290610846679,6.38894542841228,
6.39725734210314,6.4173641758281,6.43402967186209,6.50292904282763,6.55352949228307,
6.60928860884352,6.62917724565551,6.64573248053629,6.6637233983993,6.69868752994647,
6.76567353545787,6.78130164492111,6.79215629301713,6.8127917352042,6.86091174150864,
6.90239216188215,6.92119599242194,6.93770625900967,6.95978757369098,7.01948714791512,
7.14094312901029,7.16892247457594,7.17856865200984,7.18424866420476,7.19021870124338,
7.19906483130723,7.23023236254152,7.30076375127872,7.36746137937351,7.38497608701334,
7.39510334423278,7.40575546678763,7.41999617638211,7.45440835533803,7.51473037295328,
7.57087991766468,7.58227458628751,7.58933212802182,7.59490048906351,7.60152077370934,
7.61537544191856,7.63406479057055,7.68262778203271,7.82251934479748,7.88815860391264,
7.90751965824174,7.91964916324831,7.9307745069614,7.94549359367843,7.97779488883906,
8.13216671623121,8.36358374414034,8.37904091615512,8.3832642057436,8.38574952740638,
8.38789972132987,8.39052529235364,8.395505046581,8.42752811672482,8.48146159713842,
8.64367310446665,8.80311868340908,8.81291476662083,8.81672126626415,8.81946711462304,
8.82238504936972,8.82625324933647,8.83468849200978,8.91758419458684,9.04022973465267,
9.22489764793346,9.23554697745061,9.23934449189476,9.2415358536265,9.24357090924747,
9.24634704820871,9.25169818356904,9.28628376534383,9.36875076707217,9.47836524403668,
9.50485501420989,9.59589938945606,9.61104968965221,9.61902732485961,9.62546043080808,
9.63157929807612,9.64155373233103,9.66824360650781,9.79991339906604,9.98219948507729,
9.99796931467612,10.0023460116868,10.0049361715052,10.0071860348159,10.0099446596262,
10.0152113752771,10.0498221746028,10.0797479890141,10.2255100735221),
 .UNSPECIFIED.);
#3205=B_SPLINE_CURVE_WITH_KNOTS('',3,(#168437,#168438,#168439,#168440,#168441,
#168442,#168443,#168444,#168445,#168446,#168447,#168448,#168449,#168450,
#168451),.UNSPECIFIED.,.F.,.F.,(4,1,1,1,1,1,1,1,1,1,1,1,4),(210.486707790517,
211.242325136762,211.74079368007,212.239262223377,212.737730766685,213.236199309992,
213.7346678533,214.233136396607,214.731604939915,215.230073483222,216.227010569838,
216.725479113145,216.769893097696),.UNSPECIFIED.);
#3206=B_SPLINE_CURVE_WITH_KNOTS('',3,(#168453,#168454,#168455,#168456,#168457,
#168458,#168459,#168460,#168461,#168462,#168463,#168464,#168465,#168466,
#168467,#168468,#168469,#168470,#168471,#168472,#168473,#168474,#168475,
#168476,#168477,#168478,#168479,#168480,#168481,#168482,#168483,#168484,
#168485,#168486,#168487,#168488,#168489,#168490,#168491,#168492,#168493,
#168494,#168495,#168496,#168497,#168498,#168499,#168500,#168501,#168502,
#168503,#168504,#168505,#168506,#168507,#168508,#168509,#168510,#168511,
#168512,#168513,#168514,#168515,#168516,#168517,#168518,#168519,#168520,
#168521,#168522,#168523,#168524,#168525,#168526,#168527,#168528,#168529,
#168530,#168531,#168532,#168533,#168534,#168535,#168536,#168537,#168538,
#168539,#168540,#168541,#168542,#168543,#168544,#168545,#168546,#168547,
#168548,#168549,#168550,#168551,#168552,#168553,#168554,#168555,#168556,
#168557,#168558,#168559,#168560,#168561,#168562,#168563,#168564,#168565,
#168566,#168567,#168568,#168569,#168570,#168571,#168572,#168573,#168574,
#168575,#168576,#168577,#168578,#168579,#168580,#168581,#168582,#168583,
#168584,#168585,#168586,#168587,#168588,#168589,#168590,#168591,#168592,
#168593,#168594,#168595,#168596,#168597,#168598,#168599,#168600,#168601,
#168602,#168603,#168604,#168605,#168606,#168607,#168608,#168609,#168610,
#168611,#168612,#168613,#168614,#168615,#168616,#168617,#168618,#168619,
#168620,#168621,#168622,#168623,#168624,#168625,#168626,#168627,#168628,
#168629,#168630,#168631,#168632,#168633,#168634,#168635,#168636,#168637,
#168638,#168639,#168640,#168641,#168642,#168643,#168644,#168645,#168646,
#168647,#168648,#168649,#168650,#168651,#168652,#168653,#168654,#168655,
#168656,#168657,#168658,#168659,#168660,#168661,#168662,#168663,#168664,
#168665,#168666,#168667,#168668,#168669,#168670,#168671,#168672,#168673,
#168674,#168675,#168676,#168677,#168678,#168679,#168680,#168681,#168682,
#168683,#168684,#168685,#168686,#168687,#168688,#168689,#168690,#168691,
#168692,#168693,#168694,#168695,#168696,#168697,#168698,#168699,#168700,
#168701,#168702,#168703,#168704,#168705,#168706,#168707,#168708),
 .UNSPECIFIED.,.F.,.F.,(4,3,3,3,3,3,3,3,3,3,3,3,3,3,3,3,3,3,3,3,3,3,3,3,
3,3,3,3,3,3,3,3,3,3,3,3,3,3,3,3,3,3,3,3,3,3,3,3,3,3,3,3,3,3,3,3,3,3,3,3,
3,3,3,3,3,3,3,3,3,3,3,3,3,3,3,3,3,3,3,3,3,3,3,3,3,4),(216.769893133811,
216.846463313756,216.923103012482,216.999878057372,217.076723021884,217.153710500839,
217.223947656453,217.300158236927,217.376300841179,217.452385927519,217.528423913791,
217.604425184346,217.681482629186,217.757447891311,217.833409483176,217.909376810237,
217.987253793445,218.063283590877,218.142084166973,218.220884743068,218.292308017918,
218.363678144831,218.435008716353,218.506322053838,218.577622740661,218.648948222153,
218.719353286375,218.807058775715,218.895235138133,218.98383954875,219.072539855632,
219.161136115566,219.217821829683,219.290791274133,219.363715265227,219.436606791968,
219.509488990889,219.582363908933,219.655266858643,219.71629037299,219.795591156939,
219.874914087416,219.954256689426,220.033629766598,220.113011447596,220.192408224704,
220.214758916298,220.294156310967,220.373539984795,220.452907436436,220.532252620248,
220.611575639514,220.690869869136,220.713227459606,220.786129859875,220.85900971692,
220.931879986353,221.004776330759,221.077684986544,221.150653299492,221.211696002913,
221.300270334525,221.388970699998,221.477537512099,221.565880925662,221.653650642287,
221.710164546221,221.781488044571,221.852791794727,221.924089297999,221.995421793646,
222.066770152385,222.138190807352,222.208633089528,222.283749424407,222.358810363004,
222.43382811189,222.511234398514,222.586208928398,222.661179643841,222.736157562242,
222.811153703102,222.886205945411,222.96129135231,223.036446415907,223.053078404876),
 .UNSPECIFIED.);
#3207=B_SPLINE_CURVE_WITH_KNOTS('',3,(#168710,#168711,#168712,#168713,#168714,
#168715,#168716,#168717,#168718,#168719,#168720,#168721,#168722,#168723,
#168724,#168725),.UNSPECIFIED.,.F.,.F.,(4,1,1,1,1,1,1,1,1,1,1,1,1,4),(223.053078404876,
223.205570176143,223.704038719451,224.202507262759,225.199444349374,225.697912892681,
226.196381435989,226.694849979296,227.193318522604,227.691787065911,228.190255609219,
228.688724152527,229.187192695834,229.336263712055),.UNSPECIFIED.);
#3208=B_SPLINE_CURVE_WITH_KNOTS('',3,(#168727,#168728,#168729,#168730,#168731,
#168732,#168733,#168734,#168735,#168736,#168737,#168738,#168739,#168740,
#168741,#168742,#168743,#168744,#168745,#168746,#168747,#168748,#168749,
#168750,#168751,#168752,#168753,#168754,#168755,#168756,#168757,#168758,
#168759,#168760,#168761,#168762,#168763,#168764,#168765,#168766,#168767,
#168768,#168769,#168770,#168771,#168772,#168773,#168774,#168775,#168776,
#168777,#168778,#168779,#168780,#168781,#168782,#168783,#168784,#168785,
#168786,#168787,#168788,#168789,#168790,#168791,#168792,#168793,#168794,
#168795,#168796,#168797,#168798,#168799,#168800,#168801,#168802,#168803,
#168804,#168805,#168806,#168807,#168808,#168809,#168810,#168811,#168812,
#168813,#168814,#168815,#168816,#168817,#168818,#168819,#168820,#168821,
#168822,#168823,#168824,#168825,#168826,#168827,#168828,#168829,#168830,
#168831,#168832,#168833,#168834,#168835,#168836,#168837,#168838,#168839,
#168840,#168841,#168842,#168843,#168844,#168845,#168846,#168847,#168848,
#168849,#168850,#168851,#168852,#168853,#168854,#168855,#168856,#168857,
#168858,#168859,#168860,#168861,#168862,#168863,#168864,#168865,#168866,
#168867,#168868,#168869,#168870,#168871,#168872,#168873,#168874,#168875,
#168876,#168877,#168878,#168879,#168880,#168881,#168882,#168883,#168884,
#168885,#168886,#168887,#168888,#168889,#168890,#168891,#168892,#168893,
#168894,#168895,#168896,#168897,#168898,#168899,#168900,#168901,#168902,
#168903,#168904,#168905,#168906,#168907,#168908,#168909,#168910,#168911,
#168912,#168913,#168914,#168915,#168916,#168917,#168918,#168919,#168920,
#168921,#168922,#168923,#168924,#168925,#168926,#168927,#168928,#168929,
#168930,#168931,#168932,#168933,#168934,#168935,#168936,#168937,#168938,
#168939,#168940,#168941,#168942,#168943,#168944,#168945,#168946,#168947,
#168948,#168949,#168950,#168951,#168952,#168953,#168954,#168955,#168956,
#168957,#168958,#168959,#168960,#168961,#168962,#168963,#168964,#168965,
#168966,#168967,#168968,#168969,#168970,#168971,#168972,#168973,#168974,
#168975,#168976,#168977,#168978,#168979,#168980,#168981,#168982),
 .UNSPECIFIED.,.F.,.F.,(4,3,3,3,3,3,3,3,3,3,3,3,3,3,3,3,3,3,3,3,3,3,3,3,
3,3,3,3,3,3,3,3,3,3,3,3,3,3,3,3,3,3,3,3,3,3,3,3,3,3,3,3,3,3,3,3,3,3,3,3,
3,3,3,3,3,3,3,3,3,3,3,3,3,3,3,3,3,3,3,3,3,3,3,3,3,4),(229.336263712055,
229.411092925826,229.485870339396,229.560608562626,229.638548715104,229.713256024592,
229.787964681614,229.862686074969,229.937431598213,230.012243669549,230.087094611738,
230.162026109137,230.184129782449,230.260262654694,230.336302355765,230.412258361136,
230.488116803673,230.563917867227,230.639657187961,230.682598325757,230.75834069058,
230.834128811329,230.909971982171,230.985926940431,231.061943372765,231.138079168265,
231.181066869064,231.257277449538,231.33342005379,231.40950514013,231.485543126402,
231.561544396957,231.638601841798,231.714567103922,231.790528695787,231.866496022848,
231.944373006056,232.020402803488,232.099203379584,232.178003955679,232.249427230529,
232.320797357442,232.392127928964,232.46344126645,232.534741953272,232.606067434765,
232.676472498987,232.764177988327,232.852354350746,232.940958761363,233.029659068245,
233.11825532818,233.174941042295,233.247910486745,233.320834477839,233.393726004581,
233.466608203502,233.539483121546,233.612386071256,233.673409585602,233.752710369551,
233.832033300026,233.911375902035,233.990748979207,234.070130660204,234.149527437312,
234.17187812891,234.251275523579,234.330659197407,234.410026649048,234.489371832861,
234.568694852128,234.647989081749,234.670346672217,234.743249072485,234.816128929531,
234.888999198964,234.961895543369,235.034804199154,235.107772512102,235.168815215525,
235.257873628456,235.34826747615,235.437366543456,235.528407781346,235.619449019235),
 .UNSPECIFIED.);
#3209=B_SPLINE_CURVE_WITH_KNOTS('',3,(#168984,#168985,#168986,#168987,#168988,
#168989,#168990,#168991,#168992,#168993,#168994,#168995,#168996,#168997,
#168998,#168999,#169000,#169001),.UNSPECIFIED.,.F.,.F.,(4,2,2,2,2,2,2,2,
4),(235.619449019235,236.448806795673,237.278164572111,238.107522348549,
238.936880124987,239.766237901425,240.595595677862,241.4249534543,241.902634326414),
 .UNSPECIFIED.);
#3210=B_SPLINE_CURVE_WITH_KNOTS('',3,(#169003,#169004,#169005,#169006,#169007,
#169008,#169009,#169010,#169011,#169012,#169013,#169014,#169015,#169016,
#169017),.UNSPECIFIED.,.F.,.F.,(4,1,1,1,1,1,1,1,1,1,1,1,4),(241.902634326414,
242.147374821831,242.645843365138,243.144311908446,244.141248995061,244.639717538368,
245.138186081676,246.135123168291,246.633591711599,247.132060254906,247.630528798214,
248.128997341521,248.1858196054),.UNSPECIFIED.);
#3211=B_SPLINE_CURVE_WITH_KNOTS('',3,(#169019,#169020,#169021,#169022,#169023,
#169024,#169025,#169026,#169027,#169028,#169029,#169030,#169031,#169032,
#169033,#169034,#169035,#169036,#169037,#169038,#169039,#169040,#169041,
#169042,#169043,#169044,#169045,#169046,#169047,#169048,#169049,#169050,
#169051,#169052,#169053,#169054,#169055,#169056,#169057,#169058,#169059,
#169060,#169061,#169062,#169063,#169064,#169065,#169066,#169067,#169068,
#169069,#169070,#169071,#169072,#169073,#169074,#169075,#169076,#169077,
#169078,#169079,#169080,#169081,#169082,#169083,#169084,#169085,#169086,
#169087,#169088,#169089,#169090,#169091,#169092,#169093,#169094,#169095,
#169096,#169097,#169098,#169099,#169100,#169101,#169102,#169103,#169104,
#169105,#169106,#169107,#169108,#169109,#169110,#169111,#169112,#169113,
#169114,#169115,#169116,#169117,#169118,#169119,#169120,#169121,#169122,
#169123,#169124,#169125,#169126,#169127,#169128,#169129,#169130,#169131,
#169132,#169133,#169134,#169135,#169136,#169137,#169138,#169139,#169140,
#169141,#169142,#169143,#169144,#169145,#169146,#169147,#169148,#169149,
#169150,#169151,#169152,#169153,#169154,#169155,#169156,#169157,#169158,
#169159,#169160,#169161,#169162,#169163,#169164,#169165,#169166,#169167,
#169168,#169169,#169170,#169171,#169172,#169173,#169174,#169175,#169176,
#169177,#169178,#169179,#169180,#169181,#169182,#169183,#169184,#169185,
#169186,#169187,#169188,#169189,#169190,#169191,#169192,#169193,#169194,
#169195,#169196,#169197,#169198,#169199,#169200,#169201,#169202,#169203,
#169204,#169205,#169206,#169207,#169208,#169209,#169210,#169211,#169212,
#169213,#169214,#169215,#169216,#169217,#169218,#169219,#169220,#169221,
#169222,#169223,#169224,#169225,#169226,#169227,#169228,#169229,#169230,
#169231,#169232,#169233,#169234,#169235,#169236,#169237,#169238,#169239,
#169240,#169241,#169242,#169243,#169244,#169245,#169246,#169247,#169248,
#169249,#169250,#169251,#169252,#169253,#169254,#169255,#169256,#169257,
#169258,#169259,#169260,#169261,#169262,#169263,#169264,#169265,#169266,
#169267,#169268,#169269,#169270,#169271),.UNSPECIFIED.,.F.,.F.,(4,3,3,3,
3,3,3,3,3,3,3,3,3,3,3,3,3,3,3,3,3,3,3,3,3,3,3,3,3,3,3,3,3,3,3,3,3,3,3,3,
3,3,3,3,3,3,3,3,3,3,3,3,3,3,3,3,3,3,3,3,3,3,3,3,3,3,3,3,3,3,3,3,3,3,3,3,
3,3,3,3,3,3,3,3,4),(248.185819633594,248.265215616196,248.34459622705,248.423955987765,
248.503293808868,248.582602862825,248.627465884829,248.700368285098,248.773248142143,
248.846118411576,248.919014755981,248.991923411766,249.064891724714,249.125934428136,
249.214508759749,249.303209125222,249.391775937325,249.48011935089,249.567889067515,
249.624402971444,249.695726469794,249.76703021995,249.838327723222,249.909660218868,
249.981008577608,250.052429232575,250.122871514752,250.198975010773,250.275028156844,
250.351041347079,250.427024946959,250.502989300287,250.580091712922,250.656063440961,
250.73204776822,250.808054109892,250.885992732761,250.962101772189,251.040955186778,
251.119808601367,251.195941473612,251.271981174683,251.347937180054,251.423795622591,
251.499596686144,251.575336006878,251.618277144674,251.694019509497,251.769807630246,
251.845650801089,251.921605759348,251.997622191683,252.073757987183,252.116745687982,
252.192956268456,252.269098872708,252.345183959048,252.42122194532,252.497223215875,
252.574280660715,252.65024592284,252.726207514705,252.802174841766,252.880051824974,
252.956081622406,253.034882198502,253.113682774597,253.185106049447,253.25647617636,
253.327806747881,253.399120085367,253.470420772189,253.541746253681,253.612151317904,
253.699856807244,253.788033169662,253.876637580279,253.965337887162,254.053934147096,
254.110619861212,254.183367085814,254.256062969947,254.328728085723,254.401385195274,
254.469004940773),.UNSPECIFIED.);
#3212=B_SPLINE_CURVE_WITH_KNOTS('',3,(#169273,#169274,#169275,#169276,#169277,
#169278,#169279,#169280,#169281,#169282,#169283,#169284,#169285,#169286,
#169287,#169288,#169289,#169290),.UNSPECIFIED.,.F.,.F.,(4,2,2,2,2,2,2,2,
4),(254.469004940773,255.298362717211,256.127720493649,256.957078270087,
257.786436046525,258.615793822963,259.445151599401,260.274509375839,260.752190247953),
 .UNSPECIFIED.);
#3213=B_SPLINE_CURVE_WITH_KNOTS('',3,(#169292,#169293,#169294,#169295,#169296,
#169297,#169298,#169299,#169300,#169301,#169302,#169303,#169304,#169305,
#169306,#169307,#169308,#169309,#169310,#169311,#169312,#169313,#169314,
#169315,#169316,#169317,#169318,#169319,#169320,#169321,#169322,#169323,
#169324,#169325,#169326,#169327,#169328,#169329,#169330,#169331,#169332,
#169333,#169334,#169335,#169336,#169337,#169338,#169339,#169340,#169341,
#169342,#169343,#169344,#169345,#169346,#169347,#169348,#169349,#169350,
#169351,#169352,#169353,#169354,#169355,#169356,#169357,#169358,#169359,
#169360,#169361,#169362,#169363,#169364,#169365,#169366,#169367,#169368,
#169369,#169370,#169371,#169372,#169373,#169374,#169375,#169376,#169377,
#169378,#169379,#169380,#169381,#169382,#169383,#169384,#169385,#169386,
#169387,#169388,#169389,#169390,#169391,#169392,#169393,#169394,#169395,
#169396,#169397,#169398,#169399,#169400,#169401,#169402,#169403,#169404,
#169405,#169406,#169407,#169408,#169409,#169410,#169411,#169412,#169413,
#169414,#169415,#169416,#169417,#169418,#169419,#169420,#169421,#169422,
#169423,#169424,#169425,#169426,#169427,#169428,#169429,#169430,#169431,
#169432,#169433,#169434,#169435,#169436,#169437,#169438,#169439,#169440,
#169441,#169442,#169443,#169444,#169445,#169446,#169447,#169448,#169449,
#169450,#169451,#169452,#169453,#169454,#169455,#169456,#169457,#169458,
#169459,#169460,#169461,#169462,#169463,#169464,#169465,#169466,#169467,
#169468,#169469,#169470,#169471,#169472,#169473,#169474,#169475,#169476,
#169477,#169478,#169479,#169480,#169481,#169482,#169483,#169484,#169485,
#169486,#169487,#169488,#169489,#169490,#169491,#169492,#169493,#169494,
#169495,#169496,#169497,#169498,#169499,#169500,#169501,#169502,#169503,
#169504,#169505,#169506,#169507,#169508,#169509,#169510,#169511,#169512,
#169513,#169514,#169515,#169516,#169517,#169518,#169519,#169520,#169521,
#169522,#169523,#169524,#169525,#169526,#169527,#169528,#169529,#169530,
#169531,#169532,#169533,#169534,#169535,#169536,#169537,#169538,#169539,
#169540,#169541,#169542,#169543,#169544,#169545,#169546,#169547,#169548,
#169549,#169550,#169551,#169552,#169553,#169554,#169555,#169556,#169557,
#169558,#169559,#169560,#169561,#169562,#169563,#169564,#169565,#169566,
#169567,#169568,#169569,#169570,#169571,#169572,#169573,#169574,#169575,
#169576,#169577,#169578,#169579,#169580,#169581,#169582,#169583,#169584,
#169585,#169586,#169587,#169588,#169589,#169590,#169591,#169592,#169593,
#169594,#169595,#169596,#169597,#169598,#169599,#169600,#169601,#169602,
#169603,#169604,#169605,#169606,#169607,#169608,#169609,#169610,#169611,
#169612,#169613,#169614,#169615,#169616,#169617,#169618,#169619,#169620,
#169621,#169622,#169623,#169624,#169625,#169626,#169627,#169628,#169629,
#169630,#169631,#169632,#169633,#169634,#169635,#169636,#169637,#169638,
#169639,#169640,#169641,#169642,#169643,#169644,#169645,#169646,#169647,
#169648,#169649,#169650,#169651,#169652,#169653,#169654,#169655,#169656,
#169657,#169658,#169659,#169660,#169661,#169662,#169663,#169664,#169665,
#169666,#169667,#169668,#169669,#169670,#169671,#169672,#169673,#169674,
#169675,#169676,#169677,#169678,#169679,#169680,#169681,#169682,#169683,
#169684,#169685,#169686,#169687,#169688,#169689,#169690,#169691,#169692,
#169693,#169694,#169695,#169696,#169697,#169698,#169699,#169700,#169701,
#169702,#169703,#169704,#169705,#169706,#169707,#169708,#169709,#169710,
#169711,#169712,#169713,#169714,#169715,#169716,#169717,#169718,#169719,
#169720,#169721,#169722,#169723,#169724,#169725,#169726,#169727,#169728,
#169729,#169730,#169731,#169732,#169733,#169734,#169735,#169736,#169737,
#169738,#169739,#169740,#169741,#169742,#169743,#169744,#169745,#169746,
#169747,#169748,#169749,#169750,#169751,#169752,#169753,#169754,#169755,
#169756,#169757,#169758,#169759,#169760,#169761,#169762,#169763,#169764,
#169765,#169766,#169767,#169768,#169769,#169770,#169771,#169772,#169773,
#169774,#169775,#169776,#169777,#169778,#169779,#169780,#169781,#169782,
#169783,#169784,#169785,#169786,#169787,#169788,#169789,#169790,#169791,
#169792,#169793,#169794,#169795,#169796,#169797,#169798,#169799,#169800,
#169801,#169802,#169803,#169804,#169805,#169806,#169807,#169808,#169809,
#169810,#169811,#169812,#169813,#169814,#169815,#169816,#169817,#169818,
#169819,#169820,#169821,#169822,#169823,#169824,#169825,#169826,#169827,
#169828,#169829,#169830,#169831,#169832,#169833,#169834,#169835,#169836,
#169837,#169838,#169839,#169840,#169841,#169842,#169843,#169844,#169845,
#169846,#169847,#169848,#169849,#169850,#169851,#169852,#169853,#169854,
#169855,#169856,#169857,#169858,#169859,#169860,#169861,#169862,#169863,
#169864,#169865,#169866,#169867,#169868,#169869,#169870,#169871,#169872,
#169873,#169874,#169875,#169876,#169877,#169878,#169879,#169880,#169881,
#169882,#169883,#169884,#169885,#169886,#169887,#169888,#169889,#169890,
#169891,#169892,#169893,#169894,#169895,#169896,#169897,#169898,#169899,
#169900,#169901,#169902,#169903,#169904,#169905,#169906,#169907,#169908,
#169909,#169910,#169911,#169912,#169913,#169914,#169915,#169916,#169917,
#169918,#169919,#169920,#169921,#169922,#169923,#169924,#169925,#169926,
#169927,#169928,#169929,#169930,#169931,#169932,#169933,#169934,#169935,
#169936,#169937,#169938,#169939,#169940,#169941,#169942,#169943,#169944,
#169945,#169946,#169947,#169948,#169949,#169950,#169951,#169952,#169953,
#169954,#169955,#169956,#169957,#169958,#169959,#169960,#169961,#169962,
#169963,#169964,#169965,#169966,#169967,#169968,#169969,#169970,#169971,
#169972,#169973,#169974,#169975,#169976,#169977,#169978,#169979,#169980,
#169981,#169982,#169983,#169984,#169985,#169986,#169987,#169988,#169989,
#169990,#169991,#169992,#169993,#169994,#169995,#169996,#169997,#169998,
#169999,#170000,#170001,#170002,#170003,#170004,#170005,#170006,#170007,
#170008,#170009,#170010,#170011,#170012,#170013,#170014,#170015,#170016,
#170017,#170018,#170019,#170020,#170021,#170022,#170023,#170024,#170025,
#170026,#170027,#170028,#170029,#170030,#170031,#170032,#170033,#170034,
#170035,#170036,#170037,#170038,#170039,#170040,#170041,#170042,#170043,
#170044,#170045,#170046,#170047,#170048,#170049,#170050,#170051,#170052,
#170053,#170054,#170055,#170056,#170057),.UNSPECIFIED.,.F.,.F.,(4,2,2,2,
2,2,2,2,2,2,2,2,2,2,2,2,2,2,2,2,2,2,2,2,2,2,2,2,2,2,2,2,2,2,2,2,2,2,2,2,
2,2,2,2,2,2,2,2,2,2,2,2,2,2,2,2,2,2,2,2,2,2,2,2,2,2,2,2,2,2,2,2,2,2,2,2,
2,2,2,2,2,2,2,2,2,2,2,2,2,2,2,2,2,2,2,2,2,2,2,2,2,2,2,2,2,2,2,2,2,2,2,2,
2,2,2,2,2,2,2,2,2,2,2,2,2,2,2,2,2,2,2,2,2,2,2,2,2,2,2,2,2,2,2,2,2,2,2,2,
2,2,2,2,2,2,2,2,2,2,2,2,2,2,2,2,2,2,2,2,2,2,2,2,2,2,2,2,2,2,2,2,2,2,2,2,
2,2,2,2,2,2,2,2,2,2,2,2,2,2,2,2,2,2,2,2,2,2,2,2,2,2,2,2,2,2,2,2,2,2,2,2,
2,2,2,2,2,2,2,2,2,2,2,2,2,2,2,2,2,2,2,2,2,2,2,2,2,2,2,2,2,2,2,2,2,2,2,2,
2,2,2,2,2,2,2,2,2,2,2,2,2,2,2,2,2,2,2,2,2,2,2,2,2,2,2,2,2,2,2,2,2,2,2,2,
2,2,2,2,2,2,2,2,2,2,2,2,2,2,2,2,2,2,2,2,2,2,2,2,2,2,2,2,2,2,2,2,2,2,2,2,
2,2,2,2,2,2,2,2,2,2,2,2,2,2,2,2,2,2,2,2,2,2,2,2,2,2,2,2,2,2,2,2,2,2,2,2,
2,2,2,2,2,2,2,2,2,2,2,2,2,2,2,2,2,2,4),(0.00175515510389137,0.233477217887913,
0.25413703343595,0.26458559800326,0.271154459994723,0.276282396962432,0.281849533512794,
0.288901966614316,0.300280715426606,0.357262708118248,0.415603903548912,
0.45085908282636,0.465215104594165,0.475293962475098,0.486357255560859,
0.503385792319506,0.564701835533945,0.6398356464392,0.661581926413047,0.672185324833179,
0.678797981477316,0.684240763060695,0.690212940547745,0.697982880634005,
0.71123025721564,0.791283504926808,0.866715769811109,0.914874922190495,
0.935584029401951,0.951600003526206,0.968969172068741,1.00932986584437,
1.06420270912661,1.06459270061813,1.06497063122061,1.06533745121251,1.06569402661649,
1.06604114927938,1.0663795455561,1.06670988380967,1.0670327809382,1.06734880806243,
1.0676584955139,1.06796233720735,1.06826079452005,1.06855429971448,1.06884325898597,
1.06912805519464,1.06940905029064,1.06968658751496,1.06996099338418,1.07023257948723,
1.07050164412487,1.07076847380039,1.07103334460418,1.07129652347151,1.07155826937261,
1.07181883440759,1.0720784648375,1.072337402053,1.0725958834945,1.07285414354116,
1.07311241434677,1.07337092666556,1.07362991063493,1.07388959655672,1.07415021567128,
1.07441200091583,1.07467518767515,1.07494001454384,1.07520672410221,1.07547556369038,
1.07574678619495,1.07602065087022,1.07629742416933,1.07657738060112,1.07686080361825,
1.08781962073341,1.10197716490331,1.15002880852661,1.18625581917963,1.21257682033107,
1.22824407953828,1.2449993049137,1.27056306991027,1.39867339113269,1.44524476935404,
1.46333843076665,1.47584638964651,1.47585815312406,1.47586991439948,1.47588167353886,
1.47589343053064,1.47590518543313,1.47591693828364,1.47592868900168,1.47594043759191,
1.47595218416309,1.4759639286548,1.47597567104591,1.47598741141739,1.47599914969255,
1.47601088592738,1.47602262012269,1.4760343523083,1.47604608250151,1.47605781074983,
1.4760695369906,1.47608126127869,1.47609298362109,1.47610470397389,1.47611642236231,
1.47612813880026,1.47613985331399,1.47615156591528,1.47616327665493,1.47617498546208,
1.47618669242915,1.4761983974872,1.47621010062884,1.47622180192393,1.47623350133894,
1.47624519889774,1.47625689464955,1.4762685885908,1.47628028073621,1.47629197106438,
1.47630365961983,1.47631534644594,1.4763270314473,1.47633871472641,1.47635039624674,
1.4763620760455,1.4763737541165,1.47638543049538,1.47639710516244,1.47640877814654,
1.47642044938156,1.47643211898983,1.47644378683111,1.47645545303301,1.47646711759522,
1.47647878053287,1.47649044188986,1.47650210161836,1.47651375972637,1.47652541618465,
1.47653707105855,1.47654872438652,1.4765603761387,1.47657202634678,1.47658367504197,
1.47659532223396,1.47660696788615,1.48257240671224,1.48855891242022,1.49511239671956,
1.50801037252183,1.5634835740125,1.61004197639941,1.63133733756868,1.67389501185857,
1.6892645502926,1.69922365512451,1.70935745468947,1.72436020873488,1.76382280958394,
1.84609078677853,1.86825711214699,1.8791488358587,1.88678270785041,1.89214181958446,
1.89712855586481,1.90401414228836,1.91933549196333,2.05051976628145,2.14045537791271,
2.17604001437676,2.19540302882133,2.20835915391724,2.22074635752232,2.22078260957332,
2.22081900314508,2.2208555396054,2.23176488230404,2.24609451722107,2.2761792622228,
2.37728760371622,2.58709277620618,2.67603376760491,2.68311216447253,2.68614184150776,
2.68834541786443,2.69036122329734,2.69306796494391,2.69959586351883,2.8055016929206,
2.95583583270476,3.10677991989484,3.11521508027641,3.11908303531526,3.12200068954504,
3.12474623967715,3.12855228198413,3.13624469868799,3.2088398194217,3.25521222803167,
3.45867078089983,3.48681670119209,3.5286285783174,3.5376978331576,3.54113789529451,
3.54349635396022,3.54579847973153,3.54856463728212,3.55542538286991,3.62938312966554,
3.87440341521721,3.90644803481321,3.91712992632398,3.92414739352503,3.93073506575537,
3.93905435529049,3.95533569309754,4.12316938130341,4.16704554026442,4.28491574368914,
4.30007338439049,4.30424803637416,4.3067675632827,4.30902613948356,4.31188890947859,
4.31766152280319,4.35811393803448,4.37097403415593,4.39865388396153,4.62303097563096,
4.71566436585532,4.72362076631482,4.72739693827814,4.73030072319465,4.73307492052381,
4.73778090938272,4.75040116928648,4.9593422547546,5.07893771558406,5.11367129404802,
5.15331585190229,5.15884497898514,5.16158380561712,5.16374311567003,5.16615037184357,
5.17013544370944,5.18456712682551,5.29649760092421,5.4431241269617,5.56966840778963,
5.60322224863298,5.61799147295701,5.6293651187069,5.64173231640786,5.661854789329,
5.74119636823205,5.83015418058168,5.93016731041987,5.94650556636355,5.95349327340243,
5.95903657991471,5.96567826631202,5.97819338784467,6.02544957701399,6.11361693750067,
6.13528811288873,6.14749318726828,6.15801978640242,6.17109926704762,6.19793600523263,
6.21794073482931,6.29117843336744,6.34759750657495,6.35777166329348,6.36328461872042,
6.36938176163861,6.37801321498269,6.40023911392053,6.48552621733961,6.53204991383895,
6.58885642938433,6.60888601772983,6.62546853419877,6.64338734369971,6.67767451557907,
6.73366769184109,6.75393387992771,6.76519738058678,6.77890519915598,6.82326897067486,
6.87933026136105,6.89906914405145,6.91385486732147,6.93375865598872,6.97628364780968,
7.00961022733493,7.07042720479597,7.07740954194317,7.0969449960031,7.1454868082527,
7.15679494648413,7.16345505888059,7.16937602255614,7.17759268574359,7.20239410292237,
7.24833049987884,7.34187808713147,7.3622144920666,7.37404282418338,7.38356079744233,
7.39665914385762,7.4237882756603,7.46202336420416,7.53433530408394,7.55809713228422,
7.56590552075492,7.57130756773959,7.57691744331908,7.58506318876277,7.60862790139616,
7.62979070396718,7.72361099869899,7.79631111824225,7.86697847717529,7.88678330214175,
7.89901298487519,7.91010975546727,7.92461905636662,7.95571488185342,8.09650862064676,
8.33256820221607,8.3573507268996,8.36189061219046,8.36469692759916,8.36686475342219,
8.36923646362575,8.37306162192178,8.3859218083503,8.46890109816707,8.64294715347879,
8.78291563982107,8.79256563867432,8.79634738452495,8.79908644324316,8.80200747254907,
8.80589738368821,8.81420847091793,8.88890657519997,9.00435405993594,9.20295840426713,
9.21477221130106,9.21873385251936,9.22095787865279,9.22319013651098,9.2259944467728,
9.23148175640772,9.26993303922492,9.33011201574586,9.46706674441134,9.57459592702731,
9.59026327815184,9.59843681238614,9.6047593279856,9.61172843283533,9.62218051806888,
9.65239298224312,9.86570930835225,9.97338547415581,9.98039934692653,9.98319056743156,
9.98549922691861,9.9878498695486,9.99125223818228,10.0000748706393,10.0399943403384,
10.2253631395449),.UNSPECIFIED.);
#3214=B_SPLINE_CURVE_WITH_KNOTS('',3,(#170059,#170060,#170061,#170062,#170063,
#170064,#170065,#170066,#170067,#170068,#170069,#170070,#170071,#170072,
#170073),.UNSPECIFIED.,.F.,.F.,(4,1,1,1,1,1,1,1,1,1,1,1,4),(273.318560862312,
274.049361593514,274.547830136822,275.046298680129,275.544767223437,276.043235766745,
276.541704310052,277.04017285336,277.538641396667,278.037109939975,279.03404702659,
279.532515569897,279.601746169492),.UNSPECIFIED.);
#3215=B_SPLINE_CURVE_WITH_KNOTS('',3,(#170075,#170076,#170077,#170078,#170079,
#170080,#170081,#170082,#170083,#170084,#170085,#170086,#170087,#170088),
 .UNSPECIFIED.,.F.,.F.,(4,1,1,1,1,1,1,1,1,1,1,4),(279.601746169492,280.030984113205,
281.02792119982,281.526389743128,282.024858286435,282.523326829743,283.02179537305,
283.520263916358,284.018732459666,284.517201002973,285.015669546281,285.884931476671),
 .UNSPECIFIED.);
#3216=B_SPLINE_CURVE_WITH_KNOTS('',3,(#170090,#170091,#170092,#170093,#170094,
#170095,#170096,#170097,#170098,#170099,#170100,#170101,#170102,#170103,
#170104,#170105),.UNSPECIFIED.,.F.,.F.,(4,1,1,1,1,1,1,1,1,1,1,1,1,4),(285.884931476671,
286.012606632896,286.511075176203,287.009543719511,288.006480806126,288.504949349434,
289.003417892741,289.501886436049,290.000354979356,290.498823522664,290.997292065971,
291.495760609279,291.994229152586,292.168116783851),.UNSPECIFIED.);
#3217=B_SPLINE_CURVE_WITH_KNOTS('',3,(#170107,#170108,#170109,#170110,#170111,
#170112,#170113,#170114,#170115,#170116,#170117,#170118,#170119,#170120,
#170121,#170122,#170123,#170124,#170125,#170126,#170127,#170128,#170129,
#170130,#170131,#170132,#170133,#170134,#170135,#170136,#170137,#170138,
#170139,#170140,#170141,#170142,#170143,#170144,#170145,#170146,#170147,
#170148,#170149,#170150,#170151,#170152,#170153,#170154,#170155,#170156,
#170157,#170158,#170159,#170160,#170161,#170162,#170163,#170164,#170165,
#170166,#170167,#170168,#170169,#170170,#170171,#170172,#170173,#170174,
#170175,#170176,#170177,#170178,#170179,#170180,#170181,#170182,#170183,
#170184,#170185,#170186,#170187,#170188,#170189,#170190,#170191,#170192,
#170193,#170194,#170195,#170196,#170197,#170198,#170199,#170200,#170201,
#170202,#170203,#170204,#170205,#170206,#170207,#170208,#170209,#170210,
#170211,#170212,#170213,#170214,#170215,#170216,#170217,#170218,#170219,
#170220,#170221,#170222,#170223,#170224,#170225,#170226,#170227,#170228,
#170229,#170230,#170231,#170232,#170233,#170234,#170235,#170236,#170237,
#170238,#170239,#170240,#170241,#170242,#170243,#170244,#170245,#170246,
#170247,#170248,#170249,#170250,#170251,#170252,#170253,#170254,#170255,
#170256,#170257,#170258,#170259,#170260,#170261,#170262,#170263,#170264,
#170265,#170266,#170267,#170268,#170269,#170270,#170271,#170272,#170273,
#170274,#170275,#170276,#170277,#170278,#170279,#170280,#170281,#170282,
#170283,#170284,#170285,#170286,#170287,#170288,#170289,#170290,#170291,
#170292,#170293,#170294,#170295,#170296,#170297,#170298,#170299,#170300,
#170301,#170302,#170303,#170304,#170305,#170306,#170307,#170308,#170309,
#170310,#170311,#170312,#170313,#170314,#170315,#170316,#170317,#170318,
#170319,#170320,#170321,#170322,#170323,#170324,#170325,#170326,#170327,
#170328,#170329,#170330,#170331,#170332,#170333,#170334,#170335,#170336,
#170337,#170338,#170339,#170340,#170341,#170342,#170343,#170344,#170345,
#170346,#170347,#170348,#170349,#170350,#170351,#170352,#170353,#170354,
#170355,#170356,#170357,#170358,#170359,#170360,#170361,#170362),
 .UNSPECIFIED.,.F.,.F.,(4,3,3,3,3,3,3,3,3,3,3,3,3,3,3,3,3,3,3,3,3,3,3,3,
3,3,3,3,3,3,3,3,3,3,3,3,3,3,3,3,3,3,3,3,3,3,3,3,3,3,3,3,3,3,3,3,3,3,3,3,
3,3,3,3,3,3,3,3,3,3,3,3,3,3,3,3,3,3,3,3,3,3,3,3,3,4),(292.168116783851,
292.242892619617,292.317620259225,292.392312354933,292.467169090467,292.541838664995,
292.616512565346,292.691202226417,292.766193229613,292.840977674388,292.916071956795,
292.991166239202,293.067299111447,293.143338812519,293.21929481789,293.295153260427,
293.370954323981,293.446693644715,293.489634782509,293.565377147332,293.641165268081,
293.717008438923,293.792963397183,293.868979829517,293.945115625018,293.988103325817,
294.064313906291,294.140456510543,294.216541596883,294.292579583156,294.368580853711,
294.445638298551,294.521603560676,294.59756515254,294.673532479602,294.751409462809,
294.827439260242,294.906239836337,294.985040412432,295.056463687282,295.127833814195,
295.199164385717,295.270477723203,295.341778410025,295.413103891517,295.483508955739,
295.571214445079,295.659390807497,295.747995218113,295.836695524995,295.92529178493,
295.981977499047,296.054946943497,296.127870934591,296.200762461333,296.273644660254,
296.346519578297,296.419422528008,296.480446042354,296.559746826303,296.63906975678,
296.71841235879,296.797785435963,296.87716711696,296.956563894069,296.978914585662,
297.058311980331,297.13769565416,297.217063105802,297.296408289614,297.37573130888,
297.455025538502,297.47738312897,297.550285529238,297.623165386283,297.696035655715,
297.76893200012,297.841840655905,297.914808968853,297.975851672277,298.064621143056,
298.153528187369,298.242313953431,298.330875461396,298.418895475305,298.45130209103),
 .UNSPECIFIED.);
#3218=B_SPLINE_CURVE_WITH_KNOTS('',3,(#170364,#170365,#170366,#170367,#170368,
#170369,#170370,#170371,#170372,#170373,#170374,#170375,#170376,#170377,
#170378,#170379,#170380,#170381,#170382,#170383,#170384,#170385,#170386,
#170387,#170388,#170389,#170390,#170391,#170392,#170393,#170394,#170395,
#170396,#170397,#170398,#170399,#170400,#170401,#170402,#170403,#170404,
#170405,#170406,#170407,#170408,#170409,#170410,#170411,#170412,#170413,
#170414,#170415,#170416,#170417,#170418,#170419,#170420,#170421,#170422,
#170423,#170424,#170425,#170426,#170427,#170428,#170429,#170430,#170431,
#170432,#170433,#170434,#170435,#170436,#170437,#170438,#170439,#170440,
#170441,#170442,#170443,#170444,#170445,#170446,#170447,#170448,#170449,
#170450,#170451,#170452,#170453,#170454,#170455,#170456,#170457,#170458,
#170459,#170460,#170461,#170462,#170463,#170464,#170465,#170466,#170467,
#170468,#170469,#170470,#170471,#170472,#170473,#170474,#170475,#170476,
#170477,#170478,#170479,#170480,#170481,#170482,#170483,#170484,#170485,
#170486,#170487,#170488,#170489,#170490,#170491,#170492,#170493,#170494,
#170495,#170496,#170497,#170498,#170499,#170500,#170501,#170502,#170503,
#170504,#170505,#170506,#170507,#170508,#170509,#170510,#170511,#170512,
#170513,#170514,#170515,#170516,#170517,#170518,#170519,#170520,#170521,
#170522,#170523,#170524,#170525,#170526,#170527,#170528,#170529,#170530,
#170531,#170532,#170533,#170534,#170535,#170536,#170537,#170538,#170539,
#170540,#170541,#170542,#170543,#170544,#170545,#170546,#170547,#170548,
#170549,#170550,#170551,#170552,#170553,#170554,#170555,#170556,#170557,
#170558,#170559,#170560,#170561,#170562,#170563,#170564,#170565,#170566,
#170567,#170568,#170569,#170570,#170571,#170572,#170573,#170574,#170575,
#170576,#170577,#170578,#170579,#170580,#170581,#170582,#170583,#170584,
#170585,#170586,#170587,#170588,#170589,#170590,#170591,#170592,#170593,
#170594,#170595,#170596,#170597,#170598,#170599,#170600,#170601,#170602,
#170603,#170604,#170605,#170606,#170607,#170608,#170609,#170610,#170611,
#170612,#170613,#170614,#170615,#170616,#170617,#170618,#170619,#170620,
#170621,#170622,#170623,#170624,#170625,#170626,#170627,#170628,#170629,
#170630,#170631,#170632,#170633,#170634,#170635,#170636,#170637,#170638,
#170639,#170640,#170641,#170642,#170643,#170644,#170645,#170646,#170647,
#170648,#170649,#170650,#170651,#170652,#170653,#170654,#170655,#170656,
#170657,#170658,#170659,#170660,#170661,#170662,#170663,#170664,#170665,
#170666,#170667,#170668,#170669,#170670,#170671,#170672,#170673,#170674,
#170675,#170676,#170677,#170678,#170679,#170680,#170681,#170682,#170683,
#170684,#170685,#170686,#170687,#170688,#170689,#170690,#170691,#170692,
#170693,#170694,#170695,#170696,#170697,#170698,#170699,#170700,#170701,
#170702,#170703,#170704,#170705,#170706,#170707,#170708,#170709,#170710,
#170711,#170712,#170713,#170714,#170715,#170716,#170717,#170718,#170719,
#170720,#170721,#170722,#170723,#170724,#170725,#170726,#170727,#170728,
#170729,#170730,#170731,#170732,#170733,#170734,#170735,#170736,#170737,
#170738,#170739,#170740,#170741,#170742,#170743,#170744,#170745,#170746,
#170747,#170748,#170749,#170750,#170751,#170752,#170753,#170754,#170755,
#170756,#170757,#170758,#170759,#170760,#170761,#170762,#170763,#170764,
#170765,#170766,#170767,#170768,#170769,#170770,#170771,#170772,#170773,
#170774,#170775,#170776,#170777,#170778,#170779,#170780,#170781,#170782,
#170783,#170784,#170785,#170786,#170787,#170788,#170789,#170790,#170791,
#170792,#170793,#170794,#170795,#170796,#170797,#170798,#170799,#170800,
#170801,#170802,#170803,#170804,#170805,#170806,#170807,#170808,#170809,
#170810,#170811,#170812,#170813,#170814,#170815,#170816,#170817,#170818,
#170819,#170820,#170821,#170822,#170823,#170824,#170825,#170826,#170827,
#170828,#170829,#170830,#170831,#170832,#170833,#170834,#170835,#170836,
#170837,#170838,#170839,#170840,#170841,#170842,#170843,#170844,#170845,
#170846,#170847,#170848,#170849,#170850,#170851,#170852,#170853,#170854,
#170855,#170856,#170857,#170858,#170859,#170860,#170861,#170862,#170863,
#170864,#170865,#170866,#170867,#170868,#170869,#170870,#170871,#170872,
#170873,#170874,#170875,#170876,#170877,#170878,#170879,#170880,#170881,
#170882,#170883,#170884,#170885,#170886,#170887,#170888,#170889,#170890,
#170891,#170892,#170893,#170894,#170895,#170896,#170897),.UNSPECIFIED.,
 .F.,.F.,(4,2,2,2,2,2,2,2,2,2,2,2,2,2,2,2,2,2,2,2,2,2,2,2,2,2,2,2,2,2,2,
2,2,2,2,2,2,2,2,2,2,2,2,2,2,2,2,2,2,2,2,2,2,2,2,2,2,2,2,2,2,2,2,2,2,2,2,
2,2,2,2,2,2,2,2,2,2,2,2,2,2,2,2,2,2,2,2,2,2,2,2,2,2,2,2,2,2,2,2,2,2,2,2,
2,2,2,2,2,2,2,2,2,2,2,2,2,2,2,2,2,2,2,2,2,2,2,2,2,2,2,2,2,2,2,2,2,2,2,2,
2,2,2,2,2,2,2,2,2,2,2,2,2,2,2,2,2,2,2,2,2,2,2,2,2,2,2,2,2,2,2,2,2,2,2,2,
2,2,2,2,2,2,2,2,2,2,2,2,2,2,2,2,2,2,2,2,2,2,2,2,2,2,2,2,2,2,2,2,2,2,2,2,
2,2,2,2,2,2,2,2,2,2,2,2,2,2,2,2,2,2,2,2,2,2,2,2,2,2,2,2,2,2,2,2,2,2,2,2,
2,2,2,2,2,2,2,2,2,2,2,2,2,2,2,2,2,2,2,4),(0.00122791027254725,0.0770820827091792,
0.249473293479002,0.35938565459511,0.396222145161444,0.401470223157442,
0.404151400110561,0.406285224019235,0.408410814910348,0.412196213564084,
0.423475551746603,0.602149485012172,0.659425583079787,0.677777713760731,
0.704614520043833,0.823643580796911,0.832382970895941,0.836307131751904,
0.83923348903228,0.841962843712299,0.845708201067346,0.855144521174502,
0.979824151879159,1.05588477287752,1.17520667966232,1.24210984092913,1.25397834072015,
1.25779707324021,1.26023699649726,1.2625174720715,1.26549224401887,1.27048069588069,
1.30077755015236,1.42946571425106,1.53656613983677,1.58858242833206,1.610956029209,
1.62309297067942,1.63366928033205,1.64056720086361,1.64673459641745,1.65473566225044,
1.66678353740102,1.72157774112728,1.76395016251119,1.91948843800925,2.0043737721778,
2.0171235096307,2.02104482676514,2.02350753158127,2.0257799452495,2.02870241098462,
2.03493914970703,2.09505126887309,2.14929829547459,2.27094440408111,2.43123907130445,
2.43970363795816,2.44357682189537,2.44649501217603,2.4492385319426,2.4530377241848,
2.46279293163981,2.61559574606392,2.79152728449851,2.86112861009212,2.87285807117308,
2.87655489027948,2.87889784844497,2.88107441616306,2.88389483183564,2.88858367266565,
2.91600477782473,3.07519780857927,3.2838046531056,3.31901744763817,3.33421568568152,
3.34561465457157,3.35790744572186,3.37768042746172,3.44354325987826,3.58315168023071,
3.63171911978052,3.65040882157333,3.66426321037291,3.67088300815463,3.67645076278207,
3.68350732620053,3.69489996863144,3.7510813816026,3.80996282193589,3.84539816707146,
3.85977915942087,3.87045071776729,3.88053485765473,3.89781657101398,3.95876325979922,
4.03434661989895,4.0665096349813,4.07543900336064,4.081416536214,4.08708021207258,
4.09505547764317,4.11715568455006,4.24506756066764,4.30569274491526,4.32786694565951,
4.34438577868516,4.36313385068249,4.42998159343901,4.46793891923492,4.48120285085966,
4.49455810178358,4.55445365760738,4.58542587726186,4.60946657218916,4.62613071232053,
4.64427836545532,4.67623618368438,4.70663472748092,4.7373624594192,4.81561241655197,
4.84025709922769,4.86642423927287,4.87558460205099,4.88178618611138,4.88720679323757,
4.89660711334873,4.93103608333354,5.02615194728681,5.05482932556069,5.07725386175143,
5.08950182858655,5.10002505632894,5.11305050546241,5.13976166004577,5.1771318085889,
5.22058818729292,5.27139924944099,5.28168312523945,5.28725146017345,5.2922596135758,
5.29944319754572,5.31648707991604,5.34102676807479,5.46085939185313,5.57978880817953,
5.60179261053654,5.61468668116615,5.62595418018708,5.64003114539705,5.66872970313352,
5.788362176433,5.95823962779432,6.05306548968299,6.0741849720216,6.07848847249037,
6.08122261170812,6.0833814236841,6.08579146829691,6.0897887433754,6.10433480837078,
6.21618231086416,6.42404036705696,6.5010029633691,6.50968361712007,6.51320547988452,
6.51614647868682,6.51916762023086,6.52358833811566,6.53531831464861,6.59141922782749,
6.71389724819145,6.91950030055133,6.93115959405315,6.93510073760973,6.93732040167437,
6.93955303450742,6.94236501532933,6.94789084758862,6.98756279271893,7.05058094010175,
7.2790725721291,7.30276588050363,7.31157743500253,7.31787243245515,7.32376954551401,
7.3314900735133,7.34542178253661,7.42027116082209,7.51692417093367,7.67635742431983,
7.69356773735894,7.69808839982265,7.70071146794937,7.70295843532122,7.70567442477478,
7.70853673660549,7.71300050279924,7.72136320684039,7.79747418562558,7.93128789258829,
8.10604481814092,8.11631022754147,8.1201927066759,8.12295826933843,8.12586521562977,
8.12966567965862,8.13774893473,8.24094238431121,8.40820621626666,8.54261131083952,
8.55114852540975,8.55452114093056,8.55656512754395,8.55874796400886,8.56165906580973,
8.5680802936016,8.5767049402225,8.6679032131965,8.76219829244233,8.95939214377268,
8.99508448427386,9.00924348783601,9.02080950713053,9.03134619390067,9.04662060841632,
9.08202327295041,9.13336157038587,9.22333375485016,9.32338677381066,9.33966071708891,
9.34627494337092,9.35185710994299,9.35716155295603,9.36486048767306,9.3751531169544,
9.39546283920925,9.46184059702045,9.51748793901424,9.53378365225853,9.544685548757,
9.55456395319087,9.56512369349176,9.59237362292246,9.61281862834854,9.70805983410475,
9.742769081438,9.7521998228333,9.7576230284564,9.7632589780941,9.76944815665706,
9.77803153874953,9.79275870214336,9.82617109120628,9.90426362675867,9.97874077013341,
10.0026568325412,10.019234100866,10.0339356097584,10.0621071748144,10.1037487198327,
10.1424488115996,10.1567160209096,10.1677229097695,10.1830828621877,10.2246332076101),
 .UNSPECIFIED.);
#3219=B_SPLINE_CURVE_WITH_KNOTS('',3,(#170899,#170900,#170901,#170902,#170903,
#170904,#170905,#170906,#170907,#170908,#170909,#170910,#170911,#170912),
 .UNSPECIFIED.,.F.,.F.,(4,1,1,1,1,1,1,1,1,1,1,4),(311.017745311523,311.434502341581,
311.932970884889,312.431439428196,312.929907971504,313.926845058119,314.425313601427,
314.923782144734,315.920719231349,316.419187774657,316.917656317964,317.300850558385),
 .UNSPECIFIED.);
#3220=B_SPLINE_CURVE_WITH_KNOTS('',3,(#170914,#170915,#170916,#170917,#170918,
#170919,#170920,#170921,#170922,#170923,#170924,#170925,#170926,#170927,
#170928,#170929,#170930,#170931),.UNSPECIFIED.,.F.,.F.,(4,2,2,2,2,2,2,2,
4),(317.300858012569,318.130215789007,318.959573565445,319.788931341883,
320.618289118321,321.447646894759,322.277004671197,323.106362447635,323.584043319749),
 .UNSPECIFIED.);
#3221=B_SPLINE_CURVE_WITH_KNOTS('',3,(#170933,#170934,#170935,#170936,#170937,
#170938,#170939,#170940,#170941,#170942,#170943,#170944,#170945,#170946,
#170947,#170948,#170949,#170950,#170951,#170952,#170953,#170954,#170955,
#170956,#170957,#170958,#170959,#170960,#170961,#170962,#170963,#170964,
#170965,#170966,#170967,#170968,#170969,#170970,#170971,#170972,#170973,
#170974,#170975,#170976,#170977,#170978,#170979,#170980,#170981,#170982,
#170983,#170984,#170985,#170986,#170987),.UNSPECIFIED.,.F.,.F.,(4,3,3,3,
3,3,3,3,3,3,3,3,3,3,3,3,3,3,4),(323.584043319749,323.665206603477,323.746378549093,
323.82754791565,323.89621592427,323.972076794865,324.047910661161,324.12372725779,
324.199547384246,324.275367646974,324.351214673505,324.394684467578,324.473160269805,
324.551626766589,324.630085813129,324.708544612275,324.786997107681,324.865450438762,
324.893153010885),.UNSPECIFIED.);
#3222=B_SPLINE_CURVE_WITH_KNOTS('',3,(#170991,#170992,#170993,#170994,#170995,
#170996,#170997,#170998),.UNSPECIFIED.,.F.,.F.,(4,2,2,4),(323.584043319749,
324.413401096187,325.242758872624,325.416526282203),.UNSPECIFIED.);
#3223=B_SPLINE_CURVE_WITH_KNOTS('',3,(#171000,#171001,#171002,#171003,#171004,
#171005,#171006,#171007,#171008,#171009,#171010,#171011,#171012,#171013,
#171014),.UNSPECIFIED.,.F.,.F.,(4,1,1,1,1,1,1,1,1,1,1,1,4),(317.300858012569,
317.467727907809,318.464664994424,318.963133537731,319.461602081039,319.960070624347,
320.458539167654,320.957007710962,321.455476254269,321.953944797577,322.452413340884,
323.449350427499,323.584043319749),.UNSPECIFIED.);
#3224=B_SPLINE_CURVE_WITH_KNOTS('',3,(#171016,#171017,#171018,#171019,#171020,
#171021,#171022,#171023,#171024,#171025,#171026,#171027,#171028,#171029,
#171030,#171031,#171032,#171033,#171034,#171035,#171036,#171037,#171038,
#171039,#171040,#171041,#171042,#171043,#171044,#171045,#171046,#171047,
#171048,#171049,#171050,#171051,#171052,#171053,#171054,#171055,#171056,
#171057,#171058,#171059,#171060,#171061,#171062,#171063,#171064,#171065,
#171066,#171067,#171068,#171069,#171070,#171071,#171072,#171073,#171074,
#171075,#171076,#171077,#171078,#171079,#171080,#171081,#171082,#171083,
#171084,#171085,#171086,#171087,#171088,#171089,#171090,#171091,#171092,
#171093,#171094,#171095,#171096,#171097,#171098,#171099,#171100,#171101,
#171102,#171103,#171104,#171105,#171106,#171107,#171108,#171109,#171110,
#171111,#171112,#171113,#171114,#171115,#171116,#171117,#171118,#171119,
#171120,#171121,#171122,#171123,#171124,#171125,#171126,#171127,#171128,
#171129,#171130,#171131,#171132,#171133,#171134,#171135,#171136,#171137,
#171138,#171139,#171140,#171141,#171142,#171143,#171144,#171145,#171146,
#171147,#171148,#171149,#171150,#171151,#171152,#171153,#171154,#171155,
#171156,#171157,#171158,#171159,#171160,#171161,#171162,#171163,#171164,
#171165,#171166,#171167,#171168,#171169,#171170,#171171,#171172,#171173,
#171174,#171175,#171176,#171177,#171178,#171179,#171180,#171181,#171182,
#171183,#171184,#171185,#171186,#171187,#171188,#171189,#171190,#171191,
#171192,#171193,#171194,#171195,#171196,#171197,#171198,#171199,#171200,
#171201,#171202,#171203,#171204,#171205,#171206,#171207,#171208,#171209,
#171210,#171211,#171212,#171213,#171214,#171215,#171216,#171217,#171218,
#171219,#171220,#171221,#171222,#171223,#171224,#171225,#171226,#171227,
#171228,#171229,#171230,#171231,#171232,#171233,#171234,#171235,#171236,
#171237,#171238,#171239,#171240,#171241,#171242,#171243,#171244,#171245,
#171246,#171247,#171248,#171249,#171250,#171251,#171252,#171253,#171254,
#171255,#171256,#171257,#171258,#171259,#171260,#171261,#171262,#171263,
#171264,#171265,#171266,#171267,#171268,#171269,#171270,#171271,#171272,
#171273,#171274,#171275,#171276,#171277,#171278,#171279,#171280,#171281,
#171282,#171283,#171284,#171285,#171286,#171287,#171288,#171289,#171290,
#171291,#171292,#171293,#171294,#171295,#171296,#171297,#171298,#171299,
#171300,#171301,#171302,#171303,#171304,#171305,#171306,#171307,#171308,
#171309,#171310,#171311,#171312,#171313,#171314,#171315,#171316,#171317,
#171318,#171319,#171320,#171321,#171322,#171323,#171324,#171325,#171326,
#171327,#171328,#171329,#171330,#171331,#171332,#171333,#171334,#171335,
#171336,#171337,#171338,#171339,#171340,#171341,#171342,#171343,#171344,
#171345,#171346,#171347,#171348,#171349,#171350,#171351,#171352,#171353,
#171354,#171355,#171356,#171357,#171358,#171359,#171360,#171361,#171362,
#171363,#171364,#171365,#171366,#171367,#171368,#171369,#171370,#171371,
#171372,#171373,#171374,#171375,#171376,#171377,#171378,#171379,#171380,
#171381,#171382,#171383,#171384,#171385,#171386,#171387,#171388,#171389,
#171390,#171391,#171392,#171393,#171394,#171395,#171396,#171397,#171398,
#171399,#171400,#171401,#171402,#171403,#171404,#171405,#171406,#171407,
#171408,#171409,#171410,#171411,#171412,#171413,#171414,#171415,#171416,
#171417,#171418,#171419,#171420,#171421,#171422,#171423,#171424,#171425,
#171426,#171427,#171428,#171429,#171430,#171431,#171432,#171433,#171434,
#171435,#171436,#171437,#171438,#171439,#171440,#171441,#171442,#171443,
#171444,#171445,#171446,#171447,#171448,#171449,#171450,#171451,#171452,
#171453,#171454,#171455,#171456,#171457,#171458,#171459,#171460,#171461,
#171462,#171463,#171464,#171465,#171466,#171467,#171468,#171469,#171470,
#171471,#171472,#171473,#171474,#171475,#171476,#171477,#171478,#171479,
#171480,#171481,#171482,#171483,#171484,#171485,#171486,#171487,#171488,
#171489,#171490,#171491,#171492,#171493,#171494,#171495,#171496,#171497,
#171498,#171499,#171500,#171501,#171502,#171503,#171504,#171505,#171506,
#171507,#171508,#171509,#171510,#171511,#171512,#171513,#171514,#171515,
#171516,#171517,#171518,#171519,#171520,#171521,#171522,#171523,#171524,
#171525,#171526,#171527,#171528,#171529,#171530,#171531,#171532,#171533,
#171534,#171535,#171536,#171537,#171538,#171539,#171540,#171541,#171542,
#171543,#171544,#171545,#171546,#171547,#171548,#171549,#171550,#171551,
#171552,#171553,#171554,#171555,#171556,#171557,#171558,#171559,#171560,
#171561,#171562,#171563,#171564,#171565,#171566,#171567,#171568,#171569,
#171570,#171571,#171572,#171573,#171574,#171575,#171576,#171577,#171578,
#171579,#171580,#171581,#171582,#171583,#171584,#171585,#171586,#171587,
#171588,#171589,#171590,#171591,#171592,#171593,#171594,#171595,#171596,
#171597,#171598,#171599,#171600,#171601,#171602,#171603,#171604,#171605,
#171606,#171607,#171608,#171609,#171610,#171611,#171612,#171613,#171614,
#171615,#171616,#171617,#171618,#171619,#171620,#171621,#171622,#171623,
#171624,#171625,#171626,#171627,#171628,#171629,#171630,#171631,#171632,
#171633,#171634,#171635,#171636,#171637,#171638,#171639,#171640,#171641,
#171642,#171643,#171644,#171645,#171646,#171647,#171648,#171649,#171650,
#171651,#171652,#171653,#171654,#171655,#171656,#171657,#171658,#171659,
#171660,#171661,#171662,#171663,#171664,#171665,#171666,#171667,#171668,
#171669,#171670,#171671,#171672,#171673,#171674,#171675,#171676,#171677,
#171678,#171679,#171680,#171681,#171682,#171683,#171684,#171685,#171686,
#171687,#171688,#171689,#171690,#171691,#171692,#171693,#171694,#171695,
#171696,#171697,#171698,#171699,#171700,#171701,#171702,#171703,#171704,
#171705,#171706,#171707,#171708,#171709,#171710,#171711,#171712,#171713,
#171714,#171715,#171716,#171717,#171718,#171719,#171720,#171721,#171722,
#171723,#171724,#171725,#171726,#171727,#171728,#171729,#171730,#171731,
#171732,#171733,#171734,#171735,#171736,#171737,#171738,#171739,#171740,
#171741,#171742,#171743,#171744,#171745,#171746,#171747,#171748,#171749,
#171750,#171751,#171752,#171753,#171754,#171755,#171756,#171757,#171758,
#171759,#171760,#171761,#171762,#171763,#171764,#171765,#171766,#171767,
#171768,#171769,#171770,#171771,#171772,#171773,#171774,#171775,#171776,
#171777,#171778,#171779,#171780,#171781,#171782,#171783,#171784,#171785,
#171786,#171787,#171788,#171789,#171790,#171791,#171792,#171793,#171794,
#171795,#171796,#171797,#171798,#171799,#171800,#171801),.UNSPECIFIED.,
 .F.,.F.,(4,2,2,2,2,2,2,2,2,2,2,2,2,2,2,2,2,2,2,2,2,2,2,2,2,2,2,2,2,2,2,
2,2,2,2,2,2,2,2,2,2,2,2,2,2,2,2,2,2,2,2,2,2,2,2,2,2,2,2,2,2,2,2,2,2,2,2,
2,2,2,2,2,2,2,2,2,2,2,2,2,2,2,2,2,2,2,2,2,2,2,2,2,2,2,2,2,2,2,2,2,2,2,2,
2,2,2,2,2,2,2,2,2,2,2,2,2,2,2,2,2,2,2,2,2,2,2,2,2,2,2,2,2,2,2,2,2,2,2,2,
2,2,2,2,2,2,2,2,2,2,2,2,2,2,2,2,2,2,2,2,2,2,2,2,2,2,2,2,2,2,2,2,2,2,2,2,
2,2,2,2,2,2,2,2,2,2,2,2,2,2,2,2,2,2,2,2,2,2,2,2,2,2,2,2,2,2,2,2,2,2,2,2,
2,2,2,2,2,2,2,2,2,2,2,2,2,2,2,2,2,2,2,2,2,2,2,2,2,2,2,2,2,2,2,2,2,2,2,2,
2,2,2,2,2,2,2,2,2,2,2,2,2,2,2,2,2,2,2,2,2,2,2,2,2,2,2,2,2,2,2,2,2,2,2,2,
2,2,2,2,2,2,2,2,2,2,2,2,2,2,2,2,2,2,2,2,2,2,2,2,2,2,2,2,2,2,2,2,2,2,2,2,
2,2,2,2,2,2,2,2,2,2,2,2,2,2,2,2,2,2,2,2,2,2,2,2,2,2,2,2,2,2,2,2,2,2,2,2,
2,2,2,2,2,2,2,2,2,2,2,2,2,2,2,2,2,2,2,2,2,2,2,2,2,2,2,2,2,2,2,2,2,2,2,2,
2,4),(0.00175773553931062,0.219103254936723,0.24130675056173,0.253373369810396,
0.26400885429678,0.271010046070725,0.277588550997247,0.285910960050424,
0.302249272794649,0.441652005642513,0.517334035163842,0.573661124162176,
0.642628906649389,0.649141964325655,0.651548363312784,0.653662174922928,
0.655941397471844,0.658910732938449,0.665158306217353,0.730535299668664,
0.821431482018592,0.897670017795671,1.06124648248905,1.06972199635467,1.07359686257024,
1.07651494469592,1.07925735443216,1.08305340993945,1.09070766589037,1.16168760892158,
1.35647748551397,1.44920633297773,1.48326282640086,1.49517679124251,1.50361653908362,
1.50691092124709,1.50891569300446,1.51109605320493,1.51394152432146,1.52017635765003,
1.57374086012011,1.77004040456218,1.85380542168094,1.9323194264709,1.95550614639026,
1.9684984695291,1.97975037107685,1.99367251838452,2.02045895169309,2.18177440747651,
2.27676677816675,2.29298497237854,2.300026587392,2.30546542550424,2.3119241945082,
2.32361280667504,2.39430370226642,2.44426104636348,2.47638132625004,2.49001048845845,
2.49002447912599,2.49003848384626,2.4900525027195,2.49006653573498,2.49008058294009,
2.49009464438562,2.49010872016212,2.49012281031995,2.49013691483824,2.49015103381578,
2.49016516733543,2.49017931535028,2.49019347789304,2.49020765510122,2.49022184709889,
2.49023605378203,2.4902502752544,2.49026451164043,2.49027876290929,2.49029302907541,
2.49030731024939,2.49032160654275,2.49033591798422,2.50094928211647,2.51262434213112,
2.53221097121147,2.64706595965801,2.67939037980069,2.69926914385526,2.706878152016,
2.71220448103205,2.71807930181039,2.72873337570024,2.76686250023774,2.87828861367725,
2.93623224914979,2.95812530346132,2.97461351130785,2.99352213844178,3.03836168476794,
3.0879662388034,3.10562500164156,3.11747068542495,3.13304124034964,3.16671683525354,
3.19802874601558,3.23215616702389,3.25005725735955,3.26664612597028,3.28670977963142,
3.34368868867307,3.45264000311483,3.48023195286248,3.4988624845606,3.50693398937084,
3.51293219071194,3.51944501984934,3.53209183362207,3.60222639506482,3.68263921607325,
3.70627320395919,3.71875708277615,3.72926934321183,3.74201478281325,3.76636627514229,
3.85326945144904,3.8860865292963,3.90618166566052,3.91412477598333,3.91982250854305,
3.92511658531051,3.93503465805392,3.971631087357,4.04353339413235,4.12914377562721,
4.21300180379531,4.23342185086128,4.24585236336118,4.25720668401509,4.27184147911976,
4.30458249145143,4.42621249308663,4.60599934339915,4.67471734931112,4.70367241661355,
4.7086174106494,4.71123509451903,4.713176138818,4.71559382117842,4.7196254021198,
4.73283657596282,4.98808542030521,5.0771886966021,5.1143485646209,5.13565526533211,
5.14138094821278,5.144724154391,5.14759961151006,5.15108920504921,5.15764163483308,
5.19469059275185,5.2665560182974,5.54043555121987,5.559890466168,5.56419146418071,
5.56699335906224,5.56924618975467,5.57180457526152,5.57615245472894,5.59319977208206,
5.62393500696221,5.70261396549574,5.77935373268335,5.84915966813338,5.92339501433832,
5.93658395048812,5.9449358131758,5.95152838298344,5.9585335786119,5.96915481581509,
6.00070014138159,6.24784710410159,6.31422215349762,6.32543161127122,6.32930608349613,
6.33151434571518,6.3335472115256,6.33629285799145,6.34149805304394,6.37427083004007,
6.42221888210893,6.61240639593722,6.73790331560348,6.74735376784438,6.75110200563635,
6.75383249807268,6.7567591688638,6.7606821759407,6.769412506671,6.88848865610534,
7.14796800782987,7.1788927888432,7.18359207325653,7.18642040719891,7.18859886790867,
7.19093923000229,7.19462234215071,7.20623859633274,7.22478654868713,7.28975036595375,
7.50311638502679,7.60123389903768,7.63062995911758,7.64483776206688,7.65611911412314,
7.66893180015192,7.69113395071036,7.80677850944997,7.91149078331142,7.92724116144502,
7.93040424426407,7.95674358126864,7.97187318474109,7.97881485293055,7.98422898749944,
7.98423449530929,7.9842399911831,7.98424548058366,7.98425096343306,7.98425643994694,
7.98426190998369,7.98426737340359,7.98427283034096,7.98427828094693,7.98428372516629,
7.98428916298115,7.98429459438308,7.98430001941677,7.98430543803675,7.98431085028059,
7.98431625629666,7.98432165597753,7.98432704948173,7.9843324366821,7.98433781760566,
7.98434319220649,7.98434856053036,7.9843539226696,7.98435927860954,7.98436462821854,
7.98436997161479,7.98437530864554,7.98438063968183,7.98438596461978,7.98439128334387,
7.98439659583971,7.98440190224997,7.98440720262674,7.98976232166622,8.0003894723859,
8.06228631435481,8.14324823959832,8.16265105506578,8.1742638683533,8.18486821820486,
8.18488608151234,8.18490394305623,8.18492179598146,8.18493964028774,8.18495747603514,
8.18497530328501,8.18499312210091,8.18501093255323,8.18502873465068,8.18504652844231,
8.18506431401927,8.18508209143511,8.18509986069162,8.185117621884,8.18513537511171,
8.18515312033165,8.1851708576113,8.18518858705245,8.18520630868814,8.18522402254627,
8.18524172866618,8.18525942709194,8.18527711792504,8.18529480122889,8.18531247704046,
8.18533014539189,8.18534780632293,8.18536545987528,8.18538310613759,8.18540074518451,
8.18541837704094,8.18543600174093,8.19926806755702,8.23235884162917,8.28275511167052,
8.35854144903252,8.3772875446188,8.38486286081928,8.39032494313797,8.39036375199302,
8.39040046422107,8.39042357730001,8.39044638217812,8.39046888768473,8.3904910984323,
8.39051301885942,8.3905346533365,8.39055600620307,8.39057708163389,8.39059788382034,
8.39061841680037,8.39063868452902,8.39065869099236,8.3906784400369,8.39069793540036,
8.39071718075312,8.39073617983866,8.39075493622398,8.39077345341528,8.39079173484714,
8.39080978396012,8.39082760410349,8.39084519854574,8.39086257046582,8.39087414482491,
8.39088572026534,8.39089726116498,8.39090876770239,8.39092024008883,8.39093167839267,
8.39659483682501,8.40729864480983,8.45002625920061,8.57499910953089,8.61849057401589,
8.63893061114731,8.65536095720363,8.67513341979719,8.67539319551005,8.67565556400815,
8.67592064609455,8.67618856667261,8.67645945499847,8.67673344495327,8.73466225979669,
8.77601763080902,8.78803432447916,8.79924360381503,8.82258803183516,8.86148297575841,
8.90767426342444,8.92664310148138,8.94315597067937,8.96307983800104,9.01380549014799,
9.09709794554847,9.11800517335987,9.17141096545959,9.18270125807024,9.18894189376735,
9.19482167955657,9.20238899876156,9.22190300163407,9.23889919255774,9.32076450653238,
9.37527822464089,9.39215945163949,9.40218321154727,9.41291704052995,9.42353223026847,
9.44839252377286,9.53305464133504,9.58186561512102,9.58871930503183,9.5956740002792,
9.60101753776024,9.60732353642894,9.61946888376378,9.63523148033024,9.77791606178537,
9.89069508729099,9.91274824832863,9.92566695546978,9.93695339681467,9.95105061597933,
9.96638042027543,9.99188617045719,10.2304410678172),.UNSPECIFIED.);
#3225=B_SPLINE_CURVE_WITH_KNOTS('',3,(#171803,#171804,#171805,#171806,#171807,
#171808,#171809,#171810,#171811,#171812,#171813,#171814,#171815,#171816,
#171817,#171818,#171819,#171820,#171821,#171822,#171823,#171824,#171825,
#171826,#171827,#171828,#171829,#171830,#171831,#171832,#171833,#171834,
#171835,#171836,#171837,#171838,#171839,#171840,#171841,#171842,#171843,
#171844,#171845,#171846,#171847,#171848,#171849,#171850,#171851,#171852,
#171853,#171854,#171855,#171856,#171857,#171858,#171859,#171860,#171861,
#171862,#171863,#171864,#171865,#171866,#171867,#171868,#171869,#171870,
#171871,#171872,#171873,#171874,#171875,#171876,#171877,#171878,#171879,
#171880,#171881,#171882,#171883,#171884,#171885,#171886,#171887,#171888,
#171889,#171890,#171891,#171892,#171893,#171894,#171895,#171896,#171897,
#171898,#171899,#171900,#171901,#171902,#171903,#171904,#171905,#171906,
#171907,#171908,#171909,#171910,#171911,#171912,#171913,#171914,#171915,
#171916,#171917,#171918,#171919,#171920,#171921,#171922,#171923,#171924,
#171925,#171926,#171927,#171928,#171929,#171930,#171931,#171932,#171933,
#171934,#171935,#171936,#171937,#171938,#171939,#171940,#171941,#171942,
#171943,#171944,#171945,#171946,#171947,#171948,#171949,#171950,#171951,
#171952,#171953,#171954,#171955,#171956,#171957,#171958,#171959,#171960,
#171961,#171962,#171963,#171964,#171965,#171966,#171967,#171968,#171969,
#171970,#171971,#171972,#171973,#171974,#171975,#171976,#171977,#171978,
#171979,#171980,#171981,#171982,#171983,#171984,#171985,#171986,#171987,
#171988,#171989,#171990,#171991,#171992,#171993,#171994,#171995,#171996,
#171997,#171998,#171999,#172000,#172001,#172002,#172003,#172004,#172005,
#172006,#172007,#172008,#172009,#172010,#172011,#172012,#172013,#172014,
#172015,#172016,#172017,#172018,#172019,#172020,#172021,#172022,#172023,
#172024,#172025,#172026,#172027,#172028,#172029,#172030,#172031,#172032,
#172033,#172034,#172035,#172036,#172037,#172038,#172039,#172040,#172041,
#172042,#172043,#172044,#172045,#172046,#172047,#172048,#172049,#172050,
#172051,#172052,#172053,#172054,#172055,#172056,#172057,#172058,#172059,
#172060,#172061,#172062,#172063,#172064,#172065,#172066,#172067,#172068,
#172069,#172070,#172071,#172072,#172073,#172074,#172075,#172076,#172077,
#172078,#172079,#172080,#172081,#172082,#172083,#172084,#172085,#172086,
#172087,#172088,#172089,#172090,#172091,#172092,#172093,#172094,#172095,
#172096,#172097,#172098,#172099,#172100,#172101,#172102,#172103,#172104,
#172105,#172106,#172107,#172108,#172109,#172110,#172111,#172112,#172113,
#172114,#172115,#172116,#172117,#172118,#172119,#172120,#172121,#172122,
#172123,#172124,#172125,#172126,#172127,#172128,#172129,#172130,#172131,
#172132,#172133,#172134,#172135,#172136,#172137,#172138,#172139,#172140,
#172141,#172142,#172143,#172144,#172145,#172146,#172147,#172148,#172149,
#172150,#172151,#172152,#172153,#172154,#172155,#172156,#172157,#172158,
#172159,#172160,#172161,#172162,#172163,#172164,#172165,#172166,#172167,
#172168,#172169,#172170,#172171,#172172,#172173,#172174,#172175,#172176,
#172177,#172178,#172179,#172180,#172181,#172182,#172183,#172184,#172185,
#172186,#172187,#172188,#172189,#172190,#172191,#172192,#172193,#172194,
#172195,#172196,#172197,#172198,#172199,#172200,#172201,#172202,#172203,
#172204,#172205,#172206,#172207,#172208,#172209,#172210,#172211,#172212,
#172213,#172214,#172215,#172216,#172217,#172218,#172219,#172220,#172221,
#172222,#172223,#172224,#172225,#172226,#172227,#172228,#172229,#172230,
#172231,#172232,#172233,#172234,#172235,#172236,#172237,#172238,#172239,
#172240,#172241,#172242,#172243,#172244,#172245,#172246,#172247,#172248,
#172249,#172250,#172251,#172252,#172253,#172254,#172255,#172256,#172257,
#172258,#172259,#172260,#172261,#172262,#172263,#172264,#172265,#172266,
#172267,#172268,#172269,#172270,#172271,#172272,#172273,#172274,#172275,
#172276,#172277,#172278,#172279,#172280,#172281,#172282,#172283,#172284,
#172285,#172286,#172287,#172288,#172289,#172290,#172291,#172292,#172293,
#172294,#172295,#172296,#172297,#172298,#172299,#172300,#172301,#172302,
#172303,#172304,#172305,#172306,#172307,#172308,#172309,#172310,#172311,
#172312,#172313,#172314,#172315,#172316,#172317,#172318,#172319,#172320,
#172321,#172322,#172323,#172324,#172325,#172326,#172327,#172328,#172329,
#172330,#172331,#172332,#172333,#172334,#172335,#172336,#172337,#172338,
#172339,#172340,#172341,#172342,#172343,#172344,#172345,#172346,#172347,
#172348,#172349,#172350,#172351,#172352,#172353,#172354,#172355,#172356,
#172357,#172358,#172359,#172360,#172361,#172362,#172363,#172364,#172365,
#172366,#172367,#172368,#172369,#172370,#172371,#172372,#172373,#172374,
#172375,#172376,#172377,#172378,#172379,#172380,#172381,#172382,#172383,
#172384,#172385,#172386,#172387,#172388,#172389,#172390,#172391,#172392,
#172393,#172394,#172395,#172396,#172397,#172398,#172399,#172400,#172401,
#172402,#172403,#172404,#172405,#172406,#172407,#172408,#172409,#172410,
#172411,#172412,#172413,#172414,#172415,#172416,#172417,#172418,#172419,
#172420,#172421,#172422,#172423,#172424,#172425,#172426,#172427,#172428,
#172429,#172430,#172431,#172432,#172433,#172434,#172435,#172436,#172437,
#172438,#172439,#172440,#172441,#172442,#172443,#172444,#172445,#172446,
#172447,#172448,#172449,#172450,#172451,#172452,#172453,#172454,#172455,
#172456,#172457,#172458,#172459,#172460,#172461,#172462,#172463,#172464,
#172465,#172466,#172467,#172468,#172469,#172470,#172471,#172472,#172473,
#172474,#172475,#172476,#172477,#172478,#172479,#172480,#172481,#172482,
#172483,#172484,#172485,#172486,#172487,#172488,#172489,#172490,#172491,
#172492,#172493,#172494,#172495,#172496,#172497,#172498,#172499,#172500,
#172501,#172502,#172503,#172504,#172505,#172506),.UNSPECIFIED.,.F.,.F.,
(4,2,2,2,2,2,2,2,2,2,2,2,2,2,2,2,2,2,2,2,2,2,2,2,2,2,2,2,2,2,2,2,2,2,2,
2,2,2,2,2,2,2,2,2,2,2,2,2,2,2,2,2,2,2,2,2,2,2,2,2,2,2,2,2,2,2,2,2,2,2,2,
2,2,2,2,2,2,2,2,2,2,2,2,2,2,2,2,2,2,2,2,2,2,2,2,2,2,2,2,2,2,2,2,2,2,2,2,
2,2,2,2,2,2,2,2,2,2,2,2,2,2,2,2,2,2,2,2,2,2,2,2,2,2,2,2,2,2,2,2,2,2,2,2,
2,2,2,2,2,2,2,2,2,2,2,2,2,2,2,2,2,2,2,2,2,2,2,2,2,2,2,2,2,2,2,2,2,2,2,2,
2,2,2,2,2,2,2,2,2,2,2,2,2,2,2,2,2,2,2,2,2,2,2,2,2,2,2,2,2,2,2,2,2,2,2,2,
2,2,2,2,2,2,2,2,2,2,2,2,2,2,2,2,2,2,2,2,2,2,2,2,2,2,2,2,2,2,2,2,2,2,2,2,
2,2,2,2,2,2,2,2,2,2,2,2,2,2,2,2,2,2,2,2,2,2,2,2,2,2,2,2,2,2,2,2,2,2,2,2,
2,2,2,2,2,2,2,2,2,2,2,2,2,2,2,2,2,2,2,2,2,2,2,2,2,2,2,2,2,2,2,2,2,2,2,2,
2,2,2,2,2,2,2,2,2,2,2,2,2,2,2,2,2,2,2,2,2,2,2,2,2,2,2,2,4),(0.00222864392066332,
0.145752713813109,0.154791928451702,0.159396326581129,0.162264130794258,
0.164425517493528,0.166614639667749,0.168649290422639,0.171430485007103,
0.178384690789793,0.293562036677726,0.334592796162703,0.375675830641575,
0.465288439484411,0.584332488052246,0.593073292281324,0.59699800374325,
0.599924737670028,0.602654419157341,0.606400186788489,0.61385331218668,
0.678208354816265,0.873987252073665,0.922852180608173,0.979251475758716,
1.00070058020002,1.01434587787992,1.01837491691129,1.02049685833035,1.02252096157089,
1.02512984125736,1.02958757197051,1.0461410535428,1.1666078661986,1.30957250923845,
1.36136959646054,1.38605540093741,1.39585889250909,1.40269625282933,1.40936447496336,
1.41807350376215,1.43278605609214,1.55778909834871,1.71832385764177,1.76945439376248,
1.77903896584968,1.78254831562554,1.78466332692828,1.78693861525808,1.78987733445077,
1.79619734647444,1.86085768472907,2.08004265511586,2.19307531945937,2.20125313871922,
2.20507240359412,2.20798277593868,2.21074336851788,2.21537819555806,2.22754200321335,
2.43134625567394,2.56529135977613,2.62398890534212,2.63466156520055,2.63822881060265,
2.64054335950563,2.64273205632357,2.645624170723,2.65055742981425,2.68296170204597,
2.71882011910063,2.71982889577092,2.84973315290992,3.04593951658693,3.08071161858082,
3.09584105917549,3.10723166525579,3.11955668343999,3.13947380995051,3.20684683879622,
3.39454293907706,3.41263260619009,3.42614325388338,3.43270012242929,3.43827643518663,
3.44540570134363,3.45705148776271,3.54516724342479,3.57401033941666,3.60774680608874,
3.62189249785948,3.63253209545195,3.64269043738467,3.6603718965382,3.72983649015465,
3.78013601586695,3.80485432996246,3.82974349605703,3.83797114468403,3.84389394217918,
3.85055200107205,3.86184645097685,3.91004441181189,3.91238676080507,3.91371674091713,
3.91798156111839,4.01452135062403,4.06913856121101,4.09066209709999,4.10711943595327,
4.12627322391632,4.19048740211883,4.2296160630797,4.24293079069542,4.25623972954272,
4.29002536606598,4.33647312532537,4.35857595535477,4.37805095417511,4.3944748981709,
4.41519528751392,4.46215696094581,4.48714231091662,4.58634661497921,4.61296853788919,
4.63113087895284,4.63912460249245,4.64511174704584,4.65166953203201,4.66458763746315,
4.72058719053112,4.79078718389885,4.81032924055283,4.83672779543976,4.8497302190135,
4.86025446558893,4.87252386886401,4.89449856271038,4.9825450664432,5.0172538813494,
5.03808423035349,5.04613248111265,5.05185023962814,5.05787026577873,5.06853148641755,
5.1147251600168,5.23689491567324,5.27769883775891,5.3460594407408,5.36606667969574,
5.37841100607796,5.38979530389436,5.40488017087536,5.43937554834491,5.62916506115224,
5.75641739225734,5.83341941371237,5.83940444222344,5.84230436713257,5.84437090824065,
5.84654426827029,5.84938938459321,5.85545670814646,5.95726587322646,6.02248734172103,
6.10456251384157,6.26128579029209,6.27106833757507,6.2748727718778,6.27761822474729,
6.28053675355615,6.28440746415585,6.29285501588599,6.44828668234007,6.68131890665693,
6.6935382803584,6.69755492512495,6.69979043630343,6.70204308107137,6.70483720911909,
6.71027300180708,6.74716427713634,6.84800337643436,7.0381354625443,7.06439164361406,
7.0746092049952,7.08083496991808,7.08740878186555,7.09560116775854,7.11180070221573,
7.29162721837968,7.32321026075574,7.42781077739799,7.45503999791139,7.4598666418968,
7.46279433077781,7.46506821205946,7.46753039808207,7.47144620864666,7.48412805875149,
7.55963608588631,7.6984497095742,7.80839021325637,7.8721658441708,7.87960238993289,
7.88334450371148,7.88607375087583,7.88900212370012,7.89293268505709,7.90170162012449,
8.02080993220388,8.19202724149539,8.30772092336658,8.31485996978492,8.3176731951105,
8.31971663695966,8.32190143486072,8.32481953081665,8.33114439338697,8.3833592251149,
8.44224454137476,8.53318766649393,8.7228258852945,8.75844365625477,8.77259399323171,
8.78416173982891,8.79470232994797,8.80998127479262,8.84831254640901,8.90377103333723,
8.98929993120174,9.02087970194307,9.06920266201967,9.09891662976408,9.10822406193392,
9.11342323407321,9.11810506104238,9.1181206857969,9.11813627721229,9.11815183436659,
9.11816735763323,9.11818284736614,9.1181983038891,9.11821372750712,9.11822911861957,
9.11824447757168,9.11825980476813,9.11827510051404,9.11829036505129,9.11830559881839,
9.11832080219563,9.1183359754508,9.11835111896383,9.11836623296018,9.11838131780409,
9.11839637385397,9.11841140145639,9.11842640087208,9.1184413723903,9.11845631639496,
9.11847123315721,9.118486123009,9.11850098624138,9.11851582319342,9.11853063412191,
9.11854541930116,9.11856017903026,9.11857491367371,9.11858962350373,9.11860430874351,
9.11861896976863,9.1186336068464,9.11864822025547,9.1186628102186,9.1186773771369,
9.11869192132261,9.11870644293731,9.11872094228361,9.11873541958983,9.11874987514441,
9.11876430926325,9.11877872223553,9.11879311423609,9.11880748557093,9.11882183652364,
9.11883616734598,9.11885047827484,9.11886476965527,9.11887904169879,9.12447633339158,
9.13240972233585,9.14600325565374,9.17750894663704,9.26362320253015,9.2901178103735,
9.30310897002314,9.31292058209694,9.3131613658508,9.31338600044482,9.31359556748995,
9.31379107967034,9.31397348401925,9.31414366534419,9.31430244967537,9.31445060771165,
9.31458885819979,9.31471787119976,9.3148382712068,9.31495064015506,9.31505552022617,
9.31515341656896,9.31524479977996,9.31533010827759,9.31540975052063,9.31548410706331,
9.31560936332118,9.31573283957854,9.31585456886046,9.31597458659128,9.31609292622285,
9.327766496573,9.35284995356795,9.38655198407043,9.44127074805844,9.44967862585153,
9.50509500327044,9.51526810100552,9.52078290411029,9.52638001347458,9.53411889183065,
9.55219993613889,9.57898607067872,9.67970075853278,9.74551653714096,9.76590818147345,
9.7810397483565,9.79680409738449,9.81460486887346,9.82302515137781,9.84575828938478,
9.90731600452193,9.91744145069483,9.92843559728806,9.94057770605154,9.95994393761197,
10.0132912485553,10.0448031802273,10.0606934176668,10.0760958206565,10.0920438422306,
10.1134746853582,10.2281817080754),.UNSPECIFIED.);
#3226=B_SPLINE_CURVE_WITH_KNOTS('',3,(#172508,#172509,#172510,#172511,#172512,
#172513,#172514,#172515,#172516,#172517,#172518,#172519,#172520,#172521,
#172522,#172523,#172524,#172525,#172526,#172527,#172528,#172529,#172530,
#172531,#172532,#172533,#172534,#172535,#172536,#172537,#172538,#172539,
#172540,#172541,#172542,#172543,#172544,#172545,#172546,#172547,#172548,
#172549,#172550,#172551,#172552,#172553,#172554,#172555,#172556,#172557,
#172558,#172559,#172560,#172561,#172562,#172563,#172564,#172565,#172566,
#172567,#172568,#172569,#172570,#172571,#172572,#172573,#172574,#172575,
#172576,#172577,#172578,#172579,#172580,#172581,#172582,#172583,#172584,
#172585,#172586,#172587,#172588,#172589,#172590,#172591,#172592,#172593,
#172594,#172595,#172596,#172597,#172598,#172599,#172600,#172601,#172602,
#172603,#172604,#172605,#172606,#172607,#172608,#172609,#172610,#172611,
#172612,#172613,#172614,#172615,#172616,#172617,#172618,#172619,#172620,
#172621,#172622,#172623,#172624,#172625,#172626,#172627,#172628,#172629,
#172630,#172631,#172632,#172633,#172634,#172635,#172636,#172637,#172638,
#172639,#172640,#172641,#172642,#172643,#172644,#172645,#172646,#172647,
#172648,#172649,#172650,#172651,#172652,#172653,#172654,#172655,#172656,
#172657,#172658,#172659,#172660,#172661,#172662,#172663,#172664,#172665,
#172666,#172667,#172668,#172669,#172670,#172671,#172672,#172673,#172674,
#172675,#172676,#172677,#172678,#172679,#172680,#172681,#172682,#172683,
#172684,#172685,#172686,#172687,#172688,#172689,#172690,#172691,#172692,
#172693,#172694,#172695,#172696,#172697,#172698,#172699,#172700,#172701,
#172702,#172703,#172704,#172705,#172706,#172707,#172708,#172709,#172710,
#172711,#172712,#172713,#172714,#172715,#172716,#172717,#172718,#172719,
#172720,#172721,#172722,#172723,#172724,#172725,#172726,#172727,#172728,
#172729,#172730,#172731,#172732,#172733,#172734,#172735,#172736,#172737,
#172738,#172739,#172740,#172741,#172742,#172743,#172744,#172745,#172746,
#172747,#172748,#172749,#172750,#172751,#172752,#172753,#172754,#172755,
#172756,#172757,#172758,#172759,#172760,#172761,#172762,#172763,#172764,
#172765,#172766,#172767,#172768,#172769,#172770,#172771,#172772,#172773,
#172774,#172775,#172776,#172777,#172778,#172779,#172780,#172781,#172782,
#172783,#172784,#172785,#172786,#172787,#172788,#172789,#172790,#172791,
#172792,#172793,#172794,#172795,#172796,#172797,#172798,#172799,#172800,
#172801,#172802,#172803,#172804,#172805,#172806,#172807,#172808,#172809,
#172810,#172811,#172812,#172813,#172814,#172815,#172816,#172817,#172818,
#172819,#172820,#172821,#172822,#172823,#172824,#172825,#172826,#172827,
#172828,#172829,#172830,#172831,#172832,#172833,#172834,#172835,#172836,
#172837,#172838,#172839,#172840,#172841,#172842,#172843,#172844,#172845,
#172846,#172847,#172848,#172849,#172850,#172851,#172852,#172853,#172854,
#172855,#172856,#172857,#172858,#172859,#172860,#172861,#172862,#172863,
#172864,#172865,#172866,#172867,#172868,#172869,#172870,#172871,#172872,
#172873,#172874,#172875,#172876,#172877,#172878,#172879,#172880,#172881,
#172882,#172883,#172884,#172885,#172886,#172887,#172888,#172889,#172890,
#172891,#172892,#172893,#172894,#172895,#172896,#172897,#172898,#172899,
#172900,#172901,#172902,#172903,#172904,#172905,#172906,#172907,#172908,
#172909,#172910,#172911,#172912,#172913,#172914,#172915,#172916,#172917,
#172918,#172919,#172920,#172921,#172922,#172923,#172924,#172925,#172926,
#172927,#172928,#172929,#172930,#172931,#172932,#172933,#172934,#172935,
#172936,#172937,#172938,#172939,#172940,#172941,#172942,#172943,#172944,
#172945,#172946,#172947,#172948,#172949,#172950,#172951,#172952,#172953,
#172954,#172955,#172956,#172957,#172958,#172959,#172960,#172961,#172962,
#172963,#172964,#172965,#172966,#172967,#172968,#172969,#172970,#172971,
#172972,#172973,#172974,#172975,#172976,#172977,#172978,#172979,#172980,
#172981,#172982,#172983,#172984,#172985,#172986,#172987,#172988,#172989,
#172990,#172991,#172992,#172993,#172994,#172995,#172996,#172997,#172998,
#172999,#173000,#173001,#173002,#173003,#173004,#173005,#173006,#173007,
#173008,#173009,#173010,#173011,#173012,#173013,#173014,#173015,#173016,
#173017,#173018,#173019,#173020,#173021,#173022,#173023,#173024,#173025,
#173026,#173027,#173028,#173029,#173030,#173031,#173032,#173033,#173034,
#173035,#173036,#173037,#173038,#173039,#173040,#173041,#173042,#173043,
#173044,#173045,#173046,#173047,#173048,#173049),.UNSPECIFIED.,.F.,.F.,
(4,2,2,2,2,2,2,2,2,2,2,2,2,2,2,2,2,2,2,2,2,2,2,2,2,2,2,2,2,2,2,2,2,2,2,
2,2,2,2,2,2,2,2,2,2,2,2,2,2,2,2,2,2,2,2,2,2,2,2,2,2,2,2,2,2,2,2,2,2,2,2,
2,2,2,2,2,2,2,2,2,2,2,2,2,2,2,2,2,2,2,2,2,2,2,2,2,2,2,2,2,2,2,2,2,2,2,2,
2,2,2,2,2,2,2,2,2,2,2,2,2,2,2,2,2,2,2,2,2,2,2,2,2,2,2,2,2,2,2,2,2,2,2,2,
2,2,2,2,2,2,2,2,2,2,2,2,2,2,2,2,2,2,2,2,2,2,2,2,2,2,2,2,2,2,2,2,2,2,2,2,
2,2,2,2,2,2,2,2,2,2,2,2,2,2,2,2,2,2,2,2,2,2,2,2,2,2,2,2,2,2,2,2,2,2,2,2,
2,2,2,2,2,2,2,2,2,2,2,2,2,2,2,2,2,2,2,2,2,2,2,2,2,2,2,2,2,2,2,2,2,2,2,2,
2,2,2,2,2,2,2,2,2,2,2,2,2,2,2,2,2,2,2,4),(0.00102620614831673,0.0568395121519397,
0.0781476365882496,0.0858676499435164,0.0917549942783009,0.0975572177948521,
0.104209418963546,0.117718867000098,0.140873799900062,0.209787996764556,
0.26788818954445,0.290631847902776,0.291838944442536,0.292976648736238,
0.294064243783625,0.303958307270033,0.313682779774412,0.326502687937221,
0.35206394367747,0.452291696904518,0.475942494000112,0.487297021785289,
0.496439627916323,0.502253254910401,0.507828595969424,0.514762713683678,
0.533565358816321,0.663095578600488,0.773113263412681,0.807680316258092,
0.819786924111683,0.83027169013811,0.841634979043136,0.856335739853958,
0.889475990545155,1.0131264482929,1.17708042018566,1.25584166138584,1.27710490670949,
1.28566214189708,1.29008815764266,1.29385144559114,1.29620902902076,1.29838044441402,
1.30116747301061,1.30709407909758,1.3624960905748,1.40713069174675,1.47985115846917,
1.62910456283263,1.70712778795053,1.72150504741987,1.72629207696349,1.72939233653898,
1.73231950809825,1.73617982125951,1.74480201657441,1.81999982901002,1.94156121740033,
2.04967966638447,2.09256965895016,2.13649170847692,2.14273173807503,2.14778281122737,
2.15051958331156,2.15276763605195,2.15503559523524,2.15920895211213,2.17273127648019,
2.19737282608329,2.33787485357274,2.48276778677318,2.50365514423809,2.52010767786161,
2.52832174848353,2.5349166870894,2.54108069464312,2.55096840605079,2.57518623818831,
2.82351302936569,2.89713462538576,2.9089308613311,2.9127400507745,2.91517800892091,
2.91745962621654,2.9204394926797,2.92542886341437,2.95913901053721,3.16527192909523,
3.31878458652489,3.33022950419429,3.33460722095287,3.33761955029446,3.3405680232154,
3.344118179065,3.35296936006526,3.43615778853247,3.47739647774249,3.65769297450708,
3.75889393773878,3.76601887945577,3.76905667726209,3.77126150588284,3.77327672903998,
3.77598033625042,3.78262863393014,3.87729116904309,3.9992328027486,4.17717068951971,
4.21105794054042,4.22604057998807,4.23740762100006,4.24979121894257,4.26999426569961,
4.34063532123631,4.47399507575917,4.52296005770062,4.54174800167084,4.55565806888299,
4.56228766908029,4.5678536670028,4.57489815576959,4.58625007921004,4.66130630310504,
4.69733594625616,4.73581835933664,4.7505931595773,4.76132488053928,4.77130402813517,
4.78800615115649,4.84027806722212,4.92406750407647,4.94122737007191,4.96085691906785,
4.96843123511866,4.97375515784402,4.98049903936461,4.99219915201916,5.05814786787396,
5.06035259520831,5.11299003324026,5.15333939368309,5.20018219283488,5.22089788552376,
5.23731682048131,5.25678425594725,5.27887761985863,5.32529602977783,5.35908659909043,
5.37239467096206,5.38570201862689,5.42473549139449,5.48907346569522,5.50820482570642,
5.52465923770158,5.54620071201092,5.60101164646442,5.69834810586112,5.69952624098705,
5.75298522091397,5.76448850334058,5.77119018169888,5.77651889804539,5.78418010036951,
5.80445314908984,5.83775300740412,5.95009407008174,5.97023191300291,5.98201897393524,
5.99154346447942,6.00470531232457,6.03220697741315,6.07122550678907,6.1143254579551,
6.16279184324237,6.17298598539828,6.17853665761317,6.18354712192532,6.19077406487219,
6.20808051575612,6.23312690623326,6.35352320174268,6.47108190878521,6.49302678200077,
6.50590685009901,6.5171745302817,6.53126813749671,6.56006184105458,6.68043930490046,
6.85276470404648,6.96233246301301,6.96902159425894,6.97168705873444,6.97389302898849,
6.97614048663521,6.97939599249955,6.98785169056937,6.99956481915813,7.03274949209682,
7.06293335360849,7.2264084602597,7.39001246041463,7.39990812393551,7.40373015881433,
7.4064794461922,7.40939386817519,7.41324529367254,7.42159628135234,7.55858141389394,
7.74702234239047,7.81794604807203,7.82435751917478,7.82731288274965,7.82959009956768,
7.83203745955296,7.83549914248941,7.8458633106777,7.95964018618104,8.03807234203696,
8.09222144809225,8.18267184424082,8.19657053303832,8.20504110127206,8.21166880083292,
8.21857443138875,8.22839176053112,8.23957346880838,8.25952622133303,8.4715944205025,
8.58049382172193,8.58749981543922,8.59028929281688,8.59259705304038,8.59494732825187,
8.59802126450257,8.6055234310155,8.68912148674426,8.7770536055165,8.96806131025238,
9.00231795104721,9.00848674831538,9.01223287077243,9.01514129081237,9.01828873566096,
9.02328957663687,9.03943295244869,9.13345696586996,9.23629817586924,9.305119643732,
9.43348863068548,9.44192383883372,9.44494233413934,9.44704071362441,9.44898441250636,
9.45162829417569,9.4566985443934,9.48811950804353,9.59970117365182,9.69165753739034,
9.82764257374894,9.88035604089167,9.89839256157906,9.90912512694945,9.92055423769859,
9.9317274060158,9.94653493357267,9.97043295938086,10.018872567841,10.1115261152096,
10.1999744616998,10.2235615089747),.UNSPECIFIED.);
#3227=B_SPLINE_CURVE_WITH_KNOTS('',3,(#173051,#173052,#173053,#173054,#173055,
#173056,#173057,#173058,#173059,#173060,#173061,#173062,#173063,#173064,
#173065),.UNSPECIFIED.,.F.,.F.,(4,1,1,1,1,1,1,1,1,1,1,1,4),(273.318560862312,
273.602496096744,274.599433183359,275.097901726666,275.596370269974,276.593307356589,
277.091775899897,277.590244443204,278.088712986512,278.587181529819,279.085650073127,
279.584118616434,279.601746169492),.UNSPECIFIED.);
#3228=B_SPLINE_CURVE_WITH_KNOTS('',3,(#173067,#173068,#173069,#173070,#173071,
#173072,#173073,#173074,#173075,#173076,#173077,#173078,#173079,#173080,
#173081,#173082,#173083,#173084,#173085,#173086,#173087,#173088,#173089,
#173090,#173091,#173092,#173093,#173094,#173095,#173096,#173097,#173098,
#173099,#173100,#173101,#173102,#173103,#173104,#173105,#173106,#173107,
#173108,#173109,#173110,#173111,#173112,#173113,#173114,#173115,#173116,
#173117,#173118,#173119,#173120,#173121,#173122,#173123,#173124,#173125,
#173126,#173127,#173128,#173129,#173130,#173131,#173132,#173133,#173134,
#173135,#173136,#173137,#173138,#173139,#173140,#173141,#173142,#173143,
#173144,#173145,#173146,#173147,#173148,#173149,#173150,#173151,#173152,
#173153,#173154,#173155,#173156,#173157,#173158,#173159,#173160,#173161,
#173162,#173163,#173164,#173165,#173166,#173167,#173168,#173169,#173170,
#173171,#173172,#173173,#173174,#173175,#173176,#173177,#173178,#173179,
#173180,#173181,#173182,#173183,#173184,#173185,#173186,#173187,#173188,
#173189,#173190,#173191,#173192,#173193,#173194,#173195,#173196,#173197,
#173198,#173199,#173200,#173201,#173202,#173203,#173204,#173205,#173206,
#173207,#173208,#173209,#173210,#173211,#173212,#173213,#173214,#173215,
#173216,#173217,#173218,#173219,#173220,#173221,#173222,#173223,#173224,
#173225,#173226,#173227,#173228,#173229,#173230,#173231,#173232,#173233,
#173234,#173235,#173236,#173237,#173238,#173239,#173240,#173241,#173242,
#173243,#173244,#173245,#173246,#173247,#173248,#173249,#173250,#173251,
#173252,#173253,#173254,#173255,#173256,#173257,#173258,#173259,#173260,
#173261,#173262,#173263,#173264,#173265,#173266,#173267,#173268,#173269,
#173270,#173271,#173272,#173273,#173274,#173275,#173276,#173277,#173278,
#173279,#173280,#173281,#173282,#173283,#173284,#173285,#173286,#173287,
#173288,#173289,#173290,#173291,#173292,#173293,#173294,#173295,#173296,
#173297,#173298,#173299,#173300,#173301,#173302,#173303,#173304,#173305,
#173306,#173307,#173308,#173309,#173310,#173311,#173312,#173313,#173314,
#173315,#173316,#173317,#173318,#173319,#173320,#173321,#173322,#173323,
#173324,#173325),.UNSPECIFIED.,.F.,.F.,(4,3,3,3,3,3,3,3,3,3,3,3,3,3,3,3,
3,3,3,3,3,3,3,3,3,3,3,3,3,3,3,3,3,3,3,3,3,3,3,3,3,3,3,3,3,3,3,3,3,3,3,3,
3,3,3,3,3,3,3,3,3,3,3,3,3,3,3,3,3,3,3,3,3,3,3,3,3,3,3,3,3,3,3,3,3,3,4),
(267.035375555133,267.112204324455,267.189064455074,267.26596304077,267.342907197631,
267.419944352232,267.497030673745,267.574214775759,267.620873577053,267.697006449298,
267.77304615037,267.849002155741,267.924860598278,268.000661661832,268.076400982566,
268.11934212036,268.195084485183,268.270872605932,268.346715776774,268.422670735034,
268.498687167368,268.574822962869,268.617810663668,268.694021244142,268.770163848394,
268.846248934735,268.922286921007,268.998288191562,269.075345636402,269.151310898527,
269.227272490392,269.303239817453,269.381116800661,269.457146598094,269.535947174188,
269.614747750283,269.686171025133,269.757541152046,269.828871723567,269.900185061053,
269.971485747875,270.042811229367,270.113216293591,270.200921782932,270.289098145351,
270.377702555969,270.466402862852,270.554999122788,270.611684836898,270.684654281348,
270.757578272441,270.830469799182,270.903351998102,270.976226916146,271.049129865855,
271.110153380206,271.189454164155,271.268777094632,271.348119696642,271.427492773815,
271.506874454812,271.586271231921,271.608621923513,271.688019318182,271.76740299201,
271.846770443651,271.926115627463,272.00543864673,272.084732876351,272.107090466821,
272.17999286709,272.252872724135,272.325742993569,272.398639337974,272.471547993759,
272.544516306707,272.605559010129,272.694133341742,272.782833707216,272.871400519319,
272.959743932883,273.047513649509,273.104027553436,273.172188286623,273.240326894936,
273.308462615678,273.318560862312),.UNSPECIFIED.);
#3229=B_SPLINE_CURVE_WITH_KNOTS('',3,(#173327,#173328,#173329,#173330,#173331,
#173332,#173333,#173334,#173335,#173336,#173337,#173338,#173339,#173340,
#173341,#173342,#173343,#173344,#173345,#173346,#173347,#173348,#173349,
#173350,#173351,#173352,#173353,#173354,#173355,#173356,#173357,#173358,
#173359,#173360,#173361,#173362,#173363,#173364,#173365,#173366,#173367,
#173368,#173369,#173370,#173371,#173372,#173373,#173374,#173375,#173376,
#173377,#173378,#173379,#173380,#173381,#173382,#173383,#173384,#173385,
#173386,#173387,#173388,#173389,#173390,#173391,#173392,#173393,#173394,
#173395,#173396,#173397,#173398,#173399,#173400,#173401,#173402,#173403,
#173404,#173405,#173406,#173407,#173408,#173409,#173410,#173411,#173412,
#173413,#173414,#173415,#173416,#173417,#173418,#173419,#173420,#173421,
#173422,#173423,#173424,#173425,#173426,#173427,#173428,#173429,#173430,
#173431,#173432,#173433,#173434,#173435,#173436,#173437,#173438,#173439,
#173440,#173441,#173442,#173443,#173444,#173445,#173446,#173447,#173448,
#173449,#173450,#173451,#173452,#173453,#173454,#173455,#173456,#173457,
#173458,#173459,#173460,#173461,#173462,#173463,#173464,#173465,#173466,
#173467,#173468,#173469,#173470,#173471,#173472,#173473,#173474,#173475,
#173476,#173477,#173478,#173479,#173480,#173481,#173482,#173483,#173484,
#173485,#173486,#173487,#173488,#173489,#173490,#173491,#173492,#173493,
#173494,#173495,#173496,#173497,#173498,#173499,#173500,#173501,#173502,
#173503,#173504,#173505,#173506,#173507,#173508,#173509,#173510,#173511,
#173512,#173513,#173514,#173515,#173516,#173517,#173518,#173519,#173520,
#173521,#173522,#173523,#173524,#173525,#173526,#173527,#173528,#173529,
#173530,#173531,#173532,#173533,#173534,#173535,#173536,#173537,#173538,
#173539,#173540,#173541,#173542,#173543,#173544,#173545,#173546,#173547,
#173548,#173549,#173550,#173551,#173552,#173553,#173554,#173555,#173556,
#173557,#173558,#173559,#173560,#173561,#173562,#173563,#173564,#173565,
#173566,#173567,#173568,#173569,#173570,#173571,#173572,#173573,#173574,
#173575,#173576,#173577,#173578,#173579,#173580,#173581,#173582),
 .UNSPECIFIED.,.F.,.F.,(4,3,3,3,3,3,3,3,3,3,3,3,3,3,3,3,3,3,3,3,3,3,3,3,
3,3,3,3,3,3,3,3,3,3,3,3,3,3,3,3,3,3,3,3,3,3,3,3,3,3,3,3,3,3,3,3,3,3,3,3,
3,3,3,3,3,3,3,3,3,3,3,3,3,3,3,3,3,3,3,3,3,3,3,3,3,4),(260.752190247953,
260.825502775604,260.89874534631,260.971919280042,261.045053716347,261.118158903979,
261.140782514055,261.216524878878,261.292312999627,261.368156170469,261.444111128729,
261.520127561063,261.596263356563,261.639251057362,261.715461637835,261.791604242088,
261.867689328428,261.943727314701,262.019728585256,262.096786030096,262.172751292221,
262.248712884085,262.324680211146,262.402557194354,262.478586991787,262.557387567882,
262.636188143977,262.707611418827,262.77898154574,262.850312117261,262.921625454747,
262.992926141569,263.064251623061,263.134656687285,263.222362176625,263.310538539043,
263.399142949661,263.487843256543,263.576439516478,263.633125230592,263.706094675042,
263.779018666136,263.851910192877,263.924792391797,263.997667309841,264.070570259551,
264.1315937739,264.210894557849,264.290217488325,264.369560090336,264.448933167509,
264.528314848507,264.607711625615,264.630062317208,264.709459711877,264.788843385705,
264.868210837346,264.947556021158,265.026879040424,265.106173270045,265.128530860515,
265.201433260783,265.274313117828,265.347183387261,265.420079731666,265.492988387451,
265.565956700399,265.626999403823,265.715573735436,265.80427410091,265.892840913013,
265.981184326577,266.068954043202,266.12546794713,266.19679144548,266.268095195635,
266.339392698906,266.410725194553,266.482073553292,266.553494208259,266.623936490438,
266.709040194389,266.793997180456,266.878810120939,266.963290026646,267.035375555065),
 .UNSPECIFIED.);
#3230=B_SPLINE_CURVE_WITH_KNOTS('',3,(#173584,#173585,#173586,#173587,#173588,
#173589,#173590,#173591,#173592,#173593,#173594,#173595,#173596,#173597,
#173598),.UNSPECIFIED.,.F.,.F.,(4,1,1,1,1,1,1,1,1,1,1,1,4),(254.469004940773,
254.660691451056,255.657628537672,256.156097080979,256.654565624287,257.153034167594,
257.651502710902,258.149971254209,258.648439797517,259.146908340824,259.645376884132,
260.642313970747,260.752190247953),.UNSPECIFIED.);
#3231=B_SPLINE_CURVE_WITH_KNOTS('',3,(#173600,#173601,#173602,#173603,#173604,
#173605,#173606,#173607,#173608,#173609,#173610,#173611,#173612,#173613,
#173614,#173615,#173616,#173617,#173618,#173619,#173620,#173621,#173622,
#173623,#173624,#173625,#173626,#173627,#173628,#173629,#173630,#173631,
#173632,#173633,#173634,#173635,#173636,#173637,#173638,#173639,#173640,
#173641,#173642,#173643,#173644,#173645,#173646,#173647,#173648,#173649,
#173650,#173651,#173652,#173653,#173654,#173655,#173656,#173657,#173658,
#173659,#173660,#173661,#173662,#173663,#173664,#173665,#173666,#173667,
#173668,#173669,#173670,#173671,#173672,#173673,#173674,#173675,#173676,
#173677,#173678,#173679,#173680,#173681,#173682,#173683,#173684,#173685,
#173686,#173687,#173688,#173689,#173690,#173691,#173692,#173693,#173694,
#173695,#173696,#173697,#173698,#173699,#173700,#173701,#173702,#173703,
#173704,#173705,#173706,#173707,#173708,#173709,#173710,#173711,#173712,
#173713,#173714,#173715,#173716,#173717,#173718,#173719,#173720,#173721,
#173722,#173723,#173724,#173725,#173726,#173727,#173728,#173729,#173730,
#173731,#173732,#173733,#173734,#173735,#173736,#173737,#173738,#173739,
#173740,#173741,#173742,#173743,#173744,#173745,#173746,#173747,#173748,
#173749,#173750,#173751,#173752,#173753,#173754,#173755,#173756,#173757,
#173758,#173759,#173760,#173761,#173762,#173763,#173764,#173765,#173766,
#173767,#173768,#173769,#173770,#173771,#173772,#173773,#173774,#173775,
#173776,#173777,#173778,#173779,#173780,#173781,#173782,#173783,#173784,
#173785,#173786,#173787,#173788,#173789,#173790,#173791,#173792,#173793,
#173794,#173795,#173796,#173797,#173798,#173799,#173800,#173801,#173802,
#173803,#173804,#173805,#173806,#173807,#173808,#173809,#173810,#173811,
#173812,#173813,#173814,#173815,#173816,#173817,#173818,#173819,#173820,
#173821,#173822,#173823,#173824,#173825,#173826,#173827,#173828,#173829,
#173830,#173831,#173832,#173833,#173834,#173835,#173836,#173837,#173838,
#173839,#173840,#173841,#173842,#173843,#173844,#173845,#173846,#173847,
#173848,#173849,#173850,#173851,#173852,#173853,#173854,#173855),
 .UNSPECIFIED.,.F.,.F.,(4,3,3,3,3,3,3,3,3,3,3,3,3,3,3,3,3,3,3,3,3,3,3,3,
3,3,3,3,3,3,3,3,3,3,3,3,3,3,3,3,3,3,3,3,3,3,3,3,3,3,3,3,3,3,3,3,3,3,3,3,
3,3,3,3,3,3,3,3,3,3,3,3,3,3,3,3,3,3,3,3,3,3,3,3,3,4),(248.185820251478,
248.266341504436,248.346973689163,248.429997499714,248.510857010287,248.594962970826,
248.679068931366,248.750492206216,248.821862333129,248.893192904651,248.964506242137,
249.035806928959,249.107132410451,249.177537474673,249.265242964013,249.353419326431,
249.442023737048,249.53072404393,249.619320303864,249.676006017981,249.748975462431,
249.821899453525,249.894790980266,249.967673179187,250.040548097231,250.113451046941,
250.174474561288,250.253775345237,250.333098275714,250.412440877725,250.491813954897,
250.571195635894,250.650592413002,250.672943104596,250.752340499265,250.831724173093,
250.911091624734,250.990436808546,251.069759827812,251.149054057433,251.171411647904,
251.244314048173,251.317193905218,251.390064174651,251.462960519057,251.535869174842,
251.60883748779,251.669880191211,251.758454522823,251.847154888296,251.935721700398,
252.024065113961,252.111834830586,252.168348734519,252.239672232869,252.310975983024,
252.382273486296,252.453605981943,252.524954340682,252.596374995649,252.666817277826,
252.742920773847,252.818973919918,252.894987110153,252.970970710034,253.046935063362,
253.124037475997,253.200009204035,253.275993531294,253.351999872967,253.429938495836,
253.506047535264,253.584900949852,253.663754364441,253.739887236686,253.815926937757,
253.891882943129,253.967741385666,254.043542449219,254.119281769953,254.162222907749,
254.234133288965,254.306079971583,254.378048461525,254.450075949408,254.469004940773),
 .UNSPECIFIED.);
#3232=B_SPLINE_CURVE_WITH_KNOTS('',3,(#173857,#173858,#173859,#173860,#173861,
#173862,#173863,#173864,#173865,#173866,#173867,#173868,#173869,#173870,
#173871,#173872,#173873,#173874,#173875,#173876,#173877,#173878,#173879,
#173880,#173881,#173882,#173883,#173884,#173885,#173886,#173887,#173888,
#173889,#173890,#173891,#173892,#173893,#173894,#173895,#173896,#173897,
#173898,#173899,#173900,#173901,#173902,#173903,#173904,#173905,#173906,
#173907,#173908,#173909,#173910,#173911,#173912,#173913,#173914,#173915,
#173916,#173917,#173918,#173919,#173920,#173921,#173922,#173923,#173924,
#173925,#173926,#173927,#173928,#173929,#173930,#173931,#173932,#173933,
#173934,#173935,#173936,#173937,#173938,#173939,#173940,#173941,#173942,
#173943,#173944,#173945,#173946,#173947,#173948,#173949,#173950,#173951,
#173952,#173953,#173954,#173955,#173956,#173957,#173958,#173959,#173960,
#173961,#173962,#173963,#173964,#173965,#173966,#173967,#173968,#173969,
#173970,#173971,#173972,#173973,#173974,#173975,#173976,#173977,#173978,
#173979,#173980,#173981,#173982,#173983,#173984,#173985,#173986,#173987,
#173988,#173989,#173990,#173991,#173992,#173993,#173994,#173995,#173996,
#173997,#173998,#173999,#174000,#174001,#174002,#174003,#174004,#174005,
#174006,#174007,#174008,#174009,#174010,#174011,#174012,#174013,#174014,
#174015,#174016,#174017,#174018,#174019,#174020,#174021,#174022,#174023,
#174024,#174025,#174026,#174027,#174028,#174029,#174030,#174031,#174032,
#174033,#174034,#174035,#174036,#174037,#174038,#174039,#174040,#174041,
#174042,#174043,#174044,#174045,#174046,#174047,#174048,#174049,#174050,
#174051,#174052,#174053,#174054,#174055,#174056,#174057,#174058,#174059,
#174060,#174061,#174062,#174063,#174064,#174065,#174066,#174067,#174068,
#174069,#174070,#174071,#174072,#174073,#174074,#174075,#174076,#174077,
#174078,#174079,#174080,#174081,#174082,#174083,#174084,#174085,#174086,
#174087,#174088,#174089,#174090,#174091,#174092,#174093,#174094,#174095,
#174096,#174097,#174098,#174099,#174100,#174101,#174102,#174103,#174104,
#174105,#174106,#174107,#174108,#174109,#174110,#174111,#174112,#174113,
#174114,#174115),.UNSPECIFIED.,.F.,.F.,(4,3,3,3,3,3,3,3,3,3,3,3,3,3,3,3,
3,3,3,3,3,3,3,3,3,3,3,3,3,3,3,3,3,3,3,3,3,3,3,3,3,3,3,3,3,3,3,3,3,3,3,3,
3,3,3,3,3,3,3,3,3,3,3,3,3,3,3,3,3,3,3,3,3,3,3,3,3,3,3,3,3,3,3,3,3,3,4),
(241.902634326414,241.971086085413,242.039528364561,242.107964736407,242.176423951892,
242.198977868367,242.286683357707,242.374859720126,242.463464130744,242.552164437627,
242.640760697563,242.697446411675,242.770415856125,242.843339847219,242.91623137396,
242.989113572881,243.061988490924,243.134891440634,243.195914954983,243.275215738932,
243.354538669409,243.43388127142,243.513254348593,243.59263602959,243.672032806699,
243.69438349829,243.773780892958,243.853164566786,243.932532018426,244.011877202238,
244.091200221503,244.170494451125,244.192852041598,244.265754441867,244.338634298912,
244.411504568346,244.484400912751,244.557309568536,244.630277881485,244.691320584905,
244.779894916517,244.86859528199,244.957162094092,245.045505507656,245.133275224281,
245.189789128213,245.261112626563,245.332416376718,245.403713879991,245.475046375638,
245.546394734377,245.617815389344,245.68825767152,245.764361167541,245.840414313611,
245.916427503847,245.992411103727,246.068375457055,246.14547786969,246.221449597729,
246.297433924988,246.37344026666,246.451378889529,246.527487928957,246.606341343547,
246.685194758136,246.761327630381,246.837367331453,246.913323336824,246.989181779361,
247.064982842916,247.14072216365,247.183663301443,247.259405666265,247.335193787014,
247.411036957855,247.486991916115,247.563008348449,247.639144143949,247.682131844751,
247.761518664415,247.840814500136,247.92001827371,247.999090510025,248.078078319358,
248.156948820267,248.185819633594),.UNSPECIFIED.);
#3233=B_SPLINE_CURVE_WITH_KNOTS('',3,(#174117,#174118,#174119,#174120,#174121,
#174122,#174123,#174124,#174125,#174126,#174127,#174128,#174129,#174130,
#174131,#174132,#174133,#174134,#174135,#174136,#174137,#174138,#174139,
#174140,#174141,#174142,#174143,#174144,#174145,#174146,#174147,#174148,
#174149,#174150,#174151,#174152,#174153,#174154,#174155,#174156,#174157,
#174158,#174159,#174160,#174161,#174162,#174163,#174164,#174165,#174166,
#174167,#174168,#174169,#174170,#174171,#174172,#174173,#174174,#174175,
#174176,#174177,#174178,#174179,#174180,#174181,#174182,#174183,#174184,
#174185,#174186,#174187,#174188,#174189,#174190,#174191,#174192,#174193,
#174194,#174195,#174196,#174197,#174198,#174199,#174200,#174201,#174202,
#174203,#174204,#174205,#174206,#174207,#174208,#174209,#174210,#174211,
#174212,#174213,#174214,#174215,#174216,#174217,#174218,#174219,#174220,
#174221,#174222,#174223,#174224,#174225,#174226,#174227,#174228,#174229,
#174230,#174231,#174232,#174233,#174234,#174235,#174236,#174237,#174238,
#174239,#174240,#174241,#174242,#174243,#174244,#174245,#174246,#174247,
#174248,#174249,#174250,#174251,#174252,#174253,#174254,#174255,#174256,
#174257,#174258,#174259,#174260,#174261,#174262,#174263,#174264,#174265,
#174266,#174267,#174268,#174269,#174270,#174271,#174272,#174273,#174274,
#174275,#174276,#174277,#174278,#174279,#174280,#174281,#174282,#174283,
#174284,#174285,#174286,#174287,#174288,#174289,#174290,#174291,#174292,
#174293,#174294,#174295,#174296,#174297,#174298,#174299,#174300,#174301,
#174302,#174303,#174304,#174305,#174306,#174307,#174308,#174309,#174310,
#174311,#174312,#174313,#174314,#174315,#174316,#174317,#174318,#174319,
#174320,#174321,#174322,#174323,#174324,#174325,#174326,#174327,#174328,
#174329,#174330,#174331,#174332,#174333,#174334,#174335,#174336,#174337,
#174338,#174339,#174340,#174341,#174342,#174343,#174344,#174345,#174346,
#174347,#174348,#174349,#174350,#174351,#174352,#174353,#174354,#174355,
#174356,#174357,#174358,#174359,#174360,#174361,#174362,#174363,#174364,
#174365,#174366,#174367,#174368,#174369,#174370,#174371,#174372,#174373,
#174374,#174375,#174376,#174377,#174378,#174379,#174380,#174381,#174382,
#174383,#174384,#174385,#174386,#174387,#174388,#174389,#174390,#174391,
#174392,#174393,#174394,#174395,#174396,#174397,#174398,#174399,#174400,
#174401,#174402,#174403,#174404,#174405,#174406,#174407,#174408,#174409,
#174410,#174411,#174412,#174413,#174414,#174415,#174416,#174417,#174418,
#174419,#174420,#174421,#174422,#174423,#174424,#174425,#174426,#174427,
#174428,#174429,#174430,#174431,#174432,#174433,#174434,#174435,#174436,
#174437,#174438,#174439,#174440,#174441,#174442,#174443,#174444,#174445,
#174446,#174447,#174448,#174449,#174450,#174451,#174452,#174453,#174454,
#174455,#174456,#174457,#174458,#174459,#174460,#174461,#174462,#174463,
#174464,#174465,#174466,#174467,#174468,#174469,#174470,#174471,#174472,
#174473,#174474,#174475,#174476,#174477,#174478,#174479,#174480,#174481,
#174482,#174483,#174484,#174485,#174486,#174487,#174488,#174489,#174490,
#174491,#174492,#174493,#174494,#174495,#174496,#174497,#174498,#174499,
#174500,#174501,#174502,#174503,#174504,#174505,#174506,#174507,#174508,
#174509,#174510,#174511,#174512,#174513,#174514,#174515,#174516,#174517,
#174518,#174519,#174520,#174521,#174522,#174523,#174524,#174525,#174526,
#174527,#174528,#174529,#174530,#174531,#174532,#174533,#174534,#174535,
#174536,#174537,#174538,#174539,#174540,#174541,#174542,#174543,#174544,
#174545,#174546,#174547,#174548,#174549,#174550,#174551,#174552,#174553,
#174554,#174555,#174556,#174557,#174558,#174559,#174560,#174561,#174562,
#174563,#174564,#174565,#174566,#174567,#174568,#174569,#174570,#174571,
#174572,#174573,#174574,#174575,#174576,#174577,#174578,#174579,#174580,
#174581,#174582,#174583,#174584,#174585,#174586,#174587,#174588,#174589,
#174590,#174591,#174592,#174593,#174594,#174595,#174596,#174597,#174598,
#174599,#174600,#174601,#174602,#174603,#174604,#174605,#174606,#174607,
#174608,#174609,#174610,#174611,#174612,#174613,#174614,#174615,#174616,
#174617,#174618,#174619,#174620,#174621,#174622,#174623,#174624,#174625,
#174626,#174627,#174628,#174629,#174630,#174631,#174632,#174633,#174634,
#174635,#174636,#174637,#174638,#174639,#174640,#174641,#174642,#174643,
#174644,#174645,#174646,#174647,#174648,#174649,#174650,#174651,#174652,
#174653,#174654,#174655,#174656,#174657,#174658,#174659,#174660,#174661,
#174662,#174663,#174664,#174665,#174666,#174667,#174668,#174669,#174670,
#174671,#174672,#174673,#174674,#174675,#174676,#174677,#174678,#174679,
#174680,#174681,#174682,#174683,#174684,#174685,#174686,#174687,#174688,
#174689,#174690,#174691,#174692,#174693,#174694,#174695,#174696,#174697,
#174698,#174699,#174700,#174701,#174702,#174703,#174704,#174705,#174706,
#174707,#174708,#174709,#174710,#174711,#174712,#174713,#174714,#174715,
#174716,#174717,#174718,#174719,#174720,#174721,#174722,#174723,#174724,
#174725,#174726,#174727,#174728,#174729,#174730,#174731,#174732,#174733,
#174734,#174735,#174736,#174737,#174738,#174739,#174740,#174741,#174742,
#174743,#174744,#174745,#174746,#174747,#174748,#174749,#174750,#174751,
#174752,#174753,#174754,#174755,#174756,#174757,#174758,#174759,#174760,
#174761,#174762,#174763,#174764,#174765,#174766,#174767,#174768,#174769,
#174770,#174771,#174772,#174773,#174774,#174775,#174776,#174777,#174778,
#174779,#174780,#174781,#174782,#174783,#174784,#174785,#174786,#174787,
#174788,#174789,#174790,#174791,#174792,#174793,#174794,#174795,#174796,
#174797,#174798,#174799,#174800,#174801,#174802,#174803,#174804,#174805,
#174806,#174807,#174808,#174809,#174810,#174811,#174812,#174813,#174814,
#174815,#174816,#174817,#174818,#174819,#174820,#174821,#174822,#174823,
#174824,#174825,#174826,#174827,#174828,#174829,#174830,#174831,#174832,
#174833,#174834,#174835,#174836,#174837,#174838,#174839,#174840),
 .UNSPECIFIED.,.F.,.F.,(4,2,2,2,2,2,2,2,2,2,2,2,2,2,2,2,2,2,2,2,2,2,2,2,
2,2,2,2,2,2,2,2,2,2,2,2,2,2,2,2,2,2,2,2,2,2,2,2,2,2,2,2,2,2,2,2,2,2,2,2,
2,2,2,2,2,2,2,2,2,2,2,2,2,2,2,2,2,2,2,2,2,2,2,2,2,2,2,2,2,2,2,2,2,2,2,2,
2,2,2,2,2,2,2,2,2,2,2,2,2,2,2,2,2,2,2,2,2,2,2,2,2,2,2,2,2,2,2,2,2,2,2,2,
2,2,2,2,2,2,2,2,2,2,2,2,2,2,2,2,2,2,2,2,2,2,2,2,2,2,2,2,2,2,2,2,2,2,2,2,
2,2,2,2,2,2,2,2,2,2,2,2,2,2,2,2,2,2,2,2,2,2,2,2,2,2,2,2,2,2,2,2,2,2,2,2,
2,2,2,2,2,2,2,2,2,2,2,2,2,2,2,2,2,2,2,2,2,2,2,2,2,2,2,2,2,2,2,2,2,2,2,2,
2,2,2,2,2,2,2,2,2,2,2,2,2,2,2,2,2,2,2,2,2,2,2,2,2,2,2,2,2,2,2,2,2,2,2,2,
2,2,2,2,2,2,2,2,2,2,2,2,2,2,2,2,2,2,2,2,2,2,2,2,2,2,2,2,2,2,2,2,2,2,2,2,
2,2,2,2,2,2,2,2,2,2,2,2,2,2,2,2,2,2,2,2,2,2,2,2,2,2,2,2,2,2,2,2,2,2,2,2,
2,2,2,2,2,2,2,2,2,2,2,2,2,4),(0.0017506814511106,0.134011037079277,0.13863498196845,
0.141510894125579,0.143675180075276,0.145865863922226,0.147898130505966,
0.150670150933493,0.156128800685242,0.218904837886574,0.253373309699606,
0.2713995518874,0.297725977712415,0.334632156279759,0.409083522008049,0.520385300887421,
0.566345439752942,0.573275582751303,0.576845253339605,0.579699806771832,
0.582555458912094,0.587669036252463,0.603126829471007,0.870804288318988,
0.927422212127102,0.970581601793251,0.9848918686534,0.994813468929493,0.998399462885633,
1.0004990220348,1.0027655650585,1.00569105317595,1.01177742138225,1.05391349914012,
1.18009622661855,1.28059987564952,1.33131222945727,1.36347350583833,1.3742407439205,
1.38127738763749,1.38786127635502,1.39614133189458,1.40909256450011,1.47859758061937,
1.49115531215296,1.5587183989163,1.64005073066659,1.74326408723159,1.75266721780301,
1.75746543533536,1.76146386815625,1.76392991630215,1.76618948822263,1.76905778179412,
1.77485609908085,1.81613207590194,1.82162002063461,2.04722861024931,2.15967583498945,
2.17763716563563,2.18283861937298,2.18603146174995,2.18892818765682,2.19264720171819,
2.19859053623103,2.22922431341702,2.44839372180056,2.60656808930926,2.61498178858879,
2.61823134145179,2.62047800348131,2.62268580660917,2.62535667148648,2.63207638564006,
2.73649002110687,2.91260549609256,3.03413850890854,3.06308448618106,3.07720855502232,
3.08848141520548,3.10134674053766,3.12321576501316,3.23927938517667,3.3604710191477,
3.38606604048794,3.40365610122618,3.41093105008172,3.41647652943451,3.42301903706092,
3.43471694238046,3.50662666864935,3.58033455075747,3.59745100796469,3.60861788178852,
3.61933499038916,3.63222292267813,3.66402294061125,3.71871535749359,3.77935003360823,
3.79899838911008,3.81301679475049,3.81975197170663,3.82569941757997,3.83341569888974,
3.84617818421831,3.95715494259211,4.00589568999809,4.05167657705705,4.07205958729372,
4.08830036339894,4.10831340240641,4.15752203024455,4.19208662808957,4.2027216608629,
4.21868518394084,4.23070701819041,4.24812679100687,4.30446165678307,4.32279884076342,
4.3487908836774,4.36569830305274,4.38118537683877,4.40800691424252,4.54680591499908,
4.58521538211865,4.60130133601558,4.61380268835446,4.62071771776603,4.62661544475266,
4.63413771099004,4.65163166787588,4.72859306170826,4.7794707773513,4.81290323400089,
4.82706742233238,4.83771048642375,4.84786367870627,4.86553245227002,4.96137712836724,
4.99648683897189,5.01746877316622,5.02553782008216,5.03125923409228,5.03651960013234,
5.04622401492361,5.07989691039116,5.11427385054093,5.25314699160246,5.25623071765815,
5.3253695358523,5.34544566896279,5.35780433985531,5.36918328765182,5.38423334677144,
5.4185170504197,5.60387741534106,5.73060731515254,5.81277345777961,5.81945616126802,
5.82212094537614,5.82432708697088,5.82657546225993,5.82983364057102,5.83830374325064,
5.87559419445762,5.91338371254504,6.00121395149035,6.08349114182264,6.24063115025451,
6.25041489811844,6.25421925095062,6.25696445715838,6.25988254961366,6.2637523856324,
6.27219685473291,6.42713990977992,6.66057725614571,6.67282472039797,6.67684476981671,
6.67908078259702,6.68133301734677,6.6841252642536,6.68955303741645,6.72623011507484,
6.82397057895111,6.89647080034816,7.03199978699402,7.04829129586106,7.05661374353084,
7.06320296543036,7.07022129295673,7.0809025643062,7.11293057704927,7.3581229076199,
7.43204234632018,7.4389039121332,7.44167054404701,7.44397311887888,7.44633209434472,
7.44977301371144,7.4588451102699,7.50066990425859,7.52835637073232,7.67275058015654,
7.84764416310736,7.85846617419166,7.86243743371532,7.8652279573796,7.86783720469648,
7.87142341399599,7.87843011827409,7.92648394143464,7.98435147450019,8.17240101845266,
8.28706843464876,8.29428068063963,8.29710617341732,8.29915281170705,8.30133568396748,
8.30424203996012,8.31050509690418,8.36196506764097,8.42013955385869,8.51054997994833,
8.61358512606202,8.71226957498,8.74173864000045,8.75595989721054,8.76724261118356,
8.77777253047674,8.79268410061458,8.83872656420922,8.91210062435603,8.98107783247322,
9.03942036151044,9.07690273371647,9.0868965295736,9.09220416584354,9.09722909586111,
9.09724519404607,9.09726125470968,9.09727727820422,9.09729326492776,9.09730921524664,
9.09732512954939,9.09734100822504,9.09735685168681,9.09737266033171,9.09738843450381,
9.09740417465555,9.09741988105226,9.09743555410995,9.09745119426574,9.0974668018405,
9.09748237710095,9.09749792042229,9.09751343221599,9.09752891280702,9.09754436252808,
9.09755978170931,9.09757517077558,9.09759053003072,9.0976058597598,9.09762116025292,
9.09763643191778,9.09765167518182,9.09766689031797,9.09768207759256,9.09769723736394,
9.09771236991245,9.09772747555218,9.09774255465622,9.09775760754086,9.09777263449457,
9.09778763578268,9.0978026117394,9.09781756268493,9.09783248889226,9.09784739071474,
9.09786226846576,9.0978771224258,9.09789195287733,9.09790676006307,9.09792154429873,
9.09793630585734,9.0979510450589,9.09796576219781,9.09798045756381,9.09799513138782,
9.09800978391952,9.09802441549316,9.09803902644034,9.09805361694611,9.09806818736886,
9.09808273795104,9.09809726888821,9.09811178050891,9.09812627306761,9.09814074681622,
9.09815520201693,9.09816963896134,9.10376758873861,9.111705228767,9.12531131906822,
9.15686789419644,9.25454872956124,9.27408222205404,9.28573872111132,9.29592704517915,
9.29603595381324,9.29614336899312,9.29624931848151,9.29635382943915,9.2964569284654,
9.29655864159056,9.29665899427572,9.29675801144607,9.29685571750476,9.29695213632015,
9.31092150276583,9.34412332454436,9.3948351083356,9.47158009032108,9.4894396755397,
9.49702250064662,9.50259915727206,9.50890866066505,9.5089498433501,9.50899116245939,
9.50903262050805,9.50907422032181,9.50911596471042,9.50915785653998,9.50919989870679,
9.50924209410722,9.50928444563142,9.50932695623728,9.50936962886592,9.52063089822793,
9.53504891151008,9.56736593875558,9.63206451171904,9.67800823402137,9.71867947861838,
9.74403185537591,9.75929422515171,9.77511822310509,9.79265678210112,9.80203837035258,
9.82518662032188,9.8865267092225,9.89677661176384,9.90769244598511,9.91987359611358,
9.93937083100793,9.99371491344264,10.0244018205133,10.0401994715322,10.0555506604875,
10.0715617790068,10.0931872119106,10.2274941457884),.UNSPECIFIED.);
#3234=B_SPLINE_CURVE_WITH_KNOTS('',3,(#174842,#174843,#174844,#174845,#174846,
#174847,#174848,#174849,#174850,#174851,#174852,#174853,#174854,#174855,
#174856,#174857,#174858,#174859,#174860,#174861,#174862,#174863,#174864,
#174865,#174866,#174867,#174868,#174869,#174870,#174871,#174872,#174873,
#174874,#174875,#174876,#174877,#174878,#174879,#174880,#174881,#174882,
#174883,#174884,#174885,#174886,#174887,#174888,#174889,#174890,#174891,
#174892,#174893,#174894,#174895,#174896,#174897,#174898,#174899,#174900,
#174901,#174902,#174903,#174904,#174905,#174906,#174907,#174908,#174909,
#174910,#174911,#174912,#174913,#174914,#174915,#174916,#174917,#174918,
#174919,#174920,#174921,#174922,#174923,#174924,#174925,#174926,#174927,
#174928,#174929,#174930,#174931,#174932,#174933,#174934,#174935,#174936,
#174937,#174938,#174939,#174940,#174941,#174942,#174943,#174944,#174945,
#174946,#174947,#174948,#174949,#174950,#174951,#174952,#174953,#174954,
#174955,#174956,#174957,#174958,#174959,#174960,#174961,#174962,#174963,
#174964,#174965,#174966,#174967,#174968,#174969,#174970,#174971,#174972,
#174973,#174974,#174975,#174976,#174977,#174978,#174979,#174980,#174981,
#174982,#174983,#174984,#174985,#174986,#174987,#174988,#174989,#174990,
#174991,#174992,#174993,#174994,#174995,#174996,#174997,#174998,#174999,
#175000,#175001,#175002,#175003,#175004,#175005,#175006,#175007,#175008,
#175009,#175010,#175011,#175012,#175013,#175014,#175015,#175016,#175017,
#175018,#175019,#175020,#175021,#175022,#175023,#175024,#175025,#175026,
#175027,#175028,#175029,#175030,#175031,#175032,#175033,#175034,#175035,
#175036,#175037,#175038,#175039,#175040,#175041,#175042,#175043,#175044,
#175045,#175046,#175047,#175048,#175049,#175050,#175051,#175052,#175053,
#175054,#175055,#175056,#175057,#175058,#175059,#175060,#175061,#175062,
#175063,#175064,#175065,#175066,#175067,#175068,#175069,#175070,#175071,
#175072,#175073,#175074,#175075,#175076,#175077,#175078,#175079,#175080,
#175081,#175082,#175083,#175084,#175085,#175086,#175087,#175088,#175089,
#175090,#175091,#175092,#175093,#175094,#175095,#175096,#175097,#175098,
#175099,#175100,#175101,#175102,#175103,#175104,#175105,#175106,#175107,
#175108,#175109,#175110,#175111,#175112,#175113,#175114,#175115,#175116,
#175117,#175118,#175119,#175120,#175121,#175122,#175123,#175124,#175125,
#175126,#175127,#175128,#175129,#175130,#175131,#175132,#175133,#175134,
#175135,#175136,#175137,#175138,#175139,#175140,#175141,#175142,#175143,
#175144,#175145,#175146,#175147,#175148,#175149,#175150,#175151,#175152,
#175153,#175154,#175155,#175156,#175157,#175158,#175159,#175160,#175161,
#175162,#175163,#175164,#175165,#175166,#175167,#175168,#175169,#175170,
#175171,#175172,#175173,#175174,#175175,#175176,#175177,#175178,#175179,
#175180,#175181,#175182,#175183,#175184,#175185,#175186,#175187,#175188,
#175189,#175190,#175191,#175192,#175193,#175194,#175195,#175196,#175197,
#175198,#175199,#175200,#175201,#175202,#175203,#175204,#175205,#175206,
#175207,#175208,#175209,#175210,#175211,#175212,#175213,#175214,#175215,
#175216,#175217,#175218,#175219,#175220,#175221,#175222,#175223,#175224,
#175225,#175226,#175227,#175228,#175229,#175230,#175231,#175232,#175233,
#175234,#175235,#175236,#175237,#175238,#175239,#175240,#175241,#175242,
#175243,#175244,#175245,#175246,#175247,#175248,#175249,#175250,#175251,
#175252,#175253,#175254,#175255,#175256,#175257,#175258,#175259,#175260,
#175261,#175262,#175263,#175264,#175265,#175266,#175267,#175268,#175269,
#175270,#175271,#175272,#175273,#175274,#175275,#175276,#175277,#175278,
#175279,#175280,#175281,#175282,#175283,#175284,#175285,#175286,#175287,
#175288,#175289,#175290,#175291,#175292,#175293,#175294,#175295,#175296,
#175297,#175298,#175299,#175300,#175301,#175302,#175303,#175304,#175305,
#175306,#175307,#175308,#175309,#175310,#175311,#175312,#175313,#175314,
#175315,#175316,#175317,#175318,#175319,#175320,#175321,#175322,#175323,
#175324,#175325,#175326,#175327,#175328,#175329,#175330,#175331,#175332,
#175333,#175334,#175335,#175336,#175337,#175338,#175339,#175340,#175341,
#175342,#175343,#175344,#175345,#175346,#175347,#175348,#175349,#175350,
#175351,#175352,#175353,#175354,#175355,#175356,#175357,#175358,#175359,
#175360,#175361,#175362,#175363,#175364,#175365,#175366,#175367,#175368,
#175369,#175370,#175371,#175372,#175373,#175374,#175375,#175376,#175377),
 .UNSPECIFIED.,.F.,.F.,(4,2,2,2,2,2,2,2,2,2,2,2,2,2,2,2,2,2,2,2,2,2,2,2,
2,2,2,2,2,2,2,2,2,2,2,2,2,2,2,2,2,2,2,2,2,2,2,2,2,2,2,2,2,2,2,2,2,2,2,2,
2,2,2,2,2,2,2,2,2,2,2,2,2,2,2,2,2,2,2,2,2,2,2,2,2,2,2,2,2,2,2,2,2,2,2,2,
2,2,2,2,2,2,2,2,2,2,2,2,2,2,2,2,2,2,2,2,2,2,2,2,2,2,2,2,2,2,2,2,2,2,2,2,
2,2,2,2,2,2,2,2,2,2,2,2,2,2,2,2,2,2,2,2,2,2,2,2,2,2,2,2,2,2,2,2,2,2,2,2,
2,2,2,2,2,2,2,2,2,2,2,2,2,2,2,2,2,2,2,2,2,2,2,2,2,2,2,2,2,2,2,2,2,2,2,2,
2,2,2,2,2,2,2,2,2,2,2,2,2,2,2,2,2,2,2,2,2,2,2,2,2,2,2,2,2,2,2,2,2,2,2,2,
2,2,2,2,2,2,2,2,2,2,2,2,2,2,2,2,2,2,2,2,2,2,2,2,2,2,2,4),(0.00186199678217356,
0.0534072979824111,0.0629898090321268,0.0695601494279824,0.0751767148818409,
0.081119914342048,0.0882323224250048,0.108582833537339,0.120014112296188,
0.203904176637935,0.250671400770191,0.272139577502702,0.273284294429323,
0.274372228732696,0.275421424796998,0.28528162156847,0.295223186251498,
0.308477269692847,0.33651753295084,0.431316100633483,0.455932033728342,
0.467580263714209,0.476973769804133,0.482500531018475,0.487972346737579,
0.4945887990737,0.510873655122722,0.610289448462213,0.660207728472387,0.766253107149157,
0.792238054434032,0.803560964927062,0.815072251199551,0.825684800096252,
0.840229596362484,0.879090724950023,1.00301836409177,1.16210646173142,1.23756629235987,
1.25810633829328,1.26645302392921,1.27268951732162,1.27557748692769,1.27775685346682,
1.27980775996973,1.28265112476593,1.28997396512792,1.41279317645232,1.52105185422502,
1.69582821530593,1.70435400707048,1.70823872164865,1.71115880351145,1.71389916748984,
1.71768619160247,1.72736823423339,1.87816109685742,1.95516211163061,2.11858483014467,
2.12426447842029,2.12878884687946,2.13148577607152,2.13351329618611,2.13607255430391,
2.1404260284835,2.15550520917435,2.15747627858046,2.17616517692931,2.21389904244859,
2.32342555704627,2.46812510259257,2.48680693445919,2.50181511942128,2.50964131649009,
2.51620535040733,2.52245013671291,2.53278012677793,2.55973231510332,2.74841402331646,
2.873114803034,2.88870314273191,2.89291871757978,2.89544723103635,2.89770390617979,
2.90055083225084,2.90606143705936,2.94070146978887,3.14963064321459,3.30360678583918,
3.31204459005846,3.31591247137814,3.3188295461504,3.32157413169692,3.32537815969253,
3.33516397015224,3.49316497869749,3.57607230090745,3.67668993474441,3.69985539312709,
3.72796268969078,3.74414131525996,3.74828426164853,3.75072678303652,3.75288041094717,
3.75556263903683,3.75969819528162,3.77853987043052,4.00154252461507,4.09065663081161,
4.17489935622442,4.19790193134568,4.21085880797874,4.22211801530399,4.23609854206547,
4.2631543396556,4.45156081044648,4.50267536253318,4.52199090878683,4.53620024361153,
4.54288460809449,4.54844502206459,4.55543249288046,4.56658636389042,4.63221635151138,
4.68498349709671,4.71827272971454,4.73235048010506,4.74297760046393,4.7545960508579,
4.77391251574424,4.87686220568772,4.93135915160501,4.94442023131774,4.95099951915212,
4.95697812575695,4.96479371962575,4.97820825493997,5.04856759527427,5.11385388301294,
5.17705707378499,5.19722334136655,5.21383241490362,5.23168332090402,5.26535862352199,
5.29572252496139,5.33867414986147,5.35238743352054,5.36533766955413,5.39789401081938,
5.45766394357715,5.48155591903656,5.49820056457008,5.5163916527567,5.54860467717707,
5.58925602725705,5.71820743358845,5.73942154051105,5.74726212401161,5.75289030180623,
5.75888748102626,5.76801484153087,5.80272905916415,5.89390196145271,5.93893469869855,
5.95497420334539,5.96483716868131,5.97566020513873,5.99097636918636,6.03419831920534,
6.12597397133509,6.14732351179798,6.15483762352221,6.16016213165038,6.16581649880847,
6.17431904181378,6.2007947281686,6.35067156021419,6.38480538282014,6.45549630701774,
6.47570277153914,6.48808666366836,6.49945279733003,6.51443249269318,6.54830479557834,
6.72600471931166,6.82483162071745,6.9430956073783,6.94961596574745,6.95229720944739,
6.95450724002338,6.95674978735377,6.95998194976302,6.96828806985215,7.1265360373614,
7.21853174650482,7.37086070386074,7.38061188920959,7.38441023446956,7.38715339001454,
7.39007142252451,7.3939447849756,7.40241128529133,7.56334721790338,7.73852412333251,
7.79888961203032,7.80513076217893,7.80805399045748,7.81032643284637,7.81278860423803,
7.81532062805158,7.82296003664465,7.83380438231452,7.97204126044276,8.14589521011125,
8.17305740099466,8.18341283674055,8.18966211179188,8.19557021959188,8.20267129028787,
8.21529299392772,8.23072956420941,8.36777838079023,8.53969866739713,8.55793286765043,
8.56716912042244,8.57074506539148,8.5728938704501,8.57517246422569,8.57818675319267,
8.58460735667885,8.63391710960613,8.74802283071234,8.82531502385275,8.97843621313215,
8.98813079430965,8.99191974870661,8.99466048371041,8.99758000590887,9.00146234191693,
9.00997636464759,9.18113179060977,9.28168368875777,9.41381921510857,9.42265232114481,
9.4260740300293,9.4281275422882,9.43030537944654,9.43318405168816,9.43634545633717,
9.45187636663706,9.5049671831726,9.63864459027471,9.70180423477838,9.83478022474929,
9.86854322981692,9.88334565242782,9.8947232432244,9.90520541755825,9.91726476300876,
9.93440758216976,10.0757893204251,10.0782104616455,10.130921252948,10.2026985925259,
10.2141748651263,10.2201503452187,10.2233006616878,10.2246888159593),
 .UNSPECIFIED.);
#3235=B_SPLINE_CURVE_WITH_KNOTS('',3,(#175379,#175380,#175381,#175382,#175383,
#175384,#175385,#175386,#175387,#175388,#175389,#175390,#175391,#175392,
#175393,#175394,#175395,#175396,#175397,#175398,#175399,#175400,#175401,
#175402,#175403,#175404,#175405,#175406,#175407,#175408,#175409,#175410,
#175411,#175412,#175413,#175414,#175415,#175416,#175417,#175418,#175419,
#175420,#175421,#175422,#175423,#175424,#175425,#175426,#175427,#175428,
#175429,#175430,#175431,#175432,#175433,#175434,#175435,#175436,#175437,
#175438,#175439,#175440,#175441,#175442,#175443,#175444,#175445,#175446,
#175447,#175448,#175449,#175450,#175451,#175452,#175453,#175454,#175455,
#175456,#175457,#175458,#175459,#175460,#175461,#175462,#175463,#175464,
#175465,#175466,#175467,#175468,#175469,#175470,#175471,#175472,#175473,
#175474,#175475,#175476,#175477,#175478,#175479,#175480,#175481,#175482,
#175483,#175484,#175485,#175486,#175487,#175488,#175489,#175490,#175491,
#175492,#175493,#175494,#175495,#175496,#175497,#175498,#175499,#175500,
#175501,#175502,#175503,#175504,#175505,#175506,#175507,#175508,#175509,
#175510,#175511,#175512,#175513,#175514,#175515,#175516,#175517,#175518,
#175519,#175520,#175521,#175522,#175523,#175524,#175525,#175526,#175527,
#175528,#175529,#175530,#175531,#175532,#175533,#175534,#175535,#175536,
#175537,#175538,#175539,#175540,#175541,#175542,#175543,#175544,#175545,
#175546,#175547,#175548,#175549,#175550,#175551,#175552,#175553,#175554,
#175555,#175556,#175557,#175558,#175559,#175560,#175561,#175562,#175563,
#175564,#175565,#175566,#175567,#175568,#175569,#175570,#175571,#175572,
#175573,#175574,#175575,#175576,#175577,#175578,#175579,#175580,#175581,
#175582,#175583,#175584,#175585,#175586,#175587,#175588,#175589,#175590,
#175591,#175592,#175593,#175594,#175595,#175596,#175597,#175598,#175599,
#175600,#175601,#175602,#175603,#175604,#175605,#175606,#175607,#175608,
#175609,#175610,#175611,#175612,#175613,#175614,#175615,#175616,#175617,
#175618,#175619,#175620,#175621,#175622,#175623,#175624,#175625,#175626,
#175627,#175628,#175629,#175630,#175631,#175632,#175633,#175634,#175635,
#175636,#175637,#175638,#175639,#175640,#175641,#175642,#175643,#175644,
#175645,#175646,#175647,#175648,#175649,#175650,#175651,#175652,#175653,
#175654,#175655,#175656,#175657,#175658,#175659,#175660,#175661,#175662,
#175663,#175664,#175665,#175666,#175667,#175668,#175669,#175670,#175671,
#175672,#175673,#175674,#175675,#175676,#175677,#175678,#175679,#175680,
#175681,#175682,#175683,#175684,#175685,#175686,#175687,#175688,#175689,
#175690,#175691,#175692,#175693,#175694,#175695,#175696,#175697,#175698,
#175699,#175700,#175701,#175702,#175703,#175704,#175705,#175706,#175707,
#175708,#175709,#175710,#175711,#175712,#175713,#175714,#175715,#175716,
#175717,#175718,#175719,#175720,#175721,#175722,#175723,#175724,#175725,
#175726,#175727,#175728,#175729,#175730,#175731,#175732,#175733,#175734,
#175735,#175736,#175737,#175738,#175739,#175740,#175741,#175742,#175743,
#175744,#175745,#175746,#175747,#175748,#175749,#175750,#175751,#175752,
#175753,#175754,#175755,#175756,#175757,#175758,#175759,#175760,#175761,
#175762,#175763,#175764,#175765,#175766,#175767,#175768,#175769,#175770,
#175771,#175772,#175773,#175774,#175775,#175776,#175777,#175778,#175779,
#175780,#175781,#175782,#175783,#175784,#175785,#175786,#175787,#175788,
#175789,#175790,#175791,#175792,#175793,#175794,#175795,#175796,#175797,
#175798,#175799,#175800,#175801,#175802,#175803,#175804,#175805,#175806,
#175807,#175808,#175809,#175810,#175811,#175812,#175813,#175814,#175815,
#175816,#175817,#175818,#175819,#175820,#175821,#175822,#175823,#175824,
#175825,#175826,#175827,#175828,#175829,#175830,#175831,#175832,#175833,
#175834,#175835,#175836,#175837,#175838,#175839,#175840,#175841,#175842,
#175843,#175844,#175845,#175846,#175847,#175848,#175849,#175850,#175851,
#175852,#175853,#175854,#175855,#175856,#175857,#175858,#175859,#175860,
#175861,#175862,#175863,#175864,#175865,#175866,#175867,#175868,#175869,
#175870,#175871,#175872,#175873,#175874,#175875,#175876,#175877,#175878,
#175879,#175880,#175881,#175882,#175883,#175884,#175885,#175886,#175887,
#175888,#175889,#175890,#175891,#175892,#175893,#175894,#175895,#175896,
#175897,#175898,#175899,#175900,#175901,#175902,#175903,#175904,#175905,
#175906,#175907,#175908,#175909,#175910,#175911,#175912,#175913,#175914,
#175915,#175916,#175917,#175918,#175919,#175920,#175921,#175922,#175923,
#175924,#175925,#175926,#175927,#175928,#175929,#175930,#175931,#175932,
#175933,#175934,#175935,#175936,#175937,#175938,#175939,#175940,#175941,
#175942,#175943,#175944,#175945,#175946),.UNSPECIFIED.,.F.,.F.,(4,2,2,2,
2,2,2,2,2,2,2,2,2,2,2,2,2,2,2,2,2,2,2,2,2,2,2,2,2,2,2,2,2,2,2,2,2,2,2,2,
2,2,2,2,2,2,2,2,2,2,2,2,2,2,2,2,2,2,2,2,2,2,2,2,2,2,2,2,2,2,2,2,2,2,2,2,
2,2,2,2,2,2,2,2,2,2,2,2,2,2,2,2,2,2,2,2,2,2,2,2,2,2,2,2,2,2,2,2,2,2,2,2,
2,2,2,2,2,2,2,2,2,2,2,2,2,2,2,2,2,2,2,2,2,2,2,2,2,2,2,2,2,2,2,2,2,2,2,2,
2,2,2,2,2,2,2,2,2,2,2,2,2,2,2,2,2,2,2,2,2,2,2,2,2,2,2,2,2,2,2,2,2,2,2,2,
2,2,2,2,2,2,2,2,2,2,2,2,2,2,2,2,2,2,2,2,2,2,2,2,2,2,2,2,2,2,2,2,2,2,2,2,
2,2,2,2,2,2,2,2,2,2,2,2,2,2,2,2,2,2,2,2,2,2,2,2,2,2,2,2,2,2,2,2,2,2,2,2,
2,2,2,2,2,2,2,2,2,2,2,2,2,2,2,2,2,2,2,2,2,2,2,2,2,2,2,4),(0.00188190206533328,
0.00394021362682194,0.00859255636028643,0.0192593108961252,0.0763073776529958,
0.13039204283185,0.169294902247269,0.181048040623909,0.190948316303338,
0.201514682354913,0.215072105645199,0.24468029956132,0.33646633764414,0.37325433031622,
0.388089829256446,0.396316335471121,0.402008134682251,0.407631898860544,
0.41333215793546,0.421447689260994,0.444585169692429,0.571292694284215,
0.611756096805257,0.621064326911909,0.626383090426756,0.629608099546713,
0.631433580688767,0.633723600211907,0.635549775856493,0.636984939885039,
0.638099289844188,0.638956115619663,0.639609811136581,0.655217908181767,
0.670970293096031,0.689956399348377,0.736273085148862,0.774843265168787,
0.798067317351602,0.809276671969745,0.823393418882983,0.867810357299684,
0.924145869669683,0.940207667926138,0.954967542592683,0.97419169732368,
1.01241387708126,1.12796747826932,1.16867623363583,1.18535156836009,1.19466719712562,
1.20113402152816,1.20674535197142,1.21271936258327,1.22008102801901,1.24238664980676,
1.31661522242514,1.36534685560889,1.38771851572256,1.40579596117075,1.41569901214977,
1.42538064937492,1.43811426835037,1.4624073585641,1.54933480888982,1.59755983691416,
1.60774331583143,1.61307769051002,1.61829702453316,1.6253205419314,1.64061451933967,
1.76875418237282,1.86032773109508,1.8962906893597,1.92355280407125,1.93486202201446,
1.94636558129077,1.95698804989473,1.97157338927446,2.00176953722281,2.12630672902658,
2.23993389259797,2.36123028584463,2.39766834475812,2.40382249096465,2.40673334814975,
2.40891631772271,2.4109606576616,2.41377921658978,2.41942082491633,2.49461972866057,
2.64569242208153,2.82703154397473,2.835575305209,2.83946328527691,2.8423838006839,
2.84512309637037,2.84890631420152,2.85856616420846,3.00596244379951,3.16599919944367,
3.24404448987258,3.25694787007714,3.26088798024286,3.26335499830134,3.26562622589582,
3.26854062568793,3.27332438101888,3.29982333355065,3.46299596640571,3.55027865537353,
3.6205775003343,3.6342887330012,3.64196274858779,3.64849189093521,3.65589402960894,
3.66834956363616,3.71248765073057,3.75167699345357,3.82050701850602,3.90111983843628,
4.00577542185636,4.01524398632385,4.02222494379172,4.02531871996827,4.02761033249559,
4.02973602398435,4.03263515997484,4.0383433526799,4.10475750941039,4.25406004791312,
4.4239570695574,4.4403738408984,4.44540624053903,4.44856092631052,4.45146742589732,
4.45519910434056,4.46131853482933,4.49473268794736,4.78254012027149,4.86371722699902,
4.87643753794344,4.88024766622227,4.88261618216237,4.88478520008413,4.88759891162846,
4.89350437599001,4.93618641792744,5.11408454039127,5.28591262776393,5.32154040317637,
5.3356913067907,5.34725807638374,5.35903874373822,5.37634481016825,5.42561552312411,
5.54737889030724,5.59345699241652,5.64874871993721,5.66584711736607,5.67260176558865,
5.67820532253348,5.68438899738462,5.69469923302105,5.74710161830624,5.84130773624172,
5.85929414249924,5.86950537565795,5.88012537562142,5.89411664934785,5.92641219551067,
5.97461979844949,6.04585903950909,6.07122786329442,6.07894089839188,6.08436165927916,
6.09056584153224,6.09973477018372,6.1259617990716,6.15069112060431,6.22838161100326,
6.3058878893645,6.32965232916615,6.34621240367765,6.36419669778839,6.39908343992429,
6.47025454937043,6.48414476414463,6.49697452545205,6.52787592629551,6.58747888407595,
6.61248395614754,6.62926707273742,6.64714617489393,6.67759380475321,6.78292088530635,
6.86035494872068,6.87365418039129,6.88143944712878,6.88741509808642,6.89401725735288,
6.90720959851432,6.92530419994896,6.9771355598698,7.06132736608888,7.08213927786219,
7.09418175483623,7.10462687852032,7.11789222589014,7.14598535119953,7.18626007253536,
7.22913279705064,7.27579414277792,7.28596129674123,7.2915079086961,7.29652101487956,
7.3037656569116,7.32117059646132,7.3464049971747,7.46707325528123,7.5841775558822,
7.60610010136548,7.61897772187771,7.63024971760534,7.64435727239795,7.67321145775631,
7.79402629132358,7.96772044760927,8.07551532636859,8.08221781876246,8.08488595778167,
8.08709310913079,8.08934072673616,8.0925945809095,8.10103555068788,8.25914363427256,
8.47633848470989,8.50868295190553,8.51473707560164,8.51844966251296,8.5213539394339,
8.52445540843903,8.52936040052161,8.53512389444153,8.54605109495126,8.6440613137291,
8.76895956265577,8.92724585772357,8.93653949457682,8.94012794504473,8.9422781867819,
8.94455608695947,8.94756279957616,8.95407144357245,9.09339671263441,9.21559569567429,
9.29718064547672,9.31196046140954,9.31984406107301,9.32640851503893,9.33352024462134,
9.34463967878358,9.38044694322873,9.43611586327997,9.57602308524526,9.69437094429324,
9.70062017611394,9.70365083835392,9.70581172726951,9.70808537828086,9.71106351264648,
9.71742103396116,9.81172048805468,10.0261267527293,10.0423886006616,10.1137206403557,
10.1213803219175,10.1251783738698,10.1279219944405,10.1306892248764,10.1335219851595,
10.1371966236365,10.1429500464066,10.2269540975582),.UNSPECIFIED.);
#3236=B_SPLINE_CURVE_WITH_KNOTS('',3,(#175948,#175949,#175950,#175951,#175952,
#175953,#175954,#175955,#175956,#175957,#175958,#175959,#175960,#175961,
#175962,#175963,#175964,#175965,#175966,#175967,#175968,#175969,#175970,
#175971,#175972,#175973,#175974,#175975,#175976,#175977,#175978,#175979,
#175980,#175981,#175982,#175983,#175984,#175985,#175986,#175987,#175988,
#175989,#175990,#175991,#175992,#175993,#175994,#175995,#175996,#175997,
#175998,#175999,#176000,#176001,#176002,#176003,#176004,#176005,#176006,
#176007,#176008,#176009,#176010,#176011,#176012,#176013,#176014,#176015,
#176016,#176017,#176018,#176019,#176020,#176021,#176022,#176023,#176024,
#176025,#176026,#176027,#176028,#176029,#176030,#176031,#176032,#176033,
#176034,#176035,#176036,#176037,#176038,#176039,#176040,#176041,#176042,
#176043,#176044,#176045,#176046,#176047,#176048,#176049,#176050,#176051,
#176052,#176053,#176054,#176055,#176056,#176057,#176058,#176059,#176060,
#176061,#176062,#176063,#176064,#176065,#176066,#176067,#176068,#176069,
#176070,#176071,#176072,#176073,#176074,#176075,#176076,#176077,#176078,
#176079,#176080,#176081,#176082,#176083,#176084,#176085,#176086,#176087,
#176088,#176089,#176090,#176091,#176092,#176093,#176094,#176095,#176096,
#176097,#176098,#176099,#176100,#176101,#176102,#176103,#176104,#176105,
#176106,#176107,#176108,#176109,#176110,#176111,#176112,#176113,#176114,
#176115,#176116,#176117,#176118,#176119,#176120,#176121,#176122,#176123,
#176124,#176125,#176126,#176127,#176128,#176129,#176130,#176131,#176132,
#176133,#176134,#176135,#176136,#176137,#176138,#176139,#176140,#176141,
#176142,#176143,#176144,#176145,#176146,#176147,#176148,#176149,#176150,
#176151,#176152,#176153,#176154,#176155,#176156,#176157,#176158,#176159,
#176160,#176161,#176162,#176163,#176164,#176165,#176166,#176167,#176168,
#176169,#176170,#176171,#176172,#176173,#176174,#176175,#176176,#176177,
#176178,#176179,#176180,#176181,#176182,#176183,#176184,#176185,#176186,
#176187,#176188,#176189,#176190,#176191,#176192,#176193,#176194,#176195,
#176196,#176197,#176198,#176199,#176200,#176201,#176202,#176203),
 .UNSPECIFIED.,.F.,.F.,(4,3,3,3,3,3,3,3,3,3,3,3,3,3,3,3,3,3,3,3,3,3,3,3,
3,3,3,3,3,3,3,3,3,3,3,3,3,3,3,3,3,3,3,3,3,3,3,3,3,3,3,3,3,3,3,3,3,3,3,3,
3,3,3,3,3,3,3,3,3,3,3,3,3,3,3,3,3,3,3,3,3,3,3,3,3,4),(197.920337176157,
197.994164212812,198.067915796059,198.141589609895,198.21521846511,198.288810978896,
198.333746057302,198.409488422125,198.485276542875,198.561119713718,198.637074671978,
198.713091104313,198.789226899813,198.83221460061,198.908425181084,198.984567785336,
199.060652871676,199.136690857949,199.212692128503,199.289749573344,199.365714835468,
199.441676427333,199.517643754394,199.595520737602,199.671550535035,199.75035111113,
199.829151687225,199.900574962075,199.971945088988,200.043275660509,200.114588997995,
200.185889684817,200.257215166309,200.327620230533,200.415325719874,200.503502082292,
200.59210649291,200.680806799793,200.769403059729,200.82608877384,200.89905821829,
200.971982209383,201.044873736124,201.117755935044,201.190630853087,201.263533802797,
201.324557317148,201.403858101098,201.483181031574,201.562523633586,201.641896710759,
201.721278391757,201.800675168866,201.823025860455,201.902423255123,201.981806928951,
202.061174380592,202.140519564404,202.21984258367,202.299136813291,202.321494403763,
202.394396804032,202.467276661077,202.54014693051,202.613043274915,202.6859519307,
202.758920243649,202.81996294707,202.908537278682,202.997237644155,203.085804456258,
203.174147869823,203.261917586448,203.318431490378,203.389754988728,203.461058738883,
203.532356242156,203.603688737803,203.675037096542,203.746457751509,203.816900033686,
203.903674402841,203.990284356058,204.076705714213,204.162709280465,204.203522318931),
 .UNSPECIFIED.);
#3237=B_SPLINE_CURVE_WITH_KNOTS('',3,(#176205,#176206,#176207,#176208,#176209,
#176210,#176211,#176212,#176213,#176214,#176215,#176216,#176217,#176218,
#176219),.UNSPECIFIED.,.F.,.F.,(4,1,1,1,1,1,1,1,1,1,1,1,4),(191.637151868978,
191.853654994304,192.850592080919,193.349060624227,193.847529167534,194.345997710842,
194.844466254149,195.342934797457,195.841403340765,196.339871884072,196.83834042738,
197.835277513995,197.920337176157),.UNSPECIFIED.);
#3238=B_SPLINE_CURVE_WITH_KNOTS('',3,(#176221,#176222,#176223,#176224,#176225,
#176226,#176227,#176228,#176229,#176230,#176231,#176232,#176233,#176234,
#176235,#176236,#176237,#176238,#176239,#176240,#176241,#176242,#176243,
#176244,#176245,#176246,#176247,#176248,#176249,#176250,#176251,#176252,
#176253,#176254,#176255,#176256,#176257,#176258,#176259,#176260,#176261,
#176262,#176263,#176264,#176265,#176266,#176267,#176268,#176269,#176270,
#176271,#176272,#176273,#176274,#176275,#176276,#176277,#176278,#176279,
#176280,#176281,#176282,#176283,#176284,#176285,#176286,#176287,#176288,
#176289,#176290,#176291,#176292,#176293,#176294,#176295,#176296,#176297,
#176298,#176299,#176300,#176301,#176302,#176303,#176304,#176305,#176306,
#176307,#176308,#176309,#176310,#176311,#176312,#176313,#176314,#176315,
#176316,#176317,#176318,#176319,#176320,#176321,#176322,#176323,#176324,
#176325,#176326,#176327,#176328,#176329,#176330,#176331,#176332,#176333,
#176334,#176335,#176336,#176337,#176338,#176339,#176340,#176341,#176342,
#176343,#176344,#176345,#176346,#176347,#176348,#176349,#176350,#176351,
#176352,#176353,#176354,#176355,#176356,#176357,#176358,#176359,#176360,
#176361,#176362,#176363,#176364,#176365,#176366,#176367,#176368,#176369,
#176370,#176371,#176372,#176373,#176374,#176375,#176376,#176377,#176378,
#176379,#176380,#176381,#176382,#176383,#176384,#176385,#176386,#176387,
#176388,#176389,#176390,#176391,#176392,#176393,#176394,#176395,#176396,
#176397,#176398,#176399,#176400,#176401,#176402,#176403,#176404,#176405,
#176406,#176407,#176408,#176409,#176410,#176411,#176412,#176413,#176414,
#176415,#176416,#176417,#176418,#176419,#176420,#176421,#176422,#176423,
#176424,#176425,#176426,#176427,#176428,#176429,#176430,#176431,#176432,
#176433,#176434,#176435,#176436,#176437,#176438,#176439,#176440,#176441,
#176442,#176443,#176444,#176445,#176446,#176447,#176448,#176449,#176450,
#176451,#176452,#176453,#176454,#176455,#176456,#176457,#176458,#176459,
#176460,#176461,#176462,#176463,#176464,#176465,#176466,#176467,#176468,
#176469,#176470,#176471,#176472,#176473,#176474,#176475,#176476),
 .UNSPECIFIED.,.F.,.F.,(4,3,3,3,3,3,3,3,3,3,3,3,3,3,3,3,3,3,3,3,3,3,3,3,
3,3,3,3,3,3,3,3,3,3,3,3,3,3,3,3,3,3,3,3,3,3,3,3,3,3,3,3,3,3,3,3,3,3,3,3,
3,3,3,3,3,3,3,3,3,3,3,3,3,3,3,3,3,3,3,3,3,3,3,3,3,4),(185.353968266458,
185.433608279155,185.513330531198,185.593129643172,185.673039876824,185.753001540758,
185.833039193569,185.872032474613,185.943456083504,186.014826544482,186.086157450001,
186.157471120795,186.228772140797,186.300097954107,186.370501017921,186.458205923838,
186.546381642246,186.634985357635,186.723684960917,186.812280540737,186.868969561229,
186.941939130312,187.014863246311,187.08775489816,187.1606372222,187.233512265437,
187.306415339985,187.367438104536,187.446738835565,187.526061712239,187.605404259861,
187.684777282415,187.764158908868,187.843555632021,187.865906647844,187.94530403915,
188.024687709446,188.104055157406,188.183400337357,188.262723352672,188.342017578244,
188.364375191151,188.437277603237,188.510157472198,188.583027753639,188.655924110162,
188.728832778134,188.801801103328,188.862843734459,188.951418041443,189.040118380849,
189.12868516653,189.217028554337,189.304798247261,189.361312277766,189.432635780675,
189.503939535424,189.575237043324,189.646569543641,189.717917907078,189.78933856677,
189.859780821074,189.935884316139,190.011937461231,190.087950650469,190.163934249335,
190.239898601634,190.317001014891,190.392972741875,190.468957068073,190.54496340868,
190.622902033432,190.699011071797,190.777864489743,190.856717907689,190.932850779911,
191.008890480957,191.084846486298,191.160704928803,191.236505992322,191.312245313017,
191.355186450997,191.426863904643,191.498550254089,191.570294990333,191.637151868978),
 .UNSPECIFIED.);
#3239=B_SPLINE_CURVE_WITH_KNOTS('',3,(#176478,#176479,#176480,#176481,#176482,
#176483,#176484,#176485,#176486,#176487,#176488,#176489,#176490,#176491,
#176492,#176493,#176494,#176495,#176496,#176497,#176498,#176499,#176500,
#176501,#176502,#176503,#176504,#176505,#176506,#176507,#176508,#176509,
#176510,#176511,#176512,#176513,#176514,#176515,#176516,#176517,#176518,
#176519,#176520,#176521,#176522,#176523,#176524,#176525,#176526,#176527,
#176528,#176529,#176530,#176531,#176532,#176533,#176534,#176535,#176536,
#176537,#176538,#176539,#176540,#176541,#176542,#176543,#176544,#176545,
#176546,#176547,#176548,#176549,#176550,#176551,#176552,#176553,#176554,
#176555,#176556,#176557,#176558,#176559,#176560,#176561,#176562,#176563,
#176564,#176565,#176566,#176567,#176568,#176569,#176570,#176571,#176572,
#176573,#176574,#176575,#176576,#176577,#176578,#176579,#176580,#176581,
#176582,#176583,#176584,#176585,#176586,#176587,#176588,#176589,#176590,
#176591,#176592,#176593,#176594,#176595,#176596,#176597,#176598,#176599,
#176600,#176601,#176602,#176603,#176604,#176605,#176606,#176607,#176608,
#176609,#176610,#176611,#176612,#176613,#176614,#176615,#176616,#176617,
#176618,#176619,#176620,#176621,#176622,#176623,#176624,#176625,#176626,
#176627,#176628,#176629,#176630,#176631,#176632,#176633,#176634,#176635,
#176636,#176637,#176638,#176639,#176640,#176641,#176642,#176643,#176644,
#176645,#176646,#176647,#176648,#176649,#176650,#176651,#176652,#176653,
#176654,#176655,#176656,#176657,#176658,#176659,#176660,#176661,#176662,
#176663,#176664,#176665,#176666,#176667,#176668,#176669,#176670,#176671,
#176672,#176673,#176674,#176675,#176676,#176677,#176678,#176679,#176680,
#176681,#176682,#176683,#176684,#176685,#176686,#176687,#176688,#176689,
#176690,#176691,#176692,#176693,#176694,#176695,#176696,#176697,#176698,
#176699,#176700,#176701,#176702,#176703,#176704,#176705,#176706,#176707,
#176708,#176709,#176710,#176711,#176712,#176713,#176714,#176715,#176716,
#176717,#176718,#176719,#176720,#176721,#176722,#176723,#176724,#176725,
#176726,#176727,#176728,#176729,#176730,#176731,#176732,#176733),
 .UNSPECIFIED.,.F.,.F.,(4,3,3,3,3,3,3,3,3,3,3,3,3,3,3,3,3,3,3,3,3,3,3,3,
3,3,3,3,3,3,3,3,3,3,3,3,3,3,3,3,3,3,3,3,3,3,3,3,3,3,3,3,3,3,3,3,3,3,3,3,
3,3,3,3,3,3,3,3,3,3,3,3,3,3,3,3,3,3,3,3,3,3,3,3,3,4),(179.071060446364,
179.140082435305,179.209090416259,179.278088452461,179.347109745067,179.391941411615,
179.478877889249,179.566207692725,179.653898138385,179.74167150702,179.829365837672,
179.890409954923,179.963618397179,180.03678211922,180.109913970165,180.183036814402,
180.256152680139,180.329296142636,180.38887849823,180.468009009373,180.547158375392,
180.626325060468,180.705520759866,180.784724865077,180.863945321648,180.887347041538,
180.966805552748,181.04625110072,181.125680838219,181.205088211607,181.284473109547,
181.363828276015,181.385815584845,181.458712668952,181.53158721015,181.604452166954,
181.677343218298,181.750246588051,181.823209649975,181.884284128153,181.972844519505,
182.061529962692,182.150081408985,182.238409708929,182.326165309575,182.382752671461,
182.454080858286,182.525389340606,182.59669161852,182.66802894482,182.739382169653,
182.810807728317,182.881221214768,182.957322968518,183.033374332627,183.109385705406,
183.185367456511,183.261329933897,183.338433479833,183.414403285331,183.490385678004,
183.566390076668,183.644332132847,183.720439231401,183.799298766392,183.878158301383,
183.954292780035,184.030334077574,184.106291666431,184.182151666093,184.257954270009,
184.333695099835,184.376626844691,184.452368681572,184.528156266499,184.603998894723,
184.679953303427,184.755969182361,184.832104422473,184.875095387998,184.955360700984,
185.035527324997,185.115534876663,185.195441645898,185.275182204737,185.353966561798),
 .UNSPECIFIED.);
#3240=B_SPLINE_CURVE_WITH_KNOTS('',3,(#176735,#176736,#176737,#176738,#176739,
#176740,#176741,#176742,#176743,#176744,#176745,#176746,#176747,#176748,
#176749,#176750,#176751,#176752),.UNSPECIFIED.,.F.,.F.,(4,2,2,2,2,2,2,2,
4),(172.787615115558,173.616953723877,174.446311500315,175.275669276753,
176.105027053191,176.934384829629,177.763742606067,178.593100382505,179.070559707459),
 .UNSPECIFIED.);
#3241=B_SPLINE_CURVE_WITH_KNOTS('',3,(#176754,#176755,#176756,#176757,#176758,
#176759,#176760,#176761,#176762,#176763,#176764,#176765,#176766,#176767,
#176768,#176769,#176770,#176771,#176772,#176773,#176774,#176775,#176776,
#176777,#176778,#176779,#176780,#176781,#176782,#176783,#176784,#176785,
#176786,#176787,#176788,#176789,#176790,#176791,#176792,#176793,#176794,
#176795,#176796,#176797,#176798,#176799,#176800,#176801,#176802,#176803,
#176804,#176805,#176806,#176807,#176808,#176809,#176810,#176811,#176812,
#176813,#176814,#176815,#176816,#176817,#176818,#176819,#176820,#176821,
#176822,#176823,#176824,#176825,#176826,#176827,#176828,#176829,#176830,
#176831,#176832,#176833,#176834,#176835,#176836,#176837,#176838,#176839,
#176840,#176841,#176842,#176843,#176844,#176845,#176846,#176847,#176848,
#176849,#176850,#176851,#176852,#176853,#176854,#176855,#176856,#176857,
#176858,#176859,#176860,#176861,#176862,#176863,#176864,#176865,#176866,
#176867,#176868,#176869,#176870,#176871,#176872,#176873,#176874,#176875,
#176876,#176877,#176878,#176879,#176880,#176881,#176882,#176883,#176884,
#176885,#176886,#176887,#176888,#176889,#176890,#176891,#176892,#176893,
#176894,#176895,#176896,#176897,#176898,#176899,#176900,#176901,#176902,
#176903,#176904,#176905,#176906,#176907,#176908,#176909,#176910,#176911,
#176912,#176913,#176914,#176915,#176916,#176917,#176918,#176919,#176920,
#176921,#176922,#176923,#176924,#176925,#176926,#176927,#176928,#176929,
#176930,#176931,#176932,#176933,#176934,#176935,#176936,#176937,#176938,
#176939,#176940,#176941,#176942,#176943,#176944,#176945,#176946,#176947,
#176948,#176949,#176950,#176951,#176952,#176953,#176954,#176955,#176956,
#176957,#176958,#176959,#176960,#176961,#176962,#176963,#176964,#176965,
#176966,#176967,#176968,#176969,#176970,#176971,#176972,#176973,#176974,
#176975,#176976,#176977,#176978,#176979,#176980,#176981,#176982,#176983,
#176984,#176985,#176986,#176987,#176988,#176989,#176990,#176991,#176992,
#176993,#176994,#176995,#176996,#176997,#176998,#176999,#177000,#177001,
#177002,#177003,#177004,#177005,#177006,#177007,#177008,#177009,#177010,
#177011,#177012),.UNSPECIFIED.,.F.,.F.,(4,3,3,3,3,3,3,3,3,3,3,3,3,3,3,3,
3,3,3,3,3,3,3,3,3,3,3,3,3,3,3,3,3,3,3,3,3,3,3,3,3,3,3,3,3,3,3,3,3,3,3,3,
3,3,3,3,3,3,3,3,3,3,3,3,3,3,3,3,3,3,3,3,3,3,3,3,3,3,3,3,3,3,3,3,3,3,4),
(166.50441064026,166.591077657514,166.678165952141,166.765382727969,166.852612902676,
166.930227828926,167.004952485645,167.07962597182,167.154259832905,167.228868307067,
167.303460981558,167.3780613422,167.428696372234,167.504955810607,167.581218455649,
167.657492989338,167.733812277222,167.810154807913,167.886556388693,167.927164915541,
168.009045625696,168.090907992134,168.174589358813,168.256321060986,168.340977259917,
168.425633458849,168.500342464523,168.575047121226,168.649758778482,168.724515678092,
168.799296472705,168.874146305281,168.924102002156,168.999080317636,169.074001238328,
169.148877146241,169.223720393406,169.298543309392,169.376355281814,169.451193529657,
169.526049886415,169.600935534566,169.67586167053,169.750877546777,169.825946010883,
169.901113334991,169.921039088772,169.993549286924,170.065971833029,170.138321444504,
170.210612766232,170.282860386779,170.35507885297,170.42729625324,170.499516401872,
170.571752443362,170.644017533473,170.716368450606,170.788765235898,170.861274470341,
170.917976175387,170.992828246169,171.067594179148,171.142286845693,171.216919070322,
171.291503638633,171.369429841554,171.44396293689,171.518490023338,171.593022627302,
171.66757227602,171.74217856016,171.816817859411,171.891530059673,171.914913262002,
171.991308989042,172.067640616653,172.143917021567,172.220137494927,172.296323925243,
172.37248297344,172.413381805309,172.489576062331,172.565831662664,172.642117280169,
172.718482558834,172.787248854564),.UNSPECIFIED.);
#3242=B_SPLINE_CURVE_WITH_KNOTS('',3,(#177014,#177015,#177016,#177017,#177018,
#177019,#177020,#177021,#177022,#177023,#177024,#177025,#177026,#177027,
#177028,#177029,#177030,#177031),.UNSPECIFIED.,.F.,.F.,(4,2,2,2,2,2,2,2,
4),(160.22122533308,161.050583109518,161.879940885956,162.709298662394,
163.538656438832,164.36801421527,165.197371991708,166.026729768145,166.50441064026),
 .UNSPECIFIED.);
#3243=B_SPLINE_CURVE_WITH_KNOTS('',3,(#177033,#177034,#177035,#177036,#177037,
#177038,#177039,#177040,#177041,#177042,#177043,#177044,#177045,#177046,
#177047,#177048,#177049,#177050,#177051,#177052,#177053,#177054,#177055,
#177056,#177057,#177058,#177059,#177060,#177061,#177062,#177063,#177064,
#177065,#177066,#177067,#177068,#177069,#177070,#177071,#177072,#177073,
#177074,#177075,#177076,#177077,#177078,#177079,#177080,#177081,#177082,
#177083,#177084,#177085,#177086,#177087,#177088,#177089,#177090,#177091,
#177092,#177093,#177094,#177095,#177096,#177097,#177098,#177099,#177100,
#177101,#177102,#177103,#177104,#177105,#177106,#177107,#177108,#177109,
#177110,#177111,#177112,#177113,#177114,#177115,#177116,#177117,#177118,
#177119,#177120,#177121,#177122,#177123,#177124,#177125,#177126,#177127,
#177128,#177129,#177130,#177131,#177132,#177133,#177134,#177135,#177136,
#177137,#177138,#177139,#177140,#177141,#177142,#177143,#177144,#177145,
#177146,#177147,#177148,#177149,#177150,#177151,#177152,#177153,#177154,
#177155,#177156,#177157,#177158,#177159,#177160,#177161,#177162,#177163,
#177164,#177165,#177166,#177167,#177168,#177169,#177170,#177171,#177172,
#177173,#177174,#177175,#177176,#177177,#177178,#177179,#177180,#177181,
#177182,#177183,#177184,#177185,#177186,#177187,#177188,#177189,#177190,
#177191,#177192,#177193,#177194,#177195,#177196,#177197,#177198,#177199,
#177200,#177201,#177202,#177203,#177204,#177205,#177206,#177207,#177208,
#177209,#177210,#177211,#177212,#177213,#177214,#177215,#177216,#177217,
#177218,#177219,#177220,#177221,#177222,#177223,#177224,#177225,#177226,
#177227,#177228,#177229,#177230,#177231,#177232,#177233,#177234,#177235,
#177236,#177237,#177238,#177239,#177240,#177241,#177242,#177243,#177244,
#177245,#177246,#177247,#177248,#177249,#177250,#177251,#177252,#177253,
#177254,#177255,#177256,#177257,#177258,#177259,#177260,#177261,#177262,
#177263,#177264,#177265,#177266,#177267,#177268,#177269,#177270,#177271,
#177272,#177273,#177274,#177275,#177276,#177277,#177278,#177279,#177280,
#177281,#177282,#177283,#177284,#177285,#177286,#177287,#177288,#177289,
#177290,#177291,#177292,#177293,#177294,#177295,#177296,#177297,#177298,
#177299,#177300,#177301,#177302,#177303,#177304,#177305,#177306,#177307,
#177308,#177309,#177310,#177311,#177312,#177313,#177314,#177315,#177316,
#177317,#177318,#177319,#177320,#177321,#177322,#177323,#177324,#177325,
#177326,#177327,#177328,#177329,#177330,#177331,#177332,#177333,#177334,
#177335,#177336,#177337,#177338,#177339,#177340,#177341,#177342,#177343,
#177344,#177345,#177346,#177347,#177348,#177349,#177350,#177351,#177352,
#177353,#177354,#177355,#177356,#177357,#177358,#177359,#177360,#177361,
#177362,#177363,#177364,#177365,#177366,#177367,#177368,#177369,#177370,
#177371,#177372,#177373,#177374,#177375,#177376,#177377,#177378,#177379,
#177380,#177381,#177382,#177383,#177384,#177385,#177386,#177387,#177388,
#177389,#177390,#177391,#177392,#177393,#177394,#177395,#177396,#177397,
#177398,#177399,#177400,#177401,#177402,#177403,#177404,#177405,#177406,
#177407,#177408,#177409,#177410,#177411,#177412,#177413,#177414,#177415,
#177416,#177417,#177418,#177419,#177420,#177421,#177422,#177423,#177424,
#177425,#177426,#177427,#177428,#177429,#177430,#177431,#177432,#177433,
#177434,#177435,#177436,#177437,#177438,#177439,#177440,#177441,#177442,
#177443,#177444,#177445,#177446,#177447,#177448,#177449,#177450,#177451,
#177452,#177453,#177454,#177455,#177456,#177457,#177458,#177459,#177460,
#177461,#177462,#177463,#177464,#177465,#177466,#177467,#177468,#177469,
#177470,#177471,#177472,#177473,#177474,#177475,#177476,#177477,#177478,
#177479,#177480,#177481,#177482,#177483,#177484,#177485,#177486,#177487,
#177488,#177489,#177490,#177491,#177492,#177493,#177494,#177495,#177496,
#177497,#177498,#177499,#177500,#177501,#177502,#177503,#177504,#177505,
#177506,#177507,#177508,#177509,#177510,#177511,#177512,#177513,#177514,
#177515,#177516,#177517,#177518,#177519,#177520,#177521,#177522,#177523,
#177524,#177525,#177526,#177527,#177528,#177529,#177530,#177531,#177532,
#177533,#177534,#177535,#177536,#177537,#177538,#177539,#177540,#177541,
#177542,#177543,#177544,#177545,#177546,#177547,#177548,#177549,#177550,
#177551,#177552,#177553,#177554,#177555,#177556,#177557,#177558,#177559,
#177560,#177561,#177562,#177563,#177564,#177565,#177566,#177567,#177568,
#177569,#177570,#177571,#177572,#177573,#177574,#177575,#177576,#177577,
#177578,#177579,#177580,#177581,#177582,#177583,#177584,#177585,#177586,
#177587,#177588,#177589,#177590,#177591,#177592,#177593,#177594,#177595,
#177596,#177597,#177598,#177599,#177600,#177601,#177602,#177603,#177604,
#177605,#177606,#177607,#177608,#177609,#177610,#177611,#177612,#177613,
#177614,#177615,#177616,#177617,#177618,#177619,#177620,#177621,#177622,
#177623,#177624,#177625,#177626,#177627,#177628,#177629,#177630,#177631,
#177632,#177633,#177634,#177635,#177636,#177637,#177638,#177639,#177640,
#177641,#177642,#177643,#177644,#177645,#177646,#177647,#177648,#177649,
#177650,#177651,#177652,#177653,#177654,#177655,#177656,#177657,#177658,
#177659,#177660,#177661,#177662,#177663,#177664,#177665,#177666,#177667,
#177668,#177669,#177670,#177671,#177672,#177673,#177674,#177675,#177676,
#177677,#177678,#177679,#177680,#177681,#177682,#177683,#177684,#177685,
#177686,#177687,#177688,#177689,#177690,#177691,#177692,#177693,#177694,
#177695,#177696,#177697,#177698,#177699,#177700,#177701,#177702,#177703,
#177704,#177705,#177706,#177707,#177708,#177709,#177710,#177711,#177712,
#177713,#177714,#177715,#177716,#177717,#177718,#177719,#177720,#177721,
#177722,#177723,#177724,#177725,#177726,#177727,#177728,#177729,#177730,
#177731,#177732,#177733,#177734,#177735,#177736,#177737,#177738),
 .UNSPECIFIED.,.F.,.F.,(4,2,2,2,2,2,2,2,2,2,2,2,2,2,2,2,2,2,2,2,2,2,2,2,
2,2,2,2,2,2,2,2,2,2,2,2,2,2,2,2,2,2,2,2,2,2,2,2,2,2,2,2,2,2,2,2,2,2,2,2,
2,2,2,2,2,2,2,2,2,2,2,2,2,2,2,2,2,2,2,2,2,2,2,2,2,2,2,2,2,2,2,2,2,2,2,2,
2,2,2,2,2,2,2,2,2,2,2,2,2,2,2,2,2,2,2,2,2,2,2,2,2,2,2,2,2,2,2,2,2,2,2,2,
2,2,2,2,2,2,2,2,2,2,2,2,2,2,2,2,2,2,2,2,2,2,2,2,2,2,2,2,2,2,2,2,2,2,2,2,
2,2,2,2,2,2,2,2,2,2,2,2,2,2,2,2,2,2,2,2,2,2,2,2,2,2,2,2,2,2,2,2,2,2,2,2,
2,2,2,2,2,2,2,2,2,2,2,2,2,2,2,2,2,2,2,2,2,2,2,2,2,2,2,2,2,2,2,2,2,2,2,2,
2,2,2,2,2,2,2,2,2,2,2,2,2,2,2,2,2,2,2,2,2,2,2,2,2,2,2,2,2,2,2,2,2,2,2,2,
2,2,2,2,2,2,2,2,2,2,2,2,2,2,2,2,2,2,2,2,2,2,2,2,2,2,2,2,2,2,2,2,2,2,2,2,
2,2,2,2,2,2,2,2,2,2,2,2,2,2,2,2,2,2,2,2,2,2,2,2,2,2,2,2,2,2,2,2,2,2,2,2,
2,2,2,2,4),(0.00175465339390005,0.0106630426745053,0.0205737566905323,0.0309773363492851,
0.0449011586812518,0.0761970396275529,0.110081740051457,0.154906126710259,
0.200342621344964,0.207965395092099,0.213623201483809,0.219015379887419,
0.224348799802594,0.234505119131874,0.27387986478419,0.288553455097379,
0.388871765465751,0.469520721251558,0.502286847933687,0.520588609152811,
0.533113087069208,0.543643727004756,0.554918022868189,0.569085328398199,
0.598276863271334,0.694955163729441,0.811946713382373,0.880397741089542,
0.96229181838556,1.00023598821217,1.00664366631311,1.00955245326006,1.01173511729369,
1.01378007837786,1.01715694034604,1.02571813211193,1.15960646309933,1.231986951194,
1.34743429563182,1.38505278697767,1.4321260925016,1.43909640371432,1.4426743327216,
1.44528177472768,1.44807436584836,1.45287312965519,1.4661022137583,1.67529778998201,
1.8024443972039,1.83881086531281,1.85851956117606,1.86282671355505,1.86550927311032,
1.86773473192657,1.87038114418582,1.87500070315741,1.89326354117798,2.0727824063289,
2.20422558955622,2.22200261636897,2.23230807818747,2.23949750633857,2.24650235364747,
2.24652257494582,2.24654297632481,2.24656355833462,2.24658432149997,2.24660526645583,
2.24662639375394,2.24664769464303,2.24666916054298,2.2466908111234,2.24671264688734,
2.2467346682356,2.24675687559219,2.24677927627373,2.24680627064681,2.24683419169507,
2.24686306339174,2.24689290983735,2.24692375523848,2.24695562378715,2.24698853961937,
2.24702252685742,2.25361008826048,2.26193037459867,2.27821743186043,2.41520024762271,
2.48881652761243,2.6076408893715,2.62285978351591,2.62704023172776,2.62956097730095,
2.63181919109457,2.63467952694543,2.64025152628893,2.67667100073445,2.6801632819919,
2.69056279498917,2.72056249537698,2.91564057921407,3.03335529309531,3.04479184239345,
3.04916827364992,3.05218033215583,3.05512902020671,3.05868001523823,3.0675363391675,
3.1509224182157,3.18722207954488,3.35078207476329,3.46387140953021,3.47846893056943,
3.48247117967666,3.48488238195192,3.48704105782159,3.48977343510445,3.49407105574737,
3.51510532041173,3.7344276894245,3.82416355405774,3.88343516625509,3.92336487043767,
3.93927255370562,3.95078478007927,3.96138522400681,3.97870994025716,4.02418286121904,
4.1737049466551,4.18252609574143,4.23574345235269,4.25556443317704,4.27005853099795,
4.27679522408149,4.28235194516456,4.28928991730693,4.30027104546849,4.36774209505622,
4.43681407794521,4.45843073202738,4.47050223284609,4.48104127754417,4.49430469426287,
4.52218683432077,4.57961413039601,4.64336742114334,4.67304495397062,4.68175748704295,
4.6877144503396,4.69341952019469,4.70155340097515,4.72485052229376,4.85138041973883,
4.9118145690509,4.93396798052398,4.95048327675692,4.96924017146467,5.01057576283585,
5.04739173511335,5.06772829715546,5.08360580623047,5.09564070909482,5.11317589063816,
5.16474993950931,5.20547379823957,5.22412641548529,5.24066341876892,5.26300899796339,
5.32537880021096,5.39101363735221,5.39906571605438,5.40035361936073,5.46211468215961,
5.47550908975743,5.48331945846958,5.48929762005054,5.49588098440515,5.50896510218919,
5.56368369698623,5.66631926184257,5.68567031924147,5.69729647557725,5.70792244553632,
5.72198641865309,5.75517563499079,5.80767104934377,5.8737097394826,5.88487605179403,
5.8918673988831,5.89742854249273,5.90411011167432,5.91830238739391,5.92885619821949,
5.96300869569586,6.11185166782372,6.11929222299259,6.18967837912216,6.20985978979228,
6.22223892173322,6.23360762312449,6.24860097277379,6.28255221263302,6.46164481129914,
6.59247447434857,6.67713295465579,6.68383452192659,6.68650199132543,6.68870847137145,
6.69095528677782,6.69420776563978,6.70264398301759,6.71932666896524,6.76469003875785,
6.86356758228398,6.94667238445084,7.10489559386326,7.11468240686054,7.11848659865712,
7.12123122538557,7.12414827255336,7.128015993173,7.13645295447768,7.29021169177013,
7.47340440680141,7.53298727518265,7.53921394630333,7.54213434162317,7.54440629322068,
7.54686964948646,7.55079448358226,7.56357697402388,7.64886521123102,7.80119831084339,
7.89725186175797,7.91129831311978,7.91981244548549,7.92644721782896,7.92646983873642,
7.92649212757603,7.92651409368743,7.92653574125443,7.9265570742788,7.92657809683473,
7.9265988129232,7.92661922649932,7.92663934148035,7.92665916174584,7.92667869115172,
7.92669793348641,7.92671059496794,7.92672322682934,7.92673581245944,7.92674835200075,
7.92676084553945,7.926773293208,7.92678569521957,7.92679805172078,7.92681036282717,
7.92682262863064,7.92683484930343,7.92684702499527,7.9268591558101,7.92687124181451,
7.92688328314052,7.92689527996041,7.92690723240912,7.92691914063808,7.9269310047965,
7.9269428249828,7.92695460131494,7.92696633396561,7.92697802308025,7.92698966874453,
7.92700127104353,7.92701283020738,7.92702434638551,7.92703581957529,7.92704724996283,
7.92705863769546,7.92706998285827,7.9270812856316,7.92709254620274,7.92710376466872,
7.92711494110861,7.92712607559759,7.92713716830416,7.92714821942435,7.9271592289824,
7.92717019719085,7.92718112429855,7.93409296492652,7.94449066890801,7.95646001647683,
7.97840188989325,8.02902241025803,8.13194487355008,8.2315272125584,8.26283442960562,
8.2869942785653,8.30001614832129,8.30412917955994,8.30638538712158,8.30863524778826,
8.31139387138297,8.31645258709696,8.34724690705752,8.37395317190365,8.50062970178918,
8.70800855314985,8.72109115279372,8.72586826469461,8.72865681581129,8.73126596948673,
8.73485477498857,8.74187610203238,8.79038432614299,8.85345721372875,8.93561109011806,
9.01725103177075,9.14674864326658,9.1565051177784,9.16007193310238,9.16215410963622,
9.16410306830219,9.16678551338433,9.17203869378283,9.20662789031212,9.28874525756097,
9.44383117227937,9.56948340111591,9.60296114310369,9.61771876351963,9.62909157337525,
9.63957667520273,9.65165989305312,9.68605312085834,9.73502300585954,9.90252745862155,
9.94013907325383,9.95012727135301,9.95543321301889,9.96081296631798,9.96649105514681,
9.96938421486085,9.98947207774057,10.0313602480716,10.1165080946907,10.1367043676512,
10.1484933387437,10.1587468895274,10.1689780306746,10.1822069942301,10.2248098208976),
 .UNSPECIFIED.);
#3244=B_SPLINE_CURVE_WITH_KNOTS('',3,(#177740,#177741,#177742,#177743,#177744,
#177745,#177746,#177747,#177748,#177749,#177750,#177751,#177752,#177753,
#177754,#177755,#177756,#177757),.UNSPECIFIED.,.F.,.F.,(4,2,2,2,2,2,2,2,
4),(141.371669411541,142.201027187979,143.030384964417,143.859742740855,
144.689100517293,145.518458293731,146.347816070169,147.177173846607,147.654854718721),
 .UNSPECIFIED.);
#3245=B_SPLINE_CURVE_WITH_KNOTS('',3,(#177759,#177760,#177761,#177762,#177763,
#177764,#177765,#177766,#177767,#177768,#177769,#177770,#177771,#177772,
#177773,#177774,#177775,#177776,#177777,#177778,#177779,#177780,#177781,
#177782,#177783,#177784,#177785,#177786,#177787,#177788,#177789,#177790,
#177791,#177792,#177793,#177794,#177795,#177796,#177797,#177798,#177799,
#177800,#177801,#177802,#177803,#177804,#177805,#177806,#177807,#177808,
#177809,#177810,#177811,#177812,#177813,#177814,#177815,#177816,#177817,
#177818,#177819,#177820,#177821,#177822,#177823,#177824,#177825,#177826,
#177827,#177828,#177829,#177830,#177831,#177832,#177833,#177834,#177835,
#177836,#177837,#177838,#177839,#177840,#177841,#177842,#177843,#177844,
#177845,#177846,#177847,#177848,#177849,#177850,#177851,#177852,#177853,
#177854,#177855,#177856,#177857,#177858,#177859,#177860,#177861,#177862,
#177863,#177864,#177865,#177866,#177867,#177868,#177869,#177870,#177871,
#177872,#177873,#177874,#177875,#177876,#177877,#177878,#177879,#177880,
#177881,#177882,#177883,#177884,#177885,#177886,#177887,#177888,#177889,
#177890,#177891,#177892,#177893,#177894,#177895,#177896,#177897,#177898,
#177899,#177900,#177901,#177902,#177903,#177904,#177905,#177906,#177907,
#177908,#177909,#177910,#177911,#177912,#177913,#177914,#177915,#177916,
#177917,#177918,#177919,#177920,#177921,#177922,#177923,#177924,#177925,
#177926,#177927,#177928,#177929,#177930,#177931,#177932,#177933,#177934,
#177935,#177936,#177937,#177938,#177939,#177940,#177941,#177942,#177943,
#177944,#177945,#177946,#177947,#177948,#177949,#177950,#177951,#177952,
#177953,#177954,#177955,#177956,#177957,#177958,#177959,#177960,#177961,
#177962,#177963,#177964,#177965,#177966,#177967,#177968,#177969,#177970,
#177971,#177972,#177973,#177974,#177975,#177976,#177977,#177978,#177979,
#177980,#177981,#177982,#177983,#177984,#177985,#177986,#177987,#177988,
#177989,#177990,#177991,#177992,#177993,#177994,#177995,#177996,#177997,
#177998,#177999,#178000,#178001,#178002,#178003,#178004,#178005,#178006,
#178007,#178008,#178009,#178010,#178011,#178012,#178013,#178014,#178015,
#178016,#178017,#178018,#178019,#178020,#178021,#178022,#178023,#178024,
#178025,#178026,#178027,#178028,#178029,#178030,#178031,#178032,#178033,
#178034,#178035,#178036,#178037,#178038,#178039,#178040,#178041,#178042,
#178043,#178044,#178045,#178046,#178047,#178048,#178049,#178050,#178051,
#178052,#178053,#178054,#178055,#178056,#178057,#178058,#178059,#178060,
#178061,#178062,#178063,#178064,#178065,#178066,#178067,#178068,#178069,
#178070,#178071,#178072,#178073,#178074,#178075,#178076,#178077,#178078,
#178079,#178080,#178081,#178082,#178083,#178084,#178085,#178086,#178087,
#178088,#178089,#178090,#178091,#178092,#178093,#178094,#178095,#178096,
#178097,#178098,#178099,#178100,#178101,#178102,#178103,#178104,#178105,
#178106,#178107,#178108,#178109,#178110,#178111,#178112,#178113,#178114,
#178115,#178116,#178117,#178118,#178119,#178120,#178121,#178122,#178123,
#178124,#178125,#178126,#178127,#178128,#178129,#178130,#178131,#178132,
#178133,#178134,#178135,#178136,#178137,#178138,#178139,#178140,#178141,
#178142,#178143,#178144,#178145,#178146,#178147,#178148,#178149,#178150,
#178151,#178152,#178153,#178154,#178155,#178156,#178157,#178158,#178159,
#178160,#178161,#178162,#178163,#178164,#178165,#178166,#178167,#178168,
#178169,#178170,#178171,#178172,#178173,#178174,#178175,#178176,#178177,
#178178,#178179,#178180,#178181,#178182,#178183,#178184,#178185,#178186,
#178187,#178188,#178189,#178190,#178191,#178192,#178193,#178194,#178195,
#178196,#178197,#178198,#178199,#178200,#178201,#178202,#178203,#178204,
#178205,#178206,#178207,#178208,#178209,#178210,#178211,#178212,#178213,
#178214,#178215,#178216,#178217,#178218,#178219,#178220,#178221,#178222,
#178223,#178224,#178225,#178226,#178227,#178228,#178229,#178230,#178231,
#178232,#178233,#178234,#178235,#178236,#178237,#178238,#178239,#178240,
#178241,#178242,#178243,#178244,#178245,#178246,#178247,#178248,#178249,
#178250,#178251,#178252,#178253,#178254,#178255,#178256,#178257,#178258,
#178259,#178260,#178261,#178262,#178263,#178264,#178265,#178266,#178267,
#178268,#178269,#178270,#178271,#178272,#178273,#178274,#178275,#178276,
#178277,#178278,#178279,#178280,#178281,#178282,#178283,#178284,#178285,
#178286,#178287,#178288,#178289,#178290,#178291,#178292,#178293,#178294,
#178295,#178296,#178297,#178298,#178299,#178300,#178301,#178302,#178303,
#178304,#178305,#178306,#178307,#178308,#178309,#178310,#178311,#178312,
#178313,#178314,#178315,#178316,#178317,#178318,#178319,#178320,#178321,
#178322,#178323,#178324,#178325,#178326,#178327,#178328,#178329,#178330,
#178331,#178332,#178333,#178334,#178335,#178336,#178337,#178338,#178339,
#178340,#178341,#178342,#178343,#178344,#178345,#178346,#178347,#178348,
#178349,#178350,#178351,#178352,#178353,#178354,#178355,#178356,#178357,
#178358,#178359,#178360,#178361,#178362,#178363,#178364,#178365,#178366,
#178367,#178368,#178369,#178370,#178371,#178372,#178373,#178374,#178375,
#178376,#178377,#178378,#178379,#178380,#178381,#178382,#178383,#178384,
#178385,#178386,#178387,#178388,#178389,#178390,#178391,#178392,#178393,
#178394,#178395,#178396,#178397,#178398,#178399,#178400,#178401,#178402,
#178403,#178404,#178405,#178406,#178407,#178408,#178409,#178410,#178411,
#178412,#178413,#178414,#178415,#178416,#178417,#178418,#178419,#178420,
#178421,#178422,#178423,#178424,#178425,#178426,#178427,#178428,#178429,
#178430,#178431,#178432,#178433,#178434,#178435,#178436,#178437,#178438,
#178439,#178440,#178441,#178442,#178443,#178444,#178445,#178446,#178447,
#178448,#178449,#178450,#178451,#178452,#178453,#178454,#178455,#178456,
#178457,#178458,#178459,#178460,#178461,#178462,#178463,#178464,#178465,
#178466,#178467,#178468,#178469,#178470,#178471,#178472,#178473,#178474,
#178475,#178476,#178477,#178478,#178479,#178480,#178481,#178482,#178483,
#178484,#178485,#178486,#178487,#178488,#178489,#178490,#178491,#178492,
#178493,#178494,#178495,#178496,#178497,#178498,#178499,#178500,#178501,
#178502,#178503,#178504,#178505,#178506,#178507,#178508,#178509,#178510,
#178511,#178512,#178513,#178514,#178515,#178516,#178517,#178518,#178519,
#178520,#178521,#178522,#178523,#178524,#178525,#178526,#178527,#178528,
#178529,#178530,#178531,#178532,#178533,#178534,#178535,#178536,#178537,
#178538,#178539,#178540,#178541,#178542,#178543,#178544,#178545,#178546,
#178547,#178548,#178549,#178550,#178551,#178552,#178553,#178554,#178555,
#178556,#178557,#178558,#178559,#178560,#178561,#178562,#178563,#178564,
#178565,#178566,#178567,#178568,#178569,#178570,#178571,#178572,#178573,
#178574,#178575,#178576,#178577,#178578,#178579,#178580,#178581,#178582,
#178583,#178584,#178585,#178586,#178587,#178588),.UNSPECIFIED.,.F.,.F.,
(4,2,2,2,2,2,2,2,2,2,2,2,2,2,2,2,2,2,2,2,2,2,2,2,2,2,2,2,2,2,2,2,2,2,2,
2,2,2,2,2,2,2,2,2,2,2,2,2,2,2,2,2,2,2,2,2,2,2,2,2,2,2,2,2,2,2,2,2,2,2,2,
2,2,2,2,2,2,2,2,2,2,2,2,2,2,2,2,2,2,2,2,2,2,2,2,2,2,2,2,2,2,2,2,2,2,2,2,
2,2,2,2,2,2,2,2,2,2,2,2,2,2,2,2,2,2,2,2,2,2,2,2,2,2,2,2,2,2,2,2,2,2,2,2,
2,2,2,2,2,2,2,2,2,2,2,2,2,2,2,2,2,2,2,2,2,2,2,2,2,2,2,2,2,2,2,2,2,2,2,2,
2,2,2,2,2,2,2,2,2,2,2,2,2,2,2,2,2,2,2,2,2,2,2,2,2,2,2,2,2,2,2,2,2,2,2,2,
2,2,2,2,2,2,2,2,2,2,2,2,2,2,2,2,2,2,2,2,2,2,2,2,2,2,2,2,2,2,2,2,2,2,2,2,
2,2,2,2,2,2,2,2,2,2,2,2,2,2,2,2,2,2,2,2,2,2,2,2,2,2,2,2,2,2,2,2,2,2,2,2,
2,2,2,2,2,2,2,2,2,2,2,2,2,2,2,2,2,2,2,2,2,2,2,2,2,2,2,2,2,2,2,2,2,2,2,2,
2,2,2,2,2,2,2,2,2,2,2,2,2,2,2,2,2,2,2,2,2,2,2,2,2,2,2,2,2,2,2,2,2,2,2,2,
2,2,2,2,2,2,2,2,2,2,2,2,2,2,2,2,2,2,2,2,2,2,2,2,2,2,2,2,2,2,2,2,2,2,2,2,
2,2,2,2,2,2,2,2,2,2,2,2,2,2,2,2,2,2,2,4),(0.00176456259827877,0.0354791527871678,
0.196790374928931,0.253475429305457,0.274104640931416,0.284542362063342,
0.291106759236629,0.296234103287553,0.301801626125252,0.308859133551379,
0.320255975232913,0.375844817145895,0.436723782681839,0.471107303508008,
0.485342329110856,0.495446801019947,0.506562977151543,0.52383811378267,
0.593911156180744,0.645311576428964,0.675832753848066,0.68904210448208,
0.696662161924079,0.70222372346386,0.707553383937515,0.714249923353767,
0.725728347426913,0.778491074454082,0.781901393209374,0.789453164869791,
0.795349999311394,0.881736644163965,0.933512344967916,0.954689503265999,
0.970495528921234,0.98801843038599,1.02550304076582,1.07115699475392,1.08937890788177,
1.08978372106954,1.09018835678865,1.09059290617634,1.09099746387978,1.09140212797604,
1.09152900457176,1.09166693085191,1.09181677872865,1.09197947475155,1.09215600158882,
1.09234739933733,1.09255476669435,1.09277926193263,1.0930221037706,1.09328457217315,
1.09356800910783,1.09387381935848,1.09420347150509,1.09455849913191,1.09494050241539,
1.09535115018395,1.09579218253321,1.09626541404477,1.09677273757903,1.10773187688626,
1.12189044429227,1.1722941283807,1.21992713444815,1.23648429998304,1.24858918538963,
1.25693154003857,1.25966051052207,1.28119014990021,1.33576359763709,1.38291416136558,
1.39212273810709,1.45783968648324,1.47980349801168,1.49099185023654,1.49819518039571,
1.49821670782662,1.49823828167337,1.4982599017126,1.49828156774536,1.49830327944473,
1.49832503654937,1.49834683880696,1.49836868594379,1.49839057774008,1.49841251393612,
1.49843449429614,1.49845651855282,1.49847858645597,1.49850069771643,1.49852285209534,
1.49854504937112,1.49856728930827,1.49858957164872,1.49861189613101,1.49863426252369,
1.49865667055174,1.49867912003272,1.49870161072068,1.49872414235811,1.49874671470344,
1.49876932749285,1.49879198051203,1.49881467353265,1.49883740633635,1.49886017868396,
1.49888299034453,1.49890584110256,1.49892873070505,1.49895165892418,1.4989746255198,
1.49899763026166,1.49902067297547,1.49903716916745,1.49905385501501,1.49907073186526,
1.49908780110115,1.49910506406012,1.49912252210605,1.49914017662258,1.49915802890491,
1.49917608029301,1.49919433208919,1.49921278560538,1.49923144215337,1.49925030306319,
1.49926936957892,1.49928864295883,1.49930812451787,1.49932781547836,1.49934771704632,
1.49936783047152,1.49938815696596,1.49940869777694,1.49942945408252,1.49945042703776,
1.49947161784768,1.49949302765423,1.49951465758479,1.49953650877522,1.4995585823223,
1.4995808793697,1.49960340099519,1.49962614825878,1.49964912220659,1.49967232393198,
1.4996957544459,1.49971941473267,1.4997433058091,1.4997674286692,1.49979178422447,
1.4998163734471,1.49984119728414,1.4998662566769,1.49989155253477,1.49991708572863,
1.49994285712852,1.49996886757687,1.49999511791439,1.50002160896151,1.50004834149911,
1.50007531638276,1.50010253434762,1.50012999613522,1.50015770247099,1.50018565407055,
1.50021385165837,1.50024229590577,1.50027098748616,1.50029992705122,1.50032911523616,
1.50035855264421,1.50038823987576,1.50041817752817,1.50044836614614,1.50047880626074,
1.50050949842875,1.50054044318518,1.50057164101083,1.50060309237956,1.50063479773321,
1.50066675752057,1.50069897218229,1.5007314421186,1.50076416778191,1.50079714952683,
1.50083038769501,1.50702540507998,1.51244979352563,1.52188748072014,1.55668088106553,
1.65196236997401,1.68033067283415,1.70257492163237,1.71478668718972,1.72465178687218,
1.73704873894653,1.76036066872376,1.80004982262211,1.86867673800575,1.88928675816551,
1.89967799802112,1.90748492114413,1.91352229794141,1.91912163103238,1.92763418465396,
1.95196850978629,2.07782744874913,2.20516308820483,2.22115638308586,2.23276745579396,
2.24425164814534,2.25552369799069,2.26969075125086,2.30544133276245,2.49260908038558,
2.64617741777159,2.6931855037452,2.70219623701958,2.70553466718051,2.70779941017734,
2.70999145348589,2.71260036041286,2.71895972417339,2.80100785950158,2.94292982500032,
3.12643034188675,3.13497963351553,3.13886867330947,3.14178938695999,3.14452843248949,
3.14831061641904,3.15796414989909,3.30442510247435,3.35061035880158,3.37813430684796,
3.4834989510071,3.54528322898499,3.55663737668665,3.56039246600406,3.56281836588369,
3.56510478343668,3.56811494310066,3.57456969955984,3.63143821143155,3.7577848189724,
3.8479580806371,3.91968438709121,3.93346707829773,3.94115629558767,3.94768590481128,
3.95507518827764,3.96747224807948,4.01100664604917,4.05124291903256,4.12003136034331,
4.20090663395229,4.28349379219818,4.3170493522518,4.32235961251955,4.32512677127682,
4.32737652459947,4.32962480832831,4.33370809211677,4.34644786312021,4.58511203099722,
4.6914512353215,4.73638562037628,4.74327594231664,4.74683695210505,4.74971678841823,
4.75258296204812,4.75775043593847,4.77361954292603,5.0559477177722,5.1129200885104,
5.17194616267539,5.17734298994204,5.18009915954189,5.18212738984376,5.18432100063871,
5.18729493348649,5.19405880470557,5.30131858674226,5.49609129412834,5.59513670410783,
5.62464431153861,5.63886932521267,5.65014869399534,5.66294249014855,5.68506891353167,
5.81065496176032,5.94157457944028,5.96342611523451,5.97078553059454,5.97592582894265,
5.98175577276171,5.99038844365837,6.01589895685601,6.04163797059443,6.12850894084205,
6.15291950848832,6.16567627040948,6.17618845590054,6.18866124285288,6.21223890940093,
6.22892942538726,6.28319089459611,6.3640231741719,6.37596540008591,6.38236490647448,
6.38840324677182,6.39671374320434,6.41681679171683,6.54571678983377,6.60690032467193,
6.62747657931358,6.64263950993826,6.65992693290219,6.68887409008805,6.73223134724458,
6.76978566477348,6.78343913038217,6.79643871098364,6.82968938781901,6.90304451460922,
6.92150115273641,6.93808613749624,6.96082506224678,7.02747689065037,7.08936670584393,
7.15853563616157,7.17347324265738,7.18097568687398,7.1868972796558,7.19380301320175,
7.20889901403962,7.23065358138959,7.30585780195192,7.36723562955551,7.3845225652254,
7.39460718468134,7.40527743858945,7.41965344658761,7.45505656801025,7.4862749203777,
7.52899705512248,7.57450461618095,7.58465981227175,7.5902031813613,7.5952153072515,
7.602462828953,7.61989211721044,7.64517597551845,7.76588879668253,7.88280610038466,
7.90453091707306,7.91719498257534,7.92822552206921,7.94202474915843,7.96925057697626,
8.07833510960258,8.1598204084289,8.29367565917721,8.34876412057702,8.37618687653631,
8.3808755109823,8.383695728477,8.38587210186303,8.3882148097889,8.39191114634577,
8.40363834136371,8.47321284704257,8.64167553943684,8.80176361182149,8.81156010263576,
8.81536589195685,8.81811101313506,8.82102797618225,8.82489455028041,8.83332490961036,
8.91619784478626,9.03880575830107,9.22341643153359,9.2340624577903,9.23785879425779,
9.2400494762243,9.24208390055859,9.24485917833223,9.25020865367425,9.28478350506138,
9.36722493322371,9.476805404586,9.5032869716063,9.59430308675518,9.60944868662987,
9.61742384699808,9.62385495733904,9.62997192649443,9.63994326682273,9.66662486304035,
9.79825382322865,9.98048350089048,9.99624831128481,10.0006236372703,10.0032129904916,
10.0054621561332,10.0082199292609,10.0134850303902,10.0480856911902,10.0780029776344,
10.2237184582249),.UNSPECIFIED.);
#3246=B_SPLINE_CURVE_WITH_KNOTS('',3,(#178590,#178591,#178592,#178593,#178594,
#178595,#178596,#178597,#178598,#178599,#178600,#178601,#178602,#178603,
#178604),.UNSPECIFIED.,.F.,.F.,(4,1,1,1,1,1,1,1,1,1,1,1,4),(122.522113490003,
122.566527474554,123.064996017861,124.061933104476,124.560401647784,125.058870191091,
125.557338734399,126.055807277706,126.554275821014,127.052744364322,127.551212907629,
128.049681450937,128.805298797182),.UNSPECIFIED.);
#3247=B_SPLINE_CURVE_WITH_KNOTS('',3,(#178606,#178607,#178608,#178609,#178610,
#178611,#178612,#178613,#178614,#178615,#178616,#178617,#178618,#178619,
#178620,#178621,#178622,#178623,#178624,#178625,#178626,#178627,#178628,
#178629,#178630,#178631,#178632,#178633,#178634,#178635,#178636,#178637,
#178638,#178639,#178640,#178641,#178642,#178643,#178644,#178645,#178646,
#178647,#178648,#178649,#178650,#178651,#178652,#178653,#178654,#178655,
#178656,#178657,#178658,#178659,#178660,#178661,#178662,#178663,#178664,
#178665,#178666,#178667,#178668,#178669,#178670,#178671,#178672,#178673,
#178674,#178675,#178676,#178677,#178678,#178679,#178680,#178681,#178682,
#178683,#178684,#178685,#178686,#178687,#178688,#178689,#178690,#178691,
#178692,#178693,#178694,#178695,#178696,#178697,#178698,#178699,#178700,
#178701,#178702,#178703,#178704,#178705,#178706,#178707,#178708,#178709,
#178710,#178711,#178712,#178713,#178714,#178715,#178716,#178717,#178718,
#178719,#178720,#178721,#178722,#178723,#178724,#178725,#178726,#178727,
#178728,#178729,#178730,#178731,#178732,#178733,#178734,#178735,#178736,
#178737,#178738,#178739,#178740,#178741,#178742,#178743,#178744,#178745,
#178746,#178747,#178748,#178749,#178750,#178751,#178752,#178753,#178754,
#178755,#178756,#178757,#178758,#178759,#178760,#178761,#178762,#178763,
#178764,#178765,#178766,#178767,#178768,#178769,#178770,#178771,#178772,
#178773,#178774,#178775,#178776,#178777,#178778,#178779,#178780,#178781,
#178782,#178783,#178784,#178785,#178786,#178787,#178788,#178789,#178790,
#178791,#178792,#178793,#178794,#178795,#178796,#178797,#178798,#178799,
#178800,#178801,#178802,#178803,#178804,#178805,#178806,#178807,#178808,
#178809,#178810,#178811,#178812,#178813,#178814,#178815,#178816,#178817,
#178818,#178819,#178820,#178821,#178822,#178823,#178824,#178825,#178826,
#178827,#178828,#178829,#178830,#178831,#178832,#178833,#178834,#178835,
#178836,#178837,#178838,#178839,#178840,#178841,#178842,#178843,#178844,
#178845,#178846,#178847,#178848,#178849,#178850,#178851,#178852,#178853,
#178854,#178855,#178856,#178857,#178858,#178859,#178860,#178861),
 .UNSPECIFIED.,.F.,.F.,(4,3,3,3,3,3,3,3,3,3,3,3,3,3,3,3,3,3,3,3,3,3,3,3,
3,3,3,3,3,3,3,3,3,3,3,3,3,3,3,3,3,3,3,3,3,3,3,3,3,3,3,3,3,3,3,3,3,3,3,3,
3,3,3,3,3,3,3,3,3,3,3,3,3,3,3,3,3,3,3,3,3,3,3,3,3,4),(116.238928182823,
116.314078890482,116.389167626035,116.46420661482,116.541602475239,116.616581818432,
116.691551253406,116.766521798447,116.841504470604,116.916534326775,116.991592107213,
117.066712158694,117.08337349817,117.15479677302,117.226166899934,117.297497471455,
117.36881080894,117.440111495763,117.511436977255,117.581842041478,117.669547530819,
117.757723893237,117.846328303855,117.935028610738,118.023624870673,118.080310584786,
118.153280029236,118.22620402033,118.299095547071,118.371977745992,118.444852664036,
118.517755613746,118.578779128093,118.658079912042,118.737402842518,118.816745444527,
118.896118521699,118.975500202695,119.054896979803,119.077247671401,119.15664506607,
119.236028739899,119.315396191541,119.394741375354,119.474064394621,119.553358624243,
119.575716214708,119.648618614976,119.721498472021,119.794368741454,119.867265085859,
119.940173741644,120.013142054592,120.074184758016,120.162759089629,120.251459455103,
120.340026267206,120.42836968077,120.516139397397,120.572653301323,120.643976799673,
120.715280549828,120.7865780531,120.857910548747,120.929258907486,121.000679562453,
121.071121844631,121.147225340652,121.223278486723,121.299291676958,121.375275276839,
121.451239630168,121.528342042803,121.604313770841,121.6802980981,121.756304439773,
121.834243062641,121.910352102069,121.989205516658,122.068058931246,122.145066413229,
122.221970743137,122.298741465248,122.375434319171,122.452027422789,122.522113453888),
 .UNSPECIFIED.);
#3248=B_SPLINE_CURVE_WITH_KNOTS('',3,(#178863,#178864,#178865,#178866,#178867,
#178868,#178869,#178870,#178871,#178872,#178873,#178874,#178875,#178876,
#178877,#178878),.UNSPECIFIED.,.F.,.F.,(4,1,1,1,1,1,1,1,1,1,1,1,1,4),(109.955742875643,
110.104813891865,110.603282435172,111.10175097848,111.600219521787,112.098688065095,
112.597156608402,113.09562515171,113.594093695018,114.092562238325,115.08949932494,
115.587967868248,116.086436411555,116.238928182823),.UNSPECIFIED.);
#3249=B_SPLINE_CURVE_WITH_KNOTS('',3,(#178880,#178881,#178882,#178883,#178884,
#178885,#178886,#178887,#178888,#178889,#178890,#178891,#178892,#178893,
#178894,#178895,#178896,#178897,#178898,#178899,#178900,#178901,#178902,
#178903,#178904,#178905,#178906,#178907,#178908,#178909,#178910,#178911,
#178912,#178913,#178914,#178915,#178916,#178917,#178918,#178919,#178920,
#178921,#178922,#178923,#178924,#178925,#178926,#178927,#178928,#178929,
#178930,#178931,#178932,#178933,#178934,#178935,#178936,#178937,#178938,
#178939,#178940,#178941,#178942,#178943,#178944,#178945,#178946,#178947,
#178948,#178949,#178950,#178951,#178952,#178953,#178954,#178955,#178956,
#178957,#178958,#178959,#178960,#178961,#178962,#178963,#178964,#178965,
#178966,#178967,#178968,#178969,#178970,#178971,#178972,#178973,#178974,
#178975,#178976,#178977,#178978,#178979,#178980,#178981,#178982,#178983,
#178984,#178985,#178986,#178987,#178988,#178989,#178990,#178991,#178992,
#178993,#178994,#178995,#178996,#178997,#178998,#178999,#179000,#179001,
#179002,#179003,#179004,#179005,#179006,#179007,#179008,#179009,#179010,
#179011,#179012,#179013,#179014,#179015,#179016,#179017,#179018,#179019,
#179020,#179021,#179022,#179023,#179024,#179025,#179026,#179027,#179028,
#179029,#179030,#179031,#179032,#179033,#179034,#179035,#179036,#179037,
#179038,#179039,#179040,#179041,#179042,#179043,#179044,#179045,#179046,
#179047,#179048,#179049,#179050,#179051,#179052,#179053,#179054,#179055,
#179056,#179057,#179058,#179059,#179060,#179061,#179062,#179063,#179064,
#179065,#179066,#179067,#179068,#179069,#179070,#179071,#179072,#179073,
#179074,#179075,#179076,#179077,#179078,#179079,#179080,#179081,#179082,
#179083,#179084,#179085,#179086,#179087,#179088,#179089,#179090,#179091,
#179092,#179093,#179094,#179095,#179096,#179097,#179098,#179099,#179100,
#179101,#179102,#179103,#179104,#179105,#179106,#179107,#179108,#179109,
#179110,#179111,#179112,#179113,#179114,#179115,#179116,#179117,#179118,
#179119,#179120,#179121,#179122,#179123,#179124,#179125,#179126,#179127,
#179128,#179129,#179130,#179131,#179132,#179133,#179134,#179135),
 .UNSPECIFIED.,.F.,.F.,(4,3,3,3,3,3,3,3,3,3,3,3,3,3,3,3,3,3,3,3,3,3,3,3,
3,3,3,3,3,3,3,3,3,3,3,3,3,3,3,3,3,3,3,3,3,3,3,3,3,3,3,3,3,3,3,3,3,3,3,3,
3,3,3,3,3,3,3,3,3,3,3,3,3,3,3,3,3,3,3,3,3,3,3,3,3,4),(103.672557568464,
103.760974723913,103.851528885978,103.940713177353,104.031952274763,104.123191372174,
104.196160816624,104.269084807718,104.341976334459,104.41485853338,104.487733451423,
104.560636401133,104.621659915481,104.70096069943,104.780283629907,104.859626231917,
104.93899930909,105.018380990087,105.097777767196,105.120128458789,105.199525853458,
105.278909527286,105.358276978927,105.437622162739,105.516945182005,105.596239411627,
105.618597002097,105.691499402366,105.764379259411,105.837249528844,105.91014587325,
105.983054529035,106.056022841983,106.117065545404,106.205639877016,106.294340242489,
106.382907054591,106.471250468154,106.559020184779,106.615534088712,106.686857587062,
106.758161337217,106.82945884049,106.900791336136,106.972139694875,107.043560349842,
107.114002632019,107.19010612804,107.266159274111,107.342172464346,107.418156064227,
107.494120417555,107.57122283019,107.647194558229,107.723178885488,107.79918522716,
107.877123850028,107.953232889457,108.032086304045,108.110939718634,108.187072590879,
108.26311229195,108.339068297321,108.414926739859,108.490727803412,108.566467124146,
108.609408261942,108.685150626765,108.760938747515,108.836781918357,108.912736876617,
108.988753308951,109.064889104452,109.107876805249,109.182804990125,109.257662582641,
109.332462245684,109.410372324429,109.485093837599,109.559799282389,109.634500050476,
109.709207529054,109.783955887192,109.858728142048,109.933559479095,109.955742875643),
 .UNSPECIFIED.);
#3250=B_SPLINE_CURVE_WITH_KNOTS('',3,(#179137,#179138,#179139,#179140,#179141,
#179142,#179143,#179144,#179145,#179146,#179147,#179148,#179149,#179150,
#179151,#179152,#179153,#179154),.UNSPECIFIED.,.F.,.F.,(4,2,2,2,2,2,2,2,
4),(97.3893722612842,98.2187300377222,99.0480878141601,99.877445590598,
100.706803367036,101.536161143474,102.365518919912,103.19487669635,103.672557568464),
 .UNSPECIFIED.);
#3251=B_SPLINE_CURVE_WITH_KNOTS('',3,(#179156,#179157,#179158,#179159,#179160,
#179161,#179162,#179163,#179164,#179165,#179166,#179167,#179168,#179169,
#179170),.UNSPECIFIED.,.F.,.F.,(4,1,1,1,1,1,1,1,1,1,1,1,4),(91.106186982299,
91.1630092461774,91.661477789485,92.1599463327925,92.6584148761001,93.1568834194076,
94.1538205060227,94.6522890493303,95.1507575926379,96.147694679253,96.6461632225605,
97.1446317658681,97.3893722612842),.UNSPECIFIED.);
#3252=B_SPLINE_CURVE_WITH_KNOTS('',3,(#179172,#179173,#179174,#179175,#179176,
#179177,#179178,#179179,#179180,#179181,#179182,#179183,#179184,#179185,
#179186,#179187,#179188,#179189,#179190,#179191,#179192,#179193,#179194,
#179195,#179196,#179197,#179198,#179199,#179200,#179201,#179202,#179203,
#179204,#179205,#179206,#179207,#179208,#179209,#179210,#179211,#179212,
#179213,#179214,#179215,#179216,#179217,#179218,#179219,#179220,#179221,
#179222,#179223,#179224,#179225,#179226,#179227,#179228,#179229,#179230,
#179231,#179232,#179233,#179234,#179235,#179236,#179237,#179238,#179239,
#179240,#179241,#179242,#179243,#179244,#179245,#179246,#179247,#179248,
#179249,#179250,#179251,#179252,#179253,#179254,#179255,#179256,#179257,
#179258,#179259,#179260,#179261,#179262,#179263,#179264,#179265,#179266,
#179267,#179268,#179269,#179270,#179271,#179272,#179273,#179274,#179275,
#179276,#179277,#179278,#179279,#179280,#179281,#179282,#179283,#179284,
#179285,#179286,#179287,#179288,#179289,#179290,#179291,#179292,#179293,
#179294,#179295,#179296,#179297,#179298,#179299,#179300,#179301,#179302,
#179303,#179304,#179305,#179306,#179307,#179308,#179309,#179310,#179311,
#179312,#179313,#179314,#179315,#179316,#179317,#179318,#179319,#179320,
#179321,#179322,#179323,#179324,#179325,#179326,#179327,#179328,#179329,
#179330,#179331,#179332,#179333,#179334,#179335,#179336,#179337,#179338,
#179339,#179340,#179341,#179342,#179343,#179344,#179345,#179346,#179347,
#179348,#179349,#179350,#179351,#179352,#179353,#179354,#179355,#179356,
#179357,#179358,#179359,#179360,#179361,#179362,#179363,#179364,#179365,
#179366,#179367,#179368,#179369,#179370,#179371,#179372,#179373,#179374,
#179375,#179376,#179377,#179378,#179379,#179380,#179381,#179382,#179383,
#179384,#179385,#179386,#179387,#179388,#179389,#179390,#179391,#179392,
#179393,#179394,#179395,#179396,#179397,#179398,#179399,#179400,#179401,
#179402,#179403,#179404,#179405,#179406,#179407,#179408,#179409,#179410,
#179411,#179412,#179413,#179414,#179415,#179416,#179417,#179418,#179419,
#179420,#179421,#179422,#179423,#179424),.UNSPECIFIED.,.F.,.F.,(4,3,3,3,
3,3,3,3,3,3,3,3,3,3,3,3,3,3,3,3,3,3,3,3,3,3,3,3,3,3,3,3,3,3,3,3,3,3,3,3,
3,3,3,3,3,3,3,3,3,3,3,3,3,3,3,3,3,3,3,3,3,3,3,3,3,3,3,3,3,3,3,3,3,3,3,3,
3,3,3,3,3,3,3,3,4),(84.8230016469251,84.8956472635889,84.9683166584872,
85.0409964770063,85.113736009744,85.1813867264867,85.2699610580999,85.3586614235737,
85.4472282356765,85.5355716492405,85.6233413658659,85.6798552697942,85.7511787681441,
85.8224825182994,85.8937800215718,85.9651125172181,86.0364608759574,86.1078815309242,
86.1783238131018,86.2544273091229,86.3304804551935,86.4064936454288,86.4824772453094,
86.5584415986381,86.6355440112729,86.7115157393116,86.7875000665704,86.8635064082429,
86.9414450311114,87.0175540705395,87.0964074851282,87.1752608997169,87.251393771962,
87.3274334730333,87.403389478404,87.4792479209413,87.555048984495,87.630788305229,
87.6737294430245,87.7494718078472,87.8252599285969,87.9011030994388,87.9770580576987,
88.0530744900329,88.1292102855333,88.1721979863321,88.2484085668057,88.3245511710578,
88.4006362573982,88.4766742436705,88.5526755142256,88.6297329590658,88.7056982211906,
88.7816598130553,88.8576271401166,88.9355041233242,89.0115339207569,89.0903344968521,
89.1691350729472,89.2405583477971,89.3119284747104,89.3832590462316,89.4545723837173,
89.5258730705395,89.597198552032,89.6676036162547,89.7553091055951,89.8434854680136,
89.932089878631,90.0207901855136,90.1093864454484,90.1660721595623,90.2390416040124,
90.3119655951063,90.3848571218472,90.4577393207681,90.5306142388117,90.6035171885217,
90.6645407028698,90.7438457847053,90.8231735900791,90.902538090652,90.9819133289185,
91.0613095087734,91.1061869541046),.UNSPECIFIED.);
#3253=B_SPLINE_CURVE_WITH_KNOTS('',3,(#179426,#179427,#179428,#179429,#179430,
#179431,#179432,#179433,#179434,#179435,#179436,#179437,#179438,#179439,
#179440,#179441,#179442,#179443),.UNSPECIFIED.,.F.,.F.,(4,2,2,2,2,2,2,2,
4),(78.5398163397455,79.3691741161834,80.1985318926214,81.0278896690593,
81.8572474454973,82.6866052219353,83.5159629983732,84.3453207748112,84.8230016469251),
 .UNSPECIFIED.);
#3254=B_SPLINE_CURVE_WITH_KNOTS('',3,(#179445,#179446,#179447,#179448,#179449,
#179450,#179451,#179452,#179453,#179454,#179455,#179456,#179457,#179458),
 .UNSPECIFIED.,.F.,.F.,(4,1,1,1,1,1,1,1,1,1,1,4),(72.2566310325659,73.2181416871053,
73.7166102304129,74.2150787737204,75.2120158603355,75.7104844036431,76.2089529469506,
76.7074214902582,77.2058900335658,77.7043585768733,78.2028271201809,78.5398163397455),
 .UNSPECIFIED.);
#3255=B_SPLINE_CURVE_WITH_KNOTS('',3,(#179460,#179461,#179462,#179463,#179464,
#179465,#179466,#179467,#179468,#179469,#179470,#179471,#179472,#179473,
#179474,#179475),.UNSPECIFIED.,.F.,.F.,(4,1,1,1,1,1,1,1,1,1,1,1,1,4),(65.9734457253863,
66.2395820807995,66.738050624107,67.2365191674146,68.2334562540297,68.7319247973373,
69.2303933406448,69.7288618839524,70.22733042726,70.7257989705675,71.2242675138751,
71.7227360571826,72.2212046004902,72.2566310325659),.UNSPECIFIED.);
#3256=B_SPLINE_CURVE_WITH_KNOTS('',3,(#179477,#179478,#179479,#179480,#179481,
#179482,#179483,#179484,#179485,#179486,#179487,#179488,#179489,#179490,
#179491),.UNSPECIFIED.,.F.,.F.,(4,1,1,1,1,1,1,1,1,1,1,1,4),(59.6902604182067,
59.7594910178012,60.2579595611088,61.2548966477239,61.7533651910315,62.251833734339,
62.7503022776466,63.2487708209541,63.7472393642617,64.2457079075693,64.7441764508768,
65.2426449941844,65.9734457253863),.UNSPECIFIED.);
#3257=B_SPLINE_CURVE_WITH_KNOTS('',3,(#179493,#179494,#179495,#179496,#179497,
#179498,#179499,#179500,#179501,#179502,#179503,#179504,#179505,#179506),
 .UNSPECIFIED.,.F.,.F.,(4,1,1,1,1,1,1,1,1,1,1,4),(53.4070751110271,54.2763370414181,
54.7748055847256,55.2732741280332,55.7717426713408,56.2702112146483,56.7686797579559,
57.2671483012634,57.765616844571,58.2640853878786,59.2610224744937,59.6902604182067),
 .UNSPECIFIED.);
#3258=B_SPLINE_CURVE_WITH_KNOTS('',3,(#179508,#179509,#179510,#179511,#179512,
#179513,#179514,#179515,#179516,#179517,#179518,#179519,#179520,#179521,
#179522,#179523),.UNSPECIFIED.,.F.,.F.,(4,1,1,1,1,1,1,1,1,1,1,1,1,4),(47.1238898038475,
47.2977774351123,47.7962459784198,48.2947145217274,48.793183065035,49.2916516083425,
49.7901201516501,50.2885886949576,50.7870572382652,51.2855257815727,52.2824628681879,
52.7809314114954,53.279399954803,53.4070751110271),.UNSPECIFIED.);
#3259=B_SPLINE_CURVE_WITH_KNOTS('',3,(#179525,#179526,#179527,#179528,#179529,
#179530,#179531,#179532,#179533,#179534,#179535,#179536,#179537,#179538,
#179539,#179540,#179541,#179542,#179543,#179544,#179545,#179546,#179547,
#179548,#179549,#179550,#179551,#179552,#179553,#179554,#179555,#179556,
#179557,#179558,#179559,#179560,#179561,#179562,#179563,#179564,#179565,
#179566,#179567,#179568,#179569,#179570,#179571,#179572,#179573,#179574,
#179575,#179576,#179577,#179578,#179579,#179580,#179581,#179582,#179583,
#179584,#179585,#179586,#179587,#179588,#179589,#179590,#179591,#179592,
#179593,#179594,#179595,#179596,#179597,#179598,#179599,#179600,#179601,
#179602,#179603,#179604,#179605,#179606,#179607,#179608,#179609,#179610,
#179611,#179612,#179613,#179614,#179615,#179616,#179617,#179618,#179619,
#179620,#179621,#179622,#179623,#179624,#179625,#179626,#179627,#179628,
#179629,#179630,#179631,#179632,#179633,#179634,#179635,#179636,#179637,
#179638,#179639,#179640,#179641,#179642,#179643,#179644,#179645,#179646,
#179647,#179648,#179649,#179650,#179651,#179652,#179653,#179654,#179655,
#179656,#179657,#179658,#179659,#179660,#179661,#179662,#179663,#179664,
#179665,#179666,#179667,#179668,#179669,#179670,#179671,#179672,#179673,
#179674,#179675,#179676,#179677,#179678,#179679,#179680,#179681,#179682,
#179683,#179684,#179685,#179686,#179687,#179688,#179689,#179690,#179691,
#179692,#179693,#179694,#179695,#179696,#179697,#179698,#179699,#179700,
#179701,#179702,#179703,#179704,#179705,#179706,#179707,#179708,#179709,
#179710,#179711,#179712,#179713,#179714,#179715,#179716,#179717,#179718,
#179719,#179720,#179721,#179722,#179723,#179724,#179725,#179726,#179727,
#179728,#179729,#179730,#179731,#179732,#179733,#179734,#179735,#179736,
#179737,#179738,#179739,#179740,#179741,#179742,#179743,#179744,#179745,
#179746,#179747,#179748,#179749,#179750,#179751,#179752,#179753,#179754,
#179755,#179756,#179757,#179758,#179759,#179760,#179761,#179762,#179763,
#179764,#179765,#179766,#179767,#179768,#179769,#179770,#179771,#179772,
#179773,#179774,#179775,#179776,#179777,#179778,#179779,#179780),
 .UNSPECIFIED.,.F.,.F.,(4,3,3,3,3,3,3,3,3,3,3,3,3,3,3,3,3,3,3,3,3,3,3,3,
3,3,3,3,3,3,3,3,3,3,3,3,3,3,3,3,3,3,3,3,3,3,3,3,3,3,3,3,3,3,3,3,3,3,3,3,
3,3,3,3,3,3,3,3,3,3,3,3,3,3,3,3,3,3,3,3,3,3,3,3,3,4),(40.8407044966679,
40.9287194581187,41.0171879336625,41.1060348097448,41.1949478868379,41.2837202383404,
41.3161549154216,41.3891243598713,41.4620483509647,41.5349398777054,41.6078220766259,
41.680696994669,41.7535999443787,41.8146234587291,41.8939242426787,41.9732471731551,
42.0525897751658,42.1319628523385,42.2113445333359,42.2907413104448,42.3130920020367,
42.3924893967055,42.4718730705334,42.5512405221744,42.6305857059864,42.7099087252525,
42.7892029548742,42.8115605453443,42.884462945613,42.9573428026582,43.0302130720914,
43.1031094164965,43.1760180722814,43.2489863852298,43.3100290886518,43.3986034202646,
43.4873037857379,43.5758705978406,43.6642140114044,43.7519837280299,43.8084976319594,
43.8798211303094,43.9511248804646,44.0224223837369,44.0937548793832,44.1651032381225,
44.2365238930893,44.3069661752669,44.383069671288,44.4591228173586,44.5351360075938,
44.6111196074745,44.6870839608031,44.764186373438,44.8401581014766,44.9161424287355,
44.9921487704079,45.0700873932764,45.1461964327046,45.2250498472933,45.303903261882,
45.3800361341271,45.4560758351984,45.5320318405693,45.6078902831066,45.6836913466604,
45.7594306673943,45.8023718051896,45.8781141700123,45.953902290762,46.0297454616037,
46.1057004198636,46.181716852198,46.2578526476984,46.3008403484972,46.3757317456465,
46.4505523614497,46.5253149096933,46.6001367714626,46.6748213521227,46.7494893194585,
46.8241521107267,46.8990865340069,46.9737930881712,47.0488414460093,47.1238898038475),
 .UNSPECIFIED.);
#3260=B_SPLINE_CURVE_WITH_KNOTS('',3,(#179782,#179783,#179784,#179785,#179786,
#179787,#179788,#179789,#179790,#179791,#179792,#179793,#179794,#179795,
#179796,#179797,#179798,#179799,#179800,#179801,#179802,#179803,#179804,
#179805,#179806,#179807,#179808,#179809,#179810,#179811,#179812,#179813,
#179814,#179815,#179816,#179817,#179818,#179819,#179820,#179821,#179822,
#179823,#179824,#179825,#179826,#179827,#179828,#179829,#179830,#179831,
#179832,#179833,#179834,#179835,#179836,#179837,#179838,#179839,#179840,
#179841,#179842,#179843,#179844,#179845,#179846,#179847,#179848,#179849,
#179850,#179851,#179852,#179853,#179854,#179855,#179856,#179857,#179858,
#179859,#179860,#179861,#179862,#179863,#179864,#179865,#179866,#179867,
#179868,#179869,#179870,#179871,#179872,#179873,#179874,#179875,#179876,
#179877,#179878,#179879,#179880,#179881,#179882,#179883,#179884,#179885,
#179886,#179887,#179888,#179889,#179890,#179891,#179892,#179893,#179894,
#179895,#179896,#179897,#179898,#179899,#179900,#179901,#179902,#179903,
#179904,#179905,#179906,#179907,#179908,#179909,#179910,#179911,#179912,
#179913,#179914,#179915,#179916,#179917,#179918,#179919,#179920,#179921,
#179922,#179923,#179924,#179925,#179926,#179927,#179928,#179929,#179930,
#179931,#179932,#179933,#179934,#179935,#179936,#179937,#179938,#179939,
#179940,#179941,#179942,#179943,#179944,#179945,#179946,#179947,#179948,
#179949,#179950,#179951,#179952,#179953,#179954,#179955,#179956,#179957,
#179958,#179959,#179960,#179961,#179962,#179963,#179964,#179965,#179966,
#179967,#179968,#179969,#179970,#179971,#179972,#179973,#179974,#179975,
#179976,#179977,#179978,#179979,#179980,#179981,#179982,#179983,#179984,
#179985,#179986,#179987,#179988,#179989,#179990,#179991,#179992,#179993,
#179994,#179995,#179996,#179997,#179998,#179999,#180000,#180001,#180002,
#180003,#180004,#180005,#180006,#180007,#180008,#180009,#180010,#180011,
#180012,#180013,#180014,#180015,#180016,#180017,#180018,#180019,#180020,
#180021,#180022,#180023,#180024,#180025,#180026,#180027,#180028,#180029,
#180030,#180031,#180032,#180033,#180034,#180035,#180036,#180037,#180038,
#180039,#180040,#180041,#180042,#180043,#180044,#180045,#180046,#180047,
#180048,#180049,#180050,#180051,#180052,#180053,#180054,#180055,#180056,
#180057,#180058,#180059,#180060,#180061,#180062,#180063,#180064,#180065,
#180066,#180067,#180068,#180069,#180070,#180071,#180072,#180073,#180074,
#180075,#180076,#180077,#180078,#180079,#180080,#180081,#180082,#180083,
#180084,#180085,#180086,#180087,#180088,#180089,#180090,#180091,#180092,
#180093,#180094,#180095,#180096,#180097,#180098,#180099,#180100,#180101,
#180102,#180103,#180104,#180105,#180106,#180107,#180108,#180109,#180110,
#180111,#180112,#180113,#180114,#180115,#180116,#180117,#180118,#180119,
#180120,#180121,#180122,#180123,#180124,#180125,#180126,#180127,#180128,
#180129,#180130,#180131,#180132,#180133,#180134,#180135,#180136,#180137,
#180138,#180139,#180140,#180141,#180142,#180143,#180144,#180145,#180146,
#180147,#180148,#180149,#180150,#180151,#180152,#180153,#180154,#180155,
#180156,#180157,#180158,#180159,#180160,#180161,#180162,#180163,#180164,
#180165,#180166,#180167,#180168,#180169,#180170,#180171,#180172,#180173,
#180174,#180175,#180176,#180177,#180178,#180179,#180180,#180181,#180182,
#180183,#180184,#180185,#180186,#180187,#180188,#180189,#180190,#180191,
#180192,#180193,#180194,#180195,#180196,#180197,#180198,#180199,#180200,
#180201,#180202,#180203,#180204,#180205,#180206,#180207,#180208,#180209,
#180210,#180211,#180212,#180213,#180214,#180215,#180216,#180217,#180218,
#180219,#180220,#180221,#180222,#180223,#180224,#180225,#180226,#180227,
#180228,#180229,#180230,#180231,#180232,#180233,#180234,#180235,#180236,
#180237,#180238,#180239,#180240,#180241,#180242,#180243,#180244,#180245,
#180246,#180247,#180248,#180249,#180250,#180251,#180252,#180253,#180254,
#180255,#180256,#180257,#180258,#180259,#180260,#180261,#180262,#180263,
#180264,#180265,#180266,#180267,#180268,#180269,#180270,#180271,#180272,
#180273,#180274,#180275,#180276,#180277,#180278,#180279,#180280,#180281,
#180282,#180283,#180284,#180285,#180286,#180287,#180288,#180289,#180290,
#180291,#180292,#180293,#180294,#180295,#180296,#180297,#180298,#180299,
#180300,#180301,#180302,#180303,#180304,#180305,#180306,#180307,#180308,
#180309,#180310,#180311,#180312,#180313,#180314,#180315,#180316,#180317,
#180318,#180319),.UNSPECIFIED.,.F.,.F.,(4,2,2,2,2,2,2,2,2,2,2,2,2,2,2,2,
2,2,2,2,2,2,2,2,2,2,2,2,2,2,2,2,2,2,2,2,2,2,2,2,2,2,2,2,2,2,2,2,2,2,2,2,
2,2,2,2,2,2,2,2,2,2,2,2,2,2,2,2,2,2,2,2,2,2,2,2,2,2,2,2,2,2,2,2,2,2,2,2,
2,2,2,2,2,2,2,2,2,2,2,2,2,2,2,2,2,2,2,2,2,2,2,2,2,2,2,2,2,2,2,2,2,2,2,2,
2,2,2,2,2,2,2,2,2,2,2,2,2,2,2,2,2,2,2,2,2,2,2,2,2,2,2,2,2,2,2,2,2,2,2,2,
2,2,2,2,2,2,2,2,2,2,2,2,2,2,2,2,2,2,2,2,2,2,2,2,2,2,2,2,2,2,2,2,2,2,2,2,
2,2,2,2,2,2,2,2,2,2,2,2,2,2,2,2,2,2,2,2,2,2,2,2,2,2,2,2,2,2,2,2,2,2,2,2,
2,2,2,2,2,2,2,2,2,2,2,2,2,2,2,2,2,2,2,2,2,2,2,2,2,2,2,2,2,2,2,2,2,2,2,2,
4),(0.00125752731703474,0.0770073154476629,0.2473678712053,0.359216152094507,
0.396265044239058,0.401520059173252,0.404202671083985,0.40633662724841,
0.40846151340549,0.412243402032006,0.423499164554404,0.602221708117882,
0.659613308106922,0.678019555852865,0.824234587801754,0.832645120334795,
0.836508081954302,0.839424590093864,0.842170989525301,0.846734519621614,
0.858458669930312,1.0574495708609,1.19049216789867,1.22517431510643,1.25212306331559,
1.25709375790634,1.25978895949415,1.26201454534388,1.26464883530674,1.2692165403338,
1.28692165845471,1.3320047190122,1.57970137127534,1.60706411844689,1.621101524216,
1.62985766206543,1.63798949437402,1.6444108018159,1.65057324303309,1.66045160573835,
1.68461343508822,1.9097790368194,1.9717667989585,2.01504389710494,2.02067686614194,
2.02351104993524,2.02555350002419,2.0277199385567,2.03077249380004,2.03891591081125,
2.16432114872236,2.30947209752093,2.43049437670148,2.44016938379904,2.4442604069529,
2.44721651275976,2.44990808177577,2.45350318561752,2.46226321896282,2.54636941134557,
2.57278292334523,2.70862982716858,2.80635390048645,2.84736612524927,2.8662928686644,
2.87473060032628,2.87798378089784,2.88023112023578,2.88243814596076,2.88510631155454,
2.89180983983446,2.97658473540921,3.10732956764125,3.2864238980362,3.32038130446213,
3.33537788547056,3.34674924321235,3.35913147235969,3.37931839964686,3.44972880413065,
3.45736116975926,3.6060804967098,3.64022881803426,3.65078217030559,3.66497474572718,
3.67165734304444,3.6772198761296,3.68421346999125,3.6953844345894,3.76147536757163,
3.81395235498242,3.84713795423668,3.86120358132372,3.871831864406,3.88346158649701,
3.90282107936014,4.00545389148317,4.06020985544135,4.07329957436829,4.07988492004892,
4.08586441651803,4.0936759947102,4.10707119856584,4.1687391476082,4.17010235673242,
4.19321050138007,4.26446602536726,4.28658885519433,4.31876022490759,4.33694782439542,
4.35360098806555,4.37752879739541,4.43731636404158,4.46983736229162,4.48278848797526,
4.49455750606592,4.52136498319555,4.57317616923912,4.59619998024701,4.61618720411073,
4.63258225492629,4.6530743427674,4.69559315704525,4.73557735688723,4.82700483158738,
4.84636140789915,4.86865313957536,4.87729501266872,4.88339485579818,4.8889067259845,
4.8990671487418,4.95161815332911,5.02710307701641,5.05583577825819,5.07829332758265,
5.09054902454767,5.10107347109147,5.11409344527995,5.14076609356116,5.1780545075291,
5.22153728595093,5.2724906679816,5.28277547964281,5.28834455049688,5.29335349931155,
5.30053851711047,5.31758695377241,5.34213411718773,5.4619890317345,5.58092706752411,
5.60293409166045,5.61583011758335,5.62709936589149,5.64117857020607,5.66988189226538,
5.78953534958973,5.95944705606483,6.05438733500089,6.07541254432156,6.07970988967138,
6.08244235744867,6.08460127660217,6.08701292940233,6.09101634202681,6.1056226459851,
6.21888960861495,6.42711593918513,6.50235988325432,6.51099187121482,6.51485406205035,
6.51778164529541,6.52088136303134,6.5256655856898,6.54002028993751,6.61812562599479,
6.73212454043503,6.86014688614911,6.9281568542819,6.93388575899285,6.93679019599724,
6.93891725431871,6.94120793924899,6.94429625266686,6.95124710861183,6.96066391199125,
7.06419576110389,7.14517730308026,7.29115987226083,7.30750948719825,7.31584271110859,
7.32243169581325,7.32944239977542,7.34009436004049,7.37189978384187,7.61804813286514,
7.67657730672564,7.69462222939699,7.69886979261845,7.7016513016184,7.7039023121736,
7.70647454335507,7.71088503758533,7.71611488781535,7.83936747883278,7.95529740506117,
8.10824053927392,8.11793614343996,8.12172575261313,8.12446704921031,8.12738725152405,
8.13127063177518,8.1397875047071,8.311275372298,8.42328494910654,8.54474739630907,
8.5528327931149,8.55579824978388,8.55788234428144,8.55983073363021,8.56250871438552,
8.5677402442379,8.60406009269718,8.70936993451049,8.9427573652302,8.99242929539948,
9.01005736126804,9.02071721814504,9.03141607675681,9.04558410355352,9.07388479213853,
9.11297774009509,9.21915080595416,9.32533433501506,9.34155791825231,9.34816423732876,
9.3537464576593,9.35905271635354,9.36675785568267,9.37706681138417,9.39742373908967,
9.46413102200946,9.51940157069119,9.53570044500064,9.54660471173925,9.55648523811236,
9.5670474691921,9.59430454729861,9.61475521428189,9.71001743759616,9.74473307909,
9.75416585364841,9.75959028267143,9.7652275119229,9.77141812278283,9.78000351965131,
9.7947341927376,9.82815473955098,9.90626691052985,9.98075854684207,10.0046799645723,
10.0212609973963,10.0359669130552,10.0641470934526,10.1058036993865,10.1445205585375,
10.1587841267585,10.1697904557197,10.1851584547576,10.2266614198589),
 .UNSPECIFIED.);
#3261=B_SPLINE_CURVE_WITH_KNOTS('',3,(#180321,#180322,#180323,#180324,#180325,
#180326,#180327,#180328,#180329,#180330,#180331,#180332,#180333,#180334),
 .UNSPECIFIED.,.F.,.F.,(4,1,1,1,1,1,1,1,1,1,1,4),(21.991148636497,22.3743502697344,
22.8728188130419,23.3712873563495,24.3682244429646,24.8666929862722,25.3651615295797,
26.3620986161948,26.8605671595024,27.35903570281,27.8575042461175,28.2743171305593),
 .UNSPECIFIED.);
#3262=B_SPLINE_CURVE_WITH_KNOTS('',3,(#180335,#180336,#180337,#180338,#180339,
#180340,#180341,#180342,#180343,#180344,#180345,#180346,#180347,#180348,
#180349,#180350,#180351,#180352),.UNSPECIFIED.,.F.,.F.,(4,2,2,2,2,2,2,2,
4),(15.7079632679496,16.5373210443875,17.3666788208254,18.1960365972634,
19.0253943737013,19.8547521501392,20.6841099265772,21.5134677030151,21.9911411882542),
 .UNSPECIFIED.);
#3263=B_SPLINE_CURVE_WITH_KNOTS('',3,(#180386,#180387,#180388,#180389,#180390,
#180391,#180392,#180393,#180394,#180395,#180396,#180397,#180398,#180399,
#180400,#180401,#180402,#180403,#180404,#180405,#180406,#180407,#180408,
#180409,#180410,#180411,#180412,#180413,#180414,#180415,#180416,#180417,
#180418,#180419,#180420,#180421,#180422,#180423,#180424,#180425,#180426,
#180427,#180428,#180429,#180430,#180431,#180432,#180433,#180434,#180435,
#180436,#180437,#180438,#180439,#180440,#180441,#180442,#180443,#180444,
#180445,#180446,#180447,#180448,#180449,#180450,#180451,#180452,#180453,
#180454,#180455,#180456,#180457,#180458,#180459,#180460,#180461,#180462,
#180463,#180464,#180465,#180466,#180467,#180468,#180469,#180470,#180471,
#180472,#180473,#180474,#180475,#180476,#180477,#180478,#180479,#180480,
#180481,#180482,#180483,#180484,#180485,#180486,#180487,#180488,#180489,
#180490,#180491),.UNSPECIFIED.,.F.,.F.,(4,3,3,3,3,3,3,3,3,3,3,3,3,3,3,3,
3,3,3,3,3,3,3,3,3,3,3,3,3,3,3,3,3,3,3,4),(-1.53973642054047,-1.48309553350524,
-1.42555125559393,-1.37417990184393,-1.36553101890543,-1.30722914366635,
-1.24872710196501,-1.21482678019219,-1.20381532475203,-1.19606511894002,
-1.18103104109073,-1.12346211407032,-1.06450347487904,-1.00508210571978,
-0.945643635900972,-0.91883932096823,-0.908401830512179,-0.847848726025719,
-0.808078428123881,-0.747890453958617,-0.687155807913238,-0.626486811594127,
-0.618542269912916,-0.612188487123754,-0.550651591095428,-0.486102847768932,
-0.421554104442437,-0.359682371036917,-0.317439297897168,-0.306618832338073,
-0.244672610384753,-0.181521847273755,-0.118198336282773,-0.0554614676464781,
-0.0217377859189241,-0.0002294502900981),.UNSPECIFIED.);
#3264=B_SPLINE_CURVE_WITH_KNOTS('',3,(#180492,#180493,#180494,#180495,#180496,
#180497,#180498,#180499,#180500,#180501,#180502,#180503,#180504,#180505,
#180506,#180507,#180508,#180509,#180510,#180511,#180512,#180513,#180514,
#180515,#180516,#180517,#180518,#180519,#180520,#180521,#180522,#180523,
#180524,#180525,#180526,#180527,#180528,#180529,#180530,#180531,#180532,
#180533,#180534,#180535,#180536,#180537,#180538,#180539,#180540,#180541,
#180542,#180543,#180544,#180545,#180546,#180547,#180548,#180549,#180550,
#180551,#180552,#180553,#180554,#180555,#180556,#180557,#180558,#180559,
#180560,#180561,#180562,#180563,#180564,#180565,#180566,#180567,#180568,
#180569,#180570,#180571,#180572,#180573,#180574,#180575,#180576,#180577,
#180578,#180579,#180580,#180581,#180582,#180583,#180584,#180585,#180586,
#180587,#180588,#180589,#180590,#180591,#180592,#180593,#180594,#180595,
#180596,#180597,#180598,#180599,#180600,#180601,#180602,#180603,#180604,
#180605,#180606,#180607,#180608,#180609,#180610,#180611,#180612),
 .UNSPECIFIED.,.F.,.F.,(4,3,3,3,3,3,3,3,3,3,3,3,3,3,3,3,3,3,3,3,3,3,3,3,
3,3,3,3,3,3,3,3,3,3,3,3,3,3,3,3,4),(-1.53496049794141,-1.47178129893344,
-1.40843691381202,-1.37435034446066,-1.3580964238932,-1.34490295184081,
-1.33579830849837,-1.27329007086333,-1.21151125381654,-1.17388303799248,
-1.16095961939653,-1.15226699516528,-1.13641946967192,-1.07545420701605,
-1.01382479674967,-0.95236079989948,-0.891797849505327,-0.863940613600807,
-0.856360761628214,-0.849031173886624,-0.788858717844872,-0.750528920592363,
-0.690182939490677,-0.630180622346739,-0.570395005112455,-0.562781680266923,
-0.555685406180827,-0.496667854192665,-0.437284384333118,-0.377900914473571,
-0.325131736658691,-0.298747147751252,-0.285554853297532,-0.276802264147644,
-0.272362558843812,-0.214747246406761,-0.157173822782883,-0.100144168788378,
-0.0443751750866251,-0.0188072533466611,0.),.UNSPECIFIED.);
#3265=B_SPLINE_CURVE_WITH_KNOTS('',3,(#182765,#182766,#182767,#182768,#182769,
#182770,#182771,#182772,#182773,#182774,#182775,#182776,#182777,#182778,
#182779,#182780,#182781,#182782,#182783,#182784,#182785,#182786,#182787,
#182788,#182789,#182790,#182791,#182792,#182793,#182794,#182795,#182796,
#182797,#182798,#182799,#182800,#182801,#182802,#182803,#182804,#182805,
#182806,#182807,#182808,#182809,#182810,#182811,#182812,#182813,#182814,
#182815,#182816,#182817,#182818,#182819,#182820,#182821,#182822,#182823,
#182824,#182825,#182826,#182827,#182828,#182829,#182830,#182831,#182832,
#182833,#182834,#182835,#182836,#182837,#182838,#182839,#182840,#182841,
#182842,#182843,#182844,#182845,#182846,#182847,#182848,#182849,#182850,
#182851,#182852,#182853,#182854,#182855,#182856,#182857,#182858,#182859,
#182860,#182861,#182862,#182863,#182864,#182865,#182866,#182867,#182868,
#182869,#182870,#182871,#182872,#182873,#182874,#182875,#182876),
 .UNSPECIFIED.,.F.,.F.,(4,3,3,3,3,3,3,3,3,3,3,3,3,3,3,3,3,3,3,3,3,3,3,3,
3,3,3,3,3,3,3,3,3,3,3,3,3,4),(0.,0.0561488103666945,0.113191923654328,0.170826554765673,
0.228516319046485,0.260964459841906,0.274244127071257,0.283126614449263,
0.341981702386085,0.358308882228168,0.416517661403603,0.475296887246886,
0.534320856699363,0.562024956257231,0.56908591189923,0.628813329120672,
0.689174298961302,0.730209481738314,0.790378517014038,0.849791355046748,
0.85680142973422,0.917257569468678,0.978700057224852,1.04030706425093,1.10152839748546,
1.11544043113767,1.14030590548036,1.15393052993428,1.16506174221691,1.22673611738623,
1.28912202595642,1.32139879568865,1.33812146091464,1.35285285612202,1.41610495574213,
1.4793560028455,1.51328802062074,1.53473167268384),.UNSPECIFIED.);
#3266=B_SPLINE_CURVE_WITH_KNOTS('',3,(#185029,#185030,#185031,#185032,#185033,
#185034,#185035,#185036,#185037,#185038,#185039,#185040,#185041,#185042,
#185043,#185044,#185045,#185046,#185047,#185048,#185049,#185050,#185051,
#185052,#185053,#185054,#185055,#185056,#185057,#185058,#185059,#185060,
#185061,#185062,#185063,#185064,#185065,#185066,#185067,#185068,#185069,
#185070,#185071,#185072,#185073,#185074,#185075,#185076,#185077,#185078,
#185079,#185080,#185081,#185082,#185083,#185084,#185085,#185086,#185087,
#185088,#185089,#185090,#185091,#185092,#185093,#185094,#185095,#185096,
#185097,#185098,#185099,#185100,#185101,#185102,#185103,#185104,#185105,
#185106,#185107,#185108,#185109,#185110,#185111,#185112,#185113,#185114,
#185115,#185116,#185117,#185118,#185119,#185120,#185121,#185122,#185123,
#185124,#185125,#185126,#185127,#185128,#185129,#185130,#185131,#185132,
#185133,#185134,#185135,#185136,#185137),.UNSPECIFIED.,.F.,.F.,(4,3,3,3,
3,3,3,3,3,3,3,3,3,3,3,3,3,3,3,3,3,3,3,3,3,3,3,3,3,3,3,3,3,3,3,3,4),(1.15016411802618E-14,
0.0626309539614373,0.126866904460898,0.190025003289835,0.254799879624557,
0.287187317791918,0.303381036875598,0.311555684298871,0.319574755959279,
0.381410337605684,0.400458029617128,0.462480297335892,0.524510838006131,
0.586011000797039,0.61188656071836,0.622914402619484,0.683664933035846,
0.744030234243724,0.787695734468564,0.850206746232349,0.912717757996134,
0.924462553129624,0.983970936762615,1.04337412846815,1.10239878786916,1.16142344727016,
1.1874531784305,1.20024516939136,1.21053455692135,1.2690351269772,1.32713644117412,
1.3696612965529,1.37838125041023,1.43578931046434,1.49222119376588,1.52088321921702,
1.53973642054052),.UNSPECIFIED.);
#4264=LINE('',#136543,#4901);
#4265=LINE('',#136687,#4902);
#4266=LINE('',#136902,#4903);
#4267=LINE('',#137410,#4904);
#4268=LINE('',#137921,#4905);
#4269=LINE('',#138414,#4906);
#4270=LINE('',#138922,#4907);
#4271=LINE('',#139433,#4908);
#4272=LINE('',#139941,#4909);
#4273=LINE('',#140452,#4910);
#4274=LINE('',#140960,#4911);
#4275=LINE('',#141474,#4912);
#4276=LINE('',#141967,#4913);
#4277=LINE('',#142475,#4914);
#4278=LINE('',#142983,#4915);
#4279=LINE('',#143479,#4916);
#4280=LINE('',#143993,#4917);
#4281=LINE('',#144501,#4918);
#4282=LINE('',#145015,#4919);
#4283=LINE('',#145526,#4920);
#4284=LINE('',#146034,#4921);
#4285=LINE('',#146548,#4922);
#4286=LINE('',#147038,#4923);
#4287=LINE('',#147549,#4924);
#4288=LINE('',#148060,#4925);
#4289=LINE('',#148550,#4926);
#4290=LINE('',#149049,#4927);
#4291=LINE('',#149566,#4928);
#4292=LINE('',#150059,#4929);
#4293=LINE('',#150573,#4930);
#4294=LINE('',#151084,#4931);
#4295=LINE('',#151583,#4932);
#4296=LINE('',#152088,#4933);
#4297=LINE('',#152596,#4934);
#4298=LINE('',#153110,#4935);
#4299=LINE('',#153624,#4936);
#4300=LINE('',#154138,#4937);
#4301=LINE('',#154640,#4938);
#4302=LINE('',#155133,#4939);
#4303=LINE('',#155644,#4940);
#4304=LINE('',#156155,#4941);
#4305=LINE('',#156648,#4942);
#4306=LINE('',#157153,#4943);
#4307=LINE('',#157667,#4944);
#4308=LINE('',#158181,#4945);
#4309=LINE('',#158692,#4946);
#4310=LINE('',#159203,#4947);
#4311=LINE('',#159711,#4948);
#4312=LINE('',#160204,#4949);
#4313=LINE('',#160712,#4950);
#4314=LINE('',#180360,#4951);
#4315=LINE('',#180365,#4952);
#4316=LINE('',#180367,#4953);
#4317=LINE('',#180369,#4954);
#4318=LINE('',#180370,#4955);
#4319=LINE('',#180374,#4956);
#4320=LINE('',#180375,#4957);
#4321=LINE('',#180376,#4958);
#4322=LINE('',#180380,#4959);
#4323=LINE('',#180381,#4960);
#4324=LINE('',#180382,#4961);
#4325=LINE('',#185142,#4962);
#4901=VECTOR('',#19024,7.01125);
#4902=VECTOR('',#19027,7.01125);
#4903=VECTOR('',#19034,7.01125);
#4904=VECTOR('',#19037,7.01125);
#4905=VECTOR('',#19040,7.01125);
#4906=VECTOR('',#19043,7.01125);
#4907=VECTOR('',#19046,7.01125);
#4908=VECTOR('',#19049,7.01125);
#4909=VECTOR('',#19052,7.01125);
#4910=VECTOR('',#19055,7.01125);
#4911=VECTOR('',#19058,7.01125);
#4912=VECTOR('',#19061,7.01125);
#4913=VECTOR('',#19064,7.01125);
#4914=VECTOR('',#19067,7.01125);
#4915=VECTOR('',#19070,7.01125);
#4916=VECTOR('',#19073,7.01125);
#4917=VECTOR('',#19076,7.01125);
#4918=VECTOR('',#19079,7.01125);
#4919=VECTOR('',#19082,7.01125);
#4920=VECTOR('',#19085,7.01125);
#4921=VECTOR('',#19088,7.01125);
#4922=VECTOR('',#19091,7.01125);
#4923=VECTOR('',#19094,7.01125);
#4924=VECTOR('',#19097,7.01125);
#4925=VECTOR('',#19100,7.01125);
#4926=VECTOR('',#19103,7.01125);
#4927=VECTOR('',#19106,7.01125);
#4928=VECTOR('',#19109,7.01125);
#4929=VECTOR('',#19112,7.01125);
#4930=VECTOR('',#19115,7.01125);
#4931=VECTOR('',#19118,7.01125);
#4932=VECTOR('',#19121,7.01125);
#4933=VECTOR('',#19124,7.01125);
#4934=VECTOR('',#19127,7.01125);
#4935=VECTOR('',#19130,7.01125);
#4936=VECTOR('',#19133,7.01125);
#4937=VECTOR('',#19136,7.01125);
#4938=VECTOR('',#19139,7.01125);
#4939=VECTOR('',#19142,7.01125);
#4940=VECTOR('',#19145,7.01125);
#4941=VECTOR('',#19148,7.01125);
#4942=VECTOR('',#19151,7.01125);
#4943=VECTOR('',#19154,7.01125);
#4944=VECTOR('',#19157,7.01125);
#4945=VECTOR('',#19160,7.01125);
#4946=VECTOR('',#19163,7.01125);
#4947=VECTOR('',#19166,7.01125);
#4948=VECTOR('',#19169,7.01125);
#4949=VECTOR('',#19172,7.01125);
#4950=VECTOR('',#19175,7.01125);
#4951=VECTOR('',#19194,8.5);
#4952=VECTOR('',#19199,10.);
#4953=VECTOR('',#19200,10.);
#4954=VECTOR('',#19201,10.);
#4955=VECTOR('',#19202,10.);
#4956=VECTOR('',#19205,10.);
#4957=VECTOR('',#19206,10.);
#4958=VECTOR('',#19207,10.);
#4959=VECTOR('',#19210,10.);
#4960=VECTOR('',#19211,10.);
#4961=VECTOR('',#19212,10.);
#4962=VECTOR('',#19225,4.);
#6275=VERTEX_POINT('',#136541);
#6276=VERTEX_POINT('',#136542);
#6277=VERTEX_POINT('',#136544);
#6278=VERTEX_POINT('',#136684);
#6279=VERTEX_POINT('',#136686);
#6280=VERTEX_POINT('',#136689);
#6281=VERTEX_POINT('',#136900);
#6282=VERTEX_POINT('',#136901);
#6283=VERTEX_POINT('',#136903);
#6284=VERTEX_POINT('',#137152);
#6285=VERTEX_POINT('',#137408);
#6286=VERTEX_POINT('',#137409);
#6287=VERTEX_POINT('',#137411);
#6288=VERTEX_POINT('',#137666);
#6289=VERTEX_POINT('',#137919);
#6290=VERTEX_POINT('',#137920);
#6291=VERTEX_POINT('',#137922);
#6292=VERTEX_POINT('',#138174);
#6293=VERTEX_POINT('',#138412);
#6294=VERTEX_POINT('',#138413);
#6295=VERTEX_POINT('',#138415);
#6296=VERTEX_POINT('',#138667);
#6297=VERTEX_POINT('',#138920);
#6298=VERTEX_POINT('',#138921);
#6299=VERTEX_POINT('',#138923);
#6300=VERTEX_POINT('',#139178);
#6301=VERTEX_POINT('',#139431);
#6302=VERTEX_POINT('',#139432);
#6303=VERTEX_POINT('',#139434);
#6304=VERTEX_POINT('',#139692);
#6305=VERTEX_POINT('',#139939);
#6306=VERTEX_POINT('',#139940);
#6307=VERTEX_POINT('',#139942);
#6308=VERTEX_POINT('',#140197);
#6309=VERTEX_POINT('',#140450);
#6310=VERTEX_POINT('',#140451);
#6311=VERTEX_POINT('',#140453);
#6312=VERTEX_POINT('',#140705);
#6313=VERTEX_POINT('',#140958);
#6314=VERTEX_POINT('',#140959);
#6315=VERTEX_POINT('',#140961);
#6316=VERTEX_POINT('',#141213);
#6317=VERTEX_POINT('',#141472);
#6318=VERTEX_POINT('',#141473);
#6319=VERTEX_POINT('',#141475);
#6320=VERTEX_POINT('',#141727);
#6321=VERTEX_POINT('',#141965);
#6322=VERTEX_POINT('',#141966);
#6323=VERTEX_POINT('',#141968);
#6324=VERTEX_POINT('',#142217);
#6325=VERTEX_POINT('',#142473);
#6326=VERTEX_POINT('',#142474);
#6327=VERTEX_POINT('',#142476);
#6328=VERTEX_POINT('',#142725);
#6329=VERTEX_POINT('',#142981);
#6330=VERTEX_POINT('',#142982);
#6331=VERTEX_POINT('',#142984);
#6332=VERTEX_POINT('',#143236);
#6333=VERTEX_POINT('',#143477);
#6334=VERTEX_POINT('',#143478);
#6335=VERTEX_POINT('',#143480);
#6336=VERTEX_POINT('',#143738);
#6337=VERTEX_POINT('',#143991);
#6338=VERTEX_POINT('',#143992);
#6339=VERTEX_POINT('',#143994);
#6340=VERTEX_POINT('',#144249);
#6341=VERTEX_POINT('',#144499);
#6342=VERTEX_POINT('',#144500);
#6343=VERTEX_POINT('',#144502);
#6344=VERTEX_POINT('',#144760);
#6345=VERTEX_POINT('',#145013);
#6346=VERTEX_POINT('',#145014);
#6347=VERTEX_POINT('',#145016);
#6348=VERTEX_POINT('',#145271);
#6349=VERTEX_POINT('',#145524);
#6350=VERTEX_POINT('',#145525);
#6351=VERTEX_POINT('',#145527);
#6352=VERTEX_POINT('',#145779);
#6353=VERTEX_POINT('',#146032);
#6354=VERTEX_POINT('',#146033);
#6355=VERTEX_POINT('',#146035);
#6356=VERTEX_POINT('',#146290);
#6357=VERTEX_POINT('',#146546);
#6358=VERTEX_POINT('',#146547);
#6359=VERTEX_POINT('',#146549);
#6360=VERTEX_POINT('',#146801);
#6361=VERTEX_POINT('',#147036);
#6362=VERTEX_POINT('',#147037);
#6363=VERTEX_POINT('',#147039);
#6364=VERTEX_POINT('',#147288);
#6365=VERTEX_POINT('',#147547);
#6366=VERTEX_POINT('',#147548);
#6367=VERTEX_POINT('',#147550);
#6368=VERTEX_POINT('',#147802);
#6369=VERTEX_POINT('',#148058);
#6370=VERTEX_POINT('',#148059);
#6371=VERTEX_POINT('',#148061);
#6372=VERTEX_POINT('',#148310);
#6373=VERTEX_POINT('',#148548);
#6374=VERTEX_POINT('',#148549);
#6375=VERTEX_POINT('',#148551);
#6376=VERTEX_POINT('',#148791);
#6377=VERTEX_POINT('',#149047);
#6378=VERTEX_POINT('',#149048);
#6379=VERTEX_POINT('',#149050);
#6380=VERTEX_POINT('',#149308);
#6381=VERTEX_POINT('',#149564);
#6382=VERTEX_POINT('',#149565);
#6383=VERTEX_POINT('',#149567);
#6384=VERTEX_POINT('',#149801);
#6385=VERTEX_POINT('',#150057);
#6386=VERTEX_POINT('',#150058);
#6387=VERTEX_POINT('',#150060);
#6388=VERTEX_POINT('',#150318);
#6389=VERTEX_POINT('',#150571);
#6390=VERTEX_POINT('',#150572);
#6391=VERTEX_POINT('',#150574);
#6392=VERTEX_POINT('',#150829);
#6393=VERTEX_POINT('',#151082);
#6394=VERTEX_POINT('',#151083);
#6395=VERTEX_POINT('',#151085);
#6396=VERTEX_POINT('',#151325);
#6397=VERTEX_POINT('',#151581);
#6398=VERTEX_POINT('',#151582);
#6399=VERTEX_POINT('',#151584);
#6400=VERTEX_POINT('',#151836);
#6401=VERTEX_POINT('',#152086);
#6402=VERTEX_POINT('',#152087);
#6403=VERTEX_POINT('',#152089);
#6404=VERTEX_POINT('',#152341);
#6405=VERTEX_POINT('',#152594);
#6406=VERTEX_POINT('',#152595);
#6407=VERTEX_POINT('',#152597);
#6408=VERTEX_POINT('',#152849);
#6409=VERTEX_POINT('',#153108);
#6410=VERTEX_POINT('',#153109);
#6411=VERTEX_POINT('',#153111);
#6412=VERTEX_POINT('',#153363);
#6413=VERTEX_POINT('',#153622);
#6414=VERTEX_POINT('',#153623);
#6415=VERTEX_POINT('',#153625);
#6416=VERTEX_POINT('',#153877);
#6417=VERTEX_POINT('',#154136);
#6418=VERTEX_POINT('',#154137);
#6419=VERTEX_POINT('',#154139);
#6420=VERTEX_POINT('',#154388);
#6421=VERTEX_POINT('',#154638);
#6422=VERTEX_POINT('',#154639);
#6423=VERTEX_POINT('',#154641);
#6424=VERTEX_POINT('',#154875);
#6425=VERTEX_POINT('',#155131);
#6426=VERTEX_POINT('',#155132);
#6427=VERTEX_POINT('',#155134);
#6428=VERTEX_POINT('',#155392);
#6429=VERTEX_POINT('',#155642);
#6430=VERTEX_POINT('',#155643);
#6431=VERTEX_POINT('',#155645);
#6432=VERTEX_POINT('',#155903);
#6433=VERTEX_POINT('',#156153);
#6434=VERTEX_POINT('',#156154);
#6435=VERTEX_POINT('',#156156);
#6436=VERTEX_POINT('',#156393);
#6437=VERTEX_POINT('',#156646);
#6438=VERTEX_POINT('',#156647);
#6439=VERTEX_POINT('',#156649);
#6440=VERTEX_POINT('',#156901);
#6441=VERTEX_POINT('',#157151);
#6442=VERTEX_POINT('',#157152);
#6443=VERTEX_POINT('',#157154);
#6444=VERTEX_POINT('',#157409);
#6445=VERTEX_POINT('',#157665);
#6446=VERTEX_POINT('',#157666);
#6447=VERTEX_POINT('',#157668);
#6448=VERTEX_POINT('',#157920);
#6449=VERTEX_POINT('',#158179);
#6450=VERTEX_POINT('',#158180);
#6451=VERTEX_POINT('',#158182);
#6452=VERTEX_POINT('',#158434);
#6453=VERTEX_POINT('',#158690);
#6454=VERTEX_POINT('',#158691);
#6455=VERTEX_POINT('',#158693);
#6456=VERTEX_POINT('',#158945);
#6457=VERTEX_POINT('',#159201);
#6458=VERTEX_POINT('',#159202);
#6459=VERTEX_POINT('',#159204);
#6460=VERTEX_POINT('',#159459);
#6461=VERTEX_POINT('',#159709);
#6462=VERTEX_POINT('',#159710);
#6463=VERTEX_POINT('',#159712);
#6464=VERTEX_POINT('',#159946);
#6465=VERTEX_POINT('',#160202);
#6466=VERTEX_POINT('',#160203);
#6467=VERTEX_POINT('',#160205);
#6468=VERTEX_POINT('',#160460);
#6469=VERTEX_POINT('',#160710);
#6470=VERTEX_POINT('',#160711);
#6471=VERTEX_POINT('',#160713);
#6472=VERTEX_POINT('',#160727);
#6473=VERTEX_POINT('',#160882);
#6474=VERTEX_POINT('',#160884);
#6475=VERTEX_POINT('',#161122);
#6476=VERTEX_POINT('',#161377);
#6477=VERTEX_POINT('',#161630);
#6478=VERTEX_POINT('',#161631);
#6479=VERTEX_POINT('',#161687);
#6480=VERTEX_POINT('',#161689);
#6481=VERTEX_POINT('',#161698);
#6482=VERTEX_POINT('',#161714);
#6483=VERTEX_POINT('',#161971);
#6484=VERTEX_POINT('',#162228);
#6485=VERTEX_POINT('',#162935);
#6486=VERTEX_POINT('',#163468);
#6487=VERTEX_POINT('',#163484);
#6488=VERTEX_POINT('',#163744);
#6489=VERTEX_POINT('',#164001);
#6490=VERTEX_POINT('',#164017);
#6491=VERTEX_POINT('',#164274);
#6492=VERTEX_POINT('',#164534);
#6493=VERTEX_POINT('',#165259);
#6494=VERTEX_POINT('',#165802);
#6495=VERTEX_POINT('',#166395);
#6496=VERTEX_POINT('',#166652);
#6497=VERTEX_POINT('',#166668);
#6498=VERTEX_POINT('',#166925);
#6499=VERTEX_POINT('',#167182);
#6500=VERTEX_POINT('',#167201);
#6501=VERTEX_POINT('',#167214);
#6502=VERTEX_POINT('',#167233);
#6503=VERTEX_POINT('',#167814);
#6504=VERTEX_POINT('',#167833);
#6505=VERTEX_POINT('',#168436);
#6506=VERTEX_POINT('',#168452);
#6507=VERTEX_POINT('',#168709);
#6508=VERTEX_POINT('',#168726);
#6509=VERTEX_POINT('',#168983);
#6510=VERTEX_POINT('',#169002);
#6511=VERTEX_POINT('',#169018);
#6512=VERTEX_POINT('',#169272);
#6513=VERTEX_POINT('',#169291);
#6514=VERTEX_POINT('',#170058);
#6515=VERTEX_POINT('',#170074);
#6516=VERTEX_POINT('',#170089);
#6517=VERTEX_POINT('',#170106);
#6518=VERTEX_POINT('',#170363);
#6519=VERTEX_POINT('',#170898);
#6520=VERTEX_POINT('',#170913);
#6521=VERTEX_POINT('',#170932);
#6522=VERTEX_POINT('',#170988);
#6523=VERTEX_POINT('',#170990);
#6524=VERTEX_POINT('',#170999);
#6525=VERTEX_POINT('',#171015);
#6526=VERTEX_POINT('',#171802);
#6527=VERTEX_POINT('',#172507);
#6528=VERTEX_POINT('',#173050);
#6529=VERTEX_POINT('',#173066);
#6530=VERTEX_POINT('',#173326);
#6531=VERTEX_POINT('',#173583);
#6532=VERTEX_POINT('',#173599);
#6533=VERTEX_POINT('',#173856);
#6534=VERTEX_POINT('',#174116);
#6535=VERTEX_POINT('',#174841);
#6536=VERTEX_POINT('',#175378);
#6537=VERTEX_POINT('',#175947);
#6538=VERTEX_POINT('',#176204);
#6539=VERTEX_POINT('',#176220);
#6540=VERTEX_POINT('',#176477);
#6541=VERTEX_POINT('',#176734);
#6542=VERTEX_POINT('',#176753);
#6543=VERTEX_POINT('',#177013);
#6544=VERTEX_POINT('',#177032);
#6545=VERTEX_POINT('',#177739);
#6546=VERTEX_POINT('',#177758);
#6547=VERTEX_POINT('',#178589);
#6548=VERTEX_POINT('',#178605);
#6549=VERTEX_POINT('',#178862);
#6550=VERTEX_POINT('',#178879);
#6551=VERTEX_POINT('',#179136);
#6552=VERTEX_POINT('',#179155);
#6553=VERTEX_POINT('',#179171);
#6554=VERTEX_POINT('',#179425);
#6555=VERTEX_POINT('',#179444);
#6556=VERTEX_POINT('',#179459);
#6557=VERTEX_POINT('',#179476);
#6558=VERTEX_POINT('',#179492);
#6559=VERTEX_POINT('',#179507);
#6560=VERTEX_POINT('',#179524);
#6561=VERTEX_POINT('',#179781);
#6562=VERTEX_POINT('',#180320);
#6563=VERTEX_POINT('',#180354);
#6564=VERTEX_POINT('',#180356);
#6565=VERTEX_POINT('',#180359);
#6566=VERTEX_POINT('',#180363);
#6567=VERTEX_POINT('',#180364);
#6568=VERTEX_POINT('',#180366);
#6569=VERTEX_POINT('',#180368);
#6570=VERTEX_POINT('',#180372);
#6571=VERTEX_POINT('',#180373);
#6572=VERTEX_POINT('',#180378);
#6573=VERTEX_POINT('',#180379);
#6574=VERTEX_POINT('',#185139);
#8781=EDGE_CURVE('',#6275,#6276,#4264,.T.);
#8782=EDGE_CURVE('',#6276,#6277,#2981,.T.);
#8783=EDGE_CURVE('',#6277,#6278,#1883,.T.);
#8784=EDGE_CURVE('',#6278,#6279,#4265,.T.);
#8785=EDGE_CURVE('',#6279,#6279,#1884,.F.);
#8786=EDGE_CURVE('',#6278,#6280,#1885,.T.);
#8787=EDGE_CURVE('',#6280,#6275,#2982,.T.);
#8788=EDGE_CURVE('',#6281,#6282,#4266,.T.);
#8789=EDGE_CURVE('',#6282,#6283,#2983,.T.);
#8790=EDGE_CURVE('',#6283,#6276,#2984,.T.);
#8791=EDGE_CURVE('',#6275,#6284,#2985,.T.);
#8792=EDGE_CURVE('',#6284,#6281,#2986,.T.);
#8793=EDGE_CURVE('',#6285,#6286,#4267,.T.);
#8794=EDGE_CURVE('',#6286,#6287,#2987,.T.);
#8795=EDGE_CURVE('',#6287,#6282,#2988,.T.);
#8796=EDGE_CURVE('',#6281,#6288,#2989,.T.);
#8797=EDGE_CURVE('',#6288,#6285,#2990,.T.);
#8798=EDGE_CURVE('',#6289,#6290,#4268,.T.);
#8799=EDGE_CURVE('',#6290,#6291,#2991,.T.);
#8800=EDGE_CURVE('',#6291,#6286,#2992,.T.);
#8801=EDGE_CURVE('',#6285,#6292,#2993,.T.);
#8802=EDGE_CURVE('',#6292,#6289,#2994,.T.);
#8803=EDGE_CURVE('',#6293,#6294,#4269,.T.);
#8804=EDGE_CURVE('',#6294,#6295,#2995,.T.);
#8805=EDGE_CURVE('',#6295,#6290,#2996,.T.);
#8806=EDGE_CURVE('',#6289,#6296,#2997,.T.);
#8807=EDGE_CURVE('',#6296,#6293,#2998,.T.);
#8808=EDGE_CURVE('',#6297,#6298,#4270,.T.);
#8809=EDGE_CURVE('',#6298,#6299,#2999,.T.);
#8810=EDGE_CURVE('',#6299,#6294,#3000,.T.);
#8811=EDGE_CURVE('',#6293,#6300,#3001,.T.);
#8812=EDGE_CURVE('',#6300,#6297,#3002,.T.);
#8813=EDGE_CURVE('',#6301,#6302,#4271,.T.);
#8814=EDGE_CURVE('',#6302,#6303,#3003,.T.);
#8815=EDGE_CURVE('',#6303,#6298,#3004,.T.);
#8816=EDGE_CURVE('',#6297,#6304,#3005,.T.);
#8817=EDGE_CURVE('',#6304,#6301,#3006,.T.);
#8818=EDGE_CURVE('',#6305,#6306,#4272,.T.);
#8819=EDGE_CURVE('',#6306,#6307,#3007,.T.);
#8820=EDGE_CURVE('',#6307,#6302,#3008,.T.);
#8821=EDGE_CURVE('',#6301,#6308,#3009,.T.);
#8822=EDGE_CURVE('',#6308,#6305,#3010,.T.);
#8823=EDGE_CURVE('',#6309,#6310,#4273,.T.);
#8824=EDGE_CURVE('',#6310,#6311,#3011,.T.);
#8825=EDGE_CURVE('',#6311,#6306,#3012,.T.);
#8826=EDGE_CURVE('',#6305,#6312,#3013,.T.);
#8827=EDGE_CURVE('',#6312,#6309,#3014,.T.);
#8828=EDGE_CURVE('',#6313,#6314,#4274,.T.);
#8829=EDGE_CURVE('',#6314,#6315,#3015,.T.);
#8830=EDGE_CURVE('',#6315,#6310,#3016,.T.);
#8831=EDGE_CURVE('',#6309,#6316,#3017,.T.);
#8832=EDGE_CURVE('',#6316,#6313,#3018,.T.);
#8833=EDGE_CURVE('',#6317,#6318,#4275,.T.);
#8834=EDGE_CURVE('',#6318,#6319,#3019,.T.);
#8835=EDGE_CURVE('',#6319,#6314,#3020,.T.);
#8836=EDGE_CURVE('',#6313,#6320,#3021,.T.);
#8837=EDGE_CURVE('',#6320,#6317,#3022,.T.);
#8838=EDGE_CURVE('',#6321,#6322,#4276,.T.);
#8839=EDGE_CURVE('',#6322,#6323,#3023,.T.);
#8840=EDGE_CURVE('',#6323,#6318,#3024,.T.);
#8841=EDGE_CURVE('',#6317,#6324,#3025,.T.);
#8842=EDGE_CURVE('',#6324,#6321,#3026,.T.);
#8843=EDGE_CURVE('',#6325,#6326,#4277,.T.);
#8844=EDGE_CURVE('',#6326,#6327,#3027,.T.);
#8845=EDGE_CURVE('',#6327,#6322,#3028,.T.);
#8846=EDGE_CURVE('',#6321,#6328,#3029,.T.);
#8847=EDGE_CURVE('',#6328,#6325,#3030,.T.);
#8848=EDGE_CURVE('',#6329,#6330,#4278,.T.);
#8849=EDGE_CURVE('',#6330,#6331,#3031,.T.);
#8850=EDGE_CURVE('',#6331,#6326,#3032,.T.);
#8851=EDGE_CURVE('',#6325,#6332,#3033,.T.);
#8852=EDGE_CURVE('',#6332,#6329,#3034,.T.);
#8853=EDGE_CURVE('',#6333,#6334,#4279,.T.);
#8854=EDGE_CURVE('',#6334,#6335,#3035,.T.);
#8855=EDGE_CURVE('',#6335,#6330,#3036,.T.);
#8856=EDGE_CURVE('',#6329,#6336,#3037,.T.);
#8857=EDGE_CURVE('',#6336,#6333,#3038,.T.);
#8858=EDGE_CURVE('',#6337,#6338,#4280,.T.);
#8859=EDGE_CURVE('',#6338,#6339,#3039,.T.);
#8860=EDGE_CURVE('',#6339,#6334,#3040,.T.);
#8861=EDGE_CURVE('',#6333,#6340,#3041,.T.);
#8862=EDGE_CURVE('',#6340,#6337,#3042,.T.);
#8863=EDGE_CURVE('',#6341,#6342,#4281,.T.);
#8864=EDGE_CURVE('',#6342,#6343,#3043,.T.);
#8865=EDGE_CURVE('',#6343,#6338,#3044,.T.);
#8866=EDGE_CURVE('',#6337,#6344,#3045,.T.);
#8867=EDGE_CURVE('',#6344,#6341,#3046,.T.);
#8868=EDGE_CURVE('',#6345,#6346,#4282,.T.);
#8869=EDGE_CURVE('',#6346,#6347,#3047,.T.);
#8870=EDGE_CURVE('',#6347,#6342,#3048,.T.);
#8871=EDGE_CURVE('',#6341,#6348,#3049,.T.);
#8872=EDGE_CURVE('',#6348,#6345,#3050,.T.);
#8873=EDGE_CURVE('',#6349,#6350,#4283,.T.);
#8874=EDGE_CURVE('',#6350,#6351,#3051,.T.);
#8875=EDGE_CURVE('',#6351,#6346,#3052,.T.);
#8876=EDGE_CURVE('',#6345,#6352,#3053,.T.);
#8877=EDGE_CURVE('',#6352,#6349,#3054,.T.);
#8878=EDGE_CURVE('',#6353,#6354,#4284,.T.);
#8879=EDGE_CURVE('',#6354,#6355,#3055,.T.);
#8880=EDGE_CURVE('',#6355,#6350,#3056,.T.);
#8881=EDGE_CURVE('',#6349,#6356,#3057,.T.);
#8882=EDGE_CURVE('',#6356,#6353,#3058,.T.);
#8883=EDGE_CURVE('',#6357,#6358,#4285,.T.);
#8884=EDGE_CURVE('',#6358,#6359,#3059,.T.);
#8885=EDGE_CURVE('',#6359,#6354,#3060,.T.);
#8886=EDGE_CURVE('',#6353,#6360,#3061,.T.);
#8887=EDGE_CURVE('',#6360,#6357,#3062,.T.);
#8888=EDGE_CURVE('',#6361,#6362,#4286,.T.);
#8889=EDGE_CURVE('',#6362,#6363,#3063,.T.);
#8890=EDGE_CURVE('',#6363,#6358,#3064,.T.);
#8891=EDGE_CURVE('',#6357,#6364,#3065,.T.);
#8892=EDGE_CURVE('',#6364,#6361,#3066,.T.);
#8893=EDGE_CURVE('',#6365,#6366,#4287,.T.);
#8894=EDGE_CURVE('',#6366,#6367,#3067,.T.);
#8895=EDGE_CURVE('',#6367,#6362,#3068,.T.);
#8896=EDGE_CURVE('',#6361,#6368,#3069,.T.);
#8897=EDGE_CURVE('',#6368,#6365,#3070,.T.);
#8898=EDGE_CURVE('',#6369,#6370,#4288,.T.);
#8899=EDGE_CURVE('',#6370,#6371,#3071,.T.);
#8900=EDGE_CURVE('',#6371,#6366,#3072,.T.);
#8901=EDGE_CURVE('',#6365,#6372,#3073,.T.);
#8902=EDGE_CURVE('',#6372,#6369,#3074,.T.);
#8903=EDGE_CURVE('',#6373,#6374,#4289,.T.);
#8904=EDGE_CURVE('',#6374,#6375,#3075,.T.);
#8905=EDGE_CURVE('',#6375,#6370,#3076,.T.);
#8906=EDGE_CURVE('',#6369,#6376,#3077,.T.);
#8907=EDGE_CURVE('',#6376,#6373,#3078,.T.);
#8908=EDGE_CURVE('',#6377,#6378,#4290,.T.);
#8909=EDGE_CURVE('',#6378,#6379,#3079,.T.);
#8910=EDGE_CURVE('',#6379,#6374,#3080,.T.);
#8911=EDGE_CURVE('',#6373,#6380,#3081,.T.);
#8912=EDGE_CURVE('',#6380,#6377,#3082,.T.);
#8913=EDGE_CURVE('',#6381,#6382,#4291,.T.);
#8914=EDGE_CURVE('',#6382,#6383,#3083,.T.);
#8915=EDGE_CURVE('',#6383,#6378,#3084,.T.);
#8916=EDGE_CURVE('',#6377,#6384,#3085,.T.);
#8917=EDGE_CURVE('',#6384,#6381,#3086,.T.);
#8918=EDGE_CURVE('',#6385,#6386,#4292,.T.);
#8919=EDGE_CURVE('',#6386,#6387,#3087,.T.);
#8920=EDGE_CURVE('',#6387,#6382,#3088,.T.);
#8921=EDGE_CURVE('',#6381,#6388,#3089,.T.);
#8922=EDGE_CURVE('',#6388,#6385,#3090,.T.);
#8923=EDGE_CURVE('',#6389,#6390,#4293,.T.);
#8924=EDGE_CURVE('',#6390,#6391,#3091,.T.);
#8925=EDGE_CURVE('',#6391,#6386,#3092,.T.);
#8926=EDGE_CURVE('',#6385,#6392,#3093,.T.);
#8927=EDGE_CURVE('',#6392,#6389,#3094,.T.);
#8928=EDGE_CURVE('',#6393,#6394,#4294,.T.);
#8929=EDGE_CURVE('',#6394,#6395,#3095,.T.);
#8930=EDGE_CURVE('',#6395,#6390,#3096,.T.);
#8931=EDGE_CURVE('',#6389,#6396,#3097,.T.);
#8932=EDGE_CURVE('',#6396,#6393,#3098,.T.);
#8933=EDGE_CURVE('',#6397,#6398,#4295,.T.);
#8934=EDGE_CURVE('',#6398,#6399,#3099,.T.);
#8935=EDGE_CURVE('',#6399,#6394,#3100,.T.);
#8936=EDGE_CURVE('',#6393,#6400,#3101,.T.);
#8937=EDGE_CURVE('',#6400,#6397,#3102,.T.);
#8938=EDGE_CURVE('',#6401,#6402,#4296,.T.);
#8939=EDGE_CURVE('',#6402,#6403,#3103,.T.);
#8940=EDGE_CURVE('',#6403,#6398,#3104,.T.);
#8941=EDGE_CURVE('',#6397,#6404,#3105,.T.);
#8942=EDGE_CURVE('',#6404,#6401,#3106,.T.);
#8943=EDGE_CURVE('',#6405,#6406,#4297,.T.);
#8944=EDGE_CURVE('',#6406,#6407,#3107,.T.);
#8945=EDGE_CURVE('',#6407,#6402,#3108,.T.);
#8946=EDGE_CURVE('',#6401,#6408,#3109,.T.);
#8947=EDGE_CURVE('',#6408,#6405,#3110,.T.);
#8948=EDGE_CURVE('',#6409,#6410,#4298,.T.);
#8949=EDGE_CURVE('',#6410,#6411,#3111,.T.);
#8950=EDGE_CURVE('',#6411,#6406,#3112,.T.);
#8951=EDGE_CURVE('',#6405,#6412,#3113,.T.);
#8952=EDGE_CURVE('',#6412,#6409,#3114,.T.);
#8953=EDGE_CURVE('',#6413,#6414,#4299,.T.);
#8954=EDGE_CURVE('',#6414,#6415,#3115,.T.);
#8955=EDGE_CURVE('',#6415,#6410,#3116,.T.);
#8956=EDGE_CURVE('',#6409,#6416,#3117,.T.);
#8957=EDGE_CURVE('',#6416,#6413,#3118,.T.);
#8958=EDGE_CURVE('',#6417,#6418,#4300,.T.);
#8959=EDGE_CURVE('',#6418,#6419,#3119,.T.);
#8960=EDGE_CURVE('',#6419,#6414,#3120,.T.);
#8961=EDGE_CURVE('',#6413,#6420,#3121,.T.);
#8962=EDGE_CURVE('',#6420,#6417,#3122,.T.);
#8963=EDGE_CURVE('',#6421,#6422,#4301,.T.);
#8964=EDGE_CURVE('',#6422,#6423,#3123,.T.);
#8965=EDGE_CURVE('',#6423,#6418,#3124,.T.);
#8966=EDGE_CURVE('',#6417,#6424,#3125,.T.);
#8967=EDGE_CURVE('',#6424,#6421,#3126,.T.);
#8968=EDGE_CURVE('',#6425,#6426,#4302,.T.);
#8969=EDGE_CURVE('',#6426,#6427,#3127,.T.);
#8970=EDGE_CURVE('',#6427,#6422,#3128,.T.);
#8971=EDGE_CURVE('',#6421,#6428,#3129,.T.);
#8972=EDGE_CURVE('',#6428,#6425,#3130,.T.);
#8973=EDGE_CURVE('',#6429,#6430,#4303,.T.);
#8974=EDGE_CURVE('',#6430,#6431,#3131,.T.);
#8975=EDGE_CURVE('',#6431,#6426,#3132,.T.);
#8976=EDGE_CURVE('',#6425,#6432,#3133,.T.);
#8977=EDGE_CURVE('',#6432,#6429,#3134,.T.);
#8978=EDGE_CURVE('',#6433,#6434,#4304,.T.);
#8979=EDGE_CURVE('',#6434,#6435,#3135,.T.);
#8980=EDGE_CURVE('',#6435,#6430,#3136,.T.);
#8981=EDGE_CURVE('',#6429,#6436,#3137,.T.);
#8982=EDGE_CURVE('',#6436,#6433,#3138,.T.);
#8983=EDGE_CURVE('',#6437,#6438,#4305,.T.);
#8984=EDGE_CURVE('',#6438,#6439,#3139,.T.);
#8985=EDGE_CURVE('',#6439,#6434,#3140,.T.);
#8986=EDGE_CURVE('',#6433,#6440,#3141,.T.);
#8987=EDGE_CURVE('',#6440,#6437,#3142,.T.);
#8988=EDGE_CURVE('',#6441,#6442,#4306,.T.);
#8989=EDGE_CURVE('',#6442,#6443,#3143,.T.);
#8990=EDGE_CURVE('',#6443,#6438,#3144,.T.);
#8991=EDGE_CURVE('',#6437,#6444,#3145,.T.);
#8992=EDGE_CURVE('',#6444,#6441,#3146,.T.);
#8993=EDGE_CURVE('',#6445,#6446,#4307,.T.);
#8994=EDGE_CURVE('',#6446,#6447,#3147,.T.);
#8995=EDGE_CURVE('',#6447,#6442,#3148,.T.);
#8996=EDGE_CURVE('',#6441,#6448,#3149,.T.);
#8997=EDGE_CURVE('',#6448,#6445,#3150,.T.);
#8998=EDGE_CURVE('',#6449,#6450,#4308,.T.);
#8999=EDGE_CURVE('',#6450,#6451,#3151,.T.);
#9000=EDGE_CURVE('',#6451,#6446,#3152,.T.);
#9001=EDGE_CURVE('',#6445,#6452,#3153,.T.);
#9002=EDGE_CURVE('',#6452,#6449,#3154,.T.);
#9003=EDGE_CURVE('',#6453,#6454,#4309,.T.);
#9004=EDGE_CURVE('',#6454,#6455,#3155,.T.);
#9005=EDGE_CURVE('',#6455,#6450,#3156,.T.);
#9006=EDGE_CURVE('',#6449,#6456,#3157,.T.);
#9007=EDGE_CURVE('',#6456,#6453,#3158,.T.);
#9008=EDGE_CURVE('',#6457,#6458,#4310,.T.);
#9009=EDGE_CURVE('',#6458,#6459,#3159,.T.);
#9010=EDGE_CURVE('',#6459,#6454,#3160,.T.);
#9011=EDGE_CURVE('',#6453,#6460,#3161,.T.);
#9012=EDGE_CURVE('',#6460,#6457,#3162,.T.);
#9013=EDGE_CURVE('',#6461,#6462,#4311,.T.);
#9014=EDGE_CURVE('',#6462,#6463,#3163,.T.);
#9015=EDGE_CURVE('',#6463,#6458,#3164,.T.);
#9016=EDGE_CURVE('',#6457,#6464,#3165,.T.);
#9017=EDGE_CURVE('',#6464,#6461,#3166,.T.);
#9018=EDGE_CURVE('',#6465,#6466,#4312,.T.);
#9019=EDGE_CURVE('',#6466,#6467,#3167,.T.);
#9020=EDGE_CURVE('',#6467,#6462,#3168,.T.);
#9021=EDGE_CURVE('',#6461,#6468,#3169,.T.);
#9022=EDGE_CURVE('',#6468,#6465,#3170,.T.);
#9023=EDGE_CURVE('',#6469,#6470,#4313,.T.);
#9024=EDGE_CURVE('',#6469,#6471,#3171,.T.);
#9025=EDGE_CURVE('',#6471,#6472,#3172,.T.);
#9026=EDGE_CURVE('',#6473,#6472,#1886,.F.);
#9027=EDGE_CURVE('',#6473,#6474,#3173,.T.);
#9028=EDGE_CURVE('',#6474,#6470,#3174,.T.);
#9029=EDGE_CURVE('',#6470,#6475,#3175,.T.);
#9030=EDGE_CURVE('',#6475,#6466,#3176,.T.);
#9031=EDGE_CURVE('',#6465,#6476,#3177,.T.);
#9032=EDGE_CURVE('',#6476,#6469,#3178,.T.);
#9033=EDGE_CURVE('',#6477,#6478,#3179,.T.);
#9034=EDGE_CURVE('',#6479,#6477,#1887,.T.);
#9035=EDGE_CURVE('',#6479,#6480,#3180,.T.);
#9036=EDGE_CURVE('',#6480,#6481,#3181,.T.);
#9037=EDGE_CURVE('',#6481,#6482,#3182,.T.);
#9038=EDGE_CURVE('',#6482,#6483,#3183,.T.);
#9039=EDGE_CURVE('',#6483,#6484,#3184,.T.);
#9040=EDGE_CURVE('',#6484,#6485,#3185,.T.);
#9041=EDGE_CURVE('',#6485,#6486,#3186,.T.);
#9042=EDGE_CURVE('',#6486,#6487,#3187,.T.);
#9043=EDGE_CURVE('',#6487,#6488,#3188,.T.);
#9044=EDGE_CURVE('',#6488,#6489,#3189,.T.);
#9045=EDGE_CURVE('',#6489,#6490,#3190,.T.);
#9046=EDGE_CURVE('',#6490,#6491,#3191,.T.);
#9047=EDGE_CURVE('',#6491,#6492,#3192,.T.);
#9048=EDGE_CURVE('',#6492,#6493,#3193,.T.);
#9049=EDGE_CURVE('',#6493,#6494,#3194,.T.);
#9050=EDGE_CURVE('',#6494,#6495,#3195,.T.);
#9051=EDGE_CURVE('',#6495,#6496,#3196,.T.);
#9052=EDGE_CURVE('',#6496,#6497,#3197,.T.);
#9053=EDGE_CURVE('',#6497,#6498,#3198,.T.);
#9054=EDGE_CURVE('',#6498,#6499,#3199,.T.);
#9055=EDGE_CURVE('',#6499,#6500,#3200,.T.);
#9056=EDGE_CURVE('',#6500,#6501,#3201,.T.);
#9057=EDGE_CURVE('',#6501,#6502,#3202,.T.);
#9058=EDGE_CURVE('',#6502,#6503,#3203,.T.);
#9059=EDGE_CURVE('',#6503,#6504,#3204,.T.);
#9060=EDGE_CURVE('',#6504,#6505,#3205,.T.);
#9061=EDGE_CURVE('',#6505,#6506,#3206,.T.);
#9062=EDGE_CURVE('',#6506,#6507,#3207,.T.);
#9063=EDGE_CURVE('',#6507,#6508,#3208,.T.);
#9064=EDGE_CURVE('',#6508,#6509,#3209,.T.);
#9065=EDGE_CURVE('',#6509,#6510,#3210,.T.);
#9066=EDGE_CURVE('',#6510,#6511,#3211,.T.);
#9067=EDGE_CURVE('',#6511,#6512,#3212,.T.);
#9068=EDGE_CURVE('',#6512,#6513,#3213,.T.);
#9069=EDGE_CURVE('',#6513,#6514,#3214,.T.);
#9070=EDGE_CURVE('',#6514,#6515,#3215,.T.);
#9071=EDGE_CURVE('',#6515,#6516,#3216,.T.);
#9072=EDGE_CURVE('',#6516,#6517,#3217,.T.);
#9073=EDGE_CURVE('',#6517,#6518,#3218,.T.);
#9074=EDGE_CURVE('',#6518,#6519,#3219,.T.);
#9075=EDGE_CURVE('',#6519,#6520,#3220,.T.);
#9076=EDGE_CURVE('',#6520,#6521,#3221,.T.);
#9077=EDGE_CURVE('',#6522,#6521,#1888,.T.);
#9078=EDGE_CURVE('',#6523,#6522,#3222,.T.);
#9079=EDGE_CURVE('',#6524,#6523,#3223,.T.);
#9080=EDGE_CURVE('',#6525,#6524,#3224,.F.);
#9081=EDGE_CURVE('',#6526,#6525,#3225,.F.);
#9082=EDGE_CURVE('',#6527,#6526,#3226,.F.);
#9083=EDGE_CURVE('',#6528,#6527,#3227,.T.);
#9084=EDGE_CURVE('',#6529,#6528,#3228,.T.);
#9085=EDGE_CURVE('',#6530,#6529,#3229,.T.);
#9086=EDGE_CURVE('',#6531,#6530,#3230,.T.);
#9087=EDGE_CURVE('',#6532,#6531,#3231,.T.);
#9088=EDGE_CURVE('',#6533,#6532,#3232,.T.);
#9089=EDGE_CURVE('',#6534,#6533,#3233,.F.);
#9090=EDGE_CURVE('',#6535,#6534,#3234,.F.);
#9091=EDGE_CURVE('',#6536,#6535,#3235,.F.);
#9092=EDGE_CURVE('',#6537,#6536,#3236,.T.);
#9093=EDGE_CURVE('',#6538,#6537,#3237,.T.);
#9094=EDGE_CURVE('',#6539,#6538,#3238,.T.);
#9095=EDGE_CURVE('',#6540,#6539,#3239,.T.);
#9096=EDGE_CURVE('',#6541,#6540,#3240,.T.);
#9097=EDGE_CURVE('',#6542,#6541,#3241,.T.);
#9098=EDGE_CURVE('',#6543,#6542,#3242,.T.);
#9099=EDGE_CURVE('',#6544,#6543,#3243,.F.);
#9100=EDGE_CURVE('',#6545,#6544,#3244,.T.);
#9101=EDGE_CURVE('',#6546,#6545,#3245,.F.);
#9102=EDGE_CURVE('',#6547,#6546,#3246,.T.);
#9103=EDGE_CURVE('',#6548,#6547,#3247,.T.);
#9104=EDGE_CURVE('',#6549,#6548,#3248,.T.);
#9105=EDGE_CURVE('',#6550,#6549,#3249,.T.);
#9106=EDGE_CURVE('',#6551,#6550,#3250,.T.);
#9107=EDGE_CURVE('',#6552,#6551,#3251,.T.);
#9108=EDGE_CURVE('',#6553,#6552,#3252,.T.);
#9109=EDGE_CURVE('',#6554,#6553,#3253,.T.);
#9110=EDGE_CURVE('',#6555,#6554,#3254,.T.);
#9111=EDGE_CURVE('',#6556,#6555,#3255,.T.);
#9112=EDGE_CURVE('',#6557,#6556,#3256,.T.);
#9113=EDGE_CURVE('',#6558,#6557,#3257,.T.);
#9114=EDGE_CURVE('',#6559,#6558,#3258,.T.);
#9115=EDGE_CURVE('',#6560,#6559,#3259,.T.);
#9116=EDGE_CURVE('',#6561,#6560,#3260,.F.);
#9117=EDGE_CURVE('',#6562,#6561,#3261,.T.);
#9118=EDGE_CURVE('',#6478,#6562,#3262,.T.);
#9119=EDGE_CURVE('',#6563,#6563,#1889,.T.);
#9120=EDGE_CURVE('',#6564,#6564,#1890,.T.);
#9121=EDGE_CURVE('',#6563,#6565,#4314,.T.);
#9122=EDGE_CURVE('',#6565,#6565,#1891,.T.);
#9123=EDGE_CURVE('',#6566,#6567,#4315,.T.);
#9124=EDGE_CURVE('',#6566,#6568,#4316,.T.);
#9125=EDGE_CURVE('',#6569,#6568,#4317,.T.);
#9126=EDGE_CURVE('',#6567,#6569,#4318,.T.);
#9127=EDGE_CURVE('',#6570,#6571,#4319,.T.);
#9128=EDGE_CURVE('',#6568,#6570,#4320,.T.);
#9129=EDGE_CURVE('',#6571,#6566,#4321,.T.);
#9130=EDGE_CURVE('',#6572,#6573,#4322,.T.);
#9131=EDGE_CURVE('',#6567,#6572,#4323,.T.);
#9132=EDGE_CURVE('',#6573,#6569,#4324,.T.);
#9133=EDGE_CURVE('',#6572,#6571,#1892,.T.);
#9134=EDGE_CURVE('',#6277,#6522,#3263,.T.);
#9135=EDGE_CURVE('',#6521,#6280,#3264,.T.);
#9136=EDGE_CURVE('',#6472,#6479,#3265,.T.);
#9137=EDGE_CURVE('',#6477,#6473,#3266,.T.);
#9138=EDGE_CURVE('',#6574,#6574,#1893,.T.);
#9139=EDGE_CURVE('',#6574,#6564,#4325,.T.);
#9140=EDGE_CURVE('',#6573,#6570,#1894,.T.);
#12939=ORIENTED_EDGE('',*,*,#8781,.T.);
#12940=ORIENTED_EDGE('',*,*,#8782,.T.);
#12941=ORIENTED_EDGE('',*,*,#8783,.T.);
#12942=ORIENTED_EDGE('',*,*,#8784,.T.);
#12943=ORIENTED_EDGE('',*,*,#8785,.T.);
#12944=ORIENTED_EDGE('',*,*,#8784,.F.);
#12945=ORIENTED_EDGE('',*,*,#8786,.T.);
#12946=ORIENTED_EDGE('',*,*,#8787,.T.);
#12947=ORIENTED_EDGE('',*,*,#8788,.T.);
#12948=ORIENTED_EDGE('',*,*,#8789,.T.);
#12949=ORIENTED_EDGE('',*,*,#8790,.T.);
#12950=ORIENTED_EDGE('',*,*,#8781,.F.);
#12951=ORIENTED_EDGE('',*,*,#8791,.T.);
#12952=ORIENTED_EDGE('',*,*,#8792,.T.);
#12953=ORIENTED_EDGE('',*,*,#8793,.T.);
#12954=ORIENTED_EDGE('',*,*,#8794,.T.);
#12955=ORIENTED_EDGE('',*,*,#8795,.T.);
#12956=ORIENTED_EDGE('',*,*,#8788,.F.);
#12957=ORIENTED_EDGE('',*,*,#8796,.T.);
#12958=ORIENTED_EDGE('',*,*,#8797,.T.);
#12959=ORIENTED_EDGE('',*,*,#8798,.T.);
#12960=ORIENTED_EDGE('',*,*,#8799,.T.);
#12961=ORIENTED_EDGE('',*,*,#8800,.T.);
#12962=ORIENTED_EDGE('',*,*,#8793,.F.);
#12963=ORIENTED_EDGE('',*,*,#8801,.T.);
#12964=ORIENTED_EDGE('',*,*,#8802,.T.);
#12965=ORIENTED_EDGE('',*,*,#8803,.T.);
#12966=ORIENTED_EDGE('',*,*,#8804,.T.);
#12967=ORIENTED_EDGE('',*,*,#8805,.T.);
#12968=ORIENTED_EDGE('',*,*,#8798,.F.);
#12969=ORIENTED_EDGE('',*,*,#8806,.T.);
#12970=ORIENTED_EDGE('',*,*,#8807,.T.);
#12971=ORIENTED_EDGE('',*,*,#8808,.T.);
#12972=ORIENTED_EDGE('',*,*,#8809,.T.);
#12973=ORIENTED_EDGE('',*,*,#8810,.T.);
#12974=ORIENTED_EDGE('',*,*,#8803,.F.);
#12975=ORIENTED_EDGE('',*,*,#8811,.T.);
#12976=ORIENTED_EDGE('',*,*,#8812,.T.);
#12977=ORIENTED_EDGE('',*,*,#8813,.T.);
#12978=ORIENTED_EDGE('',*,*,#8814,.T.);
#12979=ORIENTED_EDGE('',*,*,#8815,.T.);
#12980=ORIENTED_EDGE('',*,*,#8808,.F.);
#12981=ORIENTED_EDGE('',*,*,#8816,.T.);
#12982=ORIENTED_EDGE('',*,*,#8817,.T.);
#12983=ORIENTED_EDGE('',*,*,#8818,.T.);
#12984=ORIENTED_EDGE('',*,*,#8819,.T.);
#12985=ORIENTED_EDGE('',*,*,#8820,.T.);
#12986=ORIENTED_EDGE('',*,*,#8813,.F.);
#12987=ORIENTED_EDGE('',*,*,#8821,.T.);
#12988=ORIENTED_EDGE('',*,*,#8822,.T.);
#12989=ORIENTED_EDGE('',*,*,#8823,.T.);
#12990=ORIENTED_EDGE('',*,*,#8824,.T.);
#12991=ORIENTED_EDGE('',*,*,#8825,.T.);
#12992=ORIENTED_EDGE('',*,*,#8818,.F.);
#12993=ORIENTED_EDGE('',*,*,#8826,.T.);
#12994=ORIENTED_EDGE('',*,*,#8827,.T.);
#12995=ORIENTED_EDGE('',*,*,#8828,.T.);
#12996=ORIENTED_EDGE('',*,*,#8829,.T.);
#12997=ORIENTED_EDGE('',*,*,#8830,.T.);
#12998=ORIENTED_EDGE('',*,*,#8823,.F.);
#12999=ORIENTED_EDGE('',*,*,#8831,.T.);
#13000=ORIENTED_EDGE('',*,*,#8832,.T.);
#13001=ORIENTED_EDGE('',*,*,#8833,.T.);
#13002=ORIENTED_EDGE('',*,*,#8834,.T.);
#13003=ORIENTED_EDGE('',*,*,#8835,.T.);
#13004=ORIENTED_EDGE('',*,*,#8828,.F.);
#13005=ORIENTED_EDGE('',*,*,#8836,.T.);
#13006=ORIENTED_EDGE('',*,*,#8837,.T.);
#13007=ORIENTED_EDGE('',*,*,#8838,.T.);
#13008=ORIENTED_EDGE('',*,*,#8839,.T.);
#13009=ORIENTED_EDGE('',*,*,#8840,.T.);
#13010=ORIENTED_EDGE('',*,*,#8833,.F.);
#13011=ORIENTED_EDGE('',*,*,#8841,.T.);
#13012=ORIENTED_EDGE('',*,*,#8842,.T.);
#13013=ORIENTED_EDGE('',*,*,#8843,.T.);
#13014=ORIENTED_EDGE('',*,*,#8844,.T.);
#13015=ORIENTED_EDGE('',*,*,#8845,.T.);
#13016=ORIENTED_EDGE('',*,*,#8838,.F.);
#13017=ORIENTED_EDGE('',*,*,#8846,.T.);
#13018=ORIENTED_EDGE('',*,*,#8847,.T.);
#13019=ORIENTED_EDGE('',*,*,#8848,.T.);
#13020=ORIENTED_EDGE('',*,*,#8849,.T.);
#13021=ORIENTED_EDGE('',*,*,#8850,.T.);
#13022=ORIENTED_EDGE('',*,*,#8843,.F.);
#13023=ORIENTED_EDGE('',*,*,#8851,.T.);
#13024=ORIENTED_EDGE('',*,*,#8852,.T.);
#13025=ORIENTED_EDGE('',*,*,#8853,.T.);
#13026=ORIENTED_EDGE('',*,*,#8854,.T.);
#13027=ORIENTED_EDGE('',*,*,#8855,.T.);
#13028=ORIENTED_EDGE('',*,*,#8848,.F.);
#13029=ORIENTED_EDGE('',*,*,#8856,.T.);
#13030=ORIENTED_EDGE('',*,*,#8857,.T.);
#13031=ORIENTED_EDGE('',*,*,#8858,.T.);
#13032=ORIENTED_EDGE('',*,*,#8859,.T.);
#13033=ORIENTED_EDGE('',*,*,#8860,.T.);
#13034=ORIENTED_EDGE('',*,*,#8853,.F.);
#13035=ORIENTED_EDGE('',*,*,#8861,.T.);
#13036=ORIENTED_EDGE('',*,*,#8862,.T.);
#13037=ORIENTED_EDGE('',*,*,#8863,.T.);
#13038=ORIENTED_EDGE('',*,*,#8864,.T.);
#13039=ORIENTED_EDGE('',*,*,#8865,.T.);
#13040=ORIENTED_EDGE('',*,*,#8858,.F.);
#13041=ORIENTED_EDGE('',*,*,#8866,.T.);
#13042=ORIENTED_EDGE('',*,*,#8867,.T.);
#13043=ORIENTED_EDGE('',*,*,#8868,.T.);
#13044=ORIENTED_EDGE('',*,*,#8869,.T.);
#13045=ORIENTED_EDGE('',*,*,#8870,.T.);
#13046=ORIENTED_EDGE('',*,*,#8863,.F.);
#13047=ORIENTED_EDGE('',*,*,#8871,.T.);
#13048=ORIENTED_EDGE('',*,*,#8872,.T.);
#13049=ORIENTED_EDGE('',*,*,#8873,.T.);
#13050=ORIENTED_EDGE('',*,*,#8874,.T.);
#13051=ORIENTED_EDGE('',*,*,#8875,.T.);
#13052=ORIENTED_EDGE('',*,*,#8868,.F.);
#13053=ORIENTED_EDGE('',*,*,#8876,.T.);
#13054=ORIENTED_EDGE('',*,*,#8877,.T.);
#13055=ORIENTED_EDGE('',*,*,#8878,.T.);
#13056=ORIENTED_EDGE('',*,*,#8879,.T.);
#13057=ORIENTED_EDGE('',*,*,#8880,.T.);
#13058=ORIENTED_EDGE('',*,*,#8873,.F.);
#13059=ORIENTED_EDGE('',*,*,#8881,.T.);
#13060=ORIENTED_EDGE('',*,*,#8882,.T.);
#13061=ORIENTED_EDGE('',*,*,#8883,.T.);
#13062=ORIENTED_EDGE('',*,*,#8884,.T.);
#13063=ORIENTED_EDGE('',*,*,#8885,.T.);
#13064=ORIENTED_EDGE('',*,*,#8878,.F.);
#13065=ORIENTED_EDGE('',*,*,#8886,.T.);
#13066=ORIENTED_EDGE('',*,*,#8887,.T.);
#13067=ORIENTED_EDGE('',*,*,#8888,.T.);
#13068=ORIENTED_EDGE('',*,*,#8889,.T.);
#13069=ORIENTED_EDGE('',*,*,#8890,.T.);
#13070=ORIENTED_EDGE('',*,*,#8883,.F.);
#13071=ORIENTED_EDGE('',*,*,#8891,.T.);
#13072=ORIENTED_EDGE('',*,*,#8892,.T.);
#13073=ORIENTED_EDGE('',*,*,#8893,.T.);
#13074=ORIENTED_EDGE('',*,*,#8894,.T.);
#13075=ORIENTED_EDGE('',*,*,#8895,.T.);
#13076=ORIENTED_EDGE('',*,*,#8888,.F.);
#13077=ORIENTED_EDGE('',*,*,#8896,.T.);
#13078=ORIENTED_EDGE('',*,*,#8897,.T.);
#13079=ORIENTED_EDGE('',*,*,#8898,.T.);
#13080=ORIENTED_EDGE('',*,*,#8899,.T.);
#13081=ORIENTED_EDGE('',*,*,#8900,.T.);
#13082=ORIENTED_EDGE('',*,*,#8893,.F.);
#13083=ORIENTED_EDGE('',*,*,#8901,.T.);
#13084=ORIENTED_EDGE('',*,*,#8902,.T.);
#13085=ORIENTED_EDGE('',*,*,#8903,.T.);
#13086=ORIENTED_EDGE('',*,*,#8904,.T.);
#13087=ORIENTED_EDGE('',*,*,#8905,.T.);
#13088=ORIENTED_EDGE('',*,*,#8898,.F.);
#13089=ORIENTED_EDGE('',*,*,#8906,.T.);
#13090=ORIENTED_EDGE('',*,*,#8907,.T.);
#13091=ORIENTED_EDGE('',*,*,#8908,.T.);
#13092=ORIENTED_EDGE('',*,*,#8909,.T.);
#13093=ORIENTED_EDGE('',*,*,#8910,.T.);
#13094=ORIENTED_EDGE('',*,*,#8903,.F.);
#13095=ORIENTED_EDGE('',*,*,#8911,.T.);
#13096=ORIENTED_EDGE('',*,*,#8912,.T.);
#13097=ORIENTED_EDGE('',*,*,#8913,.T.);
#13098=ORIENTED_EDGE('',*,*,#8914,.T.);
#13099=ORIENTED_EDGE('',*,*,#8915,.T.);
#13100=ORIENTED_EDGE('',*,*,#8908,.F.);
#13101=ORIENTED_EDGE('',*,*,#8916,.T.);
#13102=ORIENTED_EDGE('',*,*,#8917,.T.);
#13103=ORIENTED_EDGE('',*,*,#8918,.T.);
#13104=ORIENTED_EDGE('',*,*,#8919,.T.);
#13105=ORIENTED_EDGE('',*,*,#8920,.T.);
#13106=ORIENTED_EDGE('',*,*,#8913,.F.);
#13107=ORIENTED_EDGE('',*,*,#8921,.T.);
#13108=ORIENTED_EDGE('',*,*,#8922,.T.);
#13109=ORIENTED_EDGE('',*,*,#8923,.T.);
#13110=ORIENTED_EDGE('',*,*,#8924,.T.);
#13111=ORIENTED_EDGE('',*,*,#8925,.T.);
#13112=ORIENTED_EDGE('',*,*,#8918,.F.);
#13113=ORIENTED_EDGE('',*,*,#8926,.T.);
#13114=ORIENTED_EDGE('',*,*,#8927,.T.);
#13115=ORIENTED_EDGE('',*,*,#8928,.T.);
#13116=ORIENTED_EDGE('',*,*,#8929,.T.);
#13117=ORIENTED_EDGE('',*,*,#8930,.T.);
#13118=ORIENTED_EDGE('',*,*,#8923,.F.);
#13119=ORIENTED_EDGE('',*,*,#8931,.T.);
#13120=ORIENTED_EDGE('',*,*,#8932,.T.);
#13121=ORIENTED_EDGE('',*,*,#8933,.T.);
#13122=ORIENTED_EDGE('',*,*,#8934,.T.);
#13123=ORIENTED_EDGE('',*,*,#8935,.T.);
#13124=ORIENTED_EDGE('',*,*,#8928,.F.);
#13125=ORIENTED_EDGE('',*,*,#8936,.T.);
#13126=ORIENTED_EDGE('',*,*,#8937,.T.);
#13127=ORIENTED_EDGE('',*,*,#8938,.T.);
#13128=ORIENTED_EDGE('',*,*,#8939,.T.);
#13129=ORIENTED_EDGE('',*,*,#8940,.T.);
#13130=ORIENTED_EDGE('',*,*,#8933,.F.);
#13131=ORIENTED_EDGE('',*,*,#8941,.T.);
#13132=ORIENTED_EDGE('',*,*,#8942,.T.);
#13133=ORIENTED_EDGE('',*,*,#8943,.T.);
#13134=ORIENTED_EDGE('',*,*,#8944,.T.);
#13135=ORIENTED_EDGE('',*,*,#8945,.T.);
#13136=ORIENTED_EDGE('',*,*,#8938,.F.);
#13137=ORIENTED_EDGE('',*,*,#8946,.T.);
#13138=ORIENTED_EDGE('',*,*,#8947,.T.);
#13139=ORIENTED_EDGE('',*,*,#8948,.T.);
#13140=ORIENTED_EDGE('',*,*,#8949,.T.);
#13141=ORIENTED_EDGE('',*,*,#8950,.T.);
#13142=ORIENTED_EDGE('',*,*,#8943,.F.);
#13143=ORIENTED_EDGE('',*,*,#8951,.T.);
#13144=ORIENTED_EDGE('',*,*,#8952,.T.);
#13145=ORIENTED_EDGE('',*,*,#8953,.T.);
#13146=ORIENTED_EDGE('',*,*,#8954,.T.);
#13147=ORIENTED_EDGE('',*,*,#8955,.T.);
#13148=ORIENTED_EDGE('',*,*,#8948,.F.);
#13149=ORIENTED_EDGE('',*,*,#8956,.T.);
#13150=ORIENTED_EDGE('',*,*,#8957,.T.);
#13151=ORIENTED_EDGE('',*,*,#8958,.T.);
#13152=ORIENTED_EDGE('',*,*,#8959,.T.);
#13153=ORIENTED_EDGE('',*,*,#8960,.T.);
#13154=ORIENTED_EDGE('',*,*,#8953,.F.);
#13155=ORIENTED_EDGE('',*,*,#8961,.T.);
#13156=ORIENTED_EDGE('',*,*,#8962,.T.);
#13157=ORIENTED_EDGE('',*,*,#8963,.T.);
#13158=ORIENTED_EDGE('',*,*,#8964,.T.);
#13159=ORIENTED_EDGE('',*,*,#8965,.T.);
#13160=ORIENTED_EDGE('',*,*,#8958,.F.);
#13161=ORIENTED_EDGE('',*,*,#8966,.T.);
#13162=ORIENTED_EDGE('',*,*,#8967,.T.);
#13163=ORIENTED_EDGE('',*,*,#8968,.T.);
#13164=ORIENTED_EDGE('',*,*,#8969,.T.);
#13165=ORIENTED_EDGE('',*,*,#8970,.T.);
#13166=ORIENTED_EDGE('',*,*,#8963,.F.);
#13167=ORIENTED_EDGE('',*,*,#8971,.T.);
#13168=ORIENTED_EDGE('',*,*,#8972,.T.);
#13169=ORIENTED_EDGE('',*,*,#8973,.T.);
#13170=ORIENTED_EDGE('',*,*,#8974,.T.);
#13171=ORIENTED_EDGE('',*,*,#8975,.T.);
#13172=ORIENTED_EDGE('',*,*,#8968,.F.);
#13173=ORIENTED_EDGE('',*,*,#8976,.T.);
#13174=ORIENTED_EDGE('',*,*,#8977,.T.);
#13175=ORIENTED_EDGE('',*,*,#8978,.T.);
#13176=ORIENTED_EDGE('',*,*,#8979,.T.);
#13177=ORIENTED_EDGE('',*,*,#8980,.T.);
#13178=ORIENTED_EDGE('',*,*,#8973,.F.);
#13179=ORIENTED_EDGE('',*,*,#8981,.T.);
#13180=ORIENTED_EDGE('',*,*,#8982,.T.);
#13181=ORIENTED_EDGE('',*,*,#8983,.T.);
#13182=ORIENTED_EDGE('',*,*,#8984,.T.);
#13183=ORIENTED_EDGE('',*,*,#8985,.T.);
#13184=ORIENTED_EDGE('',*,*,#8978,.F.);
#13185=ORIENTED_EDGE('',*,*,#8986,.T.);
#13186=ORIENTED_EDGE('',*,*,#8987,.T.);
#13187=ORIENTED_EDGE('',*,*,#8988,.T.);
#13188=ORIENTED_EDGE('',*,*,#8989,.T.);
#13189=ORIENTED_EDGE('',*,*,#8990,.T.);
#13190=ORIENTED_EDGE('',*,*,#8983,.F.);
#13191=ORIENTED_EDGE('',*,*,#8991,.T.);
#13192=ORIENTED_EDGE('',*,*,#8992,.T.);
#13193=ORIENTED_EDGE('',*,*,#8993,.T.);
#13194=ORIENTED_EDGE('',*,*,#8994,.T.);
#13195=ORIENTED_EDGE('',*,*,#8995,.T.);
#13196=ORIENTED_EDGE('',*,*,#8988,.F.);
#13197=ORIENTED_EDGE('',*,*,#8996,.T.);
#13198=ORIENTED_EDGE('',*,*,#8997,.T.);
#13199=ORIENTED_EDGE('',*,*,#8998,.T.);
#13200=ORIENTED_EDGE('',*,*,#8999,.T.);
#13201=ORIENTED_EDGE('',*,*,#9000,.T.);
#13202=ORIENTED_EDGE('',*,*,#8993,.F.);
#13203=ORIENTED_EDGE('',*,*,#9001,.T.);
#13204=ORIENTED_EDGE('',*,*,#9002,.T.);
#13205=ORIENTED_EDGE('',*,*,#9003,.T.);
#13206=ORIENTED_EDGE('',*,*,#9004,.T.);
#13207=ORIENTED_EDGE('',*,*,#9005,.T.);
#13208=ORIENTED_EDGE('',*,*,#8998,.F.);
#13209=ORIENTED_EDGE('',*,*,#9006,.T.);
#13210=ORIENTED_EDGE('',*,*,#9007,.T.);
#13211=ORIENTED_EDGE('',*,*,#9008,.T.);
#13212=ORIENTED_EDGE('',*,*,#9009,.T.);
#13213=ORIENTED_EDGE('',*,*,#9010,.T.);
#13214=ORIENTED_EDGE('',*,*,#9003,.F.);
#13215=ORIENTED_EDGE('',*,*,#9011,.T.);
#13216=ORIENTED_EDGE('',*,*,#9012,.T.);
#13217=ORIENTED_EDGE('',*,*,#9013,.T.);
#13218=ORIENTED_EDGE('',*,*,#9014,.T.);
#13219=ORIENTED_EDGE('',*,*,#9015,.T.);
#13220=ORIENTED_EDGE('',*,*,#9008,.F.);
#13221=ORIENTED_EDGE('',*,*,#9016,.T.);
#13222=ORIENTED_EDGE('',*,*,#9017,.T.);
#13223=ORIENTED_EDGE('',*,*,#9018,.T.);
#13224=ORIENTED_EDGE('',*,*,#9019,.T.);
#13225=ORIENTED_EDGE('',*,*,#9020,.T.);
#13226=ORIENTED_EDGE('',*,*,#9013,.F.);
#13227=ORIENTED_EDGE('',*,*,#9021,.T.);
#13228=ORIENTED_EDGE('',*,*,#9022,.T.);
#13229=ORIENTED_EDGE('',*,*,#9023,.F.);
#13230=ORIENTED_EDGE('',*,*,#9024,.T.);
#13231=ORIENTED_EDGE('',*,*,#9025,.T.);
#13232=ORIENTED_EDGE('',*,*,#9026,.F.);
#13233=ORIENTED_EDGE('',*,*,#9027,.T.);
#13234=ORIENTED_EDGE('',*,*,#9028,.T.);
#13235=ORIENTED_EDGE('',*,*,#9023,.T.);
#13236=ORIENTED_EDGE('',*,*,#9029,.T.);
#13237=ORIENTED_EDGE('',*,*,#9030,.T.);
#13238=ORIENTED_EDGE('',*,*,#9018,.F.);
#13239=ORIENTED_EDGE('',*,*,#9031,.T.);
#13240=ORIENTED_EDGE('',*,*,#9032,.T.);
#13241=ORIENTED_EDGE('',*,*,#9033,.F.);
#13242=ORIENTED_EDGE('',*,*,#9034,.F.);
#13243=ORIENTED_EDGE('',*,*,#9035,.T.);
#13244=ORIENTED_EDGE('',*,*,#9036,.T.);
#13245=ORIENTED_EDGE('',*,*,#9037,.T.);
#13246=ORIENTED_EDGE('',*,*,#9038,.T.);
#13247=ORIENTED_EDGE('',*,*,#9039,.T.);
#13248=ORIENTED_EDGE('',*,*,#9040,.T.);
#13249=ORIENTED_EDGE('',*,*,#9041,.T.);
#13250=ORIENTED_EDGE('',*,*,#9042,.T.);
#13251=ORIENTED_EDGE('',*,*,#9043,.T.);
#13252=ORIENTED_EDGE('',*,*,#9044,.T.);
#13253=ORIENTED_EDGE('',*,*,#9045,.T.);
#13254=ORIENTED_EDGE('',*,*,#9046,.T.);
#13255=ORIENTED_EDGE('',*,*,#9047,.T.);
#13256=ORIENTED_EDGE('',*,*,#9048,.T.);
#13257=ORIENTED_EDGE('',*,*,#9049,.T.);
#13258=ORIENTED_EDGE('',*,*,#9050,.T.);
#13259=ORIENTED_EDGE('',*,*,#9051,.T.);
#13260=ORIENTED_EDGE('',*,*,#9052,.T.);
#13261=ORIENTED_EDGE('',*,*,#9053,.T.);
#13262=ORIENTED_EDGE('',*,*,#9054,.T.);
#13263=ORIENTED_EDGE('',*,*,#9055,.T.);
#13264=ORIENTED_EDGE('',*,*,#9056,.T.);
#13265=ORIENTED_EDGE('',*,*,#9057,.T.);
#13266=ORIENTED_EDGE('',*,*,#9058,.T.);
#13267=ORIENTED_EDGE('',*,*,#9059,.T.);
#13268=ORIENTED_EDGE('',*,*,#9060,.T.);
#13269=ORIENTED_EDGE('',*,*,#9061,.T.);
#13270=ORIENTED_EDGE('',*,*,#9062,.T.);
#13271=ORIENTED_EDGE('',*,*,#9063,.T.);
#13272=ORIENTED_EDGE('',*,*,#9064,.T.);
#13273=ORIENTED_EDGE('',*,*,#9065,.T.);
#13274=ORIENTED_EDGE('',*,*,#9066,.T.);
#13275=ORIENTED_EDGE('',*,*,#9067,.T.);
#13276=ORIENTED_EDGE('',*,*,#9068,.T.);
#13277=ORIENTED_EDGE('',*,*,#9069,.T.);
#13278=ORIENTED_EDGE('',*,*,#9070,.T.);
#13279=ORIENTED_EDGE('',*,*,#9071,.T.);
#13280=ORIENTED_EDGE('',*,*,#9072,.T.);
#13281=ORIENTED_EDGE('',*,*,#9073,.T.);
#13282=ORIENTED_EDGE('',*,*,#9074,.T.);
#13283=ORIENTED_EDGE('',*,*,#9075,.T.);
#13284=ORIENTED_EDGE('',*,*,#9076,.T.);
#13285=ORIENTED_EDGE('',*,*,#9077,.F.);
#13286=ORIENTED_EDGE('',*,*,#9078,.F.);
#13287=ORIENTED_EDGE('',*,*,#9079,.F.);
#13288=ORIENTED_EDGE('',*,*,#9080,.F.);
#13289=ORIENTED_EDGE('',*,*,#9081,.F.);
#13290=ORIENTED_EDGE('',*,*,#9082,.F.);
#13291=ORIENTED_EDGE('',*,*,#9083,.F.);
#13292=ORIENTED_EDGE('',*,*,#9084,.F.);
#13293=ORIENTED_EDGE('',*,*,#9085,.F.);
#13294=ORIENTED_EDGE('',*,*,#9086,.F.);
#13295=ORIENTED_EDGE('',*,*,#9087,.F.);
#13296=ORIENTED_EDGE('',*,*,#9088,.F.);
#13297=ORIENTED_EDGE('',*,*,#9089,.F.);
#13298=ORIENTED_EDGE('',*,*,#9090,.F.);
#13299=ORIENTED_EDGE('',*,*,#9091,.F.);
#13300=ORIENTED_EDGE('',*,*,#9092,.F.);
#13301=ORIENTED_EDGE('',*,*,#9093,.F.);
#13302=ORIENTED_EDGE('',*,*,#9094,.F.);
#13303=ORIENTED_EDGE('',*,*,#9095,.F.);
#13304=ORIENTED_EDGE('',*,*,#9096,.F.);
#13305=ORIENTED_EDGE('',*,*,#9097,.F.);
#13306=ORIENTED_EDGE('',*,*,#9098,.F.);
#13307=ORIENTED_EDGE('',*,*,#9099,.F.);
#13308=ORIENTED_EDGE('',*,*,#9100,.F.);
#13309=ORIENTED_EDGE('',*,*,#9101,.F.);
#13310=ORIENTED_EDGE('',*,*,#9102,.F.);
#13311=ORIENTED_EDGE('',*,*,#9103,.F.);
#13312=ORIENTED_EDGE('',*,*,#9104,.F.);
#13313=ORIENTED_EDGE('',*,*,#9105,.F.);
#13314=ORIENTED_EDGE('',*,*,#9106,.F.);
#13315=ORIENTED_EDGE('',*,*,#9107,.F.);
#13316=ORIENTED_EDGE('',*,*,#9108,.F.);
#13317=ORIENTED_EDGE('',*,*,#9109,.F.);
#13318=ORIENTED_EDGE('',*,*,#9110,.F.);
#13319=ORIENTED_EDGE('',*,*,#9111,.F.);
#13320=ORIENTED_EDGE('',*,*,#9112,.F.);
#13321=ORIENTED_EDGE('',*,*,#9113,.F.);
#13322=ORIENTED_EDGE('',*,*,#9114,.F.);
#13323=ORIENTED_EDGE('',*,*,#9115,.F.);
#13324=ORIENTED_EDGE('',*,*,#9116,.F.);
#13325=ORIENTED_EDGE('',*,*,#9117,.F.);
#13326=ORIENTED_EDGE('',*,*,#9118,.F.);
#13327=ORIENTED_EDGE('',*,*,#9119,.T.);
#13328=ORIENTED_EDGE('',*,*,#9120,.F.);
#13329=ORIENTED_EDGE('',*,*,#9119,.F.);
#13330=ORIENTED_EDGE('',*,*,#9121,.T.);
#13331=ORIENTED_EDGE('',*,*,#9122,.F.);
#13332=ORIENTED_EDGE('',*,*,#9121,.F.);
#13333=ORIENTED_EDGE('',*,*,#9123,.F.);
#13334=ORIENTED_EDGE('',*,*,#9124,.T.);
#13335=ORIENTED_EDGE('',*,*,#9125,.F.);
#13336=ORIENTED_EDGE('',*,*,#9126,.F.);
#13337=ORIENTED_EDGE('',*,*,#9127,.F.);
#13338=ORIENTED_EDGE('',*,*,#9128,.F.);
#13339=ORIENTED_EDGE('',*,*,#9124,.F.);
#13340=ORIENTED_EDGE('',*,*,#9129,.F.);
#13341=ORIENTED_EDGE('',*,*,#9130,.F.);
#13342=ORIENTED_EDGE('',*,*,#9131,.F.);
#13343=ORIENTED_EDGE('',*,*,#9126,.T.);
#13344=ORIENTED_EDGE('',*,*,#9132,.F.);
#13345=ORIENTED_EDGE('',*,*,#9129,.T.);
#13346=ORIENTED_EDGE('',*,*,#9123,.T.);
#13347=ORIENTED_EDGE('',*,*,#9131,.T.);
#13348=ORIENTED_EDGE('',*,*,#9133,.T.);
#13349=ORIENTED_EDGE('',*,*,#9122,.T.);
#13350=ORIENTED_EDGE('',*,*,#8783,.F.);
#13351=ORIENTED_EDGE('',*,*,#9134,.T.);
#13352=ORIENTED_EDGE('',*,*,#9077,.T.);
#13353=ORIENTED_EDGE('',*,*,#9135,.T.);
#13354=ORIENTED_EDGE('',*,*,#8786,.F.);
#13355=ORIENTED_EDGE('',*,*,#9135,.F.);
#13356=ORIENTED_EDGE('',*,*,#9076,.F.);
#13357=ORIENTED_EDGE('',*,*,#9075,.F.);
#13358=ORIENTED_EDGE('',*,*,#9074,.F.);
#13359=ORIENTED_EDGE('',*,*,#9073,.F.);
#13360=ORIENTED_EDGE('',*,*,#9072,.F.);
#13361=ORIENTED_EDGE('',*,*,#9071,.F.);
#13362=ORIENTED_EDGE('',*,*,#9070,.F.);
#13363=ORIENTED_EDGE('',*,*,#9069,.F.);
#13364=ORIENTED_EDGE('',*,*,#9068,.F.);
#13365=ORIENTED_EDGE('',*,*,#9067,.F.);
#13366=ORIENTED_EDGE('',*,*,#9066,.F.);
#13367=ORIENTED_EDGE('',*,*,#9065,.F.);
#13368=ORIENTED_EDGE('',*,*,#9064,.F.);
#13369=ORIENTED_EDGE('',*,*,#9063,.F.);
#13370=ORIENTED_EDGE('',*,*,#9062,.F.);
#13371=ORIENTED_EDGE('',*,*,#9061,.F.);
#13372=ORIENTED_EDGE('',*,*,#9060,.F.);
#13373=ORIENTED_EDGE('',*,*,#9059,.F.);
#13374=ORIENTED_EDGE('',*,*,#9058,.F.);
#13375=ORIENTED_EDGE('',*,*,#9057,.F.);
#13376=ORIENTED_EDGE('',*,*,#9056,.F.);
#13377=ORIENTED_EDGE('',*,*,#9055,.F.);
#13378=ORIENTED_EDGE('',*,*,#9054,.F.);
#13379=ORIENTED_EDGE('',*,*,#9053,.F.);
#13380=ORIENTED_EDGE('',*,*,#9052,.F.);
#13381=ORIENTED_EDGE('',*,*,#9051,.F.);
#13382=ORIENTED_EDGE('',*,*,#9050,.F.);
#13383=ORIENTED_EDGE('',*,*,#9049,.F.);
#13384=ORIENTED_EDGE('',*,*,#9048,.F.);
#13385=ORIENTED_EDGE('',*,*,#9047,.F.);
#13386=ORIENTED_EDGE('',*,*,#9046,.F.);
#13387=ORIENTED_EDGE('',*,*,#9045,.F.);
#13388=ORIENTED_EDGE('',*,*,#9044,.F.);
#13389=ORIENTED_EDGE('',*,*,#9043,.F.);
#13390=ORIENTED_EDGE('',*,*,#9042,.F.);
#13391=ORIENTED_EDGE('',*,*,#9041,.F.);
#13392=ORIENTED_EDGE('',*,*,#9040,.F.);
#13393=ORIENTED_EDGE('',*,*,#9039,.F.);
#13394=ORIENTED_EDGE('',*,*,#9038,.F.);
#13395=ORIENTED_EDGE('',*,*,#9037,.F.);
#13396=ORIENTED_EDGE('',*,*,#9036,.F.);
#13397=ORIENTED_EDGE('',*,*,#9035,.F.);
#13398=ORIENTED_EDGE('',*,*,#9136,.F.);
#13399=ORIENTED_EDGE('',*,*,#9025,.F.);
#13400=ORIENTED_EDGE('',*,*,#9024,.F.);
#13401=ORIENTED_EDGE('',*,*,#9032,.F.);
#13402=ORIENTED_EDGE('',*,*,#9031,.F.);
#13403=ORIENTED_EDGE('',*,*,#9022,.F.);
#13404=ORIENTED_EDGE('',*,*,#9021,.F.);
#13405=ORIENTED_EDGE('',*,*,#9017,.F.);
#13406=ORIENTED_EDGE('',*,*,#9016,.F.);
#13407=ORIENTED_EDGE('',*,*,#9012,.F.);
#13408=ORIENTED_EDGE('',*,*,#9011,.F.);
#13409=ORIENTED_EDGE('',*,*,#9007,.F.);
#13410=ORIENTED_EDGE('',*,*,#9006,.F.);
#13411=ORIENTED_EDGE('',*,*,#9002,.F.);
#13412=ORIENTED_EDGE('',*,*,#9001,.F.);
#13413=ORIENTED_EDGE('',*,*,#8997,.F.);
#13414=ORIENTED_EDGE('',*,*,#8996,.F.);
#13415=ORIENTED_EDGE('',*,*,#8992,.F.);
#13416=ORIENTED_EDGE('',*,*,#8991,.F.);
#13417=ORIENTED_EDGE('',*,*,#8987,.F.);
#13418=ORIENTED_EDGE('',*,*,#8986,.F.);
#13419=ORIENTED_EDGE('',*,*,#8982,.F.);
#13420=ORIENTED_EDGE('',*,*,#8981,.F.);
#13421=ORIENTED_EDGE('',*,*,#8977,.F.);
#13422=ORIENTED_EDGE('',*,*,#8976,.F.);
#13423=ORIENTED_EDGE('',*,*,#8972,.F.);
#13424=ORIENTED_EDGE('',*,*,#8971,.F.);
#13425=ORIENTED_EDGE('',*,*,#8967,.F.);
#13426=ORIENTED_EDGE('',*,*,#8966,.F.);
#13427=ORIENTED_EDGE('',*,*,#8962,.F.);
#13428=ORIENTED_EDGE('',*,*,#8961,.F.);
#13429=ORIENTED_EDGE('',*,*,#8957,.F.);
#13430=ORIENTED_EDGE('',*,*,#8956,.F.);
#13431=ORIENTED_EDGE('',*,*,#8952,.F.);
#13432=ORIENTED_EDGE('',*,*,#8951,.F.);
#13433=ORIENTED_EDGE('',*,*,#8947,.F.);
#13434=ORIENTED_EDGE('',*,*,#8946,.F.);
#13435=ORIENTED_EDGE('',*,*,#8942,.F.);
#13436=ORIENTED_EDGE('',*,*,#8941,.F.);
#13437=ORIENTED_EDGE('',*,*,#8937,.F.);
#13438=ORIENTED_EDGE('',*,*,#8936,.F.);
#13439=ORIENTED_EDGE('',*,*,#8932,.F.);
#13440=ORIENTED_EDGE('',*,*,#8931,.F.);
#13441=ORIENTED_EDGE('',*,*,#8927,.F.);
#13442=ORIENTED_EDGE('',*,*,#8926,.F.);
#13443=ORIENTED_EDGE('',*,*,#8922,.F.);
#13444=ORIENTED_EDGE('',*,*,#8921,.F.);
#13445=ORIENTED_EDGE('',*,*,#8917,.F.);
#13446=ORIENTED_EDGE('',*,*,#8916,.F.);
#13447=ORIENTED_EDGE('',*,*,#8912,.F.);
#13448=ORIENTED_EDGE('',*,*,#8911,.F.);
#13449=ORIENTED_EDGE('',*,*,#8907,.F.);
#13450=ORIENTED_EDGE('',*,*,#8906,.F.);
#13451=ORIENTED_EDGE('',*,*,#8902,.F.);
#13452=ORIENTED_EDGE('',*,*,#8901,.F.);
#13453=ORIENTED_EDGE('',*,*,#8897,.F.);
#13454=ORIENTED_EDGE('',*,*,#8896,.F.);
#13455=ORIENTED_EDGE('',*,*,#8892,.F.);
#13456=ORIENTED_EDGE('',*,*,#8891,.F.);
#13457=ORIENTED_EDGE('',*,*,#8887,.F.);
#13458=ORIENTED_EDGE('',*,*,#8886,.F.);
#13459=ORIENTED_EDGE('',*,*,#8882,.F.);
#13460=ORIENTED_EDGE('',*,*,#8881,.F.);
#13461=ORIENTED_EDGE('',*,*,#8877,.F.);
#13462=ORIENTED_EDGE('',*,*,#8876,.F.);
#13463=ORIENTED_EDGE('',*,*,#8872,.F.);
#13464=ORIENTED_EDGE('',*,*,#8871,.F.);
#13465=ORIENTED_EDGE('',*,*,#8867,.F.);
#13466=ORIENTED_EDGE('',*,*,#8866,.F.);
#13467=ORIENTED_EDGE('',*,*,#8862,.F.);
#13468=ORIENTED_EDGE('',*,*,#8861,.F.);
#13469=ORIENTED_EDGE('',*,*,#8857,.F.);
#13470=ORIENTED_EDGE('',*,*,#8856,.F.);
#13471=ORIENTED_EDGE('',*,*,#8852,.F.);
#13472=ORIENTED_EDGE('',*,*,#8851,.F.);
#13473=ORIENTED_EDGE('',*,*,#8847,.F.);
#13474=ORIENTED_EDGE('',*,*,#8846,.F.);
#13475=ORIENTED_EDGE('',*,*,#8842,.F.);
#13476=ORIENTED_EDGE('',*,*,#8841,.F.);
#13477=ORIENTED_EDGE('',*,*,#8837,.F.);
#13478=ORIENTED_EDGE('',*,*,#8836,.F.);
#13479=ORIENTED_EDGE('',*,*,#8832,.F.);
#13480=ORIENTED_EDGE('',*,*,#8831,.F.);
#13481=ORIENTED_EDGE('',*,*,#8827,.F.);
#13482=ORIENTED_EDGE('',*,*,#8826,.F.);
#13483=ORIENTED_EDGE('',*,*,#8822,.F.);
#13484=ORIENTED_EDGE('',*,*,#8821,.F.);
#13485=ORIENTED_EDGE('',*,*,#8817,.F.);
#13486=ORIENTED_EDGE('',*,*,#8816,.F.);
#13487=ORIENTED_EDGE('',*,*,#8812,.F.);
#13488=ORIENTED_EDGE('',*,*,#8811,.F.);
#13489=ORIENTED_EDGE('',*,*,#8807,.F.);
#13490=ORIENTED_EDGE('',*,*,#8806,.F.);
#13491=ORIENTED_EDGE('',*,*,#8802,.F.);
#13492=ORIENTED_EDGE('',*,*,#8801,.F.);
#13493=ORIENTED_EDGE('',*,*,#8797,.F.);
#13494=ORIENTED_EDGE('',*,*,#8796,.F.);
#13495=ORIENTED_EDGE('',*,*,#8792,.F.);
#13496=ORIENTED_EDGE('',*,*,#8791,.F.);
#13497=ORIENTED_EDGE('',*,*,#8787,.F.);
#13498=ORIENTED_EDGE('',*,*,#9134,.F.);
#13499=ORIENTED_EDGE('',*,*,#8782,.F.);
#13500=ORIENTED_EDGE('',*,*,#8790,.F.);
#13501=ORIENTED_EDGE('',*,*,#8789,.F.);
#13502=ORIENTED_EDGE('',*,*,#8795,.F.);
#13503=ORIENTED_EDGE('',*,*,#8794,.F.);
#13504=ORIENTED_EDGE('',*,*,#8800,.F.);
#13505=ORIENTED_EDGE('',*,*,#8799,.F.);
#13506=ORIENTED_EDGE('',*,*,#8805,.F.);
#13507=ORIENTED_EDGE('',*,*,#8804,.F.);
#13508=ORIENTED_EDGE('',*,*,#8810,.F.);
#13509=ORIENTED_EDGE('',*,*,#8809,.F.);
#13510=ORIENTED_EDGE('',*,*,#8815,.F.);
#13511=ORIENTED_EDGE('',*,*,#8814,.F.);
#13512=ORIENTED_EDGE('',*,*,#8820,.F.);
#13513=ORIENTED_EDGE('',*,*,#8819,.F.);
#13514=ORIENTED_EDGE('',*,*,#8825,.F.);
#13515=ORIENTED_EDGE('',*,*,#8824,.F.);
#13516=ORIENTED_EDGE('',*,*,#8830,.F.);
#13517=ORIENTED_EDGE('',*,*,#8829,.F.);
#13518=ORIENTED_EDGE('',*,*,#8835,.F.);
#13519=ORIENTED_EDGE('',*,*,#8834,.F.);
#13520=ORIENTED_EDGE('',*,*,#8840,.F.);
#13521=ORIENTED_EDGE('',*,*,#8839,.F.);
#13522=ORIENTED_EDGE('',*,*,#8845,.F.);
#13523=ORIENTED_EDGE('',*,*,#8844,.F.);
#13524=ORIENTED_EDGE('',*,*,#8850,.F.);
#13525=ORIENTED_EDGE('',*,*,#8849,.F.);
#13526=ORIENTED_EDGE('',*,*,#8855,.F.);
#13527=ORIENTED_EDGE('',*,*,#8854,.F.);
#13528=ORIENTED_EDGE('',*,*,#8860,.F.);
#13529=ORIENTED_EDGE('',*,*,#8859,.F.);
#13530=ORIENTED_EDGE('',*,*,#8865,.F.);
#13531=ORIENTED_EDGE('',*,*,#8864,.F.);
#13532=ORIENTED_EDGE('',*,*,#8870,.F.);
#13533=ORIENTED_EDGE('',*,*,#8869,.F.);
#13534=ORIENTED_EDGE('',*,*,#8875,.F.);
#13535=ORIENTED_EDGE('',*,*,#8874,.F.);
#13536=ORIENTED_EDGE('',*,*,#8880,.F.);
#13537=ORIENTED_EDGE('',*,*,#8879,.F.);
#13538=ORIENTED_EDGE('',*,*,#8885,.F.);
#13539=ORIENTED_EDGE('',*,*,#8884,.F.);
#13540=ORIENTED_EDGE('',*,*,#8890,.F.);
#13541=ORIENTED_EDGE('',*,*,#8889,.F.);
#13542=ORIENTED_EDGE('',*,*,#8895,.F.);
#13543=ORIENTED_EDGE('',*,*,#8894,.F.);
#13544=ORIENTED_EDGE('',*,*,#8900,.F.);
#13545=ORIENTED_EDGE('',*,*,#8899,.F.);
#13546=ORIENTED_EDGE('',*,*,#8905,.F.);
#13547=ORIENTED_EDGE('',*,*,#8904,.F.);
#13548=ORIENTED_EDGE('',*,*,#8910,.F.);
#13549=ORIENTED_EDGE('',*,*,#8909,.F.);
#13550=ORIENTED_EDGE('',*,*,#8915,.F.);
#13551=ORIENTED_EDGE('',*,*,#8914,.F.);
#13552=ORIENTED_EDGE('',*,*,#8920,.F.);
#13553=ORIENTED_EDGE('',*,*,#8919,.F.);
#13554=ORIENTED_EDGE('',*,*,#8925,.F.);
#13555=ORIENTED_EDGE('',*,*,#8924,.F.);
#13556=ORIENTED_EDGE('',*,*,#8930,.F.);
#13557=ORIENTED_EDGE('',*,*,#8929,.F.);
#13558=ORIENTED_EDGE('',*,*,#8935,.F.);
#13559=ORIENTED_EDGE('',*,*,#8934,.F.);
#13560=ORIENTED_EDGE('',*,*,#8940,.F.);
#13561=ORIENTED_EDGE('',*,*,#8939,.F.);
#13562=ORIENTED_EDGE('',*,*,#8945,.F.);
#13563=ORIENTED_EDGE('',*,*,#8944,.F.);
#13564=ORIENTED_EDGE('',*,*,#8950,.F.);
#13565=ORIENTED_EDGE('',*,*,#8949,.F.);
#13566=ORIENTED_EDGE('',*,*,#8955,.F.);
#13567=ORIENTED_EDGE('',*,*,#8954,.F.);
#13568=ORIENTED_EDGE('',*,*,#8960,.F.);
#13569=ORIENTED_EDGE('',*,*,#8959,.F.);
#13570=ORIENTED_EDGE('',*,*,#8965,.F.);
#13571=ORIENTED_EDGE('',*,*,#8964,.F.);
#13572=ORIENTED_EDGE('',*,*,#8970,.F.);
#13573=ORIENTED_EDGE('',*,*,#8969,.F.);
#13574=ORIENTED_EDGE('',*,*,#8975,.F.);
#13575=ORIENTED_EDGE('',*,*,#8974,.F.);
#13576=ORIENTED_EDGE('',*,*,#8980,.F.);
#13577=ORIENTED_EDGE('',*,*,#8979,.F.);
#13578=ORIENTED_EDGE('',*,*,#8985,.F.);
#13579=ORIENTED_EDGE('',*,*,#8984,.F.);
#13580=ORIENTED_EDGE('',*,*,#8990,.F.);
#13581=ORIENTED_EDGE('',*,*,#8989,.F.);
#13582=ORIENTED_EDGE('',*,*,#8995,.F.);
#13583=ORIENTED_EDGE('',*,*,#8994,.F.);
#13584=ORIENTED_EDGE('',*,*,#9000,.F.);
#13585=ORIENTED_EDGE('',*,*,#8999,.F.);
#13586=ORIENTED_EDGE('',*,*,#9005,.F.);
#13587=ORIENTED_EDGE('',*,*,#9004,.F.);
#13588=ORIENTED_EDGE('',*,*,#9010,.F.);
#13589=ORIENTED_EDGE('',*,*,#9009,.F.);
#13590=ORIENTED_EDGE('',*,*,#9015,.F.);
#13591=ORIENTED_EDGE('',*,*,#9014,.F.);
#13592=ORIENTED_EDGE('',*,*,#9020,.F.);
#13593=ORIENTED_EDGE('',*,*,#9019,.F.);
#13594=ORIENTED_EDGE('',*,*,#9030,.F.);
#13595=ORIENTED_EDGE('',*,*,#9029,.F.);
#13596=ORIENTED_EDGE('',*,*,#9028,.F.);
#13597=ORIENTED_EDGE('',*,*,#9027,.F.);
#13598=ORIENTED_EDGE('',*,*,#9137,.F.);
#13599=ORIENTED_EDGE('',*,*,#9033,.T.);
#13600=ORIENTED_EDGE('',*,*,#9118,.T.);
#13601=ORIENTED_EDGE('',*,*,#9117,.T.);
#13602=ORIENTED_EDGE('',*,*,#9116,.T.);
#13603=ORIENTED_EDGE('',*,*,#9115,.T.);
#13604=ORIENTED_EDGE('',*,*,#9114,.T.);
#13605=ORIENTED_EDGE('',*,*,#9113,.T.);
#13606=ORIENTED_EDGE('',*,*,#9112,.T.);
#13607=ORIENTED_EDGE('',*,*,#9111,.T.);
#13608=ORIENTED_EDGE('',*,*,#9110,.T.);
#13609=ORIENTED_EDGE('',*,*,#9109,.T.);
#13610=ORIENTED_EDGE('',*,*,#9108,.T.);
#13611=ORIENTED_EDGE('',*,*,#9107,.T.);
#13612=ORIENTED_EDGE('',*,*,#9106,.T.);
#13613=ORIENTED_EDGE('',*,*,#9105,.T.);
#13614=ORIENTED_EDGE('',*,*,#9104,.T.);
#13615=ORIENTED_EDGE('',*,*,#9103,.T.);
#13616=ORIENTED_EDGE('',*,*,#9102,.T.);
#13617=ORIENTED_EDGE('',*,*,#9101,.T.);
#13618=ORIENTED_EDGE('',*,*,#9100,.T.);
#13619=ORIENTED_EDGE('',*,*,#9099,.T.);
#13620=ORIENTED_EDGE('',*,*,#9098,.T.);
#13621=ORIENTED_EDGE('',*,*,#9097,.T.);
#13622=ORIENTED_EDGE('',*,*,#9096,.T.);
#13623=ORIENTED_EDGE('',*,*,#9095,.T.);
#13624=ORIENTED_EDGE('',*,*,#9094,.T.);
#13625=ORIENTED_EDGE('',*,*,#9093,.T.);
#13626=ORIENTED_EDGE('',*,*,#9092,.T.);
#13627=ORIENTED_EDGE('',*,*,#9091,.T.);
#13628=ORIENTED_EDGE('',*,*,#9090,.T.);
#13629=ORIENTED_EDGE('',*,*,#9089,.T.);
#13630=ORIENTED_EDGE('',*,*,#9088,.T.);
#13631=ORIENTED_EDGE('',*,*,#9087,.T.);
#13632=ORIENTED_EDGE('',*,*,#9086,.T.);
#13633=ORIENTED_EDGE('',*,*,#9085,.T.);
#13634=ORIENTED_EDGE('',*,*,#9084,.T.);
#13635=ORIENTED_EDGE('',*,*,#9083,.T.);
#13636=ORIENTED_EDGE('',*,*,#9082,.T.);
#13637=ORIENTED_EDGE('',*,*,#9081,.T.);
#13638=ORIENTED_EDGE('',*,*,#9080,.T.);
#13639=ORIENTED_EDGE('',*,*,#9079,.T.);
#13640=ORIENTED_EDGE('',*,*,#9078,.T.);
#13641=ORIENTED_EDGE('',*,*,#8785,.F.);
#13642=ORIENTED_EDGE('',*,*,#9138,.F.);
#13643=ORIENTED_EDGE('',*,*,#9138,.T.);
#13644=ORIENTED_EDGE('',*,*,#9139,.T.);
#13645=ORIENTED_EDGE('',*,*,#9120,.T.);
#13646=ORIENTED_EDGE('',*,*,#9139,.F.);
#13647=ORIENTED_EDGE('',*,*,#9127,.T.);
#13648=ORIENTED_EDGE('',*,*,#9133,.F.);
#13649=ORIENTED_EDGE('',*,*,#9130,.T.);
#13650=ORIENTED_EDGE('',*,*,#9140,.T.);
#13651=ORIENTED_EDGE('',*,*,#9128,.T.);
#13652=ORIENTED_EDGE('',*,*,#9140,.F.);
#13653=ORIENTED_EDGE('',*,*,#9132,.T.);
#13654=ORIENTED_EDGE('',*,*,#9125,.T.);
#13655=ORIENTED_EDGE('',*,*,#9137,.T.);
#13656=ORIENTED_EDGE('',*,*,#9026,.T.);
#13657=ORIENTED_EDGE('',*,*,#9136,.T.);
#13658=ORIENTED_EDGE('',*,*,#9034,.T.);
#15984=CYLINDRICAL_SURFACE('',#17451,7.01125);
#15985=CYLINDRICAL_SURFACE('',#17455,7.01125);
#15986=CYLINDRICAL_SURFACE('',#17456,7.01125);
#15987=CYLINDRICAL_SURFACE('',#17457,7.01125);
#15988=CYLINDRICAL_SURFACE('',#17458,7.01125);
#15989=CYLINDRICAL_SURFACE('',#17459,7.01125);
#15990=CYLINDRICAL_SURFACE('',#17460,7.01125);
#15991=CYLINDRICAL_SURFACE('',#17461,7.01125);
#15992=CYLINDRICAL_SURFACE('',#17462,7.01125);
#15993=CYLINDRICAL_SURFACE('',#17463,7.01125);
#15994=CYLINDRICAL_SURFACE('',#17464,7.01125);
#15995=CYLINDRICAL_SURFACE('',#17465,7.01125);
#15996=CYLINDRICAL_SURFACE('',#17466,7.01125);
#15997=CYLINDRICAL_SURFACE('',#17467,7.01125);
#15998=CYLINDRICAL_SURFACE('',#17468,7.01125);
#15999=CYLINDRICAL_SURFACE('',#17469,7.01125);
#16000=CYLINDRICAL_SURFACE('',#17470,7.01125);
#16001=CYLINDRICAL_SURFACE('',#17471,7.01125);
#16002=CYLINDRICAL_SURFACE('',#17472,7.01125);
#16003=CYLINDRICAL_SURFACE('',#17473,7.01125);
#16004=CYLINDRICAL_SURFACE('',#17474,7.01125);
#16005=CYLINDRICAL_SURFACE('',#17475,7.01125);
#16006=CYLINDRICAL_SURFACE('',#17476,7.01125);
#16007=CYLINDRICAL_SURFACE('',#17477,7.01125);
#16008=CYLINDRICAL_SURFACE('',#17478,7.01125);
#16009=CYLINDRICAL_SURFACE('',#17479,7.01125);
#16010=CYLINDRICAL_SURFACE('',#17480,7.01125);
#16011=CYLINDRICAL_SURFACE('',#17481,7.01125);
#16012=CYLINDRICAL_SURFACE('',#17482,7.01125);
#16013=CYLINDRICAL_SURFACE('',#17483,7.01125);
#16014=CYLINDRICAL_SURFACE('',#17484,7.01125);
#16015=CYLINDRICAL_SURFACE('',#17485,7.01125);
#16016=CYLINDRICAL_SURFACE('',#17486,7.01125);
#16017=CYLINDRICAL_SURFACE('',#17487,7.01125);
#16018=CYLINDRICAL_SURFACE('',#17488,7.01125);
#16019=CYLINDRICAL_SURFACE('',#17489,7.01125);
#16020=CYLINDRICAL_SURFACE('',#17490,7.01125);
#16021=CYLINDRICAL_SURFACE('',#17491,7.01125);
#16022=CYLINDRICAL_SURFACE('',#17492,7.01125);
#16023=CYLINDRICAL_SURFACE('',#17493,7.01125);
#16024=CYLINDRICAL_SURFACE('',#17494,7.01125);
#16025=CYLINDRICAL_SURFACE('',#17495,7.01125);
#16026=CYLINDRICAL_SURFACE('',#17496,7.01125);
#16027=CYLINDRICAL_SURFACE('',#17497,7.01125);
#16028=CYLINDRICAL_SURFACE('',#17498,7.01125);
#16029=CYLINDRICAL_SURFACE('',#17499,7.01125);
#16030=CYLINDRICAL_SURFACE('',#17500,7.01125);
#16031=CYLINDRICAL_SURFACE('',#17501,7.01125);
#16032=CYLINDRICAL_SURFACE('',#17502,7.01125);
#16033=CYLINDRICAL_SURFACE('',#17504,7.01125);
#16034=CYLINDRICAL_SURFACE('',#17505,8.12525);
#16035=CYLINDRICAL_SURFACE('',#17521,4.);
#16036=CYLINDRICAL_SURFACE('',#17522,20.);
#16537=ADVANCED_FACE('',(#769),#15984,.F.);
#16538=ADVANCED_FACE('',(#770),#15985,.F.);
#16539=ADVANCED_FACE('',(#771),#15986,.F.);
#16540=ADVANCED_FACE('',(#772),#15987,.F.);
#16541=ADVANCED_FACE('',(#773),#15988,.F.);
#16542=ADVANCED_FACE('',(#774),#15989,.F.);
#16543=ADVANCED_FACE('',(#775),#15990,.F.);
#16544=ADVANCED_FACE('',(#776),#15991,.F.);
#16545=ADVANCED_FACE('',(#777),#15992,.F.);
#16546=ADVANCED_FACE('',(#778),#15993,.F.);
#16547=ADVANCED_FACE('',(#779),#15994,.F.);
#16548=ADVANCED_FACE('',(#780),#15995,.F.);
#16549=ADVANCED_FACE('',(#781),#15996,.F.);
#16550=ADVANCED_FACE('',(#782),#15997,.F.);
#16551=ADVANCED_FACE('',(#783),#15998,.F.);
#16552=ADVANCED_FACE('',(#784),#15999,.F.);
#16553=ADVANCED_FACE('',(#785),#16000,.F.);
#16554=ADVANCED_FACE('',(#786),#16001,.F.);
#16555=ADVANCED_FACE('',(#787),#16002,.F.);
#16556=ADVANCED_FACE('',(#788),#16003,.F.);
#16557=ADVANCED_FACE('',(#789),#16004,.F.);
#16558=ADVANCED_FACE('',(#790),#16005,.F.);
#16559=ADVANCED_FACE('',(#791),#16006,.F.);
#16560=ADVANCED_FACE('',(#792),#16007,.F.);
#16561=ADVANCED_FACE('',(#793),#16008,.F.);
#16562=ADVANCED_FACE('',(#794),#16009,.F.);
#16563=ADVANCED_FACE('',(#795),#16010,.F.);
#16564=ADVANCED_FACE('',(#796),#16011,.F.);
#16565=ADVANCED_FACE('',(#797),#16012,.F.);
#16566=ADVANCED_FACE('',(#798),#16013,.F.);
#16567=ADVANCED_FACE('',(#799),#16014,.F.);
#16568=ADVANCED_FACE('',(#800),#16015,.F.);
#16569=ADVANCED_FACE('',(#801),#16016,.F.);
#16570=ADVANCED_FACE('',(#802),#16017,.F.);
#16571=ADVANCED_FACE('',(#803),#16018,.F.);
#16572=ADVANCED_FACE('',(#804),#16019,.F.);
#16573=ADVANCED_FACE('',(#805),#16020,.F.);
#16574=ADVANCED_FACE('',(#806),#16021,.F.);
#16575=ADVANCED_FACE('',(#807),#16022,.F.);
#16576=ADVANCED_FACE('',(#808),#16023,.F.);
#16577=ADVANCED_FACE('',(#809),#16024,.F.);
#16578=ADVANCED_FACE('',(#810),#16025,.F.);
#16579=ADVANCED_FACE('',(#811),#16026,.F.);
#16580=ADVANCED_FACE('',(#812),#16027,.F.);
#16581=ADVANCED_FACE('',(#813),#16028,.F.);
#16582=ADVANCED_FACE('',(#814),#16029,.F.);
#16583=ADVANCED_FACE('',(#815),#16030,.F.);
#16584=ADVANCED_FACE('',(#816),#16031,.F.);
#16585=ADVANCED_FACE('',(#817),#16032,.F.);
#16586=ADVANCED_FACE('',(#818),#16033,.F.);
#16587=ADVANCED_FACE('',(#819),#16034,.F.);
#16588=ADVANCED_FACE('',(#820,#218),#344,.F.);
#16589=ADVANCED_FACE('',(#821),#111,.F.);
#16590=ADVANCED_FACE('',(#822),#345,.F.);
#16591=ADVANCED_FACE('',(#823),#346,.F.);
#16592=ADVANCED_FACE('',(#824),#347,.F.);
#16593=ADVANCED_FACE('',(#825,#219),#348,.T.);
#16594=ADVANCED_FACE('',(#826),#349,.F.);
#16595=ADVANCED_FACE('',(#827),#293,.F.);
#16596=ADVANCED_FACE('',(#828),#294,.F.);
#16597=ADVANCED_FACE('',(#829,#220),#350,.F.);
#16598=ADVANCED_FACE('',(#830),#16035,.F.);
#16599=ADVANCED_FACE('',(#831),#16036,.T.);
#16600=ADVANCED_FACE('',(#832,#221),#351,.F.);
#16844=CLOSED_SHELL('',(#16537,#16538,#16539,#16540,#16541,#16542,#16543,
#16544,#16545,#16546,#16547,#16548,#16549,#16550,#16551,#16552,#16553,#16554,
#16555,#16556,#16557,#16558,#16559,#16560,#16561,#16562,#16563,#16564,#16565,
#16566,#16567,#16568,#16569,#16570,#16571,#16572,#16573,#16574,#16575,#16576,
#16577,#16578,#16579,#16580,#16581,#16582,#16583,#16584,#16585,#16586,#16587,
#16588,#16589,#16590,#16591,#16592,#16593,#16594,#16595,#16596,#16597,#16598,
#16599,#16600));
#17450=AXIS2_PLACEMENT_3D('',#136539,#19020,#19021);
#17451=AXIS2_PLACEMENT_3D('',#136540,#19022,#19023);
#17452=AXIS2_PLACEMENT_3D('',#136685,#19025,#19026);
#17453=AXIS2_PLACEMENT_3D('',#136688,#19028,#19029);
#17454=AXIS2_PLACEMENT_3D('',#136690,#19030,#19031);
#17455=AXIS2_PLACEMENT_3D('',#136899,#19032,#19033);
#17456=AXIS2_PLACEMENT_3D('',#137407,#19035,#19036);
#17457=AXIS2_PLACEMENT_3D('',#137918,#19038,#19039);
#17458=AXIS2_PLACEMENT_3D('',#138411,#19041,#19042);
#17459=AXIS2_PLACEMENT_3D('',#138919,#19044,#19045);
#17460=AXIS2_PLACEMENT_3D('',#139430,#19047,#19048);
#17461=AXIS2_PLACEMENT_3D('',#139938,#19050,#19051);
#17462=AXIS2_PLACEMENT_3D('',#140449,#19053,#19054);
#17463=AXIS2_PLACEMENT_3D('',#140957,#19056,#19057);
#17464=AXIS2_PLACEMENT_3D('',#141471,#19059,#19060);
#17465=AXIS2_PLACEMENT_3D('',#141964,#19062,#19063);
#17466=AXIS2_PLACEMENT_3D('',#142472,#19065,#19066);
#17467=AXIS2_PLACEMENT_3D('',#142980,#19068,#19069);
#17468=AXIS2_PLACEMENT_3D('',#143476,#19071,#19072);
#17469=AXIS2_PLACEMENT_3D('',#143990,#19074,#19075);
#17470=AXIS2_PLACEMENT_3D('',#144498,#19077,#19078);
#17471=AXIS2_PLACEMENT_3D('',#145012,#19080,#19081);
#17472=AXIS2_PLACEMENT_3D('',#145523,#19083,#19084);
#17473=AXIS2_PLACEMENT_3D('',#146031,#19086,#19087);
#17474=AXIS2_PLACEMENT_3D('',#146545,#19089,#19090);
#17475=AXIS2_PLACEMENT_3D('',#147035,#19092,#19093);
#17476=AXIS2_PLACEMENT_3D('',#147546,#19095,#19096);
#17477=AXIS2_PLACEMENT_3D('',#148057,#19098,#19099);
#17478=AXIS2_PLACEMENT_3D('',#148547,#19101,#19102);
#17479=AXIS2_PLACEMENT_3D('',#149046,#19104,#19105);
#17480=AXIS2_PLACEMENT_3D('',#149563,#19107,#19108);
#17481=AXIS2_PLACEMENT_3D('',#150056,#19110,#19111);
#17482=AXIS2_PLACEMENT_3D('',#150570,#19113,#19114);
#17483=AXIS2_PLACEMENT_3D('',#151081,#19116,#19117);
#17484=AXIS2_PLACEMENT_3D('',#151580,#19119,#19120);
#17485=AXIS2_PLACEMENT_3D('',#152085,#19122,#19123);
#17486=AXIS2_PLACEMENT_3D('',#152593,#19125,#19126);
#17487=AXIS2_PLACEMENT_3D('',#153107,#19128,#19129);
#17488=AXIS2_PLACEMENT_3D('',#153621,#19131,#19132);
#17489=AXIS2_PLACEMENT_3D('',#154135,#19134,#19135);
#17490=AXIS2_PLACEMENT_3D('',#154637,#19137,#19138);
#17491=AXIS2_PLACEMENT_3D('',#155130,#19140,#19141);
#17492=AXIS2_PLACEMENT_3D('',#155641,#19143,#19144);
#17493=AXIS2_PLACEMENT_3D('',#156152,#19146,#19147);
#17494=AXIS2_PLACEMENT_3D('',#156645,#19149,#19150);
#17495=AXIS2_PLACEMENT_3D('',#157150,#19152,#19153);
#17496=AXIS2_PLACEMENT_3D('',#157664,#19155,#19156);
#17497=AXIS2_PLACEMENT_3D('',#158178,#19158,#19159);
#17498=AXIS2_PLACEMENT_3D('',#158689,#19161,#19162);
#17499=AXIS2_PLACEMENT_3D('',#159200,#19164,#19165);
#17500=AXIS2_PLACEMENT_3D('',#159708,#19167,#19168);
#17501=AXIS2_PLACEMENT_3D('',#160201,#19170,#19171);
#17502=AXIS2_PLACEMENT_3D('',#160709,#19173,#19174);
#17503=AXIS2_PLACEMENT_3D('',#160883,#19176,#19177);
#17504=AXIS2_PLACEMENT_3D('',#161121,#19178,#19179);
#17505=AXIS2_PLACEMENT_3D('',#161629,#19180,#19181);
#17506=AXIS2_PLACEMENT_3D('',#161688,#19182,#19183);
#17507=AXIS2_PLACEMENT_3D('',#170989,#19184,#19185);
#17508=AXIS2_PLACEMENT_3D('',#180353,#19186,#19187);
#17509=AXIS2_PLACEMENT_3D('',#180355,#19188,#19189);
#17510=AXIS2_PLACEMENT_3D('',#180357,#19190,#19191);
#17511=AXIS2_PLACEMENT_3D('',#180358,#19192,#19193);
#17512=AXIS2_PLACEMENT_3D('',#180361,#19195,#19196);
#17513=AXIS2_PLACEMENT_3D('',#180362,#19197,#19198);
#17514=AXIS2_PLACEMENT_3D('',#180371,#19203,#19204);
#17515=AXIS2_PLACEMENT_3D('',#180377,#19208,#19209);
#17516=AXIS2_PLACEMENT_3D('',#180383,#19213,#19214);
#17517=AXIS2_PLACEMENT_3D('',#180384,#19215,#19216);
#17518=AXIS2_PLACEMENT_3D('',#180385,#19217,#19218);
#17519=AXIS2_PLACEMENT_3D('',#185138,#19219,#19220);
#17520=AXIS2_PLACEMENT_3D('',#185140,#19221,#19222);
#17521=AXIS2_PLACEMENT_3D('',#185141,#19223,#19224);
#17522=AXIS2_PLACEMENT_3D('',#185143,#19226,#19227);
#17523=AXIS2_PLACEMENT_3D('',#185144,#19228,#19229);
#17524=AXIS2_PLACEMENT_3D('',#185145,#19230,#19231);
#19020=DIRECTION('axis',(0.,0.,1.));
#19021=DIRECTION('refdir',(1.,0.,0.));
#19022=DIRECTION('center_axis',(0.,0.,1.));
#19023=DIRECTION('ref_axis',(-0.937223598005796,-0.348729017062059,0.));
#19024=DIRECTION('',(0.,0.,1.));
#19025=DIRECTION('center_axis',(0.,0.,-1.));
#19026=DIRECTION('ref_axis',(-1.,0.,0.));
#19027=DIRECTION('',(0.,0.,1.));
#19028=DIRECTION('center_axis',(0.,0.,-1.));
#19029=DIRECTION('ref_axis',(-1.,0.,0.));
#19030=DIRECTION('center_axis',(0.,0.,-1.));
#19031=DIRECTION('ref_axis',(-1.,0.,0.));
#19032=DIRECTION('center_axis',(0.,0.,1.));
#19033=DIRECTION('ref_axis',(-0.937223598005796,-0.348729017062059,0.));
#19034=DIRECTION('',(0.,0.,1.));
#19035=DIRECTION('center_axis',(0.,0.,1.));
#19036=DIRECTION('ref_axis',(-0.937223598005796,-0.348729017062059,0.));
#19037=DIRECTION('',(0.,0.,1.));
#19038=DIRECTION('center_axis',(0.,0.,1.));
#19039=DIRECTION('ref_axis',(-0.937223598005796,-0.348729017062059,0.));
#19040=DIRECTION('',(0.,0.,1.));
#19041=DIRECTION('center_axis',(0.,0.,1.));
#19042=DIRECTION('ref_axis',(-0.937223598005796,-0.348729017062059,0.));
#19043=DIRECTION('',(0.,0.,1.));
#19044=DIRECTION('center_axis',(0.,0.,1.));
#19045=DIRECTION('ref_axis',(-0.937223598005796,-0.348729017062059,0.));
#19046=DIRECTION('',(0.,0.,1.));
#19047=DIRECTION('center_axis',(0.,0.,1.));
#19048=DIRECTION('ref_axis',(-0.937223598005796,-0.348729017062059,0.));
#19049=DIRECTION('',(0.,0.,1.));
#19050=DIRECTION('center_axis',(0.,0.,1.));
#19051=DIRECTION('ref_axis',(-0.937223598005796,-0.348729017062059,0.));
#19052=DIRECTION('',(0.,0.,1.));
#19053=DIRECTION('center_axis',(0.,0.,1.));
#19054=DIRECTION('ref_axis',(-0.937223598005796,-0.348729017062059,0.));
#19055=DIRECTION('',(0.,0.,1.));
#19056=DIRECTION('center_axis',(0.,0.,1.));
#19057=DIRECTION('ref_axis',(-0.937223598005796,-0.348729017062059,0.));
#19058=DIRECTION('',(0.,0.,1.));
#19059=DIRECTION('center_axis',(0.,0.,1.));
#19060=DIRECTION('ref_axis',(-0.937223598005796,-0.348729017062059,0.));
#19061=DIRECTION('',(0.,0.,1.));
#19062=DIRECTION('center_axis',(0.,0.,1.));
#19063=DIRECTION('ref_axis',(-0.937223598005796,-0.348729017062059,0.));
#19064=DIRECTION('',(0.,0.,1.));
#19065=DIRECTION('center_axis',(0.,0.,1.));
#19066=DIRECTION('ref_axis',(-0.937223598005796,-0.348729017062059,0.));
#19067=DIRECTION('',(0.,0.,1.));
#19068=DIRECTION('center_axis',(0.,0.,1.));
#19069=DIRECTION('ref_axis',(-0.937223598005796,-0.348729017062059,0.));
#19070=DIRECTION('',(0.,0.,1.));
#19071=DIRECTION('center_axis',(0.,0.,1.));
#19072=DIRECTION('ref_axis',(-0.937223598005796,-0.348729017062059,0.));
#19073=DIRECTION('',(0.,0.,1.));
#19074=DIRECTION('center_axis',(0.,0.,1.));
#19075=DIRECTION('ref_axis',(-0.937223598005796,-0.348729017062059,0.));
#19076=DIRECTION('',(0.,0.,1.));
#19077=DIRECTION('center_axis',(0.,0.,1.));
#19078=DIRECTION('ref_axis',(-0.937223598005796,-0.348729017062059,0.));
#19079=DIRECTION('',(0.,0.,1.));
#19080=DIRECTION('center_axis',(0.,0.,1.));
#19081=DIRECTION('ref_axis',(-0.937223598005796,-0.348729017062059,0.));
#19082=DIRECTION('',(0.,0.,1.));
#19083=DIRECTION('center_axis',(0.,0.,1.));
#19084=DIRECTION('ref_axis',(-0.937223598005796,-0.348729017062059,0.));
#19085=DIRECTION('',(0.,0.,1.));
#19086=DIRECTION('center_axis',(0.,0.,1.));
#19087=DIRECTION('ref_axis',(-0.937223598005796,-0.348729017062059,0.));
#19088=DIRECTION('',(0.,0.,1.));
#19089=DIRECTION('center_axis',(0.,0.,1.));
#19090=DIRECTION('ref_axis',(-0.937223598005796,-0.348729017062059,0.));
#19091=DIRECTION('',(0.,0.,1.));
#19092=DIRECTION('center_axis',(0.,0.,1.));
#19093=DIRECTION('ref_axis',(-0.937223598005796,-0.348729017062059,0.));
#19094=DIRECTION('',(0.,0.,1.));
#19095=DIRECTION('center_axis',(0.,0.,1.));
#19096=DIRECTION('ref_axis',(-0.937223598005796,-0.348729017062059,0.));
#19097=DIRECTION('',(0.,0.,1.));
#19098=DIRECTION('center_axis',(0.,0.,1.));
#19099=DIRECTION('ref_axis',(-0.937223598005796,-0.348729017062059,0.));
#19100=DIRECTION('',(0.,0.,1.));
#19101=DIRECTION('center_axis',(0.,0.,1.));
#19102=DIRECTION('ref_axis',(-0.937223598005796,-0.348729017062059,0.));
#19103=DIRECTION('',(0.,0.,1.));
#19104=DIRECTION('center_axis',(0.,0.,1.));
#19105=DIRECTION('ref_axis',(-0.937223598005796,-0.348729017062059,0.));
#19106=DIRECTION('',(0.,0.,1.));
#19107=DIRECTION('center_axis',(0.,0.,1.));
#19108=DIRECTION('ref_axis',(-0.937223598005796,-0.348729017062059,0.));
#19109=DIRECTION('',(0.,0.,1.));
#19110=DIRECTION('center_axis',(0.,0.,1.));
#19111=DIRECTION('ref_axis',(-0.937223598005796,-0.348729017062059,0.));
#19112=DIRECTION('',(0.,0.,1.));
#19113=DIRECTION('center_axis',(0.,0.,1.));
#19114=DIRECTION('ref_axis',(-0.937223598005796,-0.348729017062059,0.));
#19115=DIRECTION('',(0.,0.,1.));
#19116=DIRECTION('center_axis',(0.,0.,1.));
#19117=DIRECTION('ref_axis',(-0.937223598005796,-0.348729017062059,0.));
#19118=DIRECTION('',(0.,0.,1.));
#19119=DIRECTION('center_axis',(0.,0.,1.));
#19120=DIRECTION('ref_axis',(-0.937223598005796,-0.348729017062059,0.));
#19121=DIRECTION('',(0.,0.,1.));
#19122=DIRECTION('center_axis',(0.,0.,1.));
#19123=DIRECTION('ref_axis',(-0.937223598005796,-0.348729017062059,0.));
#19124=DIRECTION('',(0.,0.,1.));
#19125=DIRECTION('center_axis',(0.,0.,1.));
#19126=DIRECTION('ref_axis',(-0.937223598005796,-0.348729017062059,0.));
#19127=DIRECTION('',(0.,0.,1.));
#19128=DIRECTION('center_axis',(0.,0.,1.));
#19129=DIRECTION('ref_axis',(-0.937223598005796,-0.348729017062059,0.));
#19130=DIRECTION('',(0.,0.,1.));
#19131=DIRECTION('center_axis',(0.,0.,1.));
#19132=DIRECTION('ref_axis',(-0.937223598005796,-0.348729017062059,0.));
#19133=DIRECTION('',(0.,0.,1.));
#19134=DIRECTION('center_axis',(0.,0.,1.));
#19135=DIRECTION('ref_axis',(-0.937223598005796,-0.348729017062059,0.));
#19136=DIRECTION('',(0.,0.,1.));
#19137=DIRECTION('center_axis',(0.,0.,1.));
#19138=DIRECTION('ref_axis',(-0.937223598005796,-0.348729017062059,0.));
#19139=DIRECTION('',(0.,0.,1.));
#19140=DIRECTION('center_axis',(0.,0.,1.));
#19141=DIRECTION('ref_axis',(-0.937223598005796,-0.348729017062059,0.));
#19142=DIRECTION('',(0.,0.,1.));
#19143=DIRECTION('center_axis',(0.,0.,1.));
#19144=DIRECTION('ref_axis',(-0.937223598005796,-0.348729017062059,0.));
#19145=DIRECTION('',(0.,0.,1.));
#19146=DIRECTION('center_axis',(0.,0.,1.));
#19147=DIRECTION('ref_axis',(-0.937223598005796,-0.348729017062059,0.));
#19148=DIRECTION('',(0.,0.,1.));
#19149=DIRECTION('center_axis',(0.,0.,1.));
#19150=DIRECTION('ref_axis',(-0.937223598005796,-0.348729017062059,0.));
#19151=DIRECTION('',(0.,0.,1.));
#19152=DIRECTION('center_axis',(0.,0.,1.));
#19153=DIRECTION('ref_axis',(-0.937223598005796,-0.348729017062059,0.));
#19154=DIRECTION('',(0.,0.,1.));
#19155=DIRECTION('center_axis',(0.,0.,1.));
#19156=DIRECTION('ref_axis',(-0.937223598005796,-0.348729017062059,0.));
#19157=DIRECTION('',(0.,0.,1.));
#19158=DIRECTION('center_axis',(0.,0.,1.));
#19159=DIRECTION('ref_axis',(-0.937223598005796,-0.348729017062059,0.));
#19160=DIRECTION('',(0.,0.,1.));
#19161=DIRECTION('center_axis',(0.,0.,1.));
#19162=DIRECTION('ref_axis',(-0.937223598005796,-0.348729017062059,0.));
#19163=DIRECTION('',(0.,0.,1.));
#19164=DIRECTION('center_axis',(0.,0.,1.));
#19165=DIRECTION('ref_axis',(-0.937223598005796,-0.348729017062059,0.));
#19166=DIRECTION('',(0.,0.,1.));
#19167=DIRECTION('center_axis',(0.,0.,1.));
#19168=DIRECTION('ref_axis',(-0.937223598005796,-0.348729017062059,0.));
#19169=DIRECTION('',(0.,0.,1.));
#19170=DIRECTION('center_axis',(0.,0.,1.));
#19171=DIRECTION('ref_axis',(-0.937223598005796,-0.348729017062059,0.));
#19172=DIRECTION('',(0.,0.,1.));
#19173=DIRECTION('center_axis',(0.,0.,1.));
#19174=DIRECTION('ref_axis',(-0.937223598005796,-0.348729017062059,0.));
#19175=DIRECTION('',(0.,0.,1.));
#19176=DIRECTION('center_axis',(0.,0.,-1.));
#19177=DIRECTION('ref_axis',(-1.,0.,0.));
#19178=DIRECTION('center_axis',(0.,0.,1.));
#19179=DIRECTION('ref_axis',(-0.937223598005796,-0.348729017062059,0.));
#19180=DIRECTION('center_axis',(0.,0.,1.));
#19181=DIRECTION('ref_axis',(-1.,5.36091303969838E-13,0.));
#19182=DIRECTION('center_axis',(0.,0.,1.));
#19183=DIRECTION('ref_axis',(-1.,5.36091303969838E-13,0.));
#19184=DIRECTION('center_axis',(0.,0.,-1.));
#19185=DIRECTION('ref_axis',(-1.,5.36091303969838E-13,0.));
#19186=DIRECTION('center_axis',(0.,0.,-1.));
#19187=DIRECTION('ref_axis',(-1.,0.,0.));
#19188=DIRECTION('center_axis',(0.,0.,1.));
#19189=DIRECTION('ref_axis',(1.,0.,0.));
#19190=DIRECTION('center_axis',(0.,0.,1.));
#19191=DIRECTION('ref_axis',(1.,0.,0.));
#19192=DIRECTION('center_axis',(0.,0.,1.));
#19193=DIRECTION('ref_axis',(1.,0.,0.));
#19194=DIRECTION('',(-0.0747899482416343,-9.15912707225136E-18,0.997199309888457));
#19195=DIRECTION('center_axis',(0.,0.,-1.));
#19196=DIRECTION('ref_axis',(1.,0.,0.));
#19197=DIRECTION('center_axis',(0.,-1.,0.));
#19198=DIRECTION('ref_axis',(-1.,0.,0.));
#19199=DIRECTION('',(-1.,0.,0.));
#19200=DIRECTION('',(0.,0.,-1.));
#19201=DIRECTION('',(1.,0.,0.));
#19202=DIRECTION('',(0.,0.,-1.));
#19203=DIRECTION('center_axis',(1.,0.,0.));
#19204=DIRECTION('ref_axis',(0.,-1.,0.));
#19205=DIRECTION('',(0.,0.,1.));
#19206=DIRECTION('',(0.,1.,0.));
#19207=DIRECTION('',(0.,-1.,0.));
#19208=DIRECTION('center_axis',(-1.,0.,0.));
#19209=DIRECTION('ref_axis',(0.,1.,0.));
#19210=DIRECTION('',(0.,0.,-1.));
#19211=DIRECTION('',(0.,1.,0.));
#19212=DIRECTION('',(0.,-1.,0.));
#19213=DIRECTION('center_axis',(0.,0.,1.));
#19214=DIRECTION('ref_axis',(1.,0.,0.));
#19215=DIRECTION('center_axis',(0.,0.,1.));
#19216=DIRECTION('ref_axis',(1.,0.,0.));
#19217=DIRECTION('center_axis',(0.,0.,1.));
#19218=DIRECTION('ref_axis',(1.,0.,0.));
#19219=DIRECTION('center_axis',(0.,0.,1.));
#19220=DIRECTION('ref_axis',(-1.,0.,0.));
#19221=DIRECTION('center_axis',(0.,0.,-1.));
#19222=DIRECTION('ref_axis',(1.,0.,0.));
#19223=DIRECTION('center_axis',(0.,0.,1.));
#19224=DIRECTION('ref_axis',(1.,0.,0.));
#19225=DIRECTION('',(0.,0.,1.));
#19226=DIRECTION('center_axis',(0.,0.,1.));
#19227=DIRECTION('ref_axis',(6.12323399573677E-17,-1.,0.));
#19228=DIRECTION('center_axis',(0.,0.,1.));
#19229=DIRECTION('ref_axis',(1.,0.,0.));
#19230=DIRECTION('center_axis',(0.,0.,1.));
#19231=DIRECTION('ref_axis',(1.,0.,0.));
#136539=CARTESIAN_POINT('',(0.,0.,0.));
#136540=CARTESIAN_POINT('Origin',(0.,0.,50.));
#136541=CARTESIAN_POINT('',(6.57110895151819,2.44502632087623,97.3397894808225));
#136542=CARTESIAN_POINT('',(6.57110895151812,2.44502632087642,97.8872278672842));
#136543=CARTESIAN_POINT('',(6.57110895151814,2.44502632087636,50.));
#136544=CARTESIAN_POINT('',(-5.31037376991249,-4.5779424402591,99.));
#136545=CARTESIAN_POINT('Ctrl Pts',(6.57110895151812,2.44502632087642,97.8872278672842));
#136546=CARTESIAN_POINT('Ctrl Pts',(6.50938159924675,2.61092112274443,97.8952353563129));
#136547=CARTESIAN_POINT('Ctrl Pts',(6.44134635625321,2.77453469938154,97.9032428453416));
#136548=CARTESIAN_POINT('Ctrl Pts',(6.36720734438102,2.93535299345077,97.9112503343703));
#136549=CARTESIAN_POINT('Ctrl Pts',(6.29307414937843,3.09615866988426,97.9192571951398));
#136550=CARTESIAN_POINT('Ctrl Pts',(6.21283829259821,3.25416916746725,97.9272640559092));
#136551=CARTESIAN_POINT('Ctrl Pts',(6.12675141741013,3.40889184805898,97.9352709166787));
#136552=CARTESIAN_POINT('Ctrl Pts',(6.04065482482025,3.56363199359472,97.9432786812548));
#136553=CARTESIAN_POINT('Ctrl Pts',(5.94870607806213,3.7150832633239,97.9512864458308));
#136554=CARTESIAN_POINT('Ctrl Pts',(5.85120197845763,3.86277904749852,97.9592942104068));
#136555=CARTESIAN_POINT('Ctrl Pts',(5.75362458113637,4.01058586047909,97.9673079947386));
#136556=CARTESIAN_POINT('Ctrl Pts',(5.65048369152628,4.15463124245543,97.9753217790703));
#136557=CARTESIAN_POINT('Ctrl Pts',(5.54211891182822,4.29447837689935,97.9833355634021));
#136558=CARTESIAN_POINT('Ctrl Pts',(5.43371064956408,4.43438162655229,97.9913525633534));
#136559=CARTESIAN_POINT('Ctrl Pts',(5.32007455496683,4.57008299043006,97.9993695633047));
#136560=CARTESIAN_POINT('Ctrl Pts',(5.2015892770394,4.70118023005806,98.007386563256));
#136561=CARTESIAN_POINT('Ctrl Pts',(5.08296634063021,4.83242978098824,98.0154128775125));
#136562=CARTESIAN_POINT('Ctrl Pts',(4.95948322248214,4.95906425994386,98.023439191769));
#136563=CARTESIAN_POINT('Ctrl Pts',(4.8315546615639,5.08071905489963,98.0314655060255));
#136564=CARTESIAN_POINT('Ctrl Pts',(4.74373431819421,5.16423258611501,98.0369754067775));
#136565=CARTESIAN_POINT('Ctrl Pts',(4.65381976686174,5.24540023570575,98.0424853075295));
#136566=CARTESIAN_POINT('Ctrl Pts',(4.56195357994108,5.3241155225035,98.0479952082814));
#136567=CARTESIAN_POINT('Ctrl Pts',(4.42499058165131,5.44147188671584,98.0562099013319));
#136568=CARTESIAN_POINT('Ctrl Pts',(4.28336273304958,5.55365432817838,98.0644245943823));
#136569=CARTESIAN_POINT('Ctrl Pts',(4.13749531642271,5.66027906282721,98.0726392874327));
#136570=CARTESIAN_POINT('Ctrl Pts',(3.99174322317347,5.76681949952369,98.0808474859132));
#136571=CARTESIAN_POINT('Ctrl Pts',(3.84175851848353,5.86781077799742,98.0890556843936));
#136572=CARTESIAN_POINT('Ctrl Pts',(3.6880001335886,5.96290881845014,98.097263882874));
#136573=CARTESIAN_POINT('Ctrl Pts',(3.53433743431589,6.05794767829181,98.1054669732976));
#136574=CARTESIAN_POINT('Ctrl Pts',(3.37690602897598,6.14710042473671,98.1136700637211));
#136575=CARTESIAN_POINT('Ctrl Pts',(3.21619461362914,6.23006571151243,98.1218731541446));
#136576=CARTESIAN_POINT('Ctrl Pts',(3.05555571769875,6.3129935610335,98.1300725430058));
#136577=CARTESIAN_POINT('Ctrl Pts',(2.89164007015946,6.38973935585205,98.1382719318669));
#136578=CARTESIAN_POINT('Ctrl Pts',(2.72496197647721,6.46004711973941,98.146471320728));
#136579=CARTESIAN_POINT('Ctrl Pts',(2.5583282121748,6.53033618471138,98.1546685288958));
#136580=CARTESIAN_POINT('Ctrl Pts',(2.38893378668065,6.59419049689403,98.1628657370635));
#136581=CARTESIAN_POINT('Ctrl Pts',(2.21731424710863,6.65140166371488,98.1710629452312));
#136582=CARTESIAN_POINT('Ctrl Pts',(2.0456929039503,6.70861343178008,98.1792602395451));
#136583=CARTESIAN_POINT('Ctrl Pts',(1.87184672898898,6.7591818016802,98.187457533859));
#136584=CARTESIAN_POINT('Ctrl Pts',(1.69632810355969,6.80294770871963,98.195654828173));
#136585=CARTESIAN_POINT('Ctrl Pts',(1.61776226550553,6.82253825163974,98.1993241099713));
#136586=CARTESIAN_POINT('Ctrl Pts',(1.53886152202906,6.84076649049615,98.2029933917696));
#136587=CARTESIAN_POINT('Ctrl Pts',(1.4596762357207,6.8576214425537,98.2066626735679));
#136588=CARTESIAN_POINT('Ctrl Pts',(1.26036588358846,6.90004556686235,98.2158983015663));
#136589=CARTESIAN_POINT('Ctrl Pts',(1.05939543449298,6.93373583637616,98.2251339295647));
#136590=CARTESIAN_POINT('Ctrl Pts',(0.857490139543839,6.95861604222313,
98.2343695575632));
#136591=CARTESIAN_POINT('Ctrl Pts',(0.655095352708131,6.98355656674031,
98.2436275760837));
#136592=CARTESIAN_POINT('Ctrl Pts',(0.451761352173247,6.99964427887774,
98.2528855946042));
#136593=CARTESIAN_POINT('Ctrl Pts',(0.248218246296909,7.00685480545339,
98.2621436131248));
#136594=CARTESIAN_POINT('Ctrl Pts',(0.0441803191852665,7.0140828611006,
98.2714241382497));
#136595=CARTESIAN_POINT('Ctrl Pts',(-0.160067563674659,7.01239053413818,
98.2807046633747));
#136596=CARTESIAN_POINT('Ctrl Pts',(-0.363792928534682,7.00180557196843,
98.2899851884996));
#136597=CARTESIAN_POINT('Ctrl Pts',(-0.567660667947921,6.99121321244165,
98.2992721993688));
#136598=CARTESIAN_POINT('Ctrl Pts',(-0.771004994477104,6.9717158117372,
98.308559210238));
#136599=CARTESIAN_POINT('Ctrl Pts',(-0.973097359653584,6.94339312520437,
98.3178462211073));
#136600=CARTESIAN_POINT('Ctrl Pts',(-1.17520208405622,6.91506870656014,
98.3271337999359));
#136601=CARTESIAN_POINT('Ctrl Pts',(-1.37605453125945,6.87791795120786,
98.3364213787646));
#136602=CARTESIAN_POINT('Ctrl Pts',(-1.57493393018921,6.83207213647798,
98.3457089575932));
#136603=CARTESIAN_POINT('Ctrl Pts',(-1.71498653189518,6.79978711517964,
98.3522493513469));
#136604=CARTESIAN_POINT('Ctrl Pts',(-1.85406084048954,6.76319120099996,
98.3587897451006));
#136605=CARTESIAN_POINT('Ctrl Pts',(-1.99190816243168,6.72234545638188,
98.3653301388543));
#136606=CARTESIAN_POINT('Ctrl Pts',(-2.16187146483879,6.67198337791161,
98.3733943283196));
#136607=CARTESIAN_POINT('Ctrl Pts',(-2.33009322388562,6.61512101676402,
98.3814585177849));
#136608=CARTESIAN_POINT('Ctrl Pts',(-2.49603703497894,6.55190244757304,
98.3895227072502));
#136609=CARTESIAN_POINT('Ctrl Pts',(-2.66187495731322,6.48872421815607,
98.3975817509555));
#136610=CARTESIAN_POINT('Ctrl Pts',(-2.82543748715378,6.41919798424373,
98.4056407946608));
#136611=CARTESIAN_POINT('Ctrl Pts',(-2.98620339037331,6.34351762619313,
98.4136998383661));
#136612=CARTESIAN_POINT('Ctrl Pts',(-3.14689695607494,6.26787132094319,
98.4217552558597));
#136613=CARTESIAN_POINT('Ctrl Pts',(-3.30479607283688,6.18607656046159,
98.4298106733532));
#136614=CARTESIAN_POINT('Ctrl Pts',(-3.45939951679128,6.09837532017539,
98.4378660908467));
#136615=CARTESIAN_POINT('Ctrl Pts',(-3.6139828025575,6.01068551493915,98.4459204580232));
#136616=CARTESIAN_POINT('Ctrl Pts',(-3.76527095206601,5.91709093717395,
98.4539748251997));
#136617=CARTESIAN_POINT('Ctrl Pts',(-3.9127872078662,5.81787958181145,98.4620291923763));
#136618=CARTESIAN_POINT('Ctrl Pts',(-4.06029085707759,5.71867670495022,
98.4700828712348));
#136619=CARTESIAN_POINT('Ctrl Pts',(-4.20402295517393,5.61385821278636,
98.4781365500933));
#136620=CARTESIAN_POINT('Ctrl Pts',(-4.34353582520709,5.50375536317182,
98.4861902289519));
#136621=CARTESIAN_POINT('Ctrl Pts',(-4.48309818949812,5.39361345293994,
98.4942467649723));
#136622=CARTESIAN_POINT('Ctrl Pts',(-4.618438051683,5.27818366766274,98.5023033009927));
#136623=CARTESIAN_POINT('Ctrl Pts',(-4.74914061079583,5.15783772732235,
98.5103598370132));
#136624=CARTESIAN_POINT('Ctrl Pts',(-4.82288988548959,5.08993220295707,
98.514905759389));
#136625=CARTESIAN_POINT('Ctrl Pts',(-4.89516335786863,5.02046217444464,
98.5194516817649));
#136626=CARTESIAN_POINT('Ctrl Pts',(-4.96589168557372,4.94949960396501,
98.5239976041407));
#136627=CARTESIAN_POINT('Ctrl Pts',(-5.10456501019901,4.81036701181046,
98.5329105558505));
#136628=CARTESIAN_POINT('Ctrl Pts',(-5.23733419342935,4.66545741062056,
98.5418235075603));
#136629=CARTESIAN_POINT('Ctrl Pts',(-5.36375573085588,4.51527972801361,
98.55073645927));
#136630=CARTESIAN_POINT('Ctrl Pts',(-5.49025725909741,4.36500702334421,
98.5596550504799));
#136631=CARTESIAN_POINT('Ctrl Pts',(-5.610402964147,4.2094597634051,98.5685736416897));
#136632=CARTESIAN_POINT('Ctrl Pts',(-5.72378996119578,4.04917955178755,
98.5774922328996));
#136633=CARTESIAN_POINT('Ctrl Pts',(-5.83725514329902,3.88878882029207,
98.5864169738494));
#136634=CARTESIAN_POINT('Ctrl Pts',(-5.94395216187342,3.72365880958179,
98.5953417147991));
#136635=CARTESIAN_POINT('Ctrl Pts',(-6.04352085889862,3.55436101016165,
98.6042664557489));
#136636=CARTESIAN_POINT('Ctrl Pts',(-6.14310049495826,3.38504461097556,
98.6131921772081));
#136637=CARTESIAN_POINT('Ctrl Pts',(-6.23555012738276,3.21155971822971,
98.6221178986673));
#136638=CARTESIAN_POINT('Ctrl Pts',(-6.32055488329104,3.03450367108129,
98.6310436201265));
#136639=CARTESIAN_POINT('Ctrl Pts',(-6.40555790760715,2.85745123065887,
98.639969159764));
#136640=CARTESIAN_POINT('Ctrl Pts',(-6.48311625585947,2.67682799858681,
98.6488946994016));
#136641=CARTESIAN_POINT('Ctrl Pts',(-6.5529621118045,2.49325372229837,98.6578202390391));
#136642=CARTESIAN_POINT('Ctrl Pts',(-6.61776896624475,2.32292333917929,
98.6661018491684));
#136643=CARTESIAN_POINT('Ctrl Pts',(-6.6759364286139,2.15005271927232,98.6743834592978));
#136644=CARTESIAN_POINT('Ctrl Pts',(-6.72728788244172,1.97515171803403,
98.6826650694271));
#136645=CARTESIAN_POINT('Ctrl Pts',(-6.77907180886219,1.79877773241411,
98.6910164257689));
#136646=CARTESIAN_POINT('Ctrl Pts',(-6.82393755001743,1.62029056482418,
98.6993677821106));
#136647=CARTESIAN_POINT('Ctrl Pts',(-6.86172539517139,1.44026079713366,
98.7077191384523));
#136648=CARTESIAN_POINT('Ctrl Pts',(-6.89949937822043,1.26029707161937,
98.7160674311799));
#136649=CARTESIAN_POINT('Ctrl Pts',(-6.93020057416912,1.07879219770262,
98.7244157239074));
#136650=CARTESIAN_POINT('Ctrl Pts',(-6.95371995337474,0.896328830585069,
98.732764016635));
#136651=CARTESIAN_POINT('Ctrl Pts',(-6.97723395162914,0.713907208892388,
98.7411103993735));
#136652=CARTESIAN_POINT('Ctrl Pts',(-6.9935693678918,0.530527859306804,
98.749456782112));
#136653=CARTESIAN_POINT('Ctrl Pts',(-7.00266874717405,0.34678088161229,
98.7578031648505));
#136654=CARTESIAN_POINT('Ctrl Pts',(-7.01176860716349,0.163024196827935,
98.7661499885165));
#136655=CARTESIAN_POINT('Ctrl Pts',(-7.01363164572051,-0.0210998245922531,
98.7744968121825));
#136656=CARTESIAN_POINT('Ctrl Pts',(-7.00825244637519,-0.204998074079166,
98.7828436358485));
#136657=CARTESIAN_POINT('Ctrl Pts',(-7.00287315096121,-0.388899607857806,
98.7911906085828));
#136658=CARTESIAN_POINT('Ctrl Pts',(-6.99025137322791,-0.572575031011566,
98.7995375813171));
#136659=CARTESIAN_POINT('Ctrl Pts',(-6.97043378629742,-0.755433248767463,
98.8078845540514));
#136660=CARTESIAN_POINT('Ctrl Pts',(-6.95060935228493,-0.938354645013073,
98.8162344107093));
#136661=CARTESIAN_POINT('Ctrl Pts',(-6.92358418101597,-1.12045794309513,
98.8245842673672));
#136662=CARTESIAN_POINT('Ctrl Pts',(-6.88945667745396,-1.30115842693544,
98.8329341240251));
#136663=CARTESIAN_POINT('Ctrl Pts',(-6.87801469298139,-1.36174217653577,
98.8357335942546));
#136664=CARTESIAN_POINT('Ctrl Pts',(-6.8657747823401,-1.42216831972912,
98.8385330644841));
#136665=CARTESIAN_POINT('Ctrl Pts',(-6.85274193659795,-1.48241509466538,
98.8413325347136));
#136666=CARTESIAN_POINT('Ctrl Pts',(-6.81252228002241,-1.66833800403309,
98.8499717631254));
#136667=CARTESIAN_POINT('Ctrl Pts',(-6.76472908610655,-1.85263628174999,
98.8586109915372));
#136668=CARTESIAN_POINT('Ctrl Pts',(-6.70951829686725,-2.03469673084309,
98.8672502199491));
#136669=CARTESIAN_POINT('Ctrl Pts',(-6.65431427480106,-2.21673486483092,
98.8758883894528));
#136670=CARTESIAN_POINT('Ctrl Pts',(-6.59169455695587,-2.39653544071446,
98.8845265589565));
#136671=CARTESIAN_POINT('Ctrl Pts',(-6.52186501817443,-2.57350019374638,
98.8931647284602));
#136672=CARTESIAN_POINT('Ctrl Pts',(-6.44989512403187,-2.75588911919146,
98.9020676677552));
#136673=CARTESIAN_POINT('Ctrl Pts',(-6.37026650450204,-2.93526531040483,
98.9109706070502));
#136674=CARTESIAN_POINT('Ctrl Pts',(-6.28325856614577,-3.11099475304215,
98.9198735463451));
#136675=CARTESIAN_POINT('Ctrl Pts',(-6.19884731142619,-3.28147968837587,
98.9285107844039));
#136676=CARTESIAN_POINT('Ctrl Pts',(-6.10749100141248,-3.4485321420625,
98.9371480224626));
#136677=CARTESIAN_POINT('Ctrl Pts',(-6.00949230902887,-3.61159642682055,
98.9457852605213));
#136678=CARTESIAN_POINT('Ctrl Pts',(-5.90697162010975,-3.78218505820817,
98.9548210504344));
#136679=CARTESIAN_POINT('Ctrl Pts',(-5.7971811902196,-3.94840845108879,
98.9638568403475));
#136680=CARTESIAN_POINT('Ctrl Pts',(-5.68051992566416,-4.10966177886119,
98.9728926302607));
#136681=CARTESIAN_POINT('Ctrl Pts',(-5.56385866110871,-4.27091510663359,
98.9819284201738));
#136682=CARTESIAN_POINT('Ctrl Pts',(-5.44032677457857,-4.42719807501081,
98.9909642100869));
#136683=CARTESIAN_POINT('Ctrl Pts',(-5.31037376991249,-4.5779424402591,
99.));
#136684=CARTESIAN_POINT('',(6.57110895151814,2.44502632087636,99.));
#136685=CARTESIAN_POINT('Origin',(0.,0.,99.));
#136686=CARTESIAN_POINT('',(6.57110895151814,2.44502632087636,100.));
#136687=CARTESIAN_POINT('',(6.57110895151814,2.44502632087636,50.));
#136688=CARTESIAN_POINT('Origin',(0.,0.,100.));
#136689=CARTESIAN_POINT('',(5.30919883249413,-4.57930500398728,98.9999997423022));
#136690=CARTESIAN_POINT('Origin',(0.,0.,99.));
#136691=CARTESIAN_POINT('Ctrl Pts',(5.30919883249413,-4.57930500398728,
98.9999997423022));
#136692=CARTESIAN_POINT('Ctrl Pts',(5.1771100183101,-4.73244740822565,98.9907957854639));
#136693=CARTESIAN_POINT('Ctrl Pts',(5.03841024186428,-4.87985060242226,
98.9815918286256));
#136694=CARTESIAN_POINT('Ctrl Pts',(4.89359335576069,-5.02099299252198,
98.9723878717873));
#136695=CARTESIAN_POINT('Ctrl Pts',(4.74881129474558,-5.16210144116393,
98.9631861282863));
#136696=CARTESIAN_POINT('Ctrl Pts',(4.5979151966278,-5.29695196574323,98.9539843847853));
#136697=CARTESIAN_POINT('Ctrl Pts',(4.44143525768772,-5.42506031434384,
98.9447826412843));
#136698=CARTESIAN_POINT('Ctrl Pts',(4.28516511768279,-5.55299690293928,
98.9355932349301));
#136699=CARTESIAN_POINT('Ctrl Pts',(4.12332623737974,-5.67420925880788,
98.9264038285759));
#136700=CARTESIAN_POINT('Ctrl Pts',(3.95648126930452,-5.78825384102516,
98.9172144222218));
#136701=CARTESIAN_POINT('Ctrl Pts',(3.7898528000229,-5.90215043847101,98.9080369400833));
#136702=CARTESIAN_POINT('Ctrl Pts',(3.61823136495096,-6.00889772772026,
98.8988594579449));
#136703=CARTESIAN_POINT('Ctrl Pts',(3.44220988246632,-6.10809443996663,
98.8896819758064));
#136704=CARTESIAN_POINT('Ctrl Pts',(3.26664748991357,-6.2070324325884,98.8805284298921));
#136705=CARTESIAN_POINT('Ctrl Pts',(3.08670811923343,-6.298459067213,98.8713748839777));
#136706=CARTESIAN_POINT('Ctrl Pts',(2.90301021953404,-6.38201835063022,
98.8622213380634));
#136707=CARTESIAN_POINT('Ctrl Pts',(2.82012422293177,-6.41972098355495,
98.8580911831907));
#136708=CARTESIAN_POINT('Ctrl Pts',(2.73647342651385,-6.4558224925914,98.8539610283179));
#136709=CARTESIAN_POINT('Ctrl Pts',(2.65211653575429,-6.4902930937885,98.8498308734452));
#136710=CARTESIAN_POINT('Ctrl Pts',(2.484685180337,-6.55871026076219,98.8416333519125));
#136711=CARTESIAN_POINT('Ctrl Pts',(2.31456968522284,-6.62065883490146,
98.8334358303799));
#136712=CARTESIAN_POINT('Ctrl Pts',(2.14230841566089,-6.67593747833879,
98.8252383088473));
#136713=CARTESIAN_POINT('Ctrl Pts',(1.97005289241332,-6.73121427778377,
98.8170410607687));
#136714=CARTESIAN_POINT('Ctrl Pts',(1.79565206880699,-6.77982148391708,
98.8088438126901));
#136715=CARTESIAN_POINT('Ctrl Pts',(1.61966035177888,-6.82160735511621,
98.8006465646115));
#136716=CARTESIAN_POINT('Ctrl Pts',(1.44364490626395,-6.86339886019124,
98.7924482113202));
#136717=CARTESIAN_POINT('Ctrl Pts',(1.26603847867586,-6.89836711822544,
98.7842498580288));
#136718=CARTESIAN_POINT('Ctrl Pts',(1.08740676175789,-6.92641127114058,
98.7760515047374));
#136719=CARTESIAN_POINT('Ctrl Pts',(0.908653707047861,-6.95447447339171,
98.7678475826137));
#136720=CARTESIAN_POINT('Ctrl Pts',(0.728874315825774,-6.97560412070713,
98.75964366049));
#136721=CARTESIAN_POINT('Ctrl Pts',(0.548641355379238,-6.98975101313828,
98.7514397383663));
#136722=CARTESIAN_POINT('Ctrl Pts',(0.368339379079348,-7.00390332277975,
98.743232674749));
#136723=CARTESIAN_POINT('Ctrl Pts',(0.187583834699411,-7.01106752899978,
98.7350256111317));
#136724=CARTESIAN_POINT('Ctrl Pts',(0.00694885280283358,-7.0112465564937,
98.7268185475144));
#136725=CARTESIAN_POINT('Ctrl Pts',(-0.173861858941698,-7.01142575815363,
98.7186034996959));
#136726=CARTESIAN_POINT('Ctrl Pts',(-0.354551426213798,-7.0046062164084,
98.7103884518773));
#136727=CARTESIAN_POINT('Ctrl Pts',(-0.534548563102414,-6.99084289597364,
98.7021734040588));
#136728=CARTESIAN_POINT('Ctrl Pts',(-0.614960663067569,-6.98469425651313,
98.6985034054254));
#136729=CARTESIAN_POINT('Ctrl Pts',(-0.695234661301516,-6.9771604840988,
98.694833406792));
#136730=CARTESIAN_POINT('Ctrl Pts',(-0.775320191889768,-6.96824979191677,
98.6911634081586));
#136731=CARTESIAN_POINT('Ctrl Pts',(-0.953332438725084,-6.94844331346142,
98.6830058209163));
#136732=CARTESIAN_POINT('Ctrl Pts',(-1.13078883931262,-6.92178858772011,
98.674848233674));
#136733=CARTESIAN_POINT('Ctrl Pts',(-1.30712494444462,-6.888327151211,98.6666906464318));
#136734=CARTESIAN_POINT('Ctrl Pts',(-1.48330105598853,-6.85489607499189,
98.658540460746));
#136735=CARTESIAN_POINT('Ctrl Pts',(-1.65835855125987,-6.81467065416924,
98.6503902750603));
#136736=CARTESIAN_POINT('Ctrl Pts',(-1.83173834329883,-6.76774417396143,
98.6422400893746));
#136737=CARTESIAN_POINT('Ctrl Pts',(-2.00499456597536,-6.72085113868496,
98.6340957124007));
#136738=CARTESIAN_POINT('Ctrl Pts',(-2.17657512720499,-6.6672666495458,
98.6259513354268));
#136739=CARTESIAN_POINT('Ctrl Pts',(-2.34593121972154,-6.60713502774356,
98.6178069584529));
#136740=CARTESIAN_POINT('Ctrl Pts',(-2.51519956181038,-6.54703456263284,
98.609666801419));
#136741=CARTESIAN_POINT('Ctrl Pts',(-2.68224539890693,-6.48039384135971,
98.6015266443852));
#136742=CARTESIAN_POINT('Ctrl Pts',(-2.84653502872651,-6.40740703348343,
98.5933864873514));
#136743=CARTESIAN_POINT('Ctrl Pts',(-3.01077149323238,-6.33444384466663,
98.5852489645313));
#136744=CARTESIAN_POINT('Ctrl Pts',(-3.17225320489725,-6.25513880485666,
98.5771114417113));
#136745=CARTESIAN_POINT('Ctrl Pts',(-3.33046625360379,-6.16973428083466,
98.5689739188912));
#136746=CARTESIAN_POINT('Ctrl Pts',(-3.48869526370216,-6.08432114074032,
98.5608355751136));
#136747=CARTESIAN_POINT('Ctrl Pts',(-3.64365463637564,-5.99280744701719,
98.5526972313361));
#136748=CARTESIAN_POINT('Ctrl Pts',(-3.79485442333845,-5.89548186903909,
98.5445588875585));
#136749=CARTESIAN_POINT('Ctrl Pts',(-3.94606937133707,-5.79814653207519,
98.5364197277366));
#136750=CARTESIAN_POINT('Ctrl Pts',(-4.09352368424749,-5.6949983404261,
98.5282805679148));
#136751=CARTESIAN_POINT('Ctrl Pts',(-4.2367559690505,-5.58636961015067,
98.5201414080929));
#136752=CARTESIAN_POINT('Ctrl Pts',(-4.38002786946146,-5.47771083502051,
98.5119999971182));
#136753=CARTESIAN_POINT('Ctrl Pts',(-4.51907513284052,-5.36356871458079,
98.5038585861435));
#136754=CARTESIAN_POINT('Ctrl Pts',(-4.65346897011211,-5.24431626684582,
98.4957171751688));
#136755=CARTESIAN_POINT('Ctrl Pts',(-4.78792367424638,-5.12500980977154,
98.4875720769555));
#136756=CARTESIAN_POINT('Ctrl Pts',(-4.91772048849832,-5.00058864849225,
98.4794269787422));
#136757=CARTESIAN_POINT('Ctrl Pts',(-5.04246696640795,-4.87146317395345,
98.4712818805289));
#136758=CARTESIAN_POINT('Ctrl Pts',(-5.16737490010428,-4.74217057601826,
98.4631262403488));
#136759=CARTESIAN_POINT('Ctrl Pts',(-5.28721919142131,-4.60816175451725,
98.4549706001686));
#136760=CARTESIAN_POINT('Ctrl Pts',(-5.40164643868908,-4.46988168902686,
98.4468149599884));
#136761=CARTESIAN_POINT('Ctrl Pts',(-5.51614987536136,-4.33150955214528,
98.4386538895162));
#136762=CARTESIAN_POINT('Ctrl Pts',(-5.62522886349904,-4.18886078260711,
98.430492819044));
#136763=CARTESIAN_POINT('Ctrl Pts',(-5.72857299043121,-4.04240993168704,
98.4223317485718));
#136764=CARTESIAN_POINT('Ctrl Pts',(-5.83209280457585,-3.89571011120744,
98.4141568041063));
#136765=CARTESIAN_POINT('Ctrl Pts',(-5.92985807979365,-3.74519558773904,
98.4059818596407));
#136766=CARTESIAN_POINT('Ctrl Pts',(-6.02160329608752,-3.5913674703444,
98.3978069151753));
#136767=CARTESIAN_POINT('Ctrl Pts',(-6.11130449435766,-3.4409665337578,
98.3898141026454));
#136768=CARTESIAN_POINT('Ctrl Pts',(-6.19525095684959,-3.2873983863897,
98.3818212901156));
#136769=CARTESIAN_POINT('Ctrl Pts',(-6.27323931727951,-3.13114915496507,
98.3738284775858));
#136770=CARTESIAN_POINT('Ctrl Pts',(-6.35305293961989,-2.97124302180428,
98.3656485989837));
#136771=CARTESIAN_POINT('Ctrl Pts',(-6.42687058601045,-2.80803900398797,
98.3574687203816));
#136772=CARTESIAN_POINT('Ctrl Pts',(-6.49440774852088,-2.64202470814562,
98.3492888417795));
#136773=CARTESIAN_POINT('Ctrl Pts',(-6.56185810388284,-2.47622379449305,
98.3411194769732));
#136774=CARTESIAN_POINT('Ctrl Pts',(-6.62304391942586,-2.30762011976299,
98.3329501121669));
#136775=CARTESIAN_POINT('Ctrl Pts',(-6.67772617466965,-2.1367263977009,
98.3247807473606));
#136776=CARTESIAN_POINT('Ctrl Pts',(-6.73234876599036,-1.96601913813642,
98.3166202961653));
#136777=CARTESIAN_POINT('Ctrl Pts',(-6.78048182329003,-1.79302714164819,
98.3084598449701));
#136778=CARTESIAN_POINT('Ctrl Pts',(-6.82193404566059,-1.61828379438126,
98.3002993937748));
#136779=CARTESIAN_POINT('Ctrl Pts',(-6.86334908685656,-1.4436971857047,
98.2921462622151));
#136780=CARTESIAN_POINT('Ctrl Pts',(-6.8980951487709,-1.26736269732559,
98.2839931306554));
#136781=CARTESIAN_POINT('Ctrl Pts',(-6.9260304405994,-1.08982975660906,
98.2758399990957));
#136782=CARTESIAN_POINT('Ctrl Pts',(-6.95394609699602,-0.912421601986873,
98.267692598289));
#136783=CARTESIAN_POINT('Ctrl Pts',(-6.97506046598524,-0.733817021096435,
98.2595451974824));
#136784=CARTESIAN_POINT('Ctrl Pts',(-6.98928259890362,-0.55457669908059,
98.2513977966758));
#136785=CARTESIAN_POINT('Ctrl Pts',(-7.00349787038182,-0.375422851206992,
98.2432543265667));
#136786=CARTESIAN_POINT('Ctrl Pts',(-7.0108275023445,-0.195634224794824,
98.2351108564576));
#136787=CARTESIAN_POINT('Ctrl Pts',(-7.01123224688891,-0.0157779176411367,
98.2269673863485));
#136788=CARTESIAN_POINT('Ctrl Pts',(-7.01163688829294,0.164032557030121,
98.2188259914263));
#136789=CARTESIAN_POINT('Ctrl Pts',(-7.00512015578728,0.343910325018181,
98.2106845965041));
#136790=CARTESIAN_POINT('Ctrl Pts',(-6.99169489609842,0.52328676877144,
98.2025432015819));
#136791=CARTESIAN_POINT('Ctrl Pts',(-6.97827069720004,0.702649039180833,
98.1944024499482));
#136792=CARTESIAN_POINT('Ctrl Pts',(-6.95793908487443,0.881509711912927,
98.1862616983144));
#136793=CARTESIAN_POINT('Ctrl Pts',(-6.93076491789004,1.05930364647948,
98.1781209466806));
#136794=CARTESIAN_POINT('Ctrl Pts',(-6.90358812057128,1.23711479068111,
98.1699794070595));
#136795=CARTESIAN_POINT('Ctrl Pts',(-6.86956750309773,1.41385864178933,
98.1618378674384));
#136796=CARTESIAN_POINT('Ctrl Pts',(-6.8288193624975,1.58897850107521,98.1536963278174));
#136797=CARTESIAN_POINT('Ctrl Pts',(-6.7880413816028,1.76422660248681,98.1455488260607));
#136798=CARTESIAN_POINT('Ctrl Pts',(-6.74052611274211,1.93784799085549,
98.137401324304));
#136799=CARTESIAN_POINT('Ctrl Pts',(-6.686440473137,2.10929854731269,98.1292538225473));
#136800=CARTESIAN_POINT('Ctrl Pts',(-6.63233537602699,2.28081078372907,
98.1211033896973));
#136801=CARTESIAN_POINT('Ctrl Pts',(-6.57165531206145,2.45015029747929,
98.1129529568474));
#136802=CARTESIAN_POINT('Ctrl Pts',(-6.50461607236333,2.61679122469728,
98.1048025239974));
#136803=CARTESIAN_POINT('Ctrl Pts',(-6.43749721470718,2.78363006004203,
98.0966424114311));
#136804=CARTESIAN_POINT('Ctrl Pts',(-6.36400422905059,2.94776357935998,
98.0884822988648));
#136805=CARTESIAN_POINT('Ctrl Pts',(-6.28440028100436,3.10868777309853,
98.0803221862986));
#136806=CARTESIAN_POINT('Ctrl Pts',(-6.20691549353777,3.26532795560334,
98.0723793065367));
#136807=CARTESIAN_POINT('Ctrl Pts',(-6.12364114321325,3.41892726396414,
98.0644364267749));
#136808=CARTESIAN_POINT('Ctrl Pts',(-6.03485983288451,3.56904656174967,
98.056493547013));
#136809=CARTESIAN_POINT('Ctrl Pts',(-5.94312944520581,3.72415242054961,
98.0482868260585));
#136810=CARTESIAN_POINT('Ctrl Pts',(-5.84532617622673,3.87587088288904,
98.0400801051041));
#136811=CARTESIAN_POINT('Ctrl Pts',(-5.74172845038692,4.02370239512286,
98.0318733841496));
#136812=CARTESIAN_POINT('Ctrl Pts',(-5.63821157388823,4.17141853725309,
98.0236730678529));
#136813=CARTESIAN_POINT('Ctrl Pts',(-5.52890944775676,4.31525348752236,
98.0154727515562));
#136814=CARTESIAN_POINT('Ctrl Pts',(-5.41414514519593,4.45473443756767,
98.0072724352595));
#136815=CARTESIAN_POINT('Ctrl Pts',(-5.29945094383672,4.59413018880131,
97.9990771279422));
#136816=CARTESIAN_POINT('Ctrl Pts',(-5.17930143457146,4.72917697003867,
97.9908818206249));
#136817=CARTESIAN_POINT('Ctrl Pts',(-5.05406163144354,4.85943284633817,
97.9826865133076));
#136818=CARTESIAN_POINT('Ctrl Pts',(-4.92887574013236,4.98963265155837,
97.9744947338137));
#136819=CARTESIAN_POINT('Ctrl Pts',(-4.79860416295001,5.1150454105047,97.9663029543198));
#136820=CARTESIAN_POINT('Ctrl Pts',(-4.66365077155621,5.23526389434794,
97.9581111748259));
#136821=CARTESIAN_POINT('Ctrl Pts',(-4.52873164260583,5.35545185669812,
97.9499214750899));
#136822=CARTESIAN_POINT('Ctrl Pts',(-4.38913332932075,5.47044794100356,
97.9417317753539));
#136823=CARTESIAN_POINT('Ctrl Pts',(-4.24529511768192,5.57988314629313,
97.9335420756179));
#136824=CARTESIAN_POINT('Ctrl Pts',(-4.10145226324004,5.68932188392712,
97.9253521115351));
#136825=CARTESIAN_POINT('Ctrl Pts',(-3.95336951279808,5.79319917027657,
97.9171621474523));
#136826=CARTESIAN_POINT('Ctrl Pts',(-3.80151795593428,5.89118729911122,
97.9089721833696));
#136827=CARTESIAN_POINT('Ctrl Pts',(-3.73263068242256,5.93563949421112,
97.9052568161552));
#136828=CARTESIAN_POINT('Ctrl Pts',(-3.66296820624811,5.97888029959546,
97.9015414489408));
#136829=CARTESIAN_POINT('Ctrl Pts',(-3.59257642105848,6.0208820966163,97.8978260817265));
#136830=CARTESIAN_POINT('Ctrl Pts',(-3.41746583716212,6.12536814113416,
97.8885835242243));
#136831=CARTESIAN_POINT('Ctrl Pts',(-3.23796122535888,6.2221118422066,97.8793409667222));
#136832=CARTESIAN_POINT('Ctrl Pts',(-3.05472541607505,6.31080654075889,
97.87009840922));
#136833=CARTESIAN_POINT('Ctrl Pts',(-2.87104650154399,6.39971572296741,
97.8608335011427));
#136834=CARTESIAN_POINT('Ctrl Pts',(-2.68361848852826,6.48053689191889,
97.8515685930654));
#136835=CARTESIAN_POINT('Ctrl Pts',(-2.49312555264651,6.55301087602036,
97.842303684988));
#136836=CARTESIAN_POINT('Ctrl Pts',(-2.30217615924768,6.62565852165254,
97.8330165764185));
#136837=CARTESIAN_POINT('Ctrl Pts',(-2.1081472996239,6.68991889388874,97.823729467849));
#136838=CARTESIAN_POINT('Ctrl Pts',(-1.91174218984874,6.74558139540636,
97.8144423592795));
#136839=CARTESIAN_POINT('Ctrl Pts',(-1.7152055888143,6.80128116241278,97.8051490330835));
#136840=CARTESIAN_POINT('Ctrl Pts',(-1.51628971767753,6.84837151553349,
97.7958557068876));
#136841=CARTESIAN_POINT('Ctrl Pts',(-1.31571086995579,6.88669234605265,
97.7865623806916));
#136842=CARTESIAN_POINT('Ctrl Pts',(-1.1151328186216,6.92501302442102,97.7772690913943));
#136843=CARTESIAN_POINT('Ctrl Pts',(-0.91289196559286,6.95456422419558,
97.767975802097));
#136844=CARTESIAN_POINT('Ctrl Pts',(-0.70971382144022,6.97523711813131,
97.7586825127997));
#136845=CARTESIAN_POINT('Ctrl Pts',(-0.567430900862935,6.9897140675996,
97.7521745473465));
#136846=CARTESIAN_POINT('Ctrl Pts',(-0.424688526410234,6.9998381515994,
97.7456665818933));
#136847=CARTESIAN_POINT('Ctrl Pts',(-0.281737904203388,7.00558707859913,
97.7391586164402));
#136848=CARTESIAN_POINT('Ctrl Pts',(-0.104003942046718,7.01273485842714,
97.7310671057652));
#136849=CARTESIAN_POINT('Ctrl Pts',(0.074172782514224,7.01312142222496,
97.7229755950903));
#136850=CARTESIAN_POINT('Ctrl Pts',(0.252234662995551,7.00671137105586,
97.7148840844154));
#136851=CARTESIAN_POINT('Ctrl Pts',(0.430183508086654,7.00030538904875,
97.706797710309));
#136852=CARTESIAN_POINT('Ctrl Pts',(0.608017295115993,6.9871113957849,97.6987113362028));
#136853=CARTESIAN_POINT('Ctrl Pts',(0.785176856298677,6.96714603455625,
97.6906249620965));
#136854=CARTESIAN_POINT('Ctrl Pts',(0.962256743157727,6.94718965238942,
97.6825422246913));
#136855=CARTESIAN_POINT('Ctrl Pts',(1.13866265030707,6.92046800781678,97.6744594872862));
#136856=CARTESIAN_POINT('Ctrl Pts',(1.31383894351843,6.88704971616979,97.6663767498811));
#136857=CARTESIAN_POINT('Ctrl Pts',(1.48899055770657,6.85363613252741,97.6582951511807));
#136858=CARTESIAN_POINT('Ctrl Pts',(1.66291254773099,6.81352784263588,97.6502135524802));
#136859=CARTESIAN_POINT('Ctrl Pts',(1.83505767294284,6.76684489991263,97.6421319537798));
#136860=CARTESIAN_POINT('Ctrl Pts',(2.00718729147749,6.72016616234665,97.6340510830624));
#136861=CARTESIAN_POINT('Ctrl Pts',(2.17754001682589,6.66691404980923,97.6259702123451));
#136862=CARTESIAN_POINT('Ctrl Pts',(2.3455822066528,6.60725893804184,97.6178893416278));
#136863=CARTESIAN_POINT('Ctrl Pts',(2.51368048927288,6.54758391328802,97.6098057735009));
#136864=CARTESIAN_POINT('Ctrl Pts',(2.6794663562817,6.48150174259789,97.601722205374));
#136865=CARTESIAN_POINT('Ctrl Pts',(2.84242424134802,6.40923170081229,97.5936386372471));
#136866=CARTESIAN_POINT('Ctrl Pts',(2.93077163506064,6.37005059685612,97.5892561418826));
#136867=CARTESIAN_POINT('Ctrl Pts',(3.01828816611891,6.32905155411019,97.5848736465181));
#136868=CARTESIAN_POINT('Ctrl Pts',(3.10489448994278,6.28627526988939,97.5804911511536));
#136869=CARTESIAN_POINT('Ctrl Pts',(3.277718236653,6.20091478600125,97.5717458397792));
#136870=CARTESIAN_POINT('Ctrl Pts',(3.44697940374861,6.10844346605425,97.5630005284048));
#136871=CARTESIAN_POINT('Ctrl Pts',(3.61211310649003,6.00918176363663,97.5542552170304));
#136872=CARTESIAN_POINT('Ctrl Pts',(3.77730538342132,5.90988485233246,97.545506803627));
#136873=CARTESIAN_POINT('Ctrl Pts',(3.9383670408984,5.8037928900154,97.5367583902237));
#136874=CARTESIAN_POINT('Ctrl Pts',(4.09476082785114,5.69127053698872,97.5280099768203));
#136875=CARTESIAN_POINT('Ctrl Pts',(4.25295023697523,5.57745626798632,97.5191611192409));
#136876=CARTESIAN_POINT('Ctrl Pts',(4.40636368953413,5.45706319407653,97.5103122616615));
#136877=CARTESIAN_POINT('Ctrl Pts',(4.55447803405557,5.3305118328173,97.5014634040821));
#136878=CARTESIAN_POINT('Ctrl Pts',(4.70102050149525,5.20530350949996,97.4927084558163));
#136879=CARTESIAN_POINT('Ctrl Pts',(4.8423755982364,5.07406717296795,97.4839535075504));
#136880=CARTESIAN_POINT('Ctrl Pts',(4.97807157498248,4.93724922976868,97.4751985592846));
#136881=CARTESIAN_POINT('Ctrl Pts',(5.11595085121495,4.79822993504611,97.4663027470484));
#136882=CARTESIAN_POINT('Ctrl Pts',(5.24798713545722,4.65344808565009,97.4574069348122));
#136883=CARTESIAN_POINT('Ctrl Pts',(5.37372534685317,4.50341009226206,97.448511122576));
#136884=CARTESIAN_POINT('Ctrl Pts',(5.49946355824921,4.35337209887392,97.4396153103398));
#136885=CARTESIAN_POINT('Ctrl Pts',(5.6189035135465,4.19807819036032,97.4307194981035));
#136886=CARTESIAN_POINT('Ctrl Pts',(5.73163312037174,4.03806987754766,97.4218236858673));
#136887=CARTESIAN_POINT('Ctrl Pts',(5.8419003989686,3.88155659143215,97.4131221829186));
#136888=CARTESIAN_POINT('Ctrl Pts',(5.94576620740795,3.72050586677001,97.4044206799699));
#136889=CARTESIAN_POINT('Ctrl Pts',(6.04287835083162,3.55545324811767,97.3957191770212));
#136890=CARTESIAN_POINT('Ctrl Pts',(6.13996630054085,3.39044174930662,97.3870198418928));
#136891=CARTESIAN_POINT('Ctrl Pts',(6.23030380207177,3.22143058842857,97.3783205067644));
#136892=CARTESIAN_POINT('Ctrl Pts',(6.31358332201366,3.04898215778495,97.369621171636));
#136893=CARTESIAN_POINT('Ctrl Pts',(6.39683952676313,2.87658200633825,97.3609242720004));
#136894=CARTESIAN_POINT('Ctrl Pts',(6.47304157317957,2.70074675880616,97.3522273723649));
#136895=CARTESIAN_POINT('Ctrl Pts',(6.54192863471235,2.52206191455139,97.3435304727293));
#136896=CARTESIAN_POINT('Ctrl Pts',(6.55180594541976,2.49644134537427,97.342283475427));
#136897=CARTESIAN_POINT('Ctrl Pts',(6.56153294711428,2.47076222716117,97.3410364781248));
#136898=CARTESIAN_POINT('Ctrl Pts',(6.57110895151819,2.44502632087623,97.3397894808225));
#136899=CARTESIAN_POINT('Origin',(0.,0.,50.));
#136900=CARTESIAN_POINT('',(6.57110895151813,2.44502632087639,95.3399143481975));
#136901=CARTESIAN_POINT('',(6.57110895151813,2.44502632087639,95.8870186122881));
#136902=CARTESIAN_POINT('',(6.57110895151814,2.44502632087636,50.));
#136903=CARTESIAN_POINT('',(7.01124672537777,-0.00677631017023138,97.77353435695));
#136904=CARTESIAN_POINT('Ctrl Pts',(6.57110895151813,2.44502632087639,95.8870186122881));
#136905=CARTESIAN_POINT('Ctrl Pts',(6.50690586284996,2.61757476628998,95.8953914287838));
#136906=CARTESIAN_POINT('Ctrl Pts',(6.43586635978878,2.78768965768491,95.9037642452794));
#136907=CARTESIAN_POINT('Ctrl Pts',(6.35819928900439,2.95481443813382,95.912137061775));
#136908=CARTESIAN_POINT('Ctrl Pts',(6.28057652111686,3.12184388716574,95.9205051022437));
#136909=CARTESIAN_POINT('Ctrl Pts',(6.19633386208586,3.28588632875983,95.9288731427123));
#136910=CARTESIAN_POINT('Ctrl Pts',(6.1057282037835,3.44640532497597,95.9372411831809));
#136911=CARTESIAN_POINT('Ctrl Pts',(6.01245558962609,3.61164915940669,95.9458555349169));
#136912=CARTESIAN_POINT('Ctrl Pts',(5.91243979135492,3.77315861949584,95.9544698866529));
#136913=CARTESIAN_POINT('Ctrl Pts',(5.80601246713503,3.93037476507936,95.9630842383889));
#136914=CARTESIAN_POINT('Ctrl Pts',(5.70269370606814,4.08299889145352,95.9714469793981));
#136915=CARTESIAN_POINT('Ctrl Pts',(5.59333289399702,4.23157669253178,95.9798097204073));
#136916=CARTESIAN_POINT('Ctrl Pts',(5.47827803891789,4.37562524570032,95.9881724614165));
#136917=CARTESIAN_POINT('Ctrl Pts',(5.36323424519919,4.51965995005766,95.9965343984328));
#136918=CARTESIAN_POINT('Ctrl Pts',(5.24249770521805,4.65916601800551,96.004896335449));
#136919=CARTESIAN_POINT('Ctrl Pts',(5.11645738452041,4.79369277226718,96.0132582724653));
#136920=CARTESIAN_POINT('Ctrl Pts',(4.99041236351663,4.92822454331179,96.0216205213156));
#136921=CARTESIAN_POINT('Ctrl Pts',(4.85906339258932,5.05777639092602,96.0299827701659));
#136922=CARTESIAN_POINT('Ctrl Pts',(4.72283733044507,5.1819334338309,96.0383450190162));
#136923=CARTESIAN_POINT('Ctrl Pts',(4.57942491439849,5.31264015185476,96.0471484028352));
#136924=CARTESIAN_POINT('Ctrl Pts',(4.43060722800965,5.43736721747777,96.0559517866542));
#136925=CARTESIAN_POINT('Ctrl Pts',(4.27692328648132,5.55567761520175,96.0647551704732));
#136926=CARTESIAN_POINT('Ctrl Pts',(4.13082347421755,5.66814952817087,96.0731241172249));
#136927=CARTESIAN_POINT('Ctrl Pts',(3.98032640648811,5.77482263252777,96.0814930639766));
#136928=CARTESIAN_POINT('Ctrl Pts',(3.82592628730087,5.87536506156343,96.0898620107283));
#136929=CARTESIAN_POINT('Ctrl Pts',(3.67147063940784,5.97594364983906,96.0982339673014));
#136930=CARTESIAN_POINT('Ctrl Pts',(3.51310941946559,6.0703869917153,96.1066059238745));
#136931=CARTESIAN_POINT('Ctrl Pts',(3.35136345900299,6.15840803521166,96.1149778804476));
#136932=CARTESIAN_POINT('Ctrl Pts',(3.18949261930352,6.24649703713312,96.1233563007589));
#136933=CARTESIAN_POINT('Ctrl Pts',(3.02423211134264,6.32815368596556,96.1317347210702));
#136934=CARTESIAN_POINT('Ctrl Pts',(2.85612568907477,6.4031377160504,96.1401131413815));
#136935=CARTESIAN_POINT('Ctrl Pts',(2.83022624279836,6.41469018877912,96.1414039692024));
#136936=CARTESIAN_POINT('Ctrl Pts',(2.80425928187736,6.42608437221039,96.1426947970233));
#136937=CARTESIAN_POINT('Ctrl Pts',(2.77822683336898,6.43731949066135,96.1439856248442));
#136938=CARTESIAN_POINT('Ctrl Pts',(2.61956441318577,6.50579522716002,96.1518529549587));
#136939=CARTESIAN_POINT('Ctrl Pts',(2.45813828963,6.56850053935752,96.1597202850731));
#136940=CARTESIAN_POINT('Ctrl Pts',(2.29442486448392,6.6251974388495,96.1675876151876));
#136941=CARTESIAN_POINT('Ctrl Pts',(2.13083753904812,6.68185066774701,96.1754488855177));
#136942=CARTESIAN_POINT('Ctrl Pts',(1.9649667732708,6.73250456367244,96.1833101558478));
#136943=CARTESIAN_POINT('Ctrl Pts',(1.79731079745251,6.7769683826812,96.1911714261779));
#136944=CARTESIAN_POINT('Ctrl Pts',(1.62974973387468,6.82140703014054,96.1990282461401));
#136945=CARTESIAN_POINT('Ctrl Pts',(1.46040583769709,6.85966247431982,96.2068850661022));
#136946=CARTESIAN_POINT('Ctrl Pts',(1.28979418669192,6.89159324963943,96.2147418860644));
#136947=CARTESIAN_POINT('Ctrl Pts',(1.11922361556596,6.92351633666586,96.2225968142612));
#136948=CARTESIAN_POINT('Ctrl Pts',(0.947386269688777,6.94911770765578,
96.230451742458));
#136949=CARTESIAN_POINT('Ctrl Pts',(0.774809094992643,6.96830663998196,
96.2383066706548));
#136950=CARTESIAN_POINT('Ctrl Pts',(0.602260058158601,6.98749244364682,
96.2461603181441));
#136951=CARTESIAN_POINT('Ctrl Pts',(0.428971811781385,7.00026785080371,
96.2540139656333));
#136952=CARTESIAN_POINT('Ctrl Pts',(0.255477670027856,7.00659387453113,
96.2618676131226));
#136953=CARTESIAN_POINT('Ctrl Pts',(0.0819260470819263,7.0129219941644,
96.2697238626422));
#136954=CARTESIAN_POINT('Ctrl Pts',(-0.0918312262693392,7.01279644828536,
96.2775801121618));
#136955=CARTESIAN_POINT('Ctrl Pts',(-0.265259376649008,7.00623037200461,
96.2854363616814));
#136956=CARTESIAN_POINT('Ctrl Pts',(-0.391946857025348,7.00143392080481,
96.2911752711645));
#136957=CARTESIAN_POINT('Ctrl Pts',(-0.518458670809771,6.99320179469873,
96.2969141806476));
#136958=CARTESIAN_POINT('Ctrl Pts',(-0.644587821142489,6.98155663898352,
96.3026530901307));
#136959=CARTESIAN_POINT('Ctrl Pts',(-0.856167445569638,6.96202207725754,
96.3122800186389));
#136960=CARTESIAN_POINT('Ctrl Pts',(-1.06656328869337,6.93289256428335,
96.3219069471471));
#136961=CARTESIAN_POINT('Ctrl Pts',(-1.27499597529445,6.89434636680541,
96.3315338756553));
#136962=CARTESIAN_POINT('Ctrl Pts',(-1.48453805742035,6.85559500487041,
96.3412120440701));
#136963=CARTESIAN_POINT('Ctrl Pts',(-1.69209598426225,6.80732651379363,
96.350890212485));
#136964=CARTESIAN_POINT('Ctrl Pts',(-1.89689796792049,6.74977071179452,
96.3605683808998));
#136965=CARTESIAN_POINT('Ctrl Pts',(-2.10266028247225,6.6919450265952,96.3702919309265));
#136966=CARTESIAN_POINT('Ctrl Pts',(-2.30564070363407,6.62474476635467,
96.3800154809532));
#136967=CARTESIAN_POINT('Ctrl Pts',(-2.50507743216264,6.54845123837457,
96.3897390309799));
#136968=CARTESIAN_POINT('Ctrl Pts',(-2.70471732201702,6.47207999204034,
96.3994724861495));
#136969=CARTESIAN_POINT('Ctrl Pts',(-2.90080625798182,6.38659697744,96.4092059413192));
#136970=CARTESIAN_POINT('Ctrl Pts',(-3.09260159059658,6.29233199730748,
96.4189393964888));
#136971=CARTESIAN_POINT('Ctrl Pts',(-3.28417339246208,6.19817687971098,
96.4286615076571));
#136972=CARTESIAN_POINT('Ctrl Pts',(-3.47146155105454,6.09526027641103,
96.4383836188253));
#136973=CARTESIAN_POINT('Ctrl Pts',(-3.65374801208486,5.98395788978214,
96.4481057299936));
#136974=CARTESIAN_POINT('Ctrl Pts',(-3.73633925582907,5.93352845859224,
96.4525106718014));
#136975=CARTESIAN_POINT('Ctrl Pts',(-3.81790402460925,5.88137818227656,
96.4569156136093));
#136976=CARTESIAN_POINT('Ctrl Pts',(-3.89837706152892,5.82754518203378,
96.4613205554172));
#136977=CARTESIAN_POINT('Ctrl Pts',(-4.04553163005805,5.72910510537479,
96.4693755181221));
#136978=CARTESIAN_POINT('Ctrl Pts',(-4.18910593293877,5.62498673950172,
96.477430480827));
#136979=CARTESIAN_POINT('Ctrl Pts',(-4.32863101602329,5.51548548086397,
96.4854854435318));
#136980=CARTESIAN_POINT('Ctrl Pts',(-4.46806543240111,5.40605537874001,
96.493535171931));
#136981=CARTESIAN_POINT('Ctrl Pts',(-4.6034555816486,5.29124957137755,96.5015849003301));
#136982=CARTESIAN_POINT('Ctrl Pts',(-4.73436169628476,5.17140656797082,
96.5096346287293));
#136983=CARTESIAN_POINT('Ctrl Pts',(-4.86520750587478,5.0516187731223,96.5176806488277));
#136984=CARTESIAN_POINT('Ctrl Pts',(-4.99157312599786,4.92679864863973,
96.5257266689261));
#136985=CARTESIAN_POINT('Ctrl Pts',(-5.11305210603228,4.79732474651226,
96.5337726890245));
#136986=CARTESIAN_POINT('Ctrl Pts',(-5.23451372401776,4.66786934908596,
96.5418175591676));
#136987=CARTESIAN_POINT('Ctrl Pts',(-5.35108983884386,4.53376175977768,
96.5498624293107));
#136988=CARTESIAN_POINT('Ctrl Pts',(-5.46241097454425,4.39541726206723,
96.5579072994538));
#136989=CARTESIAN_POINT('Ctrl Pts',(-5.57372174640787,4.25708564402948,
96.5659514206312));
#136990=CARTESIAN_POINT('Ctrl Pts',(-5.67977828811595,4.11451818967758,
96.5739955418085));
#136991=CARTESIAN_POINT('Ctrl Pts',(-5.78025169558937,3.96816291224745,
96.5820396629858));
#136992=CARTESIAN_POINT('Ctrl Pts',(-5.88076006093902,3.8217567131874,96.5900865829674));
#136993=CARTESIAN_POINT('Ctrl Pts',(-5.97568120713409,3.67156036037432,
96.5981335029489));
#136994=CARTESIAN_POINT('Ctrl Pts',(-6.06472960806618,3.5180507875165,96.6061804229304));
#136995=CARTESIAN_POINT('Ctrl Pts',(-6.1156619111596,3.43024914244823,96.6107829555214));
#136996=CARTESIAN_POINT('Ctrl Pts',(-6.16467382061371,3.34136410660787,
96.6153854881124));
#136997=CARTESIAN_POINT('Ctrl Pts',(-6.21171869217782,3.25148849786504,
96.6199880207034));
#136998=CARTESIAN_POINT('Ctrl Pts',(-6.30054239512213,3.08179764512179,
96.6286778943084));
#136999=CARTESIAN_POINT('Ctrl Pts',(-6.38239382465838,2.90849380649444,
96.6373677679135));
#137000=CARTESIAN_POINT('Ctrl Pts',(-6.45700612408139,2.73216003851814,
96.6460576415185));
#137001=CARTESIAN_POINT('Ctrl Pts',(-6.53163751285033,2.55578115604567,
96.6547497384031));
#137002=CARTESIAN_POINT('Ctrl Pts',(-6.59902596575416,2.37637105546818,
96.6634418352877));
#137003=CARTESIAN_POINT('Ctrl Pts',(-6.65895292057026,2.1945324249436,96.6721339321723));
#137004=CARTESIAN_POINT('Ctrl Pts',(-6.72015326945551,2.00882988652709,
96.6810107283238));
#137005=CARTESIAN_POINT('Ctrl Pts',(-6.77357138147929,1.82059474687604,
96.6898875244753));
#137006=CARTESIAN_POINT('Ctrl Pts',(-6.81902811021709,1.63048526352406,
96.6987643206267));
#137007=CARTESIAN_POINT('Ctrl Pts',(-6.8635689527695,1.44420620647746,96.7074622623998));
#137008=CARTESIAN_POINT('Ctrl Pts',(-6.90046611942902,1.25612789756716,
96.7161602041728));
#137009=CARTESIAN_POINT('Ctrl Pts',(-6.92960258056959,1.06688079833843,
96.7248581459458));
#137010=CARTESIAN_POINT('Ctrl Pts',(-6.95963773426022,0.871796512590155,
96.7338243692865));
#137011=CARTESIAN_POINT('Ctrl Pts',(-6.98142572935758,0.67547049536651,
96.7427905926273));
#137012=CARTESIAN_POINT('Ctrl Pts',(-6.99489582811806,0.478600999034294,
96.751756815968));
#137013=CARTESIAN_POINT('Ctrl Pts',(-7.00836592687853,0.281731502702078,
96.7607230393087));
#137014=CARTESIAN_POINT('Ctrl Pts',(-7.01351811730091,0.0843188530022396,
96.7696892626494));
#137015=CARTESIAN_POINT('Ctrl Pts',(-7.01034036778411,-0.112935779611952,
96.7786554859901));
#137016=CARTESIAN_POINT('Ctrl Pts',(-7.00723646838223,-0.305606263220677,
96.7874133365121));
#137017=CARTESIAN_POINT('Ctrl Pts',(-6.9961850954018,-0.498159174273043,
96.7961711870341));
#137018=CARTESIAN_POINT('Ctrl Pts',(-6.97722014547328,-0.689946087822666,
96.804929037556));
#137019=CARTESIAN_POINT('Ctrl Pts',(-6.95825895555,-0.881694977554558,96.81368515174));
#137020=CARTESIAN_POINT('Ctrl Pts',(-6.93138734865063,-1.07267790346411,
96.8224412659239));
#137021=CARTESIAN_POINT('Ctrl Pts',(-6.8966911077752,-1.26225129290268,
96.8311973801078));
#137022=CARTESIAN_POINT('Ctrl Pts',(-6.86164741998785,-1.45372306346503,
96.8400411777052));
#137023=CARTESIAN_POINT('Ctrl Pts',(-6.81862155666789,-1.64375663390734,
96.8488849753026));
#137024=CARTESIAN_POINT('Ctrl Pts',(-6.76775516826958,-1.83169772202196,
96.8577287729));
#137025=CARTESIAN_POINT('Ctrl Pts',(-6.71742360910297,-2.01766272355116,
96.866479583328));
#137026=CARTESIAN_POINT('Ctrl Pts',(-6.65941568651039,-2.20157876790658,
96.8752303937559));
#137027=CARTESIAN_POINT('Ctrl Pts',(-6.59391944735461,-2.38282456011741,
96.8839812041839));
#137028=CARTESIAN_POINT('Ctrl Pts',(-6.52737925176729,-2.56695926187337,
96.892871495366));
#137029=CARTESIAN_POINT('Ctrl Pts',(-6.45311007031312,-2.748337590493,96.9017617865481));
#137030=CARTESIAN_POINT('Ctrl Pts',(-6.37136138372586,-2.92632545703087,
96.9106520777301));
#137031=CARTESIAN_POINT('Ctrl Pts',(-6.28961269713865,-3.10431332356862,
96.9195423689122));
#137032=CARTESIAN_POINT('Ctrl Pts',(-6.2003846137979,-3.2789104543812,96.9284326600943));
#137033=CARTESIAN_POINT('Ctrl Pts',(-6.10397786506111,-3.44950442605079,
96.9373229512763));
#137034=CARTESIAN_POINT('Ctrl Pts',(-6.01631887157888,-3.6046190424717,
96.9454065552459));
#137035=CARTESIAN_POINT('Ctrl Pts',(-5.92269477698949,-3.75647621605383,
96.9534901592155));
#137036=CARTESIAN_POINT('Ctrl Pts',(-5.82338398339227,-3.90459031711016,
96.9615737631851));
#137037=CARTESIAN_POINT('Ctrl Pts',(-5.72410160994706,-4.05266203178416,
96.9696550538387));
#137038=CARTESIAN_POINT('Ctrl Pts',(-5.61913597920715,-4.19699250786991,
96.9777363444922));
#137039=CARTESIAN_POINT('Ctrl Pts',(-5.50880960624656,-4.33712384935289,
96.9858176351457));
#137040=CARTESIAN_POINT('Ctrl Pts',(-5.39849438982002,-4.47724102033392,
96.9938981085949));
#137041=CARTESIAN_POINT('Ctrl Pts',(-5.28281973492689,-4.61315961982725,
97.0019785820441));
#137042=CARTESIAN_POINT('Ctrl Pts',(-5.16214935538114,-4.74445366667629,
97.0100590554932));
#137043=CARTESIAN_POINT('Ctrl Pts',(-5.04143258981634,-4.87579818331071,
97.0181426350982));
#137044=CARTESIAN_POINT('Ctrl Pts',(-4.91571650573474,-5.00251432844391,
97.0262262147031));
#137045=CARTESIAN_POINT('Ctrl Pts',(-4.78540306382844,-5.124211556835,97.034309794308));
#137046=CARTESIAN_POINT('Ctrl Pts',(-4.65506242598126,-5.24593418299459,
97.0423950609266));
#137047=CARTESIAN_POINT('Ctrl Pts',(-4.52012278783041,-5.36263556517435,
97.0504803275451));
#137048=CARTESIAN_POINT('Ctrl Pts',(-4.38102025936743,-5.47396456414473,
97.0585655941637));
#137049=CARTESIAN_POINT('Ctrl Pts',(-4.24180835106944,-5.58538110392168,
97.0666572184318));
#137050=CARTESIAN_POINT('Ctrl Pts',(-4.0984273015312,-5.69141660437987,
97.0747488427));
#137051=CARTESIAN_POINT('Ctrl Pts',(-3.95134388296962,-5.79176208774312,
97.0828404669681));
#137052=CARTESIAN_POINT('Ctrl Pts',(-3.87166727432526,-5.84612027363079,
97.0872237834997));
#137053=CARTESIAN_POINT('Ctrl Pts',(-3.79090469082852,-5.89880948512701,
97.0916071000313));
#137054=CARTESIAN_POINT('Ctrl Pts',(-3.7091334728529,-5.94978616784353,
97.095990416563));
#137055=CARTESIAN_POINT('Ctrl Pts',(-3.53577909345808,-6.05785635946724,
97.1052830153018));
#137056=CARTESIAN_POINT('Ctrl Pts',(-3.357755268331,-6.15831162867937,97.1145756140406));
#137057=CARTESIAN_POINT('Ctrl Pts',(-3.17570664581012,-6.25080105764513,
97.1238682127794));
#137058=CARTESIAN_POINT('Ctrl Pts',(-2.99361604881999,-6.34331181165382,
97.1331629540881));
#137059=CARTESIAN_POINT('Ctrl Pts',(-2.80749894708967,-6.42785298311338,
97.1424576953968));
#137060=CARTESIAN_POINT('Ctrl Pts',(-2.618023238361,-6.50412030069415,97.1517524367055));
#137061=CARTESIAN_POINT('Ctrl Pts',(-2.42873892818923,-6.58031057697701,
97.1610377889474));
#137062=CARTESIAN_POINT('Ctrl Pts',(-2.23610294378876,-6.64824364361344,
97.1703231411894));
#137063=CARTESIAN_POINT('Ctrl Pts',(-2.04080166490915,-6.70766390981272,
97.1796084934314));
#137064=CARTESIAN_POINT('Ctrl Pts',(-1.84574325224158,-6.76701028415091,
97.1888822989066));
#137065=CARTESIAN_POINT('Ctrl Pts',(-1.64802632051038,-6.81786495122178,
97.1981561043817));
#137066=CARTESIAN_POINT('Ctrl Pts',(-1.44835289836396,-6.8600218982377,
97.2074299098569));
#137067=CARTESIAN_POINT('Ctrl Pts',(-1.24927025245782,-6.90205411496957,
97.2166762768083));
#137068=CARTESIAN_POINT('Ctrl Pts',(-1.04824283215503,-6.93543994729541,
97.2259226437597));
#137069=CARTESIAN_POINT('Ctrl Pts',(-0.84598226594813,-6.96002446606341,
97.2351690107111));
#137070=CARTESIAN_POINT('Ctrl Pts',(-0.703878521063625,-6.97729699846373,
97.2416653010905));
#137071=CARTESIAN_POINT('Ctrl Pts',(-0.56116640908754,-6.99022608997791,
97.2481615914699));
#137072=CARTESIAN_POINT('Ctrl Pts',(-0.418096783378159,-6.9987728668838,
97.2546578818492));
#137073=CARTESIAN_POINT('Ctrl Pts',(-0.237722289166256,-7.00954818382404,
97.2628480555889));
#137074=CARTESIAN_POINT('Ctrl Pts',(-0.0568894238677824,-7.01334864684193,
97.2710382293286));
#137075=CARTESIAN_POINT('Ctrl Pts',(0.123828300587959,-7.01015642582058,
97.2792284030682));
#137076=CARTESIAN_POINT('Ctrl Pts',(0.30453686052778,-7.00696436668241,
97.2874181614697));
#137077=CARTESIAN_POINT('Ctrl Pts',(0.485129942473077,-6.99678033663556,
97.2956079198712));
#137078=CARTESIAN_POINT('Ctrl Pts',(0.665034749132413,-6.97963862567013,
97.3037976782726));
#137079=CARTESIAN_POINT('Ctrl Pts',(0.844960925353261,-6.96249487856762,
97.3119884094749));
#137080=CARTESIAN_POINT('Ctrl Pts',(1.02419831621588,-6.93839183785199,
97.3201791406772));
#137081=CARTESIAN_POINT('Ctrl Pts',(1.20217976787424,-6.90741560702799,
97.3283698718795));
#137082=CARTESIAN_POINT('Ctrl Pts',(1.38027861074408,-6.87641894521397,
97.3365660054417));
#137083=CARTESIAN_POINT('Ctrl Pts',(1.55711951551482,-6.8385400968028,97.3447621390039));
#137084=CARTESIAN_POINT('Ctrl Pts',(1.73214522941971,-6.79391635705788,
97.3529582725661));
#137085=CARTESIAN_POINT('Ctrl Pts',(1.90723594945678,-6.74927604365266,
97.3611574502464));
#137086=CARTESIAN_POINT('Ctrl Pts',(2.08050979910627,-6.69788594001674,
97.3693566279267));
#137087=CARTESIAN_POINT('Ctrl Pts',(2.25142498320302,-6.63993314028909,
97.377555805607));
#137088=CARTESIAN_POINT('Ctrl Pts',(2.42250439565238,-6.58192465508867,
97.3857628616829));
#137089=CARTESIAN_POINT('Ctrl Pts',(2.59122028845276,-6.51734099885269,
97.3939699177588));
#137090=CARTESIAN_POINT('Ctrl Pts',(2.75705029626706,-6.44641762736124,
97.4021769738348));
#137091=CARTESIAN_POINT('Ctrl Pts',(2.83213750636617,-6.41430378882076,
97.4058930982684));
#137092=CARTESIAN_POINT('Ctrl Pts',(2.90663335370148,-6.38089078951168,
97.4096092227021));
#137093=CARTESIAN_POINT('Ctrl Pts',(2.98049102249596,-6.34620357594373,
97.4133253471357));
#137094=CARTESIAN_POINT('Ctrl Pts',(3.1426872115658,-6.2700282248664,97.421486195306));
#137095=CARTESIAN_POINT('Ctrl Pts',(3.3021447895156,-6.18754464539115,97.4296470434764));
#137096=CARTESIAN_POINT('Ctrl Pts',(3.4583426123271,-6.09897474484545,97.4378078916467));
#137097=CARTESIAN_POINT('Ctrl Pts',(3.61439977055824,-6.01048460628149,
97.4459613905322));
#137098=CARTESIAN_POINT('Ctrl Pts',(3.76720271514291,-5.91591923681794,
97.4541148894177));
#137099=CARTESIAN_POINT('Ctrl Pts',(3.91625210871414,-5.81554778017446,
97.4622683883033));
#137100=CARTESIAN_POINT('Ctrl Pts',(4.06519620138751,-5.71524723428244,
97.4704161268785));
#137101=CARTESIAN_POINT('Ctrl Pts',(4.21039173357565,-5.60914896883006,
97.4785638654538));
#137102=CARTESIAN_POINT('Ctrl Pts',(4.35136559320438,-5.4975671016166,97.4867116040291));
#137103=CARTESIAN_POINT('Ctrl Pts',(4.49226720969654,-5.38604241538756,
97.4948551672332));
#137104=CARTESIAN_POINT('Ctrl Pts',(4.62895118739581,-5.26903994476594,
97.5029987304372));
#137105=CARTESIAN_POINT('Ctrl Pts',(4.76097481787534,-5.14691610054573,
97.5111422936413));
#137106=CARTESIAN_POINT('Ctrl Pts',(4.89295640335875,-5.02483114857942,
97.5192832633999));
#137107=CARTESIAN_POINT('Ctrl Pts',(5.0202803399946,-4.89762831270213,97.5274242331586));
#137108=CARTESIAN_POINT('Ctrl Pts',(5.14253822139877,-4.7657032223957,97.5355652029172));
#137109=CARTESIAN_POINT('Ctrl Pts',(5.26480917503177,-4.63376402620956,
97.543707043136));
#137110=CARTESIAN_POINT('Ctrl Pts',(5.38201274438944,-4.49710181989524,
97.5518488833549));
#137111=CARTESIAN_POINT('Ctrl Pts',(5.49377815387643,-4.35614831686091,
97.5599907235737));
#137112=CARTESIAN_POINT('Ctrl Pts',(5.60555517407996,-4.21518017091355,
97.5681334096052));
#137113=CARTESIAN_POINT('Ctrl Pts',(5.71189268820996,-4.06992011644646,
97.5762760956367));
#137114=CARTESIAN_POINT('Ctrl Pts',(5.81246104027801,-3.92083195479611,
97.5844187816682));
#137115=CARTESIAN_POINT('Ctrl Pts',(5.91305752228111,-3.77170209175345,
97.5925637452873));
#137116=CARTESIAN_POINT('Ctrl Pts',(6.0078814288968,-3.61874228092341,97.6007087089063));
#137117=CARTESIAN_POINT('Ctrl Pts',(6.09664710191051,-3.46244432117921,
97.6088536725254));
#137118=CARTESIAN_POINT('Ctrl Pts',(6.18545321120843,-3.3060751615161,97.6170023464984));
#137119=CARTESIAN_POINT('Ctrl Pts',(6.26819541349938,-3.14636513010987,
97.6251510204714));
#137120=CARTESIAN_POINT('Ctrl Pts',(6.34463450985768,-2.98382966987445,
97.6332996944444));
#137121=CARTESIAN_POINT('Ctrl Pts',(6.42117264675738,-2.82108361583628,
97.6414589264842));
#137122=CARTESIAN_POINT('Ctrl Pts',(6.49139120984816,-2.6555051388503,97.6496181585239));
#137123=CARTESIAN_POINT('Ctrl Pts',(6.55509911664866,-2.48762982242373,
97.6577773905637));
#137124=CARTESIAN_POINT('Ctrl Pts',(6.61884953612063,-2.31964248178336,
97.6659420673083));
#137125=CARTESIAN_POINT('Ctrl Pts',(6.67608052612848,-2.14935558071816,
97.6741067440529));
#137126=CARTESIAN_POINT('Ctrl Pts',(6.72665123373126,-1.97731882665436,
97.6822714207976));
#137127=CARTESIAN_POINT('Ctrl Pts',(6.77730780081443,-1.8049899867762,97.6904499596165));
#137128=CARTESIAN_POINT('Ctrl Pts',(6.82128139901214,-1.63090569873286,
97.6986284984353));
#137129=CARTESIAN_POINT('Ctrl Pts',(6.85848223425342,-1.45562632736915,
97.7068070372542));
#137130=CARTESIAN_POINT('Ctrl Pts',(6.8946484528475,-1.28522176471197,97.7147581174056));
#137131=CARTESIAN_POINT('Ctrl Pts',(6.92441362007722,-1.11368800155236,
97.7227091975571));
#137132=CARTESIAN_POINT('Ctrl Pts',(6.94774241808964,-0.941542274344565,
97.7306602777085));
#137133=CARTESIAN_POINT('Ctrl Pts',(6.98967385862435,-0.632125633166784,
97.7449516374424));
#137134=CARTESIAN_POINT('Ctrl Pts',(7.01094414743396,-0.319844675255263,
97.7592429971764));
#137135=CARTESIAN_POINT('Ctrl Pts',(7.01124672537693,-0.0067763110370816,
97.7735343569104));
#137136=CARTESIAN_POINT('Ctrl Pts',(7.01124672537777,-0.00677631017023138,
97.77353435695));
#137137=CARTESIAN_POINT('Ctrl Pts',(7.01141684865851,0.169245191947657,
97.7815696198356));
#137138=CARTESIAN_POINT('Ctrl Pts',(7.00495425607265,0.34555057630013,97.7896048827212));
#137139=CARTESIAN_POINT('Ctrl Pts',(6.99182159260741,0.521591199742505,
97.7976401456068));
#137140=CARTESIAN_POINT('Ctrl Pts',(6.97870710397494,0.697388193330068,
97.8056642881618));
#137141=CARTESIAN_POINT('Ctrl Pts',(6.95894096047927,0.872920793783318,
97.8136884307168));
#137142=CARTESIAN_POINT('Ctrl Pts',(6.93253776919222,1.04763860239271,97.8217125732719));
#137143=CARTESIAN_POINT('Ctrl Pts',(6.90615562336565,1.22221714689968,97.8297303199419));
#137144=CARTESIAN_POINT('Ctrl Pts',(6.87314700967083,1.3959818317732,97.8377480666119));
#137145=CARTESIAN_POINT('Ctrl Pts',(6.83357848984267,1.56838502468607,97.8457658132819));
#137146=CARTESIAN_POINT('Ctrl Pts',(6.79403798413458,1.74066615784624,97.8537778834667));
#137147=CARTESIAN_POINT('Ctrl Pts',(6.74794690239303,1.91158736264453,97.8617899536515));
#137148=CARTESIAN_POINT('Ctrl Pts',(6.69542324046895,2.08060909194597,97.8698020238363));
#137149=CARTESIAN_POINT('Ctrl Pts',(6.65734447976229,2.20314696818164,97.875610638319));
#137150=CARTESIAN_POINT('Ctrl Pts',(6.61588583364576,2.324686605734,97.8814192528015));
#137151=CARTESIAN_POINT('Ctrl Pts',(6.57110895151812,2.44502632087642,97.8872278672842));
#137152=CARTESIAN_POINT('',(7.01124999980813,5.18702180079971E-5,97.226465643065));
#137153=CARTESIAN_POINT('Ctrl Pts',(6.57110895151819,2.44502632087623,97.3397894808225));
#137154=CARTESIAN_POINT('Ctrl Pts',(6.6378710550212,2.26560041768449,97.331095649925));
#137155=CARTESIAN_POINT('Ctrl Pts',(6.69728975529657,2.08341282781443,97.3224018190275));
#137156=CARTESIAN_POINT('Ctrl Pts',(6.74915972893131,1.89907069796566,97.31370798813));
#137157=CARTESIAN_POINT('Ctrl Pts',(6.80101268375869,1.71478905172579,97.3050170097236));
#137158=CARTESIAN_POINT('Ctrl Pts',(6.84532178129947,1.52835454671171,97.2963260313171));
#137159=CARTESIAN_POINT('Ctrl Pts',(6.88193170502248,1.34038896216973,97.2876350529106));
#137160=CARTESIAN_POINT('Ctrl Pts',(6.91630329291163,1.16391561963831,97.279475442134));
#137161=CARTESIAN_POINT('Ctrl Pts',(6.94388877474474,0.986093012273329,
97.2713158313574));
#137162=CARTESIAN_POINT('Ctrl Pts',(6.9646004601257,0.807444730812538,97.2631562205808));
#137163=CARTESIAN_POINT('Ctrl Pts',(6.98611826354919,0.621843292218288,
97.25467903017));
#137164=CARTESIAN_POINT('Ctrl Pts',(7.00022244399454,0.435295819211352,
97.2462018397591));
#137165=CARTESIAN_POINT('Ctrl Pts',(7.00684800478483,0.248410145410525,
97.2377246493483));
#137166=CARTESIAN_POINT('Ctrl Pts',(7.00978125769811,0.165672553155592,
97.233971647262));
#137167=CARTESIAN_POINT('Ctrl Pts',(7.01124938711066,0.0828687677128226,
97.2302186451757));
#137168=CARTESIAN_POINT('Ctrl Pts',(7.01124999980813,5.18707570270757E-5,
97.2264656430894));
#137169=CARTESIAN_POINT('Ctrl Pts',(7.01124999980813,5.18702180126676E-5,
97.226465643065));
#137170=CARTESIAN_POINT('Ctrl Pts',(7.01125130797657,-0.176772062939251,
97.21845253687));
#137171=CARTESIAN_POINT('Ctrl Pts',(7.00455901490281,-0.35364297051039,
97.210439430675));
#137172=CARTESIAN_POINT('Ctrl Pts',(6.99118851967943,-0.530009098792206,
97.2024263244799));
#137173=CARTESIAN_POINT('Ctrl Pts',(6.97757047767512,-0.709640541229728,
97.1942648603812));
#137174=CARTESIAN_POINT('Ctrl Pts',(6.95702452002822,-0.888747936457469,
97.1861033962824));
#137175=CARTESIAN_POINT('Ctrl Pts',(6.92962233224002,-1.06675249942078,
97.1779419321836));
#137176=CARTESIAN_POINT('Ctrl Pts',(6.90270740403597,-1.24159182499501,
97.1699255934169));
#137177=CARTESIAN_POINT('Ctrl Pts',(6.86917813764389,-1.4153668476734,97.1619092546501));
#137178=CARTESIAN_POINT('Ctrl Pts',(6.82915424017152,-1.58753863778095,
97.1538929158834));
#137179=CARTESIAN_POINT('Ctrl Pts',(6.78804347219975,-1.76438584560927,
97.1456588891186));
#137180=CARTESIAN_POINT('Ctrl Pts',(6.7400804338736,-1.93954110860752,97.1374248623538));
#137181=CARTESIAN_POINT('Ctrl Pts',(6.68544970243736,-2.11243670643175,
97.1291908355889));
#137182=CARTESIAN_POINT('Ctrl Pts',(6.63081897100112,-2.28533230425599,
97.1209568088241));
#137183=CARTESIAN_POINT('Ctrl Pts',(6.56952071889578,-2.45596785500244,
97.1127227820592));
#137184=CARTESIAN_POINT('Ctrl Pts',(6.50179287697718,-2.62379800049257,
97.1044887552944));
#137185=CARTESIAN_POINT('Ctrl Pts',(6.42183274031629,-2.82193987227016,
97.0947675846985));
#137186=CARTESIAN_POINT('Ctrl Pts',(6.33286264442571,-3.01629711354463,
97.0850464141025));
#137187=CARTESIAN_POINT('Ctrl Pts',(6.23524423677151,-3.20614345753706,
97.0753252435066));
#137188=CARTESIAN_POINT('Ctrl Pts',(6.1375012290424,-3.39623212128508,97.0655916648145));
#137189=CARTESIAN_POINT('Ctrl Pts',(6.03108785350573,-3.58179832930889,
97.0558580861225));
#137190=CARTESIAN_POINT('Ctrl Pts',(5.91641222425415,-3.76213941198304,
97.0461245074304));
#137191=CARTESIAN_POINT('Ctrl Pts',(5.80193074152675,-3.94217517612877,
97.0364074077452));
#137192=CARTESIAN_POINT('Ctrl Pts',(5.67921498596527,-4.11700345416213,
97.0266903080599));
#137193=CARTESIAN_POINT('Ctrl Pts',(5.54871539220533,-4.28595194312811,
97.0169732083747));
#137194=CARTESIAN_POINT('Ctrl Pts',(5.41856219448823,-4.45445197791631,
97.007281901604));
#137195=CARTESIAN_POINT('Ctrl Pts',(5.28066643649339,-4.61710334260077,
96.9975905948333));
#137196=CARTESIAN_POINT('Ctrl Pts',(5.13551887238781,-4.77326643650327,
96.9878992880627));
#137197=CARTESIAN_POINT('Ctrl Pts',(4.9912958501846,-4.92843482322756,96.9782697117059));
#137198=CARTESIAN_POINT('Ctrl Pts',(4.83991312755717,-5.07719727213506,
96.968640135349));
#137199=CARTESIAN_POINT('Ctrl Pts',(4.68189530176782,-5.21895420039153,
96.9590105589922));
#137200=CARTESIAN_POINT('Ctrl Pts',(4.60975160851087,-5.2836739134878,96.9546141359974));
#137201=CARTESIAN_POINT('Ctrl Pts',(4.53622547744085,-5.34693377426904,
96.9502177130027));
#137202=CARTESIAN_POINT('Ctrl Pts',(4.46136984459314,-5.408678736277,96.9458212900079));
#137203=CARTESIAN_POINT('Ctrl Pts',(4.32760616633227,-5.51901423032146,
96.9379650781426));
#137204=CARTESIAN_POINT('Ctrl Pts',(4.18964934262419,-5.62446438578562,
96.9301088662772));
#137205=CARTESIAN_POINT('Ctrl Pts',(4.04791025671619,-5.72468768720809,
96.9222526544118));
#137206=CARTESIAN_POINT('Ctrl Pts',(3.90621079716929,-5.8248829689442,96.9143986389278));
#137207=CARTESIAN_POINT('Ctrl Pts',(3.76073148972796,-5.91985408365195,
96.9065446234438));
#137208=CARTESIAN_POINT('Ctrl Pts',(3.61191480974728,-6.00930095515513,
96.8986906079598));
#137209=CARTESIAN_POINT('Ctrl Pts',(3.46310945214526,-6.09874102129649,
96.8908371900307));
#137210=CARTESIAN_POINT('Ctrl Pts',(3.31096755453098,-6.18265748529902,
96.8829837721016));
#137211=CARTESIAN_POINT('Ctrl Pts',(3.15595874177031,-6.26079475647809,
96.8751303541724));
#137212=CARTESIAN_POINT('Ctrl Pts',(3.00087080883146,-6.33897191077548,
96.8672729276724));
#137213=CARTESIAN_POINT('Ctrl Pts',(2.84291337770821,-6.411363806658,96.8594155011723));
#137214=CARTESIAN_POINT('Ctrl Pts',(2.68257905108029,-6.47776166566856,
96.8515580746722));
#137215=CARTESIAN_POINT('Ctrl Pts',(2.52220354052918,-6.54417657981875,
96.8436986298916));
#137216=CARTESIAN_POINT('Ctrl Pts',(2.35945027543758,-6.60459425709406,
96.835839185111));
#137217=CARTESIAN_POINT('Ctrl Pts',(2.19482919392977,-6.65885510969969,
96.8279797403304));
#137218=CARTESIAN_POINT('Ctrl Pts',(2.03004440776971,-6.71316992109313,
96.8201124798578));
#137219=CARTESIAN_POINT('Ctrl Pts',(1.86338846140871,-6.76131557379297,
96.8122452193852));
#137220=CARTESIAN_POINT('Ctrl Pts',(1.69538428261051,-6.80318298274986,
96.8043779589125));
#137221=CARTESIAN_POINT('Ctrl Pts',(1.57277800687915,-6.83373702684237,
96.7986365808489));
#137222=CARTESIAN_POINT('Ctrl Pts',(1.44945394977167,-6.86094846313517,
96.7928952027852));
#137223=CARTESIAN_POINT('Ctrl Pts',(1.32561746232401,-6.88479229215244,
96.7871538247215));
#137224=CARTESIAN_POINT('Ctrl Pts',(1.14492041564119,-6.91958421474191,
96.7787762448872));
#137225=CARTESIAN_POINT('Ctrl Pts',(0.96273255722168,-6.94728122495442,
96.7703986650528));
#137226=CARTESIAN_POINT('Ctrl Pts',(0.779636631869397,-6.96776817099617,
96.7620210852185));
#137227=CARTESIAN_POINT('Ctrl Pts',(0.596666158169756,-6.98824108001753,
96.7536492454422));
#137228=CARTESIAN_POINT('Ctrl Pts',(0.412789183682782,-7.00151373752115,
96.7452774056659));
#137229=CARTESIAN_POINT('Ctrl Pts',(0.228596728859201,-7.00752239368915,
96.7369055658896));
#137230=CARTESIAN_POINT('Ctrl Pts',(0.0445034356030402,-7.01352781504623,
96.7285382331641));
#137231=CARTESIAN_POINT('Ctrl Pts',(-0.139904671463392,-7.01227702179111,
96.7201709004386));
#137232=CARTESIAN_POINT('Ctrl Pts',(-0.32403292833021,-7.00375822140212,
96.7118035677131));
#137233=CARTESIAN_POINT('Ctrl Pts',(-0.50808906108166,-6.99524275787707,
96.7034395125208));
#137234=CARTESIAN_POINT('Ctrl Pts',(-0.691865234286078,-6.97946497954286,
96.6950754573285));
#137235=CARTESIAN_POINT('Ctrl Pts',(-0.874767803894187,-6.9564651836813,
96.6867114021362));
#137236=CARTESIAN_POINT('Ctrl Pts',(-1.05762553124577,-6.93347102668392,
96.6783493975608));
#137237=CARTESIAN_POINT('Ctrl Pts',(-1.23960975628846,-6.90325842461056,
96.6699873929854));
#137238=CARTESIAN_POINT('Ctrl Pts',(-1.4201325112331,-6.86591947324164,
96.6616253884101));
#137239=CARTESIAN_POINT('Ctrl Pts',(-1.60066950233367,-6.82857757729583,
96.6532627244009));
#137240=CARTESIAN_POINT('Ctrl Pts',(-1.77974446992953,-6.78410826993594,
96.6449000603918));
#137241=CARTESIAN_POINT('Ctrl Pts',(-1.95677942633535,-6.7326548136059,
96.6365373963826));
#137242=CARTESIAN_POINT('Ctrl Pts',(-2.13382636960631,-6.68119787341226,
96.6281741661456));
#137243=CARTESIAN_POINT('Ctrl Pts',(-2.30883271037858,-6.6227559328789,
96.6198109359086));
#137244=CARTESIAN_POINT('Ctrl Pts',(-2.48123525206485,-6.55752225969616,
96.6114477056716));
#137245=CARTESIAN_POINT('Ctrl Pts',(-2.65367247664211,-6.49227546320124,
96.603082792971));
#137246=CARTESIAN_POINT('Ctrl Pts',(-2.82350455006597,-6.42023432597916,
96.5947178802704));
#137247=CARTESIAN_POINT('Ctrl Pts',(-2.99018749977474,-6.34164058258515,
96.5863529675697));
#137248=CARTESIAN_POINT('Ctrl Pts',(-3.1569262368509,-6.26302053453283,
96.5779852552039));
#137249=CARTESIAN_POINT('Ctrl Pts',(-3.32051345121546,-6.17784364740537,
96.5696175428381));
#137250=CARTESIAN_POINT('Ctrl Pts',(-3.48042866701478,-6.08639818417443,
96.5612498304722));
#137251=CARTESIAN_POINT('Ctrl Pts',(-3.6404921740431,-5.99486792250788,
96.5528743586299));
#137252=CARTESIAN_POINT('Ctrl Pts',(-3.79687659236227,-5.89705763219977,
96.5444988867876));
#137253=CARTESIAN_POINT('Ctrl Pts',(-3.94908834714537,-5.7933002501977,
96.5361234149453));
#137254=CARTESIAN_POINT('Ctrl Pts',(-4.10137476011892,-5.68949197634172,
96.5277438350263));
#137255=CARTESIAN_POINT('Ctrl Pts',(-4.24948416029372,-5.57973098428988,
96.5193642551072));
#137256=CARTESIAN_POINT('Ctrl Pts',(-4.39295460256064,-5.46439167907474,
96.5109846751882));
#137257=CARTESIAN_POINT('Ctrl Pts',(-4.53658908445954,-5.34892049849293,
96.5025955143186));
#137258=CARTESIAN_POINT('Ctrl Pts',(-4.67557375763408,-5.22785847120942,
96.4942063534491));
#137259=CARTESIAN_POINT('Ctrl Pts',(-4.80948121261135,-5.10161905947891,
96.4858171925795));
#137260=CARTESIAN_POINT('Ctrl Pts',(-4.89460261550108,-5.02137202746491,
96.4804844264359));
#137261=CARTESIAN_POINT('Ctrl Pts',(-4.97767315106773,-4.93903366360074,
96.4751516602922));
#137262=CARTESIAN_POINT('Ctrl Pts',(-5.05859124150688,-4.85471741853734,
96.4698188941486));
#137263=CARTESIAN_POINT('Ctrl Pts',(-5.18575276667672,-4.72221574603534,
96.4614385347936));
#137264=CARTESIAN_POINT('Ctrl Pts',(-5.30785359630069,-4.58456025632651,
96.4530581754386));
#137265=CARTESIAN_POINT('Ctrl Pts',(-5.42446601166263,-4.44216107889133,
96.4446778160836));
#137266=CARTESIAN_POINT('Ctrl Pts',(-5.54093063954025,-4.29994236951467,
96.4363080774865));
#137267=CARTESIAN_POINT('Ctrl Pts',(-5.65192050907952,-4.15299220491517,
96.4279383388894));
#137268=CARTESIAN_POINT('Ctrl Pts',(-5.75704484462385,-4.00175726643808,
96.4195686002923));
#137269=CARTESIAN_POINT('Ctrl Pts',(-5.86204990942323,-3.85069391433708,
96.4112083577357));
#137270=CARTESIAN_POINT('Ctrl Pts',(-5.9612025180922,-3.69535574506816,
96.4028481151792));
#137271=CARTESIAN_POINT('Ctrl Pts',(-6.05415201487409,-3.53622255285157,
96.3944878726226));
#137272=CARTESIAN_POINT('Ctrl Pts',(-6.14698098335289,-3.37729570982766,
96.3861384708547));
#137273=CARTESIAN_POINT('Ctrl Pts',(-6.23362271922645,-3.21458394104537,
96.3777890690868));
#137274=CARTESIAN_POINT('Ctrl Pts',(-6.31376980096844,-3.04859598223166,
96.369439667319));
#137275=CARTESIAN_POINT('Ctrl Pts',(-6.39385526815713,-2.88273562973513,
96.3610966843083));
#137276=CARTESIAN_POINT('Ctrl Pts',(-6.46745588918309,-2.7136044002763,
96.3527537012976));
#137277=CARTESIAN_POINT('Ctrl Pts',(-6.5343095759154,-2.54173659701399,
96.3444107182869));
#137278=CARTESIAN_POINT('Ctrl Pts',(-6.60110965728785,-2.3700066026878,
96.3360744249389));
#137279=CARTESIAN_POINT('Ctrl Pts',(-6.66117347513572,-2.19554471529376,
96.3277381315908));
#137280=CARTESIAN_POINT('Ctrl Pts',(-6.71428653058147,-2.01890637419179,
96.3194018382427));
#137281=CARTESIAN_POINT('Ctrl Pts',(-6.73180848478713,-1.96063352775552,
96.3166517017826));
#137282=CARTESIAN_POINT('Ctrl Pts',(-6.74857435224168,-1.90212397241415,
96.3139015653225));
#137283=CARTESIAN_POINT('Ctrl Pts',(-6.76457759240424,-1.84339810101954,
96.3111514288623));
#137284=CARTESIAN_POINT('Ctrl Pts',(-6.81310307226853,-1.66532784393885,
96.3028123868893));
#137285=CARTESIAN_POINT('Ctrl Pts',(-6.85457308635309,-1.48541385332468,
96.2944733449163));
#137286=CARTESIAN_POINT('Ctrl Pts',(-6.88887368500138,-1.30424150930549,
96.2861343029433));
#137287=CARTESIAN_POINT('Ctrl Pts',(-6.92319593805226,-1.12295478888968,
96.2777899964274));
#137288=CARTESIAN_POINT('Ctrl Pts',(-6.95033968674496,-0.940408452334087,
96.2694456899115));
#137289=CARTESIAN_POINT('Ctrl Pts',(-6.97024261627621,-0.757195108771167,
96.2611013833957));
#137290=CARTESIAN_POINT('Ctrl Pts',(-6.99016072631823,-0.573842023361132,
96.2527507124481));
#137291=CARTESIAN_POINT('Ctrl Pts',(-7.0028269656921,-0.389821241423341,
96.2444000415006));
#137292=CARTESIAN_POINT('Ctrl Pts',(-7.00823105916851,-0.205727936376796,
96.236049370553));
#137293=CARTESIAN_POINT('Ctrl Pts',(-7.0136432704791,-0.0213580930115474,
96.227686155529));
#137294=CARTESIAN_POINT('Ctrl Pts',(-7.01177152674709,0.163084163470667,
96.2193229405049));
#137295=CARTESIAN_POINT('Ctrl Pts',(-7.00265765997775,0.347004696877467,
96.2109597254809));
#137296=CARTESIAN_POINT('Ctrl Pts',(-6.99353598803808,0.531082740935358,
96.2025893481492));
#137297=CARTESIAN_POINT('Ctrl Pts',(-6.97715984707511,0.714637844944345,
96.1942189708175));
#137298=CARTESIAN_POINT('Ctrl Pts',(-6.95362270461207,0.897082964058278,
96.1858485934858));
#137299=CARTESIAN_POINT('Ctrl Pts',(-6.93004923143176,1.07980969603362,
96.177465296072));
#137300=CARTESIAN_POINT('Ctrl Pts',(-6.89929272341157,1.2614226970706,96.1690819986582));
#137301=CARTESIAN_POINT('Ctrl Pts',(-6.8614975969031,1.44134565257364,96.1606987012444));
#137302=CARTESIAN_POINT('Ctrl Pts',(-6.84915253210376,1.50011409045881,
96.1579604553549));
#137303=CARTESIAN_POINT('Ctrl Pts',(-6.83605692651224,1.55870234781369,
96.1552222094654));
#137304=CARTESIAN_POINT('Ctrl Pts',(-6.82221694956074,1.61709073821666,
96.1524839635759));
#137305=CARTESIAN_POINT('Ctrl Pts',(-6.77981297178154,1.79598554547597,
96.1440943168113));
#137306=CARTESIAN_POINT('Ctrl Pts',(-6.73033202143919,1.97336413161707,
96.1357046700468));
#137307=CARTESIAN_POINT('Ctrl Pts',(-6.67390018366913,2.1486467603869,96.1273150232822));
#137308=CARTESIAN_POINT('Ctrl Pts',(-6.61752044903762,2.32376755187741,
96.1189331226224));
#137309=CARTESIAN_POINT('Ctrl Pts',(-6.55420272091976,2.49679593235515,
96.1105512219626));
#137310=CARTESIAN_POINT('Ctrl Pts',(-6.4841235365135,2.66716488536642,96.1021693213028));
#137311=CARTESIAN_POINT('Ctrl Pts',(-6.41409874967221,2.83740159288612,
96.0937939269257));
#137312=CARTESIAN_POINT('Ctrl Pts',(-6.33732309494555,3.00498268562966,
96.0854185325486));
#137313=CARTESIAN_POINT('Ctrl Pts',(-6.25402224617961,3.1693583430705,96.0770431381715));
#137314=CARTESIAN_POINT('Ctrl Pts',(-6.17077382624229,3.33363054390435,
96.0686730151947));
#137315=CARTESIAN_POINT('Ctrl Pts',(-6.08100854927491,3.49470103960012,
96.0603028922178));
#137316=CARTESIAN_POINT('Ctrl Pts',(-5.98499950918569,3.65204154378713,
96.051932769241));
#137317=CARTESIAN_POINT('Ctrl Pts',(-5.88903681621092,3.80930609389369,
96.0435666868321));
#137318=CARTESIAN_POINT('Ctrl Pts',(-5.78683654163835,3.96284396305525,
96.0352006044232));
#137319=CARTESIAN_POINT('Ctrl Pts',(-5.67871709607843,4.11215256346437,
96.0268345220143));
#137320=CARTESIAN_POINT('Ctrl Pts',(-5.5706279211741,4.2614193613171,96.0184707818927));
#137321=CARTESIAN_POINT('Ctrl Pts',(-5.45662307117982,4.40645898464192,
96.010107041771));
#137322=CARTESIAN_POINT('Ctrl Pts',(-5.33706386300728,4.54679842138199,
96.0017433016493));
#137323=CARTESIAN_POINT('Ctrl Pts',(-5.21752307038773,4.68711624181687,
95.993380849784));
#137324=CARTESIAN_POINT('Ctrl Pts',(-5.09242983843564,4.8227350689769,95.9850183979186));
#137325=CARTESIAN_POINT('Ctrl Pts',(-4.9621855596968,4.95321522181669,95.9766559460532));
#137326=CARTESIAN_POINT('Ctrl Pts',(-4.83194397379747,5.08369267694021,
95.968293667084));
#137327=CARTESIAN_POINT('Ctrl Pts',(-4.69655178595412,5.20903143725763,
95.9599313881148));
#137328=CARTESIAN_POINT('Ctrl Pts',(-4.55644730889962,5.32882862210087,
95.9515691091456));
#137329=CARTESIAN_POINT('Ctrl Pts',(-4.41632704546271,5.44863930518636,
95.9432058879501));
#137330=CARTESIAN_POINT('Ctrl Pts',(-4.27149368437813,5.56290695473891,
95.9348426667545));
#137331=CARTESIAN_POINT('Ctrl Pts',(-4.12241899829231,5.6712686556906,95.9264794455589));
#137332=CARTESIAN_POINT('Ctrl Pts',(-3.97325651110419,5.77969417885813,
95.9181112986442));
#137333=CARTESIAN_POINT('Ctrl Pts',(-3.81984797283673,5.88220660841757,
95.9097431517295));
#137334=CARTESIAN_POINT('Ctrl Pts',(-3.66269540105741,5.97848550734824,
95.9013750048147));
#137335=CARTESIAN_POINT('Ctrl Pts',(-3.50549572968352,6.07479326165845,
95.8930043499148));
#137336=CARTESIAN_POINT('Ctrl Pts',(-3.34455007042928,6.16486359291641,
95.8846336950148));
#137337=CARTESIAN_POINT('Ctrl Pts',(-3.18038609268354,6.2484214697766,95.8762630401149));
#137338=CARTESIAN_POINT('Ctrl Pts',(-3.01608296100797,6.33205017464116,
95.8678852898123));
#137339=CARTESIAN_POINT('Ctrl Pts',(-2.84855635537664,6.40915525015822,
95.8595075395097));
#137340=CARTESIAN_POINT('Ctrl Pts',(-2.67835607620681,6.47950887734141,
95.8511297892071));
#137341=CARTESIAN_POINT('Ctrl Pts',(-2.57013572790085,6.52424261147797,
95.8458028704723));
#137342=CARTESIAN_POINT('Ctrl Pts',(-2.46083483320128,6.56624774580741,
95.8404759517375));
#137343=CARTESIAN_POINT('Ctrl Pts',(-2.3505982277259,6.60547610201656,95.8351490330028));
#137344=CARTESIAN_POINT('Ctrl Pts',(-2.18788037255691,6.66338022521259,
95.8272860841444));
#137345=CARTESIAN_POINT('Ctrl Pts',(-2.02278453155179,6.71535207099191,
95.819423135286));
#137346=CARTESIAN_POINT('Ctrl Pts',(-1.8558011838239,6.76118543811792,95.8115601864276));
#137347=CARTESIAN_POINT('Ctrl Pts',(-1.68894614424186,6.80698358739476,
95.8037032793716));
#137348=CARTESIAN_POINT('Ctrl Pts',(-1.52020684743442,6.84665253767365,
95.7958463723156));
#137349=CARTESIAN_POINT('Ctrl Pts',(-1.35009246772941,6.88003465769471,
95.7879894652596));
#137350=CARTESIAN_POINT('Ctrl Pts',(-1.1800740292694,6.9133979508408,95.7801369893483));
#137351=CARTESIAN_POINT('Ctrl Pts',(-1.00868242356118,6.94048139365944,
95.7722845134371));
#137352=CARTESIAN_POINT('Ctrl Pts',(-0.836440411773444,6.96117763026144,
95.7644320375259));
#137353=CARTESIAN_POINT('Ctrl Pts',(-0.664239081816405,6.98186897862052,
95.7565814162905));
#137354=CARTESIAN_POINT('Ctrl Pts',(-0.491188122731238,6.99617606946815,
95.748730795055));
#137355=CARTESIAN_POINT('Ctrl Pts',(-0.317818816133417,7.00404295836423,
95.7408801738196));
#137356=CARTESIAN_POINT('Ctrl Pts',(-0.144477404818297,7.01190858147057,
95.7330308157565));
#137357=CARTESIAN_POINT('Ctrl Pts',(0.0291818707769141,7.01333605117387,
95.7251814576933));
#137358=CARTESIAN_POINT('Ctrl Pts',(0.202624771202832,7.00832146555757,
95.7173320996302));
#137359=CARTESIAN_POINT('Ctrl Pts',(0.376126089240345,7.00330519096978,
95.7094800978108));
#137360=CARTESIAN_POINT('Ctrl Pts',(0.549410504846155,6.99184253813279,
95.7016280959914));
#137361=CARTESIAN_POINT('Ctrl Pts',(0.721945745383131,6.97398171084662,
95.693776094172));
#137362=CARTESIAN_POINT('Ctrl Pts',(0.848618974731505,6.96086851342602,
95.6880112520202));
#137363=CARTESIAN_POINT('Ctrl Pts',(0.974888403188787,6.94430758837837,
95.6822464098684));
#137364=CARTESIAN_POINT('Ctrl Pts',(1.1005460416562,6.92433570623889,95.6764815677167));
#137365=CARTESIAN_POINT('Ctrl Pts',(1.31100373558773,6.89088579973252,95.6668263219239));
#137366=CARTESIAN_POINT('Ctrl Pts',(1.51963775258675,6.84788416589393,95.6571710761311));
#137367=CARTESIAN_POINT('Ctrl Pts',(1.72567728557241,6.79556211571636,95.6475158303384));
#137368=CARTESIAN_POINT('Ctrl Pts',(1.93285815865945,6.74295023157737,95.6378071000562));
#137369=CARTESIAN_POINT('Ctrl Pts',(2.13741569195669,6.68091445029655,95.6280983697741));
#137370=CARTESIAN_POINT('Ctrl Pts',(2.33858964665574,6.60973713751573,95.618389639492));
#137371=CARTESIAN_POINT('Ctrl Pts',(2.54073163563266,6.5382173247394,95.6086341915136));
#137372=CARTESIAN_POINT('Ctrl Pts',(2.7394573718015,6.45746782909853,95.5988787435352));
#137373=CARTESIAN_POINT('Ctrl Pts',(2.9340196788317,6.36782184791066,95.5891232955568));
#137374=CARTESIAN_POINT('Ctrl Pts',(3.12877465505256,6.27808709300858,95.5793581870523));
#137375=CARTESIAN_POINT('Ctrl Pts',(3.31935792519388,6.17943825690808,95.5695930785477));
#137376=CARTESIAN_POINT('Ctrl Pts',(3.50504459135589,6.0722556743855,95.5598279700431));
#137377=CARTESIAN_POINT('Ctrl Pts',(3.69047816887279,5.96521918040632,95.5500761712614));
#137378=CARTESIAN_POINT('Ctrl Pts',(3.87102844850403,5.84967220599937,95.5403243724798));
#137379=CARTESIAN_POINT('Ctrl Pts',(4.04599834228836,5.72603911763619,95.5305725736982));
#137380=CARTESIAN_POINT('Ctrl Pts',(4.1223038667914,5.67212191251339,95.5263197499421));
#137381=CARTESIAN_POINT('Ctrl Pts',(4.19754838570267,5.61666740178707,95.522066926186));
#137382=CARTESIAN_POINT('Ctrl Pts',(4.27167559387061,5.55971349830458,95.51781410243));
#137383=CARTESIAN_POINT('Ctrl Pts',(4.41169191776291,5.45213523663757,95.5097810904874));
#137384=CARTESIAN_POINT('Ctrl Pts',(4.54778793700803,5.33915192180933,95.5017480785448));
#137385=CARTESIAN_POINT('Ctrl Pts',(4.67951674515514,5.22108701271226,95.4937150666022));
#137386=CARTESIAN_POINT('Ctrl Pts',(4.8111608693073,5.10309800355164,95.4856872188112));
#137387=CARTESIAN_POINT('Ctrl Pts',(4.93844309898375,4.98003414637678,95.4776593710203));
#137388=CARTESIAN_POINT('Ctrl Pts',(5.06094843304027,4.85226004255824,95.4696315232293));
#137389=CARTESIAN_POINT('Ctrl Pts',(5.18339845174301,4.72454363312346,95.4616073002866));
#137390=CARTESIAN_POINT('Ctrl Pts',(5.30107561635766,4.59212147587694,95.4535830773439));
#137391=CARTESIAN_POINT('Ctrl Pts',(5.41360077607436,4.45539596442191,95.4455588544012));
#137392=CARTESIAN_POINT('Ctrl Pts',(5.52611232760838,4.3186869878089,95.4375356018644));
#137393=CARTESIAN_POINT('Ctrl Pts',(5.63347287650376,4.17767597156114,95.4295123493277));
#137394=CARTESIAN_POINT('Ctrl Pts',(5.73534256615504,4.03279955010785,95.421489096791));
#137395=CARTESIAN_POINT('Ctrl Pts',(5.83720390686241,3.88793500230533,95.4134665018168));
#137396=CARTESIAN_POINT('Ctrl Pts',(5.93357507710645,3.73920598256375,95.4054439068425));
#137397=CARTESIAN_POINT('Ctrl Pts',(6.02415887194168,3.5870790969961,95.3974213118683));
#137398=CARTESIAN_POINT('Ctrl Pts',(6.11477671916688,3.43489502367163,95.3893957010287));
#137399=CARTESIAN_POINT('Ctrl Pts',(6.19960265977088,3.27931084955247,95.381370090189));
#137400=CARTESIAN_POINT('Ctrl Pts',(6.27838469185183,3.12081915907036,95.3733444793494));
#137401=CARTESIAN_POINT('Ctrl Pts',(6.32484158601581,3.02735835974708,95.3686118652808));
#137402=CARTESIAN_POINT('Ctrl Pts',(6.3691976891623,2.93288697901579,95.3638792512122));
#137403=CARTESIAN_POINT('Ctrl Pts',(6.41140909568922,2.83750946610113,95.3591466371436));
#137404=CARTESIAN_POINT('Ctrl Pts',(6.46858834556246,2.70831181333498,95.3527358741616));
#137405=CARTESIAN_POINT('Ctrl Pts',(6.52185266125821,2.57740462988759,95.3463251111796));
#137406=CARTESIAN_POINT('Ctrl Pts',(6.57110895151813,2.44502632087639,95.3399143481975));
#137407=CARTESIAN_POINT('Origin',(0.,0.,50.));
#137408=CARTESIAN_POINT('',(6.57110895151818,2.44502632087624,93.3398552680816));
#137409=CARTESIAN_POINT('',(6.5711089515182,2.44502632087621,93.8869739242502));
#137410=CARTESIAN_POINT('',(6.57110895151814,2.44502632087636,50.));
#137411=CARTESIAN_POINT('',(7.01124720379832,0.00626176734431896,95.7735343568769));
#137412=CARTESIAN_POINT('Ctrl Pts',(6.5711089515182,2.44502632087621,93.8869739242502));
#137413=CARTESIAN_POINT('Ctrl Pts',(6.50187635357225,2.63109177964659,93.8960060995485));
#137414=CARTESIAN_POINT('Ctrl Pts',(6.42476030326037,2.81415210874128,93.9050382748468));
#137415=CARTESIAN_POINT('Ctrl Pts',(6.34004140271719,2.99357671929948,93.9140704501451));
#137416=CARTESIAN_POINT('Ctrl Pts',(6.31324472208978,3.05032891928082,93.9169273370415));
#137417=CARTESIAN_POINT('Ctrl Pts',(6.2856877567968,3.10671754768292,93.9197842239379));
#137418=CARTESIAN_POINT('Ctrl Pts',(6.25738035770925,3.1627231338602,93.9226411108343));
#137419=CARTESIAN_POINT('Ctrl Pts',(6.17947165912967,3.31686383462762,93.9305039434245));
#137420=CARTESIAN_POINT('Ctrl Pts',(6.09575013385189,3.4683483313514,93.9383667760146));
#137421=CARTESIAN_POINT('Ctrl Pts',(6.00642878203697,3.61668907273185,93.9462296086048));
#137422=CARTESIAN_POINT('Ctrl Pts',(5.91717606190045,3.76491583381699,93.9540863996451));
#137423=CARTESIAN_POINT('Ctrl Pts',(5.82233226722473,3.91000331873197,93.9619431906854));
#137424=CARTESIAN_POINT('Ctrl Pts',(5.7221574308434,4.05148625804699,93.9697999817257));
#137425=CARTESIAN_POINT('Ctrl Pts',(5.62203908834727,4.19288940765416,93.9776523419063));
#137426=CARTESIAN_POINT('Ctrl Pts',(5.51659590430895,4.33069174515327,93.9855047020868));
#137427=CARTESIAN_POINT('Ctrl Pts',(5.40613242074995,4.46445504085507,93.9933570622674));
#137428=CARTESIAN_POINT('Ctrl Pts',(5.2956950189893,4.59818675338393,94.0012075684083));
#137429=CARTESIAN_POINT('Ctrl Pts',(5.18023991294407,4.72788102308838,94.0090580745493));
#137430=CARTESIAN_POINT('Ctrl Pts',(5.06011326816006,4.85313097658517,94.0169085806902));
#137431=CARTESIAN_POINT('Ctrl Pts',(4.94000594799955,4.97836078127818,94.02475782393));
#137432=CARTESIAN_POINT('Ctrl Pts',(4.81522885138723,5.09914741974926,94.0326070671699));
#137433=CARTESIAN_POINT('Ctrl Pts',(4.68616617400958,5.2151196680487,94.0404563104097));
#137434=CARTESIAN_POINT('Ctrl Pts',(4.55706001303342,5.33113098953945,94.0483081982044));
#137435=CARTESIAN_POINT('Ctrl Pts',(4.4236656712448,5.44232442567005,94.0561600859992));
#137436=CARTESIAN_POINT('Ctrl Pts',(4.28640185159585,5.54836784371185,94.0640119737939));
#137437=CARTESIAN_POINT('Ctrl Pts',(4.18561090108865,5.62623407916122,94.0697775079028));
#137438=CARTESIAN_POINT('Ctrl Pts',(4.08273435009313,5.70132435415834,94.0755430420118));
#137439=CARTESIAN_POINT('Ctrl Pts',(3.97794824856921,5.77352182763737,94.0813085761207));
#137440=CARTESIAN_POINT('Ctrl Pts',(3.80246749989206,5.89442781148875,94.0909638665385));
#137441=CARTESIAN_POINT('Ctrl Pts',(3.6217206210363,6.00715877938681,94.1006191569563));
#137442=CARTESIAN_POINT('Ctrl Pts',(3.43642534723564,6.1113507013897,94.110274447374));
#137443=CARTESIAN_POINT('Ctrl Pts',(3.25010359377656,6.21611981506249,94.1199832251744));
#137444=CARTESIAN_POINT('Ctrl Pts',(3.05918298027622,6.31225503790836,94.1296920029748));
#137445=CARTESIAN_POINT('Ctrl Pts',(2.86440879581883,6.39943660121231,94.1394007807752));
#137446=CARTESIAN_POINT('Ctrl Pts',(2.66869735528858,6.48703768340617,94.1491562773488));
#137447=CARTESIAN_POINT('Ctrl Pts',(2.46909521699324,6.56559873268788,94.1589117739224));
#137448=CARTESIAN_POINT('Ctrl Pts',(2.26637326359146,6.63484580021102,94.1686672704961));
#137449=CARTESIAN_POINT('Ctrl Pts',(2.06345058232361,6.70416143364852,94.1784324266057));
#137450=CARTESIAN_POINT('Ctrl Pts',(1.85740194688975,6.76414463667469,94.1881975827153));
#137451=CARTESIAN_POINT('Ctrl Pts',(1.64901461151091,6.81457096034105,94.197962738825));
#137452=CARTESIAN_POINT('Ctrl Pts',(1.44091138814327,6.86492853355188,94.2077145812746));
#137453=CARTESIAN_POINT('Ctrl Pts',(1.23047587448614,6.90575526020403,94.2174664237241));
#137454=CARTESIAN_POINT('Ctrl Pts',(1.01850554816107,6.9368777566615,94.2272182661737));
#137455=CARTESIAN_POINT('Ctrl Pts',(0.926069348082637,6.95044968137077,
94.2314708579182));
#137456=CARTESIAN_POINT('Ctrl Pts',(0.833341447425697,6.96217683158084,
94.2357234496627));
#137457=CARTESIAN_POINT('Ctrl Pts',(0.740388755512456,6.97204783784583,
94.2399760414071));
#137458=CARTESIAN_POINT('Ctrl Pts',(0.564802974259925,6.99069397182121,
94.2480091024023));
#137459=CARTESIAN_POINT('Ctrl Pts',(0.38832900081566,7.00272228021506,94.2560421633975));
#137460=CARTESIAN_POINT('Ctrl Pts',(0.211513544993474,7.00805883128733,
94.2640752243926));
#137461=CARTESIAN_POINT('Ctrl Pts',(0.0348117535537583,7.01339195180099,
94.2721031213996));
#137462=CARTESIAN_POINT('Ctrl Pts',(-0.14223071843289,7.01204186670312,
94.2801310184066));
#137463=CARTESIAN_POINT('Ctrl Pts',(-0.319061895785846,7.00398644124598,
94.2881589154136));
#137464=CARTESIAN_POINT('Ctrl Pts',(-0.495813231257835,6.99593465293208,
94.2961831877069));
#137465=CARTESIAN_POINT('Ctrl Pts',(-0.672353096625605,6.9811835691255,
94.3042074600002));
#137466=CARTESIAN_POINT('Ctrl Pts',(-0.848129418562242,6.95976314624782,
94.3122317322934));
#137467=CARTESIAN_POINT('Ctrl Pts',(-1.02388448505733,6.93834531359697,
94.3202550342658));
#137468=CARTESIAN_POINT('Ctrl Pts',(-1.19887582743081,6.91025978490584,
94.3282783362381));
#137469=CARTESIAN_POINT('Ctrl Pts',(-1.37255621721105,6.87558841068132,
94.3363016382104));
#137470=CARTESIAN_POINT('Ctrl Pts',(-1.54622237432089,6.84091987768858,
94.3443242826933));
#137471=CARTESIAN_POINT('Ctrl Pts',(-1.71857743406365,6.79966664989602,
94.3523469271762));
#137472=CARTESIAN_POINT('Ctrl Pts',(-1.88908438818062,6.75196169545061,
94.3603695716592));
#137473=CARTESIAN_POINT('Ctrl Pts',(-2.05965543778592,6.70423880817445,
94.3683952319447));
#137474=CARTESIAN_POINT('Ctrl Pts',(-2.22837664149849,6.65005945107496,
94.3764208922302));
#137475=CARTESIAN_POINT('Ctrl Pts',(-2.39472581272296,6.58960657735941,
94.3844465525158));
#137476=CARTESIAN_POINT('Ctrl Pts',(-2.49281334186375,6.55396063474021,
94.389178870575));
#137477=CARTESIAN_POINT('Ctrl Pts',(-2.59007646852318,6.51613441841792,
94.3939111886343));
#137478=CARTESIAN_POINT('Ctrl Pts',(-2.68641138928797,6.47617328443301,
94.3986435066936));
#137479=CARTESIAN_POINT('Ctrl Pts',(-2.86412647933467,6.40245446608432,
94.4073735115906));
#137480=CARTESIAN_POINT('Ctrl Pts',(-3.03877054674181,6.32143101450371,
94.4161035164877));
#137481=CARTESIAN_POINT('Ctrl Pts',(-3.20976034756245,6.23338311623117,
94.4248335213847));
#137482=CARTESIAN_POINT('Ctrl Pts',(-3.3807995820536,6.14530976304394,94.4335660501527));
#137483=CARTESIAN_POINT('Ctrl Pts',(-3.54818219765204,6.0502080350156,94.4422985789206));
#137484=CARTESIAN_POINT('Ctrl Pts',(-3.71134950975104,5.94840410353657,
94.4510311076886));
#137485=CARTESIAN_POINT('Ctrl Pts',(-3.8768361273496,5.84515310269592,94.4598877630462));
#137486=CARTESIAN_POINT('Ctrl Pts',(-4.03798644675668,5.73500806498855,
94.4687444184038));
#137487=CARTESIAN_POINT('Ctrl Pts',(-4.19424763425525,5.61835503907009,
94.4776010737614));
#137488=CARTESIAN_POINT('Ctrl Pts',(-4.34841689212475,5.5032636928313,94.4863391616101));
#137489=CARTESIAN_POINT('Ctrl Pts',(-4.4978269013566,5.38183771028731,94.4950772494587));
#137490=CARTESIAN_POINT('Ctrl Pts',(-4.64197892219142,5.25448934230821,
94.5038153373073));
#137491=CARTESIAN_POINT('Ctrl Pts',(-4.78906495095671,5.12454898068643,
94.5127312764194));
#137492=CARTESIAN_POINT('Ctrl Pts',(-4.93067643527349,4.98844275982695,
94.5216472155315));
#137493=CARTESIAN_POINT('Ctrl Pts',(-5.06632123746025,4.84664994417373,
94.5305631546437));
#137494=CARTESIAN_POINT('Ctrl Pts',(-5.20196603964701,4.70485712852052,
94.5394790937558));
#137495=CARTESIAN_POINT('Ctrl Pts',(-5.33164395503715,4.55737794082213,
94.5483950328679));
#137496=CARTESIAN_POINT('Ctrl Pts',(-5.45490408292118,4.40473018567878,
94.5573109719801));
#137497=CARTESIAN_POINT('Ctrl Pts',(-5.57574224718861,4.25508183768729,
94.5660517199699));
#137498=CARTESIAN_POINT('Ctrl Pts',(-5.69042532874712,4.10045025632833,
94.5747924679597));
#137499=CARTESIAN_POINT('Ctrl Pts',(-5.79856547132695,3.94135319874214,
94.5835332159496));
#137500=CARTESIAN_POINT('Ctrl Pts',(-5.90668616011302,3.78228476180756,
94.5922723915288));
#137501=CARTESIAN_POINT('Ctrl Pts',(-6.00826610670268,3.61875267927341,
94.6010115671081));
#137502=CARTESIAN_POINT('Ctrl Pts',(-6.10296041194246,3.45130421330302,
94.6097507426873));
#137503=CARTESIAN_POINT('Ctrl Pts',(-6.19888057477878,3.28168805653517,
94.6186030505689));
#137504=CARTESIAN_POINT('Ctrl Pts',(-6.28773541960707,3.10805364859761,
94.6274553584504));
#137505=CARTESIAN_POINT('Ctrl Pts',(-6.3692135494138,2.93099732590524,94.636307666332));
#137506=CARTESIAN_POINT('Ctrl Pts',(-6.44960915198152,2.75629339265295,
94.6450423614943));
#137507=CARTESIAN_POINT('Ctrl Pts',(-6.52282273410113,2.57825816931711,
94.6537770566566));
#137508=CARTESIAN_POINT('Ctrl Pts',(-6.58860235167932,2.39748735428277,
94.6625117518188));
#137509=CARTESIAN_POINT('Ctrl Pts',(-6.6557105536364,2.21306541919246,94.6714228660601));
#137510=CARTESIAN_POINT('Ctrl Pts',(-6.71508118046351,2.02579647755037,
94.6803339803013));
#137511=CARTESIAN_POINT('Ctrl Pts',(-6.76649883805895,1.83633331316702,
94.6892450945425));
#137512=CARTESIAN_POINT('Ctrl Pts',(-6.81791649565438,1.64687014878366,
94.6981562087838));
#137513=CARTESIAN_POINT('Ctrl Pts',(-6.86138109162555,1.45521305064215,
94.707067323025));
#137514=CARTESIAN_POINT('Ctrl Pts',(-6.89673142007993,1.26203101458811,
94.7159784372663));
#137515=CARTESIAN_POINT('Ctrl Pts',(-6.92856904036444,1.08804518252959,
94.7240040676898));
#137516=CARTESIAN_POINT('Ctrl Pts',(-6.95383899451732,0.91274237675236,
94.7320296981133));
#137517=CARTESIAN_POINT('Ctrl Pts',(-6.97244213013835,0.73666634535033,
94.7400553285368));
#137518=CARTESIAN_POINT('Ctrl Pts',(-6.99103936169987,0.560646195031391,
94.7480784118736));
#137519=CARTESIAN_POINT('Ctrl Pts',(-7.00297394870145,0.383853671762942,
94.7561014952104));
#137520=CARTESIAN_POINT('Ctrl Pts',(-7.0081983319312,0.206839799885714,
94.7641245785472));
#137521=CARTESIAN_POINT('Ctrl Pts',(-7.01342205637092,0.0298482492984376,
94.7721466501804));
#137522=CARTESIAN_POINT('Ctrl Pts',(-7.01193725225356,-0.147364227972788,
94.7801687218137));
#137523=CARTESIAN_POINT('Ctrl Pts',(-7.00374843033024,-0.324244486686702,
94.7881907934469));
#137524=CARTESIAN_POINT('Ctrl Pts',(-6.99555656518016,-0.501190479732401,
94.7962158463371));
#137525=CARTESIAN_POINT('Ctrl Pts',(-6.98065571911359,-0.677803640917794,
94.8042408992274));
#137526=CARTESIAN_POINT('Ctrl Pts',(-6.95910248079875,-0.853533376172657,
94.8122659521176));
#137527=CARTESIAN_POINT('Ctrl Pts',(-6.9375449973977,-1.02929772283331,
94.8202925856076));
#137528=CARTESIAN_POINT('Ctrl Pts',(-6.90933256489799,-1.20417793416387,
94.8283192190975));
#137529=CARTESIAN_POINT('Ctrl Pts',(-6.87457325191952,-1.37763172382634,
94.8363458525874));
#137530=CARTESIAN_POINT('Ctrl Pts',(-6.83978603289908,-1.5512247685062,
94.844378930151));
#137531=CARTESIAN_POINT('Ctrl Pts',(-6.79844151683118,-1.72338874676923,
94.8524120077145));
#137532=CARTESIAN_POINT('Ctrl Pts',(-6.7506983351773,-1.89359408267308,
94.860445085278));
#137533=CARTESIAN_POINT('Ctrl Pts',(-6.7225649830702,-1.99389000932927,
94.8651786910363));
#137534=CARTESIAN_POINT('Ctrl Pts',(-6.6922107514037,-2.09350612364148,
94.8699122967947));
#137535=CARTESIAN_POINT('Ctrl Pts',(-6.65967601729563,-2.19233708794005,
94.874645902553));
#137536=CARTESIAN_POINT('Ctrl Pts',(-6.59265675514006,-2.39592191772262,
94.8843967972185));
#137537=CARTESIAN_POINT('Ctrl Pts',(-6.51634348769129,-2.59629432248839,
94.8941476918841));
#137538=CARTESIAN_POINT('Ctrl Pts',(-6.4310532843521,-2.79270124007637,
94.9038985865496));
#137539=CARTESIAN_POINT('Ctrl Pts',(-6.34564023878688,-2.9893910396604,
94.9136635252853));
#137540=CARTESIAN_POINT('Ctrl Pts',(-6.25122441023194,-3.18210389206936,
94.9234284640211));
#137541=CARTESIAN_POINT('Ctrl Pts',(-6.14817084123131,-3.37010710060276,
94.9331934027569));
#137542=CARTESIAN_POINT('Ctrl Pts',(-6.04528905667822,-3.55779691846345,
94.9429420638943));
#137543=CARTESIAN_POINT('Ctrl Pts',(-5.93379832690609,-3.74079274956557,
94.9526907250316));
#137544=CARTESIAN_POINT('Ctrl Pts',(-5.8141078602765,-3.9183895099353,94.962439386169));
#137545=CARTESIAN_POINT('Ctrl Pts',(-5.69474588169057,-4.09549885961964,
94.9721612923048));
#137546=CARTESIAN_POINT('Ctrl Pts',(-5.56722911415492,-4.26723868643634,
94.9818831984406));
#137547=CARTESIAN_POINT('Ctrl Pts',(-5.43200899594852,-4.43293411077069,
94.9916051045764));
#137548=CARTESIAN_POINT('Ctrl Pts',(-5.29768353516487,-4.59753324378936,
95.0012626876248));
#137549=CARTESIAN_POINT('Ctrl Pts',(-5.15575632937569,-4.75616763875545,
95.0109202706731));
#137550=CARTESIAN_POINT('Ctrl Pts',(-5.00671485935146,-4.90820057451296,
95.0205778537215));
#137551=CARTESIAN_POINT('Ctrl Pts',(-4.94120089186002,-4.97502949675336,
95.0248230250941));
#137552=CARTESIAN_POINT('Ctrl Pts',(-4.87431288736589,-5.04058320985438,
95.0290681964667));
#137553=CARTESIAN_POINT('Ctrl Pts',(-4.80609502587495,-5.1048092192324,
95.0333133678393));
#137554=CARTESIAN_POINT('Ctrl Pts',(-4.67991776677221,-5.22360306074709,
95.0411653303094));
#137555=CARTESIAN_POINT('Ctrl Pts',(-4.54924017819775,-5.33780310879539,
95.0490172927794));
#137556=CARTESIAN_POINT('Ctrl Pts',(-4.41444929813963,-5.44704176197086,
95.0568692552495));
#137557=CARTESIAN_POINT('Ctrl Pts',(-4.27969663340054,-5.55624944428256,
95.0647189915657));
#137558=CARTESIAN_POINT('Ctrl Pts',(-4.14083329297538,-5.66049828982078,
95.0725687278818));
#137559=CARTESIAN_POINT('Ctrl Pts',(-3.99828058059538,-5.75945995396564,
95.0804184641979));
#137560=CARTESIAN_POINT('Ctrl Pts',(-3.85573923931381,-5.85841372416864,
95.0882675743588));
#137561=CARTESIAN_POINT('Ctrl Pts',(-3.70950942571087,-5.952080935645,95.0961166845198));
#137562=CARTESIAN_POINT('Ctrl Pts',(-3.56004247387461,-6.04017583739983,
95.1039657946807));
#137563=CARTESIAN_POINT('Ctrl Pts',(-3.41049984157576,-6.12831534475366,
95.1118188791268));
#137564=CARTESIAN_POINT('Ctrl Pts',(-3.25771712513349,-6.21087671102929,
95.1196719635728));
#137565=CARTESIAN_POINT('Ctrl Pts',(-3.10217167429069,-6.28761937983912,
95.1275250480189));
#137566=CARTESIAN_POINT('Ctrl Pts',(-2.94658671213911,-6.36438154265067,
95.135380127288));
#137567=CARTESIAN_POINT('Ctrl Pts',(-2.78823796562709,-6.43532190739377,
95.1432352065571));
#137568=CARTESIAN_POINT('Ctrl Pts',(-2.62762332416813,-6.5002478590272,
95.1510902858262));
#137569=CARTESIAN_POINT('Ctrl Pts',(-2.4668492576413,-6.56523825574577,
95.1589531619968));
#137570=CARTESIAN_POINT('Ctrl Pts',(-2.30380516267747,-6.62420218633519,
95.1668160381675));
#137571=CARTESIAN_POINT('Ctrl Pts',(-2.13900521396493,-6.67699657459331,
95.1746789143381));
#137572=CARTESIAN_POINT('Ctrl Pts',(-2.01812682854345,-6.71572049691133,
95.1804462206006));
#137573=CARTESIAN_POINT('Ctrl Pts',(-1.89630412395199,-6.75112623947254,
95.1862135268632));
#137574=CARTESIAN_POINT('Ctrl Pts',(-1.77374330284097,-6.78317486566039,
95.1919808331257));
#137575=CARTESIAN_POINT('Ctrl Pts',(-1.59570600760469,-6.82973012427239,
95.2003586784964));
#137576=CARTESIAN_POINT('Ctrl Pts',(-1.41571643005545,-6.86930273055412,
95.2087365238672));
#137577=CARTESIAN_POINT('Ctrl Pts',(-1.23434857655575,-6.90173964693358,
95.2171143692379));
#137578=CARTESIAN_POINT('Ctrl Pts',(-1.05310478568801,-6.9341543752067,
95.2254864838382));
#137579=CARTESIAN_POINT('Ctrl Pts',(-0.870484921105141,-6.95944308732083,
95.2338585984384));
#137580=CARTESIAN_POINT('Ctrl Pts',(-0.687074608833712,-6.97750349655205,
95.2422307130386));
#137581=CARTESIAN_POINT('Ctrl Pts',(-0.503762847087054,-6.99555420151535,
95.2505983291116));
#137582=CARTESIAN_POINT('Ctrl Pts',(-0.319661810950971,-7.00638431563548,
95.2589659451846));
#137583=CARTESIAN_POINT('Ctrl Pts',(-0.135364160694557,-7.0099431600049,
95.2673335612576));
#137584=CARTESIAN_POINT('Ctrl Pts',(0.0488614725772959,-7.01350061370418,
95.275697907563));
#137585=CARTESIAN_POINT('Ctrl Pts',(0.233283238565757,-7.00979245737603,
95.2840622538684));
#137586=CARTESIAN_POINT('Ctrl Pts',(0.417306087186306,-6.99882005713086,
95.2924266001739));
#137587=CARTESIAN_POINT('Ctrl Pts',(0.601283974760587,-6.98785033769734,
95.3007889028757));
#137588=CARTESIAN_POINT('Ctrl Pts',(0.784862811519938,-6.96961993374775,
95.3091512055775));
#137589=CARTESIAN_POINT('Ctrl Pts',(0.967449822504712,-6.94418227032065,
95.3175135082792));
#137590=CARTESIAN_POINT('Ctrl Pts',(1.15005142105159,-6.91874257458307,
95.3258764790768));
#137591=CARTESIAN_POINT('Ctrl Pts',(1.33166070912513,-6.88609450834035,
95.3342394498744));
#137592=CARTESIAN_POINT('Ctrl Pts',(1.51169152189781,-6.84634320678728,
95.3426024206719));
#137593=CARTESIAN_POINT('Ctrl Pts',(1.69173462934614,-6.8065891905358,95.350965962594));
#137594=CARTESIAN_POINT('Ctrl Pts',(1.87019872538201,-6.75973104237719,
95.3593295045161));
#137595=CARTESIAN_POINT('Ctrl Pts',(2.04650913221067,-6.70592476354144,
95.3676930464382));
#137596=CARTESIAN_POINT('Ctrl Pts',(2.22285509622956,-6.65210763338883,
95.3760582750676));
#137597=CARTESIAN_POINT('Ctrl Pts',(2.39704619046122,-6.59133967441151,
95.384423503697));
#137598=CARTESIAN_POINT('Ctrl Pts',(2.56852374780163,-6.52382650899601,
95.3927887323264));
#137599=CARTESIAN_POINT('Ctrl Pts',(2.74005876873132,-6.45629071934403,
95.4011567642151));
#137600=CARTESIAN_POINT('Ctrl Pts',(2.90887813371224,-6.38200533641266,
95.4095247961039));
#137601=CARTESIAN_POINT('Ctrl Pts',(3.07444357629574,-6.30122394925572,
95.4178928279926));
#137602=CARTESIAN_POINT('Ctrl Pts',(3.24016260789579,-6.22036762415512,
95.426268622599));
#137603=CARTESIAN_POINT('Ctrl Pts',(3.40262138932765,-6.1330033972065,95.4346444172054));
#137604=CARTESIAN_POINT('Ctrl Pts',(3.56130557271597,-6.03943119674711,
95.4430202118118));
#137605=CARTESIAN_POINT('Ctrl Pts',(3.72006762204644,-5.94581308063694,
95.4514001164002));
#137606=CARTESIAN_POINT('Ctrl Pts',(3.87505109998967,-5.84598108878088,
95.4597800209886));
#137607=CARTESIAN_POINT('Ctrl Pts',(4.02577050543591,-5.74027859951608,
95.468159925577));
#137608=CARTESIAN_POINT('Ctrl Pts',(4.1766622325999,-5.63445525763469,95.4765494111451));
#137609=CARTESIAN_POINT('Ctrl Pts',(4.32327988004096,-5.52274820074212,
95.4849388967131));
#137610=CARTESIAN_POINT('Ctrl Pts',(4.46516985075539,-5.40554204186825,
95.4933283822812));
#137611=CARTESIAN_POINT('Ctrl Pts',(4.55530048958543,-5.33109093076485,
95.4986575094203));
#137612=CARTESIAN_POINT('Ctrl Pts',(4.64352420715487,-5.25442173762011,
95.5039866365594));
#137613=CARTESIAN_POINT('Ctrl Pts',(4.72973243973291,-5.17564079231144,
95.5093157636985));
#137614=CARTESIAN_POINT('Ctrl Pts',(4.86532809813271,-5.05172740458693,
95.5176978692297));
#137615=CARTESIAN_POINT('Ctrl Pts',(4.99620927099563,-4.92233778541204,
95.5260799747609));
#137616=CARTESIAN_POINT('Ctrl Pts',(5.12192216727446,-4.78785336814762,
95.534462080292));
#137617=CARTESIAN_POINT('Ctrl Pts',(5.2474756029481,-4.6535395377299,95.542833553536));
#137618=CARTESIAN_POINT('Ctrl Pts',(5.36787360504213,-4.51414402568894,
95.55120502678));
#137619=CARTESIAN_POINT('Ctrl Pts',(5.48269685785472,-4.37008715329226,
95.5595765000239));
#137620=CARTESIAN_POINT('Ctrl Pts',(5.59738965582937,-4.22619394910285,
95.5679384621352));
#137621=CARTESIAN_POINT('Ctrl Pts',(5.70652012533998,-4.07765019455054,
95.5763004242465));
#137622=CARTESIAN_POINT('Ctrl Pts',(5.80970681905494,-3.92491187660647,
95.5846623863578));
#137623=CARTESIAN_POINT('Ctrl Pts',(5.91275937009221,-3.77237211844001,
95.5930134779204));
#137624=CARTESIAN_POINT('Ctrl Pts',(6.00988337499843,-3.61564894348179,
95.601364569483));
#137625=CARTESIAN_POINT('Ctrl Pts',(6.10073863513935,-3.45523004562911,
95.6097156610455));
#137626=CARTESIAN_POINT('Ctrl Pts',(6.19152385067765,-3.29493482226631,
95.6180603143579));
#137627=CARTESIAN_POINT('Ctrl Pts',(6.27604979176538,-3.13094983776781,
95.6264049676704));
#137628=CARTESIAN_POINT('Ctrl Pts',(6.3540198206988,-2.96379126806644,95.6347496209828));
#137629=CARTESIAN_POINT('Ctrl Pts',(6.43192702679084,-2.79676738314655,
95.6430875507523));
#137630=CARTESIAN_POINT('Ctrl Pts',(6.50328871748195,-2.62657530869652,
95.6514254805219));
#137631=CARTESIAN_POINT('Ctrl Pts',(6.56785435721423,-2.45375542891343,
95.6597634102914));
#137632=CARTESIAN_POINT('Ctrl Pts',(6.58907136859494,-2.39696482989859,
95.662503349856));
#137633=CARTESIAN_POINT('Ctrl Pts',(6.60955487975253,-2.33989065198608,
95.6652432894205));
#137634=CARTESIAN_POINT('Ctrl Pts',(6.62929711484721,-2.28255258988231,
95.6679832289851));
#137635=CARTESIAN_POINT('Ctrl Pts',(6.68657087311171,-2.11621041572944,
95.6759320065944));
#137636=CARTESIAN_POINT('Ctrl Pts',(6.73757578283835,-1.94772267464687,
95.6838807842038));
#137637=CARTESIAN_POINT('Ctrl Pts',(6.78216126708796,-1.77761500604372,
95.6918295618131));
#137638=CARTESIAN_POINT('Ctrl Pts',(6.82677318622033,-1.60740648003483,
95.6997830522793));
#137639=CARTESIAN_POINT('Ctrl Pts',(6.86495798444069,-1.43557646827384,
95.7077365427454));
#137640=CARTESIAN_POINT('Ctrl Pts',(6.89661578464703,-1.26266277424235,
95.7156900332116));
#137641=CARTESIAN_POINT('Ctrl Pts',(6.92828431387029,-1.08969047873084,
95.723646219163));
#137642=CARTESIAN_POINT('Ctrl Pts',(6.95342138408531,-0.915634136736948,
95.7316024051145));
#137643=CARTESIAN_POINT('Ctrl Pts',(6.97197888062647,-0.741037819951529,
95.7395585910659));
#137644=CARTESIAN_POINT('Ctrl Pts',(6.99055419794442,-0.566273838202059,
95.7475224173483));
#137645=CARTESIAN_POINT('Ctrl Pts',(7.0025373003759,-0.390969216497577,
95.7554862436306));
#137646=CARTESIAN_POINT('Ctrl Pts',(7.00793215743705,-0.215669745814628,
95.7634500699129));
#137647=CARTESIAN_POINT('Ctrl Pts',(7.01020925744758,-0.141678086348179,
95.7668114989009));
#137648=CARTESIAN_POINT('Ctrl Pts',(7.01131324795972,-0.0676873138804065,
95.7701729278889));
#137649=CARTESIAN_POINT('Ctrl Pts',(7.01124720379832,0.00626176734413354,
95.7735343568769));
#137650=CARTESIAN_POINT('Ctrl Pts',(7.01124720379766,0.00626176808250687,
95.7735343569104));
#137651=CARTESIAN_POINT('Ctrl Pts',(7.01104753157553,0.229833016751859,
95.783697010235));
#137652=CARTESIAN_POINT('Ctrl Pts',(7.00015032087312,0.453038581417428,
95.7938596635596));
#137653=CARTESIAN_POINT('Ctrl Pts',(6.97868319966095,0.67498693414758,95.8040223168842));
#137654=CARTESIAN_POINT('Ctrl Pts',(6.96275015197189,0.83971855575671,95.8115651093466));
#137655=CARTESIAN_POINT('Ctrl Pts',(6.94099549368888,1.00375802951486,95.819107901809));
#137656=CARTESIAN_POINT('Ctrl Pts',(6.91348882294048,1.16674712666332,95.8266506942714));
#137657=CARTESIAN_POINT('Ctrl Pts',(6.88289091793965,1.34805314353229,95.8350411552369));
#137658=CARTESIAN_POINT('Ctrl Pts',(6.84513049928511,1.52830961949353,95.8434316162024));
#137659=CARTESIAN_POINT('Ctrl Pts',(6.80029542651758,1.70692960446064,95.8518220771679));
#137660=CARTESIAN_POINT('Ctrl Pts',(6.75550718787773,1.88536300533929,95.8602037735682));
#137661=CARTESIAN_POINT('Ctrl Pts',(6.7036591118458,2.06216300663596,95.8685854699685));
#137662=CARTESIAN_POINT('Ctrl Pts',(6.64489020906763,2.23675225984844,95.8769671663687));
#137663=CARTESIAN_POINT('Ctrl Pts',(6.62139804949321,2.3065422066155,95.8803176483419));
#137664=CARTESIAN_POINT('Ctrl Pts',(6.59680058005374,2.37597901091167,95.883668130315));
#137665=CARTESIAN_POINT('Ctrl Pts',(6.57110895151813,2.44502632087639,95.8870186122881));
#137666=CARTESIAN_POINT('',(7.01124998147128,-0.000509724478313664,95.2264656430492));
#137667=CARTESIAN_POINT('Ctrl Pts',(6.57110895151813,2.44502632087639,95.3399143481975));
#137668=CARTESIAN_POINT('Ctrl Pts',(6.63828885140506,2.26447757269324,95.3311708067522));
#137669=CARTESIAN_POINT('Ctrl Pts',(6.69801113786194,2.08119179622191,95.3224272653069));
#137670=CARTESIAN_POINT('Ctrl Pts',(6.75008250258809,1.89578816610774,95.3136837238615));
#137671=CARTESIAN_POINT('Ctrl Pts',(6.80217888112286,1.71029547262937,95.304935982233));
#137672=CARTESIAN_POINT('Ctrl Pts',(6.84661691862439,1.52268315392854,95.2961882406044));
#137673=CARTESIAN_POINT('Ctrl Pts',(6.88325357075376,1.33358420926676,95.2874404989759));
#137674=CARTESIAN_POINT('Ctrl Pts',(6.91989559434719,1.14445753995966,95.2786914748016));
#137675=CARTESIAN_POINT('Ctrl Pts',(6.94873390074258,0.95384407704325,95.2699424506274));
#137676=CARTESIAN_POINT('Ctrl Pts',(6.9696767566655,0.762386037448659,95.2611934264531));
#137677=CARTESIAN_POINT('Ctrl Pts',(6.99062463973899,0.570882040015487,
95.2524423021516));
#137678=CARTESIAN_POINT('Ctrl Pts',(7.003673256796,0.378533331093741,95.2436911778502));
#137679=CARTESIAN_POINT('Ctrl Pts',(7.00878272003862,0.185987488256714,
95.2349400535487));
#137680=CARTESIAN_POINT('Ctrl Pts',(7.01043202006958,0.123834997970955,
95.2321152500623));
#137681=CARTESIAN_POINT('Ctrl Pts',(7.0112545014055,0.0616619882938663,
95.2292904465759));
#137682=CARTESIAN_POINT('Ctrl Pts',(7.01124998147134,-0.000509723591843963,
95.2264656430895));
#137683=CARTESIAN_POINT('Ctrl Pts',(7.01124998147128,-0.000509724478307598,
95.2264656430492));
#137684=CARTESIAN_POINT('Ctrl Pts',(7.0112361212336,-0.191157015833348,
95.2178034859852));
#137685=CARTESIAN_POINT('Ctrl Pts',(7.00344264641733,-0.381774601940022,
95.2091413289212));
#137686=CARTESIAN_POINT('Ctrl Pts',(6.98789830773228,-0.571755020347335,
95.2004791718571));
#137687=CARTESIAN_POINT('Ctrl Pts',(6.97221312830826,-0.763456771714571,
95.1917385306178));
#137688=CARTESIAN_POINT('Ctrl Pts',(6.94863424231851,-0.954522918722355,
95.1829978893785));
#137689=CARTESIAN_POINT('Ctrl Pts',(6.91723779925416,-1.14431105520722,
95.1742572481392));
#137690=CARTESIAN_POINT('Ctrl Pts',(6.885847007391,-1.33406503078608,95.1655181801712));
#137691=CARTESIAN_POINT('Ctrl Pts',(6.8466415132512,-1.52254118520631,95.1567791122032));
#137692=CARTESIAN_POINT('Ctrl Pts',(6.79974892227699,-1.70910536728807,
95.1480400442352));
#137693=CARTESIAN_POINT('Ctrl Pts',(6.75224841453578,-1.89808817227066,
95.1391876827631));
#137694=CARTESIAN_POINT('Ctrl Pts',(6.69686015602426,-2.08510880351682,
95.1303353212911));
#137695=CARTESIAN_POINT('Ctrl Pts',(6.6337698661138,-2.26952063791905,95.1214829598191));
#137696=CARTESIAN_POINT('Ctrl Pts',(6.57151893982451,-2.45147902686511,
95.1127483716239));
#137697=CARTESIAN_POINT('Ctrl Pts',(6.50176975096737,-2.63089734201636,
95.1040137834287));
#137698=CARTESIAN_POINT('Ctrl Pts',(6.42475062516298,-2.80717045563105,
95.0952791952336));
#137699=CARTESIAN_POINT('Ctrl Pts',(6.34617376224076,-2.98700875086897,
95.0863679471231));
#137700=CARTESIAN_POINT('Ctrl Pts',(6.26002985133079,-3.163572988579,95.0774566990127));
#137701=CARTESIAN_POINT('Ctrl Pts',(6.16661307742381,-3.33624185511868,
95.0685454509022));
#137702=CARTESIAN_POINT('Ctrl Pts',(6.07319630351675,-3.50891072165848,
95.0596342027918));
#137703=CARTESIAN_POINT('Ctrl Pts',(5.97250679901631,-3.67768394398257,
95.0507229546813));
#137704=CARTESIAN_POINT('Ctrl Pts',(5.8648891767254,-3.84196583889411,95.0418117065708));
#137705=CARTESIAN_POINT('Ctrl Pts',(5.76796621207698,-3.98992198170726,
95.0337860266943));
#137706=CARTESIAN_POINT('Ctrl Pts',(5.66537871576854,-4.13430281766559,
95.0257603468177));
#137707=CARTESIAN_POINT('Ctrl Pts',(5.5574298503824,-4.27464618659588,95.0177346669411));
#137708=CARTESIAN_POINT('Ctrl Pts',(5.44951524391398,-4.41494501580904,
95.009711534114));
#137709=CARTESIAN_POINT('Ctrl Pts',(5.33624287911491,-4.55120863880943,
95.001688401287));
#137710=CARTESIAN_POINT('Ctrl Pts',(5.21795829983034,-4.68300520432464,
94.9936652684599));
#137711=CARTESIAN_POINT('Ctrl Pts',(5.09968863590153,-4.8147851506603,94.9856431473275));
#137712=CARTESIAN_POINT('Ctrl Pts',(4.97640826162327,-4.94209888916911,
94.9776210261951));
#137713=CARTESIAN_POINT('Ctrl Pts',(4.84850189233173,-5.064548939694,94.9695989050627));
#137714=CARTESIAN_POINT('Ctrl Pts',(4.72054799116709,-5.18704449444433,
94.9615738027931));
#137715=CARTESIAN_POINT('Ctrl Pts',(4.58796492375905,-5.30467249466362,
94.9535487005234));
#137716=CARTESIAN_POINT('Ctrl Pts',(4.45117336090242,-5.4170732202632,94.9455235982538));
#137717=CARTESIAN_POINT('Ctrl Pts',(4.3143548565839,-5.52949608348444,94.9374969154189));
#137718=CARTESIAN_POINT('Ctrl Pts',(4.17332649436964,-5.63668939519169,
94.929470232584));
#137719=CARTESIAN_POINT('Ctrl Pts',(4.02854049785834,-5.7383349518493,94.9214435497491));
#137720=CARTESIAN_POINT('Ctrl Pts',(3.88363826725005,-5.84006210948888,
94.9134104230989));
#137721=CARTESIAN_POINT('Ctrl Pts',(3.73497268268544,-5.93623241388068,
94.9053772964486));
#137722=CARTESIAN_POINT('Ctrl Pts',(3.583023820385,-6.02657173400049,94.8973441697983));
#137723=CARTESIAN_POINT('Ctrl Pts',(3.49349193255858,-6.07980181254685,
94.8926108602937));
#137724=CARTESIAN_POINT('Ctrl Pts',(3.40282062370097,-6.13100832510659,
94.8878775507891));
#137725=CARTESIAN_POINT('Ctrl Pts',(3.31111175468953,-6.18014283900112,
94.8831442412844));
#137726=CARTESIAN_POINT('Ctrl Pts',(3.12218526897516,-6.28136326770599,
94.8733933029058));
#137727=CARTESIAN_POINT('Ctrl Pts',(2.92874330649156,-6.37384810930885,
94.8636423645271));
#137728=CARTESIAN_POINT('Ctrl Pts',(2.73153480288774,-6.45727064502589,
94.8538914261484));
#137729=CARTESIAN_POINT('Ctrl Pts',(2.53404219872951,-6.5408133600872,94.8441264404698));
#137730=CARTESIAN_POINT('Ctrl Pts',(2.33277223520612,-6.61526763987094,
94.8343614547911));
#137731=CARTESIAN_POINT('Ctrl Pts',(2.12849454646976,-6.68035459598879,
94.8245964691125));
#137732=CARTESIAN_POINT('Ctrl Pts',(1.92455734717772,-6.74533306536166,
94.814847759683));
#137733=CARTESIAN_POINT('Ctrl Pts',(1.71762247828284,-6.80097540445833,
94.8050990502535));
#137734=CARTESIAN_POINT('Ctrl Pts',(1.50847251724456,-6.84705317835475,
94.795350340824));
#137735=CARTESIAN_POINT('Ctrl Pts',(1.29989658107158,-6.89300448898136,
94.785628387324));
#137736=CARTESIAN_POINT('Ctrl Pts',(1.08911772839842,-6.92944363071684,
94.775906433824));
#137737=CARTESIAN_POINT('Ctrl Pts',(0.876928290491243,-6.9561931640687,
94.7661844803241));
#137738=CARTESIAN_POINT('Ctrl Pts',(0.666142826622615,-6.98276570628123,
94.7565268531659));
#137739=CARTESIAN_POINT('Ctrl Pts',(0.453965425095591,-6.99977640646644,
94.7468692260078));
#137740=CARTESIAN_POINT('Ctrl Pts',(0.241188204550884,-7.00710031414461,
94.7372115988496));
#137741=CARTESIAN_POINT('Ctrl Pts',(0.147663498942555,-7.01031948538743,
94.732966657899));
#137742=CARTESIAN_POINT('Ctrl Pts',(0.0540231067980854,-7.01166783076978,
94.7287217169485));
#137743=CARTESIAN_POINT('Ctrl Pts',(-0.0396647883031719,-7.01113780117528,
94.7244767759979));
#137744=CARTESIAN_POINT('Ctrl Pts',(-0.212958871141005,-7.01015740779194,
94.7166249276034));
#137745=CARTESIAN_POINT('Ctrl Pts',(-0.386344281524747,-7.00274699430326,
94.708773079209));
#137746=CARTESIAN_POINT('Ctrl Pts',(-0.559287245110139,-6.98890723503733,
94.7009212308145));
#137747=CARTESIAN_POINT('Ctrl Pts',(-0.732181163604306,-6.97507140060443,
94.6930716091346));
#137748=CARTESIAN_POINT('Ctrl Pts',(-0.904632505016229,-6.95480987765999,
94.6852219874547));
#137749=CARTESIAN_POINT('Ctrl Pts',(-1.07610975018039,-6.92817539963205,
94.6773723657749));
#137750=CARTESIAN_POINT('Ctrl Pts',(-1.24757330519985,-6.90154304800787,
94.6695233707814));
#137751=CARTESIAN_POINT('Ctrl Pts',(-1.41806254195812,-6.86853881345922,
94.6616743757879));
#137752=CARTESIAN_POINT('Ctrl Pts',(-1.58705356492891,-6.8292669844242,
94.6538253807944));
#137753=CARTESIAN_POINT('Ctrl Pts',(-1.75613014320212,-6.78997527318982,
94.6459724120802));
#137754=CARTESIAN_POINT('Ctrl Pts',(-1.92370662011442,-6.7444097139101,
94.6381194433659));
#137755=CARTESIAN_POINT('Ctrl Pts',(-2.08927142499908,-6.69272526518027,
94.6302664746516));
#137756=CARTESIAN_POINT('Ctrl Pts',(-2.25487827786347,-6.64102769031138,
94.6224115115433));
#137757=CARTESIAN_POINT('Ctrl Pts',(-2.41847208116772,-6.5832082572014,
94.6145565484349));
#137758=CARTESIAN_POINT('Ctrl Pts',(-2.57955944905294,-6.51947080761174,
94.6067015853266));
#137759=CARTESIAN_POINT('Ctrl Pts',(-2.7408067096049,-6.45567009327998,
94.5988388255113));
#137760=CARTESIAN_POINT('Ctrl Pts',(-2.89954221677495,-6.38593978369819,
94.590976065696));
#137761=CARTESIAN_POINT('Ctrl Pts',(-3.05529495226595,-6.31053082689232,
94.5831133058807));
#137762=CARTESIAN_POINT('Ctrl Pts',(-3.16955273815895,-6.25521198826018,
94.577345307491));
#137763=CARTESIAN_POINT('Ctrl Pts',(-3.28220583407523,-6.19683819014807,
94.5715773091013));
#137764=CARTESIAN_POINT('Ctrl Pts',(-3.39307799138816,-6.13552347455841,
94.5658093107116));
#137765=CARTESIAN_POINT('Ctrl Pts',(-3.55412074151983,-6.04646332941998,
94.5574312440631));
#137766=CARTESIAN_POINT('Ctrl Pts',(-3.71176189921178,-5.95099977948673,
94.5490531774146));
#137767=CARTESIAN_POINT('Ctrl Pts',(-3.86548021925314,-5.8494178545444,
94.540675110766));
#137768=CARTESIAN_POINT('Ctrl Pts',(-4.01909342862906,-5.74790539005234,
94.5323027729348));
#137769=CARTESIAN_POINT('Ctrl Pts',(-4.16878887486382,-5.64028307220438,
94.5239304351035));
#137770=CARTESIAN_POINT('Ctrl Pts',(-4.31407189674095,-5.52688069640099,
94.5155580972722));
#137771=CARTESIAN_POINT('Ctrl Pts',(-4.45927688174548,-5.41353923319868,
94.5071902565325));
#137772=CARTESIAN_POINT('Ctrl Pts',(-4.60007390954955,-5.29442410429784,
94.4988224157929));
#137773=CARTESIAN_POINT('Ctrl Pts',(-4.73599881429735,-5.16990732929267,
94.4904545750532));
#137774=CARTESIAN_POINT('Ctrl Pts',(-4.87187062076578,-5.04543919604686,
94.4820900031622));
#137775=CARTESIAN_POINT('Ctrl Pts',(-5.00287385753673,-4.91557384629412,
94.4737254312712));
#137776=CARTESIAN_POINT('Ctrl Pts',(-5.12857851876945,-4.78072263777314,
94.4653608593803));
#137777=CARTESIAN_POINT('Ctrl Pts',(-5.25425247432167,-4.64590436914542,
94.4569983306901));
#137778=CARTESIAN_POINT('Ctrl Pts',(-5.37463021182608,-4.50610291102031,
94.448635802));
#137779=CARTESIAN_POINT('Ctrl Pts',(-5.48931927309987,-4.36176575259083,
94.4402732733099));
#137780=CARTESIAN_POINT('Ctrl Pts',(-5.60401748697299,-4.21741707553731,
94.4319100772599));
#137781=CARTESIAN_POINT('Ctrl Pts',(-5.71302590843547,-4.06853222859119,
94.42354688121));
#137782=CARTESIAN_POINT('Ctrl Pts',(-5.81599252567866,-3.91559159051987,
94.41518368516));
#137783=CARTESIAN_POINT('Ctrl Pts',(-5.91896616506448,-3.76264052216538,
94.4068199187547));
#137784=CARTESIAN_POINT('Ctrl Pts',(-6.01589699479677,-3.60563338378847,
94.3984561523495));
#137785=CARTESIAN_POINT('Ctrl Pts',(-6.10647639890076,-3.44507946964479,
94.3900923859442));
#137786=CARTESIAN_POINT('Ctrl Pts',(-6.19707405672115,-3.2844932004018,
94.3817269340584));
#137787=CARTESIAN_POINT('Ctrl Pts',(-6.28131757511919,-3.12035901652222,
94.3733614821727));
#137788=CARTESIAN_POINT('Ctrl Pts',(-6.35894415134763,-2.9532111070057,
94.3649960302869));
#137789=CARTESIAN_POINT('Ctrl Pts',(-6.43659672457433,-2.78600721996028,
94.3566277768266));
#137790=CARTESIAN_POINT('Ctrl Pts',(-6.50762779842954,-2.61578789279873,
94.3482595233663));
#137791=CARTESIAN_POINT('Ctrl Pts',(-6.57182242155886,-2.44310798410473,
94.339891269906));
#137792=CARTESIAN_POINT('Ctrl Pts',(-6.63607656226229,-2.27026797649961,
94.3315152578809));
#137793=CARTESIAN_POINT('Ctrl Pts',(-6.69348147161074,-2.09496313711963,
94.3231392458558));
#137794=CARTESIAN_POINT('Ctrl Pts',(-6.743871475126,-1.91776538958285,94.3147632338307));
#137795=CARTESIAN_POINT('Ctrl Pts',(-6.79428619052218,-1.74048074207921,
94.3063831141056));
#137796=CARTESIAN_POINT('Ctrl Pts',(-6.8376790560864,-1.56130165302996,
94.2980029943806));
#137797=CARTESIAN_POINT('Ctrl Pts',(-6.87393525062261,-1.38081162102146,
94.2896228746556));
#137798=CARTESIAN_POINT('Ctrl Pts',(-6.91023287244487,-1.2001153563324,
94.2812331795843));
#137799=CARTESIAN_POINT('Ctrl Pts',(-6.93937747039629,-1.01810547921289,
94.272843484513));
#137800=CARTESIAN_POINT('Ctrl Pts',(-6.96130576314877,-0.835373350336043,
94.2644537894417));
#137801=CARTESIAN_POINT('Ctrl Pts',(-6.97522765034631,-0.719359937239801,
94.259127319674));
#137802=CARTESIAN_POINT('Ctrl Pts',(-6.98624186628942,-0.603055503846008,
94.2538008499063));
#137803=CARTESIAN_POINT('Ctrl Pts',(-6.99434311623776,-0.486611687937667,
94.2484743801386));
#137804=CARTESIAN_POINT('Ctrl Pts',(-7.00709058383352,-0.303385176043139,
94.2400930808086));
#137805=CARTESIAN_POINT('Ctrl Pts',(-7.0126488046885,-0.119443890516184,
94.2317117814786));
#137806=CARTESIAN_POINT('Ctrl Pts',(-7.01095217616346,0.0646231077001102,
94.2233304821486));
#137807=CARTESIAN_POINT('Ctrl Pts',(-7.00925769786619,0.248456827997535,
94.214959804886));
#137808=CARTESIAN_POINT('Ctrl Pts',(-7.00032669678299,0.432415618489739,
94.2065891276235));
#137809=CARTESIAN_POINT('Ctrl Pts',(-6.98414535408088,0.615906028197919,
94.1982184503609));
#137810=CARTESIAN_POINT('Ctrl Pts',(-6.96798237441505,0.79918820790225,
94.189857272375));
#137811=CARTESIAN_POINT('Ctrl Pts',(-6.94458548082508,0.982002741823236,
94.181496094389));
#137812=CARTESIAN_POINT('Ctrl Pts',(-6.91399287360932,1.16375646343191,
94.173134916403));
#137813=CARTESIAN_POINT('Ctrl Pts',(-6.8834399638653,1.34527433841344,94.1647845880196));
#137814=CARTESIAN_POINT('Ctrl Pts',(-6.84571001881183,1.52573382513217,
94.1564342596361));
#137815=CARTESIAN_POINT('Ctrl Pts',(-6.80089297609951,1.70454723904631,
94.1480839312526));
#137816=CARTESIAN_POINT('Ctrl Pts',(-6.75611041737517,1.88322306691632,
94.1397400279388));
#137817=CARTESIAN_POINT('Ctrl Pts',(-6.70425170732731,2.06025502952005,
94.1313961246251));
#137818=CARTESIAN_POINT('Ctrl Pts',(-6.645457971086,2.23506485745482,94.1230522213113));
#137819=CARTESIAN_POINT('Ctrl Pts',(-6.58671145822696,2.40973427738261,
94.1147150198566));
#137820=CARTESIAN_POINT('Ctrl Pts',(-6.52104113237696,2.58218481256943,
94.106377818402));
#137821=CARTESIAN_POINT('Ctrl Pts',(-6.4486381991627,2.75185245585582,94.0980406169473));
#137822=CARTESIAN_POINT('Ctrl Pts',(-6.42480349531027,2.80770624314788,
94.0952960495823));
#137823=CARTESIAN_POINT('Ctrl Pts',(-6.40023958291021,2.86325857395583,
94.0925514822173));
#137824=CARTESIAN_POINT('Ctrl Pts',(-6.37495445485872,2.91848972260946,
94.0898069148523));
#137825=CARTESIAN_POINT('Ctrl Pts',(-6.29813533133327,3.08628829662637,
94.0814686039287));
#137826=CARTESIAN_POINT('Ctrl Pts',(-6.21471876978014,3.25098310266206,
94.0731302930051));
#137827=CARTESIAN_POINT('Ctrl Pts',(-6.12499220819052,3.41205173057289,
94.0647919820815));
#137828=CARTESIAN_POINT('Ctrl Pts',(-6.03520919354575,3.57322169766326,
94.056448424962));
#137829=CARTESIAN_POINT('Ctrl Pts',(-5.93910841956179,3.73076064971112,
94.0481048678425));
#137830=CARTESIAN_POINT('Ctrl Pts',(-5.83702160499475,3.88417370174462,
94.0397613107229));
#137831=CARTESIAN_POINT('Ctrl Pts',(-5.73485712307489,4.03770346998374,
94.0314114058493));
#137832=CARTESIAN_POINT('Ctrl Pts',(-5.62669769781489,4.18710080451423,
94.0230615009756));
#137833=CARTESIAN_POINT('Ctrl Pts',(-5.51291665075698,4.33190218775845,
94.014711596102));
#137834=CARTESIAN_POINT('Ctrl Pts',(-5.3989649403619,4.47692076259944,94.0063491669752));
#137835=CARTESIAN_POINT('Ctrl Pts',(-5.27937496094393,4.61732935273054,
93.9979867378485));
#137836=CARTESIAN_POINT('Ctrl Pts',(-5.15455938017851,4.75269861854439,
93.9896243087217));
#137837=CARTESIAN_POINT('Ctrl Pts',(-5.0296370649608,4.88818364365972,93.9812547285704));
#137838=CARTESIAN_POINT('Ctrl Pts',(-4.89948046325432,5.01862051488014,
93.972885148419));
#137839=CARTESIAN_POINT('Ctrl Pts',(-4.76453734851546,5.14361841674723,
93.9645155682676));
#137840=CARTESIAN_POINT('Ctrl Pts',(-4.62938610035829,5.26880911274574,
93.9561330790521));
#137841=CARTESIAN_POINT('Ctrl Pts',(-4.48943383498332,5.38854386317474,
93.9477505898365));
#137842=CARTESIAN_POINT('Ctrl Pts',(-4.34516057201049,5.50247273195838,
93.939368100621));
#137843=CARTESIAN_POINT('Ctrl Pts',(-4.29795206758839,5.53975206837146,
93.9366252169359));
#137844=CARTESIAN_POINT('Ctrl Pts',(-4.25028113534035,5.57641011894225,
93.9338823332509));
#137845=CARTESIAN_POINT('Ctrl Pts',(-4.20216521516159,5.6124356626144,93.9311394495658));
#137846=CARTESIAN_POINT('Ctrl Pts',(-4.05498959952533,5.72262957658055,
93.9227495945351));
#137847=CARTESIAN_POINT('Ctrl Pts',(-3.90335144205516,5.82712488836485,
93.9143597395044));
#137848=CARTESIAN_POINT('Ctrl Pts',(-3.74771901562641,5.92555725163569,
93.9059698844737));
#137849=CARTESIAN_POINT('Ctrl Pts',(-3.5922302046576,6.02389878287717,93.8975877714857));
#137850=CARTESIAN_POINT('Ctrl Pts',(-3.43275474896218,6.11618834397735,
93.8892056584976));
#137851=CARTESIAN_POINT('Ctrl Pts',(-3.26979150759557,6.20210368015208,
93.8808235455096));
#137852=CARTESIAN_POINT('Ctrl Pts',(-3.10695469120048,6.28795236421656,
93.8724479352666));
#137853=CARTESIAN_POINT('Ctrl Pts',(-2.9406357733876,6.36743652952064,93.8640723250235));
#137854=CARTESIAN_POINT('Ctrl Pts',(-2.77136032176782,6.44027860650694,
93.8556967147804));
#137855=CARTESIAN_POINT('Ctrl Pts',(-2.60219134695188,6.51307486473176,
93.8473263729221));
#137856=CARTESIAN_POINT('Ctrl Pts',(-2.43006984759072,6.57923723554096,
93.8389560310638));
#137857=CARTESIAN_POINT('Ctrl Pts',(-2.25554400260022,6.63853506542175,
93.8305856892055));
#137858=CARTESIAN_POINT('Ctrl Pts',(-2.0811023534555,6.69780428847391,93.8222193854197));
#137859=CARTESIAN_POINT('Ctrl Pts',(-1.90425898244262,6.75021546897039,
93.8138530816339));
#137860=CARTESIAN_POINT('Ctrl Pts',(-1.72558039696885,6.79558671904765,
93.805486777848));
#137861=CARTESIAN_POINT('Ctrl Pts',(-1.54695178291362,6.84094528005129,
93.7971228138841));
#137862=CARTESIAN_POINT('Ctrl Pts',(-1.36648929573607,6.87926775432321,
93.7887588499202));
#137863=CARTESIAN_POINT('Ctrl Pts',(-1.18477343692728,6.9104224520395,93.7803948859562));
#137864=CARTESIAN_POINT('Ctrl Pts',(-1.00308554118196,6.94157235556337,
93.772032209068));
#137865=CARTESIAN_POINT('Ctrl Pts',(-0.820144982193359,6.96555662617638,
93.7636695321797));
#137866=CARTESIAN_POINT('Ctrl Pts',(-0.63654167632221,6.98229484172682,
93.7553068552914));
#137867=CARTESIAN_POINT('Ctrl Pts',(-0.452942150515298,6.99903271266728,
93.7469443505757));
#137868=CARTESIAN_POINT('Ctrl Pts',(-0.26868023236139,7.00852479657975,
93.73858184586));
#137869=CARTESIAN_POINT('Ctrl Pts',(-0.0843506078644922,7.01074258102898,
93.7302193411443));
#137870=CARTESIAN_POINT('Ctrl Pts',(0.0999997914473017,7.01296061543294,
93.721855893935));
#137871=CARTESIAN_POINT('Ctrl Pts',(0.284417583697126,7.00790271241574,
93.7134924467257));
#137872=CARTESIAN_POINT('Ctrl Pts',(0.468307997641202,6.99559248254537,
93.7051289995165));
#137873=CARTESIAN_POINT('Ctrl Pts',(0.65230669144216,6.98327500406481,93.6967606276738));
#137874=CARTESIAN_POINT('Ctrl Pts',(0.835777058083837,6.96369668652283,
93.6883922558312));
#137875=CARTESIAN_POINT('Ctrl Pts',(1.01812831911072,6.93693313275577,93.6800238839885));
#137876=CARTESIAN_POINT('Ctrl Pts',(1.20053421734851,6.91016155992746,93.6716530047626));
#137877=CARTESIAN_POINT('Ctrl Pts',(1.38182001689554,6.87620051104445,93.6632821255368));
#137878=CARTESIAN_POINT('Ctrl Pts',(1.56140433387198,6.83517688642114,93.6549112463109));
#137879=CARTESIAN_POINT('Ctrl Pts',(1.74114081073084,6.79411850291686,93.646533274528));
#137880=CARTESIAN_POINT('Ctrl Pts',(1.91917260489268,6.74598566497688,93.6381553027452));
#137881=CARTESIAN_POINT('Ctrl Pts',(2.09493158789428,6.69095570188166,93.6297773309623));
#137882=CARTESIAN_POINT('Ctrl Pts',(2.2066278814681,6.65598370324884,93.6244530603058));
#137883=CARTESIAN_POINT('Ctrl Pts',(2.31740656456287,6.61822716054034,93.6191287896493));
#137884=CARTESIAN_POINT('Ctrl Pts',(2.42712577899684,6.5777417869227,93.6138045189929));
#137885=CARTESIAN_POINT('Ctrl Pts',(2.58915804863564,6.51795338059584,93.6059416878279));
#137886=CARTESIAN_POINT('Ctrl Pts',(2.74921560712617,6.45208674590067,93.598078856663));
#137887=CARTESIAN_POINT('Ctrl Pts',(2.90678976092369,6.38029778680347,93.5902160254981));
#137888=CARTESIAN_POINT('Ctrl Pts',(3.06424283977971,6.30856398804705,93.5823592358812));
#137889=CARTESIAN_POINT('Ctrl Pts',(3.21921596389303,6.23091707131086,93.5745024462643));
#137890=CARTESIAN_POINT('Ctrl Pts',(3.37121720233194,6.14756221092566,93.5666456566475));
#137891=CARTESIAN_POINT('Ctrl Pts',(3.52313271926429,6.0642543587378,93.5587932978882));
#137892=CARTESIAN_POINT('Ctrl Pts',(3.6720793512138,5.97524514900516,93.5509409391289));
#137893=CARTESIAN_POINT('Ctrl Pts',(3.81758694488272,5.88078706303511,93.5430885803697));
#137894=CARTESIAN_POINT('Ctrl Pts',(3.96306018250727,5.7863512797237,93.5352380756441));
#137895=CARTESIAN_POINT('Ctrl Pts',(4.10509567385016,5.68646938108812,93.5273875709186));
#137896=CARTESIAN_POINT('Ctrl Pts',(4.24324966123014,5.58143878179904,93.5195370661931));
#137897=CARTESIAN_POINT('Ctrl Pts',(4.38138142398535,5.47642507862495,93.5116878243664));
#137898=CARTESIAN_POINT('Ctrl Pts',(4.51563262389453,5.36626455692521,93.5038385825398));
#137899=CARTESIAN_POINT('Ctrl Pts',(4.64559057444722,5.25129648535552,93.4959893407132));
#137900=CARTESIAN_POINT('Ctrl Pts',(4.77559231037527,5.13628967879387,93.4881374543235));
#137901=CARTESIAN_POINT('Ctrl Pts',(4.90129762168367,5.01647234001401,93.4802855679338));
#137902=CARTESIAN_POINT('Ctrl Pts',(5.02232871476421,4.89222248506289,93.4724336815441));
#137903=CARTESIAN_POINT('Ctrl Pts',(5.11120034254362,4.80098736043657,93.4666681389316));
#137904=CARTESIAN_POINT('Ctrl Pts',(5.19755245282571,4.70736313794788,93.4609025963191));
#137905=CARTESIAN_POINT('Ctrl Pts',(5.2812488557258,4.61151136682921,93.4551370537066));
#137906=CARTESIAN_POINT('Ctrl Pts',(5.42169490992746,4.45066809787859,93.4454622327801));
#137907=CARTESIAN_POINT('Ctrl Pts',(5.55459064656223,4.28363423164376,93.4357874118535));
#137908=CARTESIAN_POINT('Ctrl Pts',(5.67948977168029,4.11108531848695,93.4261125909269));
#137909=CARTESIAN_POINT('Ctrl Pts',(5.80493927127263,3.93777605959292,93.4163951374));
#137910=CARTESIAN_POINT('Ctrl Pts',(5.92232155496781,3.75890311672121,93.4066776838731));
#137911=CARTESIAN_POINT('Ctrl Pts',(6.03123283846315,3.57517230504261,93.3969602303463));
#137912=CARTESIAN_POINT('Ctrl Pts',(6.14059089548186,3.39068779678229,93.3872029140906));
#137913=CARTESIAN_POINT('Ctrl Pts',(6.24140831485485,3.20130553418335,93.377445597835));
#137914=CARTESIAN_POINT('Ctrl Pts',(6.33332481320793,3.0077605245273,93.3676882815794));
#137915=CARTESIAN_POINT('Ctrl Pts',(6.420722928028,2.82372970003056,93.3584106104134));
#137916=CARTESIAN_POINT('Ctrl Pts',(6.50007406274316,2.63593551048871,93.3491329392475));
#137917=CARTESIAN_POINT('Ctrl Pts',(6.57110895151818,2.44502632087624,93.3398552680815));
#137918=CARTESIAN_POINT('Origin',(0.,0.,50.));
#137919=CARTESIAN_POINT('',(6.57110895151809,2.44502632087648,91.3398522865014));
#137920=CARTESIAN_POINT('',(6.57110895151815,2.44502632087634,91.8867110819877));
#137921=CARTESIAN_POINT('',(6.57110895151814,2.44502632087636,50.));
#137922=CARTESIAN_POINT('',(7.01124988024546,-0.00129586190521006,93.7735343569429));
#137923=CARTESIAN_POINT('Ctrl Pts',(6.57110895151815,2.44502632087633,91.8867110819877));
#137924=CARTESIAN_POINT('Ctrl Pts',(6.49658038200761,2.64532492137524,91.8964163541283));
#137925=CARTESIAN_POINT('Ctrl Pts',(6.41296961192863,2.84199954216427,91.906121626269));
#137926=CARTESIAN_POINT('Ctrl Pts',(6.32064029350384,3.03432576409253,91.9158268984097));
#137927=CARTESIAN_POINT('Ctrl Pts',(6.22784560331244,3.22762137684042,91.9255810884858));
#137928=CARTESIAN_POINT('Ctrl Pts',(6.12624429569234,3.41652461670562,91.935335278562));
#137929=CARTESIAN_POINT('Ctrl Pts',(6.01624928643395,3.60032930243651,91.9450894686381));
#137930=CARTESIAN_POINT('Ctrl Pts',(5.90613302167974,3.78433660943589,91.9548544114672));
#137931=CARTESIAN_POINT('Ctrl Pts',(5.78760457649126,3.96323409270066,91.9646193542962));
#137932=CARTESIAN_POINT('Ctrl Pts',(5.66112132326098,4.13634282015162,91.9743842971252));
#137933=CARTESIAN_POINT('Ctrl Pts',(5.53479698692768,4.30923404922944,91.9841369710224));
#137934=CARTESIAN_POINT('Ctrl Pts',(5.40053784331265,4.47635103032932,91.9938896449196));
#137935=CARTESIAN_POINT('Ctrl Pts',(5.25884201864718,4.63704724856356,92.0036423188168));
#137936=CARTESIAN_POINT('Ctrl Pts',(5.1862496782191,4.71937370106917,92.0086387216769));
#137937=CARTESIAN_POINT('Ctrl Pts',(5.11170616989284,4.80001542755109,92.013635124537));
#137938=CARTESIAN_POINT('Ctrl Pts',(5.03528278304015,4.87888858832823,92.0186315273972));
#137939=CARTESIAN_POINT('Ctrl Pts',(4.91241187589721,5.00569815818672,92.0266645730022));
#137940=CARTESIAN_POINT('Ctrl Pts',(4.78461915748322,5.12799552921085,92.0346976186072));
#137941=CARTESIAN_POINT('Ctrl Pts',(4.6522770315614,5.24537367440169,92.0427306642123));
#137942=CARTESIAN_POINT('Ctrl Pts',(4.52001998025353,5.36267636440152,92.0507585458663));
#137943=CARTESIAN_POINT('Ctrl Pts',(4.38321961589444,5.4750658809183,92.0587864275203));
#137944=CARTESIAN_POINT('Ctrl Pts',(4.24228557003029,5.58217159399573,92.0668143091743));
#137945=CARTESIAN_POINT('Ctrl Pts',(4.10141515727746,5.68922894778763,92.0748385661606));
#137946=CARTESIAN_POINT('Ctrl Pts',(3.95641507047926,5.79100702698233,92.0828628231469));
#137947=CARTESIAN_POINT('Ctrl Pts',(3.80772838995929,5.887175135054,92.0908870801332));
#137948=CARTESIAN_POINT('Ctrl Pts',(3.65905968717411,5.98333161542145,92.098910366905));
#137949=CARTESIAN_POINT('Ctrl Pts',(3.50670558195138,6.07387927029186,92.1069336536769));
#137950=CARTESIAN_POINT('Ctrl Pts',(3.35113868181342,6.15853035210137,92.1149569404488));
#137951=CARTESIAN_POINT('Ctrl Pts',(3.19558452899533,6.24317449750979,92.1229795697838));
#137952=CARTESIAN_POINT('Ctrl Pts',(3.03681842962385,6.32192286057425,92.1310021991189));
#137953=CARTESIAN_POINT('Ctrl Pts',(2.87533789366954,6.39453349039068,92.139024828454));
#137954=CARTESIAN_POINT('Ctrl Pts',(2.71379665253087,6.46717141663416,92.1470504737265));
#137955=CARTESIAN_POINT('Ctrl Pts',(2.54953927210264,6.53366685261774,92.155076118999));
#137956=CARTESIAN_POINT('Ctrl Pts',(2.38308390612597,6.59382572251219,92.1631017642715));
#137957=CARTESIAN_POINT('Ctrl Pts',(2.2849316798991,6.62929905779812,92.1678341737422));
#137958=CARTESIAN_POINT('Ctrl Pts',(2.18601556914653,6.66257009134217,92.172566583213));
#137959=CARTESIAN_POINT('Ctrl Pts',(2.08644434055908,6.69360714235972,92.1772989926837));
#137960=CARTESIAN_POINT('Ctrl Pts',(1.90276165401402,6.75086232534996,92.1860290414915));
#137961=CARTESIAN_POINT('Ctrl Pts',(1.71675704446937,6.80054131086434,92.1947590902993));
#137962=CARTESIAN_POINT('Ctrl Pts',(1.52905784930129,6.84248556125551,92.203489139107));
#137963=CARTESIAN_POINT('Ctrl Pts',(1.34130438068395,6.8844419398774,92.2122217122189));
#137964=CARTESIAN_POINT('Ctrl Pts',(1.15185561574201,6.91865905944214,92.2209542853308));
#137965=CARTESIAN_POINT('Ctrl Pts',(0.961349496006262,6.94502942463374,
92.2296868584428));
#137966=CARTESIAN_POINT('Ctrl Pts',(0.768136931837252,6.97177442308215,
92.2385434917367));
#137967=CARTESIAN_POINT('Ctrl Pts',(0.573837028173539,6.99044797678191,
92.2474001250306));
#137968=CARTESIAN_POINT('Ctrl Pts',(0.379121580823421,7.00099231462612,
92.2562567583246));
#137969=CARTESIAN_POINT('Ctrl Pts',(0.187011414307042,7.01139556987177,
92.2649948904041));
#137970=CARTESIAN_POINT('Ctrl Pts',(-0.00550296645281556,7.01388580322916,
92.2737330224836));
#137971=CARTESIAN_POINT('Ctrl Pts',(-0.197774497688282,7.00846001704827,
92.2824711545632));
#137972=CARTESIAN_POINT('Ctrl Pts',(-0.393957232669249,7.00292385906611,
92.2913870384643));
#137973=CARTESIAN_POINT('Ctrl Pts',(-0.589886835965058,6.98914617974315,
92.3003029223654));
#137974=CARTESIAN_POINT('Ctrl Pts',(-0.784878401697783,6.96717966303786,
92.3092188062666));
#137975=CARTESIAN_POINT('Ctrl Pts',(-0.979869967430377,6.94521314633259,
92.3181346901677));
#137976=CARTESIAN_POINT('Ctrl Pts',(-1.1739231957695,6.91505783214349,92.3270505740688));
#137977=CARTESIAN_POINT('Ctrl Pts',(-1.36636015085261,6.87682241305256,
92.33596645797));
#137978=CARTESIAN_POINT('Ctrl Pts',(-1.55501567164262,6.83933832950889,
92.3447071425227));
#137979=CARTESIAN_POINT('Ctrl Pts',(-1.74213788700856,6.79408476441352,
92.3534478270754));
#137980=CARTESIAN_POINT('Ctrl Pts',(-1.9270972911706,6.74121076609113,92.3621885116282));
#137981=CARTESIAN_POINT('Ctrl Pts',(-2.11202341806955,6.68834628067759,
92.3709276235869));
#137982=CARTESIAN_POINT('Ctrl Pts',(-2.29478724772302,6.62786417534074,
92.3796667355455));
#137983=CARTESIAN_POINT('Ctrl Pts',(-2.47477335421947,6.55996367427026,
92.3884058475042));
#137984=CARTESIAN_POINT('Ctrl Pts',(-2.65709143800249,6.49118342514963,
92.3972581871503));
#137985=CARTESIAN_POINT('Ctrl Pts',(-2.83655904351329,6.41479128797725,
92.4061105267963));
#137986=CARTESIAN_POINT('Ctrl Pts',(-3.01255500788337,6.33104563930611,
92.4149628664423));
#137987=CARTESIAN_POINT('Ctrl Pts',(-3.18621080600325,6.24841353173985,
92.423697499148));
#137988=CARTESIAN_POINT('Ctrl Pts',(-3.35648646468692,6.15862238644116,
92.4324321318538));
#137989=CARTESIAN_POINT('Ctrl Pts',(-3.52280689856363,6.0619681719663,92.4411667645595));
#137990=CARTESIAN_POINT('Ctrl Pts',(-3.69248930598494,5.96336020530079,
92.4500779576757));
#137991=CARTESIAN_POINT('Ctrl Pts',(-3.85805462312663,5.85760888369109,
92.4589891507919));
#137992=CARTESIAN_POINT('Ctrl Pts',(-4.01891922819944,5.74507744070599,
92.4679003439081));
#137993=CARTESIAN_POINT('Ctrl Pts',(-4.17978383327213,5.63254599772096,
92.4768115370242));
#137994=CARTESIAN_POINT('Ctrl Pts',(-4.33594747016542,5.51323459607686,
92.4857227301405));
#137995=CARTESIAN_POINT('Ctrl Pts',(-4.48685773943029,5.38755363672739,
92.4946339232566));
#137996=CARTESIAN_POINT('Ctrl Pts',(-4.6227716646709,5.27436191958049,92.50265958805));
#137997=CARTESIAN_POINT('Ctrl Pts',(-4.75448655588055,5.15595124616417,
92.5106852528434));
#137998=CARTESIAN_POINT('Ctrl Pts',(-4.8815779151895,5.03267559260819,92.5187109176367));
#137999=CARTESIAN_POINT('Ctrl Pts',(-5.00862893881793,4.9094390637213,92.5267340352809));
#138000=CARTESIAN_POINT('Ctrl Pts',(-5.13105908918112,4.78134088362524,
92.5347571529251));
#138001=CARTESIAN_POINT('Ctrl Pts',(-5.24847882071841,4.64877366957892,
92.5427802705693));
#138002=CARTESIAN_POINT('Ctrl Pts',(-5.36588374459979,4.51622317341866,
92.5508023764281));
#138003=CARTESIAN_POINT('Ctrl Pts',(-5.47827926570231,4.37920504062483,
92.558824482287));
#138004=CARTESIAN_POINT('Ctrl Pts',(-5.58531445970553,4.23814687672624,
92.5668465881458));
#138005=CARTESIAN_POINT('Ctrl Pts',(-5.69238942835092,4.09703629513413,
92.5748716750465));
#138006=CARTESIAN_POINT('Ctrl Pts',(-5.7940998664976,3.95188297381343,92.5828967619471));
#138007=CARTESIAN_POINT('Ctrl Pts',(-5.89013647042712,3.80314592439527,
92.5909218488478));
#138008=CARTESIAN_POINT('Ctrl Pts',(-5.98619198828606,3.6543795819582,92.5989485162492));
#138009=CARTESIAN_POINT('Ctrl Pts',(-6.07657125438079,3.50202841808603,
92.6069751836506));
#138010=CARTESIAN_POINT('Ctrl Pts',(-6.1610098145062,3.34657804750737,92.6150018510521));
#138011=CARTESIAN_POINT('Ctrl Pts',(-6.2455161616141,3.1910028819117,92.6230349622342));
#138012=CARTESIAN_POINT('Ctrl Pts',(-6.32407211074119,3.03232386687623,
92.6310680734163));
#138013=CARTESIAN_POINT('Ctrl Pts',(-6.39646017369505,2.87104925224788,
92.6391011845984));
#138014=CARTESIAN_POINT('Ctrl Pts',(-6.43911385351985,2.77602038290777,
92.6438345859132));
#138015=CARTESIAN_POINT('Ctrl Pts',(-6.47962695837723,2.68009070374381,
92.6485679872279));
#138016=CARTESIAN_POINT('Ctrl Pts',(-6.51796300787231,2.58336694848179,
92.6533013885427));
#138017=CARTESIAN_POINT('Ctrl Pts',(-6.59693645836791,2.38411301390743,
92.6630523420012));
#138018=CARTESIAN_POINT('Ctrl Pts',(-6.66671560835843,2.18137117766134,
92.6728032954596));
#138019=CARTESIAN_POINT('Ctrl Pts',(-6.72706144207604,1.97592280138518,
92.6825542489181));
#138020=CARTESIAN_POINT('Ctrl Pts',(-6.78749421531238,1.77017843809784,
92.6923192504583));
#138021=CARTESIAN_POINT('Ctrl Pts',(-6.83846647645742,1.56171977214095,
92.7020842519984));
#138022=CARTESIAN_POINT('Ctrl Pts',(-6.87978909168864,1.35134326371283,
92.7118492535385));
#138023=CARTESIAN_POINT('Ctrl Pts',(-6.92104283065779,1.1413174094591,92.7215979788386));
#138024=CARTESIAN_POINT('Ctrl Pts',(-6.95267906172259,0.929380138731923,
92.7313467041387));
#138025=CARTESIAN_POINT('Ctrl Pts',(-6.9745602529191,0.716335006055907,
92.7410954294388));
#138026=CARTESIAN_POINT('Ctrl Pts',(-6.99638138871114,0.503874599846359,
92.7508173982596));
#138027=CARTESIAN_POINT('Ctrl Pts',(-7.00850093009097,0.290312441578205,
92.7605393670803));
#138028=CARTESIAN_POINT('Ctrl Pts',(-7.01083312098405,0.0764559494937864,
92.770261335901));
#138029=CARTESIAN_POINT('Ctrl Pts',(-7.01314988037477,-0.135985509638587,
92.7799189769751));
#138030=CARTESIAN_POINT('Ctrl Pts',(-7.00580835251308,-0.348717374046775,
92.7895766180492));
#138031=CARTESIAN_POINT('Ctrl Pts',(-6.98877490237346,-0.560938433747238,
92.7992342591232));
#138032=CARTESIAN_POINT('Ctrl Pts',(-6.98128811609675,-0.654216877302292,
92.8034791240253));
#138033=CARTESIAN_POINT('Ctrl Pts',(-6.97192960369455,-0.747396515695329,
92.8077239889274));
#138034=CARTESIAN_POINT('Ctrl Pts',(-6.96069965522477,-0.840408753080196,
92.8119688538295));
#138035=CARTESIAN_POINT('Ctrl Pts',(-6.93992730107195,-1.01245612628972,
92.8198207008182));
#138036=CARTESIAN_POINT('Ctrl Pts',(-6.91275659676443,-1.18385961718799,
92.827672547807));
#138037=CARTESIAN_POINT('Ctrl Pts',(-6.87924919440198,-1.35408902359475,
92.8355243947958));
#138038=CARTESIAN_POINT('Ctrl Pts',(-6.84575129446743,-1.52427015432067,
92.8433740150644));
#138039=CARTESIAN_POINT('Ctrl Pts',(-6.80592034469012,-1.69327748895823,
92.8512236353329));
#138040=CARTESIAN_POINT('Ctrl Pts',(-6.75986945775756,-1.86058901334403,
92.8590732556015));
#138041=CARTESIAN_POINT('Ctrl Pts',(-6.71382224739865,-2.02788718004698,
92.8669222491784));
#138042=CARTESIAN_POINT('Ctrl Pts',(-6.66155619039601,-2.19348943843175,
92.8747712427553));
#138043=CARTESIAN_POINT('Ctrl Pts',(-6.60323474590385,-2.3568872380723,
92.8826202363322));
#138044=CARTESIAN_POINT('Ctrl Pts',(-6.54488377497063,-2.52036776123838,
92.8904732036249));
#138045=CARTESIAN_POINT('Ctrl Pts',(-6.4804714195939,-2.68164123599705,
92.8983261709177));
#138046=CARTESIAN_POINT('Ctrl Pts',(-6.41021006923355,-2.84021714500789,
92.9061791382104));
#138047=CARTESIAN_POINT('Ctrl Pts',(-6.33993087485026,-2.99883332697316,
92.914034099893));
#138048=CARTESIAN_POINT('Ctrl Pts',(-6.2637998935171,-3.15475023550444,
92.9218890615757));
#138049=CARTESIAN_POINT('Ctrl Pts',(-6.18207600022578,-3.30750100376892,
92.9297440232583));
#138050=CARTESIAN_POINT('Ctrl Pts',(-6.10027098913611,-3.46040338994489,
92.9376067816473));
#138051=CARTESIAN_POINT('Ctrl Pts',(-6.01286217069728,-3.61013302986991,
92.9454695400363));
#138052=CARTESIAN_POINT('Ctrl Pts',(-5.92015266229698,-3.75625065958038,
92.9533322984252));
#138053=CARTESIAN_POINT('Ctrl Pts',(-5.85214229527367,-3.86344045916682,
92.959100305322));
#138054=CARTESIAN_POINT('Ctrl Pts',(-5.78128029462328,-3.96868704918374,
92.9648683122188));
#138055=CARTESIAN_POINT('Ctrl Pts',(-5.70770009220849,-4.0718283632667,
92.9706363191156));
#138056=CARTESIAN_POINT('Ctrl Pts',(-5.60082438494211,-4.22164177134705,
92.9790143854484));
#138057=CARTESIAN_POINT('Ctrl Pts',(-5.48797582339854,-4.36734428812502,
92.9873924517812));
#138058=CARTESIAN_POINT('Ctrl Pts',(-5.36949712189468,-4.50845064522888,
92.995770518114));
#138059=CARTESIAN_POINT('Ctrl Pts',(-5.25109943473359,-4.64946051546518,
93.0041428556236));
#138060=CARTESIAN_POINT('Ctrl Pts',(-5.1270794937273,-4.78588024089271,
93.0125151931331));
#138061=CARTESIAN_POINT('Ctrl Pts',(-4.99782144854968,-4.91725607741928,
93.0208875306427));
#138062=CARTESIAN_POINT('Ctrl Pts',(-4.86863283272206,-5.04856134705058,
93.0292553710554));
#138063=CARTESIAN_POINT('Ctrl Pts',(-4.73421195277145,-5.17482789599279,
93.0376232114681));
#138064=CARTESIAN_POINT('Ctrl Pts',(-4.594981422085,-5.29563709983924,93.0459910518808));
#138065=CARTESIAN_POINT('Ctrl Pts',(-4.4558052810778,-5.4163991102015,93.0543556234403));
#138066=CARTESIAN_POINT('Ctrl Pts',(-4.31182348397202,-5.53170781163574,
93.0627201949999));
#138067=CARTESIAN_POINT('Ctrl Pts',(-4.16349382203865,-5.6411830103575,
93.0710847665595));
#138068=CARTESIAN_POINT('Ctrl Pts',(-4.01520039242536,-5.7506314676953,
93.0794472949145));
#138069=CARTESIAN_POINT('Ctrl Pts',(-3.86256148044469,-5.85424906933691,
93.0878098232696));
#138070=CARTESIAN_POINT('Ctrl Pts',(-3.70606648252838,-5.95169705122663,
93.0961723516246));
#138071=CARTESIAN_POINT('Ctrl Pts',(-3.54955899581629,-6.04915280977349,
93.1045355473359));
#138072=CARTESIAN_POINT('Ctrl Pts',(-3.38919508417897,-6.14043778605298,
93.1128987430472));
#138073=CARTESIAN_POINT('Ctrl Pts',(-3.2254921973847,-6.22525715509893,
93.1212619387584));
#138074=CARTESIAN_POINT('Ctrl Pts',(-3.06177814637423,-6.3100823086597,
93.1296257048233));
#138075=CARTESIAN_POINT('Ctrl Pts',(-2.89472495800528,-6.38844082427534,
93.1379894708881));
#138076=CARTESIAN_POINT('Ctrl Pts',(-2.72487385034963,-6.46008429218852,
93.146353236953));
#138077=CARTESIAN_POINT('Ctrl Pts',(-2.55498851402849,-6.53174219780734,
93.1547186884972));
#138078=CARTESIAN_POINT('Ctrl Pts',(-2.38230443705217,-6.59668222958763,
93.1630841400415));
#138079=CARTESIAN_POINT('Ctrl Pts',(-2.20738233519697,-6.65470433518728,
93.1714495915858));
#138080=CARTESIAN_POINT('Ctrl Pts',(-2.03240165225578,-6.71274587228199,
93.1798178447042));
#138081=CARTESIAN_POINT('Ctrl Pts',(-1.85518176183064,-6.76386475995934,
93.1881860978226));
#138082=CARTESIAN_POINT('Ctrl Pts',(-1.67629844705204,-6.80791084539971,
93.196554350941));
#138083=CARTESIAN_POINT('Ctrl Pts',(-1.4972492818744,-6.8519977678564,93.2049303626261));
#138084=CARTESIAN_POINT('Ctrl Pts',(-1.31653393008176,-6.8889987055489,
93.2133063743111));
#138085=CARTESIAN_POINT('Ctrl Pts',(-1.1347394983527,-6.91881440951976,
93.2216823859962));
#138086=CARTESIAN_POINT('Ctrl Pts',(-0.952855912361967,-6.94864473548453,
93.2300625053821));
#138087=CARTESIAN_POINT('Ctrl Pts',(-0.76989251641903,-6.97128275400893,
93.238442624768));
#138088=CARTESIAN_POINT('Ctrl Pts',(-0.58644210653064,-6.98668105885677,
93.2468227441539));
#138089=CARTESIAN_POINT('Ctrl Pts',(-0.402782081247787,-7.00209695822372,
93.2552124388906));
#138090=CARTESIAN_POINT('Ctrl Pts',(-0.218634258294711,-7.01025659315699,
93.2636021336272));
#138091=CARTESIAN_POINT('Ctrl Pts',(-0.0345933559949973,-7.01116465804513,
93.2719918283639));
#138092=CARTESIAN_POINT('Ctrl Pts',(0.0822510668802292,-7.01174117292014,
93.2773183021388));
#138093=CARTESIAN_POINT('Ctrl Pts',(0.199052410905949,-7.00939580229311,
93.2826447759137));
#138094=CARTESIAN_POINT('Ctrl Pts',(0.315659425914194,-7.00414061033411,
93.2879712496886));
#138095=CARTESIAN_POINT('Ctrl Pts',(0.499142634924546,-6.99587147245649,
93.2963525507695));
#138096=CARTESIAN_POINT('Ctrl Pts',(0.682514584854368,-6.9803784966304,
93.3047338518504));
#138097=CARTESIAN_POINT('Ctrl Pts',(0.865182576579053,-6.95766380846934,
93.3131151529312));
#138098=CARTESIAN_POINT('Ctrl Pts',(1.04761906322595,-6.93497790786761,
93.3214858319335));
#138099=CARTESIAN_POINT('Ctrl Pts',(1.22935304714765,-6.90508857495471,
93.3298565109358));
#138100=CARTESIAN_POINT('Ctrl Pts',(1.40979338409746,-6.86804988163707,
93.3382271899382));
#138101=CARTESIAN_POINT('Ctrl Pts',(1.59002895207705,-6.83105322091158,
93.3465883696492));
#138102=CARTESIAN_POINT('Ctrl Pts',(1.76897348009913,-6.78692343596931,
93.3549495493602));
#138103=CARTESIAN_POINT('Ctrl Pts',(1.94604204955618,-6.73576624474597,
93.3633107290713));
#138104=CARTESIAN_POINT('Ctrl Pts',(2.12288085134561,-6.68467543610281,
93.3716610591506));
#138105=CARTESIAN_POINT('Ctrl Pts',(2.29784823671038,-6.62657550030675,
93.3800113892299));
#138106=CARTESIAN_POINT('Ctrl Pts',(2.47037064399503,-6.56162292758336,
93.3883617193093));
#138107=CARTESIAN_POINT('Ctrl Pts',(2.64276030541053,-6.49672033205339,
93.3967056242996));
#138108=CARTESIAN_POINT('Ctrl Pts',(2.81270843243221,-6.42497572208659,
93.40504952929));
#138109=CARTESIAN_POINT('Ctrl Pts',(2.9796566649287,-6.34659536457509,93.4133934342803));
#138110=CARTESIAN_POINT('Ctrl Pts',(3.14647080324539,-6.26827796280499,
93.4217306373782));
#138111=CARTESIAN_POINT('Ctrl Pts',(3.31028955678935,-6.18333558203157,
93.4300678404761));
#138112=CARTESIAN_POINT('Ctrl Pts',(3.47057445585026,-6.09202261231027,
93.438405043574));
#138113=CARTESIAN_POINT('Ctrl Pts',(3.5233392809322,-6.06196293168356,93.4411496007077));
#138114=CARTESIAN_POINT('Ctrl Pts',(3.57572131606691,-6.03121326287645,
93.4438941578413));
#138115=CARTESIAN_POINT('Ctrl Pts',(3.6277018781199,-5.99978379993691,93.446638714975));
#138116=CARTESIAN_POINT('Ctrl Pts',(3.78562535409396,-5.90429714416836,
93.4549770242474));
#138117=CARTESIAN_POINT('Ctrl Pts',(3.93971164680622,-5.80261084754877,
93.4633153335199));
#138118=CARTESIAN_POINT('Ctrl Pts',(4.08947460582195,-5.69507014977317,
93.4716536427924));
#138119=CARTESIAN_POINT('Ctrl Pts',(4.23933179035607,-5.58746179122176,
93.479997198232));
#138120=CARTESIAN_POINT('Ctrl Pts',(4.38485994949817,-5.4739918756634,93.4883407536717));
#138121=CARTESIAN_POINT('Ctrl Pts',(4.52560533671168,-5.35504648895103,
93.4966843091113));
#138122=CARTESIAN_POINT('Ctrl Pts',(4.66645780220064,-5.23601060927733,
93.5050342122795));
#138123=CARTESIAN_POINT('Ctrl Pts',(4.80251998776185,-5.11149116047647,
93.5133841154478));
#138124=CARTESIAN_POINT('Ctrl Pts',(4.93337406187235,-4.98191197515021,
93.5217340186161));
#138125=CARTESIAN_POINT('Ctrl Pts',(5.06442440724541,-4.85213843079863,
93.5300964460106));
#138126=CARTESIAN_POINT('Ctrl Pts',(5.19025079776647,-4.71729021501269,
93.5384588734052));
#138127=CARTESIAN_POINT('Ctrl Pts',(5.31047385128581,-4.57782634416266,
93.5468213007998));
#138128=CARTESIAN_POINT('Ctrl Pts',(5.43079971182085,-4.43824321278862,
93.5551908792039));
#138129=CARTESIAN_POINT('Ctrl Pts',(5.5455124713578,-4.29403680684988,93.5635604576081));
#138130=CARTESIAN_POINT('Ctrl Pts',(5.65427503039319,-4.14569661735782,
93.5719300360122));
#138131=CARTESIAN_POINT('Ctrl Pts',(5.76320534241099,-3.99712763121534,
93.5803125234703));
#138132=CARTESIAN_POINT('Ctrl Pts',(5.86616693181994,-3.8444123918016,93.5886950109283));
#138133=CARTESIAN_POINT('Ctrl Pts',(5.96286699487306,-3.6880677547943,93.5970774983864));
#138134=CARTESIAN_POINT('Ctrl Pts',(5.99450891739913,-3.63690910261397,
93.5998203923447));
#138135=CARTESIAN_POINT('Ctrl Pts',(6.02548078590497,-3.58536202772217,
93.6025632863031));
#138136=CARTESIAN_POINT('Ctrl Pts',(6.05577344516353,-3.53344513801364,
93.6053061802615));
#138137=CARTESIAN_POINT('Ctrl Pts',(6.15135272838851,-3.36963716515603,
93.6139605488419));
#138138=CARTESIAN_POINT('Ctrl Pts',(6.2403469671373,-3.20183720168851,93.6226149174223));
#138139=CARTESIAN_POINT('Ctrl Pts',(6.32243412465044,-3.03058629673461,
93.6312692860027));
#138140=CARTESIAN_POINT('Ctrl Pts',(6.40442935905294,-2.85952716253222,
93.6399139632196));
#138141=CARTESIAN_POINT('Ctrl Pts',(6.4795328162126,-2.68502505664373,93.6485586404365));
#138142=CARTESIAN_POINT('Ctrl Pts',(6.54746804963009,-2.50764604790492,
93.6572033176535));
#138143=CARTESIAN_POINT('Ctrl Pts',(6.61532939781575,-2.33045995363071,
93.665838593063));
#138144=CARTESIAN_POINT('Ctrl Pts',(6.67603797031742,-2.15040346857582,
93.6744738684725));
#138145=CARTESIAN_POINT('Ctrl Pts',(6.72936485001155,-1.9680638399018,93.683109143882));
#138146=CARTESIAN_POINT('Ctrl Pts',(6.78261394694754,-1.7859901723963,93.6917318238511));
#138147=CARTESIAN_POINT('Ctrl Pts',(6.82850275937022,-1.60164028610003,
93.7003545038201));
#138148=CARTESIAN_POINT('Ctrl Pts',(6.86685172246869,-1.41561788068984,
93.7089771837892));
#138149=CARTESIAN_POINT('Ctrl Pts',(6.90516539300715,-1.22976667174432,
93.7175919283038));
#138150=CARTESIAN_POINT('Ctrl Pts',(6.93595299467261,-1.04224629711538,
93.7262066728184));
#138151=CARTESIAN_POINT('Ctrl Pts',(6.95908526839225,-0.853673702152075,
93.734821417333));
#138152=CARTESIAN_POINT('Ctrl Pts',(6.98218948500649,-0.665329826649574,
93.7434257130349));
#138153=CARTESIAN_POINT('Ctrl Pts',(6.99765686810607,-0.475936565373441,
93.7520300087368));
#138154=CARTESIAN_POINT('Ctrl Pts',(7.00540950305875,-0.286119305455343,
93.7606343044387));
#138155=CARTESIAN_POINT('Ctrl Pts',(7.00928390103963,-0.191257672855264,
93.7649343219293));
#138156=CARTESIAN_POINT('Ctrl Pts',(7.01123232278772,-0.0962902859571281,
93.7692343394198));
#138157=CARTESIAN_POINT('Ctrl Pts',(7.01124988024532,-0.0012958626227105,
93.7735343569104));
#138158=CARTESIAN_POINT('Ctrl Pts',(7.01124988024546,-0.00129586190520921,
93.7735343569429));
#138159=CARTESIAN_POINT('Ctrl Pts',(7.01128650959441,0.196886920880268,
93.7825052986297));
#138160=CARTESIAN_POINT('Ctrl Pts',(7.00291594834133,0.394899238328634,
93.7914762403165));
#138161=CARTESIAN_POINT('Ctrl Pts',(6.98620743083789,0.59205767945829,93.8004471820033));
#138162=CARTESIAN_POINT('Ctrl Pts',(6.9694530897394,0.789756833344971,93.8094427267586));
#138163=CARTESIAN_POINT('Ctrl Pts',(6.9443150481448,0.986597201599815,93.8184382715138));
#138164=CARTESIAN_POINT('Ctrl Pts',(6.91091440251724,1.18190045417529,93.827433816269));
#138165=CARTESIAN_POINT('Ctrl Pts',(6.87747032770891,1.37745764975403,93.836441057479));
#138166=CARTESIAN_POINT('Ctrl Pts',(6.83574222156793,1.5714735175026,93.8454482986889));
#138167=CARTESIAN_POINT('Ctrl Pts',(6.78590204018911,1.7632810506148,93.8544555398989));
#138168=CARTESIAN_POINT('Ctrl Pts',(6.7359867488886,1.9553776406364,93.8634763551602));
#138169=CARTESIAN_POINT('Ctrl Pts',(6.6779349940371,2.14525902654792,93.8724971704215));
#138170=CARTESIAN_POINT('Ctrl Pts',(6.61196886361562,2.33227234882154,93.8815179856828));
#138171=CARTESIAN_POINT('Ctrl Pts',(6.59866972731505,2.36997526768381,93.8833366318719));
#138172=CARTESIAN_POINT('Ctrl Pts',(6.58504907073195,2.40756167627561,93.8851552780611));
#138173=CARTESIAN_POINT('Ctrl Pts',(6.5711089515182,2.44502632087621,93.8869739242502));
#138174=CARTESIAN_POINT('',(7.01125,-3.18920671121825E-12,93.2264656430894));
#138175=CARTESIAN_POINT('Ctrl Pts',(6.57110895151818,2.44502632087624,93.3398552680815));
#138176=CARTESIAN_POINT('Ctrl Pts',(6.64577834864258,2.24434924036419,93.3301029037909));
#138177=CARTESIAN_POINT('Ctrl Pts',(6.71125832242542,2.04023012470171,93.3203505395003));
#138178=CARTESIAN_POINT('Ctrl Pts',(6.76728319995022,1.83344066011736,93.3105981752096));
#138179=CARTESIAN_POINT('Ctrl Pts',(6.79433825794756,1.73357964828215,93.3058886462798));
#138180=CARTESIAN_POINT('Ctrl Pts',(6.81918907502626,1.63309618322025,93.3011791173499));
#138181=CARTESIAN_POINT('Ctrl Pts',(6.84180979817924,1.53207873428182,93.2964695884201));
#138182=CARTESIAN_POINT('Ctrl Pts',(6.8809812374534,1.35715068976432,93.2883142776796));
#138183=CARTESIAN_POINT('Ctrl Pts',(6.91347900255196,1.18054410538854,93.2801589669392));
#138184=CARTESIAN_POINT('Ctrl Pts',(6.93916435907465,1.00280833674639,93.2720036561988));
#138185=CARTESIAN_POINT('Ctrl Pts',(6.9648279033918,0.825223502708336,93.263855271012));
#138186=CARTESIAN_POINT('Ctrl Pts',(6.98369051606048,0.646511743539516,
93.2557068858252));
#138187=CARTESIAN_POINT('Ctrl Pts',(6.99566433661717,0.467233401933904,
93.2475585006385));
#138188=CARTESIAN_POINT('Ctrl Pts',(7.00599612160807,0.312540480804345,
93.2405275481222));
#138189=CARTESIAN_POINT('Ctrl Pts',(7.0111997408877,0.157426046800206,93.2334965956058));
#138190=CARTESIAN_POINT('Ctrl Pts',(7.01124963752017,0.00225452284965846,
93.2264656430895));
#138191=CARTESIAN_POINT('Ctrl Pts',(7.01125,-8.58630487052188E-16,93.2264656430895));
#138192=CARTESIAN_POINT('Ctrl Pts',(7.01125,-0.191009525814093,93.2177938341508));
#138193=CARTESIAN_POINT('Ctrl Pts',(7.00344006572044,-0.382018909627989,
93.209122025212));
#138194=CARTESIAN_POINT('Ctrl Pts',(6.98784625534326,-0.572390840409932,
93.2004502162732));
#138195=CARTESIAN_POINT('Ctrl Pts',(6.97225246786089,-0.762762491687998,
93.1917784200664));
#138196=CARTESIAN_POINT('Ctrl Pts',(6.9488748503355,-0.952496408756031,
93.1831066238596));
#138197=CARTESIAN_POINT('Ctrl Pts',(6.91779140296552,-1.14095953808901,
93.1744348276528));
#138198=CARTESIAN_POINT('Ctrl Pts',(6.88670800059831,-1.32942239456418,
93.165763044001));
#138199=CARTESIAN_POINT('Ctrl Pts',(6.84791883692753,-1.5166141867748,93.1570912603492));
#138200=CARTESIAN_POINT('Ctrl Pts',(6.80155333291357,-1.7019103448867,93.1484194766975));
#138201=CARTESIAN_POINT('Ctrl Pts',(6.75518789508256,-1.88720623850351,
93.139747705424));
#138202=CARTESIAN_POINT('Ctrl Pts',(6.70124620748647,-2.07060622793538,
93.1310759341505));
#138203=CARTESIAN_POINT('Ctrl Pts',(6.63990824732617,-2.25149839653282,
93.122404162877));
#138204=CARTESIAN_POINT('Ctrl Pts',(6.57857037347023,-2.43239031060956,
93.113732403805));
#138205=CARTESIAN_POINT('Ctrl Pts',(6.50983633907283,-2.61077414196143,
93.1050606447329));
#138206=CARTESIAN_POINT('Ctrl Pts',(6.43393547556373,-2.78605471209424,
93.0963888856609));
#138207=CARTESIAN_POINT('Ctrl Pts',(6.35803471730125,-2.96133503917729,
93.0877171386134));
#138208=CARTESIAN_POINT('Ctrl Pts',(6.27496726266285,-3.13351185304551,
93.0790453915659));
#138209=CARTESIAN_POINT('Ctrl Pts',(6.18501026583461,-3.30201068653941,
93.0703736445184));
#138210=CARTESIAN_POINT('Ctrl Pts',(6.09151188668885,-3.47714289831958,
93.0613605124453));
#138211=CARTESIAN_POINT('Ctrl Pts',(5.99057066119227,-3.64830137930906,
93.0523473803723));
#138212=CARTESIAN_POINT('Ctrl Pts',(5.88255038916651,-3.81486926137935,
93.0433342482993));
#138213=CARTESIAN_POINT('Ctrl Pts',(5.77621793389113,-3.97883452029231,
93.034461946415));
#138214=CARTESIAN_POINT('Ctrl Pts',(5.66302622906441,-4.13835132493652,
93.0255896445306));
#138215=CARTESIAN_POINT('Ctrl Pts',(5.54337059052969,-4.2928625715891,93.0167173426462));
#138216=CARTESIAN_POINT('Ctrl Pts',(5.42558457134711,-4.44495958001268,
93.0079836704788));
#138217=CARTESIAN_POINT('Ctrl Pts',(5.30153533575011,-4.59220608124017,
92.9992499983114));
#138218=CARTESIAN_POINT('Ctrl Pts',(5.17164269972391,-4.7341037534989,92.990516326144));
#138219=CARTESIAN_POINT('Ctrl Pts',(5.04265587431657,-4.87501189761919,
92.98184355853));
#138220=CARTESIAN_POINT('Ctrl Pts',(4.907907101642,-5.01064538261891,92.973170790916));
#138221=CARTESIAN_POINT('Ctrl Pts',(4.76784607609309,-5.14055156157233,
92.964498023302));
#138222=CARTESIAN_POINT('Ctrl Pts',(4.62778576967448,-5.27045707353458,
92.9558253002175));
#138223=CARTESIAN_POINT('Ctrl Pts',(4.48241347329876,-5.39463514506421,
92.947152577133));
#138224=CARTESIAN_POINT('Ctrl Pts',(4.33221433005583,-5.51267136340984,
92.9384798540486));
#138225=CARTESIAN_POINT('Ctrl Pts',(4.1820159457358,-5.63070698534468,92.9298071747854));
#138226=CARTESIAN_POINT('Ctrl Pts',(4.02699098676565,-5.74260064062495,
92.9211344955223));
#138227=CARTESIAN_POINT('Ctrl Pts',(3.86765680432031,-5.84797891638597,
92.9124618162592));
#138228=CARTESIAN_POINT('Ctrl Pts',(3.70832341394961,-5.95335666829543,
92.9037891801093));
#138229=CARTESIAN_POINT('Ctrl Pts',(3.54468107996629,-6.05221894875867,
92.8951165439594));
#138230=CARTESIAN_POINT('Ctrl Pts',(3.37727590612964,-6.14423583665017,
92.8864439078095));
#138231=CARTESIAN_POINT('Ctrl Pts',(3.20987155082599,-6.23625227462213,
92.8777713140647));
#138232=CARTESIAN_POINT('Ctrl Pts',(3.03870464148166,-6.32142325013675,
92.8690987203199));
#138233=CARTESIAN_POINT('Ctrl Pts',(2.86434638713045,-6.39946453518048,
92.8604261265751));
#138234=CARTESIAN_POINT('Ctrl Pts',(2.68998897107841,-6.47750544500857,
92.8517535745274));
#138235=CARTESIAN_POINT('Ctrl Pts',(2.51244050005598,-6.54841661688668,
92.8430810224797));
#138236=CARTESIAN_POINT('Ctrl Pts',(2.33229347361078,-6.61196141212671,
92.834408470432));
#138237=CARTESIAN_POINT('Ctrl Pts',(2.15214729859382,-6.67550590703519,
92.8257359593733));
#138238=CARTESIAN_POINT('Ctrl Pts',(1.96940286066775,-6.73168400046379,
92.8170634483147));
#138239=CARTESIAN_POINT('Ctrl Pts',(1.78466999315702,-6.78030822146198,
92.808390937256));
#138240=CARTESIAN_POINT('Ctrl Pts',(1.59993798367215,-6.82893221661602,
92.7997184664784));
#138241=CARTESIAN_POINT('Ctrl Pts',(1.4132178378366,-6.87000233723057,92.7910459957008));
#138242=CARTESIAN_POINT('Ctrl Pts',(1.225132650459,-6.90338153018355,92.7823735249232));
#138243=CARTESIAN_POINT('Ctrl Pts',(1.03704832132761,-6.93676057082487,
92.7737010937188));
#138244=CARTESIAN_POINT('Ctrl Pts',(0.847599242851915,-6.96244870438812,
92.7650286625143));
#138245=CARTESIAN_POINT('Ctrl Pts',(0.657417610666475,-6.98036020902114,
92.7563562313098));
#138246=CARTESIAN_POINT('Ctrl Pts',(0.467236830773526,-6.99827163338436,
92.7476838389706));
#138247=CARTESIAN_POINT('Ctrl Pts',(0.27632378658647,-7.00840647191856,
92.7390114466313));
#138248=CARTESIAN_POINT('Ctrl Pts',(0.0853155533204496,-7.0107309047532,
92.730339054292));
#138249=CARTESIAN_POINT('Ctrl Pts',(-0.105691839535918,-7.01305532736066,
92.7216667001101));
#138250=CARTESIAN_POINT('Ctrl Pts',(-0.296794136562634,-7.00756940957907,
92.7129943459281));
#138251=CARTESIAN_POINT('Ctrl Pts',(-0.487353636615438,-6.99429145770876,
92.7043219917462));
#138252=CARTESIAN_POINT('Ctrl Pts',(-0.677912313783102,-6.98101356317608,
92.6956496750137));
#138253=CARTESIAN_POINT('Ctrl Pts',(-0.867927915269078,-6.95994372163481,
92.6869773582812));
#138254=CARTESIAN_POINT('Ctrl Pts',(-1.05676637166177,-6.93115224174342,
92.6783050415487));
#138255=CARTESIAN_POINT('Ctrl Pts',(-1.24560402801049,-6.90236088383169,
92.6696327615578));
#138256=CARTESIAN_POINT('Ctrl Pts',(-1.43326426841181,-6.86584799585162,
92.660960481567));
#138257=CARTESIAN_POINT('Ctrl Pts',(-1.61912088843801,-6.82173541784814,
92.6522882015762));
#138258=CARTESIAN_POINT('Ctrl Pts',(-1.80497673621847,-6.77762302313515,
92.6436159576192));
#138259=CARTESIAN_POINT('Ctrl Pts',(-1.98902870222556,-6.72591106718967,
92.6349437136622));
#138260=CARTESIAN_POINT('Ctrl Pts',(-2.17066262759971,-6.66677210647266,
92.6262714697052));
#138261=CARTESIAN_POINT('Ctrl Pts',(-2.35229581309404,-6.60763338665627,
92.6175992610743));
#138262=CARTESIAN_POINT('Ctrl Pts',(-2.53151070755523,-6.54106781055567,
92.6089270524434));
#138263=CARTESIAN_POINT('Ctrl Pts',(-2.70770929770595,-6.46729749753456,
92.6002548438126));
#138264=CARTESIAN_POINT('Ctrl Pts',(-2.8839071844938,-6.39352747899536,
92.5915826698));
#138265=CARTESIAN_POINT('Ctrl Pts',(-3.05708852904238,-6.31255289079159,
92.5829104957875));
#138266=CARTESIAN_POINT('Ctrl Pts',(-3.22667545573632,-6.22464393084848,
92.574238321775));
#138267=CARTESIAN_POINT('Ctrl Pts',(-3.39626171929686,-6.13673531465455,
92.5655661816732));
#138268=CARTESIAN_POINT('Ctrl Pts',(-3.56225334094128,-6.04189251170875,
92.5568940415714));
#138269=CARTESIAN_POINT('Ctrl Pts',(-3.72409644021936,-5.94043199325146,
92.5482219014696));
#138270=CARTESIAN_POINT('Ctrl Pts',(-3.88593891984915,-5.83897186325582,
92.5395497945707));
#138271=CARTESIAN_POINT('Ctrl Pts',(-4.04363266822892,-5.73089421932768,
92.5308776876719));
#138272=CARTESIAN_POINT('Ctrl Pts',(-4.19665149725753,-5.61655969193475,
92.5222055807731));
#138273=CARTESIAN_POINT('Ctrl Pts',(-4.34966975290729,-5.50222559296622,
92.5135335063696));
#138274=CARTESIAN_POINT('Ctrl Pts',(-4.49801289671758,-5.38163482746752,
92.5048614319662));
#138275=CARTESIAN_POINT('Ctrl Pts',(-4.64118594512959,-5.25518977632888,
92.4961893575627));
#138276=CARTESIAN_POINT('Ctrl Pts',(-4.78435846873625,-5.12874518867858,
92.487517314947));
#138277=CARTESIAN_POINT('Ctrl Pts',(-4.92236072196935,-4.99644654635426,
92.4788452723313));
#138278=CARTESIAN_POINT('Ctrl Pts',(-5.05473222957939,-4.85873529323746,
92.4701732297156));
#138279=CARTESIAN_POINT('Ctrl Pts',(-5.18710326277656,-4.72102453367094,
92.4615012181801));
#138280=CARTESIAN_POINT('Ctrl Pts',(-5.31384339389981,-4.57790140690441,
92.4528292066446));
#138281=CARTESIAN_POINT('Ctrl Pts',(-5.4345297293063,-4.42984347170259,
92.4441571951091));
#138282=CARTESIAN_POINT('Ctrl Pts',(-5.55521564202443,-4.28178605505461,
92.4354852139461));
#138283=CARTESIAN_POINT('Ctrl Pts',(-5.66984762199887,-4.12879408471371,
92.4268132327832));
#138284=CARTESIAN_POINT('Ctrl Pts',(-5.77804317951667,-3.97137804523077,
92.4181412516203));
#138285=CARTESIAN_POINT('Ctrl Pts',(-5.88623836691936,-3.81396254423625,
92.4094693001225));
#138286=CARTESIAN_POINT('Ctrl Pts',(-5.98799701504499,-3.65212323845223,
92.4007973486246));
#138287=CARTESIAN_POINT('Ctrl Pts',(-6.08297959063156,-3.48640012942575,
92.3921253971268));
#138288=CARTESIAN_POINT('Ctrl Pts',(-6.17796184905024,-3.32067757378551,
92.3834534745866));
#138289=CARTESIAN_POINT('Ctrl Pts',(-6.26616793897712,-3.15107148727182,
92.3747815520463));
#138290=CARTESIAN_POINT('Ctrl Pts',(-6.34730354929289,-2.97814778270553,
92.366109629506));
#138291=CARTESIAN_POINT('Ctrl Pts',(-6.42843889529735,-2.80522464146391,
92.3574377352158));
#138292=CARTESIAN_POINT('Ctrl Pts',(-6.50250368714197,-2.62898416091716,
92.3487658409257));
#138293=CARTESIAN_POINT('Ctrl Pts',(-6.56925079960071,-2.45001438657929,
92.3400939466355));
#138294=CARTESIAN_POINT('Ctrl Pts',(-6.63599770006526,-2.2710451806638,
92.3314220798879));
#138295=CARTESIAN_POINT('Ctrl Pts',(-6.69542686840775,-2.08934696441046,
92.3227502131404));
#138296=CARTESIAN_POINT('Ctrl Pts',(-6.74734001400864,-1.90552598981435,
92.3140783463928));
#138297=CARTESIAN_POINT('Ctrl Pts',(-6.79925299896378,-1.72170558405405,
92.3054065064805));
#138298=CARTESIAN_POINT('Ctrl Pts',(-6.84364993053219,-1.53576270641256,
92.2967346665681));
#138299=CARTESIAN_POINT('Ctrl Pts',(-6.88038267538334,-1.34831776773313,
92.2880628266557));
#138300=CARTESIAN_POINT('Ctrl Pts',(-6.9171153095606,-1.16087339381573,
92.2793910128712));
#138301=CARTESIAN_POINT('Ctrl Pts',(-6.94618374861392,-0.97192724661815,
92.2707191990866));
#138302=CARTESIAN_POINT('Ctrl Pts',(-6.96749100433676,-0.782109753798213,
92.2620473853021));
#138303=CARTESIAN_POINT('Ctrl Pts',(-6.98879819759995,-0.592292817405416,
92.2533755969379));
#138304=CARTESIAN_POINT('Ctrl Pts',(-7.00234422137961,-0.401604822727352,
92.2447038085737));
#138305=CARTESIAN_POINT('Ctrl Pts',(-7.00808387899853,-0.210682005451052,
92.2360320202095));
#138306=CARTESIAN_POINT('Ctrl Pts',(-7.01382352026045,-0.0197597322708364,
92.2273602565584));
#138307=CARTESIAN_POINT('Ctrl Pts',(-7.01175683134601,0.171397078302522,
92.2186884929072));
#138308=CARTESIAN_POINT('Ctrl Pts',(-7.0018907077798,0.362150629996567,
92.2100167292561));
#138309=CARTESIAN_POINT('Ctrl Pts',(-6.99157808297275,0.561536923511939,
92.2009525163108));
#138310=CARTESIAN_POINT('Ctrl Pts',(-6.97274368607562,0.760482277942609,
92.1918883033654));
#138311=CARTESIAN_POINT('Ctrl Pts',(-6.94545616842847,0.958261537858469,
92.18282409042));
#138312=CARTESIAN_POINT('Ctrl Pts',(-6.9190213857078,1.14986019590195,92.1740431341292));
#138313=CARTESIAN_POINT('Ctrl Pts',(-6.88465388689334,1.34036422799403,
92.1652621778384));
#138314=CARTESIAN_POINT('Ctrl Pts',(-6.84247124235282,1.52912192452881,
92.1564812215476));
#138315=CARTESIAN_POINT('Ctrl Pts',(-6.80080846652355,1.71555332735902,
92.1478084838021));
#138316=CARTESIAN_POINT('Ctrl Pts',(-6.75152215882579,1.90028091508477,
92.1391357460566));
#138317=CARTESIAN_POINT('Ctrl Pts',(-6.69477680033991,2.08268820425202,
92.1304630083111));
#138318=CARTESIAN_POINT('Ctrl Pts',(-6.63803201373192,2.26509365512451,
92.1217903579692));
#138319=CARTESIAN_POINT('Ctrl Pts',(-6.57382841116713,2.44517858291517,
92.1131177076273));
#138320=CARTESIAN_POINT('Ctrl Pts',(-6.50238025225981,2.62234201002114,
92.1044450572853));
#138321=CARTESIAN_POINT('Ctrl Pts',(-6.43093279007748,2.79950370952224,
92.0957724915146));
#138322=CARTESIAN_POINT('Ctrl Pts',(-6.35224101919017,2.9737437018412,92.0870999257438));
#138323=CARTESIAN_POINT('Ctrl Pts',(-6.26656754386472,3.14448052636383,
92.078427359973));
#138324=CARTESIAN_POINT('Ctrl Pts',(-6.18089487601242,3.31521574169059,
92.0697548759412));
#138325=CARTESIAN_POINT('Ctrl Pts',(-6.08824076282263,3.48244760135376,
92.0610823919095));
#138326=CARTESIAN_POINT('Ctrl Pts',(-5.98891439681958,3.64561804226213,
92.0524099078777));
#138327=CARTESIAN_POINT('Ctrl Pts',(-5.8895889345435,3.80878699855434,92.043737502753));
#138328=CARTESIAN_POINT('Ctrl Pts',(-5.78359148866046,3.96789436736264,
92.0350650976284));
#138329=CARTESIAN_POINT('Ctrl Pts',(-5.67127577279352,4.12240920717792,
92.0263926925037));
#138330=CARTESIAN_POINT('Ctrl Pts',(-5.5589610421754,4.2769226915679,92.0177203634546));
#138331=CARTESIAN_POINT('Ctrl Pts',(-5.44032831952011,4.42684349778707,
92.0090480344055));
#138332=CARTESIAN_POINT('Ctrl Pts',(-5.31577347544833,4.5716713486667,92.0003757053563));
#138333=CARTESIAN_POINT('Ctrl Pts',(-5.19121968333364,4.71649797636881,
91.9917034495514));
#138334=CARTESIAN_POINT('Ctrl Pts',(-5.06074405512288,4.85623151942534,
91.9830311937464));
#138335=CARTESIAN_POINT('Ctrl Pts',(-4.92478197318928,4.99040570285121,
91.9743589379415));
#138336=CARTESIAN_POINT('Ctrl Pts',(-4.78882099517989,5.12457879686946,
91.9656867525496));
#138337=CARTESIAN_POINT('Ctrl Pts',(-4.64737385477933,5.25319242205283,
91.9570145671578));
#138338=CARTESIAN_POINT('Ctrl Pts',(-4.50091253739581,5.37581741628315,
91.948342381766));
#138339=CARTESIAN_POINT('Ctrl Pts',(-4.35445236138386,5.49844145489813,
91.9396702639564));
#138340=CARTESIAN_POINT('Ctrl Pts',(-4.20297830437918,5.61507677359995,
91.9309981461468));
#138341=CARTESIAN_POINT('Ctrl Pts',(-4.04699580206075,5.72533418593209,
91.9223260283372));
#138342=CARTESIAN_POINT('Ctrl Pts',(-3.89101446440852,5.83559077501111,
91.9136539752793));
#138343=CARTESIAN_POINT('Ctrl Pts',(-3.73052498075346,5.93946938906208,
91.9049819222213));
#138344=CARTESIAN_POINT('Ctrl Pts',(-3.56606286128534,6.03662341312272,
91.8963098691634));
#138345=CARTESIAN_POINT('Ctrl Pts',(-3.40160191612949,6.13377674347248,
91.8876378780267));
#138346=CARTESIAN_POINT('Ctrl Pts',(-3.23316863647378,6.22420543545133,
91.87896588689));
#138347=CARTESIAN_POINT('Ctrl Pts',(-3.06132503079821,6.30760775716978,
91.8702938957532));
#138348=CARTESIAN_POINT('Ctrl Pts',(-2.88948259606764,6.39100951058351,
91.8616219637076));
#138349=CARTESIAN_POINT('Ctrl Pts',(-2.71423013733803,6.46738486553202,
91.852950031662));
#138350=CARTESIAN_POINT('Ctrl Pts',(-2.53615240856791,6.53647898512764,
91.8442780996164));
#138351=CARTESIAN_POINT('Ctrl Pts',(-2.35807583511654,6.60557265645983,
91.8356062238318));
#138352=CARTESIAN_POINT('Ctrl Pts',(-2.17717429308594,6.66738508423325,
91.8269343480473));
#138353=CARTESIAN_POINT('Ctrl Pts',(-1.99405137755473,6.72171002544532,
91.8182624722627));
#138354=CARTESIAN_POINT('Ctrl Pts',(-1.81092959032606,6.77603463193701,
91.8095906499095));
#138355=CARTESIAN_POINT('Ctrl Pts',(-1.62558672926246,6.82287176341268,
91.8009188275563));
#138356=CARTESIAN_POINT('Ctrl Pts',(-1.4386412007099,6.86206514528389,91.7922470052031));
#138357=CARTESIAN_POINT('Ctrl Pts',(-1.25169676301938,6.9012582984544,91.7835752334516));
#138358=CARTESIAN_POINT('Ctrl Pts',(-1.0631499545079,6.93280773300174,91.7749034617));
#138359=CARTESIAN_POINT('Ctrl Pts',(-0.873629864328629,6.95660818378131,
91.7662316899485));
#138360=CARTESIAN_POINT('Ctrl Pts',(-0.679495509715768,6.98098810649672,
91.75734878571));
#138361=CARTESIAN_POINT('Ctrl Pts',(-0.484340182090771,6.99723686027455,
91.7484658814715));
#138362=CARTESIAN_POINT('Ctrl Pts',(-0.28884707897545,7.00529756166484,
91.7395829772331));
#138363=CARTESIAN_POINT('Ctrl Pts',(-0.0979805524009829,7.01316749698021,
91.7309102974767));
#138364=CARTESIAN_POINT('Ctrl Pts',(0.0932076478825197,7.01323255451612,
91.7222376177204));
#138365=CARTESIAN_POINT('Ctrl Pts',(0.284079486219721,7.00549251716174,
91.713564937964));
#138366=CARTESIAN_POINT('Ctrl Pts',(0.474947621911345,6.99775262995322,
91.7048924264455));
#138367=CARTESIAN_POINT('Ctrl Pts',(0.665499124046936,6.98220796234753,
91.696219914927));
#138368=CARTESIAN_POINT('Ctrl Pts',(0.8550981064148,6.95891038819339,91.6875474034084));
#138369=CARTESIAN_POINT('Ctrl Pts',(1.04469365841117,6.93561323555699,91.6788750487997));
#138370=CARTESIAN_POINT('Ctrl Pts',(1.23333644314947,6.90456349171743,91.6702026941909));
#138371=CARTESIAN_POINT('Ctrl Pts',(1.42039696672311,6.86586476850686,91.6615303395822));
#138372=CARTESIAN_POINT('Ctrl Pts',(1.60745435008797,6.82716669493668,91.6528581305574));
#138373=CARTESIAN_POINT('Ctrl Pts',(1.79292924725796,6.78081995649467,91.6441859215325));
#138374=CARTESIAN_POINT('Ctrl Pts',(1.97620275620757,6.72697920532371,91.6355137125077));
#138375=CARTESIAN_POINT('Ctrl Pts',(2.15947342778161,6.6731392876962,91.6268416377429));
#138376=CARTESIAN_POINT('Ctrl Pts',(2.34054250680113,6.61180566956913,91.6181695629782));
#138377=CARTESIAN_POINT('Ctrl Pts',(2.51880581148678,6.54318300573356,91.6094974882134));
#138378=CARTESIAN_POINT('Ctrl Pts',(2.69706658905564,6.4745613147145,91.6008255363867));
#138379=CARTESIAN_POINT('Ctrl Pts',(2.8725214068172,6.39865088680221,91.59215358456));
#138380=CARTESIAN_POINT('Ctrl Pts',(3.04458483294605,6.31570500874565,91.5834816327333));
#138381=CARTESIAN_POINT('Ctrl Pts',(3.21664604442544,6.23276019829566,91.5748097925244));
#138382=CARTESIAN_POINT('Ctrl Pts',(3.38531569578618,6.14278024223886,91.5661379523154));
#138383=CARTESIAN_POINT('Ctrl Pts',(3.5500310094209,6.04606536473516,91.5574661121065));
#138384=CARTESIAN_POINT('Ctrl Pts',(3.72225670715908,5.94494066119559,91.5483988693729));
#138385=CARTESIAN_POINT('Ctrl Pts',(3.89015872998488,5.83645264819735,91.5393316266394));
#138386=CARTESIAN_POINT('Ctrl Pts',(4.05312466659709,5.720997028449,91.5302643839058));
#138387=CARTESIAN_POINT('Ctrl Pts',(4.20899688867883,5.61056705531404,91.5215918275274));
#138388=CARTESIAN_POINT('Ctrl Pts',(4.36035338103765,5.49376336253727,91.512919271149));
#138389=CARTESIAN_POINT('Ctrl Pts',(4.50668904924943,5.37097573778501,91.5042467147705));
#138390=CARTESIAN_POINT('Ctrl Pts',(4.65301950883977,5.24819248349324,91.4955744670801));
#138391=CARTESIAN_POINT('Ctrl Pts',(4.79432928426883,5.11942590604071,91.4869022193897));
#138392=CARTESIAN_POINT('Ctrl Pts',(4.9301468417244,4.98510568408884,91.4782299716992));
#138393=CARTESIAN_POINT('Ctrl Pts',(5.0659602741979,4.85078954164274,91.4695579873979));
#138394=CARTESIAN_POINT('Ctrl Pts',(5.19628162053371,4.71092029195627,91.4608860030966));
#138395=CARTESIAN_POINT('Ctrl Pts',(5.320676040381,4.56596463365799,91.4522140187952));
#138396=CARTESIAN_POINT('Ctrl Pts',(5.44506733164305,4.42101262107094,91.4435422525989));
#138397=CARTESIAN_POINT('Ctrl Pts',(5.56353180975597,4.27097467138689,91.4348704864025));
#138398=CARTESIAN_POINT('Ctrl Pts',(5.67567421678132,4.11635138775393,91.4261987202062));
#138399=CARTESIAN_POINT('Ctrl Pts',(5.78782406006072,3.96171785092552,91.417526378978));
#138400=CARTESIAN_POINT('Ctrl Pts',(5.8936508265424,3.80249860162444,91.4088540377498));
#138401=CARTESIAN_POINT('Ctrl Pts',(5.99280137735924,3.63922494688377,91.4001816965216));
#138402=CARTESIAN_POINT('Ctrl Pts',(6.09194609290829,3.47596090122234,91.3915098656832));
#138403=CARTESIAN_POINT('Ctrl Pts',(6.18441523160457,3.30864317036824,91.3828380348449));
#138404=CARTESIAN_POINT('Ctrl Pts',(6.26990026462943,3.13783001995007,91.3741662040065));
#138405=CARTESIAN_POINT('Ctrl Pts',(6.35538670852376,2.96701405038272,91.3654942300457));
#138406=CARTESIAN_POINT('Ctrl Pts',(6.43388868897021,2.79270279979631,91.356822256085));
#138407=CARTESIAN_POINT('Ctrl Pts',(6.50514427077279,2.61547788729554,91.3481502821243));
#138408=CARTESIAN_POINT('Ctrl Pts',(6.52787183386205,2.55895052090607,91.3453842835833));
#138409=CARTESIAN_POINT('Ctrl Pts',(6.54986255129711,2.50212689664026,91.3426182850423));
#138410=CARTESIAN_POINT('Ctrl Pts',(6.5711089515181,2.44502632087648,91.3398522865014));
#138411=CARTESIAN_POINT('Origin',(0.,0.,50.));
#138412=CARTESIAN_POINT('',(6.57110895151813,2.4450263208764,89.3398405407985));
#138413=CARTESIAN_POINT('',(6.57110895151814,2.44502632087636,89.8869836046549));
#138414=CARTESIAN_POINT('',(6.57110895151814,2.44502632087636,50.));
#138415=CARTESIAN_POINT('',(7.01124941011649,-0.00287604611295131,91.7735343569377));
#138416=CARTESIAN_POINT('Ctrl Pts',(6.57110895151814,2.44502632087636,89.8869836046549));
#138417=CARTESIAN_POINT('Ctrl Pts',(6.50935320916737,2.61099742225222,89.8950062778613));
#138418=CARTESIAN_POINT('Ctrl Pts',(6.44129983113049,2.77464205694512,89.9030289510676));
#138419=CARTESIAN_POINT('Ctrl Pts',(6.36716265085894,2.93544993825598,89.911051624274));
#138420=CARTESIAN_POINT('Ctrl Pts',(6.29299667694928,3.09632027465242,89.9190774133522));
#138421=CARTESIAN_POINT('Ctrl Pts',(6.21274233312392,3.25435132291618,89.9271032024303));
#138422=CARTESIAN_POINT('Ctrl Pts',(6.12666066204817,3.40905495623222,89.9351289915085));
#138423=CARTESIAN_POINT('Ctrl Pts',(6.05220514875705,3.54286437561966,89.9420708205635));
#138424=CARTESIAN_POINT('Ctrl Pts',(5.97339090098604,3.67418472505594,89.9490126496185));
#138425=CARTESIAN_POINT('Ctrl Pts',(5.89041361735242,3.80271665773421,89.9559544786736));
#138426=CARTESIAN_POINT('Ctrl Pts',(5.78606133029722,3.96435850170953,89.9646845275077));
#138427=CARTESIAN_POINT('Ctrl Pts',(5.67507237409969,4.12167082861515,89.9734145763418));
#138428=CARTESIAN_POINT('Ctrl Pts',(5.55782685638255,4.27412999298956,89.9821446251758));
#138429=CARTESIAN_POINT('Ctrl Pts',(5.44054743697799,4.42663324112115,89.9908771983144));
#138430=CARTESIAN_POINT('Ctrl Pts',(5.3170080120053,4.57428030850853,89.999609771453));
#138431=CARTESIAN_POINT('Ctrl Pts',(5.18762953254229,4.71657994691017,90.0083423445916));
#138432=CARTESIAN_POINT('Ctrl Pts',(5.05641302523873,4.86090117884241,90.0171989778723));
#138433=CARTESIAN_POINT('Ctrl Pts',(4.91919048779769,4.99972167181726,90.026055611153));
#138434=CARTESIAN_POINT('Ctrl Pts',(4.77644072202909,5.13256666702365,90.0349122444337));
#138435=CARTESIAN_POINT('Ctrl Pts',(4.63560093879798,5.26363420487541,90.0436503765398));
#138436=CARTESIAN_POINT('Ctrl Pts',(4.48938113570517,5.38888498318307,90.052388508646));
#138437=CARTESIAN_POINT('Ctrl Pts',(4.33827621682943,5.50790214410098,90.0611266407522));
#138438=CARTESIAN_POINT('Ctrl Pts',(4.18409750996103,5.62934036134764,90.0700425246201));
#138439=CARTESIAN_POINT('Ctrl Pts',(4.02483304198778,5.74428844896389,90.0789584084881));
#138440=CARTESIAN_POINT('Ctrl Pts',(3.86104244637359,5.85234805781419,90.0878742923561));
#138441=CARTESIAN_POINT('Ctrl Pts',(3.69725185075939,5.96040766666449,90.096790176224));
#138442=CARTESIAN_POINT('Ctrl Pts',(3.52893538328009,6.06157863529025,90.105706060092));
#138443=CARTESIAN_POINT('Ctrl Pts',(3.3566832089298,6.15551008425693,90.11462194396));
#138444=CARTESIAN_POINT('Ctrl Pts',(3.18781583334146,6.24759575651066,90.1233626284565));
#138445=CARTESIAN_POINT('Ctrl Pts',(3.01514805499685,6.33273356532304,90.132103312953));
#138446=CARTESIAN_POINT('Ctrl Pts',(2.83925870842748,6.41063464480068,90.1408439974495));
#138447=CARTESIAN_POINT('Ctrl Pts',(2.6634010072735,6.48852170858,90.1495831093516));
#138448=CARTESIAN_POINT('Ctrl Pts',(2.48432314567789,6.55917453239809,90.1583222212538));
#138449=CARTESIAN_POINT('Ctrl Pts',(2.30262529376874,6.62235179668042,90.167061333156));
#138450=CARTESIAN_POINT('Ctrl Pts',(2.11857328468781,6.68634761334651,90.1759136728302));
#138451=CARTESIAN_POINT('Ctrl Pts',(1.93183318235458,6.74267269200077,90.1847660125044));
#138452=CARTESIAN_POINT('Ctrl Pts',(1.74304745914586,6.79112745556032,90.1936183521786));
#138453=CARTESIAN_POINT('Ctrl Pts',(1.55677196560573,6.8389379300126,90.2023529848286));
#138454=CARTESIAN_POINT('Ctrl Pts',(1.36850518901057,6.87908603184949,90.2110876174787));
#138455=CARTESIAN_POINT('Ctrl Pts',(1.17887830695027,6.91143056826169,90.2198222501287));
#138456=CARTESIAN_POINT('Ctrl Pts',(0.98541833592894,6.9444289122149,90.228733443315));
#138457=CARTESIAN_POINT('Ctrl Pts',(0.790542970481775,6.96930478037468,
90.2376446365013));
#138458=CARTESIAN_POINT('Ctrl Pts',(0.59493303747742,6.98596315789154,90.2465558296876));
#138459=CARTESIAN_POINT('Ctrl Pts',(0.399323104473196,7.00262153540839,
90.2554670228739));
#138460=CARTESIAN_POINT('Ctrl Pts',(0.202978904804958,7.01106238313513,
90.2643782160602));
#138461=CARTESIAN_POINT('Ctrl Pts',(0.00658751125685207,7.01124690530832,
90.2732894092465));
#138462=CARTESIAN_POINT('Ctrl Pts',(-0.170287961144518,7.01141309103551,
90.2813150740988));
#138463=CARTESIAN_POINT('Ctrl Pts',(-0.347283000346827,7.00488188201528,
90.2893407389511));
#138464=CARTESIAN_POINT('Ctrl Pts',(-0.52384488805084,6.99165310178952,
90.2973664038034));
#138465=CARTESIAN_POINT('Ctrl Pts',(-0.700350739342428,6.97842852005412,
90.3053895215065));
#138466=CARTESIAN_POINT('Ctrl Pts',(-0.876423347717666,6.95851062642809,
90.3134126392096));
#138467=CARTESIAN_POINT('Ctrl Pts',(-1.05151207542466,6.9319513066478,90.3214357569127));
#138468=CARTESIAN_POINT('Ctrl Pts',(-1.22657872291005,6.90539533623028,
90.3294578628304));
#138469=CARTESIAN_POINT('Ctrl Pts',(-1.4006613746394,6.8721996634916,90.3374799687481));
#138470=CARTESIAN_POINT('Ctrl Pts',(-1.57321663075256,6.83246778223093,
90.3455020746658));
#138471=CARTESIAN_POINT('Ctrl Pts',(-1.7458360089829,6.7927211364687,90.3535271616253));
#138472=CARTESIAN_POINT('Ctrl Pts',(-1.91692649951016,6.74643350946149,
90.3615522485847));
#138473=CARTESIAN_POINT('Ctrl Pts',(-2.08595653831519,6.69375917424284,
90.3695773355441));
#138474=CARTESIAN_POINT('Ctrl Pts',(-2.25501986674,6.64107446507761,90.3776040030042));
#138475=CARTESIAN_POINT('Ctrl Pts',(-2.42202158768804,6.58200065936432,
90.3856306704643));
#138476=CARTESIAN_POINT('Ctrl Pts',(-2.5864475293392,6.51674119023267,90.3936573379244));
#138477=CARTESIAN_POINT('Ctrl Pts',(-2.75100547155748,6.45142933102895,
90.4016904491649));
#138478=CARTESIAN_POINT('Ctrl Pts',(-2.9129831672907,6.37992203424297,90.4097235604054));
#138479=CARTESIAN_POINT('Ctrl Pts',(-3.07188800417212,6.30247020241456,
90.4177566716459));
#138480=CARTESIAN_POINT('Ctrl Pts',(-3.16552050660992,6.25683276950308,
90.4224900726082));
#138481=CARTESIAN_POINT('Ctrl Pts',(-3.25808657030009,6.20913227422691,
90.4272234735705));
#138482=CARTESIAN_POINT('Ctrl Pts',(-3.34948980370544,6.15942729621621,
90.4319568745328));
#138483=CARTESIAN_POINT('Ctrl Pts',(-3.53778330915744,6.0570334946037,90.4417078278273));
#138484=CARTESIAN_POINT('Ctrl Pts',(-3.72125190657123,5.94607109474755,
90.4514587811218));
#138485=CARTESIAN_POINT('Ctrl Pts',(-3.89921147911884,5.8269869060783,90.4612097344163));
#138486=CARTESIAN_POINT('Ctrl Pts',(-4.07742743581498,5.70773115429569,
90.4709747357882));
#138487=CARTESIAN_POINT('Ctrl Pts',(-4.25011845963373,5.58033022982133,
90.4807397371602));
#138488=CARTESIAN_POINT('Ctrl Pts',(-4.41662906056542,5.44527449297728,
90.4905047385321));
#138489=CARTESIAN_POINT('Ctrl Pts',(-4.58286212282468,5.31044386606437,
90.50025346367));
#138490=CARTESIAN_POINT('Ctrl Pts',(-4.74293532123849,5.16798395069382,
90.5100021888079));
#138491=CARTESIAN_POINT('Ctrl Pts',(-4.89622824128067,5.01842361422246,
90.5197509139457));
#138492=CARTESIAN_POINT('Ctrl Pts',(-5.04910043169596,4.86927376288338,
90.5294728826131));
#138493=CARTESIAN_POINT('Ctrl Pts',(-5.19522946545249,4.71306242274313,
90.5391948512805));
#138494=CARTESIAN_POINT('Ctrl Pts',(-5.33403220689424,4.550354599184,90.5489168199479));
#138495=CARTESIAN_POINT('Ctrl Pts',(-5.47191652684851,4.38872337079717,
90.5585744608878));
#138496=CARTESIAN_POINT('Ctrl Pts',(-5.60257113410021,4.22068136266675,
90.5682321018277));
#138497=CARTESIAN_POINT('Ctrl Pts',(-5.72545688972273,4.04682220593228,
90.5778897427676));
#138498=CARTESIAN_POINT('Ctrl Pts',(-5.77946940999854,3.9704051209684,90.5821346084516));
#138499=CARTESIAN_POINT('Ctrl Pts',(-5.83198149050525,3.89286473540746,
90.5863794741355));
#138500=CARTESIAN_POINT('Ctrl Pts',(-5.88294940643124,3.81425390395951,
90.5906243398194));
#138501=CARTESIAN_POINT('Ctrl Pts',(-5.97722618884616,3.66884524603762,
90.5984761868332));
#138502=CARTESIAN_POINT('Ctrl Pts',(-6.0661777107764,3.51983172051943,90.6063280338469));
#138503=CARTESIAN_POINT('Ctrl Pts',(-6.14951162340696,3.36765992286673,
90.6141798808607));
#138504=CARTESIAN_POINT('Ctrl Pts',(-6.23282190321341,3.21553127990596,
90.6220295011542));
#138505=CARTESIAN_POINT('Ctrl Pts',(-6.31051755964069,3.06024648068144,
90.6298791214476));
#138506=CARTESIAN_POINT('Ctrl Pts',(-6.38235100187132,2.90227880318418,
90.6377287417411));
#138507=CARTESIAN_POINT('Ctrl Pts',(-6.4541787091203,2.74432373738564,90.6455777353427));
#138508=CARTESIAN_POINT('Ctrl Pts',(-6.52014497665429,2.58368656727236,
90.6534267289444));
#138509=CARTESIAN_POINT('Ctrl Pts',(-6.58004949622673,2.42086248880567,
90.6612757225461));
#138510=CARTESIAN_POINT('Ctrl Pts',(-6.63998434370341,2.2579559772756,90.6691286898633));
#138511=CARTESIAN_POINT('Ctrl Pts',(-6.69385117954689,2.09286070368596,
90.6769816571806));
#138512=CARTESIAN_POINT('Ctrl Pts',(-6.74149881819082,1.9260893662631,90.6848346244979));
#138513=CARTESIAN_POINT('Ctrl Pts',(-6.78915855773392,1.75927567452434,
90.6926895862051));
#138514=CARTESIAN_POINT('Ctrl Pts',(-6.83059586229876,1.59078544140061,
90.7005445479122));
#138515=CARTESIAN_POINT('Ctrl Pts',(-6.86571039079761,1.42114298794801,
90.7083995096193));
#138516=CARTESIAN_POINT('Ctrl Pts',(-6.90085977340127,1.25133215017966,
90.7162622680325));
#138517=CARTESIAN_POINT('Ctrl Pts',(-6.92967378203119,1.08036718386781,
90.7241250264457));
#138518=CARTESIAN_POINT('Ctrl Pts',(-6.95210372993817,0.908779561103682,
90.731987784859));
#138519=CARTESIAN_POINT('Ctrl Pts',(-6.96855801787454,0.782905343161314,
90.7377557916079));
#138520=CARTESIAN_POINT('Ctrl Pts',(-6.98157782023667,0.656696184336185,
90.7435237983568));
#138521=CARTESIAN_POINT('Ctrl Pts',(-6.99116175634579,0.530362007602406,
90.7492918051057));
#138522=CARTESIAN_POINT('Ctrl Pts',(-7.00508248442123,0.346860813424763,
90.7576698715468));
#138523=CARTESIAN_POINT('Ctrl Pts',(-7.0117834348992,0.162689373238253,
90.7660479379878));
#138524=CARTESIAN_POINT('Ctrl Pts',(-7.01121685033776,-0.0215601493484155,
90.7744260044289));
#138525=CARTESIAN_POINT('Ctrl Pts',(-7.0106506532001,-0.205683684300519,
90.7827983420476));
#138526=CARTESIAN_POINT('Ctrl Pts',(-7.00282682965183,-0.389884867530377,
90.7911706796664));
#138527=CARTESIAN_POINT('Ctrl Pts',(-6.98774963364712,-0.573569193702466,
90.7995430172851));
#138528=CARTESIAN_POINT('Ctrl Pts',(-6.97268053616911,-0.757154856143024,
90.8079108578077));
#138529=CARTESIAN_POINT('Ctrl Pts',(-6.95036586143722,-0.940223888190426,
90.8162786983303));
#138530=CARTESIAN_POINT('Ctrl Pts',(-6.92086189661125,-1.12218410723665,
90.824646538853));
#138531=CARTESIAN_POINT('Ctrl Pts',(-6.89136945735317,-1.3040732444853,
90.8330111105229));
#138532=CARTESIAN_POINT('Ctrl Pts',(-6.85469338100169,-1.48485410850285,
90.8413756821929));
#138533=CARTESIAN_POINT('Ctrl Pts',(-6.81094158624387,-1.66394148673378,
90.8497402538628));
#138534=CARTESIAN_POINT('Ctrl Pts',(-6.76720047868659,-1.842985119497,90.8581027823285));
#138535=CARTESIAN_POINT('Ctrl Pts',(-6.71638717788038,-2.02033577251196,
90.8664653107942));
#138536=CARTESIAN_POINT('Ctrl Pts',(-6.65866041229904,-2.19541979497807,
90.8748278392598));
#138537=CARTESIAN_POINT('Ctrl Pts',(-6.60092903994172,-2.3705177896954,
90.8831910350814));
#138538=CARTESIAN_POINT('Ctrl Pts',(-6.53628319773679,-2.54334847844991,
90.8915542309029));
#138539=CARTESIAN_POINT('Ctrl Pts',(-6.46493130448406,-2.71335397447552,
90.8999174267244));
#138540=CARTESIAN_POINT('Ctrl Pts',(-6.39357454517533,-2.88337106453495,
90.9082811928991));
#138541=CARTESIAN_POINT('Ctrl Pts',(-6.31551094992987,-3.05056227438914,
90.9166449590738));
#138542=CARTESIAN_POINT('Ctrl Pts',(-6.2309969241478,-3.21439012780974,
90.9250087252485));
#138543=CARTESIAN_POINT('Ctrl Pts',(-6.14646586697067,-3.37825099606862,
90.9333741769021));
#138544=CARTESIAN_POINT('Ctrl Pts',(-6.05548193797086,-3.53874686417613,
90.9417396285557));
#138545=CARTESIAN_POINT('Ctrl Pts',(-5.95834749444242,-3.69536489375159,
90.9501050802093));
#138546=CARTESIAN_POINT('Ctrl Pts',(-5.86118052078041,-3.85203537439629,
90.9584733334361));
#138547=CARTESIAN_POINT('Ctrl Pts',(-5.75785909852066,-4.00482514760566,
90.966841586663));
#138548=CARTESIAN_POINT('Ctrl Pts',(-5.6487291231527,-4.15325003530326,
90.9752098398899));
#138549=CARTESIAN_POINT('Ctrl Pts',(-5.539497968728,-4.30181253404754,90.9835858516814));
#138550=CARTESIAN_POINT('Ctrl Pts',(-5.42444769460716,-4.44600179525974,
90.9919618634728));
#138551=CARTESIAN_POINT('Ctrl Pts',(-5.30396550338178,-4.58536547086883,
91.0003378752643));
#138552=CARTESIAN_POINT('Ctrl Pts',(-5.18342422620107,-4.72479749214649,
91.0087179947555));
#138553=CARTESIAN_POINT('Ctrl Pts',(-5.05744593946122,-4.85939896422367,
91.0170981142467));
#138554=CARTESIAN_POINT('Ctrl Pts',(-4.92645542832505,-4.98875369959539,
91.0254782337379));
#138555=CARTESIAN_POINT('Ctrl Pts',(-4.79531524393695,-5.11825623913802,
91.0338679285771));
#138556=CARTESIAN_POINT('Ctrl Pts',(-4.65915162977974,-5.24249983618741,
91.0422576234163));
#138557=CARTESIAN_POINT('Ctrl Pts',(-4.51842422645533,-5.36110707524869,
91.0506473182556));
#138558=CARTESIAN_POINT('Ctrl Pts',(-4.42907882658603,-5.43640876455007,
91.0559737907299));
#138559=CARTESIAN_POINT('Ctrl Pts',(-4.33789453137321,-5.50943939104233,
91.0613002632043));
#138560=CARTESIAN_POINT('Ctrl Pts',(-4.24499520189908,-5.58011131594647,
91.0666267356786));
#138561=CARTESIAN_POINT('Ctrl Pts',(-4.09881643320823,-5.69131486307623,
91.0750080360838));
#138562=CARTESIAN_POINT('Ctrl Pts',(-3.9480949743858,-5.79690056691435,
91.083389336489));
#138563=CARTESIAN_POINT('Ctrl Pts',(-3.79328726983489,-5.89649033332614,
91.0917706368942));
#138564=CARTESIAN_POINT('Ctrl Pts',(-3.63867576138784,-5.99595388428753,
91.1001413152281));
#138565=CARTESIAN_POINT('Ctrl Pts',(-3.47998860118239,-6.08943646595483,
91.1085119935619));
#138566=CARTESIAN_POINT('Ctrl Pts',(-3.3177143203471,-6.17660086544887,
91.1168826718958));
#138567=CARTESIAN_POINT('Ctrl Pts',(-3.15562419296002,-6.26366634831458,
91.1252438509469));
#138568=CARTESIAN_POINT('Ctrl Pts',(-2.98995534531866,-6.34442778560803,
91.133605029998));
#138569=CARTESIAN_POINT('Ctrl Pts',(-2.8212246166298,-6.41859160758979,
91.1419662090491));
#138570=CARTESIAN_POINT('Ctrl Pts',(-2.652712835964,-6.49265919326455,91.1503165384841));
#138571=CARTESIAN_POINT('Ctrl Pts',(-2.48114739766183,-6.56014610859738,
91.1586668679192));
#138572=CARTESIAN_POINT('Ctrl Pts',(-2.30706894933385,-6.62080504361211,
91.1670171973542));
#138573=CARTESIAN_POINT('Ctrl Pts',(-2.13312444395829,-6.68141730520504,
91.1753611017103));
#138574=CARTESIAN_POINT('Ctrl Pts',(-1.95667108998198,-6.73521194883545,
91.1837050060663));
#138575=CARTESIAN_POINT('Ctrl Pts',(-1.77826975363198,-6.78198962295119,
91.1920489104224));
#138576=CARTESIAN_POINT('Ctrl Pts',(-1.60001171034975,-6.82872972494688,
91.2003861129023));
#138577=CARTESIAN_POINT('Ctrl Pts',(-1.41980912114773,-6.86846401491194,
91.2087233153823));
#138578=CARTESIAN_POINT('Ctrl Pts',(-1.23823841131452,-6.90104283418422,
91.2170605178623));
#138579=CARTESIAN_POINT('Ctrl Pts',(-1.17846633592472,-6.91176760165052,
91.2198050788965));
#138580=CARTESIAN_POINT('Ctrl Pts',(-1.1185461148567,-6.9217173412299,91.2225496399308));
#138581=CARTESIAN_POINT('Ctrl Pts',(-1.0584986244227,-6.93088791026051,
91.225294200965));
#138582=CARTESIAN_POINT('Ctrl Pts',(-0.876067043634374,-6.9587492145863,
91.2336325112663));
#138583=CARTESIAN_POINT('Ctrl Pts',(-0.692609763919077,-6.9793919671487,
91.2419708215676));
#138584=CARTESIAN_POINT('Ctrl Pts',(-0.508721244211202,-6.9927697844408,
91.2503091318688));
#138585=CARTESIAN_POINT('Ctrl Pts',(-0.32471702808511,-7.0061560186017,
91.258652688352));
#138586=CARTESIAN_POINT('Ctrl Pts',(-0.140281357568597,-7.01226817658832,
91.2669962448353));
#138587=CARTESIAN_POINT('Ctrl Pts',(0.0439900195475317,-7.01111199744236,
91.2753398013185));
#138588=CARTESIAN_POINT('Ctrl Pts',(0.228401589524863,-7.00995493868035,
91.2836897055431));
#138589=CARTESIAN_POINT('Ctrl Pts',(0.412648289506366,-7.00151851485407,
91.2920396097678));
#138590=CARTESIAN_POINT('Ctrl Pts',(0.596137764433919,-6.98586045726049,
91.3003895139924));
#138591=CARTESIAN_POINT('Ctrl Pts',(0.779902459993951,-6.97017891373937,
91.3087519424554));
#138592=CARTESIAN_POINT('Ctrl Pts',(0.962907334103701,-6.94725411875867,
91.3171143709185));
#138593=CARTESIAN_POINT('Ctrl Pts',(1.1445670123845,-6.91719545167413,91.3254767993815));
#138594=CARTESIAN_POINT('Ctrl Pts',(1.32638203445439,-6.88711108033158,
91.3338463788608));
#138595=CARTESIAN_POINT('Ctrl Pts',(1.50684924536742,-6.84988073098574,
91.3422159583401));
#138596=CARTESIAN_POINT('Ctrl Pts',(1.68539621167435,-6.80566427119159,
91.3505855378195));
#138597=CARTESIAN_POINT('Ctrl Pts',(1.86421856492236,-6.76137961289561,
91.3589680263554));
#138598=CARTESIAN_POINT('Ctrl Pts',(2.0411144410396,-6.7100874031092,91.3673505148913));
#138599=CARTESIAN_POINT('Ctrl Pts',(2.2155278856756,-6.65199689945011,91.3757330034272));
#138600=CARTESIAN_POINT('Ctrl Pts',(2.27259882277569,-6.63298873475638,
91.3784758910353));
#138601=CARTESIAN_POINT('Ctrl Pts',(2.32940413616106,-6.61325305162709,
91.3812187786434));
#138602=CARTESIAN_POINT('Ctrl Pts',(2.38592487488105,-6.59279827189668,
91.3839616662515));
#138603=CARTESIAN_POINT('Ctrl Pts',(2.55880866657857,-6.53023185896195,
91.3923515213848));
#138604=CARTESIAN_POINT('Ctrl Pts',(2.72937738320644,-6.46080769298565,
91.400741376518));
#138605=CARTESIAN_POINT('Ctrl Pts',(2.89706946972923,-6.38471730384853,
91.4091312316513));
#138606=CARTESIAN_POINT('Ctrl Pts',(3.06460681234585,-6.30869712985561,
91.4175133447439));
#138607=CARTESIAN_POINT('Ctrl Pts',(3.22927251872187,-6.22602313087909,
91.4258954578365));
#138608=CARTESIAN_POINT('Ctrl Pts',(3.39052343719861,-6.13693550433007,
91.4342775709291));
#138609=CARTESIAN_POINT('Ctrl Pts',(3.55164925913813,-6.04791699089802,
91.4426531812784));
#138610=CARTESIAN_POINT('Ctrl Pts',(3.70936528807828,-5.95249492815169,
91.4510287916277));
#138611=CARTESIAN_POINT('Ctrl Pts',(3.86315107188018,-5.85095636270952,
91.4594044019771));
#138612=CARTESIAN_POINT('Ctrl Pts',(4.0168401221405,-5.74948166653276,91.4677747439431));
#138613=CARTESIAN_POINT('Ctrl Pts',(4.16660358295411,-5.64189831963237,
91.4761450859092));
#138614=CARTESIAN_POINT('Ctrl Pts',(4.31194781502063,-5.52853801678516,
91.4845154278752));
#138615=CARTESIAN_POINT('Ctrl Pts',(4.45722192923922,-5.41523240190433,
91.49288173177));
#138616=CARTESIAN_POINT('Ctrl Pts',(4.59808080742231,-5.29615559052077,
91.5012480356649));
#138617=CARTESIAN_POINT('Ctrl Pts',(4.73406151956882,-5.17168136019977,
91.5096143395597));
#138618=CARTESIAN_POINT('Ctrl Pts',(4.87000420172109,-5.04724194183251,
91.5179783036337));
#138619=CARTESIAN_POINT('Ctrl Pts',(5.00107119501868,-4.91740833511234,
91.5263422677078));
#138620=CARTESIAN_POINT('Ctrl Pts',(5.12683385474934,-4.78259356294219,
91.5347062317819));
#138621=CARTESIAN_POINT('Ctrl Pts',(5.25257716169686,-4.64779953652483,
91.5430689087809));
#138622=CARTESIAN_POINT('Ctrl Pts',(5.37301753839158,-4.50802611319689,
91.5514315857799));
#138623=CARTESIAN_POINT('Ctrl Pts',(5.48776403248056,-4.36372232002825,
91.559794262779));
#138624=CARTESIAN_POINT('Ctrl Pts',(5.60250816414852,-4.2194214978115,91.5681567676057));
#138625=CARTESIAN_POINT('Ctrl Pts',(5.71155844272837,-4.07059074922487,
91.5765192724325));
#138626=CARTESIAN_POINT('Ctrl Pts',(5.81456469406526,-3.91771157450746,
91.5848817772593));
#138627=CARTESIAN_POINT('Ctrl Pts',(5.91758255469326,-3.76481516958491,
91.5932452245798));
#138628=CARTESIAN_POINT('Ctrl Pts',(6.01455484679185,-3.60786970169083,
91.6016086719004));
#138629=CARTESIAN_POINT('Ctrl Pts',(6.10517492330863,-3.44738534520054,
91.6099721192209));
#138630=CARTESIAN_POINT('Ctrl Pts',(6.19584835947187,-3.28680649101334,
91.6183404911742));
#138631=CARTESIAN_POINT('Ctrl Pts',(6.28016194331338,-3.12268487031842,
91.6267088631274));
#138632=CARTESIAN_POINT('Ctrl Pts',(6.3578546834387,-2.9555558507287,91.6350772350807));
#138633=CARTESIAN_POINT('Ctrl Pts',(6.43557070233943,-2.78837675491686,
91.6434481144169));
#138634=CARTESIAN_POINT('Ctrl Pts',(6.50666178814667,-2.61818876376641,
91.6518189937531));
#138635=CARTESIAN_POINT('Ctrl Pts',(6.57091498856201,-2.44554754106132,
91.6601898730893));
#138636=CARTESIAN_POINT('Ctrl Pts',(6.63522263001914,-2.27276004131543,
91.668567844981));
#138637=CARTESIAN_POINT('Ctrl Pts',(6.6926806996216,-2.09751546674238,91.6769458168727));
#138638=CARTESIAN_POINT('Ctrl Pts',(6.74312567677145,-1.92038607310239,
91.6853237887645));
#138639=CARTESIAN_POINT('Ctrl Pts',(6.77518387048917,-1.80781890120051,
91.6906480581178));
#138640=CARTESIAN_POINT('Ctrl Pts',(6.8044106921968,-1.69449079644053,91.6959723274711));
#138641=CARTESIAN_POINT('Ctrl Pts',(6.83077487139509,-1.58055092256384,
91.7012965968244));
#138642=CARTESIAN_POINT('Ctrl Pts',(6.87364674711607,-1.39526860917314,
91.7099546101197));
#138643=CARTESIAN_POINT('Ctrl Pts',(6.90902110269616,-1.20804545735541,
91.718612623415));
#138644=CARTESIAN_POINT('Ctrl Pts',(6.93673266435465,-1.01949325930841,
91.7272706367104));
#138645=CARTESIAN_POINT('Ctrl Pts',(6.96437737102982,-0.831395949160153,
91.7359077622859));
#138646=CARTESIAN_POINT('Ctrl Pts',(6.98439612141707,-0.641976267561167,
91.7445448878615));
#138647=CARTESIAN_POINT('Ctrl Pts',(6.99667434903524,-0.451856853497069,
91.7531820134371));
#138648=CARTESIAN_POINT('Ctrl Pts',(7.00631840262471,-0.302525706148289,
91.7599661279282));
#138649=CARTESIAN_POINT('Ctrl Pts',(7.01118792571455,-0.152763206936516,
91.7667502424193));
#138650=CARTESIAN_POINT('Ctrl Pts',(7.01124941011624,-0.00287604671718754,
91.7735343569104));
#138651=CARTESIAN_POINT('Ctrl Pts',(7.01124941011649,-0.00287604611315284,
91.7735343569377));
#138652=CARTESIAN_POINT('Ctrl Pts',(7.01131757022026,0.163285228292073,
91.7810550618994));
#138653=CARTESIAN_POINT('Ctrl Pts',(7.00547459428384,0.329575821306189,
91.7885757668611));
#138654=CARTESIAN_POINT('Ctrl Pts',(6.99371928995571,0.49549677678211,91.7960964718228));
#138655=CARTESIAN_POINT('Ctrl Pts',(6.98196648505464,0.661382453943276,
91.803615577723));
#138656=CARTESIAN_POINT('Ctrl Pts',(6.96430388228248,0.826898246011775,
91.8111346836233));
#138657=CARTESIAN_POINT('Ctrl Pts',(6.94078235372727,0.991547719824008,
91.8186537895235));
#138658=CARTESIAN_POINT('Ctrl Pts',(6.91725260803701,1.15625471315322,91.826175522188));
#138659=CARTESIAN_POINT('Ctrl Pts',(6.88785990483666,1.32009438216346,91.8336972548524));
#138660=CARTESIAN_POINT('Ctrl Pts',(6.85270668801346,1.48257802848806,91.8412189875169));
#138661=CARTESIAN_POINT('Ctrl Pts',(6.82350465434371,1.61755437886365,91.8474673457148));
#138662=CARTESIAN_POINT('Ctrl Pts',(6.79032839184587,1.75159501383177,91.8537157039128));
#138663=CARTESIAN_POINT('Ctrl Pts',(6.75326300162656,1.88442707297518,91.8599640621107));
#138664=CARTESIAN_POINT('Ctrl Pts',(6.70037504303367,2.07396282053429,91.8688797354031));
#138665=CARTESIAN_POINT('Ctrl Pts',(6.63957404626945,2.26102355855614,91.8777954086954));
#138666=CARTESIAN_POINT('Ctrl Pts',(6.57110895151815,2.44502632087633,91.8867110819877));
#138667=CARTESIAN_POINT('',(7.01124860966183,-0.00441542920841772,91.2264656430895));
#138668=CARTESIAN_POINT('Ctrl Pts',(6.5711089515181,2.44502632087648,91.3398522865014));
#138669=CARTESIAN_POINT('Ctrl Pts',(6.63771924680903,2.26600840850791,91.3311805125692));
#138670=CARTESIAN_POINT('Ctrl Pts',(6.69700989700486,2.08426710051917,91.3225087386371));
#138671=CARTESIAN_POINT('Ctrl Pts',(6.7487830778944,1.90040877971718,91.313836964705));
#138672=CARTESIAN_POINT('Ctrl Pts',(6.80055978789547,1.7165379262389,91.3051645996626));
#138673=CARTESIAN_POINT('Ctrl Pts',(6.84481792613587,1.53055004459392,91.2964922346203));
#138674=CARTESIAN_POINT('Ctrl Pts',(6.88140980451109,1.34306577086852,91.2878198695779));
#138675=CARTESIAN_POINT('Ctrl Pts',(6.91799949925392,1.15559268532888,91.2791480220618));
#138676=CARTESIAN_POINT('Ctrl Pts',(6.94692379517697,0.966623665170273,
91.2704761745457));
#138677=CARTESIAN_POINT('Ctrl Pts',(6.96808618426394,0.776789219267382,
91.2618043270296));
#138678=CARTESIAN_POINT('Ctrl Pts',(6.98924897510681,0.586951169465677,
91.2531323148833));
#138679=CARTESIAN_POINT('Ctrl Pts',(7.0026495327686,0.396247943318909,91.2444603027372));
#138680=CARTESIAN_POINT('Ctrl Pts',(7.0082431436184,0.205315860141579,91.235788290591));
#138681=CARTESIAN_POINT('Ctrl Pts',(7.01024757124657,0.136896809746186,
91.2326807414238));
#138682=CARTESIAN_POINT('Ctrl Pts',(7.01125,0.0684484052927758,91.2295731922566));
#138683=CARTESIAN_POINT('Ctrl Pts',(7.01125,8.58630487052188E-16,91.2264656430895));
#138684=CARTESIAN_POINT('Ctrl Pts',(7.01124860966183,-0.00441542920841772,
91.2264656430895));
#138685=CARTESIAN_POINT('Ctrl Pts',(7.01111401898774,-0.218131612174622,
91.2167762696257));
#138686=CARTESIAN_POINT('Ctrl Pts',(7.00120369221107,-0.431553992030833,
91.2070868961619));
#138687=CARTESIAN_POINT('Ctrl Pts',(6.98162202993273,-0.643879176288536,
91.1973975226981));
#138688=CARTESIAN_POINT('Ctrl Pts',(6.96102990223338,-0.867160900070445,
91.1872081520074));
#138689=CARTESIAN_POINT('Ctrl Pts',(6.92974218381963,-1.08922910119445,
91.1770187813167));
#138690=CARTESIAN_POINT('Ctrl Pts',(6.88793931774568,-1.30916710833768,
91.1668294106261));
#138691=CARTESIAN_POINT('Ctrl Pts',(6.84780526563828,-1.52032496109034,
91.1570468102293));
#138692=CARTESIAN_POINT('Ctrl Pts',(6.79797927933411,-1.72951939372668,
91.1472642098326));
#138693=CARTESIAN_POINT('Ctrl Pts',(6.73867228106864,-1.93595517790499,
91.1374816094358));
#138694=CARTESIAN_POINT('Ctrl Pts',(6.67933190914448,-2.14250712910584,
91.1276935041041));
#138695=CARTESIAN_POINT('Ctrl Pts',(6.61049987072077,-2.34629729945448,
91.1179053987724));
#138696=CARTESIAN_POINT('Ctrl Pts',(6.53243709486289,-2.54654514276878,
91.1081172934407));
#138697=CARTESIAN_POINT('Ctrl Pts',(6.45451667045176,-2.74642782394416,
91.0983470372175));
#138698=CARTESIAN_POINT('Ctrl Pts',(6.36739914687599,-2.94278105315336,
91.0885767809943));
#138699=CARTESIAN_POINT('Ctrl Pts',(6.27139328918328,-3.13484493633847,
91.0788065247711));
#138700=CARTESIAN_POINT('Ctrl Pts',(6.25933489510154,-3.15896827680929,
91.0775793746507));
#138701=CARTESIAN_POINT('Ctrl Pts',(6.24713634688621,-3.18302397230467,
91.0763522245304));
#138702=CARTESIAN_POINT('Ctrl Pts',(6.23479831147988,-3.20701053594585,
91.0751250744101));
#138703=CARTESIAN_POINT('Ctrl Pts',(6.15403231604415,-3.36402894493563,
91.0670920288114));
#138704=CARTESIAN_POINT('Ctrl Pts',(6.06724655878398,-3.51815830011059,
91.0590589832128));
#138705=CARTESIAN_POINT('Ctrl Pts',(5.97467924385955,-3.66890099287155,
91.0510259376142));
#138706=CARTESIAN_POINT('Ctrl Pts',(5.88217143476943,-3.81954678242531,
91.0429980559665));
#138707=CARTESIAN_POINT('Ctrl Pts',(5.78388965703437,-3.96680993201838,
91.0349701743189));
#138708=CARTESIAN_POINT('Ctrl Pts',(5.68011830558371,-4.11021685523683,
91.0269422926712));
#138709=CARTESIAN_POINT('Ctrl Pts',(5.57639380792113,-4.25355902881582,
91.0189180356913));
#138710=CARTESIAN_POINT('Ctrl Pts',(5.46718488616196,-4.39304814644092,
91.0108937787113));
#138711=CARTESIAN_POINT('Ctrl Pts',(5.35281953637398,-4.5282391250367,91.0028695217314));
#138712=CARTESIAN_POINT('Ctrl Pts',(5.23846801452165,-4.66341375766616,
90.9948462349659));
#138713=CARTESIAN_POINT('Ctrl Pts',(5.11896153720162,-4.79429100171989,
90.9868229482003));
#138714=CARTESIAN_POINT('Ctrl Pts',(4.99466882434933,-4.92045830157852,
90.9787996614348));
#138715=CARTESIAN_POINT('Ctrl Pts',(4.87038629617602,-5.04661526315248,
90.970777032106));
#138716=CARTESIAN_POINT('Ctrl Pts',(4.74131857384571,-5.16806279091223,
90.9627544027773));
#138717=CARTESIAN_POINT('Ctrl Pts',(4.60787150227857,-5.28442492434031,
90.9547317734485));
#138718=CARTESIAN_POINT('Ctrl Pts',(4.47437426411301,-5.4008308016464,90.9467061281822));
#138719=CARTESIAN_POINT('Ctrl Pts',(4.33649466635002,-5.51214722677634,
90.938680482916));
#138720=CARTESIAN_POINT('Ctrl Pts',(4.19467220699311,-5.61803805953462,
90.9306548376498));
#138721=CARTESIAN_POINT('Ctrl Pts',(4.1110450427043,-5.6804777472111,90.9259224281411));
#138722=CARTESIAN_POINT('Ctrl Pts',(4.02604755291839,-5.74103173588268,
90.9211900186324));
#138723=CARTESIAN_POINT('Ctrl Pts',(3.93977462314144,-5.79963813365547,
90.9164576091237));
#138724=CARTESIAN_POINT('Ctrl Pts',(3.78062379549338,-5.90775149824303,
90.9077275602889));
#138725=CARTESIAN_POINT('Ctrl Pts',(3.6170516356225,-6.00928900419784,90.8989975114541));
#138726=CARTESIAN_POINT('Ctrl Pts',(3.4496124399988,-6.10391682252515,90.8902674626193));
#138727=CARTESIAN_POINT('Ctrl Pts',(3.28212482912266,-6.19857200260426,
90.88153488948));
#138728=CARTESIAN_POINT('Ctrl Pts',(3.11076818908052,-6.28631337226743,
90.8728023163407));
#138729=CARTESIAN_POINT('Ctrl Pts',(2.93612178164148,-6.36685286824429,
90.8640697432014));
#138730=CARTESIAN_POINT('Ctrl Pts',(2.75899424320109,-6.44853655632467,
90.855213109921));
#138731=CARTESIAN_POINT('Ctrl Pts',(2.57848301537317,-6.52281206155041,
90.8463564766407));
#138732=CARTESIAN_POINT('Ctrl Pts',(2.39521419140078,-6.58942907540648,
90.8374998433603));
#138733=CARTESIAN_POINT('Ctrl Pts',(2.21439749229441,-6.65515475797863,
90.8287617112534));
#138734=CARTESIAN_POINT('Ctrl Pts',(2.03089680063777,-6.71342554354831,
90.8200235791465));
#138735=CARTESIAN_POINT('Ctrl Pts',(1.84533044372671,-6.76405071802063,
90.8112854470396));
#138736=CARTESIAN_POINT('Ctrl Pts',(1.65598928160953,-6.81570571371346,
90.8023695631726));
#138737=CARTESIAN_POINT('Ctrl Pts',(1.46449779897392,-6.85940062961549,
90.7934536793055));
#138738=CARTESIAN_POINT('Ctrl Pts',(1.27152670013854,-6.89498704954076,
90.7845377954384));
#138739=CARTESIAN_POINT('Ctrl Pts',(1.07855560130315,-6.93057346946603,
90.7756219115713));
#138740=CARTESIAN_POINT('Ctrl Pts',(0.88410518476869,-6.95805134455265,
90.7667060277043));
#138741=CARTESIAN_POINT('Ctrl Pts',(0.688855744563673,-6.97732787861382,
90.7577901438372));
#138742=CARTESIAN_POINT('Ctrl Pts',(0.497443005196789,-6.99622562390965,
90.7490494593411));
#138743=CARTESIAN_POINT('Ctrl Pts',(0.305242022760735,-7.00724336029926,
90.740308774845));
#138744=CARTESIAN_POINT('Ctrl Pts',(0.112898462332252,-7.01034096886186,
90.7315680903489));
#138745=CARTESIAN_POINT('Ctrl Pts',(-0.0794104922946831,-7.01343802011322,
90.7228289784471));
#138746=CARTESIAN_POINT('Ctrl Pts',(-0.271861700023683,-7.00861778488938,
90.7140898665453));
#138747=CARTESIAN_POINT('Ctrl Pts',(-0.463808403006335,-6.99589224672598,
90.7053507546435));
#138748=CARTESIAN_POINT('Ctrl Pts',(-0.658242051788765,-6.98300183090023,
90.6964984149692));
#138749=CARTESIAN_POINT('Ctrl Pts',(-0.852157745644223,-6.96199983140183,
90.6876460752948));
#138750=CARTESIAN_POINT('Ctrl Pts',(-1.04488606461541,-6.93295317123032,
90.6787937356204));
#138751=CARTESIAN_POINT('Ctrl Pts',(-1.23505173034007,-6.90429273617812,
90.6700591029707));
#138752=CARTESIAN_POINT('Ctrl Pts',(-1.42406112570954,-6.86780030258419,
90.661324470321));
#138753=CARTESIAN_POINT('Ctrl Pts',(-1.61127801079577,-6.82359214303039,
90.6525898376714));
#138754=CARTESIAN_POINT('Ctrl Pts',(-1.80227926954812,-6.77849036645713,
90.6436786444846));
#138755=CARTESIAN_POINT('Ctrl Pts',(-1.99141449156612,-6.72535765834916,
90.6347674512979));
#138756=CARTESIAN_POINT('Ctrl Pts',(-2.17801974076475,-6.66437218133404,
90.6258562581111));
#138757=CARTESIAN_POINT('Ctrl Pts',(-2.36462498996338,-6.60338670431893,
90.6169450649244));
#138758=CARTESIAN_POINT('Ctrl Pts',(-2.54869997402439,-6.53454853975545,
90.6080338717376));
#138759=CARTESIAN_POINT('Ctrl Pts',(-2.72959694168776,-6.45809005034994,
90.5991226785509));
#138760=CARTESIAN_POINT('Ctrl Pts',(-2.8925177094081,-6.38922943895559,
90.5910970136984));
#138761=CARTESIAN_POINT('Ctrl Pts',(-3.05293536394538,-6.31415563055654,
90.583071348846));
#138762=CARTESIAN_POINT('Ctrl Pts',(-3.21034092784385,-6.2330841234104,
90.5750456839936));
#138763=CARTESIAN_POINT('Ctrl Pts',(-3.36769653507731,-6.15203834637203,
90.5670225662903));
#138764=CARTESIAN_POINT('Ctrl Pts',(-3.5220416294079,-6.06499882796826,
90.558999448587));
#138765=CARTESIAN_POINT('Ctrl Pts',(-3.67288946274933,-5.97222819029254,
90.5509763308837));
#138766=CARTESIAN_POINT('Ctrl Pts',(-3.82371827285875,-5.87946925180618,
90.5429542249658));
#138767=CARTESIAN_POINT('Ctrl Pts',(-3.97105038862194,-5.78098082615121,
90.5349321190479));
#138768=CARTESIAN_POINT('Ctrl Pts',(-4.11442586268974,-5.67707022881784,
90.5269100131299));
#138769=CARTESIAN_POINT('Ctrl Pts',(-4.25785461556809,-5.57312101795544,
90.5188849261704));
#138770=CARTESIAN_POINT('Ctrl Pts',(-4.39732349069979,-5.46374582317389,
90.5108598392108));
#138771=CARTESIAN_POINT('Ctrl Pts',(-4.53240325158435,-5.34929409618948,
90.5028347522512));
#138772=CARTESIAN_POINT('Ctrl Pts',(-4.66750961575186,-5.23481982851017,
90.4948080847909));
#138773=CARTESIAN_POINT('Ctrl Pts',(-4.79822486963941,-5.11526728055089,
90.4867814173306));
#138774=CARTESIAN_POINT('Ctrl Pts',(-4.92415497178524,-4.99102438146146,
90.4787547498703));
#138775=CARTESIAN_POINT('Ctrl Pts',(-5.05018617017328,-4.86668174061048,
90.4707216386297));
#138776=CARTESIAN_POINT('Ctrl Pts',(-5.17142429000805,-4.73764149220409,
90.462688527389));
#138777=CARTESIAN_POINT('Ctrl Pts',(-5.28751366213962,-4.60432686015957,
90.4546554161484));
#138778=CARTESIAN_POINT('Ctrl Pts',(-5.35591773737159,-4.52577303604585,
90.449922015187));
#138779=CARTESIAN_POINT('Ctrl Pts',(-5.42253493239662,-4.44573577772568,
90.4451886142256));
#138780=CARTESIAN_POINT('Ctrl Pts',(-5.48729935260437,-4.36430663191848,
90.4404552132643));
#138781=CARTESIAN_POINT('Ctrl Pts',(-5.62071607384014,-4.19656005730582,
90.4307042599703));
#138782=CARTESIAN_POINT('Ctrl Pts',(-5.74634700732499,-4.02280664304849,
90.4209533066762));
#138783=CARTESIAN_POINT('Ctrl Pts',(-5.86373659786333,-3.843724713527,90.4112023533822));
#138784=CARTESIAN_POINT('Ctrl Pts',(-5.98129531012859,-3.66438478289108,
90.4014373520107));
#138785=CARTESIAN_POINT('Ctrl Pts',(-6.09058890837239,-3.47970101359067,
90.3916723506393));
#138786=CARTESIAN_POINT('Ctrl Pts',(-6.19120518796534,-3.29038065928718,
90.3819073492678));
#138787=CARTESIAN_POINT('Ctrl Pts',(-6.29165376106743,-3.101375862788,90.3721586241303));
#138788=CARTESIAN_POINT('Ctrl Pts',(-6.38345390397528,-2.90774996034723,
90.3624098989929));
#138789=CARTESIAN_POINT('Ctrl Pts',(-6.46624073213302,-2.71023197468478,
90.3526611738555));
#138790=CARTESIAN_POINT('Ctrl Pts',(-6.54880034254809,-2.51325609930533,
90.3429392051884));
#138791=CARTESIAN_POINT('Ctrl Pts',(-6.62239600825781,-2.31240950291824,
90.3332172365214));
#138792=CARTESIAN_POINT('Ctrl Pts',(-6.68671126917638,-2.10843993634384,
90.3234952678544));
#138793=CARTESIAN_POINT('Ctrl Pts',(-6.75060097281172,-1.90581998311739,
90.3138376269148));
#138794=CARTESIAN_POINT('Ctrl Pts',(-6.80533263618203,-1.70011828668716,
90.3041799859752));
#138795=CARTESIAN_POINT('Ctrl Pts',(-6.85064147790634,-1.49209178795718,
90.2945223450356));
#138796=CARTESIAN_POINT('Ctrl Pts',(-6.87055627373543,-1.40065697983616,
90.2902774793498));
#138797=CARTESIAN_POINT('Ctrl Pts',(-6.88865126635209,-1.3087733510309,
90.2860326136639));
#138798=CARTESIAN_POINT('Ctrl Pts',(-6.90490681962776,-1.21650662750276,
90.281787747978));
#138799=CARTESIAN_POINT('Ctrl Pts',(-6.93497517205459,-1.04583828338269,
90.273935900964));
#138800=CARTESIAN_POINT('Ctrl Pts',(-6.95873380167374,-0.873928622336891,
90.2660840539501));
#138801=CARTESIAN_POINT('Ctrl Pts',(-6.97608778540285,-0.701302910911618,
90.2582322069362));
#138802=CARTESIAN_POINT('Ctrl Pts',(-6.99343684768249,-0.528726154742379,
90.2503825866425));
#138803=CARTESIAN_POINT('Ctrl Pts',(-7.00438483889646,-0.355434131303304,
90.2425329663489));
#138804=CARTESIAN_POINT('Ctrl Pts',(-7.008888457383,-0.181959210987826,
90.2346833460553));
#138805=CARTESIAN_POINT('Ctrl Pts',(-7.01339171631321,-0.00849814042606301,
90.2268343524535));
#138806=CARTESIAN_POINT('Ctrl Pts',(-7.01145161759495,0.165145416588549,
90.2189853588516));
#138807=CARTESIAN_POINT('Ctrl Pts',(-7.003076946412,0.338437357767773,90.2111363652498));
#138808=CARTESIAN_POINT('Ctrl Pts',(-6.99469803537824,0.511817031582644,
90.2032833979323));
#138809=CARTESIAN_POINT('Ctrl Pts',(-6.97987806139806,0.684844352367448,
90.1954304306148));
#138810=CARTESIAN_POINT('Ctrl Pts',(-6.95867786783009,0.856988269623172,
90.1875774632974));
#138811=CARTESIAN_POINT('Ctrl Pts',(-6.9374722901253,1.02917590564969,90.1797225015901));
#138812=CARTESIAN_POINT('Ctrl Pts',(-6.90988332535552,1.20047931452409,
90.1718675398828));
#138813=CARTESIAN_POINT('Ctrl Pts',(-6.87602316632931,1.37037658276937,
90.1640125781755));
#138814=CARTESIAN_POINT('Ctrl Pts',(-6.84212939826494,1.54044248825485,
90.1561498197621));
#138815=CARTESIAN_POINT('Ctrl Pts',(-6.80195209202393,1.70909909459969,
90.1482870613488));
#138816=CARTESIAN_POINT('Ctrl Pts',(-6.75565379071956,1.87583805869175,
90.1404243029354));
#138817=CARTESIAN_POINT('Ctrl Pts',(-6.72169002122517,1.99815537018289,
90.1346562961874));
#138818=CARTESIAN_POINT('Ctrl Pts',(-6.68443330329901,2.11944099995356,
90.1288882894395));
#138819=CARTESIAN_POINT('Ctrl Pts',(-6.643964273863,2.23950112528038,90.1231202826915));
#138820=CARTESIAN_POINT('Ctrl Pts',(-6.58518275153927,2.41388921996521,
90.1147422162505));
#138821=CARTESIAN_POINT('Ctrl Pts',(-6.51949218948702,2.58607740822059,
90.1063641498095));
#138822=CARTESIAN_POINT('Ctrl Pts',(-6.44707966720528,2.75550182856196,
90.0979860833685));
#138823=CARTESIAN_POINT('Ctrl Pts',(-6.37471665974586,2.9248103984978,90.0896137457498));
#138824=CARTESIAN_POINT('Ctrl Pts',(-6.29564098469229,3.09135866697528,
90.081241408131));
#138825=CARTESIAN_POINT('Ctrl Pts',(-6.21008852409923,3.25460091030391,
90.0728690705123));
#138826=CARTESIAN_POINT('Ctrl Pts',(-6.12458201693739,3.41775547010891,
90.0645012299897));
#138827=CARTESIAN_POINT('Ctrl Pts',(-6.03260581313292,3.57760725501141,
90.0561333894672));
#138828=CARTESIAN_POINT('Ctrl Pts',(-5.93444279739089,3.73363298236389,
90.0477655489446));
#138829=CARTESIAN_POINT('Ctrl Pts',(-5.83631812851218,3.88959775909052,
90.0394009772747));
#138830=CARTESIAN_POINT('Ctrl Pts',(-5.73201164201851,4.04173918095292,
90.0310364056048));
#138831=CARTESIAN_POINT('Ctrl Pts',(-5.62185104212229,4.18956052858633,
90.0226718339349));
#138832=CARTESIAN_POINT('Ctrl Pts',(-5.51171735102954,4.33734576806858,
90.0143093054693));
#138833=CARTESIAN_POINT('Ctrl Pts',(-5.39573259483276,4.48081277470348,
90.0059467770038));
#138834=CARTESIAN_POINT('Ctrl Pts',(-5.27426674904466,4.61949529953456,
89.9975842485382));
#138835=CARTESIAN_POINT('Ctrl Pts',(-5.15279120990197,4.7581888916651,89.9892210527167));
#138836=CARTESIAN_POINT('Ctrl Pts',(-5.02583391929403,4.89209698795139,
89.9808578568952));
#138837=CARTESIAN_POINT('Ctrl Pts',(-4.89380445365022,5.02078724224929,
89.9724946610737));
#138838=CARTESIAN_POINT('Ctrl Pts',(-4.7617659838616,5.14948627296449,89.964130894899));
#138839=CARTESIAN_POINT('Ctrl Pts',(-4.62465488460112,5.27296652245633,
89.9557671287243));
#138840=CARTESIAN_POINT('Ctrl Pts',(-4.48291695154835,5.39083316084077,
89.9474033625496));
#138841=CARTESIAN_POINT('Ctrl Pts',(-4.34115045525196,5.50872355188926,
89.939037910896));
#138842=CARTESIAN_POINT('Ctrl Pts',(-4.19475551872813,5.62099786585151,
89.9306724592425));
#138843=CARTESIAN_POINT('Ctrl Pts',(-4.04421063405544,5.72730188744167,
89.9223070075889));
#138844=CARTESIAN_POINT('Ctrl Pts',(-3.89361533219721,5.8336415100394,89.9139387543621));
#138845=CARTESIAN_POINT('Ctrl Pts',(-3.73886757933855,5.9340066637545,89.9055705011352));
#138846=CARTESIAN_POINT('Ctrl Pts',(-3.58047477208355,6.0280865097453,89.8972022479084));
#138847=CARTESIAN_POINT('Ctrl Pts',(-3.42193511209877,6.12225358117543,
89.8888262361169));
#138848=CARTESIAN_POINT('Ctrl Pts',(-3.25974392746922,6.21012353196851,
89.8804502243254));
#138849=CARTESIAN_POINT('Ctrl Pts',(-3.09443422831232,6.29143094765803,
89.8720742125339));
#138850=CARTESIAN_POINT('Ctrl Pts',(-2.9290434592364,6.37277823750882,89.8636940930428));
#138851=CARTESIAN_POINT('Ctrl Pts',(-2.76053142352426,6.44755643510048,
89.8553139735517));
#138852=CARTESIAN_POINT('Ctrl Pts',(-2.58945162578366,6.51554808440751,
89.8469338540605));
#138853=CARTESIAN_POINT('Ctrl Pts',(-2.41817634770284,6.58361742278663,
89.8385441592213));
#138854=CARTESIAN_POINT('Ctrl Pts',(-2.24432775286241,6.64488460241677,
89.8301544643821));
#138855=CARTESIAN_POINT('Ctrl Pts',(-2.06847631044855,6.6991814660907,89.8217647695429));
#138856=CARTESIAN_POINT('Ctrl Pts',(-1.9568312642801,6.7336536078512,89.8164382970682));
#138857=CARTESIAN_POINT('Ctrl Pts',(-1.84437920556466,6.76531719248766,
89.8111118245934));
#138858=CARTESIAN_POINT('Ctrl Pts',(-1.7312683729505,6.79413985603191,89.8057853521187));
#138859=CARTESIAN_POINT('Ctrl Pts',(-1.55328643993815,6.83949283641063,
89.7974040517138));
#138860=CARTESIAN_POINT('Ctrl Pts',(-1.37331386192984,6.87790078047739,
89.7890227513088));
#138861=CARTESIAN_POINT('Ctrl Pts',(-1.1919184300438,6.90919365907643,89.7806414509039));
#138862=CARTESIAN_POINT('Ctrl Pts',(-1.01075289031331,6.94044687853279,
89.7722707725703));
#138863=CARTESIAN_POINT('Ctrl Pts',(-0.828168410677595,6.9646029478222,
89.7639000942367));
#138864=CARTESIAN_POINT('Ctrl Pts',(-0.6447463745845,6.98154199836685,89.7555294159031));
#138865=CARTESIAN_POINT('Ctrl Pts',(-0.461532491010622,6.9984618259974,
89.7471682368522));
#138866=CARTESIAN_POINT('Ctrl Pts',(-0.2774832696751,7.0081809286607,89.7388070578013));
#138867=CARTESIAN_POINT('Ctrl Pts',(-0.0931891295747852,7.01063066696778,
89.7304458787505));
#138868=CARTESIAN_POINT('Ctrl Pts',(0.0908658671394547,7.01307722645044,
89.7220955493157));
#138869=CARTESIAN_POINT('Ctrl Pts',(0.27516482263553,7.00827323207731,89.7137452198809));
#138870=CARTESIAN_POINT('Ctrl Pts',(0.459113446347169,6.99620192718044,
89.7053948904462));
#138871=CARTESIAN_POINT('Ctrl Pts',(0.642920532596751,6.98413991043057,
89.6970509860904));
#138872=CARTESIAN_POINT('Ctrl Pts',(0.826377498685339,6.96482174788211,
89.6887070817346));
#138873=CARTESIAN_POINT('Ctrl Pts',(1.00889015051672,6.93828272893879,89.6803631773788));
#138874=CARTESIAN_POINT('Ctrl Pts',(1.19125620704777,6.91176502630103,89.6720259748991));
#138875=CARTESIAN_POINT('Ctrl Pts',(1.37267913869814,6.87803808122752,89.6636887724193));
#138876=CARTESIAN_POINT('Ctrl Pts',(1.55256981482732,6.83718900810758,89.6553515699396));
#138877=CARTESIAN_POINT('Ctrl Pts',(1.61178883243007,6.82374171871939,89.6526070089038));
#138878=CARTESIAN_POINT('Ctrl Pts',(1.67084185142367,6.80952302811871,89.649862447868));
#138879=CARTESIAN_POINT('Ctrl Pts',(1.72970803380717,6.79453726756156,89.6471178868322));
#138880=CARTESIAN_POINT('Ctrl Pts',(1.90855065694298,6.74900870397534,89.6387795765303));
#138881=CARTESIAN_POINT('Ctrl Pts',(2.08552113086848,6.69643353800226,89.6304412662285));
#138882=CARTESIAN_POINT('Ctrl Pts',(2.26005401679071,6.63700100977001,89.6221029559267));
#138883=CARTESIAN_POINT('Ctrl Pts',(2.43469671288225,6.57753108860776,89.6137593994429));
#138884=CARTESIAN_POINT('Ctrl Pts',(2.6068984517586,6.51119530515688,89.6054158429592));
#138885=CARTESIAN_POINT('Ctrl Pts',(2.77611294520814,6.43823139363193,89.5970722864755));
#138886=CARTESIAN_POINT('Ctrl Pts',(2.94545617630687,6.36521197148107,89.5887223822503));
#138887=CARTESIAN_POINT('Ctrl Pts',(3.1118073281852,6.28555449240028,89.5803724780252));
#138888=CARTESIAN_POINT('Ctrl Pts',(3.27464352289054,6.19954323805319,89.5720225738));
#138889=CARTESIAN_POINT('Ctrl Pts',(3.43772395983796,6.11340297318947,89.5636601453365));
#138890=CARTESIAN_POINT('Ctrl Pts',(3.59727861417787,6.02089004190102,89.5552977168729));
#138891=CARTESIAN_POINT('Ctrl Pts',(3.75281118747542,5.92233355643359,89.5469352884093));
#138892=CARTESIAN_POINT('Ctrl Pts',(3.9084767623256,5.82369279173571,89.5385657089294));
#138893=CARTESIAN_POINT('Ctrl Pts',(4.06011312459827,5.71899834695406,89.5301961294495));
#138894=CARTESIAN_POINT('Ctrl Pts',(4.20725559064723,5.60862077140786,89.5218265499696));
#138895=CARTESIAN_POINT('Ctrl Pts',(4.35462500602218,5.49807295189981,89.5134440614331));
#138896=CARTESIAN_POINT('Ctrl Pts',(4.49748642074404,5.38182469186916,89.5050615728966));
#138897=CARTESIAN_POINT('Ctrl Pts',(4.63540959520822,5.26028558608291,89.4966790843601));
#138898=CARTESIAN_POINT('Ctrl Pts',(4.68054031790502,5.22051599912723,89.4939361967553));
#138899=CARTESIAN_POINT('Ctrl Pts',(4.72514260622551,5.18018020007441,89.4911933091506));
#138900=CARTESIAN_POINT('Ctrl Pts',(4.76920229736218,5.13929333754509,89.4884504215458));
#138901=CARTESIAN_POINT('Ctrl Pts',(4.90162926069797,5.01640271109265,89.4802063266168));
#138902=CARTESIAN_POINT('Ctrl Pts',(5.02944669541314,4.8882574675471,89.4719622316878));
#138903=CARTESIAN_POINT('Ctrl Pts',(5.15222035192789,4.7552341695946,89.4637181367589));
#138904=CARTESIAN_POINT('Ctrl Pts',(5.27488004436522,4.62233434990166,89.4554816943728));
#138905=CARTESIAN_POINT('Ctrl Pts',(5.39250505224846,4.48456574878959,89.4472452519867));
#138906=CARTESIAN_POINT('Ctrl Pts',(5.50469634452335,4.34234322884446,89.4390088096006));
#138907=CARTESIAN_POINT('Ctrl Pts',(5.61726331324664,4.19964447183946,89.4307447872005));
#138908=CARTESIAN_POINT('Ctrl Pts',(5.72435984436157,4.05246214411264,89.4224807648003));
#138909=CARTESIAN_POINT('Ctrl Pts',(5.8256212148699,3.90125159703367,89.4142167424001));
#138910=CARTESIAN_POINT('Ctrl Pts',(5.92639877746629,3.75076350570144,89.4059922039552));
#138911=CARTESIAN_POINT('Ctrl Pts',(6.02139661800876,3.59628589032516,89.3977676655103));
#138912=CARTESIAN_POINT('Ctrl Pts',(6.11029646720853,3.43829952815617,89.3895431270653));
#138913=CARTESIAN_POINT('Ctrl Pts',(6.19983649537233,3.27917548637834,89.3812593626875));
#138914=CARTESIAN_POINT('Ctrl Pts',(6.28319014380522,3.11649224588375,89.3729755983097));
#138915=CARTESIAN_POINT('Ctrl Pts',(6.36007755959843,2.95076939092035,89.3646918339319));
#138916=CARTESIAN_POINT('Ctrl Pts',(6.43696497539165,2.78504653595695,89.3564080695541));
#138917=CARTESIAN_POINT('Ctrl Pts',(6.5073859965539,2.61628438718322,89.3481243051763));
#138918=CARTESIAN_POINT('Ctrl Pts',(6.57110895151813,2.4450263208764,89.3398405407985));
#138919=CARTESIAN_POINT('Origin',(0.,0.,50.));
#138920=CARTESIAN_POINT('',(6.57110895151811,2.44502632087644,87.3401045918022));
#138921=CARTESIAN_POINT('',(6.57110895151812,2.44502632087643,87.8869151327864));
#138922=CARTESIAN_POINT('',(6.57110895151814,2.44502632087636,50.));
#138923=CARTESIAN_POINT('',(7.01124990260052,-0.00116866771971296,89.7735343568779));
#138924=CARTESIAN_POINT('Ctrl Pts',(6.57110895151811,2.44502632087643,87.8869151327864));
#138925=CARTESIAN_POINT('Ctrl Pts',(6.55483330766612,2.48876778414593,87.8890358985076));
#138926=CARTESIAN_POINT('Ctrl Pts',(6.53812136703552,2.53234545570068,87.8911566642287));
#138927=CARTESIAN_POINT('Ctrl Pts',(6.52097655319228,2.57575063917618,87.8932774299499));
#138928=CARTESIAN_POINT('Ctrl Pts',(6.45031461865716,2.75464405040101,87.9020181144463));
#138929=CARTESIAN_POINT('Ctrl Pts',(6.37228337420513,2.93063761010274,87.9107587989428));
#138930=CARTESIAN_POINT('Ctrl Pts',(6.28714218852269,3.1031386794338,87.9194994834392));
#138931=CARTESIAN_POINT('Ctrl Pts',(6.20201632115372,3.27560871295731,87.9282385953413));
#138932=CARTESIAN_POINT('Ctrl Pts',(6.10978318834393,3.44458726555738,87.9369777072434));
#138933=CARTESIAN_POINT('Ctrl Pts',(6.01074900218543,3.60950453597538,87.9457168191455));
#138934=CARTESIAN_POINT('Ctrl Pts',(5.91043168561388,3.77655854698285,87.9545691588197));
#138935=CARTESIAN_POINT('Ctrl Pts',(5.80313597975122,3.93944504675674,87.963421498494));
#138936=CARTESIAN_POINT('Ctrl Pts',(5.68922732022858,4.0975991826025,87.9722738381682));
#138937=CARTESIAN_POINT('Ctrl Pts',(5.57683327151467,4.25365038821803,87.9810084708182));
#138938=CARTESIAN_POINT('Ctrl Pts',(5.45800121358397,4.40509407827471,87.9897431034681));
#138939=CARTESIAN_POINT('Ctrl Pts',(5.33312531499311,4.55141746460152,87.9984777361181));
#138940=CARTESIAN_POINT('Ctrl Pts',(5.20572519397344,4.70069860961348,88.0073889293045));
#138941=CARTESIAN_POINT('Ctrl Pts',(5.07203446343468,4.84465000920222,88.0163001224909));
#138942=CARTESIAN_POINT('Ctrl Pts',(4.93251499830874,4.9827625223323,88.0252113156773));
#138943=CARTESIAN_POINT('Ctrl Pts',(4.79299553318281,5.12087503546238,88.0341225088637));
#138944=CARTESIAN_POINT('Ctrl Pts',(4.64764753941913,5.25314843930193,88.0430337020501));
#138945=CARTESIAN_POINT('Ctrl Pts',(4.49697370569427,5.37911275702549,88.0519448952365));
#138946=CARTESIAN_POINT('Ctrl Pts',(4.36127272085518,5.49255967443044,88.0599705600887));
#138947=CARTESIAN_POINT('Ctrl Pts',(4.22118909180023,5.60094084191064,88.0679962249411));
#138948=CARTESIAN_POINT('Ctrl Pts',(4.07714709029934,5.70390201235643,88.0760218897933));
#138949=CARTESIAN_POINT('Ctrl Pts',(3.93315080419664,5.80683050545215,88.0840450074965));
#138950=CARTESIAN_POINT('Ctrl Pts',(3.78519894466758,5.9043422133058,88.0920681251996));
#138951=CARTESIAN_POINT('Ctrl Pts',(3.63374754084468,5.99612419583728,88.1000912429027));
#138952=CARTESIAN_POINT('Ctrl Pts',(3.48231523636932,6.08789460385748,88.1081133488205));
#138953=CARTESIAN_POINT('Ctrl Pts',(3.32738458037922,6.17393653640493,88.1161354547382));
#138954=CARTESIAN_POINT('Ctrl Pts',(3.1694391085387,6.25398131591112,88.124157560656));
#138955=CARTESIAN_POINT('Ctrl Pts',(3.01143494362723,6.3340558403278,88.1321826476154));
#138956=CARTESIAN_POINT('Ctrl Pts',(2.85041405075633,6.4081285912004,88.1402077345748));
#138957=CARTESIAN_POINT('Ctrl Pts',(2.68688341074461,6.47597746286732,88.1482328215342));
#138958=CARTESIAN_POINT('Ctrl Pts',(2.52332056419156,6.54383969703003,88.1562594889944));
#138959=CARTESIAN_POINT('Ctrl Pts',(2.35724732775964,6.60547547772827,88.1642861564545));
#138960=CARTESIAN_POINT('Ctrl Pts',(2.18918882383458,6.66071158781836,88.1723128239147));
#138961=CARTESIAN_POINT('Ctrl Pts',(2.02099540313495,6.71599204126293,88.1803459351552));
#138962=CARTESIAN_POINT('Ctrl Pts',(1.85081388286993,6.76486245735372,88.1883790463957));
#138963=CARTESIAN_POINT('Ctrl Pts',(1.67918324413966,6.80719987917944,88.1964121576362));
#138964=CARTESIAN_POINT('Ctrl Pts',(1.57805223696294,6.83214662611331,88.2011455585984));
#138965=CARTESIAN_POINT('Ctrl Pts',(1.47641830823632,6.85482608659915,88.2058789595606));
#138966=CARTESIAN_POINT('Ctrl Pts',(1.37439299910715,6.87522148345094,88.2106123605228));
#138967=CARTESIAN_POINT('Ctrl Pts',(1.16421768708813,6.9172366357074,88.220363313817));
#138968=CARTESIAN_POINT('Ctrl Pts',(0.952257338295142,6.94958151096976,
88.2301142671112));
#138969=CARTESIAN_POINT('Ctrl Pts',(0.739323485856769,6.97216088065677,
88.2398652204054));
#138970=CARTESIAN_POINT('Ctrl Pts',(0.526082862258542,6.9947727801616,88.2496302217771));
#138971=CARTESIAN_POINT('Ctrl Pts',(0.311865967991078,7.00759102779147,
88.2593952231488));
#138972=CARTESIAN_POINT('Ctrl Pts',(0.097490257987396,7.01057217437333,
88.2691602245204));
#138973=CARTESIAN_POINT('Ctrl Pts',(-0.11652813212578,7.01354835200152,
88.2789089496581));
#138974=CARTESIAN_POINT('Ctrl Pts',(-0.33070477101601,7.00672019781765,
88.2886576747957));
#138975=CARTESIAN_POINT('Ctrl Pts',(-0.544224464783171,6.99009630079811,
88.2984063999334));
#138976=CARTESIAN_POINT('Ctrl Pts',(-0.757158129782745,6.97351802993002,
88.3081283686006));
#138977=CARTESIAN_POINT('Ctrl Pts',(-0.969438409359905,6.94719769186361,
88.3178503372678));
#138978=CARTESIAN_POINT('Ctrl Pts',(-1.18025558019842,6.91119550641642,
88.327572305935));
#138979=CARTESIAN_POINT('Ctrl Pts',(-1.38967782887983,6.87543153802709,
88.3372299468748));
#138980=CARTESIAN_POINT('Ctrl Pts',(-1.59765621597616,6.83011340267251,
88.3468875878145));
#138981=CARTESIAN_POINT('Ctrl Pts',(-1.80339645972762,6.77535148693718,
88.3565452287543));
#138982=CARTESIAN_POINT('Ctrl Pts',(-1.89382638005402,6.75128173963559,
88.3607900944393));
#138983=CARTESIAN_POINT('Ctrl Pts',(-1.98382391001562,6.72538821539914,
88.3650349601243));
#138984=CARTESIAN_POINT('Ctrl Pts',(-2.0733216145128,6.69768348351085,88.3692798258093));
#138985=CARTESIAN_POINT('Ctrl Pts',(-2.23886802656909,6.64643726455077,
88.3771316728232));
#138986=CARTESIAN_POINT('Ctrl Pts',(-2.40263517021789,6.58901142800105,
88.3849835198372));
#138987=CARTESIAN_POINT('Ctrl Pts',(-2.56411245436094,6.52556157613206,
88.3928353668511));
#138988=CARTESIAN_POINT('Ctrl Pts',(-2.72554394485167,6.4621297181281,88.4006849871448));
#138989=CARTESIAN_POINT('Ctrl Pts',(-2.88468651288709,6.39267738239819,
88.4085346074384));
#138990=CARTESIAN_POINT('Ctrl Pts',(-3.04104683841114,6.31740933366595,
88.416384227732));
#138991=CARTESIAN_POINT('Ctrl Pts',(-3.19739468056335,6.24214729412458,
88.4242332213339));
#138992=CARTESIAN_POINT('Ctrl Pts',(-3.35096037900811,6.16107063202598,
88.4320822149357));
#138993=CARTESIAN_POINT('Ctrl Pts',(-3.50127287565799,6.0744312336779,88.4399312085376));
#138994=CARTESIAN_POINT('Ctrl Pts',(-3.65166147112327,5.98774797233953,
88.447784175855));
#138995=CARTESIAN_POINT('Ctrl Pts',(-3.79879324307845,5.89549653848571,
88.4556371431725));
#138996=CARTESIAN_POINT('Ctrl Pts',(-3.94222363728883,5.79797372847629,
88.46349011049));
#138997=CARTESIAN_POINT('Ctrl Pts',(-4.08569045799994,5.70042615094998,
88.4713450721973));
#138998=CARTESIAN_POINT('Ctrl Pts',(-4.22545372090904,5.59760475624016,
88.4792000339046));
#138999=CARTESIAN_POINT('Ctrl Pts',(-4.36110046444975,5.48984783955587,
88.4870549956119));
#139000=CARTESIAN_POINT('Ctrl Pts',(-4.49688184872204,5.38198396512444,
88.4949177540253));
#139001=CARTESIAN_POINT('Ctrl Pts',(-4.62853826331798,5.26917503242696,
88.5027805124387));
#139002=CARTESIAN_POINT('Ctrl Pts',(-4.75569182611874,5.15179792087068,
88.5106432708521));
#139003=CARTESIAN_POINT('Ctrl Pts',(-4.84896985523927,5.06569175609898,
88.5164112775999));
#139004=CARTESIAN_POINT('Ctrl Pts',(-4.93982542595665,4.97712803729308,
88.5221792843478));
#139005=CARTESIAN_POINT('Ctrl Pts',(-5.02812298621087,4.88626706167785,
88.5279472910957));
#139006=CARTESIAN_POINT('Ctrl Pts',(-5.15637575336652,4.75429091742694,
88.5363253575367));
#139007=CARTESIAN_POINT('Ctrl Pts',(-5.27951448298897,4.61717463325797,
88.5447034239777));
#139008=CARTESIAN_POINT('Ctrl Pts',(-5.39712312308541,4.47534228375403,
88.5530814904187));
#139009=CARTESIAN_POINT('Ctrl Pts',(-5.51465134379118,4.33360691752544,
88.5614538280374));
#139010=CARTESIAN_POINT('Ctrl Pts',(-5.62665680482392,4.18716216747682,
88.5698261656562));
#139011=CARTESIAN_POINT('Ctrl Pts',(-5.7327618889856,4.03646722849254,88.5781985032749));
#139012=CARTESIAN_POINT('Ctrl Pts',(-5.83880998013208,3.88585323340474,
88.5865663437974));
#139013=CARTESIAN_POINT('Ctrl Pts',(-5.93896382489068,3.73099386951992,
88.59493418432));
#139014=CARTESIAN_POINT('Ctrl Pts',(-6.03288724599317,3.57237988456337,
88.6033020248426));
#139015=CARTESIAN_POINT('Ctrl Pts',(-6.12677397640755,3.41382786132182,
88.6116665965125));
#139016=CARTESIAN_POINT('Ctrl Pts',(-6.21443496943469,3.25152442428976,
88.6200311681824));
#139017=CARTESIAN_POINT('Ctrl Pts',(-6.29557815673689,3.08598804840805,
88.6283957398523));
#139018=CARTESIAN_POINT('Ctrl Pts',(-6.37670152328574,2.92049210790714,
88.6367582683179));
#139019=CARTESIAN_POINT('Ctrl Pts',(-6.45131011497981,2.75176509848601,
88.6451207967834));
#139020=CARTESIAN_POINT('Ctrl Pts',(-6.51915828324742,2.58034917026099,
88.653483325249));
#139021=CARTESIAN_POINT('Ctrl Pts',(-6.58701186601111,2.40891956250863,
88.6618465210705));
#139022=CARTESIAN_POINT('Ctrl Pts',(-6.64810382092013,2.23480091062192,
88.670209716892));
#139023=CARTESIAN_POINT('Ctrl Pts',(-6.70223675191771,2.05855509611562,
88.6785729127135));
#139024=CARTESIAN_POINT('Ctrl Pts',(-6.75637337467263,1.88229726199818,
88.6869366788881));
#139025=CARTESIAN_POINT('Ctrl Pts',(-6.80354993041998,1.70391229025803,
88.6953004450628));
#139026=CARTESIAN_POINT('Ctrl Pts',(-6.84361894436214,1.52397713462755,
88.7036642112375));
#139027=CARTESIAN_POINT('Ctrl Pts',(-6.88369603307284,1.34400571819127,
88.7120296628911));
#139028=CARTESIAN_POINT('Ctrl Pts',(-6.9166626524395,1.16248381586834,88.7203951145446));
#139029=CARTESIAN_POINT('Ctrl Pts',(-6.94242239497053,0.979998904240033,
88.7287605661981));
#139030=CARTESIAN_POINT('Ctrl Pts',(-6.9681907643887,0.797452878773525,
88.737128819425));
#139031=CARTESIAN_POINT('Ctrl Pts',(-6.98674739830947,0.61394352633423,
88.7454970726519));
#139032=CARTESIAN_POINT('Ctrl Pts',(-6.99804768035478,0.430064211462848,
88.7538653258787));
#139033=CARTESIAN_POINT('Ctrl Pts',(-7.00935843937369,0.246014414233438,
88.7622413376702));
#139034=CARTESIAN_POINT('Ctrl Pts',(-7.01339938243069,0.0615942976434029,
88.7706173494616));
#139035=CARTESIAN_POINT('Ctrl Pts',(-7.01017800193812,-0.122600748948895,
88.7789933612531));
#139036=CARTESIAN_POINT('Ctrl Pts',(-7.00695504164076,-0.306886127067796,
88.7873734807442));
#139037=CARTESIAN_POINT('Ctrl Pts',(-6.99646266769394,-0.490945886667178,
88.7957536002354));
#139038=CARTESIAN_POINT('Ctrl Pts',(-6.97876039602643,-0.674188324841817,
88.8041337197265));
#139039=CARTESIAN_POINT('Ctrl Pts',(-6.96103789727112,-0.857640140714186,
88.8125234145657));
#139040=CARTESIAN_POINT('Ctrl Pts',(-6.93608907723636,-1.04027244236608,
88.8209131094049));
#139041=CARTESIAN_POINT('Ctrl Pts',(-6.90402505451861,-1.22150096564813,
88.8293028042441));
#139042=CARTESIAN_POINT('Ctrl Pts',(-6.88366815981473,-1.33655982767137,
88.8346292767189));
#139043=CARTESIAN_POINT('Ctrl Pts',(-6.86044432726614,-1.45105306635245,
88.8399557491938));
#139044=CARTESIAN_POINT('Ctrl Pts',(-6.83439251135128,-1.56483403697823,
88.8452822216686));
#139045=CARTESIAN_POINT('Ctrl Pts',(-6.7933995096405,-1.74387044421985,
88.8536635220735));
#139046=CARTESIAN_POINT('Ctrl Pts',(-6.74531936724503,-1.92150377135421,
88.8620448224783));
#139047=CARTESIAN_POINT('Ctrl Pts',(-6.69026031388915,-2.09715128088078,
88.8704261228831));
#139048=CARTESIAN_POINT('Ctrl Pts',(-6.63527103982333,-2.27257618290196,
88.8787968012167));
#139049=CARTESIAN_POINT('Ctrl Pts',(-6.57332057867142,-2.44601997278679,
88.8871674795502));
#139050=CARTESIAN_POINT('Ctrl Pts',(-6.50456798830475,-2.61691074513846,
88.8955381578837));
#139051=CARTESIAN_POINT('Ctrl Pts',(-6.4358934203239,-2.78760758580401,
88.9038993369344));
#139052=CARTESIAN_POINT('Ctrl Pts',(-6.36043222999064,-2.95575688132307,
88.9122605159852));
#139053=CARTESIAN_POINT('Ctrl Pts',(-6.27839317148957,-3.12080209989245,
88.920621695036));
#139054=CARTESIAN_POINT('Ctrl Pts',(-6.19646056834422,-3.28563315282204,
88.9289720244706));
#139055=CARTESIAN_POINT('Ctrl Pts',(-6.10796726726344,-3.44736787086974,
88.9373223539053));
#139056=CARTESIAN_POINT('Ctrl Pts',(-6.01316994023207,-3.60546998772552,
88.94567268334));
#139057=CARTESIAN_POINT('Ctrl Pts',(-5.91844555407317,-3.76345045445989,
88.9540165876956));
#139058=CARTESIAN_POINT('Ctrl Pts',(-5.81742697604407,-3.91780361025139,
88.9623604920514));
#139059=CARTESIAN_POINT('Ctrl Pts',(-5.71041712792692,-4.06801705841788,
88.970704396407));
#139060=CARTESIAN_POINT('Ctrl Pts',(-5.60349323078715,-4.21810985420599,
88.9790415988867));
#139061=CARTESIAN_POINT('Ctrl Pts',(-5.49058785041384,-4.36406930759813,
88.9873788013663));
#139062=CARTESIAN_POINT('Ctrl Pts',(-5.37204769194044,-4.50541120853773,
88.995716003846));
#139063=CARTESIAN_POINT('Ctrl Pts',(-5.33302492609325,-4.55194018214291,
88.9984605648823));
#139064=CARTESIAN_POINT('Ctrl Pts',(-5.29339187258074,-4.59796899144018,
89.0012051259186));
#139065=CARTESIAN_POINT('Ctrl Pts',(-5.2531619064357,-4.64348108074889,
89.0039496869549));
#139066=CARTESIAN_POINT('Ctrl Pts',(-5.1309383753439,-4.78175234457795,
89.0122879972569));
#139067=CARTESIAN_POINT('Ctrl Pts',(-5.00330256798195,-4.9151382411288,
89.0206263075589));
#139068=CARTESIAN_POINT('Ctrl Pts',(-4.87068120155903,-5.04322230278217,
89.0289646178609));
#139069=CARTESIAN_POINT('Ctrl Pts',(-4.73797639427257,-5.17138695058088,
89.0373081743447));
#139070=CARTESIAN_POINT('Ctrl Pts',(-4.60028000697832,-5.29424288232747,
89.0456517308286));
#139071=CARTESIAN_POINT('Ctrl Pts',(-4.45805313999055,-5.4114128250874,
89.0539952873125));
#139072=CARTESIAN_POINT('Ctrl Pts',(-4.3157180674225,-5.52867191022891,
89.0623451915377));
#139073=CARTESIAN_POINT('Ctrl Pts',(-4.16884589258228,-5.64023616957493,
89.070695095763));
#139074=CARTESIAN_POINT('Ctrl Pts',(-4.01792842082438,-5.74577042420176,
89.0790449999882));
#139075=CARTESIAN_POINT('Ctrl Pts',(-3.86678458402651,-5.85146297240116,
89.087407428452));
#139076=CARTESIAN_POINT('Ctrl Pts',(-3.71158359399111,-5.95110725407478,
89.0957698569157));
#139077=CARTESIAN_POINT('Ctrl Pts',(-3.55284498571996,-6.04441221873099,
89.1041322853794));
#139078=CARTESIAN_POINT('Ctrl Pts',(-3.39397063429936,-6.13779697185141,
89.1125018648594));
#139079=CARTESIAN_POINT('Ctrl Pts',(-3.23155291680686,-6.22483143730628,
89.1208714443395));
#139080=CARTESIAN_POINT('Ctrl Pts',(-3.06613377843793,-6.30527162105028,
89.1292410238195));
#139081=CARTESIAN_POINT('Ctrl Pts',(-2.90045950120278,-6.38583587397684,
89.1376235123561));
#139082=CARTESIAN_POINT('Ctrl Pts',(-2.73177485181647,-6.45978538945171,
89.1460060008928));
#139083=CARTESIAN_POINT('Ctrl Pts',(-2.56064076546608,-6.52692465352047,
89.1543884894294));
#139084=CARTESIAN_POINT('Ctrl Pts',(-2.50464288822122,-6.54889372086299,
89.1571313770334));
#139085=CARTESIAN_POINT('Ctrl Pts',(-2.44838285924254,-6.57013401149291,
89.1598742646375));
#139086=CARTESIAN_POINT('Ctrl Pts',(-2.39188062497519,-6.59063985045218,
89.1626171522415));
#139087=CARTESIAN_POINT('Ctrl Pts',(-2.2190534338493,-6.65336244177911,
89.1710070073743));
#139088=CARTESIAN_POINT('Ctrl Pts',(-2.04361021329518,-6.70933634883609,
89.1793968625071));
#139089=CARTESIAN_POINT('Ctrl Pts',(-1.86610484110356,-6.75834885785795,
89.1877867176399));
#139090=CARTESIAN_POINT('Ctrl Pts',(-1.68876326838081,-6.80731613882364,
89.1961688307319));
#139091=CARTESIAN_POINT('Ctrl Pts',(-1.5093636528376,-6.84933474068121,
89.204550943824));
#139092=CARTESIAN_POINT('Ctrl Pts',(-1.32847692186191,-6.88424110781866,
89.2129330569161));
#139093=CARTESIAN_POINT('Ctrl Pts',(-1.14773052065156,-6.91912039501342,
89.221308667265));
#139094=CARTESIAN_POINT('Ctrl Pts',(-0.965499625721542,-6.94689838581216,
89.2296842776139));
#139095=CARTESIAN_POINT('Ctrl Pts',(-0.782367750468291,-6.96746203904458,
89.2380598879627));
#139096=CARTESIAN_POINT('Ctrl Pts',(-0.599351067884293,-6.98801275743371,
89.2464302299283));
#139097=CARTESIAN_POINT('Ctrl Pts',(-0.415434860817747,-7.00135814988565,
89.2548005718939));
#139098=CARTESIAN_POINT('Ctrl Pts',(-0.231210660257582,-7.0074366349674,
89.2631709138595));
#139099=CARTESIAN_POINT('Ctrl Pts',(-0.0470753342562295,-7.01351218762942,
89.2715372177538));
#139100=CARTESIAN_POINT('Ctrl Pts',(0.137367360978798,-7.01232781312482,
89.2799035216481));
#139101=CARTESIAN_POINT('Ctrl Pts',(0.321522512185865,-7.00387391638782,
89.2882698255424));
#139102=CARTESIAN_POINT('Ctrl Pts',(0.505626160358737,-6.9954223839688,
89.296633789616));
#139103=CARTESIAN_POINT('Ctrl Pts',(0.689442096770567,-6.97970539686847,
89.3049977536896));
#139104=CARTESIAN_POINT('Ctrl Pts',(0.872376589459558,-6.95676545879354,
89.3133617177632));
#139105=CARTESIAN_POINT('Ctrl Pts',(1.05528293157012,-6.93382905079387,
89.3217243947617));
#139106=CARTESIAN_POINT('Ctrl Pts',(1.23730777438678,-6.90367194879413,
89.3300870717603));
#139107=CARTESIAN_POINT('Ctrl Pts',(1.41786325977379,-6.866388449475,89.3384497487588));
#139108=CARTESIAN_POINT('Ctrl Pts',(1.59841502785335,-6.82910571775498,
89.3468122535851));
#139109=CARTESIAN_POINT('Ctrl Pts',(1.77749717704757,-6.78469694812975,
89.3551747584114));
#139110=CARTESIAN_POINT('Ctrl Pts',(1.95453235461152,-6.73330749611784,
89.3635372632377));
#139111=CARTESIAN_POINT('Ctrl Pts',(2.13158748487358,-6.68191225227273,
89.3719007105576));
#139112=CARTESIAN_POINT('Ctrl Pts',(2.30659486809076,-6.62353484960551,
89.3802641578776));
#139113=CARTESIAN_POINT('Ctrl Pts',(2.47899220149334,-6.55837054667051,
89.3886276051976));
#139114=CARTESIAN_POINT('Ctrl Pts',(2.65149104729088,-6.49316787316256,
89.3969959771504));
#139115=CARTESIAN_POINT('Ctrl Pts',(2.821376464151,-6.42117042921992,89.4053643491032));
#139116=CARTESIAN_POINT('Ctrl Pts',(2.98810506373111,-6.34262206745795,
89.413732721056));
#139117=CARTESIAN_POINT('Ctrl Pts',(3.15488361955717,-6.26405017055391,
89.4221036003917));
#139118=CARTESIAN_POINT('Ctrl Pts',(3.31850317695323,-6.17892358688698,
89.4304744797274));
#139119=CARTESIAN_POINT('Ctrl Pts',(3.47844422945862,-6.08753253010167,
89.4388453590632));
#139120=CARTESIAN_POINT('Ctrl Pts',(3.63852079828832,-5.99606403866218,
89.4472233309544));
#139121=CARTESIAN_POINT('Ctrl Pts',(3.79491235147865,-5.8983206359863,89.4556013028457));
#139122=CARTESIAN_POINT('Ctrl Pts',(3.94712670688908,-5.79463694481915,
89.463979274737));
#139123=CARTESIAN_POINT('Ctrl Pts',(4.04386016924046,-5.72874511478165,
89.4693035440961));
#139124=CARTESIAN_POINT('Ctrl Pts',(4.13890717369779,-5.66045504662359,
89.4746278134552));
#139125=CARTESIAN_POINT('Ctrl Pts',(4.23214814517178,-5.58986123618637,
89.4799520828143));
#139126=CARTESIAN_POINT('Ctrl Pts',(4.36984553972061,-5.48560895722776,
89.4878149140036));
#139127=CARTESIAN_POINT('Ctrl Pts',(4.50388872817933,-5.37611348052323,
89.4956777451928));
#139128=CARTESIAN_POINT('Ctrl Pts',(4.63383618386507,-5.26167167196917,
89.5035405763821));
#139129=CARTESIAN_POINT('Ctrl Pts',(4.76368379208412,-5.14731779683873,
89.5113973660235));
#139130=CARTESIAN_POINT('Ctrl Pts',(4.88944164157191,-5.02802539826377,
89.5192541556649));
#139131=CARTESIAN_POINT('Ctrl Pts',(5.0106985497752,-4.90413362438063,89.5271109453062));
#139132=CARTESIAN_POINT('Ctrl Pts',(5.13188707482215,-4.78031171959336,
89.5349633040902));
#139133=CARTESIAN_POINT('Ctrl Pts',(5.24857944202502,-4.65189587085254,
89.5428156628741));
#139134=CARTESIAN_POINT('Ctrl Pts',(5.36039904202529,-4.51926417381794,
89.5506680216581));
#139135=CARTESIAN_POINT('Ctrl Pts',(5.47219224011345,-4.38666379267438,
89.5585185264085));
#139136=CARTESIAN_POINT('Ctrl Pts',(5.57911470886249,-4.24984983017631,
89.5663690311589));
#139137=CARTESIAN_POINT('Ctrl Pts',(5.68082814214389,-4.1092357174937,89.5742195359094));
#139138=CARTESIAN_POINT('Ctrl Pts',(5.78252521293952,-3.96864422519018,
89.582068777761));
#139139=CARTESIAN_POINT('Ctrl Pts',(5.87901469524462,-3.82425411056422,
89.5899180196126));
#139140=CARTESIAN_POINT('Ctrl Pts',(5.97000016640154,-3.67650983619867,
89.5977672614642));
#139141=CARTESIAN_POINT('Ctrl Pts',(6.06101629234464,-3.52871578389516,
89.6056191478791));
#139142=CARTESIAN_POINT('Ctrl Pts',(6.14652450283191,-3.37756563973382,
89.6134710342939));
#139143=CARTESIAN_POINT('Ctrl Pts',(6.22627301396429,-3.22353081543826,
89.6213229207088));
#139144=CARTESIAN_POINT('Ctrl Pts',(6.28483135307921,-3.11042496119059,
89.6270884631728));
#139145=CARTESIAN_POINT('Ctrl Pts',(6.3402851136845,-2.99576432463122,89.6328540056367));
#139146=CARTESIAN_POINT('Ctrl Pts',(6.39255086948626,-2.87974303428804,
89.6386195481007));
#139147=CARTESIAN_POINT('Ctrl Pts',(6.47849319973308,-2.68896534634728,
89.6481000223977));
#139148=CARTESIAN_POINT('Ctrl Pts',(6.55577935381089,-2.4945874012626,89.6575804966947));
#139149=CARTESIAN_POINT('Ctrl Pts',(6.62418441874926,-2.29734789461664,
89.6670609709917));
#139150=CARTESIAN_POINT('Ctrl Pts',(6.69302324126454,-2.09885768920228,
89.6766015611231));
#139151=CARTESIAN_POINT('Ctrl Pts',(6.75286798945196,-1.89746962490714,
89.6861421512546));
#139152=CARTESIAN_POINT('Ctrl Pts',(6.80354173911682,-1.69394402699595,
89.695682741386));
#139153=CARTESIAN_POINT('Ctrl Pts',(6.85433638479804,-1.48993286339886,
89.7052460931908));
#139154=CARTESIAN_POINT('Ctrl Pts',(6.89591623823064,-1.28377405662141,
89.7148094449957));
#139155=CARTESIAN_POINT('Ctrl Pts',(6.92815527618832,-1.07623930030637,
89.7243727968005));
#139156=CARTESIAN_POINT('Ctrl Pts',(6.9604478597256,-0.868359851050176,
89.7339520323056));
#139157=CARTESIAN_POINT('Ctrl Pts',(6.98336857798893,-0.659099972771663,
89.7435312678107));
#139158=CARTESIAN_POINT('Ctrl Pts',(6.99684288020564,-0.449239660109893,
89.7531105033158));
#139159=CARTESIAN_POINT('Ctrl Pts',(7.00641905063446,-0.300092187537877,
89.7599184545032));
#139160=CARTESIAN_POINT('Ctrl Pts',(7.0112249877683,-0.150641534984156,
89.7667264056905));
#139161=CARTESIAN_POINT('Ctrl Pts',(7.01124990260052,-0.00116866771990912,
89.7735343568778));
#139162=CARTESIAN_POINT('Ctrl Pts',(7.01124990260064,-0.00116866700483817,
89.7735343569104));
#139163=CARTESIAN_POINT('Ctrl Pts',(7.01127887818485,0.172666190259039,
89.7814519090693));
#139164=CARTESIAN_POINT('Ctrl Pts',(7.00484218383642,0.346555053651736,
89.7893694612282));
#139165=CARTESIAN_POINT('Ctrl Pts',(6.99193196050225,0.520109625182234,
89.7972870133871));
#139166=CARTESIAN_POINT('Ctrl Pts',(6.97883374054472,0.696191470840531,
89.805319859684));
#139167=CARTESIAN_POINT('Ctrl Pts',(6.95906597300057,0.871962073712557,
89.8133527059809));
#139168=CARTESIAN_POINT('Ctrl Pts',(6.93265382099713,1.04687036480829,89.8213855522778));
#139169=CARTESIAN_POINT('Ctrl Pts',(6.90625792285003,1.22167101854697,89.8294134552165));
#139170=CARTESIAN_POINT('Ctrl Pts',(6.87322583208172,1.39561005565585,89.8374413581551));
#139171=CARTESIAN_POINT('Ctrl Pts',(6.83363461634404,1.56814045697588,89.8454692610938));
#139172=CARTESIAN_POINT('Ctrl Pts',(6.79406011725628,1.74059801056267,89.8534937744006));
#139173=CARTESIAN_POINT('Ctrl Pts',(6.74793208756169,1.91164775566082,89.8615182877075));
#139174=CARTESIAN_POINT('Ctrl Pts',(6.69537887420091,2.08075185771975,89.8695428010143));
#139175=CARTESIAN_POINT('Ctrl Pts',(6.65730511031184,2.20326443578542,89.8753564022279));
#139176=CARTESIAN_POINT('Ctrl Pts',(6.61586002755452,2.32475596066717,89.8811700034414));
#139177=CARTESIAN_POINT('Ctrl Pts',(6.57110895151814,2.44502632087636,89.8869836046549));
#139178=CARTESIAN_POINT('',(7.01124998073505,-0.000519752638901176,89.2264656431278));
#139179=CARTESIAN_POINT('Ctrl Pts',(6.57110895151813,2.4450263208764,89.3398405407985));
#139180=CARTESIAN_POINT('Ctrl Pts',(6.63433766300281,2.27509655427943,89.3316210263686));
#139181=CARTESIAN_POINT('Ctrl Pts',(6.69097174824357,2.10270978866334,89.3234015119385));
#139182=CARTESIAN_POINT('Ctrl Pts',(6.74083387325627,1.92841521868627,89.3151819975085));
#139183=CARTESIAN_POINT('Ctrl Pts',(6.79071773222913,1.75404467699245,89.3069589003472));
#139184=CARTESIAN_POINT('Ctrl Pts',(6.83382363633967,1.57776500168886,89.2987358031858));
#139185=CARTESIAN_POINT('Ctrl Pts',(6.87002445706047,1.40013946515733,89.2905127060244));
#139186=CARTESIAN_POINT('Ctrl Pts',(6.90623358362138,1.22247317459653,89.282287722173));
#139187=CARTESIAN_POINT('Ctrl Pts',(6.93553440626854,1.043460747489,89.2740627383215));
#139188=CARTESIAN_POINT('Ctrl Pts',(6.95785121770788,0.863674125316405,
89.26583775447));
#139189=CARTESIAN_POINT('Ctrl Pts',(6.9801856822653,0.683745287734539,89.2576062644646));
#139190=CARTESIAN_POINT('Ctrl Pts',(6.99552506285632,0.503041375759832,
89.2493747744591));
#139191=CARTESIAN_POINT('Ctrl Pts',(7.00384559704583,0.322138813621992,
89.2411432844537));
#139192=CARTESIAN_POINT('Ctrl Pts',(7.00879106930715,0.214615837010341,
89.2362507373451));
#139193=CARTESIAN_POINT('Ctrl Pts',(7.01125795299141,0.10702271672289,89.2313581902364));
#139194=CARTESIAN_POINT('Ctrl Pts',(7.01124998073505,-0.000519752639105816,
89.2264656431278));
#139195=CARTESIAN_POINT('Ctrl Pts',(7.01124998073499,-0.000519753477888864,
89.2264656430896));
#139196=CARTESIAN_POINT('Ctrl Pts',(7.0112254927832,-0.330851648839633,
89.2114374931025));
#139197=CARTESIAN_POINT('Ctrl Pts',(6.98785181831592,-0.660634656290872,
89.1964093431154));
#139198=CARTESIAN_POINT('Ctrl Pts',(6.9413845472389,-0.987323214480959,
89.1813811931284));
#139199=CARTESIAN_POINT('Ctrl Pts',(6.93080397754665,-1.06171000280479,
89.1779592924099));
#139200=CARTESIAN_POINT('Ctrl Pts',(6.9190262741439,-1.13593643033091,89.1745373916915));
#139201=CARTESIAN_POINT('Ctrl Pts',(6.9060548208089,-1.20997246848107,89.171115490973));
#139202=CARTESIAN_POINT('Ctrl Pts',(6.87624906189091,-1.38009221122353,
89.1632526597835));
#139203=CARTESIAN_POINT('Ctrl Pts',(6.84010970381206,-1.54935763176299,
89.155389828594));
#139204=CARTESIAN_POINT('Ctrl Pts',(6.79769903530169,-1.71724034076727,
89.1475269974045));
#139205=CARTESIAN_POINT('Ctrl Pts',(6.75532095379201,-1.8849940540696,89.1396702077629));
#139206=CARTESIAN_POINT('Ctrl Pts',(6.70668123725754,-2.05136680136492,
89.1318134181213));
#139207=CARTESIAN_POINT('Ctrl Pts',(6.65189365013445,-2.21583786180331,
89.1239566284797));
#139208=CARTESIAN_POINT('Ctrl Pts',(6.59713696061686,-2.38021616834961,
89.1161042696955));
#139209=CARTESIAN_POINT('Ctrl Pts',(6.53623941750465,-2.54269456080801,
89.1082519109113));
#139210=CARTESIAN_POINT('Ctrl Pts',(6.46936522736334,-2.70276527236126,
89.1003995521271));
#139211=CARTESIAN_POINT('Ctrl Pts',(6.40250682699863,-2.86279818935177,
89.0925490473765));
#139212=CARTESIAN_POINT('Ctrl Pts',(6.3296747272547,-3.02042420213621,89.0846985426258));
#139213=CARTESIAN_POINT('Ctrl Pts',(6.25108206855452,-3.17515346632192,
89.0768480378752));
#139214=CARTESIAN_POINT('Ctrl Pts',(6.17250205293624,-3.3298578394454,89.0689987960233));
#139215=CARTESIAN_POINT('Ctrl Pts',(6.08816349859701,-3.48166605282902,
89.0611495541715));
#139216=CARTESIAN_POINT('Ctrl Pts',(5.99832628749871,-3.63011133592374,
89.0533003123196));
#139217=CARTESIAN_POINT('Ctrl Pts',(5.90845880848544,-3.7786066331401,89.0454484259046));
#139218=CARTESIAN_POINT('Ctrl Pts',(5.81308916995875,-3.92373641020055,
89.0375965394895));
#139219=CARTESIAN_POINT('Ctrl Pts',(5.71252162342565,-4.06506128667138,
89.0297446530744));
#139220=CARTESIAN_POINT('Ctrl Pts',(5.63867612576406,-4.16883438440243,
89.0239791106118));
#139221=CARTESIAN_POINT('Ctrl Pts',(5.56202896335448,-4.27055652372627,
89.0182135681491));
#139222=CARTESIAN_POINT('Ctrl Pts',(5.48271468558665,-4.37006478658526,
89.0124480256864));
#139223=CARTESIAN_POINT('Ctrl Pts',(5.34989049828883,-4.53670696647567,
89.0027927213265));
#139224=CARTESIAN_POINT('Ctrl Pts',(5.20965370605494,-4.6970549548856,88.9931374169666));
#139225=CARTESIAN_POINT('Ctrl Pts',(5.06258545705823,-4.85055203584938,
88.9834821126067));
#139226=CARTESIAN_POINT('Ctrl Pts',(4.91470247755191,-5.00489946184581,
88.973773319672));
#139227=CARTESIAN_POINT('Ctrl Pts',(4.75991221379916,-5.15231986845056,
88.9640645267373));
#139228=CARTESIAN_POINT('Ctrl Pts',(4.59883503057965,-5.29229089563428,
88.9543557338025));
#139229=CARTESIAN_POINT('Ctrl Pts',(4.43698273027734,-5.43293547528582,
88.9446002213318));
#139230=CARTESIAN_POINT('Ctrl Pts',(4.26878290694304,-5.56605879865805,
88.9348447088611));
#139231=CARTESIAN_POINT('Ctrl Pts',(4.09489371856678,-5.69117492229349,
88.9250891963904));
#139232=CARTESIAN_POINT('Ctrl Pts',(3.92083235314166,-5.8164149301401,88.9153240244615));
#139233=CARTESIAN_POINT('Ctrl Pts',(3.74107039234419,-5.9336318663998,88.9055588525326));
#139234=CARTESIAN_POINT('Ctrl Pts',(3.55629603072071,-6.0423824030245,88.8957936806036));
#139235=CARTESIAN_POINT('Ctrl Pts',(3.37177360474716,-6.15098466075983,
88.8860418232651));
#139236=CARTESIAN_POINT('Ctrl Pts',(3.18225246997043,-6.25114357144375,
88.8762899659266));
#139237=CARTESIAN_POINT('Ctrl Pts',(2.98844542841925,-6.34246170535228,
88.866538108588));
#139238=CARTESIAN_POINT('Ctrl Pts',(2.90393152213085,-6.38228302530952,
88.8622855925254));
#139239=CARTESIAN_POINT('Ctrl Pts',(2.81860296076562,-6.42042375869046,
88.8580330764627));
#139240=CARTESIAN_POINT('Ctrl Pts',(2.73252046822376,-6.4568536032063,88.8537805604001));
#139241=CARTESIAN_POINT('Ctrl Pts',(2.56990977430644,-6.52566994577608,
88.8457475148014));
#139242=CARTESIAN_POINT('Ctrl Pts',(2.40452796168875,-6.58841133439395,
88.8377144692026));
#139243=CARTESIAN_POINT('Ctrl Pts',(2.23687673118098,-6.64484830917916,
88.8296814236039));
#139244=CARTESIAN_POINT('Ctrl Pts',(2.06933327333954,-6.70124900410389,
88.8216535419562));
#139245=CARTESIAN_POINT('Ctrl Pts',(1.89952364748619,-6.7513532357706,88.8136256603085));
#139246=CARTESIAN_POINT('Ctrl Pts',(1.72796962998575,-6.79497958204047,
88.8055977786608));
#139247=CARTESIAN_POINT('Ctrl Pts',(1.55649307081515,-6.838586230585,88.7975735216808));
#139248=CARTESIAN_POINT('Ctrl Pts',(1.3832740427442,-6.87572072724718,88.7895492647008));
#139249=CARTESIAN_POINT('Ctrl Pts',(1.20884953838428,-6.906251469216,88.7815250077207));
#139250=CARTESIAN_POINT('Ctrl Pts',(1.03444612372354,-6.93677851970714,
88.7735017209551));
#139251=CARTESIAN_POINT('Ctrl Pts',(0.85883788263153,-6.96070333514361,
88.7654784341895));
#139252=CARTESIAN_POINT('Ctrl Pts',(0.682572236614536,-6.97794537842645,
88.7574551474239));
#139253=CARTESIAN_POINT('Ctrl Pts',(0.506321033995005,-6.99518600887764,
88.749432518095));
#139254=CARTESIAN_POINT('Ctrl Pts',(0.329412899045756,-7.00574492623365,
88.7414098887662));
#139255=CARTESIAN_POINT('Ctrl Pts',(0.15240031286515,-7.0095934765961,88.7333872594374));
#139256=CARTESIAN_POINT('Ctrl Pts',(-0.0246788174460834,-7.01344347373951,
88.725361614171));
#139257=CARTESIAN_POINT('Ctrl Pts',(-0.201862110634656,-7.01057805956335,
88.7173359689047));
#139258=CARTESIAN_POINT('Ctrl Pts',(-0.378596758095502,-7.00102071538569,
88.7093103236384));
#139259=CARTESIAN_POINT('Ctrl Pts',(-0.482810275928425,-6.99538512286208,
88.7045779141302));
#139260=CARTESIAN_POINT('Ctrl Pts',(-0.586867832591532,-6.98742373395514,
88.6998455046219));
#139261=CARTESIAN_POINT('Ctrl Pts',(-0.69065692121176,-6.97714981777533,
88.6951130951137));
#139262=CARTESIAN_POINT('Ctrl Pts',(-0.882120447475528,-6.95819714898831,
88.6863830462789));
#139263=CARTESIAN_POINT('Ctrl Pts',(-1.07276576004198,-6.93136281656169,
88.6776529974441));
#139264=CARTESIAN_POINT('Ctrl Pts',(-1.26195338716545,-6.89674562464947,
88.6689229486093));
#139265=CARTESIAN_POINT('Ctrl Pts',(-1.45119571812696,-6.86211842313309,
88.66019037547));
#139266=CARTESIAN_POINT('Ctrl Pts',(-1.63897925285721,-6.81970391947092,
88.6514578023307));
#139267=CARTESIAN_POINT('Ctrl Pts',(-1.82467467176382,-6.76965205196867,
88.6427252291914));
#139268=CARTESIAN_POINT('Ctrl Pts',(-2.0130081905177,-6.7188891177918,88.6338685959111));
#139269=CARTESIAN_POINT('Ctrl Pts',(-2.19919353137445,-6.66027023944496,
88.6250119626307));
#139270=CARTESIAN_POINT('Ctrl Pts',(-2.38258960533027,-6.59400434751693,
88.6161553293504));
#139271=CARTESIAN_POINT('Ctrl Pts',(-2.563531851823,-6.52862508888465,88.6074171972435));
#139272=CARTESIAN_POINT('Ctrl Pts',(-2.74175875493713,-6.45580229509339,
88.5986790651366));
#139273=CARTESIAN_POINT('Ctrl Pts',(-2.91667336900007,-6.37578567872743,
88.5899409330297));
#139274=CARTESIAN_POINT('Ctrl Pts',(-3.09514610969175,-6.294141358153,88.5810250491626));
#139275=CARTESIAN_POINT('Ctrl Pts',(-3.27017008926267,-6.20500752522193,
88.5721091652956));
#139276=CARTESIAN_POINT('Ctrl Pts',(-3.4411352453543,-6.10869992598101,
88.5631932814285));
#139277=CARTESIAN_POINT('Ctrl Pts',(-3.61210040144593,-6.01239232674009,
88.5542773975614));
#139278=CARTESIAN_POINT('Ctrl Pts',(-3.77900647356079,-5.90891111491378,
88.5453615136943));
#139279=CARTESIAN_POINT('Ctrl Pts',(-3.9412716704522,-5.79862088622725,
88.5364456298272));
#139280=CARTESIAN_POINT('Ctrl Pts',(-4.10034831522093,-5.69049788840432,
88.5277049453311));
#139281=CARTESIAN_POINT('Ctrl Pts',(-4.25498167604321,-5.57581950384457,
88.518964260835));
#139282=CARTESIAN_POINT('Ctrl Pts',(-4.40465029916025,-5.45496858878284,
88.5102235763389));
#139283=CARTESIAN_POINT('Ctrl Pts',(-4.55429199440605,-5.33413941680803,
88.5014844644371));
#139284=CARTESIAN_POINT('Ctrl Pts',(-4.69897052286826,-5.20714010410923,
88.4927453525354));
#139285=CARTESIAN_POINT('Ctrl Pts',(-4.83819697237339,-5.07439421202344,
88.4840062406336));
#139286=CARTESIAN_POINT('Ctrl Pts',(-4.97922730091604,-4.93992840584875,
88.4751539009592));
#139287=CARTESIAN_POINT('Ctrl Pts',(-5.11466306479463,-4.79956625222803,
88.4663015612848));
#139288=CARTESIAN_POINT('Ctrl Pts',(-5.24403314977661,-4.65378801478366,
88.4574492216104));
#139289=CARTESIAN_POINT('Ctrl Pts',(-5.37168303779884,-4.50994814880194,
88.4487145889607));
#139290=CARTESIAN_POINT('Ctrl Pts',(-5.49342737627533,-4.36083555612009,
88.4399799563111));
#139291=CARTESIAN_POINT('Ctrl Pts',(-5.6088521440018,-4.20694713411357,
88.4312453236614));
#139292=CARTESIAN_POINT('Ctrl Pts',(-5.72661009044385,-4.04994803492858,
88.4223341304747));
#139293=CARTESIAN_POINT('Ctrl Pts',(-5.83779006783849,-3.88797819358361,
88.4134229372879));
#139294=CARTESIAN_POINT('Ctrl Pts',(-5.9419964407593,-3.72159977167129,
88.4045117441011));
#139295=CARTESIAN_POINT('Ctrl Pts',(-6.04620281368011,-3.55522134975898,
88.3956005509144));
#139296=CARTESIAN_POINT('Ctrl Pts',(-6.14343540980544,-3.3844345970281,
88.3866893577276));
#139297=CARTESIAN_POINT('Ctrl Pts',(-6.23334574516367,-3.20983292146958,
88.3777781645409));
#139298=CARTESIAN_POINT('Ctrl Pts',(-6.31432145775738,-3.0525818663815,
88.3697524996884));
#139299=CARTESIAN_POINT('Ctrl Pts',(-6.38939461832771,-2.89216390866809,
88.3617268348359));
#139300=CARTESIAN_POINT('Ctrl Pts',(-6.45831249077132,-2.72907059894887,
88.3537011699835));
#139301=CARTESIAN_POINT('Ctrl Pts',(-6.5272084903727,-2.56602905104567,
88.3456780522801));
#139302=CARTESIAN_POINT('Ctrl Pts',(-6.58995294864213,-2.40031417885692,
88.3376549345769));
#139303=CARTESIAN_POINT('Ctrl Pts',(-6.64634038845979,-2.23243947358674,
88.3296318168736));
#139304=CARTESIAN_POINT('Ctrl Pts',(-6.70272071732769,-2.06458593878639,
88.3216097109556));
#139305=CARTESIAN_POINT('Ctrl Pts',(-6.75274550846451,-1.89457346102356,
88.3135876050377));
#139306=CARTESIAN_POINT('Ctrl Pts',(-6.79625849657735,-1.72293267721062,
88.3055654991198));
#139307=CARTESIAN_POINT('Ctrl Pts',(-6.83978765426365,-1.55122811110228,
88.2975404121601));
#139308=CARTESIAN_POINT('Ctrl Pts',(-6.87680008184139,-1.37789438510245,
88.2895153252005));
#139309=CARTESIAN_POINT('Ctrl Pts',(-6.90719008977293,-1.203474813298,88.2814902382409));
#139310=CARTESIAN_POINT('Ctrl Pts',(-6.93758608286446,-1.02902089043172,
88.2734635707806));
#139311=CARTESIAN_POINT('Ctrl Pts',(-6.96135700378236,-0.853481058366916,
88.2654369033203));
#139312=CARTESIAN_POINT('Ctrl Pts',(-6.9784488376788,-0.677405626194098,
88.25741023586));
#139313=CARTESIAN_POINT('Ctrl Pts',(-6.99555439283926,-0.501188841284845,
88.2493771246193));
#139314=CARTESIAN_POINT('Ctrl Pts',(-7.00597012566691,-0.324435963176175,
88.2413440133786));
#139315=CARTESIAN_POINT('Ctrl Pts',(-7.00969409651052,-0.147699816674087,
88.233310902138));
#139316=CARTESIAN_POINT('Ctrl Pts',(-7.01188839541199,-0.0435604588742939,
88.2285775011767));
#139317=CARTESIAN_POINT('Ctrl Pts',(-7.0117603066995,0.0605730947243702,
88.2238441002155));
#139318=CARTESIAN_POINT('Ctrl Pts',(-7.00931788707192,0.164588336383908,
88.2191106992543));
#139319=CARTESIAN_POINT('Ctrl Pts',(-7.00428642662566,0.378862971384742,
88.2093597459603));
#139320=CARTESIAN_POINT('Ctrl Pts',(-6.98942851048105,0.592761598639739,
88.1996087926664));
#139321=CARTESIAN_POINT('Ctrl Pts',(-6.96482894103494,0.805471529367834,
88.1898578393724));
#139322=CARTESIAN_POINT('Ctrl Pts',(-6.94019393129426,1.01848790865469,
88.180092838001));
#139323=CARTESIAN_POINT('Ctrl Pts',(-6.90578919920208,1.23031212745225,
88.1703278366296));
#139324=CARTESIAN_POINT('Ctrl Pts',(-6.86175136653043,1.44013705820586,
88.1605628352582));
#139325=CARTESIAN_POINT('Ctrl Pts',(-6.81778693580143,1.64961225427453,
88.1508141101208));
#139326=CARTESIAN_POINT('Ctrl Pts',(-6.76422150246786,1.85709478531047,
88.1410653849834));
#139327=CARTESIAN_POINT('Ctrl Pts',(-6.70124196815976,2.06179112585982,
88.131316659846));
#139328=CARTESIAN_POINT('Ctrl Pts',(-6.638435288253,2.26592565432542,88.1215946911791));
#139329=CARTESIAN_POINT('Ctrl Pts',(-6.56626610057202,2.46728922014703,
88.1118727225121));
#139330=CARTESIAN_POINT('Ctrl Pts',(-6.48497048631654,2.6651049424185,88.1021507538452));
#139331=CARTESIAN_POINT('Ctrl Pts',(-6.40421278390713,2.86161176972283,
88.0924931129057));
#139332=CARTESIAN_POINT('Ctrl Pts',(-6.31444902112373,3.05461749445678,
88.0828354719661));
#139333=CARTESIAN_POINT('Ctrl Pts',(-6.21596084663406,3.2433712885842,88.0731778310266));
#139334=CARTESIAN_POINT('Ctrl Pts',(-6.172671903195,3.32633507951881,88.0689329653404));
#139335=CARTESIAN_POINT('Ctrl Pts',(-6.12769814221996,3.40847758267797,
88.0646880996542));
#139336=CARTESIAN_POINT('Ctrl Pts',(-6.08106659565621,3.48973575241654,
88.060443233968));
#139337=CARTESIAN_POINT('Ctrl Pts',(-5.99481091721764,3.64004126608623,
88.052591386954));
#139338=CARTESIAN_POINT('Ctrl Pts',(-5.90291526748684,3.7872574119496,88.0447395399401));
#139339=CARTESIAN_POINT('Ctrl Pts',(-5.80564328722587,3.93092006837956,
88.0368876929261));
#139340=CARTESIAN_POINT('Ctrl Pts',(-5.70839889251204,4.07454198324171,
88.0290380726325));
#139341=CARTESIAN_POINT('Ctrl Pts',(-5.60578141378518,4.21461209768095,
88.0211884523389));
#139342=CARTESIAN_POINT('Ctrl Pts',(-5.49809867869656,4.35069390808123,
88.0133388320453));
#139343=CARTESIAN_POINT('Ctrl Pts',(-5.39042454069712,4.48676485408938,
88.0054898384434));
#139344=CARTESIAN_POINT('Ctrl Pts',(-5.27768618867496,4.6188478312632,87.9976408448416));
#139345=CARTESIAN_POINT('Ctrl Pts',(-5.16023255286608,4.74653837684278,
87.9897918512397));
#139346=CARTESIAN_POINT('Ctrl Pts',(-5.04271945372065,4.87429356840657,
87.9819388839223));
#139347=CARTESIAN_POINT('Ctrl Pts',(-4.92048655960672,4.99765160407217,
87.9740859166048));
#139348=CARTESIAN_POINT('Ctrl Pts',(-4.79392081655473,5.11624371654667,
87.9662329492873));
#139349=CARTESIAN_POINT('Ctrl Pts',(-4.66732293005673,5.23486594743293,
87.95837798758));
#139350=CARTESIAN_POINT('Ctrl Pts',(-4.53639029026041,5.34871959342211,
87.9505230258727));
#139351=CARTESIAN_POINT('Ctrl Pts',(-4.40154341617814,5.45747580095404,
87.9426680641654));
#139352=CARTESIAN_POINT('Ctrl Pts',(-4.26656269530157,5.56633995811281,
87.9348053057521));
#139353=CARTESIAN_POINT('Ctrl Pts',(-4.12766028587753,5.67009634325023,
87.9269425473387));
#139354=CARTESIAN_POINT('Ctrl Pts',(-3.98528667242015,5.76845878039623,
87.9190797889253));
#139355=CARTESIAN_POINT('Ctrl Pts',(-3.88084343253242,5.84061605286622,
87.9133117821774));
#139356=CARTESIAN_POINT('Ctrl Pts',(-3.77453279139011,5.90987148297301,
87.9075437754294));
#139357=CARTESIAN_POINT('Ctrl Pts',(-3.66654084010868,5.97612791281404,
87.9017757686815));
#139358=CARTESIAN_POINT('Ctrl Pts',(-3.50968184488341,6.07236579803378,
87.8933977022405));
#139359=CARTESIAN_POINT('Ctrl Pts',(-3.34892741293785,6.16248813004656,
87.8850196357995));
#139360=CARTESIAN_POINT('Ctrl Pts',(-3.1847824372808,6.24618182489814,87.8766415693584));
#139361=CARTESIAN_POINT('Ctrl Pts',(-3.02074970200762,6.32981829099568,
87.8682692317397));
#139362=CARTESIAN_POINT('Ctrl Pts',(-2.85333133717389,6.40703473506444,
87.859896894121));
#139363=CARTESIAN_POINT('Ctrl Pts',(-2.68305808667884,6.47756326607524,
87.8515245565022));
#139364=CARTESIAN_POINT('Ctrl Pts',(-2.51287629632487,6.54805391357012,
87.8431567159796));
#139365=CARTESIAN_POINT('Ctrl Pts',(-2.33984298091883,6.6118636852555,87.834788875457));
#139366=CARTESIAN_POINT('Ctrl Pts',(-2.16451059628316,6.66877203397132,
87.8264210349344));
#139367=CARTESIAN_POINT('Ctrl Pts',(-1.98924670431671,6.72565815174153,
87.8180564632645));
#139368=CARTESIAN_POINT('Ctrl Pts',(-1.81168584629373,6.77564812142904,
87.8096918915946));
#139369=CARTESIAN_POINT('Ctrl Pts',(-1.63239787270496,6.81857050617564,
87.8013273199246));
#139370=CARTESIAN_POINT('Ctrl Pts',(-1.45315369358412,6.86148240632049,
87.792964791459));
#139371=CARTESIAN_POINT('Ctrl Pts',(-1.27218355970037,6.89733008832511,
87.7846022629935));
#139372=CARTESIAN_POINT('Ctrl Pts',(-1.09007025647445,6.92599259301147,
87.7762397345279));
#139373=CARTESIAN_POINT('Ctrl Pts',(-0.907942420037334,6.95465738505535,
87.7678765387063));
#139374=CARTESIAN_POINT('Ctrl Pts',(-0.724671555730224,6.97613579714193,
87.7595133428848));
#139375=CARTESIAN_POINT('Ctrl Pts',(-0.540849134497942,6.99035827237867,
87.7511501470633));
#139376=CARTESIAN_POINT('Ctrl Pts',(-0.357014176944991,7.0045817175597,
87.7427863808886));
#139377=CARTESIAN_POINT('Ctrl Pts',(-0.172627915286944,7.01154821358835,
87.7344226147139));
#139378=CARTESIAN_POINT('Ctrl Pts',(0.0117144055360298,7.01124021377124,
87.7260588485392));
#139379=CARTESIAN_POINT('Ctrl Pts',(0.196093875303305,7.01093215188553,
87.7176933968856));
#139380=CARTESIAN_POINT('Ctrl Pts',(0.380429057793061,7.00334667154169,
87.709327945232));
#139381=CARTESIAN_POINT('Ctrl Pts',(0.564125623985237,6.98851835819749,
87.7009624935785));
#139382=CARTESIAN_POINT('Ctrl Pts',(0.747883709796349,6.97368507888029,
87.6925942403516));
#139383=CARTESIAN_POINT('Ctrl Pts',(0.931002425257209,6.9516041562705,87.6842259871247));
#139384=CARTESIAN_POINT('Ctrl Pts',(1.11289303816102,6.92236199921044,87.6758577338978));
#139385=CARTESIAN_POINT('Ctrl Pts',(1.29495228961241,6.89309273049896,87.6674817221063));
#139386=CARTESIAN_POINT('Ctrl Pts',(1.47578083824098,6.85664901190533,87.6591057103148));
#139387=CARTESIAN_POINT('Ctrl Pts',(1.65479938759216,6.81316853962418,87.6507296985234));
#139388=CARTESIAN_POINT('Ctrl Pts',(1.83390572985186,6.76966674398218,87.6423495790322));
#139389=CARTESIAN_POINT('Ctrl Pts',(2.01119998495003,6.71912139677559,87.633969459541));
#139390=CARTESIAN_POINT('Ctrl Pts',(2.18611784614881,6.66172014762326,87.6255893400499));
#139391=CARTESIAN_POINT('Ctrl Pts',(2.36123557316148,6.60425331027255,87.6171996452107));
#139392=CARTESIAN_POINT('Ctrl Pts',(2.53397117007375,6.53991502627818,87.6088099503714));
#139393=CARTESIAN_POINT('Ctrl Pts',(2.70377888892343,6.46894166632472,87.6004202555322));
#139394=CARTESIAN_POINT('Ctrl Pts',(2.81158687929119,6.42388190486002,87.5950937830577));
#139395=CARTESIAN_POINT('Ctrl Pts',(2.91821513878084,6.37614866300008,87.5897673105832));
#139396=CARTESIAN_POINT('Ctrl Pts',(3.0235291129734,6.32581206371975,87.5844408381086));
#139397=CARTESIAN_POINT('Ctrl Pts',(3.18924254878909,6.24660651784633,87.5760595377038));
#139398=CARTESIAN_POINT('Ctrl Pts',(3.35203493321549,6.16079312393803,87.567678237299));
#139399=CARTESIAN_POINT('Ctrl Pts',(3.51136137524174,6.06860509960571,87.5592969368942));
#139400=CARTESIAN_POINT('Ctrl Pts',(3.67048589432642,5.97653391009889,87.5509262585607));
#139401=CARTESIAN_POINT('Ctrl Pts',(3.82615294365552,5.87810435336198,87.5425555802273));
#139402=CARTESIAN_POINT('Ctrl Pts',(3.97783933235964,5.77359686923434,87.5341849018938));
#139403=CARTESIAN_POINT('Ctrl Pts',(4.12935358305575,5.66920798315822,87.525823722843));
#139404=CARTESIAN_POINT('Ctrl Pts',(4.27689590856263,5.55875510173926,87.5174625437923));
#139405=CARTESIAN_POINT('Ctrl Pts',(4.41996900154205,5.44256378813398,87.5091013647416));
#139406=CARTESIAN_POINT('Ctrl Pts',(4.56285644030657,5.32652324646393,87.5007510353069));
#139407=CARTESIAN_POINT('Ctrl Pts',(4.70128596083273,5.20475933060727,87.4924007058723));
#139408=CARTESIAN_POINT('Ctrl Pts',(4.8347905229894,5.07763992040711,87.4840503764376));
#139409=CARTESIAN_POINT('Ctrl Pts',(4.96819236137198,4.95061832098858,87.475706472082));
#139410=CARTESIAN_POINT('Ctrl Pts',(5.09667655680907,4.81824966407688,87.4673625677263));
#139411=CARTESIAN_POINT('Ctrl Pts',(5.21980948774704,4.68094172940938,87.4590186633706));
#139412=CARTESIAN_POINT('Ctrl Pts',(5.34284351754677,4.54374408133153,87.450681460891));
#139413=CARTESIAN_POINT('Ctrl Pts',(5.46053463681588,4.40161531085645,87.4423442584113));
#139414=CARTESIAN_POINT('Ctrl Pts',(5.57248631465527,4.25499974564979,87.4340070559317));
#139415=CARTESIAN_POINT('Ctrl Pts',(5.60934018904769,4.20673471087422,87.4312624948952));
#139416=CARTESIAN_POINT('Ctrl Pts',(5.6455723915579,4.15798373429106,87.4285179338587));
#139417=CARTESIAN_POINT('Ctrl Pts',(5.68116969739625,4.10876349184114,87.4257733728222));
#139418=CARTESIAN_POINT('Ctrl Pts',(5.78932614965062,3.95921602814664,87.4174344837487));
#139419=CARTESIAN_POINT('Ctrl Pts',(5.89152974577147,3.80545693513836,87.4090955946751));
#139420=CARTESIAN_POINT('Ctrl Pts',(5.98746751139421,3.64799388191632,87.4007567056016));
#139421=CARTESIAN_POINT('Ctrl Pts',(6.08345224150094,3.49045374569161,87.3924137343856));
#139422=CARTESIAN_POINT('Ctrl Pts',(6.17316485926343,3.32920631627555,87.3840707631696));
#139423=CARTESIAN_POINT('Ctrl Pts',(6.25633828466472,3.16478401006112,87.3757277919537));
#139424=CARTESIAN_POINT('Ctrl Pts',(6.33959903975453,3.00018906518574,87.3673760608595));
#139425=CARTESIAN_POINT('Ctrl Pts',(6.41630674350125,2.83241287896471,87.3590243297653));
#139426=CARTESIAN_POINT('Ctrl Pts',(6.48624191583394,2.66200908559286,87.3506725986712));
#139427=CARTESIAN_POINT('Ctrl Pts',(6.5157398076786,2.59013462673128,87.3471499297148));
#139428=CARTESIAN_POINT('Ctrl Pts',(6.54403342565351,2.51779291191753,87.3436272607585));
#139429=CARTESIAN_POINT('Ctrl Pts',(6.57110895151811,2.44502632087644,87.3401045918022));
#139430=CARTESIAN_POINT('Origin',(0.,0.,50.));
#139431=CARTESIAN_POINT('',(6.57110895151817,2.44502632087629,85.3396537828137));
#139432=CARTESIAN_POINT('',(6.57110895151818,2.44502632087624,85.8868857406669));
#139433=CARTESIAN_POINT('',(6.57110895151814,2.44502632087636,50.));
#139434=CARTESIAN_POINT('',(7.0112498809707,0.00129193205181663,87.7735343569467));
#139435=CARTESIAN_POINT('Ctrl Pts',(6.57110895151818,2.44502632087624,85.8868857406669));
#139436=CARTESIAN_POINT('Ctrl Pts',(6.50935605589572,2.61098977155252,85.894907851644));
#139437=CARTESIAN_POINT('Ctrl Pts',(6.44130892498698,2.77461939656621,85.9029299626212));
#139438=CARTESIAN_POINT('Ctrl Pts',(6.3671830232513,2.93540574894178,85.9109520735983));
#139439=CARTESIAN_POINT('Ctrl Pts',(6.29302610813646,3.09625937237905,85.9189775409295));
#139440=CARTESIAN_POINT('Ctrl Pts',(6.21278549548188,3.25426701379564,85.9270030082606));
#139441=CARTESIAN_POINT('Ctrl Pts',(6.12672374464935,3.40894158343171,85.9350284755918));
#139442=CARTESIAN_POINT('Ctrl Pts',(6.04064005609317,3.56365558066401,85.943055988669));
#139443=CARTESIAN_POINT('Ctrl Pts',(5.94873246003207,3.71503449823715,85.9510835017461));
#139444=CARTESIAN_POINT('Ctrl Pts',(5.85130785221275,3.86261866887393,85.9591110148233));
#139445=CARTESIAN_POINT('Ctrl Pts',(5.75380918994399,4.01031502127616,85.9671446297784));
#139446=CARTESIAN_POINT('Ctrl Pts',(5.65078535490969,4.15421056905528,85.9751782447335));
#139447=CARTESIAN_POINT('Ctrl Pts',(5.54258492985198,4.29387690297215,85.9832118596886));
#139448=CARTESIAN_POINT('Ctrl Pts',(5.51539665690139,4.32897183357445,85.9852305219633));
#139449=CARTESIAN_POINT('Ctrl Pts',(5.48788172555063,4.363799902097,85.9872491842381));
#139450=CARTESIAN_POINT('Ctrl Pts',(5.4600460449783,4.39835466387339,85.9892678465129));
#139451=CARTESIAN_POINT('Ctrl Pts',(5.32558847644155,4.56526810569665,85.9990187998067));
#139452=CARTESIAN_POINT('Ctrl Pts',(5.18356484758662,4.72590019856649,86.0087697531006));
#139453=CARTESIAN_POINT('Ctrl Pts',(5.03453725450321,4.87965789738577,86.0185207063945));
#139454=CARTESIAN_POINT('Ctrl Pts',(4.88529495921571,5.03363711301378,86.0282857077657));
#139455=CARTESIAN_POINT('Ctrl Pts',(4.72902854256956,5.18072209622687,86.038050709137));
#139456=CARTESIAN_POINT('Ctrl Pts',(4.56633782116094,5.32035576494046,86.0478157105083));
#139457=CARTESIAN_POINT('Ctrl Pts',(4.40391827147514,5.45975669326061,86.0575644356456));
#139458=CARTESIAN_POINT('Ctrl Pts',(4.23509584670664,5.59173110452241,86.0673131607829));
#139459=CARTESIAN_POINT('Ctrl Pts',(4.06050196682992,5.71576332084091,86.0770618859202));
#139460=CARTESIAN_POINT('Ctrl Pts',(3.88638727945389,5.83945511681967,86.0867838545872));
#139461=CARTESIAN_POINT('Ctrl Pts',(3.70653279230673,5.95524821136194,86.0965058232541));
#139462=CARTESIAN_POINT('Ctrl Pts',(3.52159880345178,6.06267007431767,86.106227791921));
#139463=CARTESIAN_POINT('Ctrl Pts',(3.33788847449887,6.16938115486333,86.1158854328605));
#139464=CARTESIAN_POINT('Ctrl Pts',(3.14916566698421,6.26783136975615,86.1255430738));
#139465=CARTESIAN_POINT('Ctrl Pts',(2.95611096321559,6.35759660057609,86.1352007147395));
#139466=CARTESIAN_POINT('Ctrl Pts',(2.87125677441394,6.39705150996253,86.1394455804261));
#139467=CARTESIAN_POINT('Ctrl Pts',(2.78556613655165,6.43482907719253,86.1436904461126));
#139468=CARTESIAN_POINT('Ctrl Pts',(2.69909888003785,6.47089574929765,86.1479353117992));
#139469=CARTESIAN_POINT('Ctrl Pts',(2.53915797259907,6.53760928338404,86.1557871588132));
#139470=CARTESIAN_POINT('Ctrl Pts',(2.37662409889162,6.5984380918566,86.1636390058272));
#139471=CARTESIAN_POINT('Ctrl Pts',(2.2119889880388,6.65317452644188,86.1714908528412));
#139472=CARTESIAN_POINT('Ctrl Pts',(2.04740056637242,6.70789543821682,86.1793404731349));
#139473=CARTESIAN_POINT('Ctrl Pts',(1.88071245452038,6.75652729266079,86.1871900934285));
#139474=CARTESIAN_POINT('Ctrl Pts',(1.71243461770912,6.79891125420618,86.1950397137221));
#139475=CARTESIAN_POINT('Ctrl Pts',(1.54417021573067,6.84129183193438,86.202888707324));
#139476=CARTESIAN_POINT('Ctrl Pts',(1.37431671154859,6.87742541732396,86.2107377009259));
#139477=CARTESIAN_POINT('Ctrl Pts',(1.20339716686006,6.90720361805653,86.2185866945278));
#139478=CARTESIAN_POINT('Ctrl Pts',(1.03239109061104,6.93699689462014,86.2264396618453));
#139479=CARTESIAN_POINT('Ctrl Pts',(0.860318271790911,6.96042829215117,
86.2342926291628));
#139480=CARTESIAN_POINT('Ctrl Pts',(0.687710194721222,6.97744088119538,
86.2421455964802));
#139481=CARTESIAN_POINT('Ctrl Pts',(0.515058280999615,6.99445779086558,
86.2500005581876));
#139482=CARTESIAN_POINT('Ctrl Pts',(0.341871219006416,7.00505262109014,
86.2578555198949));
#139483=CARTESIAN_POINT('Ctrl Pts',(0.16868282295875,7.00922054637594,86.2657104816022));
#139484=CARTESIAN_POINT('Ctrl Pts',(-0.00467747704870131,7.01339260867599,
86.2735732400157));
#139485=CARTESIAN_POINT('Ctrl Pts',(-0.178038732489622,7.01112503005644,
86.2814359984291));
#139486=CARTESIAN_POINT('Ctrl Pts',(-0.350869343786947,7.00246508496048,
86.2892987568425));
#139487=CARTESIAN_POINT('Ctrl Pts',(-0.477655400252421,6.99611227350142,
86.2950667635902));
#139488=CARTESIAN_POINT('Ctrl Pts',(-0.60415594756938,6.98632051437324,
86.300834770338));
#139489=CARTESIAN_POINT('Ctrl Pts',(-0.730164208890737,6.97312604149351,
86.3066027770857));
#139490=CARTESIAN_POINT('Ctrl Pts',(-0.913192008898027,6.9539609858209,
86.3149808435267));
#139491=CARTESIAN_POINT('Ctrl Pts',(-1.09558632776169,6.92757283386561,
86.3233589099677));
#139492=CARTESIAN_POINT('Ctrl Pts',(-1.27675602187379,6.89402064278234,
86.3317369764087));
#139493=CARTESIAN_POINT('Ctrl Pts',(-1.4578018343017,6.86049139428867,86.3401093140274));
#139494=CARTESIAN_POINT('Ctrl Pts',(-1.63762436927603,6.81980793286539,
86.3484816516461));
#139495=CARTESIAN_POINT('Ctrl Pts',(-1.81563949333606,6.7720809056551,86.3568539892648));
#139496=CARTESIAN_POINT('Ctrl Pts',(-1.99355899880536,6.72437951441875,
86.3652218297874));
#139497=CARTESIAN_POINT('Ctrl Pts',(-2.16967271229878,6.66964218599931,
86.37358967031));
#139498=CARTESIAN_POINT('Ctrl Pts',(-2.34340810346253,6.60803034368988,
86.3819575108326));
#139499=CARTESIAN_POINT('Ctrl Pts',(-2.51707562581287,6.54644256972139,
86.3903220825025));
#139500=CARTESIAN_POINT('Ctrl Pts',(-2.6883663691981,6.47798574682362,86.3986866541724));
#139501=CARTESIAN_POINT('Ctrl Pts',(-2.85672390664179,6.40287084702802,
86.4070512258423));
#139502=CARTESIAN_POINT('Ctrl Pts',(-3.02504031958242,6.32777429546305,
86.4154137543078));
#139503=CARTESIAN_POINT('Ctrl Pts',(-3.19042465571283,6.2460230445545,86.4237762827733));
#139504=CARTESIAN_POINT('Ctrl Pts',(-3.35234096175784,6.15787598434887,
86.4321388112388));
#139505=CARTESIAN_POINT('Ctrl Pts',(-3.51427018923155,6.06972188973156,
86.4405020070603));
#139506=CARTESIAN_POINT('Ctrl Pts',(-3.67273054213885,5.97517111794213,
86.4488652028818));
#139507=CARTESIAN_POINT('Ctrl Pts',(-3.82721047478691,5.87452862314768,
86.4572283987033));
#139508=CARTESIAN_POINT('Ctrl Pts',(-3.98170094265674,5.77387926473681,
86.465592164878));
#139509=CARTESIAN_POINT('Ctrl Pts',(-4.13221017334873,5.66713753423044,
86.4739559310527));
#139510=CARTESIAN_POINT('Ctrl Pts',(-4.27825529504834,5.55465194165133,
86.4823196972274));
#139511=CARTESIAN_POINT('Ctrl Pts',(-4.42432984798277,5.4421436808047,86.4906851488809));
#139512=CARTESIAN_POINT('Ctrl Pts',(-4.56593823760048,5.3238894504136,86.4990506005345));
#139513=CARTESIAN_POINT('Ctrl Pts',(-4.70263006057313,5.20027855752881,
86.5074160521881));
#139514=CARTESIAN_POINT('Ctrl Pts',(-4.83936766136822,5.07662626759933,
86.5157843054149));
#139515=CARTESIAN_POINT('Ctrl Pts',(-4.97118516849089,4.94761395845391,
86.5241525586418));
#139516=CARTESIAN_POINT('Ctrl Pts',(-5.09766817229645,4.81366863916242,
86.5325208118686));
#139517=CARTESIAN_POINT('Ctrl Pts',(-5.22426844389133,4.67959913345053,
86.5408968236601));
#139518=CARTESIAN_POINT('Ctrl Pts',(-5.34552410293012,4.54058771746286,
86.5492728354515));
#139519=CARTESIAN_POINT('Ctrl Pts',(-5.46105945237866,4.39709633964116,
86.557648847243));
#139520=CARTESIAN_POINT('Ctrl Pts',(-5.57665146179003,4.25353459187493,
86.5660289667341));
#139521=CARTESIAN_POINT('Ctrl Pts',(-5.68651736631053,4.10548876100266,
86.5744090862252));
#139522=CARTESIAN_POINT('Ctrl Pts',(-5.79032377509833,3.95345129501187,
86.5827892057164));
#139523=CARTESIAN_POINT('Ctrl Pts',(-5.89424879585793,3.80124010695673,
86.5911789005556));
#139524=CARTESIAN_POINT('Ctrl Pts',(-5.99210030578251,3.64502844531357,
86.5995685953948));
#139525=CARTESIAN_POINT('Ctrl Pts',(-6.08358930108757,3.48533610691895,
86.607958290234));
#139526=CARTESIAN_POINT('Ctrl Pts',(-6.14167408540737,3.38395019703713,
86.6132847627088));
#139527=CARTESIAN_POINT('Ctrl Pts',(-6.19719521531603,3.28116181133347,
86.6186112351837));
#139528=CARTESIAN_POINT('Ctrl Pts',(-6.25008864931542,3.17710850274248,
86.6239377076585));
#139529=CARTESIAN_POINT('Ctrl Pts',(-6.33331742068157,3.01337874697146,
86.6323190080634));
#139530=CARTESIAN_POINT('Ctrl Pts',(-6.41020567117982,2.84618575687431,
86.6407003084684));
#139531=CARTESIAN_POINT('Ctrl Pts',(-6.48046315699178,2.67604630628324,
86.6490816088733));
#139532=CARTESIAN_POINT('Ctrl Pts',(-6.55063160172563,2.50612248253869,
86.6574522872069));
#139533=CARTESIAN_POINT('Ctrl Pts',(-6.61418590507908,2.33325994057912,
86.6658229655405));
#139534=CARTESIAN_POINT('Ctrl Pts',(-6.67088178962929,2.15799970141156,
86.6741936438741));
#139535=CARTESIAN_POINT('Ctrl Pts',(-6.72751333408461,1.98293835252513,
86.682554822925));
#139536=CARTESIAN_POINT('Ctrl Pts',(-6.7773018721317,1.80548503948199,86.6909160019759));
#139537=CARTESIAN_POINT('Ctrl Pts',(-6.82005113331489,1.62620081830946,
86.6992771810268));
#139538=CARTESIAN_POINT('Ctrl Pts',(-6.8627449222889,1.44714923956262,86.7076275104615));
#139539=CARTESIAN_POINT('Ctrl Pts',(-6.89841757807585,1.26627180872092,
86.7159778398962));
#139540=CARTESIAN_POINT('Ctrl Pts',(-6.92692260572745,1.08414472131816,
86.724328169331));
#139541=CARTESIAN_POINT('Ctrl Pts',(-6.95540570046527,0.902157769815413,
86.7326720736867));
#139542=CARTESIAN_POINT('Ctrl Pts',(-6.97673210713103,0.718923400253159,
86.7410159780424));
#139543=CARTESIAN_POINT('Ctrl Pts',(-6.99080613463922,0.535029111722596,
86.7493598823982));
#139544=CARTESIAN_POINT('Ctrl Pts',(-7.00486885780083,0.351282528230385,
86.7576970848779));
#139545=CARTESIAN_POINT('Ctrl Pts',(-7.01169079431785,0.16687740863043,
86.7660342873576));
#139546=CARTESIAN_POINT('Ctrl Pts',(-7.01122792897929,-0.0175923392648725,
86.7743714898374));
#139547=CARTESIAN_POINT('Ctrl Pts',(-7.0110755562648,-0.0783187620189622,
86.7771160508733));
#139548=CARTESIAN_POINT('Ctrl Pts',(-7.01013415446036,-0.139052146393013,
86.7798606119091));
#139549=CARTESIAN_POINT('Ctrl Pts',(-7.00840338632719,-0.199771211683747,
86.782605172945));
#139550=CARTESIAN_POINT('Ctrl Pts',(-7.00314510219132,-0.384243118488884,
86.7909434832468));
#139551=CARTESIAN_POINT('Ctrl Pts',(-6.99060127451497,-0.568431470742194,
86.7992817935487));
#139552=CARTESIAN_POINT('Ctrl Pts',(-6.97083272321741,-0.751743112653088,
86.8076201038505));
#139553=CARTESIAN_POINT('Ctrl Pts',(-6.951051734218,-0.935170088030384,
86.8159636603343));
#139554=CARTESIAN_POINT('Ctrl Pts',(-6.92403699006115,-1.11771892707604,
86.8243072168182));
#139555=CARTESIAN_POINT('Ctrl Pts',(-6.88990082146536,-1.29880453990238,
86.832650773302));
#139556=CARTESIAN_POINT('Ctrl Pts',(-6.85573868222145,-1.48002792187275,
86.8410006775271));
#139557=CARTESIAN_POINT('Ctrl Pts',(-6.81444437212664,-1.65978553550522,
86.8493505817523));
#139558=CARTESIAN_POINT('Ctrl Pts',(-6.7661807661487,-1.83750493939454,
86.8577004859775));
#139559=CARTESIAN_POINT('Ctrl Pts',(-6.71784476833355,-2.01549090923758,
86.8660629144411));
#139560=CARTESIAN_POINT('Ctrl Pts',(-6.6625186713434,-2.19143224369014,
86.8744253429047));
#139561=CARTESIAN_POINT('Ctrl Pts',(-6.60041491324566,-2.36477261813992,
86.8827877713682));
#139562=CARTESIAN_POINT('Ctrl Pts',(-6.53825804796865,-2.5382612222399,
86.8911573508481));
#139563=CARTESIAN_POINT('Ctrl Pts',(-6.46931207971855,-2.7091441254031,
86.899526930328));
#139564=CARTESIAN_POINT('Ctrl Pts',(-6.3938368012109,-2.87688677601,86.9078965098079));
#139565=CARTESIAN_POINT('Ctrl Pts',(-6.31824511128187,-3.04488814921811,
86.9162789983444));
#139566=CARTESIAN_POINT('Ctrl Pts',(-6.23610413274333,-3.20973929850563,
86.924661486881));
#139567=CARTESIAN_POINT('Ctrl Pts',(-6.14771929897067,-3.37093072957063,
86.9330439754175));
#139568=CARTESIAN_POINT('Ctrl Pts',(-6.11879833308613,-3.42367520709833,
86.9357868630221));
#139569=CARTESIAN_POINT('Ctrl Pts',(-6.08920917596968,-3.47602807320321,
86.9385297506267));
#139570=CARTESIAN_POINT('Ctrl Pts',(-6.05896350698851,-3.5279721914269,
86.9412726382314));
#139571=CARTESIAN_POINT('Ctrl Pts',(-5.96644904131462,-3.68685716584613,
86.9496624933641));
#139572=CARTESIAN_POINT('Ctrl Pts',(-5.86760225278239,-3.8422364254221,
86.9580523484969));
#139573=CARTESIAN_POINT('Ctrl Pts',(-5.7627121365476,-3.99359179108068,
86.9664422036297));
#139574=CARTESIAN_POINT('Ctrl Pts',(-5.65791881144161,-4.1448074881297,
86.9748243167217));
#139575=CARTESIAN_POINT('Ctrl Pts',(-5.54709346211167,-4.29200642462329,
86.9832064298138));
#139576=CARTESIAN_POINT('Ctrl Pts',(-5.43056966892759,-4.43469724258869,
86.9915885429059));
#139577=CARTESIAN_POINT('Ctrl Pts',(-5.31413627351006,-4.57727736272235,
86.9999641532548));
#139578=CARTESIAN_POINT('Ctrl Pts',(-5.19201345511359,-4.71535608326536,
87.0083397636037));
#139579=CARTESIAN_POINT('Ctrl Pts',(-5.06457682105358,-4.84847276842377,
87.0167153739525));
#139580=CARTESIAN_POINT('Ctrl Pts',(-4.93722034652814,-4.98150572121115,
87.0250857159182));
#139581=CARTESIAN_POINT('Ctrl Pts',(-4.80455694766025,-5.10958262515081,
87.0334560578838));
#139582=CARTESIAN_POINT('Ctrl Pts',(-4.66700135664259,-5.2322772192991,
87.0418263998494));
#139583=CARTESIAN_POINT('Ctrl Pts',(-4.52951212603039,-5.35491262237448,
87.0501927037438));
#139584=CARTESIAN_POINT('Ctrl Pts',(-4.38713565461108,-5.47217067520983,
87.0585590076381));
#139585=CARTESIAN_POINT('Ctrl Pts',(-4.24032257778898,-5.58366286578918,
87.0669253115324));
#139586=CARTESIAN_POINT('Ctrl Pts',(-4.0935505604693,-5.69512387512795,
87.075289275606));
#139587=CARTESIAN_POINT('Ctrl Pts',(-3.94234467250425,-5.80082203787116,
87.0836532396797));
#139588=CARTESIAN_POINT('Ctrl Pts',(-3.78718802055007,-5.90040960099399,
87.0920172037533));
#139589=CARTESIAN_POINT('Ctrl Pts',(-3.63205524462613,-5.99998183924587,
87.1003798807519));
#139590=CARTESIAN_POINT('Ctrl Pts',(-3.47297319336365,-6.09344517521102,
87.1087425577504));
#139591=CARTESIAN_POINT('Ctrl Pts',(-3.31045364576688,-6.18049538643374,
87.1171052347489));
#139592=CARTESIAN_POINT('Ctrl Pts',(-3.14793744415068,-6.26754380545165,
87.1254677395753));
#139593=CARTESIAN_POINT('Ctrl Pts',(-2.98198417721644,-6.34817920818278,
87.1338302444016));
#139594=CARTESIAN_POINT('Ctrl Pts',(-2.81313026979528,-6.42214330637845,
87.1421927492279));
#139595=CARTESIAN_POINT('Ctrl Pts',(-2.64425733174381,-6.49611574067621,
87.1505561965479));
#139596=CARTESIAN_POINT('Ctrl Pts',(-2.47248340266744,-6.5634152400237,
87.1589196438678));
#139597=CARTESIAN_POINT('Ctrl Pts',(-2.29836532333784,-6.62383147453029,
87.1672830911878));
#139598=CARTESIAN_POINT('Ctrl Pts',(-2.1241447183896,-6.68428328381374,
87.1756514631406));
#139599=CARTESIAN_POINT('Ctrl Pts',(-1.94757751552329,-6.73784362051997,
87.1840198350934));
#139600=CARTESIAN_POINT('Ctrl Pts',(-1.7692371656464,-6.78435158391688,
87.1923882070462));
#139601=CARTESIAN_POINT('Ctrl Pts',(-1.59084338034021,-6.83087348231499,
87.2007590863819));
#139602=CARTESIAN_POINT('Ctrl Pts',(-1.41067570808094,-6.87033871615273,
87.2091299657177));
#139603=CARTESIAN_POINT('Ctrl Pts',(-1.22931896518779,-6.90263728181697,
87.2175008450534));
#139604=CARTESIAN_POINT('Ctrl Pts',(-1.04780856068732,-6.93496321370668,
87.2258788169447));
#139605=CARTESIAN_POINT('Ctrl Pts',(-0.86510739717758,-6.96011029163013,
87.2342567888359));
#139606=CARTESIAN_POINT('Ctrl Pts',(-0.681807762689802,-6.97802011585206,
87.2426347607272));
#139607=CARTESIAN_POINT('Ctrl Pts',(-0.565319352357486,-6.98940195498542,
87.2479590300862));
#139608=CARTESIAN_POINT('Ctrl Pts',(-0.448589341810954,-6.9978619255989,
87.2532832994453));
#139609=CARTESIAN_POINT('Ctrl Pts',(-0.331770083394625,-7.00339597440159,
87.2586075688043));
#139610=CARTESIAN_POINT('Ctrl Pts',(-0.159252495223688,-7.01156860591117,
87.2664703999936));
#139611=CARTESIAN_POINT('Ctrl Pts',(0.0138185171086572,-7.01337428630968,
87.2743332311829));
#139612=CARTESIAN_POINT('Ctrl Pts',(0.186913749327192,-7.00875807920437,
87.2821960623723));
#139613=CARTESIAN_POINT('Ctrl Pts',(0.359875980707844,-7.00414541904489,
87.2900528520137));
#139614=CARTESIAN_POINT('Ctrl Pts',(0.532862016293961,-6.99312069419043,
87.2979096416551));
#139615=CARTESIAN_POINT('Ctrl Pts',(0.705338861372208,-6.9756808738028,
87.3057664312966));
#139616=CARTESIAN_POINT('Ctrl Pts',(0.877718437672965,-6.95825088864846,
87.3136187900805));
#139617=CARTESIAN_POINT('Ctrl Pts',(1.04958901653653,-6.93441304285145,
87.3214711488644));
#139618=CARTESIAN_POINT('Ctrl Pts',(1.22041919640894,-6.90421636013361,
87.3293235076484));
#139619=CARTESIAN_POINT('Ctrl Pts',(1.39120904128379,-6.87402680720469,
87.3371740123988));
#139620=CARTESIAN_POINT('Ctrl Pts',(1.560958599501,-6.83748146354632,87.3450245171493));
#139621=CARTESIAN_POINT('Ctrl Pts',(1.72914324075803,-6.79468102381862,
87.3528750218997));
#139622=CARTESIAN_POINT('Ctrl Pts',(1.8973008264071,-6.75188746933269,87.3607242637514));
#139623=CARTESIAN_POINT('Ctrl Pts',(2.0638936272454,-6.70284091893024,87.3685735056031));
#139624=CARTESIAN_POINT('Ctrl Pts',(2.22840929069917,-6.64769272722692,
87.3764227474547));
#139625=CARTESIAN_POINT('Ctrl Pts',(2.39298038270055,-6.59252595501821,
87.3842746338697));
#139626=CARTESIAN_POINT('Ctrl Pts',(2.55547257739125,-6.53125355661724,
87.3921265202845));
#139627=CARTESIAN_POINT('Ctrl Pts',(2.71539053087561,-6.46407617740781,
87.3999784066995));
#139628=CARTESIAN_POINT('Ctrl Pts',(2.83281629365509,-6.41474866399658,
87.4057439491632));
#139629=CARTESIAN_POINT('Ctrl Pts',(2.94885442459499,-6.36223834778985,
87.4115094916269));
#139630=CARTESIAN_POINT('Ctrl Pts',(3.06331649494052,-6.30664083441616,
87.4172750340907));
#139631=CARTESIAN_POINT('Ctrl Pts',(3.25500116880469,-6.21353408572183,
87.4269303384503));
#139632=CARTESIAN_POINT('Ctrl Pts',(3.44216773556263,-6.11181628212727,
87.4365856428098));
#139633=CARTESIAN_POINT('Ctrl Pts',(3.62414572569807,-6.00193254888827,
87.4462409471694));
#139634=CARTESIAN_POINT('Ctrl Pts',(3.80713183976366,-5.89144008037898,
87.455949740104));
#139635=CARTESIAN_POINT('Ctrl Pts',(3.98487171838707,-5.77269102740675,
87.4656585330386));
#139636=CARTESIAN_POINT('Ctrl Pts',(4.1567198259205,-5.64617630359693,87.4753673259732));
#139637=CARTESIAN_POINT('Ctrl Pts',(4.32939488113772,-5.51905278019471,
87.4851228384437));
#139638=CARTESIAN_POINT('Ctrl Pts',(4.49612130481291,-5.3840887129702,87.4948783509142));
#139639=CARTESIAN_POINT('Ctrl Pts',(4.65628081749642,-5.24181986633601,
87.5046338633848));
#139640=CARTESIAN_POINT('Ctrl Pts',(4.81659891273631,-5.09941015165712,
87.5143990353134));
#139641=CARTESIAN_POINT('Ctrl Pts',(4.97033706975347,-4.94968122402455,
87.524164207242));
#139642=CARTESIAN_POINT('Ctrl Pts',(5.11691201231409,-4.7932074877618,87.5339293791707));
#139643=CARTESIAN_POINT('Ctrl Pts',(5.26328710326691,-4.63694709988742,
87.543681236509));
#139644=CARTESIAN_POINT('Ctrl Pts',(5.4025184743354,-4.47396031139054,87.5534330938473));
#139645=CARTESIAN_POINT('Ctrl Pts',(5.53406224465387,-4.30485558814656,
87.5631849511856));
#139646=CARTESIAN_POINT('Ctrl Pts',(5.59142485538193,-4.23111368164473,
87.5674374672494));
#139647=CARTESIAN_POINT('Ctrl Pts',(5.6473260762211,-4.15620885909643,87.5716899833132));
#139648=CARTESIAN_POINT('Ctrl Pts',(5.70172304235925,-4.08019373446037,
87.575942499377));
#139649=CARTESIAN_POINT('Ctrl Pts',(5.80447945829518,-3.93660039977533,
87.5839755449759));
#139650=CARTESIAN_POINT('Ctrl Pts',(5.9019152335504,-3.78897284309355,87.5920085905748));
#139651=CARTESIAN_POINT('Ctrl Pts',(5.99369660943177,-3.63775033730822,
87.6000416361736));
#139652=CARTESIAN_POINT('Ctrl Pts',(6.08541898471072,-3.48662504317239,
87.6080695178214));
#139653=CARTESIAN_POINT('Ctrl Pts',(6.17149400650488,-3.33190971203974,
87.6160973994693));
#139654=CARTESIAN_POINT('Ctrl Pts',(6.25163039143314,-3.17407372494868,
87.6241252811171));
#139655=CARTESIAN_POINT('Ctrl Pts',(6.33173059399445,-3.01630900236009,
87.6321495380973));
#139656=CARTESIAN_POINT('Ctrl Pts',(6.40589733296575,-2.85542675548335,
87.6401737950775));
#139657=CARTESIAN_POINT('Ctrl Pts',(6.47388460276936,-2.69192212229958,
87.6481980520578));
#139658=CARTESIAN_POINT('Ctrl Pts',(6.54186365221889,-2.52843725849294,
87.6562213388235));
#139659=CARTESIAN_POINT('Ctrl Pts',(6.60366457293895,-2.36233097525184,
87.6642446255892));
#139660=CARTESIAN_POINT('Ctrl Pts',(6.65908890167848,-2.19411976930214,
87.672267912355));
#139661=CARTESIAN_POINT('Ctrl Pts',(6.71450868888864,-2.02592234676039,
87.6802905416839));
#139662=CARTESIAN_POINT('Ctrl Pts',(6.76355281397507,-1.8556206945594,87.6883131710128));
#139663=CARTESIAN_POINT('Ctrl Pts',(6.80607232949424,-1.68374760822189,
87.6963358003418));
#139664=CARTESIAN_POINT('Ctrl Pts',(6.84860782932424,-1.51180990983968,
87.7043614456082));
#139665=CARTESIAN_POINT('Ctrl Pts',(6.88461373455662,-1.33829995400738,
87.7123870908747));
#139666=CARTESIAN_POINT('Ctrl Pts',(6.91399189574394,-1.16376227301248,
87.7204127361411));
#139667=CARTESIAN_POINT('Ctrl Pts',(6.93131504979576,-1.06084422050252,
87.7251451456486));
#139668=CARTESIAN_POINT('Ctrl Pts',(6.94633470816353,-0.957569012097593,
87.7298775551561));
#139669=CARTESIAN_POINT('Ctrl Pts',(6.95903917973927,-0.854049329578666,
87.7346099646636));
#139670=CARTESIAN_POINT('Ctrl Pts',(6.98457816244076,-0.645950364946275,
87.744123223348));
#139671=CARTESIAN_POINT('Ctrl Pts',(7.00076663816503,-0.436802360049345,
87.7536364820323));
#139672=CARTESIAN_POINT('Ctrl Pts',(7.00756193006239,-0.227381527042749,
87.7631497407167));
#139673=CARTESIAN_POINT('Ctrl Pts',(7.01003449670575,-0.151180684762784,
87.766611279448));
#139674=CARTESIAN_POINT('Ctrl Pts',(7.01126392857062,-0.0749437292124329,
87.7700728181792));
#139675=CARTESIAN_POINT('Ctrl Pts',(7.01124988097084,0.00129193125224031,
87.7735343569104));
#139676=CARTESIAN_POINT('Ctrl Pts',(7.0112498809707,0.00129193205161908,
87.7735343569467));
#139677=CARTESIAN_POINT('Ctrl Pts',(7.0112148332025,0.191494396890641,87.7821706459852));
#139678=CARTESIAN_POINT('Ctrl Pts',(7.00343567581073,0.381684631459496,
87.7908069350237));
#139679=CARTESIAN_POINT('Ctrl Pts',(6.98794117335139,0.571230881763605,
87.7994432240622));
#139680=CARTESIAN_POINT('Ctrl Pts',(6.97244273416072,0.760825290610734,
87.8080817073467));
#139681=CARTESIAN_POINT('Ctrl Pts',(6.94922505512906,0.949775098930185,
87.8167201906312));
#139682=CARTESIAN_POINT('Ctrl Pts',(6.91836885256738,1.13745284839657,87.8253586739157));
#139683=CARTESIAN_POINT('Ctrl Pts',(6.88751073242885,1.3251422612071,87.8339976940438));
#139684=CARTESIAN_POINT('Ctrl Pts',(6.8490131915845,1.51155917165626,87.8426367141719));
#139685=CARTESIAN_POINT('Ctrl Pts',(6.80300829948206,1.69608509211013,87.8512757343));
#139686=CARTESIAN_POINT('Ctrl Pts',(6.75699271969402,1.8806538809402,87.8599167614132));
#139687=CARTESIAN_POINT('Ctrl Pts',(6.70346637489318,2.06333052071484,87.8685577885263));
#139688=CARTESIAN_POINT('Ctrl Pts',(6.64261183550849,2.24350943061592,87.8771988156395));
#139689=CARTESIAN_POINT('Ctrl Pts',(6.61980274129825,2.31104289274028,87.8804375880218));
#139690=CARTESIAN_POINT('Ctrl Pts',(6.59596464646165,2.37822561687374,87.8836763604041));
#139691=CARTESIAN_POINT('Ctrl Pts',(6.57110895151811,2.44502632087643,87.8869151327864));
#139692=CARTESIAN_POINT('',(7.01124965431583,0.00220167122758261,87.2264656430642));
#139693=CARTESIAN_POINT('Ctrl Pts',(6.57110895151811,2.44502632087644,87.3401045918022));
#139694=CARTESIAN_POINT('Ctrl Pts',(6.63540548261139,2.27222674509633,87.3317392734252));
#139695=CARTESIAN_POINT('Ctrl Pts',(6.69282938016015,2.09703047627333,87.3233739550482));
#139696=CARTESIAN_POINT('Ctrl Pts',(6.74323173931865,1.92001361254175,87.3150086366712));
#139697=CARTESIAN_POINT('Ctrl Pts',(6.79372178829562,1.74268877559408,87.3066287643475));
#139698=CARTESIAN_POINT('Ctrl Pts',(6.83716579752875,1.56353732978274,87.2982488920238));
#139699=CARTESIAN_POINT('Ctrl Pts',(6.87346582618015,1.383146448802,87.2898690197001));
#139700=CARTESIAN_POINT('Ctrl Pts',(6.90633433108634,1.21980832547748,87.2822813156454));
#139701=CARTESIAN_POINT('Ctrl Pts',(6.93334632752058,1.05545429802191,87.2746936115906));
#139702=CARTESIAN_POINT('Ctrl Pts',(6.95446591090124,0.890522575015729,
87.2671059075359));
#139703=CARTESIAN_POINT('Ctrl Pts',(6.99217189097095,0.596060693431974,
87.2535591527205));
#139704=CARTESIAN_POINT('Ctrl Pts',(7.01115634495757,0.299346418726003,
87.240012397905));
#139705=CARTESIAN_POINT('Ctrl Pts',(7.01124965431565,0.00220167178242508,
87.2264656430895));
#139706=CARTESIAN_POINT('Ctrl Pts',(7.01124965431583,0.00220167122758728,
87.2264656430642));
#139707=CARTESIAN_POINT('Ctrl Pts',(7.0113066794161,-0.179395476228933,
87.2181866744569));
#139708=CARTESIAN_POINT('Ctrl Pts',(7.00430416044149,-0.361169552020984,
87.2099077058496));
#139709=CARTESIAN_POINT('Ctrl Pts',(6.99022718875038,-0.542540700920188,
87.2016287372423));
#139710=CARTESIAN_POINT('Ctrl Pts',(6.97616290082495,-0.723748429077766,
87.1933572282293));
#139711=CARTESIAN_POINT('Ctrl Pts',(6.95503688927996,-0.904553615145572,
87.1850857192163));
#139712=CARTESIAN_POINT('Ctrl Pts',(6.92688628859189,-1.08437673684824,
87.1768142102033));
#139713=CARTESIAN_POINT('Ctrl Pts',(6.89875615964076,-1.26406908721555,
87.1685487164139));
#139714=CARTESIAN_POINT('Ctrl Pts',(6.8636116756909,-1.44278046049112,87.1602832226244));
#139715=CARTESIAN_POINT('Ctrl Pts',(6.821541788702,-1.61993647637567,87.152017728835));
#139716=CARTESIAN_POINT('Ctrl Pts',(6.77865012864773,-1.80055297320375,
87.1435907808403));
#139717=CARTESIAN_POINT('Ctrl Pts',(6.72855974717477,-1.97955236337847,
87.1351638328456));
#139718=CARTESIAN_POINT('Ctrl Pts',(6.67141989610619,-2.15633557971353,
87.126736884851));
#139719=CARTESIAN_POINT('Ctrl Pts',(6.61542495399234,-2.32957659767665,
87.1184787872827));
#139720=CARTESIAN_POINT('Ctrl Pts',(6.55266047395911,-2.50068907097207,
87.1102206897145));
#139721=CARTESIAN_POINT('Ctrl Pts',(6.48331758590733,-2.66912338470231,
87.1019625921463));
#139722=CARTESIAN_POINT('Ctrl Pts',(6.41398579047937,-2.83753075437914,
87.0937058156071));
#139723=CARTESIAN_POINT('Ctrl Pts',(6.33807781423758,-3.00326050280816,
87.0854490390679));
#139724=CARTESIAN_POINT('Ctrl Pts',(6.2558332555195,-3.1657821848062,87.0771922625288));
#139725=CARTESIAN_POINT('Ctrl Pts',(6.17358889881209,-3.32830346761533,
87.06893550627));
#139726=CARTESIAN_POINT('Ctrl Pts',(6.08500814531612,-3.48761639543208,
87.0606787500113));
#139727=CARTESIAN_POINT('Ctrl Pts',(5.99037707635064,-3.64321410922179,
87.0524219937526));
#139728=CARTESIAN_POINT('Ctrl Pts',(5.89233640169151,-3.80441808802212,
87.0438677423535));
#139729=CARTESIAN_POINT('Ctrl Pts',(5.78780148794633,-3.96163379975225,
87.0353134909543));
#139730=CARTESIAN_POINT('Ctrl Pts',(5.67714016313336,-4.11432936584301,
87.0267592395552));
#139731=CARTESIAN_POINT('Ctrl Pts',(5.57024169369452,-4.26183277168771,
87.0184958613306));
#139732=CARTESIAN_POINT('Ctrl Pts',(5.45762683920251,-4.40511811963978,
87.010232483106));
#139733=CARTESIAN_POINT('Ctrl Pts',(5.33966885850479,-4.54373888378438,
87.0019691048814));
#139734=CARTESIAN_POINT('Ctrl Pts',(5.21548264801218,-4.6896788811706,86.993269416895));
#139735=CARTESIAN_POINT('Ctrl Pts',(5.08537409387772,-4.83044805700159,
86.9845697289086));
#139736=CARTESIAN_POINT('Ctrl Pts',(4.94982358379145,-4.96556875411488,
86.9758700409222));
#139737=CARTESIAN_POINT('Ctrl Pts',(4.81427307370527,-5.10068945122808,
86.9671703529358));
#139738=CARTESIAN_POINT('Ctrl Pts',(4.67328095355334,-5.23016139735379,
86.9584706649493));
#139739=CARTESIAN_POINT('Ctrl Pts',(4.527368704802,-5.35355575045964,86.9497709769629));
#139740=CARTESIAN_POINT('Ctrl Pts',(4.39549232231815,-5.46508032119165,
86.9419081457736));
#139741=CARTESIAN_POINT('Ctrl Pts',(4.25930025509381,-5.57189116622378,
86.9340453145843));
#139742=CARTESIAN_POINT('Ctrl Pts',(4.11917885399775,-5.67362248755395,
86.926182483395));
#139743=CARTESIAN_POINT('Ctrl Pts',(3.97916511770259,-5.77527564179207,
86.9183256937535));
#139744=CARTESIAN_POINT('Ctrl Pts',(3.83522835813542,-5.87185681133976,
86.9104689041121));
#139745=CARTESIAN_POINT('Ctrl Pts',(3.68778953694237,-5.96303906525175,
86.9026121144707));
#139746=CARTESIAN_POINT('Ctrl Pts',(3.54043386426488,-6.05416989668899,
86.8947597556866));
#139747=CARTESIAN_POINT('Ctrl Pts',(3.38958038194236,-6.13990766924507,
86.8869073969027));
#139748=CARTESIAN_POINT('Ctrl Pts',(3.23568048249427,-6.21996771516587,
86.8790550381187));
#139749=CARTESIAN_POINT('Ctrl Pts',(3.08181692060817,-6.30000885797566,
86.8712045333682));
#139750=CARTESIAN_POINT('Ctrl Pts',(2.92490870723316,-6.37437475898989,
86.8633540286177));
#139751=CARTESIAN_POINT('Ctrl Pts',(2.76543332457585,-6.44282586213731,
86.8555035238673));
#139752=CARTESIAN_POINT('Ctrl Pts',(2.60598359648129,-6.51126595365966,
86.8476542820156));
#139753=CARTESIAN_POINT('Ctrl Pts',(2.44396787300339,-6.57379299375918,
86.8398050401639));
#139754=CARTESIAN_POINT('Ctrl Pts',(2.27988474236866,-6.63021508881986,
86.8319557983122));
#139755=CARTESIAN_POINT('Ctrl Pts',(2.11574632891598,-6.6866561935886,86.8241039118973));
#139756=CARTESIAN_POINT('Ctrl Pts',(1.94953947810042,-6.73698812066281,
86.8162520254824));
#139757=CARTESIAN_POINT('Ctrl Pts',(1.78177929760037,-6.78106843330332,
86.8084001390675));
#139758=CARTESIAN_POINT('Ctrl Pts',(1.65859508513453,-6.81343605821695,
86.8026345966039));
#139759=CARTESIAN_POINT('Ctrl Pts',(1.53457370880756,-6.8424339780357,86.7968690541402));
#139760=CARTESIAN_POINT('Ctrl Pts',(1.4099228546989,-6.86802330414638,86.7911035116765));
#139761=CARTESIAN_POINT('Ctrl Pts',(1.20117546576048,-6.91087664076003,
86.7814482073168));
#139762=CARTESIAN_POINT('Ctrl Pts',(0.990769093090478,-6.94414815441042,
86.7717929029572));
#139763=CARTESIAN_POINT('Ctrl Pts',(0.779506623183717,-6.96778271668346,
86.7621375985975));
#139764=CARTESIAN_POINT('Ctrl Pts',(0.567073798822291,-6.99154820999812,
86.7524288056629));
#139765=CARTESIAN_POINT('Ctrl Pts',(0.353775418683256,-7.00556973150932,
86.7427200127282));
#139766=CARTESIAN_POINT('Ctrl Pts',(0.140422469402555,-7.00984365678628,
86.7330112197935));
#139767=CARTESIAN_POINT('Ctrl Pts',(-0.0739571523842897,-7.01413814855455,
86.7232557073229));
#139768=CARTESIAN_POINT('Ctrl Pts',(-0.288391826022229,-7.00859102897364,
86.7135001948524));
#139769=CARTESIAN_POINT('Ctrl Pts',(-0.502064877831008,-6.99325084784956,
86.7037446823818));
#139770=CARTESIAN_POINT('Ctrl Pts',(-0.715949498834876,-6.97789547758606,
86.693979510453));
#139771=CARTESIAN_POINT('Ctrl Pts',(-0.929070952150075,-6.95272766418326,
86.6842143385242));
#139772=CARTESIAN_POINT('Ctrl Pts',(-1.14061680414627,-6.91784792176,86.6744491665954));
#139773=CARTESIAN_POINT('Ctrl Pts',(-1.35187421817187,-6.88301573707434,
86.664697309257));
#139774=CARTESIAN_POINT('Ctrl Pts',(-1.56156028711736,-6.83849809557125,
86.6549454519186));
#139775=CARTESIAN_POINT('Ctrl Pts',(-1.76887308919542,-6.78444651808976,
86.6451935945802));
#139776=CARTESIAN_POINT('Ctrl Pts',(-1.85927648522427,-6.76087611570234,
86.6409410785168));
#139777=CARTESIAN_POINT('Ctrl Pts',(-1.94922867855122,-6.73549340808156,
86.6366885624534));
#139778=CARTESIAN_POINT('Ctrl Pts',(-2.03866363066388,-6.70831403286313,
86.6324360463901));
#139779=CARTESIAN_POINT('Ctrl Pts',(-2.20760715439179,-6.65697191981162,
86.6244030007912));
#139780=CARTESIAN_POINT('Ctrl Pts',(-2.37478632349822,-6.59918999176723,
86.6163699551923));
#139781=CARTESIAN_POINT('Ctrl Pts',(-2.53966891637932,-6.5351134923333,
86.6083369095934));
#139782=CARTESIAN_POINT('Ctrl Pts',(-2.70444551638085,-6.47107818374049,
86.6003090279456));
#139783=CARTESIAN_POINT('Ctrl Pts',(-2.86692813857277,-6.4007564904291,
86.5922811462977));
#139784=CARTESIAN_POINT('Ctrl Pts',(-3.02659992353864,-6.32434340191422,
86.5842532646499));
#139785=CARTESIAN_POINT('Ctrl Pts',(-3.18619961512002,-6.24796481466186,
86.5762290076697));
#139786=CARTESIAN_POINT('Ctrl Pts',(-3.34299066647081,-6.1655004663301,
86.5682047506895));
#139787=CARTESIAN_POINT('Ctrl Pts',(-3.49647645282019,-6.07719334704549,
86.5601804937094));
#139788=CARTESIAN_POINT('Ctrl Pts',(-3.64994368117478,-5.98889690499099,
86.5521572069436));
#139789=CARTESIAN_POINT('Ctrl Pts',(-3.80010611914945,-5.89475927512961,
86.5441339201778));
#139790=CARTESIAN_POINT('Ctrl Pts',(-3.94649185093902,-5.7950693380642,
86.536110633412));
#139791=CARTESIAN_POINT('Ctrl Pts',(-4.0928655877237,-5.69538756969987,
86.528088004083));
#139792=CARTESIAN_POINT('Ctrl Pts',(-4.23546293396804,-5.59015461007032,
86.520065374754));
#139793=CARTESIAN_POINT('Ctrl Pts',(-4.37384132920086,-5.4797024179671,
86.512042745425));
#139794=CARTESIAN_POINT('Ctrl Pts',(-4.51227174485862,-5.36920870370314,
86.5040171001586));
#139795=CARTESIAN_POINT('Ctrl Pts',(-4.64647975633978,-5.25349206860225,
86.4959914548921));
#139796=CARTESIAN_POINT('Ctrl Pts',(-4.776055953328,-5.13292471142722,86.4879658096256));
#139797=CARTESIAN_POINT('Ctrl Pts',(-4.85246197504882,-5.06183085063136,
86.4832334001183));
#139798=CARTESIAN_POINT('Ctrl Pts',(-4.927258172949,-4.98905113101414,86.478500990611));
#139799=CARTESIAN_POINT('Ctrl Pts',(-5.00036666384089,-4.91466782088563,
86.4737685811036));
#139800=CARTESIAN_POINT('Ctrl Pts',(-5.13523256982733,-4.77745020924617,
86.465038532269));
#139801=CARTESIAN_POINT('Ctrl Pts',(-5.26442067180578,-4.6347051536203,
86.4563084834345));
#139802=CARTESIAN_POINT('Ctrl Pts',(-5.38750327558942,-4.48691820941872,
86.4475784345999));
#139803=CARTESIAN_POINT('Ctrl Pts',(-5.51062146886109,-4.33908853243833,
86.4388458614608));
#139804=CARTESIAN_POINT('Ctrl Pts',(-5.62763046476733,-4.18621426739769,
86.4301132883218));
#139805=CARTESIAN_POINT('Ctrl Pts',(-5.73814312435031,-4.02881372701336,
86.4213807151827));
#139806=CARTESIAN_POINT('Ctrl Pts',(-5.85022579267595,-3.86917706069164,
86.4125240819023));
#139807=CARTESIAN_POINT('Ctrl Pts',(-5.95562596969108,-3.70488477014028,
86.4036674486218));
#139808=CARTESIAN_POINT('Ctrl Pts',(-6.05398527447523,-3.53650800351661,
86.3948108153414));
#139809=CARTESIAN_POINT('Ctrl Pts',(-6.15102853819702,-3.37038410701347,
86.3860726832347));
#139810=CARTESIAN_POINT('Ctrl Pts',(-6.24121805230625,-3.20028460721418,
86.3773345511281));
#139811=CARTESIAN_POINT('Ctrl Pts',(-6.32425545766644,-3.02678368382616,
86.3685964190214));
#139812=CARTESIAN_POINT('Ctrl Pts',(-6.40898201636357,-2.8497533912047,
86.3596805351541));
#139813=CARTESIAN_POINT('Ctrl Pts',(-6.48626224072858,-2.66918207420734,
86.3507646512867));
#139814=CARTESIAN_POINT('Ctrl Pts',(-6.55583000629885,-2.48570301746038,
86.3418487674193));
#139815=CARTESIAN_POINT('Ctrl Pts',(-6.62539777186917,-2.30222396071329,
86.332932883552));
#139816=CARTESIAN_POINT('Ctrl Pts',(-6.68725297711821,-2.11583744914202,
86.3240169996846));
#139817=CARTESIAN_POINT('Ctrl Pts',(-6.74118250120147,-1.92719616230293,
86.3151011158173));
#139818=CARTESIAN_POINT('Ctrl Pts',(-6.79405229650787,-1.74226172442209,
86.3063604313211));
#139819=CARTESIAN_POINT('Ctrl Pts',(-6.83931061792881,-1.55514066064912,
86.2976197468249));
#139820=CARTESIAN_POINT('Ctrl Pts',(-6.87680237159808,-1.36646101462248,
86.2888790623286));
#139821=CARTESIAN_POINT('Ctrl Pts',(-6.91428737987824,-1.17781531519754,
86.2801399504267));
#139822=CARTESIAN_POINT('Ctrl Pts',(-6.94400855764818,-0.987611861976894,
86.2714008385248));
#139823=CARTESIAN_POINT('Ctrl Pts',(-6.9658618755798,-0.796489104033331,
86.2626617266229));
#139824=CARTESIAN_POINT('Ctrl Pts',(-6.98799833469756,-0.602890075687711,
86.2538093869486));
#139825=CARTESIAN_POINT('Ctrl Pts',(-7.00206157913031,-0.408348035341609,
86.2449570472742));
#139826=CARTESIAN_POINT('Ctrl Pts',(-7.00799757267361,-0.21353356621558,
86.2361047075999));
#139827=CARTESIAN_POINT('Ctrl Pts',(-7.01385463701136,-0.0213094892736308,
86.2273700749501));
#139828=CARTESIAN_POINT('Ctrl Pts',(-7.0117992450298,0.171179535380497,
86.2186354423004));
#139829=CARTESIAN_POINT('Ctrl Pts',(-7.0018318541426,0.363286730853184,
86.2099008096506));
#139830=CARTESIAN_POINT('Ctrl Pts',(-6.9916629839309,0.559277151977933,
86.200989616464));
#139831=CARTESIAN_POINT('Ctrl Pts',(-6.97325883762919,0.7548698519352,86.1920784232773));
#139832=CARTESIAN_POINT('Ctrl Pts',(-6.94667580252165,0.949379722324112,
86.1831672300907));
#139833=CARTESIAN_POINT('Ctrl Pts',(-6.92009276741413,1.14388959271289,
86.1742560369041));
#139834=CARTESIAN_POINT('Ctrl Pts',(-6.88533087119709,1.3373163313709,86.1653448437175));
#139835=CARTESIAN_POINT('Ctrl Pts',(-6.84250272341944,1.52898104713482,
86.1564336505308));
#139836=CARTESIAN_POINT('Ctrl Pts',(-6.80393051954978,1.70159954395731,
86.1484079856783));
#139837=CARTESIAN_POINT('Ctrl Pts',(-6.75879730526788,1.87286802781756,
86.1403823208259));
#139838=CARTESIAN_POINT('Ctrl Pts',(-6.70722394941671,2.04224715812532,
86.1323566559734));
#139839=CARTESIAN_POINT('Ctrl Pts',(-6.65566696168361,2.21157253165193,
86.12433353827));
#139840=CARTESIAN_POINT('Ctrl Pts',(-6.59767400832791,2.37900939518393,
86.1163104205667));
#139841=CARTESIAN_POINT('Ctrl Pts',(-6.5334163010369,2.54403183939299,86.1082873028634));
#139842=CARTESIAN_POINT('Ctrl Pts',(-6.46916669720532,2.70903347282719,
86.1002651969454));
#139843=CARTESIAN_POINT('Ctrl Pts',(-6.39865404663154,2.87162095215027,
86.0922430910274));
#139844=CARTESIAN_POINT('Ctrl Pts',(-6.32209833132043,3.03128673200268,
86.0842209851095));
#139845=CARTESIAN_POINT('Ctrl Pts',(-6.24551416764698,3.19101184419805,
86.0761958981499));
#139846=CARTESIAN_POINT('Ctrl Pts',(-6.16288260911893,3.34781275586464,
86.0681708111903));
#139847=CARTESIAN_POINT('Ctrl Pts',(-6.07447059243358,3.50120459044592,
86.0601457242307));
#139848=CARTESIAN_POINT('Ctrl Pts',(-5.98604116344338,3.65462663478246,
86.0521190567703));
#139849=CARTESIAN_POINT('Ctrl Pts',(-5.89182919903346,3.80463795130602,
86.0440923893099));
#139850=CARTESIAN_POINT('Ctrl Pts',(-5.792145793958,3.95078139917089,86.0360657218495));
#139851=CARTESIAN_POINT('Ctrl Pts',(-5.69238236339647,4.09704217048035,
86.0280326106088));
#139852=CARTESIAN_POINT('Ctrl Pts',(-5.5871389335373,4.23942857391079,86.0199994993681));
#139853=CARTESIAN_POINT('Ctrl Pts',(-5.47676819494788,4.37751490018107,
86.0119663881273));
#139854=CARTESIAN_POINT('Ctrl Pts',(-5.41173374634506,4.45888037986663,
86.0072329871663));
#139855=CARTESIAN_POINT('Ctrl Pts',(-5.34491985472404,4.53875351225276,
86.0024995862054));
#139856=CARTESIAN_POINT('Ctrl Pts',(-5.27640478678675,4.61705307403694,
85.9977661852444));
#139857=CARTESIAN_POINT('Ctrl Pts',(-5.13526161449251,4.77835260817125,
85.9880152319506));
#139858=CARTESIAN_POINT('Ctrl Pts',(-4.98681445037594,4.9330678946744,85.9782642786568));
#139859=CARTESIAN_POINT('Ctrl Pts',(-4.83164907455954,5.08062927035696,
85.968513325363));
#139860=CARTESIAN_POINT('Ctrl Pts',(-4.67626015391105,5.22840323588296,
85.9587483239918));
#139861=CARTESIAN_POINT('Ctrl Pts',(-4.51413368902129,5.36900264783073,
85.9489833226206));
#139862=CARTESIAN_POINT('Ctrl Pts',(-4.34589168472511,5.50189531226623,
85.9392183212493));
#139863=CARTESIAN_POINT('Ctrl Pts',(-4.1779301049904,5.63456647216544,85.9294695961121));
#139864=CARTESIAN_POINT('Ctrl Pts',(-4.00387338793853,5.75955653409464,
85.9197208709749));
#139865=CARTESIAN_POINT('Ctrl Pts',(-3.82437342948381,5.87637596094381,
85.9099721458376));
#139866=CARTESIAN_POINT('Ctrl Pts',(-3.64536612881235,5.99287476376404,
85.9002501771707));
#139867=CARTESIAN_POINT('Ctrl Pts',(-3.46094544465128,6.10124767801816,
85.8905282085038));
#139868=CARTESIAN_POINT('Ctrl Pts',(-3.27179036996444,6.20104945452848,
85.8808062398369));
#139869=CARTESIAN_POINT('Ctrl Pts',(-3.08388688500338,6.30019086874981,
85.8711485988975));
#139870=CARTESIAN_POINT('Ctrl Pts',(-2.89131148268681,6.39087414896381,
85.8614909579581));
#139871=CARTESIAN_POINT('Ctrl Pts',(-2.69476145194911,6.47270324359067,
85.8518333170187));
#139872=CARTESIAN_POINT('Ctrl Pts',(-2.60837094659956,6.50866994789785,
85.8475884513318));
#139873=CARTESIAN_POINT('Ctrl Pts',(-2.52121299164009,6.5429266390945,85.8433435856449));
#139874=CARTESIAN_POINT('Ctrl Pts',(-2.43334873421181,6.57544222849002,
85.839098719958));
#139875=CARTESIAN_POINT('Ctrl Pts',(-2.27082375504642,6.63558722537196,
85.831246872944));
#139876=CARTESIAN_POINT('Ctrl Pts',(-2.10594760139136,6.68974678591728,
85.82339502593));
#139877=CARTESIAN_POINT('Ctrl Pts',(-1.93922005044005,6.73773345855053,
85.815543178916));
#139878=CARTESIAN_POINT('Ctrl Pts',(-1.77253978207427,6.78570652255137,
85.8076935586224));
#139879=CARTESIAN_POINT('Ctrl Pts',(-1.6040095270302,6.82751007544145,85.7998439383287));
#139880=CARTESIAN_POINT('Ctrl Pts',(-1.43414529570062,6.86300618048096,
85.7919943180351));
#139881=CARTESIAN_POINT('Ctrl Pts',(-1.26429462585716,6.89849945161051,
85.7841453244332));
#139882=CARTESIAN_POINT('Ctrl Pts',(-1.09311056529415,6.92768620006259,
85.7762963308313));
#139883=CARTESIAN_POINT('Ctrl Pts',(-0.921120155835015,6.95047942382498,
85.7684473372294));
#139884=CARTESIAN_POINT('Ctrl Pts',(-0.749042672667633,6.97328418712916,
85.7605943699119));
#139885=CARTESIAN_POINT('Ctrl Pts',(-0.576158403589205,6.98968890816532,
85.7527414025944));
#139886=CARTESIAN_POINT('Ctrl Pts',(-0.403000710362994,6.99965834808721,
85.7448884352769));
#139887=CARTESIAN_POINT('Ctrl Pts',(-0.229799040901227,7.00963031991184,
85.7370334735696));
#139888=CARTESIAN_POINT('Ctrl Pts',(-0.0563241903801478,7.01316374685525,
85.7291785118623));
#139889=CARTESIAN_POINT('Ctrl Pts',(0.116890273279048,7.01027554569097,
85.7213235501549));
#139890=CARTESIAN_POINT('Ctrl Pts',(0.290276666772179,7.00738447774561,
85.7134607917415));
#139891=CARTESIAN_POINT('Ctrl Pts',(0.463401776455177,6.99805907169471,
85.7055980333281));
#139892=CARTESIAN_POINT('Ctrl Pts',(0.635736368850849,6.98236821084511,
85.6977352749147));
#139893=CARTESIAN_POINT('Ctrl Pts',(0.762158552967875,6.97085762047723,
85.691967268167));
#139894=CARTESIAN_POINT('Ctrl Pts',(0.888155422128745,6.95592256172243,
85.6861992614192));
#139895=CARTESIAN_POINT('Ctrl Pts',(1.01352184654572,6.93760765891778,85.6804312546715));
#139896=CARTESIAN_POINT('Ctrl Pts',(1.19561737437222,6.91100514625288,85.6720531882305));
#139897=CARTESIAN_POINT('Ctrl Pts',(1.37678580379833,6.87721132586099,85.6636751217895));
#139898=CARTESIAN_POINT('Ctrl Pts',(1.55643888652997,6.83630927877004,85.6552970553485));
#139899=CARTESIAN_POINT('Ctrl Pts',(1.73596912461776,6.79543520001302,85.6469247177298));
#139900=CARTESIAN_POINT('Ctrl Pts',(1.9139857623391,6.7474626577391,85.6385523801111));
#139901=CARTESIAN_POINT('Ctrl Pts',(2.08990965660681,6.69252599469899,85.6301800424924));
#139902=CARTESIAN_POINT('Ctrl Pts',(2.26573905556112,6.63761884019842,85.6218122019698));
#139903=CARTESIAN_POINT('Ctrl Pts',(2.43947763931337,6.57575512128039,85.6134443614473));
#139904=CARTESIAN_POINT('Ctrl Pts',(2.61055992599161,6.50711944221917,85.6050765209247));
#139905=CARTESIAN_POINT('Ctrl Pts',(2.78157538027929,6.438510575323,85.5967119492548));
#139906=CARTESIAN_POINT('Ctrl Pts',(2.94993630212426,6.36313514586129,85.5883473775849));
#139907=CARTESIAN_POINT('Ctrl Pts',(3.1150953174239,6.28122660997545,85.579982805915));
#139908=CARTESIAN_POINT('Ctrl Pts',(3.28021398952197,6.1993380817929,85.5716202774493));
#139909=CARTESIAN_POINT('Ctrl Pts',(3.4421320208119,6.11091977595752,85.5632577489837));
#139910=CARTESIAN_POINT('Ctrl Pts',(3.60032444525188,6.01625219313667,85.554895220518));
#139911=CARTESIAN_POINT('Ctrl Pts',(3.75852949394097,5.92157705554729,85.5465320246965));
#139912=CARTESIAN_POINT('Ctrl Pts',(3.91300805665764,5.82065180820689,85.5381688288749));
#139913=CARTESIAN_POINT('Ctrl Pts',(4.06326143054369,5.71380198375443,85.5298056330534));
#139914=CARTESIAN_POINT('Ctrl Pts',(4.21352505140834,5.60694487235836,85.5214418668787));
#139915=CARTESIAN_POINT('Ctrl Pts',(4.35956264076882,5.49416256856521,85.513078100704));
#139916=CARTESIAN_POINT('Ctrl Pts',(4.50090591956449,5.37582295706707,85.5047143345293));
#139917=CARTESIAN_POINT('Ctrl Pts',(4.64227768207256,5.25745949759054,85.4963488828757));
#139918=CARTESIAN_POINT('Ctrl Pts',(4.77895299557398,5.1335367083427,85.4879834312221));
#139919=CARTESIAN_POINT('Ctrl Pts',(4.91049768391965,5.00446191500343,85.4796179795685));
#139920=CARTESIAN_POINT('Ctrl Pts',(5.04208642632258,4.87534389476987,85.4712497263417));
#139921=CARTESIAN_POINT('Ctrl Pts',(5.16854088277385,4.74107066013652,85.4628814731148));
#139922=CARTESIAN_POINT('Ctrl Pts',(5.28946437627248,4.60208574177453,85.4545132198879));
#139923=CARTESIAN_POINT('Ctrl Pts',(5.41049998310104,4.46297196456503,85.4461372080964));
#139924=CARTESIAN_POINT('Ctrl Pts',(5.52599416368788,4.31913802255369,85.4377611963049));
#139925=CARTESIAN_POINT('Ctrl Pts',(5.63559034434976,4.17106078032577,85.4293851845135));
#139926=CARTESIAN_POINT('Ctrl Pts',(5.74524027233294,4.02291091918843,85.4210050650223));
#139927=CARTESIAN_POINT('Ctrl Pts',(5.84898624206912,3.8705138759804,85.4126249455312));
#139928=CARTESIAN_POINT('Ctrl Pts',(5.94651519299266,3.71437526671814,85.40424482604));
#139929=CARTESIAN_POINT('Ctrl Pts',(6.04415558309692,3.55805824931626,85.3958551312008));
#139930=CARTESIAN_POINT('Ctrl Pts',(6.13556459098704,3.39799140545263,85.3874654363616));
#139931=CARTESIAN_POINT('Ctrl Pts',(6.22047462004968,3.23470586975352,85.3790757415223));
#139932=CARTESIAN_POINT('Ctrl Pts',(6.27438253223083,3.13103870091498,85.3737492690477));
#139933=CARTESIAN_POINT('Ctrl Pts',(6.32567180420869,3.02607461810293,85.3684227965732));
#139934=CARTESIAN_POINT('Ctrl Pts',(6.37428404911103,2.91995366808254,85.3630963240986));
#139935=CARTESIAN_POINT('Ctrl Pts',(6.44560045119588,2.76426934705427,85.3552821436703));
#139936=CARTESIAN_POINT('Ctrl Pts',(6.51127951872477,2.60582038596922,85.347467963242));
#139937=CARTESIAN_POINT('Ctrl Pts',(6.57110895151817,2.44502632087629,85.3396537828137));
#139938=CARTESIAN_POINT('Origin',(0.,0.,50.));
#139939=CARTESIAN_POINT('',(6.57110895151814,2.44502632087636,83.3399710686702));
#139940=CARTESIAN_POINT('',(6.57110895151815,2.44502632087632,83.8871228390383));
#139941=CARTESIAN_POINT('',(6.57110895151814,2.44502632087636,50.));
#139942=CARTESIAN_POINT('',(7.0112498931807,-0.00122387650377896,85.7735343569104));
#139943=CARTESIAN_POINT('Ctrl Pts',(6.57110895151815,2.44502632087633,83.8871228390383));
#139944=CARTESIAN_POINT('Ctrl Pts',(6.49738773721382,2.64315512100245,83.8967308308781));
#139945=CARTESIAN_POINT('Ctrl Pts',(6.41463613204344,2.83812450534434,83.9063388227179));
#139946=CARTESIAN_POINT('Ctrl Pts',(6.32310674446419,3.02918267204397,83.9159468145576));
#139947=CARTESIAN_POINT('Ctrl Pts',(6.28930719915407,3.09973574065968,83.9194948089682));
#139948=CARTESIAN_POINT('Ctrl Pts',(6.25431117822531,3.1697555530712,83.9230428033786));
#139949=CARTESIAN_POINT('Ctrl Pts',(6.21813317189162,3.23920459667509,83.9265907977892));
#139950=CARTESIAN_POINT('Ctrl Pts',(6.13806986340311,3.39289798019116,83.9344426448032));
#139951=CARTESIAN_POINT('Ctrl Pts',(6.0522454551493,3.54373423243355,83.9422944918172));
#139952=CARTESIAN_POINT('Ctrl Pts',(5.96090446899515,3.69123888064884,83.9501463388312));
#139953=CARTESIAN_POINT('Ctrl Pts',(5.86958938640614,3.83870169773852,83.9579959591249));
#139954=CARTESIAN_POINT('Ctrl Pts',(5.77276103852171,3.98283446620419,83.9658455794185));
#139955=CARTESIAN_POINT('Ctrl Pts',(5.67070922211792,4.12318850899238,83.9736951997122));
#139956=CARTESIAN_POINT('Ctrl Pts',(5.56866555324701,4.26353134630457,83.9815441933141));
#139957=CARTESIAN_POINT('Ctrl Pts',(5.46139947098157,4.40009575041923,83.9893931869159));
#139958=CARTESIAN_POINT('Ctrl Pts',(5.3492431453722,4.53246338475984,83.9972421805178));
#139959=CARTESIAN_POINT('Ctrl Pts',(5.23703003829871,4.66489803295845,84.0050951478353));
#139960=CARTESIAN_POINT('Ctrl Pts',(5.1199219880559,4.79313137470459,84.0129481151528));
#139961=CARTESIAN_POINT('Ctrl Pts',(4.99829060256407,4.91677919117991,84.0208010824703));
#139962=CARTESIAN_POINT('Ctrl Pts',(4.87662832678725,5.04045841004593,84.0286560441777));
#139963=CARTESIAN_POINT('Ctrl Pts',(4.75044070458944,5.1595495216934,84.036511005885));
#139964=CARTESIAN_POINT('Ctrl Pts',(4.62013451441192,5.27370682075139,84.0443659675924));
#139965=CARTESIAN_POINT('Ctrl Pts',(4.48969898444844,5.38797743047103,84.0522287260058));
#139966=CARTESIAN_POINT('Ctrl Pts',(4.35513701761826,5.49730420616521,84.0600914844192));
#139967=CARTESIAN_POINT('Ctrl Pts',(4.21688707094716,5.60138286438078,84.0679542428327));
#139968=CARTESIAN_POINT('Ctrl Pts',(4.11546889384688,5.67773347460112,84.0737222495804));
#139969=CARTESIAN_POINT('Ctrl Pts',(4.01206669415905,5.75126069485251,84.0794902563281));
#139970=CARTESIAN_POINT('Ctrl Pts',(3.90686245212008,5.82185986972499,84.0852582630758));
#139971=CARTESIAN_POINT('Ctrl Pts',(3.7540526222726,5.92440561969238,84.0936363295168));
#139972=CARTESIAN_POINT('Ctrl Pts',(3.59710154621307,6.02099952136874,84.1020143959579));
#139973=CARTESIAN_POINT('Ctrl Pts',(3.43650094856868,6.11130818998573,84.1103924623988));
#139974=CARTESIAN_POINT('Ctrl Pts',(3.27601016770459,6.20155510660821,84.1187648000176));
#139975=CARTESIAN_POINT('Ctrl Pts',(3.11187512616021,6.2855251980408,84.1271371376363));
#139976=CARTESIAN_POINT('Ctrl Pts',(2.94461521837978,6.36292918223881,84.135509475255));
#139977=CARTESIAN_POINT('Ctrl Pts',(2.77744515216083,6.4402915898576,84.1438773157776));
#139978=CARTESIAN_POINT('Ctrl Pts',(2.60715386410196,6.5110947848003,84.1522451563002));
#139979=CARTESIAN_POINT('Ctrl Pts',(2.43428437052244,6.57509590545493,84.1606129968227));
#139980=CARTESIAN_POINT('Ctrl Pts',(2.26148240749738,6.63907202440986,84.1689775684926));
#139981=CARTESIAN_POINT('Ctrl Pts',(2.08610455518692,6.69625125394156,84.1773421401625));
#139982=CARTESIAN_POINT('Ctrl Pts',(1.90871321004522,6.74643909364777,84.1857067118324));
#139983=CARTESIAN_POINT('Ctrl Pts',(1.73136519608381,6.79661467402796,84.1940692402979));
#139984=CARTESIAN_POINT('Ctrl Pts',(1.55200498623576,6.83980218131971,84.2024317687635));
#139985=CARTESIAN_POINT('Ctrl Pts',(1.37120995673436,6.87585702418634,84.2107942972291));
#139986=CARTESIAN_POINT('Ctrl Pts',(1.19040049922412,6.91191474434219,84.2191574930506));
#139987=CARTESIAN_POINT('Ctrl Pts',(1.00815631444084,6.94083859267037,84.227520688872));
#139988=CARTESIAN_POINT('Ctrl Pts',(0.825065550168112,6.9625349837847,84.2358838846935));
#139989=CARTESIAN_POINT('Ctrl Pts',(0.641962299472255,6.98423285454941,
84.2442476508682));
#139990=CARTESIAN_POINT('Ctrl Pts',(0.458012680673799,6.99870224634197,
84.2526114170429));
#139991=CARTESIAN_POINT('Ctrl Pts',(0.273810730407882,7.00590138714595,
84.2609751832175));
#139992=CARTESIAN_POINT('Ctrl Pts',(0.0895716594854847,7.01310197873171,
84.2693406348711));
#139993=CARTESIAN_POINT('Ctrl Pts',(-0.0949195157654676,7.01302938503284,
84.2777060865246));
#139994=CARTESIAN_POINT('Ctrl Pts',(-0.279067550917249,7.0056939602387,
84.2860715381781));
#139995=CARTESIAN_POINT('Ctrl Pts',(-0.463277256884167,6.99835607882522,
84.294439791405));
#139996=CARTESIAN_POINT('Ctrl Pts',(-0.647143265211987,6.98375052930749,
84.3028080446318));
#139997=CARTESIAN_POINT('Ctrl Pts',(-0.830073813264486,6.96193967418798,
84.3111762978587));
#139998=CARTESIAN_POINT('Ctrl Pts',(-1.01317396403281,6.94010859729412,
84.3195523096501));
#139999=CARTESIAN_POINT('Ctrl Pts',(-1.19533659458277,6.91105890443951,
84.3279283214416));
#140000=CARTESIAN_POINT('Ctrl Pts',(-1.37597728165275,6.87490458718341,
84.336304333233));
#140001=CARTESIAN_POINT('Ctrl Pts',(-1.55670655714751,6.83873253940344,
84.3446844527241));
#140002=CARTESIAN_POINT('Ctrl Pts',(-1.7359120798368,6.7954489899599,84.3530645722152));
#140003=CARTESIAN_POINT('Ctrl Pts',(-1.913022369512,6.74521845281876,84.3614446917064));
#140004=CARTESIAN_POINT('Ctrl Pts',(-2.09033503012848,6.69493052092602,
84.3698343865455));
#140005=CARTESIAN_POINT('Ctrl Pts',(-2.26554735930746,6.63767983593957,
84.3782240813847));
#140006=CARTESIAN_POINT('Ctrl Pts',(-2.43810443617646,6.57368034823695,
84.3866137762239));
#140007=CARTESIAN_POINT('Ctrl Pts',(-2.54765794651259,6.53304817791536,
84.3919402486987));
#140008=CARTESIAN_POINT('Ctrl Pts',(-2.65614157544202,6.4896967032441,84.3972667211736));
#140009=CARTESIAN_POINT('Ctrl Pts',(-2.76341802457471,6.44369050963465,
84.4025931936484));
#140010=CARTESIAN_POINT('Ctrl Pts',(-2.9322194500587,6.37129893510777,84.4109744940533));
#140011=CARTESIAN_POINT('Ctrl Pts',(-3.09837133545325,6.29218604120235,
84.4193557944583));
#140012=CARTESIAN_POINT('Ctrl Pts',(-3.26131974452749,6.20656266273492,
84.4277370948632));
#140013=CARTESIAN_POINT('Ctrl Pts',(-3.42406164034726,6.12104779936529,
84.4361077731968));
#140014=CARTESIAN_POINT('Ctrl Pts',(-3.58360786318481,6.02903904616464,
84.4444784515304));
#140015=CARTESIAN_POINT('Ctrl Pts',(-3.73942423594185,5.9307953046915,84.452849129864));
#140016=CARTESIAN_POINT('Ctrl Pts',(-3.89506378386816,5.83266305299731,
84.4612103089149));
#140017=CARTESIAN_POINT('Ctrl Pts',(-4.04698164255542,5.7283100892508,84.4695714879657));
#140018=CARTESIAN_POINT('Ctrl Pts',(-4.19466765943043,5.61804145494036,
84.4779326670166));
#140019=CARTESIAN_POINT('Ctrl Pts',(-4.34216203627732,5.50791590719037,
84.4862829964514));
#140020=CARTESIAN_POINT('Ctrl Pts',(-4.48543526301602,5.39189019513191,
84.4946333258861));
#140021=CARTESIAN_POINT('Ctrl Pts',(-4.6240057059312,5.2703128743952,84.5029836553209));
#140022=CARTESIAN_POINT('Ctrl Pts',(-4.76246952717969,5.14882910013415,
84.5113275596767));
#140023=CARTESIAN_POINT('Ctrl Pts',(-4.89623753039063,5.02180244494933,
84.5196714640324));
#140024=CARTESIAN_POINT('Ctrl Pts',(-5.02485984788077,4.8896226921569,84.5280153683882));
#140025=CARTESIAN_POINT('Ctrl Pts',(-5.15337885512325,4.75754910696635,
84.5363525708679));
#140026=CARTESIAN_POINT('Ctrl Pts',(-5.27676019157693,4.62033091295654,
84.5446897733477));
#140027=CARTESIAN_POINT('Ctrl Pts',(-5.39458956112217,4.47839592148034,
84.5530269758274));
#140028=CARTESIAN_POINT('Ctrl Pts',(-5.43337833917123,4.431671705752,84.5557715368633));
#140029=CARTESIAN_POINT('Ctrl Pts',(-5.47156574979735,4.38443663525802,
84.5585160978992));
#140030=CARTESIAN_POINT('Ctrl Pts',(-5.50913790009451,4.33670683355957,
84.5612606589351));
#140031=CARTESIAN_POINT('Ctrl Pts',(-5.62328666333559,4.19169788968678,
84.5695989692369));
#140032=CARTESIAN_POINT('Ctrl Pts',(-5.73165981888591,4.04223901281819,
84.5779372795388));
#140033=CARTESIAN_POINT('Ctrl Pts',(-5.8339240463015,3.88882460191832,84.5862755898406));
#140034=CARTESIAN_POINT('Ctrl Pts',(-5.93625261489894,3.73531366787678,
84.5946191463244));
#140035=CARTESIAN_POINT('Ctrl Pts',(-6.03246440722958,3.57784250843815,
84.6029627028082));
#140036=CARTESIAN_POINT('Ctrl Pts',(-6.12227082116504,3.41693233102605,
84.6113062592919));
#140037=CARTESIAN_POINT('Ctrl Pts',(-6.21214555942866,3.25589973385256,
84.6196561635171));
#140038=CARTESIAN_POINT('Ctrl Pts',(-6.29560503938557,3.09142318564503,
84.6280060677423));
#140039=CARTESIAN_POINT('Ctrl Pts',(-6.3724075710268,2.92404656447539,84.6363559719674));
#140040=CARTESIAN_POINT('Ctrl Pts',(-6.44932530078216,2.75641889075973,
84.644718400431));
#140041=CARTESIAN_POINT('Ctrl Pts',(-6.51956599242606,2.58588274967877,
84.6530808288946));
#140042=CARTESIAN_POINT('Ctrl Pts',(-6.58293633678099,2.41300139833954,
84.6614432573583));
#140043=CARTESIAN_POINT('Ctrl Pts',(-6.646360871419,2.23997220987769,84.6698128368382));
#140044=CARTESIAN_POINT('Ctrl Pts',(-6.70290323615627,2.06459412081998,
84.6781824163181));
#140045=CARTESIAN_POINT('Ctrl Pts',(-6.7524204307408,1.88744400950446,84.686551995798));
#140046=CARTESIAN_POINT('Ctrl Pts',(-6.80201399956481,1.71002066572614,
84.6949344843345));
#140047=CARTESIAN_POINT('Ctrl Pts',(-6.84456067019608,1.53082015625442,
84.703316972871));
#140048=CARTESIAN_POINT('Ctrl Pts',(-6.87996853946176,1.35042936080212,
84.7116994614076));
#140049=CARTESIAN_POINT('Ctrl Pts',(-6.89155457447877,1.29140253664688,
84.7144423490122));
#140050=CARTESIAN_POINT('Ctrl Pts',(-6.90237666812842,1.23224830520737,
84.7171852366167));
#140051=CARTESIAN_POINT('Ctrl Pts',(-6.91243280912772,1.17298730674917,
84.7199281242213));
#140052=CARTESIAN_POINT('Ctrl Pts',(-6.94319220518818,0.991721697740565,
84.7283179793541));
#140053=CARTESIAN_POINT('Ctrl Pts',(-6.96684353899479,0.809090878000783,
84.7367078344869));
#140054=CARTESIAN_POINT('Ctrl Pts',(-6.98327672178235,0.62567786401048,
84.7450976896197));
#140055=CARTESIAN_POINT('Ctrl Pts',(-6.99969474025922,0.442434100978206,
84.7534798027118));
#140056=CARTESIAN_POINT('Ctrl Pts',(-7.00890785683715,0.258409908432713,
84.7618619158039));
#140057=CARTESIAN_POINT('Ctrl Pts',(-7.01085739945249,0.0741962737761583,
84.7702440288959));
#140058=CARTESIAN_POINT('Ctrl Pts',(-7.01280542963595,-0.109874450142781,
84.7786196392448));
#140059=CARTESIAN_POINT('Ctrl Pts',(-7.00750111685177,-0.294133995636706,
84.7869952495937));
#140060=CARTESIAN_POINT('Ctrl Pts',(-6.99493774077816,-0.477988038696947,
84.7953708599425));
#140061=CARTESIAN_POINT('Ctrl Pts',(-6.98238226725466,-0.661726434833925,
84.8037412019081));
#140062=CARTESIAN_POINT('Ctrl Pts',(-6.96257685710609,-0.845059510001265,
84.8121115438737));
#140063=CARTESIAN_POINT('Ctrl Pts',(-6.93556685367154,-1.02739426743224,
84.8204818858393));
#140064=CARTESIAN_POINT('Ctrl Pts',(-6.90856988056705,-1.20964106182103,
84.8288481897336));
#140065=CARTESIAN_POINT('Ctrl Pts',(-6.87437529333649,-1.39089017429523,
84.8372144936279));
#140066=CARTESIAN_POINT('Ctrl Pts',(-6.83308018701985,-1.5705545900276,
84.8455807975222));
#140067=CARTESIAN_POINT('Ctrl Pts',(-6.79179662978701,-1.75016875865863,
84.8539447615958));
#140068=CARTESIAN_POINT('Ctrl Pts',(-6.74341658530487,-1.92819879392908,
84.8623087256695));
#140069=CARTESIAN_POINT('Ctrl Pts',(-6.6880881936738,-2.10406817288346,
84.8706726897431));
#140070=CARTESIAN_POINT('Ctrl Pts',(-6.63276831616276,-2.279910488463,84.8790353667416));
#140071=CARTESIAN_POINT('Ctrl Pts',(-6.57050232194515,-2.45359249722489,
84.8873980437401));
#140072=CARTESIAN_POINT('Ctrl Pts',(-6.50148825500511,-2.62455272999623,
84.8957607207387));
#140073=CARTESIAN_POINT('Ctrl Pts',(-6.43247560893857,-2.79550944300883,
84.904123225565));
#140074=CARTESIAN_POINT('Ctrl Pts',(-6.35671529057448,-2.96374418716424,
84.9124857303913));
#140075=CARTESIAN_POINT('Ctrl Pts',(-6.27445369610728,-3.12871497230183,
84.9208482352176));
#140076=CARTESIAN_POINT('Ctrl Pts',(-6.19218283037093,-3.29370435042393,
84.9292116825376));
#140077=CARTESIAN_POINT('Ctrl Pts',(-6.10340937482096,-3.45542874225314,
84.9375751298576));
#140078=CARTESIAN_POINT('Ctrl Pts',(-6.00842612691498,-3.61336990078589,
84.9459385771775));
#140079=CARTESIAN_POINT('Ctrl Pts',(-5.9133869502033,-3.77140405951145,
84.9543069491303));
#140080=CARTESIAN_POINT('Ctrl Pts',(-5.81213084331041,-3.92565025107858,
84.9626753210831));
#140081=CARTESIAN_POINT('Ctrl Pts',(-5.70499502510914,-4.07561753921783,
84.9710436930359));
#140082=CARTESIAN_POINT('Ctrl Pts',(-5.59782710621671,-4.22562976147604,
84.9794145723717));
#140083=CARTESIAN_POINT('Ctrl Pts',(-5.48477615858953,-4.37136025948501,
84.9877854517074));
#140084=CARTESIAN_POINT('Ctrl Pts',(-5.36622073602579,-4.5123498949823,
84.9961563310432));
#140085=CARTESIAN_POINT('Ctrl Pts',(-5.24756486273458,-4.6534589894731,
85.0045343029345));
#140086=CARTESIAN_POINT('Ctrl Pts',(-5.12339541104173,-4.78981894672686,
85.0129122748258));
#140087=CARTESIAN_POINT('Ctrl Pts',(-4.99412973283502,-4.92100546373536,
85.021290246717));
#140088=CARTESIAN_POINT('Ctrl Pts',(-4.91198034171884,-5.00437556355154,
85.0266145160761));
#140089=CARTESIAN_POINT('Ctrl Pts',(-4.8277734846779,-5.08565699865557,
85.0319387854352));
#140090=CARTESIAN_POINT('Ctrl Pts',(-4.74162354313436,-5.1647490488594,
85.0372630547943));
#140091=CARTESIAN_POINT('Ctrl Pts',(-4.6143981152607,-5.28155144881807,
85.0451258859836));
#140092=CARTESIAN_POINT('Ctrl Pts',(-4.4826686277116,-5.3938197787296,85.0529887171729));
#140093=CARTESIAN_POINT('Ctrl Pts',(-4.34680621465642,-5.50117281083992,
85.0608515483622));
#140094=CARTESIAN_POINT('Ctrl Pts',(-4.2110481939321,-5.60844335631544,
85.0687083380035));
#140095=CARTESIAN_POINT('Ctrl Pts',(-4.07116386007433,-5.71080587976405,
85.0765651276449));
#140096=CARTESIAN_POINT('Ctrl Pts',(-3.92756051208471,-5.80791657880973,
85.0844219172863));
#140097=CARTESIAN_POINT('Ctrl Pts',(-3.78403814958545,-5.90497251201818,
85.0922742760703));
#140098=CARTESIAN_POINT('Ctrl Pts',(-3.63680125991,-5.99678229956863,85.1001266348543));
#140099=CARTESIAN_POINT('Ctrl Pts',(-3.48628926875464,-6.08304312799657,
85.1079789936382));
#140100=CARTESIAN_POINT('Ctrl Pts',(-3.33581281523649,-6.16928358923646,
85.1158294983887));
#140101=CARTESIAN_POINT('Ctrl Pts',(-3.18206312559944,-6.24997750223117,
85.1236800031391));
#140102=CARTESIAN_POINT('Ctrl Pts',(-3.02550753064711,-6.32486606534064,
85.1315305078896));
#140103=CARTESIAN_POINT('Ctrl Pts',(-2.86897712055583,-6.39974258124058,
85.1393797497412));
#140104=CARTESIAN_POINT('Ctrl Pts',(-2.70964204919406,-6.46881544444646,
85.1472289915928));
#140105=CARTESIAN_POINT('Ctrl Pts',(-2.5479926768134,-6.53187261674669,
85.1550782334445));
#140106=CARTESIAN_POINT('Ctrl Pts',(-2.3862888415952,-6.59495103424251,
85.1629301198593));
#140107=CARTESIAN_POINT('Ctrl Pts',(-2.22226950364215,-6.65200957364057,
85.1707820062742));
#140108=CARTESIAN_POINT('Ctrl Pts',(-2.05644354296371,-6.70288493986753,
85.1786338926891));
#140109=CARTESIAN_POINT('Ctrl Pts',(-1.93467960403323,-6.74024208805458,
85.184399435153));
#140110=CARTESIAN_POINT('Ctrl Pts',(-1.81194197276745,-6.77426641776551,
85.1901649776169));
#140111=CARTESIAN_POINT('Ctrl Pts',(-1.6884365793264,-6.80491061514349,
85.1959305200808));
#140112=CARTESIAN_POINT('Ctrl Pts',(-1.4816074437768,-6.85622912583124,
85.2055858244408));
#140113=CARTESIAN_POINT('Ctrl Pts',(-1.27273050458853,-6.89804131974567,
85.2152411288009));
#140114=CARTESIAN_POINT('Ctrl Pts',(-1.06260573728889,-6.93025941863512,
85.2248964331609));
#140115=CARTESIAN_POINT('Ctrl Pts',(-0.851316918197482,-6.96265599974835,
85.2346052260958));
#140116=CARTESIAN_POINT('Ctrl Pts',(-0.638766462157638,-6.9853519393606,
85.2443140190308));
#140117=CARTESIAN_POINT('Ctrl Pts',(-0.425764535490945,-6.99831059062244,
85.2540228119657));
#140118=CARTESIAN_POINT('Ctrl Pts',(-0.211737625466373,-7.01133160001452,
85.2637783244366));
#140119=CARTESIAN_POINT('Ctrl Pts',(0.0027450660271163,-7.01452140358428,
85.2735338369075));
#140120=CARTESIAN_POINT('Ctrl Pts',(0.216865565674253,-7.00789525384939,
85.2832893493784));
#140121=CARTESIAN_POINT('Ctrl Pts',(0.431198077557214,-7.00126254320687,
85.2930545213075));
#140122=CARTESIAN_POINT('Ctrl Pts',(0.645167642284201,-6.98479445078955,
85.3028196932365));
#140123=CARTESIAN_POINT('Ctrl Pts',(0.857958406954577,-6.95855832298875,
85.3125848651656));
#140124=CARTESIAN_POINT('Ctrl Pts',(1.0704590362451,-6.93235796755296,85.3223367225043));
#140125=CARTESIAN_POINT('Ctrl Pts',(1.28178404017231,-6.89641620030262,
85.332088579843));
#140126=CARTESIAN_POINT('Ctrl Pts',(1.49112599183645,-6.85085176010763,
85.3418404371818));
#140127=CARTESIAN_POINT('Ctrl Pts',(1.58241424400673,-6.83098236425337,
85.3460929532436));
#140128=CARTESIAN_POINT('Ctrl Pts',(1.67332546939955,-6.8092837923712,85.3503454693054));
#140129=CARTESIAN_POINT('Ctrl Pts',(1.7637930474779,-6.7857689798702,85.3545979853672));
#140130=CARTESIAN_POINT('Ctrl Pts',(1.93468721209517,-6.74134926262067,
85.3626310309659));
#140131=CARTESIAN_POINT('Ctrl Pts',(2.10408073117386,-6.69042322326595,
85.3706640765646));
#140132=CARTESIAN_POINT('Ctrl Pts',(2.27143590990466,-6.63311431152031,
85.3786971221633));
#140133=CARTESIAN_POINT('Ctrl Pts',(2.43868350628287,-6.57584224014972,
85.386725003811));
#140134=CARTESIAN_POINT('Ctrl Pts',(2.60389502519156,-6.51219558208228,
85.3947528854587));
#140135=CARTESIAN_POINT('Ctrl Pts',(2.76654609548661,-6.44234811726655,
85.4027807671064));
#140136=CARTESIAN_POINT('Ctrl Pts',(2.92912372722047,-6.37253218926953,
85.4108050240864));
#140137=CARTESIAN_POINT('Ctrl Pts',(3.08914287607793,-6.29652117344199,
85.4188292810664));
#140138=CARTESIAN_POINT('Ctrl Pts',(3.24609743406952,-6.21453763453302,
85.4268535380464));
#140139=CARTESIAN_POINT('Ctrl Pts',(3.40303301465615,-6.13256400826907,
85.434876824812));
#140140=CARTESIAN_POINT('Ctrl Pts',(3.55690441413499,-6.04461946008426,
85.4429001115776));
#140141=CARTESIAN_POINT('Ctrl Pts',(3.70722834420979,-5.95097341334907,
85.4509233983432));
#140142=CARTESIAN_POINT('Ctrl Pts',(3.85753995657948,-5.85733504007206,
85.458946027672));
#140143=CARTESIAN_POINT('Ctrl Pts',(4.00430436948424,-5.75799629611166,
85.4669686570008));
#140144=CARTESIAN_POINT('Ctrl Pts',(4.14706587135866,-5.65327084271683,
85.4749912863297));
#140145=CARTESIAN_POINT('Ctrl Pts',(4.28988104139407,-5.54850602000731,
85.483016931596));
#140146=CARTESIAN_POINT('Ctrl Pts',(4.42869000029797,-5.438350661938,85.4910425768622));
#140147=CARTESIAN_POINT('Ctrl Pts',(4.56306852048824,-5.32315998630788,
85.4990682221285));
#140148=CARTESIAN_POINT('Ctrl Pts',(4.64230628462617,-5.25523654457371,
85.5038006316368));
#140149=CARTESIAN_POINT('Ctrl Pts',(4.7200042127329,-5.18556308635372,85.5085330411452));
#140150=CARTESIAN_POINT('Ctrl Pts',(4.79608113605184,-5.11421864011578,
85.5132654506535));
#140151=CARTESIAN_POINT('Ctrl Pts',(4.93642301783713,-4.98260693181908,
85.5219954994883));
#140152=CARTESIAN_POINT('Ctrl Pts',(5.07131689687424,-4.84524115005751,
85.5307255483232));
#140153=CARTESIAN_POINT('Ctrl Pts',(5.20031566070795,-4.70258903068253,
85.539455597158));
#140154=CARTESIAN_POINT('Ctrl Pts',(5.32935172469491,-4.55989566326953,
85.5481881702973));
#140155=CARTESIAN_POINT('Ctrl Pts',(5.45248908730617,-4.41191311035823,
85.5569207434366));
#140156=CARTESIAN_POINT('Ctrl Pts',(5.56931982371442,-4.25914348944499,
85.565653316576));
#140157=CARTESIAN_POINT('Ctrl Pts',(5.68781032722699,-4.10420353220479,
85.5745099498563));
#140158=CARTESIAN_POINT('Ctrl Pts',(5.7998134713801,-3.94433968467133,85.5833665831367));
#140159=CARTESIAN_POINT('Ctrl Pts',(5.90494791393622,-3.7801080270543,85.592223216417));
#140160=CARTESIAN_POINT('Ctrl Pts',(6.00867566453458,-3.61807377826315,
85.6009613485239));
#140161=CARTESIAN_POINT('Ctrl Pts',(6.10571724735984,-3.45178812195945,
85.6096994806309));
#140162=CARTESIAN_POINT('Ctrl Pts',(6.1957511687176,-3.28181261162706,85.6184376127378));
#140163=CARTESIAN_POINT('Ctrl Pts',(6.28761656707702,-3.10837944629839,
85.6273534966048));
#140164=CARTESIAN_POINT('Ctrl Pts',(6.37218600734555,-2.93110496034485,
85.6362693804719));
#140165=CARTESIAN_POINT('Ctrl Pts',(6.44916779686221,-2.75061107581852,
85.6451852643389));
#140166=CARTESIAN_POINT('Ctrl Pts',(6.52614958637886,-2.57011719129218,
85.654101148206));
#140167=CARTESIAN_POINT('Ctrl Pts',(6.59554361209846,-2.38640418874775,
85.663017032073));
#140168=CARTESIAN_POINT('Ctrl Pts',(6.6571103512007,-2.20011552752043,85.6719329159401));
#140169=CARTESIAN_POINT('Ctrl Pts',(6.71682758852012,-2.01942308945004,
85.6805809613062));
#140170=CARTESIAN_POINT('Ctrl Pts',(6.76919104950747,-1.83627650196859,
85.6892290066724));
#140171=CARTESIAN_POINT('Ctrl Pts',(6.81402159556653,-1.65128321545791,
85.6978770520385));
#140172=CARTESIAN_POINT('Ctrl Pts',(6.85884212225513,-1.46633127388795,
85.706523164616));
#140173=CARTESIAN_POINT('Ctrl Pts',(6.89613302745462,-1.27953373814732,
85.7151692771935));
#140174=CARTESIAN_POINT('Ctrl Pts',(6.92576572928662,-1.09151070793603,
85.723815389771));
#140175=CARTESIAN_POINT('Ctrl Pts',(6.95539404940833,-0.903515480199485,
85.7324602238704));
#140176=CARTESIAN_POINT('Ctrl Pts',(6.97736638061632,-0.714295404980135,
85.7411050579698));
#140177=CARTESIAN_POINT('Ctrl Pts',(6.99160555274235,-0.524479129577489,
85.7497498920692));
#140178=CARTESIAN_POINT('Ctrl Pts',(7.00466426059438,-0.350399115367159,
85.7576780470163));
#140179=CARTESIAN_POINT('Ctrl Pts',(7.01121941622546,-0.175817921304171,
85.7656062019633));
#140180=CARTESIAN_POINT('Ctrl Pts',(7.0112498931807,-0.00122387650377896,
85.7735343569104));
#140181=CARTESIAN_POINT('Ctrl Pts',(7.0112498931807,-0.00122387650377896,
85.7735343569104));
#140182=CARTESIAN_POINT('Ctrl Pts',(7.01128645483302,0.208227714535148,
85.783045360963));
#140183=CARTESIAN_POINT('Ctrl Pts',(7.00193253296366,0.417672943101291,
85.7925563650157));
#140184=CARTESIAN_POINT('Ctrl Pts',(6.98321925767691,0.626318897775227,
85.8020673690684));
#140185=CARTESIAN_POINT('Ctrl Pts',(6.96450598239016,0.834964852449163,
85.8115783731211));
#140186=CARTESIAN_POINT('Ctrl Pts',(6.936433353249,1.04281133667788,85.8210893771738));
#140187=CARTESIAN_POINT('Ctrl Pts',(6.89909079732583,1.24906874620818,85.8306003812265));
#140188=CARTESIAN_POINT('Ctrl Pts',(6.86758001900332,1.42311498777922,85.8386260541597));
#140189=CARTESIAN_POINT('Ctrl Pts',(6.82945868340738,1.59607951497589,85.8466517270929));
#140190=CARTESIAN_POINT('Ctrl Pts',(6.78482559613212,1.76741851087129,85.8546774000261));
#140191=CARTESIAN_POINT('Ctrl Pts',(6.7402070079453,1.93870184717851,85.862700465814));
#140192=CARTESIAN_POINT('Ctrl Pts',(6.68908097230586,2.10836034930558,85.8707235316019));
#140193=CARTESIAN_POINT('Ctrl Pts',(6.6315971395063,2.27586158230061,85.8787465973898));
#140194=CARTESIAN_POINT('Ctrl Pts',(6.6121586370834,2.3325031276681,85.8814596451489));
#140195=CARTESIAN_POINT('Ctrl Pts',(6.59199354854759,2.38889810609303,85.8841726929079));
#140196=CARTESIAN_POINT('Ctrl Pts',(6.57110895151818,2.44502632087624,85.8868857406669));
#140197=CARTESIAN_POINT('',(7.0112496259069,0.00229035375375721,85.2264656431173));
#140198=CARTESIAN_POINT('Ctrl Pts',(6.57110895151817,2.44502632087629,85.3396537828137));
#140199=CARTESIAN_POINT('Ctrl Pts',(6.63643246135932,2.26946669740855,85.3311220340025));
#140200=CARTESIAN_POINT('Ctrl Pts',(6.69478191749844,2.09111139416079,85.3225902851913));
#140201=CARTESIAN_POINT('Ctrl Pts',(6.7459248106977,1.91053003402543,85.3140585363801));
#140202=CARTESIAN_POINT('Ctrl Pts',(6.79696816595605,1.73030013419337,85.305543392666));
#140203=CARTESIAN_POINT('Ctrl Pts',(6.8408328570105,1.54785311280165,85.297028248952));
#140204=CARTESIAN_POINT('Ctrl Pts',(6.87733538502663,1.36377584828323,85.2885131052379));
#140205=CARTESIAN_POINT('Ctrl Pts',(6.91379513375401,1.17991431387664,85.2800079408818));
#140206=CARTESIAN_POINT('Ctrl Pts',(6.94290985966027,0.994426642296124,
85.2715027765256));
#140207=CARTESIAN_POINT('Ctrl Pts',(6.96454604335369,0.807913963554614,
85.2629976121695));
#140208=CARTESIAN_POINT('Ctrl Pts',(6.9861498619863,0.621680284763982,85.2545051704896));
#140209=CARTESIAN_POINT('Ctrl Pts',(7.00029741943712,0.434424959180303,
85.2460127288098));
#140210=CARTESIAN_POINT('Ctrl Pts',(7.00690637091511,0.246758326565235,
85.2375202871299));
#140211=CARTESIAN_POINT('Ctrl Pts',(7.00977400343826,0.165329533966482,
85.2338354057923));
#140212=CARTESIAN_POINT('Ctrl Pts',(7.01122299162676,0.083823429776159,
85.2301505244548));
#140213=CARTESIAN_POINT('Ctrl Pts',(7.0112496259069,0.00229035375353233,
85.2264656431173));
#140214=CARTESIAN_POINT('Ctrl Pts',(7.01124962590711,0.00229035313782153,
85.2264656430894));
#140215=CARTESIAN_POINT('Ctrl Pts',(7.0113027197677,-0.160241050471218,
85.2191200483304));
#140216=CARTESIAN_POINT('Ctrl Pts',(7.00570090552392,-0.322819188341104,
85.2117744535713));
#140217=CARTESIAN_POINT('Ctrl Pts',(6.99445468411541,-0.485005396213237,
85.2044288588122));
#140218=CARTESIAN_POINT('Ctrl Pts',(6.98168859955592,-0.669110151834753,
85.1960905485098));
#140219=CARTESIAN_POINT('Ctrl Pts',(6.96165456191588,-0.852634902371005,
85.1877522382073));
#140220=CARTESIAN_POINT('Ctrl Pts',(6.93443749546681,-1.03498946079852,
85.1794139279049));
#140221=CARTESIAN_POINT('Ctrl Pts',(6.90720330496308,-1.21745875052638,
85.1710703714206));
#140222=CARTESIAN_POINT('Ctrl Pts',(6.87277711967582,-1.39875605555216,
85.1627268149362));
#140223=CARTESIAN_POINT('Ctrl Pts',(6.83129500348328,-1.57830134571454,
85.1543832584519));
#140224=CARTESIAN_POINT('Ctrl Pts',(6.78978132787762,-1.75798323315082,
85.1460333542262));
#140225=CARTESIAN_POINT('Ctrl Pts',(6.74120108739037,-1.93591012809273,
85.1376834500005));
#140226=CARTESIAN_POINT('Ctrl Pts',(6.68574033314417,-2.1115166966589,85.1293335457747));
#140227=CARTESIAN_POINT('Ctrl Pts',(6.63019639187041,-2.28738666208392,
85.1209711173105));
#140228=CARTESIAN_POINT('Ctrl Pts',(6.56775141247074,-2.46092903365332,
85.1126086888463));
#140229=CARTESIAN_POINT('Ctrl Pts',(6.49864031173796,-2.63159659924433,
85.1042462603821));
#140230=CARTESIAN_POINT('Ctrl Pts',(6.42947011159252,-2.80241010887009,
85.0958766809016));
#140231=CARTESIAN_POINT('Ctrl Pts',(6.35362255080235,-2.97034360957441,
85.087507101421));
#140232=CARTESIAN_POINT('Ctrl Pts',(6.27137897487613,-3.13487357256742,
85.0791375219405));
#140233=CARTESIAN_POINT('Ctrl Pts',(6.18900854825477,-3.29965730298169,
85.0707550334034));
#140234=CARTESIAN_POINT('Ctrl Pts',(6.10022255077677,-3.46102671902273,
85.0623725448662));
#140235=CARTESIAN_POINT('Ctrl Pts',(6.00534691035419,-3.61848518703606,
85.0539900563291));
#140236=CARTESIAN_POINT('Ctrl Pts',(5.97430204621783,-3.67000817781451,
85.051247168728));
#140237=CARTESIAN_POINT('Ctrl Pts',(5.94260549252674,-3.72111267157982,
85.0485042811269));
#140238=CARTESIAN_POINT('Ctrl Pts',(5.9102696167998,-3.77178202170184,85.0457613935259));
#140239=CARTESIAN_POINT('Ctrl Pts',(5.81136169478708,-3.92676777723307,
85.0373715383932));
#140240=CARTESIAN_POINT('Ctrl Pts',(5.70626946418409,-4.07799285774473,
85.0289816832605));
#140241=CARTESIAN_POINT('Ctrl Pts',(5.59530278198467,-4.22495128260843,
85.0205918281278));
#140242=CARTESIAN_POINT('Ctrl Pts',(5.48443849828378,-4.3717740962981,85.0122097150358));
#140243=CARTESIAN_POINT('Ctrl Pts',(5.36771076660022,-4.51433784209083,
85.0038276019438));
#140244=CARTESIAN_POINT('Ctrl Pts',(5.24547289993513,-4.65216515383387,
84.9954454888518));
#140245=CARTESIAN_POINT('Ctrl Pts',(5.12332986394706,-4.78988554079461,
84.987069878503));
#140246=CARTESIAN_POINT('Ctrl Pts',(4.99568543275772,-4.92287657442269,
84.9786942681542));
#140247=CARTESIAN_POINT('Ctrl Pts',(4.86293366036747,-5.05069329670344,
84.9703186578054));
#140248=CARTESIAN_POINT('Ctrl Pts',(4.73026539081347,-5.17842962036775,
84.9619483158399));
#140249=CARTESIAN_POINT('Ctrl Pts',(4.59249642187637,-5.30099789488781,
84.9535779738744));
#140250=CARTESIAN_POINT('Ctrl Pts',(4.45005850014875,-5.41798910184894,
84.9452076319089));
#140251=CARTESIAN_POINT('Ctrl Pts',(4.30768929418927,-5.53492386920076,
84.9368413280147));
#140252=CARTESIAN_POINT('Ctrl Pts',(4.16065588070923,-5.64628672606212,
84.9284750241205));
#140253=CARTESIAN_POINT('Ctrl Pts',(4.00942434249912,-5.75170783370257,
84.9201087202262));
#140254=CARTESIAN_POINT('Ctrl Pts',(3.85823509951156,-5.85709945801394,
84.9117447561527));
#140255=CARTESIAN_POINT('Ctrl Pts',(3.70285034147758,-5.95655245762958,
84.9033807920791));
#140256=CARTESIAN_POINT('Ctrl Pts',(3.54376693569539,-6.04973904131179,
84.8950168280056));
#140257=CARTESIAN_POINT('Ctrl Pts',(3.38470801020584,-6.14291128512727,
84.8866541510071));
#140258=CARTESIAN_POINT('Ctrl Pts',(3.22195185526411,-6.22981886955667,
84.8782914740087));
#140259=CARTESIAN_POINT('Ctrl Pts',(3.05602221405779,-6.31017866543296,
84.8699287970103));
#140260=CARTESIAN_POINT('Ctrl Pts',(2.89009598903941,-6.39053680684799,
84.861566292184));
#140261=CARTESIAN_POINT('Ctrl Pts',(2.72099670399854,-6.46434728562765,
84.8532037873578));
#140262=CARTESIAN_POINT('Ctrl Pts',(2.54927085694879,-6.53137387234964,
84.8448412825316));
#140263=CARTESIAN_POINT('Ctrl Pts',(2.37752565558749,-6.59840801328356,
84.8364778352117));
#140264=CARTESIAN_POINT('Ctrl Pts',(2.20315360836471,-6.65865661882262,
84.8281143878918));
#140265=CARTESIAN_POINT('Ctrl Pts',(2.02671965931391,-6.71193220950946,
84.8197509405719));
#140266=CARTESIAN_POINT('Ctrl Pts',(1.85018182099553,-6.76523917036132,
84.8113825686192));
#140267=CARTESIAN_POINT('Ctrl Pts',(1.67157996945443,-6.81156481575794,
84.8030141966665));
#140268=CARTESIAN_POINT('Ctrl Pts',(1.49149363220141,-6.85077173080542,
84.7946458247138));
#140269=CARTESIAN_POINT('Ctrl Pts',(1.31135333637552,-6.88999039326925,
84.7862749453782));
#140270=CARTESIAN_POINT('Ctrl Pts',(1.12972799025958,-6.92208600756016,
84.7779040660425));
#140271=CARTESIAN_POINT('Ctrl Pts',(0.947206404689178,-6.94697247651204,
84.7695331867069));
#140272=CARTESIAN_POINT('Ctrl Pts',(0.764530170552582,-6.97188003150002,
84.7611552148157));
#140273=CARTESIAN_POINT('Ctrl Pts',(0.580956506222909,-6.98956619670947,
84.7527772429245));
#140274=CARTESIAN_POINT('Ctrl Pts',(0.397079586609618,-6.99999674031338,
84.7443992710333));
#140275=CARTESIAN_POINT('Ctrl Pts',(0.280224306853785,-7.00662543571139,
84.7390750016732));
#140276=CARTESIAN_POINT('Ctrl Pts',(0.163246613162165,-7.01032484772495,
84.7337507323131));
#140277=CARTESIAN_POINT('Ctrl Pts',(0.046298896562297,-7.01109713059783,
84.728426462953));
#140278=CARTESIAN_POINT('Ctrl Pts',(-0.126408397416104,-7.01223763072078,
84.7205636317637));
#140279=CARTESIAN_POINT('Ctrl Pts',(-0.299409378148772,-7.00699392432741,
84.7127008005744));
#140280=CARTESIAN_POINT('Ctrl Pts',(-0.47217304318999,-6.99533267113043,
84.7048379693851));
#140281=CARTESIAN_POINT('Ctrl Pts',(-0.644803962158934,-6.98368037806727,
84.6969811797436));
#140282=CARTESIAN_POINT('Ctrl Pts',(-0.817197550110116,-6.96562036978883,
84.6891243901022));
#140283=CARTESIAN_POINT('Ctrl Pts',(-0.98882113102915,-6.94117132286261,
84.6812676004608));
#140284=CARTESIAN_POINT('Ctrl Pts',(-1.16034792437314,-6.91673606404144,
84.6734152416769));
#140285=CARTESIAN_POINT('Ctrl Pts',(-1.33110519821854,-6.88591898759914,
84.6655628828929));
#140286=CARTESIAN_POINT('Ctrl Pts',(-1.50056398818207,-6.84879071660619,
84.6577105241089));
#140287=CARTESIAN_POINT('Ctrl Pts',(-1.66998276694762,-6.81167121203132,
84.6498600193585));
#140288=CARTESIAN_POINT('Ctrl Pts',(-1.83810329812025,-6.76824355199597,
84.6420095146081));
#140289=CARTESIAN_POINT('Ctrl Pts',(-2.00440548712252,-6.71862971190504,
84.6341590098576));
#140290=CARTESIAN_POINT('Ctrl Pts',(-2.17068092334406,-6.66902385311726,
84.626309768006));
#140291=CARTESIAN_POINT('Ctrl Pts',(-2.33513823495855,-6.61323390730317,
84.6184605261543));
#140292=CARTESIAN_POINT('Ctrl Pts',(-2.49727165793425,-6.55143196782034,
84.6106112843027));
#140293=CARTESIAN_POINT('Ctrl Pts',(-2.65945970683386,-6.48960920605435,
84.6027593978878));
#140294=CARTESIAN_POINT('Ctrl Pts',(-2.81932194635356,-6.42177054070239,
84.5949075114729));
#140295=CARTESIAN_POINT('Ctrl Pts',(-2.97637161427554,-6.34813662236682,
84.587055625058));
#140296=CARTESIAN_POINT('Ctrl Pts',(-3.0916912306694,-6.29406815263753,
84.5812900825942));
#140297=CARTESIAN_POINT('Ctrl Pts',(-3.20549475450005,-6.23687602814215,
84.5755245401304));
#140298=CARTESIAN_POINT('Ctrl Pts',(-3.31759780661831,-6.17666344849882,
84.5697589976666));
#140299=CARTESIAN_POINT('Ctrl Pts',(-3.50533193478754,-6.07582804811887,
84.5601036933068));
#140300=CARTESIAN_POINT('Ctrl Pts',(-3.68820103973235,-5.96657272449971,
84.5504483889469));
#140301=CARTESIAN_POINT('Ctrl Pts',(-3.86555333472027,-5.84936953687601,
84.5407930845871));
#140302=CARTESIAN_POINT('Ctrl Pts',(-4.04388812814646,-5.73151706558328,
84.5310842916527));
#140303=CARTESIAN_POINT('Ctrl Pts',(-4.21664480893165,-5.60562849867982,
84.5213754987183));
#140304=CARTESIAN_POINT('Ctrl Pts',(-4.38319836814722,-5.47222063041793,
84.5116667057838));
#140305=CARTESIAN_POINT('Ctrl Pts',(-4.55055339723575,-5.33817079216313,
84.5019111933132));
#140306=CARTESIAN_POINT('Ctrl Pts',(-4.71164544245118,-5.19652915717362,
84.4921556808426));
#140307=CARTESIAN_POINT('Ctrl Pts',(-4.86587855489121,-5.04785622334371,
84.482400168372));
#140308=CARTESIAN_POINT('Ctrl Pts',(-5.02026438184013,-4.89903608043713,
84.4726349964432));
#140309=CARTESIAN_POINT('Ctrl Pts',(-5.16777767181834,-4.7431707476206,
84.4628698245144));
#140310=CARTESIAN_POINT('Ctrl Pts',(-5.30785902361878,-4.58085790522787,
84.4531046525857));
#140311=CARTESIAN_POINT('Ctrl Pts',(-5.44774937767532,-4.41876637271192,
84.4433527952472));
#140312=CARTESIAN_POINT('Ctrl Pts',(-5.58022802157599,-4.25024492948965,
84.4336009379087));
#140313=CARTESIAN_POINT('Ctrl Pts',(-5.70477630387564,-4.07592368491352,
84.4238490805702));
#140314=CARTESIAN_POINT('Ctrl Pts',(-5.75908837518318,-3.99990699732036,
84.4195965645068));
#140315=CARTESIAN_POINT('Ctrl Pts',(-5.81189291195392,-3.92278786981612,
84.4153440484434));
#140316=CARTESIAN_POINT('Ctrl Pts',(-5.86314922750574,-3.84462061827937,
84.4110915323801));
#140317=CARTESIAN_POINT('Ctrl Pts',(-5.95997292291812,-3.6969618942268,
84.4030584867812));
#140318=CARTESIAN_POINT('Ctrl Pts',(-6.05131610743977,-3.54548896452306,
84.3950254411823));
#140319=CARTESIAN_POINT('Ctrl Pts',(-6.13686318753471,-3.39065432917916,
84.3869923955834));
#140320=CARTESIAN_POINT('Ctrl Pts',(-6.22235527467286,-3.23591922750024,
84.3789645139355));
#140321=CARTESIAN_POINT('Ctrl Pts',(-6.3020584974621,-3.07782704128684,
84.3709366322877));
#140322=CARTESIAN_POINT('Ctrl Pts',(-6.37570092852467,-2.91685862401826,
84.3629087506398));
#140323=CARTESIAN_POINT('Ctrl Pts',(-6.44931010930364,-2.75596288557692,
84.3548844936596));
#140324=CARTESIAN_POINT('Ctrl Pts',(-6.51686379487021,-2.59219383448413,
84.3468602366794));
#140325=CARTESIAN_POINT('Ctrl Pts',(-6.57813634697964,-2.42605621596975,
84.3388359796993));
#140326=CARTESIAN_POINT('Ctrl Pts',(-6.63940149061342,-2.25993868518564,
84.3308126929335));
#140327=CARTESIAN_POINT('Ctrl Pts',(-6.69438687948976,-2.09145349846441,
84.3227894061678));
#140328=CARTESIAN_POINT('Ctrl Pts',(-6.74291524803591,-1.92112480601984,
84.314766119402));
#140329=CARTESIAN_POINT('Ctrl Pts',(-6.79143964011542,-1.75081007049133,
84.306743490073));
#140330=CARTESIAN_POINT('Ctrl Pts',(-6.83350796917286,-1.57865248384781,
84.2987208607439));
#140331=CARTESIAN_POINT('Ctrl Pts',(-6.86899310809759,-1.40519046517112,
84.2906982314149));
#140332=CARTESIAN_POINT('Ctrl Pts',(-6.9044915869081,-1.23166323712545,
84.2826725861484));
#140333=CARTESIAN_POINT('Ctrl Pts',(-6.93340186116331,-1.05683095741906,
84.274646940882));
#140334=CARTESIAN_POINT('Ctrl Pts',(-6.95564803756212,-0.881241703540063,
84.2666212956155));
#140335=CARTESIAN_POINT('Ctrl Pts',(-6.96876573878057,-0.777703579582816,
84.2618888861082));
#140336=CARTESIAN_POINT('Ctrl Pts',(-6.97956731078841,-0.673902400158773,
84.2571564766009));
#140337=CARTESIAN_POINT('Ctrl Pts',(-6.98804566086238,-0.569951229670105,
84.2524240670936));
#140338=CARTESIAN_POINT('Ctrl Pts',(-7.00368598321142,-0.378188705025704,
84.2436940182591));
#140339=CARTESIAN_POINT('Ctrl Pts',(-7.01142552498646,-0.185819746794032,
84.2349639694246));
#140340=CARTESIAN_POINT('Ctrl Pts',(-7.01124697880517,0.0065088167410221,
84.22623392059));
#140341=CARTESIAN_POINT('Ctrl Pts',(-7.01106838099703,0.198892992320853,
84.217501347451));
#140342=CARTESIAN_POINT('Ctrl Pts',(-7.00296712547114,0.391236475947701,
84.2087687743119));
#140343=CARTESIAN_POINT('Ctrl Pts',(-6.98697803043323,0.582893270456414,
84.2000362011728));
#140344=CARTESIAN_POINT('Ctrl Pts',(-6.97076178477665,0.777272855676073,
84.1911795678924));
#140345=CARTESIAN_POINT('Ctrl Pts',(-6.94643189688875,0.970945803205776,
84.1823229346119));
#140346=CARTESIAN_POINT('Ctrl Pts',(-6.9140791160314,1.16324397258634,84.1734663013314));
#140347=CARTESIAN_POINT('Ctrl Pts',(-6.88215921326528,1.35296920504148,
84.1647281692248));
#140348=CARTESIAN_POINT('Ctrl Pts',(-6.84242984472171,1.54135594969713,
84.1559900371182));
#140349=CARTESIAN_POINT('Ctrl Pts',(-6.79502978745767,1.7277721927566,84.1472519050116));
#140350=CARTESIAN_POINT('Ctrl Pts',(-6.7466655145538,1.91798052948543,84.1383360211442));
#140351=CARTESIAN_POINT('Ctrl Pts',(-6.69031520398364,2.10613704969951,
84.1294201372768));
#140352=CARTESIAN_POINT('Ctrl Pts',(-6.62618024995488,2.29158500990206,
84.1205042534095));
#140353=CARTESIAN_POINT('Ctrl Pts',(-6.56204529592617,2.4770329701045,84.1115883695421));
#140354=CARTESIAN_POINT('Ctrl Pts',(-6.49012580302942,2.65977208648038,
84.1026724856747));
#140355=CARTESIAN_POINT('Ctrl Pts',(-6.41067628819547,2.83916468181548,
84.0937566018073));
#140356=CARTESIAN_POINT('Ctrl Pts',(-6.33278797640512,3.01503216731923,
84.085015917311));
#140357=CARTESIAN_POINT('Ctrl Pts',(-6.24765455686776,3.18770210982274,
84.0762752328146));
#140358=CARTESIAN_POINT('Ctrl Pts',(-6.15555931687341,3.35659292422434,
84.0675345483183));
#140359=CARTESIAN_POINT('Ctrl Pts',(-6.06348064634292,3.52545335236228,
84.0587954364164));
#140360=CARTESIAN_POINT('Ctrl Pts',(-5.96444278781828,3.69053576997316,
84.0500563245144));
#140361=CARTESIAN_POINT('Ctrl Pts',(-5.8587749031339,3.85128331818219,84.0413172126125));
#140362=CARTESIAN_POINT('Ctrl Pts',(-5.75173793892203,4.01411358223249,
84.0324648729382));
#140363=CARTESIAN_POINT('Ctrl Pts',(-5.63789808562434,4.17249561437917,
84.0236125332639));
#140364=CARTESIAN_POINT('Ctrl Pts',(-5.51764347796998,4.32587991193877,
84.0147601935896));
#140365=CARTESIAN_POINT('Ctrl Pts',(-5.39898786138037,4.47722470243869,
84.0060255609397));
#140366=CARTESIAN_POINT('Ctrl Pts',(-5.27408720561891,4.62370362733829,
83.9972909282898));
#140367=CARTESIAN_POINT('Ctrl Pts',(-5.1433562343071,4.76482037536718,83.9885562956399));
#140368=CARTESIAN_POINT('Ctrl Pts',(-5.0099826870134,4.9087896358898,83.9796451024534));
#140369=CARTESIAN_POINT('Ctrl Pts',(-4.87054078900142,5.04717740252974,
83.9707339092669));
#140370=CARTESIAN_POINT('Ctrl Pts',(-4.72551276558456,5.17949376530153,
83.9618227160803));
#140371=CARTESIAN_POINT('Ctrl Pts',(-4.5804847421677,5.31181012807331,83.9529115228938));
#140372=CARTESIAN_POINT('Ctrl Pts',(-4.42987080819885,5.43805487271669,
83.9440003297073));
#140373=CARTESIAN_POINT('Ctrl Pts',(-4.2741923740152,5.55777888300806,83.9350891365208));
#140374=CARTESIAN_POINT('Ctrl Pts',(-4.13398410882107,5.66560560848266,
83.9270634716685));
#140375=CARTESIAN_POINT('Ctrl Pts',(-3.98960312497932,5.7681923137558,83.9190378068161));
#140376=CARTESIAN_POINT('Ctrl Pts',(-3.84148776816131,5.86520232298657,
83.9110121419638));
#140377=CARTESIAN_POINT('Ctrl Pts',(-3.69341941952446,5.96218154361994,
83.9029890242606));
#140378=CARTESIAN_POINT('Ctrl Pts',(-3.54161936381682,6.05358739132223,
83.8949659065575));
#140379=CARTESIAN_POINT('Ctrl Pts',(-3.38655599560282,6.13912575625769,
83.8869427888543));
#140380=CARTESIAN_POINT('Ctrl Pts',(-3.23151218223668,6.2246533340567,83.8789206829365));
#140381=CARTESIAN_POINT('Ctrl Pts',(-3.07320619725684,6.30431472647453,
83.8708985770187));
#140382=CARTESIAN_POINT('Ctrl Pts',(-2.91213211646133,6.37786116960651,
83.8628764711009));
#140383=CARTESIAN_POINT('Ctrl Pts',(-2.75099817999322,6.45143494284522,
83.8548513841414));
#140384=CARTESIAN_POINT('Ctrl Pts',(-2.5870944253451,6.51888907226207,83.846826297182));
#140385=CARTESIAN_POINT('Ctrl Pts',(-2.42093645749568,6.58002228197354,
83.8388012102225));
#140386=CARTESIAN_POINT('Ctrl Pts',(-2.25474576566647,6.64116753156456,
83.8307745427623));
#140387=CARTESIAN_POINT('Ctrl Pts',(-2.08630032326142,6.6959892631529,83.8227478753022));
#140388=CARTESIAN_POINT('Ctrl Pts',(-1.9161318709138,6.74433578759009,83.814721207842));
#140389=CARTESIAN_POINT('Ctrl Pts',(-1.74582680793195,6.79272112444683,
83.8066880966015));
#140390=CARTESIAN_POINT('Ctrl Pts',(-1.57379632744456,6.83462078067688,
83.798654985361));
#140391=CARTESIAN_POINT('Ctrl Pts',(-1.4005839705798,6.86993385003487,83.7906218741204));
#140392=CARTESIAN_POINT('Ctrl Pts',(-1.2985209576248,6.89074159331949,83.7858884731585));
#140393=CARTESIAN_POINT('Ctrl Pts',(-1.19604776993002,6.90926345064798,
83.7811550721965));
#140394=CARTESIAN_POINT('Ctrl Pts',(-1.09327653932811,6.92548720098844,
83.7764216712345));
#140395=CARTESIAN_POINT('Ctrl Pts',(-0.881564605848198,6.95890863160438,
83.7666707179402));
#140396=CARTESIAN_POINT('Ctrl Pts',(-0.668462914409056,6.98259511557202,
83.7569197646459));
#140397=CARTESIAN_POINT('Ctrl Pts',(-0.454786202916001,6.99648455098253,
83.7471688113516));
#140398=CARTESIAN_POINT('Ctrl Pts',(-0.240801650035402,7.01039399673034,
83.7374038099798));
#140399=CARTESIAN_POINT('Ctrl Pts',(-0.0262404585607778,7.01447815828874,
83.7276388086081));
#140400=CARTESIAN_POINT('Ctrl Pts',(0.188078825298634,7.00872691135661,
83.7178738072363));
#140401=CARTESIAN_POINT('Ctrl Pts',(0.402040883318102,7.00298525056147,
83.7081250820986));
#140402=CARTESIAN_POINT('Ctrl Pts',(0.615761801679578,6.98744094641748,
83.6983763569608));
#140403=CARTESIAN_POINT('Ctrl Pts',(0.828427412456071,6.96213577753202,
83.6886276318231));
#140404=CARTESIAN_POINT('Ctrl Pts',(1.0405093385911,6.93690006152318,83.6789056631558));
#140405=CARTESIAN_POINT('Ctrl Pts',(1.25154169969661,6.901956966926,83.6691836944886));
#140406=CARTESIAN_POINT('Ctrl Pts',(1.46071789642997,6.85739963758488,83.6594617258213));
#140407=CARTESIAN_POINT('Ctrl Pts',(1.66851002890356,6.81313713245423,83.6498040848815));
#140408=CARTESIAN_POINT('Ctrl Pts',(1.87447042766209,6.75938718329072,83.6401464439417));
#140409=CARTESIAN_POINT('Ctrl Pts',(2.07780996502803,6.69629243027291,83.6304888030018));
#140410=CARTESIAN_POINT('Ctrl Pts',(2.16718469223887,6.66856011410631,83.6262439373172));
#140411=CARTESIAN_POINT('Ctrl Pts',(2.25605311895002,6.63902314186761,83.6219990716325));
#140412=CARTESIAN_POINT('Ctrl Pts',(2.34434837785268,6.6076968185412,83.6177542059479));
#140413=CARTESIAN_POINT('Ctrl Pts',(2.50767059260701,6.54975164040406,83.609902358934));
#140414=CARTESIAN_POINT('Ctrl Pts',(2.66896336522398,6.48570442701392,83.6020505119202));
#140415=CARTESIAN_POINT('Ctrl Pts',(2.82772286466146,6.41573144412785,83.5941986649063));
#140416=CARTESIAN_POINT('Ctrl Pts',(2.98643734118826,6.34577830501409,83.5863490446128));
#140417=CARTESIAN_POINT('Ctrl Pts',(3.14261962486846,6.26990289290422,83.5784994243193));
#140418=CARTESIAN_POINT('Ctrl Pts',(3.29578514339501,6.18832989190757,83.5706498040258));
#140419=CARTESIAN_POINT('Ctrl Pts',(3.44893843361477,6.10676340347126,83.562800810424));
#140420=CARTESIAN_POINT('Ctrl Pts',(3.59907510180847,6.01950041166515,83.5549518168222));
#140421=CARTESIAN_POINT('Ctrl Pts',(3.74573473808128,5.92681177653139,83.5471028232205));
#140422=CARTESIAN_POINT('Ctrl Pts',(3.89246862383267,5.83407621585626,83.5392498559031));
#140423=CARTESIAN_POINT('Ctrl Pts',(4.03572163757369,5.73590972758238,83.5313968885857));
#140424=CARTESIAN_POINT('Ctrl Pts',(4.17506168012789,5.63262696524701,83.5235439212684));
#140425=CARTESIAN_POINT('Ctrl Pts',(4.31443711037073,5.52931797256055,83.5156889595612));
#140426=CARTESIAN_POINT('Ctrl Pts',(4.44989729177311,5.42089035558698,83.507833997854));
#140427=CARTESIAN_POINT('Ctrl Pts',(4.58104338155856,5.30769894575592,83.4999790361469));
#140428=CARTESIAN_POINT('Ctrl Pts',(4.71231964480065,5.19439518398892,83.4921162777336));
#140429=CARTESIAN_POINT('Ctrl Pts',(4.83927298478556,5.07631844510113,83.4842535193203));
#140430=CARTESIAN_POINT('Ctrl Pts',(4.96154118033183,4.95386068419081,83.4763907609071));
#140431=CARTESIAN_POINT('Ctrl Pts',(5.05123537414633,4.86402742794533,83.4706227541586));
#140432=CARTESIAN_POINT('Ctrl Pts',(5.13840904119081,4.771837304849,83.4648547474101));
#140433=CARTESIAN_POINT('Ctrl Pts',(5.22293326955456,4.67745599918162,83.4590867406616));
#140434=CARTESIAN_POINT('Ctrl Pts',(5.34492379289599,4.54123914047855,83.4507620014063));
#140435=CARTESIAN_POINT('Ctrl Pts',(5.46167577438176,4.40014251146621,83.442437262151));
#140436=CARTESIAN_POINT('Ctrl Pts',(5.57279233896684,4.25459893635728,83.4341125228956));
#140437=CARTESIAN_POINT('Ctrl Pts',(5.68381015413366,4.10918470599032,83.4257951818456));
#140438=CARTESIAN_POINT('Ctrl Pts',(5.78920233765805,3.95933167666587,83.4174778407957));
#140439=CARTESIAN_POINT('Ctrl Pts',(5.88861173929042,3.80550631932087,83.4091604997457));
#140440=CARTESIAN_POINT('Ctrl Pts',(5.9879684936774,3.65176242792578,83.4008475635617));
#140441=CARTESIAN_POINT('Ctrl Pts',(6.08134859910948,3.49405068185793,83.3925346273777));
#140442=CARTESIAN_POINT('Ctrl Pts',(6.16843733730753,3.33286774088178,83.3842216911937));
#140443=CARTESIAN_POINT('Ctrl Pts',(6.25549188772779,3.17174807429315,83.3759120183573));
#140444=CARTESIAN_POINT('Ctrl Pts',(6.33625983486509,3.00716022353939,83.3676023455208));
#140445=CARTESIAN_POINT('Ctrl Pts',(6.41047150296468,2.83962703047032,83.3592926726843));
#140446=CARTESIAN_POINT('Ctrl Pts',(6.46799035248137,2.70977795460457,83.3528521380129));
#140447=CARTESIAN_POINT('Ctrl Pts',(6.52157155441489,2.57816011610822,83.3464116033416));
#140448=CARTESIAN_POINT('Ctrl Pts',(6.57110895151814,2.44502632087636,83.3399710686702));
#140449=CARTESIAN_POINT('Origin',(0.,0.,50.));
#140450=CARTESIAN_POINT('',(6.57110895151812,2.4450263208764,81.339842993376));
#140451=CARTESIAN_POINT('',(6.57110895151811,2.44502632087644,81.8868302382415));
#140452=CARTESIAN_POINT('',(6.57110895151814,2.44502632087636,50.));
#140453=CARTESIAN_POINT('',(7.01124961619472,0.00231989425607759,83.7735343569347));
#140454=CARTESIAN_POINT('Ctrl Pts',(6.57110895151811,2.44502632087644,81.8868302382415));
#140455=CARTESIAN_POINT('Ctrl Pts',(6.50690213833289,2.61758477608302,81.8952030318929));
#140456=CARTESIAN_POINT('Ctrl Pts',(6.43585859289123,2.78770811981673,81.9035758255444));
#140457=CARTESIAN_POINT('Ctrl Pts',(6.35818746868627,2.95483987307958,81.9119486191959));
#140458=CARTESIAN_POINT('Ctrl Pts',(6.28055906938963,3.12187969141926,81.9203168071867));
#140459=CARTESIAN_POINT('Ctrl Pts',(6.19631049858508,3.28593090300688,81.9286849951776));
#140460=CARTESIAN_POINT('Ctrl Pts',(6.10569894647632,3.4464571573571,81.9370531831684));
#140461=CARTESIAN_POINT('Ctrl Pts',(6.01512396242723,3.60691862820553,81.9454179940137));
#140462=CARTESIAN_POINT('Ctrl Pts',(5.9181912791183,3.7638576927618,81.953782804859));
#140463=CARTESIAN_POINT('Ctrl Pts',(5.81520414381981,3.9167623527859,81.9621476157043));
#140464=CARTESIAN_POINT('Ctrl Pts',(5.71224349526661,4.06962768802664,81.9705102752459));
#140465=CARTESIAN_POINT('Ctrl Pts',(5.60323168374978,4.2184604157847,81.9788729347874));
#140466=CARTESIAN_POINT('Ctrl Pts',(5.48851565883485,4.36277691673831,81.9872355943289));
#140467=CARTESIAN_POINT('Ctrl Pts',(5.37379223353033,4.50710272762341,81.9955987933499));
#140468=CARTESIAN_POINT('Ctrl Pts',(5.25336405922103,4.64691146843435,82.0039619923709));
#140469=CARTESIAN_POINT('Ctrl Pts',(5.12761928507243,4.7817514604853,82.0123251913918));
#140470=CARTESIAN_POINT('Ctrl Pts',(5.00186741468376,4.91659906205292,82.0206888623789));
#140471=CARTESIAN_POINT('Ctrl Pts',(4.87079857025712,5.04647711507872,82.029052533366));
#140472=CARTESIAN_POINT('Ctrl Pts',(4.73483890286805,5.17096965049954,82.037416204353));
#140473=CARTESIAN_POINT('Ctrl Pts',(4.59885343658502,5.29548580887988,82.0457814623803));
#140474=CARTESIAN_POINT('Ctrl Pts',(4.45797553927358,5.41461418987642,82.0541467204076));
#140475=CARTESIAN_POINT('Ctrl Pts',(4.31266599652032,5.52797780069325,82.0625119784349));
#140476=CARTESIAN_POINT('Ctrl Pts',(4.16730950067788,5.6413780420825,82.0708799394829));
#140477=CARTESIAN_POINT('Ctrl Pts',(4.01751876314148,5.74900959678093,82.0792479005309));
#140478=CARTESIAN_POINT('Ctrl Pts',(3.86378555145235,5.85053739197418,82.0876158615789));
#140479=CARTESIAN_POINT('Ctrl Pts',(3.70991018257048,5.95215906998034,82.0959915604855));
#140480=CARTESIAN_POINT('Ctrl Pts',(3.55208532887637,6.0476655279089,82.1043672593921));
#140481=CARTESIAN_POINT('Ctrl Pts',(3.39083056755593,6.13676581145381,82.1127429582987));
#140482=CARTESIAN_POINT('Ctrl Pts',(3.22949847165443,6.22590882572521,82.1211226740241));
#140483=CARTESIAN_POINT('Ctrl Pts',(3.06473347863258,6.30863938566825,82.1295023897495));
#140484=CARTESIAN_POINT('Ctrl Pts',(2.89707797346671,6.3847134452655,82.137882105475));
#140485=CARTESIAN_POINT('Ctrl Pts',(2.72922743845101,6.46087600009232,82.1462715691338));
#140486=CARTESIAN_POINT('Ctrl Pts',(2.55847997405498,6.53036645043005,82.1546610327927));
#140487=CARTESIAN_POINT('Ctrl Pts',(2.38539736604835,6.59298915277051,82.1630504964515));
#140488=CARTESIAN_POINT('Ctrl Pts',(2.26024876159711,6.63826894081584,82.1691165575139));
#140489=CARTESIAN_POINT('Ctrl Pts',(2.13387969783636,6.67995921662382,82.1751826185762));
#140490=CARTESIAN_POINT('Ctrl Pts',(2.00650681878623,6.71800245226692,82.1812486796386));
#140491=CARTESIAN_POINT('Ctrl Pts',(1.83051941084736,6.77056568613873,82.1896299800435));
#140492=CARTESIAN_POINT('Ctrl Pts',(1.65226018973621,6.81627070874339,82.1980112804485));
#140493=CARTESIAN_POINT('Ctrl Pts',(1.47228955156789,6.85492451007624,82.2063925808534));
#140494=CARTESIAN_POINT('Ctrl Pts',(1.29254699983778,6.89352932337439,82.214763259187));
#140495=CARTESIAN_POINT('Ctrl Pts',(1.11109767133269,6.92510065645381,82.2231339375206));
#140496=CARTESIAN_POINT('Ctrl Pts',(0.928517585887898,6.94949506476528,
82.2315046158542));
#140497=CARTESIAN_POINT('Ctrl Pts',(0.746144697492237,6.97386178961168,
82.2398657949051));
#140498=CARTESIAN_POINT('Ctrl Pts',(0.562643932535991,6.99106777960089,
82.248226973956));
#140499=CARTESIAN_POINT('Ctrl Pts',(0.378602425090457,7.00102040892723,
82.2565881530069));
#140500=CARTESIAN_POINT('Ctrl Pts',(0.194799733210726,7.01096012354299,
82.2649384824416));
#140501=CARTESIAN_POINT('Ctrl Pts',(0.0104580240394714,7.01366523329996,
82.2732888118764));
#140502=CARTESIAN_POINT('Ctrl Pts',(-0.173829587198575,7.00909479441635,
82.2816391413112));
#140503=CARTESIAN_POINT('Ctrl Pts',(-0.357975400143808,7.00452787221206,
82.2899830456669));
#140504=CARTESIAN_POINT('Ctrl Pts',(-0.54206687194791,6.99269656544896,
82.2983269500227));
#140505=CARTESIAN_POINT('Ctrl Pts',(-0.725508864328621,6.97361193717292,
82.3066708543785));
#140506=CARTESIAN_POINT('Ctrl Pts',(-0.908803514956873,6.95454263778934,
82.3150080568583));
#140507=CARTESIAN_POINT('Ctrl Pts',(-1.09144940160192,6.9282316696525,82.323345259338));
#140508=CARTESIAN_POINT('Ctrl Pts',(-1.27285433479264,6.89474208400137,
82.3316824618178));
#140509=CARTESIAN_POINT('Ctrl Pts',(-1.33257183746027,6.88371749726449,
82.3344270228535));
#140510=CARTESIAN_POINT('Ctrl Pts',(-1.39215489262231,6.87191538931436,
82.3371715838893));
#140511=CARTESIAN_POINT('Ctrl Pts',(-1.45158250318337,6.85933923923813,
82.339916144925));
#140512=CARTESIAN_POINT('Ctrl Pts',(-1.63213081342337,6.82113136542071,
82.3482544552268));
#140513=CARTESIAN_POINT('Ctrl Pts',(-1.81109548286814,6.7758064957697,82.3565927655286));
#140514=CARTESIAN_POINT('Ctrl Pts',(-1.98790383542348,6.72353068734044,
82.3649310758304));
#140515=CARTESIAN_POINT('Ctrl Pts',(-2.16482342979489,6.67122198874631,
82.3732746323142));
#140516=CARTESIAN_POINT('Ctrl Pts',(-2.33958368700241,6.61195372119245,
82.3816181887979));
#140517=CARTESIAN_POINT('Ctrl Pts',(-2.51162909084586,6.54594117545497,
82.3899617452816));
#140518=CARTESIAN_POINT('Ctrl Pts',(-2.68380538608278,6.47987840766038,
82.3983116495068));
#140519=CARTESIAN_POINT('Ctrl Pts',(-2.85326240249981,6.40706124421809,
82.4066615537319));
#140520=CARTESIAN_POINT('Ctrl Pts',(-3.01946611920712,6.3277524380668,82.415011457957));
#140521=CARTESIAN_POINT('Ctrl Pts',(-3.18591912918995,6.24832467457535,
82.4233738864206));
#140522=CARTESIAN_POINT('Ctrl Pts',(-3.34910879230402,6.16238595204779,
82.4317363148842));
#140523=CARTESIAN_POINT('Ctrl Pts',(-3.50852581951479,6.07024489920284,
82.4400987433477));
#140524=CARTESIAN_POINT('Ctrl Pts',(-3.66807917001557,5.97802505319702,
82.4484683228276));
#140525=CARTESIAN_POINT('Ctrl Pts',(-3.82385317134599,5.87959246895441,
82.4568379023075));
#140526=CARTESIAN_POINT('Ctrl Pts',(-3.97536843561313,5.77529846532894,
82.4652074817873));
#140527=CARTESIAN_POINT('Ctrl Pts',(-4.12711739371517,5.6708436009098,82.4735899703238));
#140528=CARTESIAN_POINT('Ctrl Pts',(-4.27459422692132,5.56050944734027,
82.4819724588603));
#140529=CARTESIAN_POINT('Ctrl Pts',(-4.41735237277946,5.44468773918208,
82.4903549473968));
#140530=CARTESIAN_POINT('Ctrl Pts',(-4.46406517734358,5.40678897841467,
82.4930978350016));
#140531=CARTESIAN_POINT('Ctrl Pts',(-4.51027304345832,5.36830295604337,
82.4958407226065));
#140532=CARTESIAN_POINT('Ctrl Pts',(-4.5559612031742,5.32924423137761,82.4985836102113));
#140533=CARTESIAN_POINT('Ctrl Pts',(-4.69571065576719,5.20977267846402,
82.5069734653442));
#140534=CARTESIAN_POINT('Ctrl Pts',(-4.83087709247407,5.0846989550127,82.515363320477));
#140535=CARTESIAN_POINT('Ctrl Pts',(-4.96100246275921,4.95440017832604,
82.5237531756098));
#140536=CARTESIAN_POINT('Ctrl Pts',(-5.09100775517699,4.82422163952374,
82.532135288702));
#140537=CARTESIAN_POINT('Ctrl Pts',(-5.21598102341299,4.68882789082791,
82.5405174017941));
#140538=CARTESIAN_POINT('Ctrl Pts',(-5.33549858863921,4.54863511101177,
82.5488995148863));
#140539=CARTESIAN_POINT('Ctrl Pts',(-5.45492343356569,4.40855109107991,
82.5572751252352));
#140540=CARTESIAN_POINT('Ctrl Pts',(-5.56890080123639,4.26367571187785,
82.5656507355841));
#140541=CARTESIAN_POINT('Ctrl Pts',(-5.67704476442226,4.11446099814372,
82.574026345933));
#140542=CARTESIAN_POINT('Ctrl Pts',(-5.78512070344939,3.96534014268033,
82.5823966878986));
#140543=CARTESIAN_POINT('Ctrl Pts',(-5.88737036183101,3.81188566056055,
82.5907670298642));
#140544=CARTESIAN_POINT('Ctrl Pts',(-5.98344863787123,3.65458191322304,
82.5991373718298));
#140545=CARTESIAN_POINT('Ctrl Pts',(-6.07948056324542,3.49735405331563,
82.6075036757242));
#140546=CARTESIAN_POINT('Ctrl Pts',(-6.16934687232832,3.33628091135612,
82.6158699796185));
#140547=CARTESIAN_POINT('Ctrl Pts',(-6.25274603156845,3.17187541167762,
82.6242362835129));
#140548=CARTESIAN_POINT('Ctrl Pts',(-6.33612186640129,3.00751589160932,
82.6326002475865));
#140549=CARTESIAN_POINT('Ctrl Pts',(-6.41303400803496,2.83982616433852,
82.6409642116602));
#140550=CARTESIAN_POINT('Ctrl Pts',(-6.48322683788517,2.66934380157849,
82.6493281757338));
#140551=CARTESIAN_POINT('Ctrl Pts',(-6.55340886622532,2.49888767322102,
82.6576908527324));
#140552=CARTESIAN_POINT('Ctrl Pts',(-6.6168735192609,2.32564007000848,82.666053529731));
#140553=CARTESIAN_POINT('Ctrl Pts',(-6.67341313985606,2.15015897721458,
82.6744162067296));
#140554=CARTESIAN_POINT('Ctrl Pts',(-6.72995159640377,1.97468149725567,
82.6827787115559));
#140555=CARTESIAN_POINT('Ctrl Pts',(-6.77956520439842,1.79697093234247,
82.6911412163822));
#140556=CARTESIAN_POINT('Ctrl Pts',(-6.82209591188067,1.61760128944096,
82.6995037212086));
#140557=CARTESIAN_POINT('Ctrl Pts',(-6.86463141277395,1.43821143073598,
82.7078671685286));
#140558=CARTESIAN_POINT('Ctrl Pts',(-6.90008234632228,1.25716244114014,
82.7162306158486));
#140559=CARTESIAN_POINT('Ctrl Pts',(-6.92834149970032,1.07503982532291,
82.7245940631686));
#140560=CARTESIAN_POINT('Ctrl Pts',(-6.95661729286205,0.892809970591258,
82.7329624351215));
#140561=CARTESIAN_POINT('Ctrl Pts',(-6.97769279247474,0.709505551352474,
82.7413308070743));
#140562=CARTESIAN_POINT('Ctrl Pts',(-6.99151239034198,0.525719562309206,
82.7496991790271));
#140563=CARTESIAN_POINT('Ctrl Pts',(-7.00533612892193,0.341878506180315,
82.7580700583629));
#140564=CARTESIAN_POINT('Ctrl Pts',(-7.01189961136644,0.157555920727849,
82.7664409376987));
#140565=CARTESIAN_POINT('Ctrl Pts',(-7.01119933913218,-0.0266531321334792,
82.7748118170345));
#140566=CARTESIAN_POINT('Ctrl Pts',(-7.01049847356482,-0.211018263333262,
82.7831897889258));
#140567=CARTESIAN_POINT('Ctrl Pts',(-7.00252156215909,-0.395269340835481,
82.7915677608171));
#140568=CARTESIAN_POINT('Ctrl Pts',(-6.98731721408861,-0.578813192835963,
82.7999457327085));
#140569=CARTESIAN_POINT('Ctrl Pts',(-6.97765472708107,-0.695456805376881,
82.8052700020671));
#140570=CARTESIAN_POINT('Ctrl Pts',(-6.96507433820147,-0.811814874622516,
82.8105942714257));
#140571=CARTESIAN_POINT('Ctrl Pts',(-6.94959934240903,-0.927736785132497,
82.8159185407843));
#140572=CARTESIAN_POINT('Ctrl Pts',(-6.92674601336525,-1.09892917831956,
82.8237813719736));
#140573=CARTESIAN_POINT('Ctrl Pts',(-6.89752954876146,-1.26952587813197,
82.8316442031629));
#140574=CARTESIAN_POINT('Ctrl Pts',(-6.86199066830925,-1.43899639698532,
82.8395070343521));
#140575=CARTESIAN_POINT('Ctrl Pts',(-6.82647909479559,-1.60833670011481,
82.8473638239935));
#140576=CARTESIAN_POINT('Ctrl Pts',(-6.78465484389672,-1.77655217235846,
82.8552206136349));
#140577=CARTESIAN_POINT('Ctrl Pts',(-6.73661038061163,-1.94311789203219,
82.8630774032762));
#140578=CARTESIAN_POINT('Ctrl Pts',(-6.6885930121295,-2.10958967652492,
82.8709297620602));
#140579=CARTESIAN_POINT('Ctrl Pts',(-6.63436251462618,-2.27441319399653,
82.8787821208441));
#140580=CARTESIAN_POINT('Ctrl Pts',(-6.57406228090888,-2.43707441191916,
82.886634479628));
#140581=CARTESIAN_POINT('Ctrl Pts',(-6.51377628478036,-2.59969722363028,
82.8944849843785));
#140582=CARTESIAN_POINT('Ctrl Pts',(-6.44742352927182,-2.76015839181148,
82.9023354891289));
#140583=CARTESIAN_POINT('Ctrl Pts',(-6.37519703030342,-2.91795979878244,
82.9101859938793));
#140584=CARTESIAN_POINT('Ctrl Pts',(-6.30298215030234,-3.07573582048045,
82.9180352357309));
#140585=CARTESIAN_POINT('Ctrl Pts',(-6.2248955693807,-3.23085258706953,
82.9258844775825));
#140586=CARTESIAN_POINT('Ctrl Pts',(-6.14117794585039,-3.3828331321395,
82.9337337194341));
#140587=CARTESIAN_POINT('Ctrl Pts',(-6.05743211621404,-3.53486488242996,
82.941585605849));
#140588=CARTESIAN_POINT('Ctrl Pts',(-5.96805163865431,-3.6837579661236,
82.9494374922638));
#140589=CARTESIAN_POINT('Ctrl Pts',(-5.87332261961814,-3.82906097736532,
82.9572893786786));
#140590=CARTESIAN_POINT('Ctrl Pts',(-5.80376428000776,-3.9357551699707,
82.9630549211426));
#140591=CARTESIAN_POINT('Ctrl Pts',(-5.73132307943708,-4.04051419631888,
82.9688204636066));
#140592=CARTESIAN_POINT('Ctrl Pts',(-5.65612682125141,-4.14316979430248,
82.9745860060706));
#140593=CARTESIAN_POINT('Ctrl Pts',(-5.53019890309834,-4.31508268003297,
82.9842413104306));
#140594=CARTESIAN_POINT('Ctrl Pts',(-5.39660821342806,-4.48100845535787,
82.9938966147905));
#140595=CARTESIAN_POINT('Ctrl Pts',(-5.25591274746692,-4.64036720028865,
83.0035519191505));
#140596=CARTESIAN_POINT('Ctrl Pts',(-5.11443785501876,-4.80060876277072,
83.0132607120853));
#140597=CARTESIAN_POINT('Ctrl Pts',(-4.96577932222475,-4.95421033393521,
83.0229695050201));
#140598=CARTESIAN_POINT('Ctrl Pts',(-4.81053572744779,-5.10062472423216,
83.0326782979549));
#140599=CARTESIAN_POINT('Ctrl Pts',(-4.65454508731076,-5.24774367300752,
83.0424338104257));
#140600=CARTESIAN_POINT('Ctrl Pts',(-4.49190590488925,-5.38760609160965,
83.0521893228965));
#140601=CARTESIAN_POINT('Ctrl Pts',(-4.32325600338168,-5.51969963781765,
83.0619448353673));
#140602=CARTESIAN_POINT('Ctrl Pts',(-4.1544391125254,-5.65192397695854,
83.0717100072962));
#140603=CARTESIAN_POINT('Ctrl Pts',(-3.97959963522644,-5.77636404234841,
83.0814751792252));
#140604=CARTESIAN_POINT('Ctrl Pts',(-3.79940714173115,-5.89254884866153,
83.0912403511542));
#140605=CARTESIAN_POINT('Ctrl Pts',(-3.61946033661267,-6.00857523962716,
83.1009922084928));
#140606=CARTESIAN_POINT('Ctrl Pts',(-3.43417513472253,-6.11636884740361,
83.1107440658314));
#140607=CARTESIAN_POINT('Ctrl Pts',(-3.24424756247317,-6.21550354483745,
83.12049592317));
#140608=CARTESIAN_POINT('Ctrl Pts',(-3.16142538577055,-6.25873345259116,
83.1247484392324));
#140609=CARTESIAN_POINT('Ctrl Pts',(-3.07772079202042,-6.300317342639,83.1290009552948));
#140610=CARTESIAN_POINT('Ctrl Pts',(-2.99319322076635,-6.34022246499746,
83.1332534713572));
#140611=CARTESIAN_POINT('Ctrl Pts',(-2.83351978878438,-6.41560364235889,
83.1412865169559));
#140612=CARTESIAN_POINT('Ctrl Pts',(-2.67083014928581,-6.48502775193599,
83.1493195625547));
#140613=CARTESIAN_POINT('Ctrl Pts',(-2.50561624273084,-6.54824509366162,
83.1573526081534));
#140614=CARTESIAN_POINT('Ctrl Pts',(-2.34050854203638,-6.61142179684586,
83.1653804898012));
#140615=CARTESIAN_POINT('Ctrl Pts',(-2.1728801452354,-6.66839954381496,
83.1734083714489));
#140616=CARTESIAN_POINT('Ctrl Pts',(-2.00324500790806,-6.71897581486877,
83.1814362530967));
#140617=CARTESIAN_POINT('Ctrl Pts',(-1.83368646251739,-6.76952925023765,
83.1894605100768));
#140618=CARTESIAN_POINT('Ctrl Pts',(-1.66212333123537,-6.81368686015066,
83.1974847670568));
#140619=CARTESIAN_POINT('Ctrl Pts',(-1.4890868020357,-6.85129528326601,
83.2055090240369));
#140620=CARTESIAN_POINT('Ctrl Pts',(-1.31607119471488,-6.88889915913995,
83.2135323108026));
#140621=CARTESIAN_POINT('Ctrl Pts',(-1.14158290067859,-6.91995534013052,
83.2215555975682));
#140622=CARTESIAN_POINT('Ctrl Pts',(-0.966165607669418,-6.94436106355774,
83.2295788843339));
#140623=CARTESIAN_POINT('Ctrl Pts',(-0.790762688542486,-6.96876478715365,
83.2376015136628));
#140624=CARTESIAN_POINT('Ctrl Pts',(-0.614431285773459,-6.98651909212087,
83.2456241429916));
#140625=CARTESIAN_POINT('Ctrl Pts',(-0.437722255315089,-6.99757284990316,
83.2536467723205));
#140626=CARTESIAN_POINT('Ctrl Pts',(-0.260946794841701,-7.00863076311143,
83.2616724175869));
#140627=CARTESIAN_POINT('Ctrl Pts',(-0.0837937893760947,-7.01298307725059,
83.2696980628532));
#140628=CARTESIAN_POINT('Ctrl Pts',(0.0931834548161807,-7.01063074239747,
83.2777237081196));
#140629=CARTESIAN_POINT('Ctrl Pts',(0.197540022458685,-7.00924366242379,
83.2824561176276));
#140630=CARTESIAN_POINT('Ctrl Pts',(0.301835470608092,-7.00552636419648,
83.2871885271356));
#140631=CARTESIAN_POINT('Ctrl Pts',(0.40595684536479,-6.99948752425501,
83.2919209366435));
#140632=CARTESIAN_POINT('Ctrl Pts',(0.59803335202259,-6.98834745543693,
83.3006509854783));
#140633=CARTESIAN_POINT('Ctrl Pts',(0.789613284956578,-6.96929894113836,
83.3093810343131));
#140634=CARTESIAN_POINT('Ctrl Pts',(0.980053679312014,-6.94241466264923,
83.3181110831478));
#140635=CARTESIAN_POINT('Ctrl Pts',(1.17054913974443,-6.91552261053752,
83.326843656287));
#140636=CARTESIAN_POINT('Ctrl Pts',(1.35990413264777,-6.8807903100262,83.3355762294263));
#140637=CARTESIAN_POINT('Ctrl Pts',(1.54748375458744,-6.83834194756214,
83.3443088025655));
#140638=CARTESIAN_POINT('Ctrl Pts',(1.73772824448788,-6.79529053834947,
83.3531654358459));
#140639=CARTESIAN_POINT('Ctrl Pts',(1.92614625231635,-6.74430222228833,
83.3620220691263));
#140640=CARTESIAN_POINT('Ctrl Pts',(2.11208871267477,-6.68555964989408,
83.3708787024066));
#140641=CARTESIAN_POINT('Ctrl Pts',(2.29554327508537,-6.62760304927318,
83.3796168345135));
#140642=CARTESIAN_POINT('Ctrl Pts',(2.47658786607273,-6.56209851230751,
83.3883549666203));
#140643=CARTESIAN_POINT('Ctrl Pts',(2.65461586620692,-6.48927123530697,
83.3970930987271));
#140644=CARTESIAN_POINT('Ctrl Pts',(2.83626532571248,-6.41496250019543,
83.4060089825943));
#140645=CARTESIAN_POINT('Ctrl Pts',(3.01477387673478,-6.33303002305587,
83.4149248664614));
#140646=CARTESIAN_POINT('Ctrl Pts',(3.18951910498884,-6.24376444474095,
83.4238407503286));
#140647=CARTESIAN_POINT('Ctrl Pts',(3.36426433324302,-6.15449886642596,
83.4327566341957));
#140648=CARTESIAN_POINT('Ctrl Pts',(3.53524597218751,-6.05790032992442,
83.4416725180629));
#140649=CARTESIAN_POINT('Ctrl Pts',(3.70186786591578,-5.9543094365174,83.45058840193));
#140650=CARTESIAN_POINT('Ctrl Pts',(3.86521559732683,-5.85275413034331,
83.4593290864261));
#140651=CARTESIAN_POINT('Ctrl Pts',(4.02439068243599,-5.74446793341555,
83.4680697709222));
#140652=CARTESIAN_POINT('Ctrl Pts',(4.1788565091602,-5.62981214947262,83.4768104554184));
#140653=CARTESIAN_POINT('Ctrl Pts',(4.33329454491655,-5.51517699400961,
83.4855495673201));
#140654=CARTESIAN_POINT('Ctrl Pts',(4.48302479458871,-5.39417470329896,
83.4942886792219));
#140655=CARTESIAN_POINT('Ctrl Pts',(4.62754150307087,-5.26720857759179,
83.5030277911237));
#140656=CARTESIAN_POINT('Ctrl Pts',(4.77393063350921,-5.13859742298823,
83.5118801307981));
#140657=CARTESIAN_POINT('Ctrl Pts',(4.91496995417719,-5.00386698718462,
83.5207324704725));
#140658=CARTESIAN_POINT('Ctrl Pts',(5.05016918408609,-4.86347795045966,
83.5295848101469));
#140659=CARTESIAN_POINT('Ctrl Pts',(5.18357070856565,-4.72495562653854,
83.5383194427966));
#140660=CARTESIAN_POINT('Ctrl Pts',(5.31128630094435,-4.58092446077574,
83.5470540754463));
#140661=CARTESIAN_POINT('Ctrl Pts',(5.43288204853427,-4.43186407837764,
83.5557887080959));
#140662=CARTESIAN_POINT('Ctrl Pts',(5.55693571408816,-4.27979061206111,
83.5646999012827));
#140663=CARTESIAN_POINT('Ctrl Pts',(5.67461928824213,-4.12248265532379,
83.5736110944694));
#140664=CARTESIAN_POINT('Ctrl Pts',(5.78551457111115,-3.9604857921675,83.5825222876561));
#140665=CARTESIAN_POINT('Ctrl Pts',(5.89640985398017,-3.7984889290112,83.5914334808429));
#140666=CARTESIAN_POINT('Ctrl Pts',(6.00051666321512,-3.63180340196017,
83.6003446740296));
#140667=CARTESIAN_POINT('Ctrl Pts',(6.09746263884109,-3.4610079356218,83.6092558672163));
#140668=CARTESIAN_POINT('Ctrl Pts',(6.18477484191618,-3.30718485689209,
83.6172815320687));
#140669=CARTESIAN_POINT('Ctrl Pts',(6.26631835344879,-3.14995713566829,
83.6253071969211));
#140670=CARTESIAN_POINT('Ctrl Pts',(6.34182062979834,-2.98980562277286,
83.6333328617735));
#140671=CARTESIAN_POINT('Ctrl Pts',(6.41729894357731,-2.8297049380394,83.6413559794767));
#140672=CARTESIAN_POINT('Ctrl Pts',(6.48673968328614,-2.66668264025154,
83.6493790971799));
#140673=CARTESIAN_POINT('Ctrl Pts',(6.5499166315901,-2.50124342712168,83.6574022148831));
#140674=CARTESIAN_POINT('Ctrl Pts',(6.613085612728,-2.33582507732441,83.665424320801));
#140675=CARTESIAN_POINT('Ctrl Pts',(6.66999224570556,-2.16799076186445,
83.6734464267189));
#140676=CARTESIAN_POINT('Ctrl Pts',(6.72045878597691,-1.99826431396994,
83.6814685326367));
#140677=CARTESIAN_POINT('Ctrl Pts',(6.77094407978509,-1.82847479515412,
83.6894936195962));
#140678=CARTESIAN_POINT('Ctrl Pts',(6.81498439266014,-1.65679209012733,
83.6975187065557));
#140679=CARTESIAN_POINT('Ctrl Pts',(6.852451997612,-1.48375475834902,83.7055437935152));
#140680=CARTESIAN_POINT('Ctrl Pts',(6.88992698162119,-1.31068334773399,
83.7135704609755));
#140681=CARTESIAN_POINT('Ctrl Pts',(6.92082660996158,-1.1362571390085,83.7215971284357));
#140682=CARTESIAN_POINT('Ctrl Pts',(6.94507450261422,-0.961023785157178,
83.7296237958959));
#140683=CARTESIAN_POINT('Ctrl Pts',(6.96934186138961,-0.785649754587056,
83.7376569071365));
#140684=CARTESIAN_POINT('Ctrl Pts',(6.98694677815085,-0.609467649039707,
83.7456900183771));
#140685=CARTESIAN_POINT('Ctrl Pts',(6.99786480243257,-0.433029755762056,
83.7537231296177));
#140686=CARTESIAN_POINT('Ctrl Pts',(7.00429809895839,-0.329066139584161,
83.7584565305794));
#140687=CARTESIAN_POINT('Ctrl Pts',(7.00841069794281,-0.225013749300497,
83.7631899315412));
#140688=CARTESIAN_POINT('Ctrl Pts',(7.01020606780221,-0.120985327412369,
83.7679233325029));
#140689=CARTESIAN_POINT('Ctrl Pts',(7.0109154847157,-0.0798798573698832,
83.7697936739721));
#140690=CARTESIAN_POINT('Ctrl Pts',(7.01126321422435,-0.0387764624473275,
83.7716640154413));
#140691=CARTESIAN_POINT('Ctrl Pts',(7.0112496161949,0.00231989372472653,
83.7735343569105));
#140692=CARTESIAN_POINT('Ctrl Pts',(7.01124961619472,0.00231989425587762,
83.7735343569347));
#140693=CARTESIAN_POINT('Ctrl Pts',(7.0111790285611,0.215651824307297,83.7832433334144));
#140694=CARTESIAN_POINT('Ctrl Pts',(7.00136754561913,0.428863000641898,
83.7929523098941));
#140695=CARTESIAN_POINT('Ctrl Pts',(6.98187348596674,0.64114677606196,83.8026612863738));
#140696=CARTESIAN_POINT('Ctrl Pts',(6.96237311657637,0.853499262413789,
83.8123734054056));
#140697=CARTESIAN_POINT('Ctrl Pts',(6.93318392099452,1.06492369523564,83.8220855244373));
#140698=CARTESIAN_POINT('Ctrl Pts',(6.89441601631981,1.27461929861933,83.8317976434691));
#140699=CARTESIAN_POINT('Ctrl Pts',(6.85574551333199,1.48378805626106,83.8414853614716));
#140700=CARTESIAN_POINT('Ctrl Pts',(6.80754438516368,1.69123660806533,83.8511730794741));
#140701=CARTESIAN_POINT('Ctrl Pts',(6.74997311842575,1.89617759269267,83.8608607974766));
#140702=CARTESIAN_POINT('Ctrl Pts',(6.69795058159319,2.08136632529099,83.8696148113305));
#140703=CARTESIAN_POINT('Ctrl Pts',(6.63827767335995,2.26450761414988,83.8783688251844));
#140704=CARTESIAN_POINT('Ctrl Pts',(6.57110895151815,2.44502632087633,83.8871228390383));
#140705=CARTESIAN_POINT('',(7.01124847424792,-0.00462545740594696,83.2264656430532));
#140706=CARTESIAN_POINT('Ctrl Pts',(6.57110895151814,2.44502632087636,83.3399710686702));
#140707=CARTESIAN_POINT('Ctrl Pts',(6.63500113977313,2.27331343312962,83.3316642161154));
#140708=CARTESIAN_POINT('Ctrl Pts',(6.69216465663035,2.09907831971231,83.3233573635606));
#140709=CARTESIAN_POINT('Ctrl Pts',(6.74241499103036,1.92287978075309,83.3150505110058));
#140710=CARTESIAN_POINT('Ctrl Pts',(6.79267769512076,1.74663786852284,83.3067416136249));
#140711=CARTESIAN_POINT('Ctrl Pts',(6.83602372137104,1.56843188663344,83.2984327162441));
#140712=CARTESIAN_POINT('Ctrl Pts',(6.87231865653561,1.38883506779339,83.2901238188632));
#140713=CARTESIAN_POINT('Ctrl Pts',(6.90861788899793,1.20921698480165,83.281813937714));
#140714=CARTESIAN_POINT('Ctrl Pts',(6.93786430419882,1.02820806611816,83.2735040565649));
#140715=CARTESIAN_POINT('Ctrl Pts',(6.95997478920127,0.846390864898014,
83.2651941754157));
#140716=CARTESIAN_POINT('Ctrl Pts',(6.98209784835813,0.664470264880261,
83.2568795684666));
#140717=CARTESIAN_POINT('Ctrl Pts',(6.99707683296611,0.481740797382236,
83.2485649615175));
#140718=CARTESIAN_POINT('Ctrl Pts',(7.00488051387247,0.298790141855086,
83.2402503545684));
#140719=CARTESIAN_POINT('Ctrl Pts',(7.00919306448075,0.197686064145291,
83.2356554507421));
#140720=CARTESIAN_POINT('Ctrl Pts',(7.011315198226,0.0965144795200406,83.2310605469158));
#140721=CARTESIAN_POINT('Ctrl Pts',(7.01124847424845,-0.00462545660722081,
83.2264656430895));
#140722=CARTESIAN_POINT('Ctrl Pts',(7.01124847424792,-0.00462545740615106,
83.2264656430532));
#140723=CARTESIAN_POINT('Ctrl Pts',(7.01109761289103,-0.233300454381342,
83.2160766744734));
#140724=CARTESIAN_POINT('Ctrl Pts',(6.99975542124624,-0.461583810264566,
83.2056877058936));
#140725=CARTESIAN_POINT('Ctrl Pts',(6.97735941040463,-0.688536288468472,
83.1952987373138));
#140726=CARTESIAN_POINT('Ctrl Pts',(6.95466206942481,-0.918542329295982,
83.1847699889598));
#140727=CARTESIAN_POINT('Ctrl Pts',(6.92061145572012,-1.14718165366891,
83.1742412406059));
#140728=CARTESIAN_POINT('Ctrl Pts',(6.87540077451661,-1.37349581443717,
83.1637124922519));
#140729=CARTESIAN_POINT('Ctrl Pts',(6.84396755419073,-1.53084320865742,
83.1563922648641));
#140730=CARTESIAN_POINT('Ctrl Pts',(6.80714072867915,-1.68706705158743,
83.1490720374764));
#140731=CARTESIAN_POINT('Ctrl Pts',(6.76499934449835,-1.84184973095988,
83.1417518100886));
#140732=CARTESIAN_POINT('Ctrl Pts',(6.71674953181093,-2.01906828778123,
83.1333705096839));
#140733=CARTESIAN_POINT('Ctrl Pts',(6.66147559423329,-2.19459632208125,
83.1249892092792));
#140734=CARTESIAN_POINT('Ctrl Pts',(6.59930940225604,-2.36785598713161,
83.1166079088745));
#140735=CARTESIAN_POINT('Ctrl Pts',(6.53722199682675,-2.54089607091964,
83.1082372305411));
#140736=CARTESIAN_POINT('Ctrl Pts',(6.46825985455144,-2.71167320878719,
83.0998665522077));
#140737=CARTESIAN_POINT('Ctrl Pts',(6.3926051907949,-2.87962244697497,83.0914958738744));
#140738=CARTESIAN_POINT('Ctrl Pts',(6.31703638209181,-3.04738109161432,
83.0831346948237));
#140739=CARTESIAN_POINT('Ctrl Pts',(6.23479032305727,-3.21231793589975,
83.074773515773));
#140740=CARTESIAN_POINT('Ctrl Pts',(6.14609825809439,-3.37388541067255,
83.0664123367223));
#140741=CARTESIAN_POINT('Ctrl Pts',(6.05752128154834,-3.53524323258756,
83.0580620072877));
#140742=CARTESIAN_POINT('Ctrl Pts',(5.96251513978702,-3.6932401198509,83.0497116778531));
#140743=CARTESIAN_POINT('Ctrl Pts',(5.86135813000353,-3.8473507033206,83.0413613484186));
#140744=CARTESIAN_POINT('Ctrl Pts',(5.76027895448811,-4.00134270791484,
83.033017444063));
#140745=CARTESIAN_POINT('Ctrl Pts',(5.65305852144119,-4.15145409504481,
83.0246735397075));
#140746=CARTESIAN_POINT('Ctrl Pts',(5.54002036745714,-4.29718522880502,
83.0163296353519));
#140747=CARTESIAN_POINT('Ctrl Pts',(5.4270730064231,-4.44279931041004,83.0079924328723));
#140748=CARTESIAN_POINT('Ctrl Pts',(5.30831744397997,-4.58403989713977,
82.9996552303928));
#140749=CARTESIAN_POINT('Ctrl Pts',(5.18411981592423,-4.72043729930202,
82.9913180279132));
#140750=CARTESIAN_POINT('Ctrl Pts',(5.14323464230844,-4.76533857121394,
82.9885734668762));
#140751=CARTESIAN_POINT('Ctrl Pts',(5.10176005521895,-4.80971524125113,
82.9858289058393));
#140752=CARTESIAN_POINT('Ctrl Pts',(5.05971009278301,-4.85355131213112,
82.9830843448023));
#140753=CARTESIAN_POINT('Ctrl Pts',(4.93195719158826,-4.98673062805631,
82.9747460345002));
#140754=CARTESIAN_POINT('Ctrl Pts',(4.79899544814047,-5.11480822757893,
82.9664077241982));
#140755=CARTESIAN_POINT('Ctrl Pts',(4.66126818529817,-5.23738536554521,
82.9580694138962));
#140756=CARTESIAN_POINT('Ctrl Pts',(4.52345426913576,-5.36003962488714,
82.9497258574123));
#140757=CARTESIAN_POINT('Ctrl Pts',(4.38086909784444,-5.4771863020379,82.9413823009283));
#140758=CARTESIAN_POINT('Ctrl Pts',(4.2339887527602,-5.58846721418316,82.9330387444444));
#140759=CARTESIAN_POINT('Ctrl Pts',(4.08699666174867,-5.69983278836207,
82.924688840219));
#140760=CARTESIAN_POINT('Ctrl Pts',(3.93570313971617,-5.80532349836861,
82.9163389359937));
#140761=CARTESIAN_POINT('Ctrl Pts',(3.78061323339439,-5.90462447086885,
82.9079890317683));
#140762=CARTESIAN_POINT('Ctrl Pts',(3.62529070369067,-6.004074387479,82.8996266033045));
#140763=CARTESIAN_POINT('Ctrl Pts',(3.46616068687968,-6.09731583710534,
82.8912641748407));
#140764=CARTESIAN_POINT('Ctrl Pts',(3.30375413931725,-6.18407916746254,
82.882901746377));
#140765=CARTESIAN_POINT('Ctrl Pts',(3.14120871201725,-6.27091669229485,
82.8745321668969));
#140766=CARTESIAN_POINT('Ctrl Pts',(2.97538145765003,-6.35126490224367,
82.8661625874168));
#140767=CARTESIAN_POINT('Ctrl Pts',(2.80682380791828,-6.4249020750361,82.8577930079367));
#140768=CARTESIAN_POINT('Ctrl Pts',(2.63800617854858,-6.49865282419573,
82.8494105194));
#140769=CARTESIAN_POINT('Ctrl Pts',(2.4664500429742,-6.56567173290775,82.8410280308633));
#140770=CARTESIAN_POINT('Ctrl Pts',(2.29272383290536,-6.62578629209604,
82.8326455423266));
#140771=CARTESIAN_POINT('Ctrl Pts',(2.23587777031499,-6.64545676089206,
82.829902654723));
#140772=CARTESIAN_POINT('Ctrl Pts',(2.1787994510767,-6.66438838201942,82.8271597671194));
#140773=CARTESIAN_POINT('Ctrl Pts',(2.12150903618854,-6.68257629749712,
82.8244168795158));
#140774=CARTESIAN_POINT('Ctrl Pts',(1.94627098386147,-6.7382089000961,82.816027024383));
#140775=CARTESIAN_POINT('Ctrl Pts',(1.7686938955959,-6.78699188517118,82.8076371692502));
#140776=CARTESIAN_POINT('Ctrl Pts',(1.58933985197956,-6.82873527070786,
82.7992473141174));
#140777=CARTESIAN_POINT('Ctrl Pts',(1.41015131376029,-6.87044013603358,
82.7908652010253));
#140778=CARTESIAN_POINT('Ctrl Pts',(1.22918940765217,-6.9051182775189,82.7824830879332));
#140779=CARTESIAN_POINT('Ctrl Pts',(1.04703124785321,-6.93262952482815,
82.7741009748411));
#140780=CARTESIAN_POINT('Ctrl Pts',(0.865014404179149,-6.9601194292403,
82.7657253644923));
#140781=CARTESIAN_POINT('Ctrl Pts',(0.681803480916146,-6.98045347548987,
82.7573497541434));
#140782=CARTESIAN_POINT('Ctrl Pts',(0.497986110754797,-6.99354247831493,
82.7489741437946));
#140783=CARTESIAN_POINT('Ctrl Pts',(0.314284364449178,-7.00662324796282,
82.740603801829));
#140784=CARTESIAN_POINT('Ctrl Pts',(0.129977258901961,-7.01246803762564,
82.7322334598635));
#140785=CARTESIAN_POINT('Ctrl Pts',(-0.0543416578249555,-7.01103940558922,
82.7238631178979));
#140786=CARTESIAN_POINT('Ctrl Pts',(-0.238571654299908,-7.00961146276215,
82.7154968140035));
#140787=CARTESIAN_POINT('Ctrl Pts',(-0.422813122463965,-7.00091709807069,
82.7071305101092));
#140788=CARTESIAN_POINT('Ctrl Pts',(-0.606471251804374,-6.9849709507796,
82.6987642062149));
#140789=CARTESIAN_POINT('Ctrl Pts',(-0.790078017113542,-6.96902926317897,
82.6904002421413));
#140790=CARTESIAN_POINT('Ctrl Pts',(-0.973101441646077,-6.94583986398626,
82.6820362780676));
#140791=CARTESIAN_POINT('Ctrl Pts',(-1.15495001680282,-6.91546939991691,
82.673672313994));
#140792=CARTESIAN_POINT('Ctrl Pts',(-1.3367706084858,-6.88510360935729,
82.6653096369955));
#140793=CARTESIAN_POINT('Ctrl Pts',(-1.51741638717774,-6.84755901128638,
82.6569469599969));
#140794=CARTESIAN_POINT('Ctrl Pts',(-1.69630382237394,-6.80295376323399,
82.6485842829984));
#140795=CARTESIAN_POINT('Ctrl Pts',(-1.8751875746048,-6.75834943352214,
82.6402217781721));
#140796=CARTESIAN_POINT('Ctrl Pts',(-2.05231273673736,-6.70668482359197,
82.6318592733458));
#140797=CARTESIAN_POINT('Ctrl Pts',(-2.22710835418838,-6.64812867965147,
82.6234967685195));
#140798=CARTESIAN_POINT('Ctrl Pts',(-2.4019236719289,-6.58956593615769,
82.6151333211995));
#140799=CARTESIAN_POINT('Ctrl Pts',(-2.5744086100923,-6.52411021501969,
82.6067698738795));
#140800=CARTESIAN_POINT('Ctrl Pts',(-2.74400928376417,-6.45197951121329,
82.5984064265595));
#140801=CARTESIAN_POINT('Ctrl Pts',(-2.91370982307877,-6.37980633482149,
82.5900380546067));
#140802=CARTESIAN_POINT('Ctrl Pts',(-3.08052240108897,-6.3009504497292,
82.5816696826539));
#140803=CARTESIAN_POINT('Ctrl Pts',(-3.24391401049085,-6.21567763442098,
82.5733013107011));
#140804=CARTESIAN_POINT('Ctrl Pts',(-3.4073545762892,-6.13037926914866,
82.5649304313653));
#140805=CARTESIAN_POINT('Ctrl Pts',(-3.56737184065762,-6.03866029666515,
82.5565595520296));
#140806=CARTESIAN_POINT('Ctrl Pts',(-3.72345854630218,-5.94083184549683,
82.5481886726938));
#140807=CARTESIAN_POINT('Ctrl Pts',(-3.87967750252453,-5.84292050533974,
82.5398107008025));
#140808=CARTESIAN_POINT('Ctrl Pts',(-4.03195896960849,-5.73888952217245,
82.5314327289113));
#140809=CARTESIAN_POINT('Ctrl Pts',(-4.17982480036541,-5.62909328406896,
82.52305475702));
#140810=CARTESIAN_POINT('Ctrl Pts',(-4.27379473988789,-5.55931688067971,
82.5177304876609));
#140811=CARTESIAN_POINT('Ctrl Pts',(-4.36598195812697,-5.4872129053503,
82.5124062183019));
#140812=CARTESIAN_POINT('Ctrl Pts',(-4.45627082729111,-5.41288064493706,
82.5070819489429));
#140813=CARTESIAN_POINT('Ctrl Pts',(-4.58960858476191,-5.30310745802053,
82.4992191177537));
#140814=CARTESIAN_POINT('Ctrl Pts',(-4.71908165106739,-5.18824423112896,
82.4913562865645));
#140815=CARTESIAN_POINT('Ctrl Pts',(-4.84426095490327,-5.06860556398894,
82.4834934553753));
#140816=CARTESIAN_POINT('Ctrl Pts',(-4.96934407496756,-4.94905882337256,
82.4756366657339));
#140817=CARTESIAN_POINT('Ctrl Pts',(-5.09013971962647,-4.82474420115755,
82.4677798760926));
#140818=CARTESIAN_POINT('Ctrl Pts',(-5.20625085837433,-4.69601730854738,
82.4599230864513));
#140819=CARTESIAN_POINT('Ctrl Pts',(-5.32229651593641,-4.56736301181096,
82.4520707276674));
#140820=CARTESIAN_POINT('Ctrl Pts',(-5.43366266823845,-4.4343016767349,
82.4442183688835));
#140821=CARTESIAN_POINT('Ctrl Pts',(-5.53998841533241,-4.29722642183102,
82.4363660100996));
#140822=CARTESIAN_POINT('Ctrl Pts',(-5.64628905767686,-4.16018353199426,
82.4285155053493));
#140823=CARTESIAN_POINT('Ctrl Pts',(-5.7475514233018,-4.01912890440158,
82.4206650005989));
#140824=CARTESIAN_POINT('Ctrl Pts',(-5.84345432266771,-3.87448940395971,
82.4128144958486));
#140825=CARTESIAN_POINT('Ctrl Pts',(-5.93934179427969,-3.72987317145484,
82.404965253997));
#140826=CARTESIAN_POINT('Ctrl Pts',(-6.02987130762786,-3.58167353377094,
82.3971160121454));
#140827=CARTESIAN_POINT('Ctrl Pts',(-6.11476478557853,-3.43034665588608,
82.3892667702939));
#140828=CARTESIAN_POINT('Ctrl Pts',(-6.19968686580361,-3.27896879301399,
82.3814148838791));
#140829=CARTESIAN_POINT('Ctrl Pts',(-6.27896893088145,-3.12446191841869,
82.3735629974643));
#140830=CARTESIAN_POINT('Ctrl Pts',(-6.35237860284588,-2.96730730606147,
82.3657111110495));
#140831=CARTESIAN_POINT('Ctrl Pts',(-6.40628241126132,-2.85191063026364,
82.3599455685852));
#140832=CARTESIAN_POINT('Ctrl Pts',(-6.45702090176905,-2.73508688813753,
82.3541800261209));
#140833=CARTESIAN_POINT('Ctrl Pts',(-6.50451862268203,-2.61703344450977,
82.3484144836566));
#140834=CARTESIAN_POINT('Ctrl Pts',(-6.58406099959887,-2.41933445329764,
82.3387591792965));
#140835=CARTESIAN_POINT('Ctrl Pts',(-6.65447352736375,-2.21828741596851,
82.3291038749364));
#140836=CARTESIAN_POINT('Ctrl Pts',(-6.7155581905773,-2.01467236826988,
82.3194485705763));
#140837=CARTESIAN_POINT('Ctrl Pts',(-6.77698125136581,-1.80992933140435,
82.3097397776413));
#140838=CARTESIAN_POINT('Ctrl Pts',(-6.82897285094932,-1.60258981367787,
82.3000309847063));
#140839=CARTESIAN_POINT('Ctrl Pts',(-6.87138419481227,-1.39345104319605,
82.2903221917714));
#140840=CARTESIAN_POINT('Ctrl Pts',(-6.91399962566314,-1.18330587919221,
82.2805666793004));
#140841=CARTESIAN_POINT('Ctrl Pts',(-6.94694239186077,-0.971344151625883,
82.2708111668294));
#140842=CARTESIAN_POINT('Ctrl Pts',(-6.97011401132134,-0.75837802689812,
82.2610556543585));
#140843=CARTESIAN_POINT('Ctrl Pts',(-6.99330857425006,-0.545201032942771,
82.2512904824293));
#140844=CARTESIAN_POINT('Ctrl Pts',(-7.00671264531918,-0.331017691907905,
82.2415253105001));
#140845=CARTESIAN_POINT('Ctrl Pts',(-7.01027962605566,-0.116645304273289,
82.231760138571));
#140846=CARTESIAN_POINT('Ctrl Pts',(-7.01384174329482,0.0974347914741832,
82.2220082812322));
#140847=CARTESIAN_POINT('Ctrl Pts',(-7.00759357667754,0.311703380708535,
82.2122564238934));
#140848=CARTESIAN_POINT('Ctrl Pts',(-6.9915405923592,0.525344370764156,
82.2025045665546));
#140849=CARTESIAN_POINT('Ctrl Pts',(-6.98454032858611,0.618507315016503,
82.1982520504931));
#140850=CARTESIAN_POINT('Ctrl Pts',(-6.97567625541477,0.711550891526119,
82.1939995344316));
#140851=CARTESIAN_POINT('Ctrl Pts',(-6.96495193175312,0.804407328950017,
82.1897470183701));
#140852=CARTESIAN_POINT('Ctrl Pts',(-6.9446935765245,0.97981407290384,82.1817139727713));
#140853=CARTESIAN_POINT('Ctrl Pts',(-6.91778355046248,1.15463820249654,
82.1736809271726));
#140854=CARTESIAN_POINT('Ctrl Pts',(-6.88426944093054,1.32833008968777,
82.1656478815738));
#140855=CARTESIAN_POINT('Ctrl Pts',(-6.85077687555863,1.5019103210461,82.1576199999261));
#140856=CARTESIAN_POINT('Ctrl Pts',(-6.81068874636665,1.67435940037502,
82.1495921182784));
#140857=CARTESIAN_POINT('Ctrl Pts',(-6.7641043335017,1.84513390516882,82.1415642366307));
#140858=CARTESIAN_POINT('Ctrl Pts',(-6.71754095395832,2.01583130359044,
82.1335399796506));
#140859=CARTESIAN_POINT('Ctrl Pts',(-6.66448722722162,2.18485528001888,
82.1255157226706));
#140860=CARTESIAN_POINT('Ctrl Pts',(-6.60509328167742,2.35167372372101,
82.1174914656906));
#140861=CARTESIAN_POINT('Ctrl Pts',(-6.54570651746624,2.51847199737403,
82.109468178925));
#140862=CARTESIAN_POINT('Ctrl Pts',(-6.4799811769958,2.68306492174575,82.1014448921593));
#140863=CARTESIAN_POINT('Ctrl Pts',(-6.40811696211129,2.84493647774456,
82.0934216053937));
#140864=CARTESIAN_POINT('Ctrl Pts',(-6.33625863585807,3.00679476981344,
82.0853989760649));
#140865=CARTESIAN_POINT('Ctrl Pts',(-6.25826258961516,3.16593180421338,
82.077376346736));
#140866=CARTESIAN_POINT('Ctrl Pts',(-6.17437616391519,3.32185272836952,
82.0693537174072));
#140867=CARTESIAN_POINT('Ctrl Pts',(-6.09045820289127,3.47783226769267,
82.0613280721408));
#140868=CARTESIAN_POINT('Ctrl Pts',(-6.00064561528805,3.63059295992614,
82.0533024268745));
#140869=CARTESIAN_POINT('Ctrl Pts',(-5.90523126755091,3.7796653607481,82.0452767816082));
#140870=CARTESIAN_POINT('Ctrl Pts',(-5.84896915385632,3.86756753230491,
82.0405443721));
#140871=CARTESIAN_POINT('Ctrl Pts',(-5.79076015133523,3.9541878003552,82.0358119625919));
#140872=CARTESIAN_POINT('Ctrl Pts',(-5.73067125139156,4.03943480835801,
82.0310795530837));
#140873=CARTESIAN_POINT('Ctrl Pts',(-5.61982306083956,4.19669308061698,
82.022349504249));
#140874=CARTESIAN_POINT('Ctrl Pts',(-5.50252001517792,4.34935516522828,
82.0136194554144));
#140875=CARTESIAN_POINT('Ctrl Pts',(-5.37916323089427,4.49691333004041,
82.0048894065797));
#140876=CARTESIAN_POINT('Ctrl Pts',(-5.25577077784271,4.6445141614798,81.9961568334405));
#140877=CARTESIAN_POINT('Ctrl Pts',(-5.1263212678867,4.78700791716026,81.9874242603013));
#140878=CARTESIAN_POINT('Ctrl Pts',(-4.99125530779243,4.92392089852527,
81.9786916871622));
#140879=CARTESIAN_POINT('Ctrl Pts',(-4.85427052012951,5.06277894734448,
81.9698350538818));
#140880=CARTESIAN_POINT('Ctrl Pts',(-4.71150868835908,5.195896239379,81.9609784206014));
#140881=CARTESIAN_POINT('Ctrl Pts',(-4.56346755050045,5.32281790765281,
81.9521217873209));
#140882=CARTESIAN_POINT('Ctrl Pts',(-4.41740719337723,5.44804137231201,
81.9433836552142));
#140883=CARTESIAN_POINT('Ctrl Pts',(-4.26620815229866,5.56723381446002,
81.9346455231074));
#140884=CARTESIAN_POINT('Ctrl Pts',(-4.11038189632247,5.67999887578198,
81.9259073910006));
#140885=CARTESIAN_POINT('Ctrl Pts',(-3.95138581057193,5.79505781271974,
81.9169915071334));
#140886=CARTESIAN_POINT('Ctrl Pts',(-3.78757247686647,5.90342489858673,
81.9080756232662));
#140887=CARTESIAN_POINT('Ctrl Pts',(-3.61951728623384,6.00472490436943,
81.899159739399));
#140888=CARTESIAN_POINT('Ctrl Pts',(-3.45146209560133,6.10602491015205,
81.8902438555318));
#140889=CARTESIAN_POINT('Ctrl Pts',(-3.27916531018032,6.20025768494158,
81.8813279716645));
#140890=CARTESIAN_POINT('Ctrl Pts',(-3.10323089411647,6.28709667337008,
81.8724120877973));
#140891=CARTESIAN_POINT('Ctrl Pts',(-2.93075363378354,6.37222925373341,
81.863671403301));
#140892=CARTESIAN_POINT('Ctrl Pts',(-2.7547620577083,6.45026497194727,81.8549307188046));
#140893=CARTESIAN_POINT('Ctrl Pts',(-2.57584628362454,6.52093877333913,
81.8461900343083));
#140894=CARTESIAN_POINT('Ctrl Pts',(-2.39696269946052,6.59159985934016,
81.8374509224062));
#140895=CARTESIAN_POINT('Ctrl Pts',(-2.21515622252979,6.65490157315621,
81.8287118105042));
#140896=CARTESIAN_POINT('Ctrl Pts',(-2.03103635225847,6.71062723583307,
81.8199726986022));
#140897=CARTESIAN_POINT('Ctrl Pts',(-1.84453094407761,6.76707490467175,
81.8111203589279));
#140898=CARTESIAN_POINT('Ctrl Pts',(-1.65565204426987,6.8157487324728,81.8022680192536));
#140899=CARTESIAN_POINT('Ctrl Pts',(-1.46504971956045,6.85647547080246,
81.7934156795793));
#140900=CARTESIAN_POINT('Ctrl Pts',(-1.27698177935366,6.89666067736108,
81.7846810469294));
#140901=CARTESIAN_POINT('Ctrl Pts',(-1.08723623904894,6.92910877721177,
81.7759464142796));
#140902=CARTESIAN_POINT('Ctrl Pts',(-0.89644950239847,6.95370439781197,
81.7672117816297));
#140903=CARTESIAN_POINT('Ctrl Pts',(-0.701806231655992,6.97879719054806,
81.7583005884432));
#140904=CARTESIAN_POINT('Ctrl Pts',(-0.506079508305626,6.99571660669627,
81.7493893952567));
#140905=CARTESIAN_POINT('Ctrl Pts',(-0.309953463710748,7.00439543521307,
81.7404782020702));
#140906=CARTESIAN_POINT('Ctrl Pts',(-0.113827419115738,7.01307426372988,
81.7315670088837));
#140907=CARTESIAN_POINT('Ctrl Pts',(0.0826976444860204,7.01351247775365,
81.7226558156972));
#140908=CARTESIAN_POINT('Ctrl Pts',(0.278933644379903,7.00569929304227,
81.7137446225107));
#140909=CARTESIAN_POINT('Ctrl Pts',(0.455669164993112,6.99866252472066,
81.7057189576585));
#140910=CARTESIAN_POINT('Ctrl Pts',(0.632251418387597,6.98492904811944,
81.6976932928062));
#140911=CARTESIAN_POINT('Ctrl Pts',(0.808128137561514,6.96452119501272,
81.6896676279539));
#140912=CARTESIAN_POINT('Ctrl Pts',(0.983949037778691,6.94411981885801,
81.6816445102508));
#140913=CARTESIAN_POINT('Ctrl Pts',(1.15906448588315,6.91704832570235,81.6736213925477));
#140914=CARTESIAN_POINT('Ctrl Pts',(1.33292641379869,6.88338098160328,81.6655982748446));
#140915=CARTESIAN_POINT('Ctrl Pts',(1.50676641620335,6.84971788325099,81.6575761689269));
#140916=CARTESIAN_POINT('Ctrl Pts',(1.67935285362559,6.80946066104508,81.6495540630091));
#140917=CARTESIAN_POINT('Ctrl Pts',(1.85014699148782,6.76273485155145,81.6415319570914));
#140918=CARTESIAN_POINT('Ctrl Pts',(2.02100459702882,6.71599167858911,81.633506870132));
#140919=CARTESIAN_POINT('Ctrl Pts',(2.1900682178033,6.66277521033667,81.6254817831726));
#140920=CARTESIAN_POINT('Ctrl Pts',(2.35681301311548,6.60326123848735,81.6174566962132));
#140921=CARTESIAN_POINT('Ctrl Pts',(2.52359064798068,6.5437355456591,81.6094300287531));
#140922=CARTESIAN_POINT('Ctrl Pts',(2.68804820532863,6.4779100099437,81.601403361293));
#140923=CARTESIAN_POINT('Ctrl Pts',(2.84968022415902,6.40600883409764,81.5933766938328));
#140924=CARTESIAN_POINT('Ctrl Pts',(3.01144200060452,6.334049936241,81.5853435825924));
#140925=CARTESIAN_POINT('Ctrl Pts',(3.17037337702122,6.25600581411277,81.5773104713519));
#140926=CARTESIAN_POINT('Ctrl Pts',(3.32599236705278,6.17214722254797,81.5692773601114));
#140927=CARTESIAN_POINT('Ctrl Pts',(3.41768872916274,6.1227346940603,81.5645439591491));
#140928=CARTESIAN_POINT('Ctrl Pts',(3.50823552402975,6.07130424261146,81.5598105581867));
#140929=CARTESIAN_POINT('Ctrl Pts',(3.59753882558452,6.01791832454645,81.5550771572244));
#140930=CARTESIAN_POINT('Ctrl Pts',(3.78150640606667,5.90794167186676,81.54532620393));
#140931=CARTESIAN_POINT('Ctrl Pts',(3.96030414582843,5.78960001109624,81.5355752506356));
#140932=CARTESIAN_POINT('Ctrl Pts',(4.13326669073003,5.66336764000022,81.5258242973412));
#140933=CARTESIAN_POINT('Ctrl Pts',(4.30647842062453,5.53695340749303,81.5160592959694));
#140934=CARTESIAN_POINT('Ctrl Pts',(4.47383810859282,5.40262574799317,81.5062942945975));
#140935=CARTESIAN_POINT('Ctrl Pts',(4.6347107770697,5.26090130827542,81.4965292932257));
#140936=CARTESIAN_POINT('Ctrl Pts',(4.79531530414036,5.11941309383397,81.4867805680879));
#140937=CARTESIAN_POINT('Ctrl Pts',(4.94945439310547,4.97055276469821,81.4770318429501));
#140938=CARTESIAN_POINT('Ctrl Pts',(5.09652968089175,4.81487401437353,81.4672831178123));
#140939=CARTESIAN_POINT('Ctrl Pts',(5.24320130404137,4.65962254185419,81.4575611491449));
#140940=CARTESIAN_POINT('Ctrl Pts',(5.38284780235387,4.49759003646098,81.4478391804775));
#140941=CARTESIAN_POINT('Ctrl Pts',(5.5149095323348,4.32936478165825,81.4381172118101));
#140942=CARTESIAN_POINT('Ctrl Pts',(5.64609744434046,4.1622526294293,81.4284595708702));
#140943=CARTESIAN_POINT('Ctrl Pts',(5.76980057758359,3.98902942740854,81.4188019299304));
#140944=CARTESIAN_POINT('Ctrl Pts',(5.88550441451674,3.81031026941429,81.4091442889905));
#140945=CARTESIAN_POINT('Ctrl Pts',(5.93636023427466,3.73175704657265,81.4048994233063));
#140946=CARTESIAN_POINT('Ctrl Pts',(5.98567111524841,3.65214255661752,81.4006545576221));
#140947=CARTESIAN_POINT('Ctrl Pts',(6.03339552127373,3.5715213910005,81.3964096919379));
#140948=CARTESIAN_POINT('Ctrl Pts',(6.12167101984821,3.42239698729973,81.3885579937008));
#140949=CARTESIAN_POINT('Ctrl Pts',(6.20447908329652,3.26988769268964,81.3807062954638));
#140950=CARTESIAN_POINT('Ctrl Pts',(6.28154580695363,3.11445161106145,81.3728545972267));
#140951=CARTESIAN_POINT('Ctrl Pts',(6.35859173350429,2.95905747517305,81.3650050178368));
#140952=CARTESIAN_POINT('Ctrl Pts',(6.42989923199527,2.80073846428882,81.3571554384468));
#140953=CARTESIAN_POINT('Ctrl Pts',(6.49524019261651,2.63997753829821,81.3493058590569));
#140954=CARTESIAN_POINT('Ctrl Pts',(6.52149691725951,2.57537708971348,81.3461515704966));
#140955=CARTESIAN_POINT('Ctrl Pts',(6.546790714195,2.5103825853856,81.3429972819363));
#140956=CARTESIAN_POINT('Ctrl Pts',(6.57110895151812,2.4450263208764,81.339842993376));
#140957=CARTESIAN_POINT('Origin',(0.,0.,50.));
#140958=CARTESIAN_POINT('',(6.57110895151812,2.44502632087641,79.3399816340719));
#140959=CARTESIAN_POINT('',(6.57110895151811,2.44502632087644,79.8868028110482));
#140960=CARTESIAN_POINT('',(6.57110895151814,2.44502632087636,50.));
#140961=CARTESIAN_POINT('',(7.01124984869581,0.00145659295747845,81.7735343568707));
#140962=CARTESIAN_POINT('Ctrl Pts',(6.57110895151811,2.44502632087645,79.8868028110482));
#140963=CARTESIAN_POINT('Ctrl Pts',(6.50601242163503,2.61997592635723,79.8952869682238));
#140964=CARTESIAN_POINT('Ctrl Pts',(6.43396319980227,2.79222176291496,79.9037711253993));
#140965=CARTESIAN_POINT('Ctrl Pts',(6.35522177652277,2.96121305105033,79.9122552825748));
#140966=CARTESIAN_POINT('Ctrl Pts',(6.27637096155742,3.13043911068377,79.9207512263834));
#140967=CARTESIAN_POINT('Ctrl Pts',(6.19080949862361,3.2964013010892,79.9292471701919));
#140968=CARTESIAN_POINT('Ctrl Pts',(6.09884419442367,3.45857283494864,79.9377431140004));
#140969=CARTESIAN_POINT('Ctrl Pts',(6.01888259155763,3.59957705278337,79.9451301312097));
#140970=CARTESIAN_POINT('Ctrl Pts',(5.93408053615291,3.73771588754854,79.9525171484191));
#140971=CARTESIAN_POINT('Ctrl Pts',(5.84466588621368,3.87266151903701,79.9599041656285));
#140972=CARTESIAN_POINT('Ctrl Pts',(5.74321613721439,4.02577066225192,79.9682854660334));
#140973=CARTESIAN_POINT('Ctrl Pts',(5.63562818842432,4.17506946424814,79.9766667664383));
#140974=CARTESIAN_POINT('Ctrl Pts',(5.52220866352461,4.32005069866012,79.9850480668433));
#140975=CARTESIAN_POINT('Ctrl Pts',(5.40893288126937,4.46484819058109,79.9934187451769));
#140976=CARTESIAN_POINT('Ctrl Pts',(5.28984045198937,4.60533876384297,80.0017894235105));
#140977=CARTESIAN_POINT('Ctrl Pts',(5.165281750719,4.74104323943468,80.0101601018441));
#140978=CARTESIAN_POINT('Ctrl Pts',(5.04086440218849,4.87659371374634,80.0185212808949));
#140979=CARTESIAN_POINT('Ctrl Pts',(4.91099336569956,5.00736867584645,80.0268824599458));
#140980=CARTESIAN_POINT('Ctrl Pts',(4.77606010814264,5.13292084547468,80.0352436389967));
#140981=CARTESIAN_POINT('Ctrl Pts',(4.64130194240444,5.2583100963524,80.0435939684315));
#140982=CARTESIAN_POINT('Ctrl Pts',(4.50149489656413,5.37848985043892,80.0519442978662));
#140983=CARTESIAN_POINT('Ctrl Pts',(4.35706814119611,5.49304867769019,80.060294627301));
#140984=CARTESIAN_POINT('Ctrl Pts',(4.21275251357704,5.60751935877656,80.0686385316568));
#140985=CARTESIAN_POINT('Ctrl Pts',(4.06382451569309,5.71637752914874,80.0769824360125));
#140986=CARTESIAN_POINT('Ctrl Pts',(3.91074819081436,5.81925039421249,80.0853263403683));
#140987=CARTESIAN_POINT('Ctrl Pts',(3.75779481779455,5.92204063114938,80.093663542848));
#140988=CARTESIAN_POINT('Ctrl Pts',(3.60070003406205,6.01885496829242,80.1020007453278));
#140989=CARTESIAN_POINT('Ctrl Pts',(3.43995892617383,6.10936241753074,80.1103379478075));
#140990=CARTESIAN_POINT('Ctrl Pts',(3.3870438407315,6.13915697022813,80.1130825088433));
#140991=CARTESIAN_POINT('Ctrl Pts',(3.33373384920756,6.1682683944196,80.1158270698792));
#140992=CARTESIAN_POINT('Ctrl Pts',(3.28004730242159,6.1966859091273,80.118571630915));
#140993=CARTESIAN_POINT('Ctrl Pts',(3.11694104233132,6.2830217757926,80.126909941217));
#140994=CARTESIAN_POINT('Ctrl Pts',(2.95049105754623,6.36287851805465,80.1352482515189));
#140995=CARTESIAN_POINT('Ctrl Pts',(2.78124344501291,6.43601673879681,80.1435865618209));
#140996=CARTESIAN_POINT('Ctrl Pts',(2.6118893476247,6.50920097562574,80.1519301183048));
#140997=CARTESIAN_POINT('Ctrl Pts',(2.43973441237396,6.57565812955311,80.1602736747887));
#140998=CARTESIAN_POINT('Ctrl Pts',(2.26534310331072,6.63519759967874,80.1686172312725));
#140999=CARTESIAN_POINT('Ctrl Pts',(2.09081911809993,6.69478236717365,80.1769671354978));
#141000=CARTESIAN_POINT('Ctrl Pts',(1.91405567501855,6.74743884726723,80.1853170397231));
#141001=CARTESIAN_POINT('Ctrl Pts',(1.73563114143768,6.79302665263222,80.1936669439483));
#141002=CARTESIAN_POINT('Ctrl Pts',(1.55693898425992,6.83868283633176,80.2020293724121));
#141003=CARTESIAN_POINT('Ctrl Pts',(1.37658107548468,6.87724907701494,80.2103918008758));
#141004=CARTESIAN_POINT('Ctrl Pts',(1.19514618438746,6.90863605644733,80.2187542293395));
#141005=CARTESIAN_POINT('Ctrl Pts',(1.0135561417248,6.94004987602587,80.2271238088195));
#141006=CARTESIAN_POINT('Ctrl Pts',(0.830887603208601,6.96427214199975,
80.2354933882996));
#141007=CARTESIAN_POINT('Ctrl Pts',(0.64773373001235,6.98126547106642,80.2438629677796));
#141008=CARTESIAN_POINT('Ctrl Pts',(0.464297364282296,6.9982850102727,80.2522454563162));
#141009=CARTESIAN_POINT('Ctrl Pts',(0.280374494561492,7.00805331469375,
80.2606279448528));
#141010=CARTESIAN_POINT('Ctrl Pts',(0.0965589714397479,7.01058506314092,
80.2690104333895));
#141011=CARTESIAN_POINT('Ctrl Pts',(0.0364115202877523,7.01141349271786,
80.2717533209934));
#141012=CARTESIAN_POINT('Ctrl Pts',(-0.0237244746587937,7.01146751427336,
80.2744962085974));
#141013=CARTESIAN_POINT('Ctrl Pts',(-0.0838283466075951,7.01074884522367,
80.2772390962014));
#141014=CARTESIAN_POINT('Ctrl Pts',(-0.267672109595901,7.00855060377677,
80.2856289513342));
#141015=CARTESIAN_POINT('Ctrl Pts',(-0.451586127756361,6.99911472365723,
80.2940188064669));
#141016=CARTESIAN_POINT('Ctrl Pts',(-0.634977094669979,6.98243730023725,
80.3024086615997));
#141017=CARTESIAN_POINT('Ctrl Pts',(-0.818198830970368,6.96577526650979,
80.3107907746918));
#141018=CARTESIAN_POINT('Ctrl Pts',(-1.0008981524198,6.94188504045496,80.3191728877839));
#141019=CARTESIAN_POINT('Ctrl Pts',(-1.18248311805108,6.910814730408,80.3275550008759));
#141020=CARTESIAN_POINT('Ctrl Pts',(-1.36392721223472,6.8797685243365,80.3359306112248));
#141021=CARTESIAN_POINT('Ctrl Pts',(-1.54425835130262,6.8415533948439,80.3443062215737));
#141022=CARTESIAN_POINT('Ctrl Pts',(-1.72289061495453,6.79626915972297,
80.3526818319225));
#141023=CARTESIAN_POINT('Ctrl Pts',(-1.9014105162599,6.75101340905842,80.3610521738881));
#141024=CARTESIAN_POINT('Ctrl Pts',(-2.07823335505137,6.69869749940276,
80.3694225158536));
#141025=CARTESIAN_POINT('Ctrl Pts',(-2.25278384019573,6.63947223293034,
80.3777928578192));
#141026=CARTESIAN_POINT('Ctrl Pts',(-2.42725011763388,6.58027553827103,
80.3861591617135));
#141027=CARTESIAN_POINT('Ctrl Pts',(-2.59944591677244,6.51417623927701,
80.3945254656078));
#141028=CARTESIAN_POINT('Ctrl Pts',(-2.76881109923561,6.44137498203992,
80.4028917695021));
#141029=CARTESIAN_POINT('Ctrl Pts',(-2.9381289150043,6.36859408527396,80.4112557335757));
#141030=CARTESIAN_POINT('Ctrl Pts',(-3.10461739037919,6.28911509603929,
80.4196196976493));
#141031=CARTESIAN_POINT('Ctrl Pts',(-3.26773585022894,6.20318700150403,
80.4279836617229));
#141032=CARTESIAN_POINT('Ctrl Pts',(-3.43082920885846,6.11727212987454,
80.4363463387215));
#141033=CARTESIAN_POINT('Ctrl Pts',(-3.59055329523153,6.02491028474506,
80.44470901572));
#141034=CARTESIAN_POINT('Ctrl Pts',(-3.7463911812716,5.92639685469936,80.4530716927186));
#141035=CARTESIAN_POINT('Ctrl Pts',(-3.90222585889429,5.82788545286521,
80.4614341975449));
#141036=CARTESIAN_POINT('Ctrl Pts',(-4.05417421814168,5.72322289460479,
80.4697967023711));
#141037=CARTESIAN_POINT('Ctrl Pts',(-4.20174715382017,5.61274865087188,
80.4781592071974));
#141038=CARTESIAN_POINT('Ctrl Pts',(-4.34933672166354,5.5022619561714,80.4865226545174));
#141039=CARTESIAN_POINT('Ctrl Pts',(-4.49254962001396,5.38596246748469,
80.4948861018374));
#141040=CARTESIAN_POINT('Ctrl Pts',(-4.63092841240748,5.2642310551169,80.5032495491573));
#141041=CARTESIAN_POINT('Ctrl Pts',(-4.76938868612286,5.14242796387245,
80.5116179211101));
#141042=CARTESIAN_POINT('Ctrl Pts',(-4.90300891832457,5.01518677422717,
80.5199862930629));
#141043=CARTESIAN_POINT('Ctrl Pts',(-5.03136649664168,4.88292716912424,
80.5283546650157));
#141044=CARTESIAN_POINT('Ctrl Pts',(-5.15976253424397,4.75062793558692,
80.5367255443515));
#141045=CARTESIAN_POINT('Ctrl Pts',(-5.28289254866523,4.61330752793419,
80.5450964236872));
#141046=CARTESIAN_POINT('Ctrl Pts',(-5.40037261364649,4.4714206015848,80.5534673030229));
#141047=CARTESIAN_POINT('Ctrl Pts',(-5.51795221821635,4.32941345597712,
80.5618452749142));
#141048=CARTESIAN_POINT('Ctrl Pts',(-5.62987210216362,4.182832317173,80.5702232468055));
#141049=CARTESIAN_POINT('Ctrl Pts',(-5.735789559204,4.03216377333887,80.5786012186967));
#141050=CARTESIAN_POINT('Ctrl Pts',(-5.80310096564505,3.93641268682976,
80.583925488056));
#141051=CARTESIAN_POINT('Ctrl Pts',(-5.86798902647246,3.83901142386068,
80.5892497574152));
#141052=CARTESIAN_POINT('Ctrl Pts',(-5.93037513265348,3.74009055351675,
80.5945740267744));
#141053=CARTESIAN_POINT('Ctrl Pts',(-6.02250635073442,3.5940051374472,80.6024368579636));
#141054=CARTESIAN_POINT('Ctrl Pts',(-6.1093702199643,3.44430041469925,80.6102996891528));
#141055=CARTESIAN_POINT('Ctrl Pts',(-6.19065813649915,3.29140978905649,
80.618162520342));
#141056=CARTESIAN_POINT('Ctrl Pts',(-6.27188359399999,3.13863663967828,
80.6260193099834));
#141057=CARTESIAN_POINT('Ctrl Pts',(-6.34754144108903,2.98268278996944,
80.6338760996247));
#141058=CARTESIAN_POINT('Ctrl Pts',(-6.41736637059734,2.82401052193974,
80.6417328892661));
#141059=CARTESIAN_POINT('Ctrl Pts',(-6.48715192215077,2.66542773755797,
80.64958524805));
#141060=CARTESIAN_POINT('Ctrl Pts',(-6.55111094658078,2.50412993235009,
80.6574376068339));
#141061=CARTESIAN_POINT('Ctrl Pts',(-6.60902421618718,2.34060365554517,
80.6652899656178));
#141062=CARTESIAN_POINT('Ctrl Pts',(-6.66692381179491,2.1771159892022,80.6731404703682));
#141063=CARTESIAN_POINT('Ctrl Pts',(-6.71878035852728,2.01140125473838,
80.6809909751185));
#141064=CARTESIAN_POINT('Ctrl Pts',(-6.76442292621371,1.84396557392331,
80.6888414798689));
#141065=CARTESIAN_POINT('Ctrl Pts',(-6.81005815144955,1.67655682823214,
80.6966907217205));
#141066=CARTESIAN_POINT('Ctrl Pts',(-6.849481290175,1.50742805619762,80.7045399635721));
#141067=CARTESIAN_POINT('Ctrl Pts',(-6.88257154375768,1.33709966253717,
80.7123892054236));
#141068=CARTESIAN_POINT('Ctrl Pts',(-6.91567294609449,1.16671388190697,
80.7202410918384));
#141069=CARTESIAN_POINT('Ctrl Pts',(-6.94243712858262,0.995128047188277,
80.7280929782533));
#141070=CARTESIAN_POINT('Ctrl Pts',(-6.96279456425622,0.822872054735126,
80.7359448646681));
#141071=CARTESIAN_POINT('Ctrl Pts',(-6.97774277588813,0.696386623498159,
80.7417104071323));
#141072=CARTESIAN_POINT('Ctrl Pts',(-6.9892376781195,0.569540069089464,
80.7474759495964));
#141073=CARTESIAN_POINT('Ctrl Pts',(-6.99726959917364,0.442543465639617,
80.7532414920606));
#141074=CARTESIAN_POINT('Ctrl Pts',(-7.01072030964118,0.229867751841124,
80.7628967964207));
#141075=CARTESIAN_POINT('Ctrl Pts',(-7.01445165797892,0.0168796950760844,
80.7725521007808));
#141076=CARTESIAN_POINT('Ctrl Pts',(-7.00852054169979,-0.195617941590344,
80.782207405141));
#141077=CARTESIAN_POINT('Ctrl Pts',(-7.00255656814913,-0.409292775300087,
80.7919161980759));
#141078=CARTESIAN_POINT('Ctrl Pts',(-6.98682283297508,-0.622471694557186,
80.8016249910109));
#141079=CARTESIAN_POINT('Ctrl Pts',(-6.96142836349325,-0.834351066669008,
80.8113337839458));
#141080=CARTESIAN_POINT('Ctrl Pts',(-6.93591169366798,-1.04725002031054,
80.8210892964168));
#141081=CARTESIAN_POINT('Ctrl Pts',(-6.90064111825457,-1.2588368495497,
80.8308448088877));
#141082=CARTESIAN_POINT('Ctrl Pts',(-6.85577812303943,-1.46830953485768,
80.8406003213587));
#141083=CARTESIAN_POINT('Ctrl Pts',(-6.81087070655703,-1.67798963035071,
80.8503654932878));
#141084=CARTESIAN_POINT('Ctrl Pts',(-6.7563518911193,-1.88555135962937,
80.860130665217));
#141085=CARTESIAN_POINT('Ctrl Pts',(-6.69243403458003,-2.09020411809346,
80.8698958371461));
#141086=CARTESIAN_POINT('Ctrl Pts',(-6.62860332858805,-2.29457783716434,
80.8796476944849));
#141087=CARTESIAN_POINT('Ctrl Pts',(-6.5553992061843,-2.49605047645186,
80.8893995518236));
#141088=CARTESIAN_POINT('Ctrl Pts',(-6.47308307805028,-2.69384892433839,
80.8991514091624));
#141089=CARTESIAN_POINT('Ctrl Pts',(-6.43718728457644,-2.78010337283751,
80.903403925224));
#141090=CARTESIAN_POINT('Ctrl Pts',(-6.39955940008401,-2.8656593266447,
80.9076564412856));
#141091=CARTESIAN_POINT('Ctrl Pts',(-6.36022408105774,-2.95045355856236,
80.9119089573472));
#141092=CARTESIAN_POINT('Ctrl Pts',(-6.28591926790672,-3.11063071524734,
80.9199420029459));
#141093=CARTESIAN_POINT('Ctrl Pts',(-6.20548203678863,-3.2681663545186,
80.9279750485447));
#141094=CARTESIAN_POINT('Ctrl Pts',(-6.11913013039224,-3.422553580271,80.9360080941434));
#141095=CARTESIAN_POINT('Ctrl Pts',(-6.03283373432616,-3.57684155997018,
80.9440359757911));
#141096=CARTESIAN_POINT('Ctrl Pts',(-5.94063040951043,-3.72798483622312,
80.9520638574389));
#141097=CARTESIAN_POINT('Ctrl Pts',(-5.84278502933152,-3.87549863417851,
80.9600917390866));
#141098=CARTESIAN_POINT('Ctrl Pts',(-5.74498382730625,-4.02294582820004,
80.9681159960666));
#141099=CARTESIAN_POINT('Ctrl Pts',(-5.64154584437271,-4.16676650200938,
80.9761402530466));
#141100=CARTESIAN_POINT('Ctrl Pts',(-5.5327806796164,-4.30650258490152,
80.9841645100267));
#141101=CARTESIAN_POINT('Ctrl Pts',(-5.42402866567635,-4.44622177227794,
80.9921877967923));
#141102=CARTESIAN_POINT('Ctrl Pts',(-5.30995097181349,-4.58185705860183,
81.0002110835579));
#141103=CARTESIAN_POINT('Ctrl Pts',(-5.1908992118005,-4.71298121526375,
81.0082343703235));
#141104=CARTESIAN_POINT('Ctrl Pts',(-5.07185720701735,-4.8440946274706,
81.0162569996524));
#141105=CARTESIAN_POINT('Ctrl Pts',(-4.9478421973795,-4.97069737756557,
81.0242796289812));
#141106=CARTESIAN_POINT('Ctrl Pts',(-4.81924438109398,-5.09239728986203,
81.03230225831));
#141107=CARTESIAN_POINT('Ctrl Pts',(-4.69059822118459,-5.21414295266153,
81.0403279035764));
#141108=CARTESIAN_POINT('Ctrl Pts',(-4.55736608151836,-5.33098184577353,
81.0483535488427));
#141109=CARTESIAN_POINT('Ctrl Pts',(-4.41997340705431,-5.44256021036357,
81.056379194109));
#141110=CARTESIAN_POINT('Ctrl Pts',(-4.33895831388655,-5.50835361338182,
81.0611116036171));
#141111=CARTESIAN_POINT('Ctrl Pts',(-4.25649724148683,-5.57231868471149,
81.0658440131253));
#141112=CARTESIAN_POINT('Ctrl Pts',(-4.17268247625876,-5.63438971982087,
81.0705764226334));
#141113=CARTESIAN_POINT('Ctrl Pts',(-4.01806631460807,-5.74889442757948,
81.0793064714681));
#141114=CARTESIAN_POINT('Ctrl Pts',(-3.85876470267636,-5.85700877924137,
81.0880365203028));
#141115=CARTESIAN_POINT('Ctrl Pts',(-3.695317882781,-5.95837665037206,81.0967665691375));
#141116=CARTESIAN_POINT('Ctrl Pts',(-3.53182380203384,-6.05977383214909,
81.1054991422767));
#141117=CARTESIAN_POINT('Ctrl Pts',(-3.36418235367307,-6.1544204952032,
81.1142317154159));
#141118=CARTESIAN_POINT('Ctrl Pts',(-3.19296058830227,-6.24200522621124,
81.122964288555));
#141119=CARTESIAN_POINT('Ctrl Pts',(-3.01930634443343,-6.33083423813458,
81.1318209218355));
#141120=CARTESIAN_POINT('Ctrl Pts',(-2.84196953804195,-6.41239900471871,
81.1406775551159));
#141121=CARTESIAN_POINT('Ctrl Pts',(-2.66156554982748,-6.4864239289821,
81.1495341883963));
#141122=CARTESIAN_POINT('Ctrl Pts',(-2.48357535516818,-6.55945840460365,
81.158272320503));
#141123=CARTESIAN_POINT('Ctrl Pts',(-2.30259981210271,-6.62515346606485,
81.1670104526098));
#141124=CARTESIAN_POINT('Ctrl Pts',(-2.11924896866071,-6.68329337761934,
81.1757485847166));
#141125=CARTESIAN_POINT('Ctrl Pts',(-1.93216838815308,-6.74261597576009,
81.1846644685838));
#141126=CARTESIAN_POINT('Ctrl Pts',(-1.74261511626696,-6.79407266353018,
81.1935803524511));
#141127=CARTESIAN_POINT('Ctrl Pts',(-1.55125325708558,-6.83748783508105,
81.2024962363183));
#141128=CARTESIAN_POINT('Ctrl Pts',(-1.35989139790407,-6.88090300663196,
81.2114121201855));
#141129=CARTESIAN_POINT('Ctrl Pts',(-1.1667212476906,-6.91627660098658,
81.2203280040528));
#141130=CARTESIAN_POINT('Ctrl Pts',(-0.972418757270449,-6.94348819564119,
81.22924388792));
#141131=CARTESIAN_POINT('Ctrl Pts',(-0.781934359883963,-6.97016507558495,
81.2379845724164));
#141132=CARTESIAN_POINT('Ctrl Pts',(-0.590341479405468,-6.98900058238748,
81.2467252569127));
#141133=CARTESIAN_POINT('Ctrl Pts',(-0.398283611584763,-6.99992833729339,
81.2554659414091));
#141134=CARTESIAN_POINT('Ctrl Pts',(-0.206260298165024,-7.01085412611466,
81.2642050533111));
#141135=CARTESIAN_POINT('Ctrl Pts',(-0.0137724377309688,-7.01387498880386,
81.2729441652131));
#141136=CARTESIAN_POINT('Ctrl Pts',(0.178533260358716,-7.0089765613423,
81.2816832771151));
#141137=CARTESIAN_POINT('Ctrl Pts',(0.373330555539247,-7.00401466770301,
81.2905356167893));
#141138=CARTESIAN_POINT('Ctrl Pts',(0.567940649624519,-6.99092682656626,
81.2993879564636));
#141139=CARTESIAN_POINT('Ctrl Pts',(0.76169195267159,-6.96975264494626,
81.3082402961379));
#141140=CARTESIAN_POINT('Ctrl Pts',(0.952867000153031,-6.94886001035272,
81.3169749287878));
#141141=CARTESIAN_POINT('Ctrl Pts',(1.1432056751845,-6.92009478765721,81.3257095614377));
#141142=CARTESIAN_POINT('Ctrl Pts',(1.33206753068949,-6.88354724369513,
81.3344441940876));
#141143=CARTESIAN_POINT('Ctrl Pts',(1.5247470110319,-6.84626093323517,81.343355387274));
#141144=CARTESIAN_POINT('Ctrl Pts',(1.71588904235505,-6.80087436321675,
81.3522665804605));
#141145=CARTESIAN_POINT('Ctrl Pts',(1.90482298408067,-6.7475385113253,81.361177773647));
#141146=CARTESIAN_POINT('Ctrl Pts',(2.09375692580615,-6.69420265943389,
81.3700889668335));
#141147=CARTESIAN_POINT('Ctrl Pts',(2.2804824825452,-6.63291759505681,81.37900016002));
#141148=CARTESIAN_POINT('Ctrl Pts',(2.46434297795493,-6.5638891100859,81.3879113532064));
#141149=CARTESIAN_POINT('Ctrl Pts',(2.62993277999947,-6.50172016435182,
81.3959370180587));
#141150=CARTESIAN_POINT('Ctrl Pts',(2.79327456229149,-6.43324124240426,
81.403962682911));
#141151=CARTESIAN_POINT('Ctrl Pts',(2.95385099394157,-6.35864693689549,
81.4119883477633));
#141152=CARTESIAN_POINT('Ctrl Pts',(3.11437646257088,-6.28407630578963,
81.4200114654664));
#141153=CARTESIAN_POINT('Ctrl Pts',(3.27213799583088,-6.20339430947099,
81.4280345831695));
#141154=CARTESIAN_POINT('Ctrl Pts',(3.42663855476052,-6.1168435305743,81.4360577008726));
#141155=CARTESIAN_POINT('Ctrl Pts',(3.58111962981761,-6.03030366648827,
81.4440798067903));
#141156=CARTESIAN_POINT('Ctrl Pts',(3.73234023025387,-5.93789667364881,
81.4521019127081));
#141157=CARTESIAN_POINT('Ctrl Pts',(3.87982827558596,-5.83991088240768,
81.4601240186258));
#141158=CARTESIAN_POINT('Ctrl Pts',(4.02737112797399,-5.74188867931549,
81.4681491055852));
#141159=CARTESIAN_POINT('Ctrl Pts',(4.17117834713499,-5.63828373696298,
81.4761741925446));
#141160=CARTESIAN_POINT('Ctrl Pts',(4.31080682206587,-5.52942773759911,
81.4841992795041));
#141161=CARTESIAN_POINT('Ctrl Pts',(4.45046279612595,-5.42055029959105,
81.4922259469642));
#141162=CARTESIAN_POINT('Ctrl Pts',(4.58593810276495,-5.30641997666109,
81.5002526144243));
#141163=CARTESIAN_POINT('Ctrl Pts',(4.71682322992565,-5.18740832980534,
81.5082792818844));
#141164=CARTESIAN_POINT('Ctrl Pts',(4.84781343120537,-5.06830114081873,
81.5163123931249));
#141165=CARTESIAN_POINT('Ctrl Pts',(4.97420582827055,-4.94430505470051,
81.5243455043654));
#141166=CARTESIAN_POINT('Ctrl Pts',(5.09562781225362,-4.81582846055457,
81.5323786156058));
#141167=CARTESIAN_POINT('Ctrl Pts',(5.16717405612213,-4.74012538410473,
81.5371120165682));
#141168=CARTESIAN_POINT('Ctrl Pts',(5.2369953112006,-4.66286733768816,81.5418454175305));
#141169=CARTESIAN_POINT('Ctrl Pts',(5.30502200952489,-4.58414310869072,
81.5465788184928));
#141170=CARTESIAN_POINT('Ctrl Pts',(5.44515912518696,-4.4219687469154,81.5563297717873));
#141171=CARTESIAN_POINT('Ctrl Pts',(5.57776152514571,-4.25347547125358,
81.5660807250817));
#141172=CARTESIAN_POINT('Ctrl Pts',(5.70234640900847,-4.07932249205284,
81.5758316783761));
#141173=CARTESIAN_POINT('Ctrl Pts',(5.82711078076822,-3.90491861281495,
81.585596679748));
#141174=CARTESIAN_POINT('Ctrl Pts',(5.94383450908284,-3.72483875133039,
81.5953616811198));
#141175=CARTESIAN_POINT('Ctrl Pts',(6.05207693009285,-3.53977278857526,
81.6051266824917));
#141176=CARTESIAN_POINT('Ctrl Pts',(6.16013893341424,-3.35501529243545,
81.6148754076296));
#141177=CARTESIAN_POINT('Ctrl Pts',(6.25974786357801,-3.16528833765755,
81.6246241327674));
#141178=CARTESIAN_POINT('Ctrl Pts',(6.35050945105486,-2.97130548321154,
81.6343728579052));
#141179=CARTESIAN_POINT('Ctrl Pts',(6.44102193316625,-2.77785503648549,
81.6440948265726));
#141180=CARTESIAN_POINT('Ctrl Pts',(6.52273553175952,-2.58017204505834,
81.6538167952399));
#141181=CARTESIAN_POINT('Ctrl Pts',(6.59530359895147,-2.37899075243218,
81.6635387639073));
#141182=CARTESIAN_POINT('Ctrl Pts',(6.6673915021967,-2.17914062387322,81.6731964048472));
#141183=CARTESIAN_POINT('Ctrl Pts',(6.73045445819763,-1.97583836989345,
81.6828540457871));
#141184=CARTESIAN_POINT('Ctrl Pts',(6.78419708066467,-1.7698295209429,81.6925116867271));
#141185=CARTESIAN_POINT('Ctrl Pts',(6.8078188134773,-1.67928153940495,81.6967565524112));
#141186=CARTESIAN_POINT('Ctrl Pts',(6.82964052972937,-1.58821100249732,
81.7010014180953));
#141187=CARTESIAN_POINT('Ctrl Pts',(6.8496399330534,-1.4966827820284,81.7052462837793));
#141188=CARTESIAN_POINT('Ctrl Pts',(6.88499295409772,-1.33488799985611,
81.7127499489352));
#141189=CARTESIAN_POINT('Ctrl Pts',(6.91464614817937,-1.17167025083209,
81.720253614091));
#141190=CARTESIAN_POINT('Ctrl Pts',(6.93848291677295,-1.00751246947618,
81.7277572792469));
#141191=CARTESIAN_POINT('Ctrl Pts',(6.9627194639257,-0.840601514549343,
81.7353867921842));
#141192=CARTESIAN_POINT('Ctrl Pts',(6.98094261072159,-0.672719122722579,
81.7430163051215));
#141193=CARTESIAN_POINT('Ctrl Pts',(6.99308397869138,-0.504383811665289,
81.7506458180588));
#141194=CARTESIAN_POINT('Ctrl Pts',(7.00522534666116,-0.336048500608132,
81.7582753309961));
#141195=CARTESIAN_POINT('Ctrl Pts',(7.01128489985528,-0.167260710844274,
81.7659048439334));
#141196=CARTESIAN_POINT('Ctrl Pts',(7.01124984869581,0.00145659295767842,
81.7735343568707));
#141197=CARTESIAN_POINT('Ctrl Pts',(7.01124984869562,0.00145659383634692,
81.7735343569104));
#141198=CARTESIAN_POINT('Ctrl Pts',(7.01121141547276,0.186453208018261,
81.7819000315001));
#141199=CARTESIAN_POINT('Ctrl Pts',(7.00384680112642,0.371311310975732,
81.7902657060898));
#141200=CARTESIAN_POINT('Ctrl Pts',(6.98921446351198,0.555434735621476,
81.7986313806795));
#141201=CARTESIAN_POINT('Ctrl Pts',(6.97456974963529,0.739713894767797,
81.8070041310889));
#141202=CARTESIAN_POINT('Ctrl Pts',(6.9526450844381,0.923256813954304,81.8153768814983));
#141203=CARTESIAN_POINT('Ctrl Pts',(6.92355038038384,1.10547577666217,81.8237496319077));
#141204=CARTESIAN_POINT('Ctrl Pts',(6.89440752844741,1.28799628762188,81.8321362381102));
#141205=CARTESIAN_POINT('Ctrl Pts',(6.85807098344372,1.46918814448923,81.8405228443127));
#141206=CARTESIAN_POINT('Ctrl Pts',(6.81470140780885,1.64847544261604,81.8489094505152));
#141207=CARTESIAN_POINT('Ctrl Pts',(6.78883754642808,1.75539513823684,81.8539108833654));
#141208=CARTESIAN_POINT('Ctrl Pts',(6.7604733779782,1.86163779181452,81.8589123162155));
#141209=CARTESIAN_POINT('Ctrl Pts',(6.72965120968403,1.96708443095315,81.8639137490656));
#141210=CARTESIAN_POINT('Ctrl Pts',(6.68257564105845,2.12813606267908,81.8715525787909));
#141211=CARTESIAN_POINT('Ctrl Pts',(6.62968735838444,2.28759443949406,81.8791914085162));
#141212=CARTESIAN_POINT('Ctrl Pts',(6.57110895151811,2.44502632087644,81.8868302382415));
#141213=CARTESIAN_POINT('',(7.01124960457286,-0.00235475623456128,81.2264656430635));
#141214=CARTESIAN_POINT('Ctrl Pts',(6.57110895151812,2.4450263208764,81.339842993376));
#141215=CARTESIAN_POINT('Ctrl Pts',(6.63162292022043,2.28239253733125,81.3319938011554));
#141216=CARTESIAN_POINT('Ctrl Pts',(6.68609251311296,2.11751758869187,81.3241446089348));
#141217=CARTESIAN_POINT('Ctrl Pts',(6.73435763417471,1.95091102245408,81.3162954167143));
#141218=CARTESIAN_POINT('Ctrl Pts',(6.78264982993078,1.78421099696964,81.3084418214284));
#141219=CARTESIAN_POINT('Ctrl Pts',(6.82473049864638,1.61577778120274,81.3005882261425));
#141220=CARTESIAN_POINT('Ctrl Pts',(6.86048993913609,1.44613428059516,81.2927346308566));
#141221=CARTESIAN_POINT('Ctrl Pts',(6.89626109718947,1.27643519163127,81.2848784621243));
#141222=CARTESIAN_POINT('Ctrl Pts',(6.92570683799432,1.10552540368255,81.277022293392));
#141223=CARTESIAN_POINT('Ctrl Pts',(6.94876907000676,0.933935208789922,
81.2691661246598));
#141224=CARTESIAN_POINT('Ctrl Pts',(6.97185266495945,0.762186066962772,
81.2613026786239));
#141225=CARTESIAN_POINT('Ctrl Pts',(6.98854091378289,0.589755639004955,
81.2534392325881));
#141226=CARTESIAN_POINT('Ctrl Pts',(6.9988277612455,0.41717685808219,81.2455757865522));
#141227=CARTESIAN_POINT('Ctrl Pts',(7.00224367819507,0.359869234436232,
81.2429645999187));
#141228=CARTESIAN_POINT('Ctrl Pts',(7.00495415094574,0.302545236695585,
81.2403534132851));
#141229=CARTESIAN_POINT('Ctrl Pts',(7.00696022589239,0.245224295823443,
81.2377422266515));
#141230=CARTESIAN_POINT('Ctrl Pts',(7.00984801535903,0.16270952759645,81.2339833654642));
#141231=CARTESIAN_POINT('Ctrl Pts',(7.01127732144654,0.0801718186302153,
81.2302245042769));
#141232=CARTESIAN_POINT('Ctrl Pts',(7.01124960457305,-0.00235475566470253,
81.2264656430895));
#141233=CARTESIAN_POINT('Ctrl Pts',(7.01124960457286,-0.00235475623456214,
81.2264656430635));
#141234=CARTESIAN_POINT('Ctrl Pts',(7.01118819206291,-0.185209537447951,
81.2181371047001));
#141235=CARTESIAN_POINT('Ctrl Pts',(7.00396906651109,-0.368204930512505,
81.2098085663366));
#141236=CARTESIAN_POINT('Ctrl Pts',(6.98958488172844,-0.550753795822862,
81.2014800279732));
#141237=CARTESIAN_POINT('Ctrl Pts',(6.97521163806677,-0.733163807993345,
81.1931578245913));
#141238=CARTESIAN_POINT('Ctrl Pts',(6.95368422473391,-0.915127636617246,
81.1848356212095));
#141239=CARTESIAN_POINT('Ctrl Pts',(6.92504733887556,-1.09605926702552,
81.1765134178276));
#141240=CARTESIAN_POINT('Ctrl Pts',(6.89642762265707,-1.27688241737952,
81.1681962041376));
#141241=CARTESIAN_POINT('Ctrl Pts',(6.86070698361759,-1.45667427311052,
81.1598789904475));
#141242=CARTESIAN_POINT('Ctrl Pts',(6.81798186851661,-1.63485467338192,
81.1515617767575));
#141243=CARTESIAN_POINT('Ctrl Pts',(6.77527549385069,-1.81295691872708,
81.1432482112309));
#141244=CARTESIAN_POINT('Ctrl Pts',(6.72557084669709,-1.98944879255069,
81.1349346457043));
#141245=CARTESIAN_POINT('Ctrl Pts',(6.66901539419426,-2.16376066941333,
81.1266210801777));
#141246=CARTESIAN_POINT('Ctrl Pts',(6.610564170535,-2.34391558021443,81.1180288391735));
#141247=CARTESIAN_POINT('Ctrl Pts',(6.54479495644247,-2.52174144346886,
81.1094365981694));
#141248=CARTESIAN_POINT('Ctrl Pts',(6.47192669577704,-2.69662593011868,
81.1008443571653));
#141249=CARTESIAN_POINT('Ctrl Pts',(6.40143816179019,-2.86579905115131,
81.0925327209809));
#141250=CARTESIAN_POINT('Ctrl Pts',(6.3243070972796,-3.03221956147002,81.0842210847965));
#141251=CARTESIAN_POINT('Ctrl Pts',(6.24078084161365,-3.19535303987652,
81.075909448612));
#141252=CARTESIAN_POINT('Ctrl Pts',(6.15724857152508,-3.3584982649329,81.0675972139368));
#141253=CARTESIAN_POINT('Ctrl Pts',(6.06732034485712,-3.51835568779264,
81.0592849792617));
#141254=CARTESIAN_POINT('Ctrl Pts',(5.97128977938191,-3.67441491031554,
81.0509727445865));
#141255=CARTESIAN_POINT('Ctrl Pts',(5.87523826249621,-3.83050818096483,
81.0426586963945));
#141256=CARTESIAN_POINT('Ctrl Pts',(5.77308192828184,-3.98280131386503,
81.0343446482026));
#141257=CARTESIAN_POINT('Ctrl Pts',(5.66515827864774,-4.1308120558032,81.0260306000106));
#141258=CARTESIAN_POINT('Ctrl Pts',(5.55719530357931,-4.27887673019018,
81.0177135223293));
#141259=CARTESIAN_POINT('Ctrl Pts',(5.44346102090149,-4.42265563212763,
81.0093964446479));
#141260=CARTESIAN_POINT('Ctrl Pts',(5.32433404808417,-4.56169853310274,
81.0010793669665));
#141261=CARTESIAN_POINT('Ctrl Pts',(5.20509635355595,-4.70087066650539,
80.9927545590369));
#141262=CARTESIAN_POINT('Ctrl Pts',(5.08045617410901,-4.83529775067298,
80.9844297511073));
#141263=CARTESIAN_POINT('Ctrl Pts',(4.95083065517876,-4.96456467237987,
80.9761049431777));
#141264=CARTESIAN_POINT('Ctrl Pts',(4.82113483814352,-5.09390169771843,
80.9677756205643));
#141265=CARTESIAN_POINT('Ctrl Pts',(4.68644853309016,-5.21807274983576,
80.959446297951));
#141266=CARTESIAN_POINT('Ctrl Pts',(4.54722334099428,-5.33670183255697,
80.9511169753377));
#141267=CARTESIAN_POINT('Ctrl Pts',(4.40784849322882,-5.45545843181838,
80.9427786993852));
#141268=CARTESIAN_POINT('Ctrl Pts',(4.26392527374218,-5.56866095281499,
80.9344404234328));
#141269=CARTESIAN_POINT('Ctrl Pts',(4.11593653879105,-5.67597506787554,
80.9261021474804));
#141270=CARTESIAN_POINT('Ctrl Pts',(4.08224556720107,-5.70040609502705,
80.9242038636798));
#141271=CARTESIAN_POINT('Ctrl Pts',(4.04834399747367,-5.72453211600507,
80.9223055798793));
#141272=CARTESIAN_POINT('Ctrl Pts',(4.0142377187011,-5.74834951096899,80.9204072960787));
#141273=CARTESIAN_POINT('Ctrl Pts',(3.86365171675426,-5.85350804521781,
80.9120259956738));
#141274=CARTESIAN_POINT('Ctrl Pts',(3.70875556564048,-5.95286840638953,
80.9036446952689));
#141275=CARTESIAN_POINT('Ctrl Pts',(3.55002072808798,-6.04607140155041,
80.895263394864));
#141276=CARTESIAN_POINT('Ctrl Pts',(3.39148706370504,-6.13915627555882,
80.8868927165305));
#141277=CARTESIAN_POINT('Ctrl Pts',(3.22912468852552,-6.22609917068564,
80.8785220381969));
#141278=CARTESIAN_POINT('Ctrl Pts',(3.06343546059892,-6.30658304799398,
80.8701513598634));
#141279=CARTESIAN_POINT('Ctrl Pts',(2.89793426149888,-6.38697558991984,
80.8617901808126));
#141280=CARTESIAN_POINT('Ctrl Pts',(2.72911402738103,-6.46092358098629,
80.8534290017617));
#141281=CARTESIAN_POINT('Ctrl Pts',(2.55750312363249,-6.52815474197036,
80.8450678227109));
#141282=CARTESIAN_POINT('Ctrl Pts',(2.38611490527457,-6.59529866259254,
80.8367174932762));
#141283=CARTESIAN_POINT('Ctrl Pts',(2.21194354383373,-6.65574301892428,
80.8283671638415));
#141284=CARTESIAN_POINT('Ctrl Pts',(2.03553930953716,-6.70926272267147,
80.8200168344068));
#141285=CARTESIAN_POINT('Ctrl Pts',(1.85927080774681,-6.76274124620805,
80.8116729300511));
#141286=CARTESIAN_POINT('Ctrl Pts',(1.68077316909256,-6.80930564038382,
80.8033290256953));
#141287=CARTESIAN_POINT('Ctrl Pts',(1.50061491265844,-6.84877955890005,
80.7949851213396));
#141288=CARTESIAN_POINT('Ctrl Pts',(1.32060136045926,-6.88822177171878,
80.7866479188599));
#141289=CARTESIAN_POINT('Ctrl Pts',(1.13893016972256,-6.92058479704774,
80.7783107163802));
#141290=CARTESIAN_POINT('Ctrl Pts',(0.956183382067479,-6.94574257386192,
80.7699735139005));
#141291=CARTESIAN_POINT('Ctrl Pts',(0.896024148308741,-6.95402437512166,
80.7672289528644));
#141292=CARTESIAN_POINT('Ctrl Pts',(0.8357484528534,-6.96152575851744,80.7644843918283));
#141293=CARTESIAN_POINT('Ctrl Pts',(0.77537732339638,-6.96824343495997,
80.7617398307922));
#141294=CARTESIAN_POINT('Ctrl Pts',(0.591962487992189,-6.9886525531939,
80.7534015204902));
#141295=CARTESIAN_POINT('Ctrl Pts',(0.407816762153555,-7.00180733844399,
80.7450632101883));
#141296=CARTESIAN_POINT('Ctrl Pts',(0.223536000561251,-7.00768565354876,
80.7367248998863));
#141297=CARTESIAN_POINT('Ctrl Pts',(0.0391392957665859,-7.01356766708993,
80.7283813434024));
#141298=CARTESIAN_POINT('Ctrl Pts',(-0.145392286761038,-7.01216406843352,
80.7200377869185));
#141299=CARTESIAN_POINT('Ctrl Pts',(-0.329463727115471,-7.00350485221615,
80.7116942304347));
#141300=CARTESIAN_POINT('Ctrl Pts',(-0.513675208219146,-6.99483904810485,
80.7033443262094));
#141301=CARTESIAN_POINT('Ctrl Pts',(-0.697425521947222,-6.97890663112914,
80.6949944219841));
#141302=CARTESIAN_POINT('Ctrl Pts',(-0.880125155567984,-6.95578940689239,
80.6866445177588));
#141303=CARTESIAN_POINT('Ctrl Pts',(-1.06309882511928,-6.93263750852999,
80.6782820892951));
#141304=CARTESIAN_POINT('Ctrl Pts',(-1.24501833999358,-6.90227930887797,
80.6699196608314));
#141305=CARTESIAN_POINT('Ctrl Pts',(-1.42530326558753,-6.86484793448519,
80.6615572323677));
#141306=CARTESIAN_POINT('Ctrl Pts',(-1.6057423593696,-6.82738455116459,
80.6531876528877));
#141307=CARTESIAN_POINT('Ctrl Pts',(-1.78454375773002,-6.78283600374846,
80.6448180734076));
#141308=CARTESIAN_POINT('Ctrl Pts',(-1.96114201226738,-6.73138533811725,
80.6364484939276));
#141309=CARTESIAN_POINT('Ctrl Pts',(-2.13801264809562,-6.67985531610305,
80.628066005391));
#141310=CARTESIAN_POINT('Ctrl Pts',(-2.31267303961262,-6.62140200642127,
80.6196835168544));
#141311=CARTESIAN_POINT('Ctrl Pts',(-2.48457621513433,-6.55625713297524,
80.6113010283177));
#141312=CARTESIAN_POINT('Ctrl Pts',(-2.54082575095673,-6.53494066292501,
80.6085581407138));
#141313=CARTESIAN_POINT('Ctrl Pts',(-2.59678025701267,-6.51290809479127,
80.6058152531098));
#141314=CARTESIAN_POINT('Ctrl Pts',(-2.65242114102988,-6.49016861515306,
80.6030723655058));
#141315=CARTESIAN_POINT('Ctrl Pts',(-2.82261366211158,-6.42061383657484,
80.594682510373));
#141316=CARTESIAN_POINT('Ctrl Pts',(-2.99021376345985,-6.34430126921104,
80.5862926552403));
#141317=CARTESIAN_POINT('Ctrl Pts',(-3.15466815543341,-6.26144515200719,
80.5779028001075));
#141318=CARTESIAN_POINT('Ctrl Pts',(-3.3189707911995,-6.17866549326676,
80.5695206870154));
#141319=CARTESIAN_POINT('Ctrl Pts',(-3.48013321219805,-6.08935446921641,
80.5611385739233));
#141320=CARTESIAN_POINT('Ctrl Pts',(-3.63762249876359,-5.99377419653001,
80.5527564608313));
#141321=CARTESIAN_POINT('Ctrl Pts',(-3.79498960702153,-5.89826807387763,
80.5443808504824));
#141322=CARTESIAN_POINT('Ctrl Pts',(-3.94868898201521,-5.79650256908246,
80.5360052401335));
#141323=CARTESIAN_POINT('Ctrl Pts',(-4.09821229258766,-5.68878568478225,
80.5276296297847));
#141324=CARTESIAN_POINT('Ctrl Pts',(-4.24764155077749,-5.58113655600174,
80.5192592878191));
#141325=CARTESIAN_POINT('Ctrl Pts',(-4.39289971612787,-5.4675437035836,
80.5108889458536));
#141326=CARTESIAN_POINT('Ctrl Pts',(-4.53350706626479,-5.34835864940144,
80.502518603888));
#141327=CARTESIAN_POINT('Ctrl Pts',(-4.6740465837488,-5.22923109319791,
80.4941522999937));
#141328=CARTESIAN_POINT('Ctrl Pts',(-4.80993950995811,-5.10451692730369,
80.4857859960994));
#141329=CARTESIAN_POINT('Ctrl Pts',(-4.94073852006193,-4.97460847091269,
80.4774196922051));
#141330=CARTESIAN_POINT('Ctrl Pts',(-5.07150094934882,-4.84473634627569,
80.4690557281315));
#141331=CARTESIAN_POINT('Ctrl Pts',(-5.19717206921479,-4.70967305816952,
80.4606917640579));
#141332=CARTESIAN_POINT('Ctrl Pts',(-5.31734040984741,-4.56984874238784,
80.4523277999843));
#141333=CARTESIAN_POINT('Ctrl Pts',(-5.43749025856936,-4.43004594324477,
80.4439651229857));
#141334=CARTESIAN_POINT('Ctrl Pts',(-5.55213880222743,-4.2854838263521,
80.4356024459872));
#141335=CARTESIAN_POINT('Ctrl Pts',(-5.66091369828302,-4.13662696687672,
80.4272397689887));
#141336=CARTESIAN_POINT('Ctrl Pts',(-5.76968635486227,-3.98777317209207,
80.4188772641624));
#141337=CARTESIAN_POINT('Ctrl Pts',(-5.8725854113914,-3.83462507662563,
80.4105147593361));
#141338=CARTESIAN_POINT('Ctrl Pts',(-5.96928059209372,-3.67767804128545,
80.4021522545098));
#141339=CARTESIAN_POINT('Ctrl Pts',(-6.06598667079832,-3.52071331727523,
80.3937888071898));
#141340=CARTESIAN_POINT('Ctrl Pts',(-6.15648730773457,-3.35994907984399,
80.3854253598699));
#141341=CARTESIAN_POINT('Ctrl Pts',(-6.24049688580549,-3.19590756761707,
80.3770619125499));
#141342=CARTESIAN_POINT('Ctrl Pts',(-6.32455593107694,-3.0317694631376,
80.3686935405971));
#141343=CARTESIAN_POINT('Ctrl Pts',(-6.4021161291593,-2.86435052015493,
80.3603251686443));
#141344=CARTESIAN_POINT('Ctrl Pts',(-6.47293850667418,-2.69419629042033,
80.3519567966915));
#141345=CARTESIAN_POINT('Ctrl Pts',(-6.54378210442428,-2.52399107803158,
80.3435859173558));
#141346=CARTESIAN_POINT('Ctrl Pts',(-6.60788373468279,-2.35104925021817,
80.3352150380201));
#141347=CARTESIAN_POINT('Ctrl Pts',(-6.66505324983001,-2.17593468179321,
80.3268441586843));
#141348=CARTESIAN_POINT('Ctrl Pts',(-6.72227120408923,-2.00067174068792,
80.318466186793));
#141349=CARTESIAN_POINT('Ctrl Pts',(-6.77254520996059,-1.82323269478883,
80.3100882149018));
#141350=CARTESIAN_POINT('Ctrl Pts',(-6.81573518618814,-1.64419598413845,
80.3017102430105));
#141351=CARTESIAN_POINT('Ctrl Pts',(-6.84318276777912,-1.53041669661422,
80.2963859736513));
#141352=CARTESIAN_POINT('Ctrl Pts',(-6.86777033888534,-1.41599240805197,
80.2910617042921));
#141353=CARTESIAN_POINT('Ctrl Pts',(-6.889472729271,-1.30107343187507,80.2857374349329));
#141354=CARTESIAN_POINT('Ctrl Pts',(-6.92152261639972,-1.13136216274916,
80.2778746037437));
#141355=CARTESIAN_POINT('Ctrl Pts',(-6.94734408917813,-0.960218692718378,
80.2700117725544));
#141356=CARTESIAN_POINT('Ctrl Pts',(-6.96680925618404,-0.788159470188911,
80.2621489413652));
#141357=CARTESIAN_POINT('Ctrl Pts',(-6.98625946677848,-0.616232452460369,
80.2542921517238));
#141358=CARTESIAN_POINT('Ctrl Pts',(-6.99936304151796,-0.443391457918423,
80.2464353620825));
#141359=CARTESIAN_POINT('Ctrl Pts',(-7.00604296529341,-0.270163896482813,
80.2385785724412));
#141360=CARTESIAN_POINT('Ctrl Pts',(-7.01271912190806,-0.0970340271916611,
80.2307262136572));
#141361=CARTESIAN_POINT('Ctrl Pts',(-7.01297881916433,0.0764815955293988,
80.2228738548733));
#141362=CARTESIAN_POINT('Ctrl Pts',(-7.00679681341454,0.249849910994238,
80.2150214960894));
#141363=CARTESIAN_POINT('Ctrl Pts',(-7.00061626730844,0.423177292176963,
80.207170991339));
#141364=CARTESIAN_POINT('Ctrl Pts',(-6.98799705047378,0.596357054343114,
80.1993204865887));
#141365=CARTESIAN_POINT('Ctrl Pts',(-6.96896602986842,0.768855667235388,
80.1914699818383));
#141366=CARTESIAN_POINT('Ctrl Pts',(-6.94993807075447,0.941326530537565,
80.1836207399867));
#141367=CARTESIAN_POINT('Ctrl Pts',(-6.92450040602607,1.11311608379987,
80.1757714981351));
#141368=CARTESIAN_POINT('Ctrl Pts',(-6.89273177670881,1.28369592071046,
80.1679222562835));
#141369=CARTESIAN_POINT('Ctrl Pts',(-6.8609524439185,1.45433322930696,80.1600703698687));
#141370=CARTESIAN_POINT('Ctrl Pts',(-6.8228379558657,1.62375963203353,80.1522184834539));
#141371=CARTESIAN_POINT('Ctrl Pts',(-6.77851822867896,1.7914567217678,80.1443665970391));
#141372=CARTESIAN_POINT('Ctrl Pts',(-6.74597480464092,1.91459460748116,
80.1386010545749));
#141373=CARTESIAN_POINT('Ctrl Pts',(-6.71008672266062,2.03680028130331,
80.1328355121108));
#141374=CARTESIAN_POINT('Ctrl Pts',(-6.67092249617117,2.1578738639173,80.1270699696466));
#141375=CARTESIAN_POINT('Ctrl Pts',(-6.60533586158603,2.36063055114458,
80.1174146652865));
#141376=CARTESIAN_POINT('Ctrl Pts',(-6.53059419910339,2.56010866817527,
80.1077593609264));
#141377=CARTESIAN_POINT('Ctrl Pts',(-6.44704521748296,2.75558242958364,
80.0981040565664));
#141378=CARTESIAN_POINT('Ctrl Pts',(-6.36303339017783,2.95213907896008,
80.0883952636314));
#141379=CARTESIAN_POINT('Ctrl Pts',(-6.27011646050716,3.14464686118867,
80.0786864706965));
#141380=CARTESIAN_POINT('Ctrl Pts',(-6.16869094438954,3.33239832479649,
80.0689776777616));
#141381=CARTESIAN_POINT('Ctrl Pts',(-6.06677736007615,3.52105326438949,
80.0592221652906));
#141382=CARTESIAN_POINT('Ctrl Pts',(-5.95627314588338,3.70490597294427,
80.0494666528197));
#141383=CARTESIAN_POINT('Ctrl Pts',(-5.83762301887757,3.8832697629666,80.0397111403488));
#141384=CARTESIAN_POINT('Ctrl Pts',(-5.71885540999204,4.06181016058183,
80.0299459684196));
#141385=CARTESIAN_POINT('Ctrl Pts',(-5.59192578557884,4.2348507429436,80.0201807964905));
#141386=CARTESIAN_POINT('Ctrl Pts',(-5.45732198892953,4.40173412096258,
80.0104156245614));
#141387=CARTESIAN_POINT('Ctrl Pts',(-5.32290172150337,4.56838995728151,
80.0006637672226));
#141388=CARTESIAN_POINT('Ctrl Pts',(-5.18082821859198,4.7289053387521,79.9909119098839));
#141389=CARTESIAN_POINT('Ctrl Pts',(-5.03162852562127,4.88265716005684,
79.9811600525451));
#141390=CARTESIAN_POINT('Ctrl Pts',(-4.96656665394707,4.94970408936498,
79.9769075364835));
#141391=CARTESIAN_POINT('Ctrl Pts',(-4.90015019908747,5.01546527432629,
79.9726550204218));
#141392=CARTESIAN_POINT('Ctrl Pts',(-4.8324253128829,5.07989095925381,79.9684025043601));
#141393=CARTESIAN_POINT('Ctrl Pts',(-4.7044923218825,5.20159172586908,79.9603694587613));
#141394=CARTESIAN_POINT('Ctrl Pts',(-4.57182535042884,5.31858360796275,
79.9523364131626));
#141395=CARTESIAN_POINT('Ctrl Pts',(-4.43481306854115,5.4304750813899,79.9443033675638));
#141396=CARTESIAN_POINT('Ctrl Pts',(-4.29788886342366,5.54229462666977,
79.9362754859161));
#141397=CARTESIAN_POINT('Ctrl Pts',(-4.15662519080637,5.64902005879458,
79.9282476042684));
#141398=CARTESIAN_POINT('Ctrl Pts',(-4.01144643543129,5.75029773647988,
79.9202197226206));
#141399=CARTESIAN_POINT('Ctrl Pts',(-3.86633322969545,5.8515296862953,79.9121954656406));
#141400=CARTESIAN_POINT('Ctrl Pts',(-3.71730876091136,5.9473185699505,79.9041712086606));
#141401=CARTESIAN_POINT('Ctrl Pts',(-3.56482920866232,6.03735200858522,
79.8961469516806));
#141402=CARTESIAN_POINT('Ctrl Pts',(-3.41236809274417,6.1273745612602,79.8881236649149));
#141403=CARTESIAN_POINT('Ctrl Pts',(-3.25645303700428,6.21164286210243,
79.8801003781493));
#141404=CARTESIAN_POINT('Ctrl Pts',(-3.0975679747414,6.28988864800932,79.8720770913837));
#141405=CARTESIAN_POINT('Ctrl Pts',(-2.93869593169206,6.36812802237203,
79.8640544620548));
#141406=CARTESIAN_POINT('Ctrl Pts',(-2.77685469757785,6.44034570640787,
79.856031832726));
#141407=CARTESIAN_POINT('Ctrl Pts',(-2.61255122253328,6.50632020977602,
79.8480092033971));
#141408=CARTESIAN_POINT('Ctrl Pts',(-2.44818598107929,6.57231951486054,
79.8399835581308));
#141409=CARTESIAN_POINT('Ctrl Pts',(-2.28135699111813,6.63207081687292,
79.8319579128645));
#141410=CARTESIAN_POINT('Ctrl Pts',(-2.11258987983676,6.685401301501,79.8239322675982));
#141411=CARTESIAN_POINT('Ctrl Pts',(-2.01307450685555,6.71684820504008,
79.81919985809));
#141412=CARTESIAN_POINT('Ctrl Pts',(-1.91288556627672,6.74606352631667,
79.8144674485818));
#141413=CARTESIAN_POINT('Ctrl Pts',(-1.81213302469277,6.77302004007945,
79.8097350390737));
#141414=CARTESIAN_POINT('Ctrl Pts',(-1.62627112775869,6.82274770653743,
79.8010049902389));
#141415=CARTESIAN_POINT('Ctrl Pts',(-1.43839775577256,6.8648109054016,79.7922749414041));
#141416=CARTESIAN_POINT('Ctrl Pts',(-1.24914618178807,6.89907677729595,
79.7835448925694));
#141417=CARTESIAN_POINT('Ctrl Pts',(-1.05983988547522,6.93335255720984,
79.7748123194301));
#141418=CARTESIAN_POINT('Ctrl Pts',(-0.869154861278288,6.95982646103044,
79.7660797462908));
#141419=CARTESIAN_POINT('Ctrl Pts',(-0.67773289903662,6.97841706120116,
79.7573471731516));
#141420=CARTESIAN_POINT('Ctrl Pts',(-0.483591482257702,6.99727177052316,
79.7484905398712));
#141421=CARTESIAN_POINT('Ctrl Pts',(-0.288692317572583,7.00801745122328,
79.7396339065908));
#141422=CARTESIAN_POINT('Ctrl Pts',(-0.0937089961110163,7.01062373733949,
79.7307772733105));
#141423=CARTESIAN_POINT('Ctrl Pts',(0.0986654612738358,7.01319515151808,
79.7220391412036));
#141424=CARTESIAN_POINT('Ctrl Pts',(0.291121559355534,7.00784364703478,
79.7133010090968));
#141425=CARTESIAN_POINT('Ctrl Pts',(0.483012649033695,6.99459257879781,
79.7045628769899));
#141426=CARTESIAN_POINT('Ctrl Pts',(0.678807202123559,6.98107195630424,
79.6956469931228));
#141427=CARTESIAN_POINT('Ctrl Pts',(0.87401321793027,6.95932695708805,79.6867311092557));
#141428=CARTESIAN_POINT('Ctrl Pts',(1.06794850414328,6.92943811250221,79.6778152253885));
#141429=CARTESIAN_POINT('Ctrl Pts',(1.26188379035636,6.89954926791636,79.6688993415214));
#141430=CARTESIAN_POINT('Ctrl Pts',(1.45454804901883,6.86151663003608,79.6599834576543));
#141431=CARTESIAN_POINT('Ctrl Pts',(1.64526833286611,6.8154764085402,79.6510675737872));
#141432=CARTESIAN_POINT('Ctrl Pts',(1.83224091494127,6.77034088903095,79.6423268892911));
#141433=CARTESIAN_POINT('Ctrl Pts',(2.01736507058887,6.71750477297077,79.633586204795));
#141434=CARTESIAN_POINT('Ctrl Pts',(2.20001788583994,6.65714262010995,79.6248455202989));
#141435=CARTESIAN_POINT('Ctrl Pts',(2.38263783881556,6.59679132740308,79.6161064083971));
#141436=CARTESIAN_POINT('Ctrl Pts',(2.56278707949173,6.5289167879364,79.6073672964953));
#141437=CARTESIAN_POINT('Ctrl Pts',(2.73985880537629,6.45374312233622,79.5986281845935));
#141438=CARTESIAN_POINT('Ctrl Pts',(2.91922475032313,6.37759547370322,79.5897758449191));
#141439=CARTESIAN_POINT('Ctrl Pts',(3.09543260615769,6.29395832975056,79.5809235052447));
#141440=CARTESIAN_POINT('Ctrl Pts',(3.26787224700597,6.20311514803233,79.5720711655703));
#141441=CARTESIAN_POINT('Ctrl Pts',(3.43801900734852,6.11347988207765,79.5633365329207));
#141442=CARTESIAN_POINT('Ctrl Pts',(3.6044968980425,6.01682916476232,79.554601900271));
#141443=CARTESIAN_POINT('Ctrl Pts',(3.76674336334902,5.91348213806097,79.5458672676214));
#141444=CARTESIAN_POINT('Ctrl Pts',(3.93226945405079,5.80804607026616,79.5369560744346));
#141445=CARTESIAN_POINT('Ctrl Pts',(4.09339097409204,5.69564023119062,79.5280448812479));
#141446=CARTESIAN_POINT('Ctrl Pts',(4.24953957757411,5.57665131966589,79.5191336880611));
#141447=CARTESIAN_POINT('Ctrl Pts',(4.40568818105612,5.4576624081412,79.5102224948744));
#141448=CARTESIAN_POINT('Ctrl Pts',(4.55686361870708,5.33209059717816,79.5013113016876));
#141449=CARTESIAN_POINT('Ctrl Pts',(4.7025306618469,5.2003684424173,79.4924001085009));
#141450=CARTESIAN_POINT('Ctrl Pts',(4.83372204101002,5.08173617820069,79.4843744652328));
#141451=CARTESIAN_POINT('Ctrl Pts',(4.96050536383317,4.95806030922865,79.4763488219647));
#141452=CARTESIAN_POINT('Ctrl Pts',(5.08247090262828,4.82971180159199,79.4683231786966));
#141453=CARTESIAN_POINT('Ctrl Pts',(5.20439720845569,4.70140458014898,79.4603001170577));
#141454=CARTESIAN_POINT('Ctrl Pts',(5.32150856365554,4.5684279780931,79.4522770554189));
#141455=CARTESIAN_POINT('Ctrl Pts',(5.43343174174833,4.43119014151522,79.4442539937801));
#141456=CARTESIAN_POINT('Ctrl Pts',(5.54534032455606,4.29397020136757,79.4362319783845));
#141457=CARTESIAN_POINT('Ctrl Pts',(5.65206184695248,4.15249041808088,79.4282099629889));
#141458=CARTESIAN_POINT('Ctrl Pts',(5.75326309952588,4.00719231758769,79.4201879475934));
#141459=CARTESIAN_POINT('Ctrl Pts',(5.85449755639625,3.86184654454942,79.4121633001614));
#141460=CARTESIAN_POINT('Ctrl Pts',(5.95020791413237,3.71268025162831,79.4041386527294));
#141461=CARTESIAN_POINT('Ctrl Pts',(6.04010386323041,3.56016458662926,79.3961140052974));
#141462=CARTESIAN_POINT('Ctrl Pts',(6.13001735862996,3.40761915292684,79.3880877915782));
#141463=CARTESIAN_POINT('Ctrl Pts',(6.21411400611913,3.25172336500418,79.3800615778589));
#141464=CARTESIAN_POINT('Ctrl Pts',(6.29214938284766,3.09297311763776,79.3720353641396));
#141465=CARTESIAN_POINT('Ctrl Pts',(6.37023961705004,2.93411127168734,79.3640035081357));
#141466=CARTESIAN_POINT('Ctrl Pts',(6.44225992040282,2.77239129287253,79.3559716521318));
#141467=CARTESIAN_POINT('Ctrl Pts',(6.50801376409652,2.60832962043341,79.3479397961278));
#141468=CARTESIAN_POINT('Ctrl Pts',(6.52973061026753,2.55414416293352,79.3452870754425));
#141469=CARTESIAN_POINT('Ctrl Pts',(6.5507643016582,2.49970340540043,79.3426343547572));
#141470=CARTESIAN_POINT('Ctrl Pts',(6.57110895151812,2.44502632087642,79.3399816340719));
#141471=CARTESIAN_POINT('Origin',(0.,0.,50.));
#141472=CARTESIAN_POINT('',(6.57110895151816,2.4450263208763,77.3398522865014));
#141473=CARTESIAN_POINT('',(6.57110895151815,2.44502632087633,77.886969536131));
#141474=CARTESIAN_POINT('',(6.57110895151814,2.44502632087636,50.));
#141475=CARTESIAN_POINT('',(7.01124999765299,0.000181413712741437,79.7735343568736));
#141476=CARTESIAN_POINT('Ctrl Pts',(6.57110895151815,2.44502632087633,77.886969536131));
#141477=CARTESIAN_POINT('Ctrl Pts',(6.54472329191852,2.51593886791374,77.8903887297223));
#141478=CARTESIAN_POINT('Ctrl Pts',(6.5171868554085,2.58643166442415,77.8938079233136));
#141479=CARTESIAN_POINT('Ctrl Pts',(6.48851466909111,2.6564645586737,77.897227116905));
#141480=CARTESIAN_POINT('Ctrl Pts',(6.4185924549299,2.82725219850838,77.9055654272069));
#141481=CARTESIAN_POINT('Ctrl Pts',(6.3419518830268,2.99520730994608,77.9139037375089));
#141482=CARTESIAN_POINT('Ctrl Pts',(6.25885887899737,3.1597962110389,77.9222420478109));
#141483=CARTESIAN_POINT('Ctrl Pts',(6.1757135956692,3.32448866588369,77.9305856042948));
#141484=CARTESIAN_POINT('Ctrl Pts',(6.08610793039912,3.48581039346846,77.9389291607787));
#141485=CARTESIAN_POINT('Ctrl Pts',(5.99035317373331,3.64325341095611,77.9472727172626));
#141486=CARTESIAN_POINT('Ctrl Pts',(5.894525567266,3.80081621040521,77.9556226214879));
#141487=CARTESIAN_POINT('Ctrl Pts',(5.79253970798148,3.95449413403783,77.9639725257131));
#141488=CARTESIAN_POINT('Ctrl Pts',(5.68474973206404,4.10380884621809,77.9723224299384));
#141489=CARTESIAN_POINT('Ctrl Pts',(5.57679807915941,4.25334751941701,77.9806848584022));
#141490=CARTESIAN_POINT('Ctrl Pts',(5.46302510475072,4.39850963731453,77.9890472868659));
#141491=CARTESIAN_POINT('Ctrl Pts',(5.34382565033219,4.53884941161874,77.9974097153296));
#141492=CARTESIAN_POINT('Ctrl Pts',(5.22452426413071,4.67930919556127,78.0057792948096));
#141493=CARTESIAN_POINT('Ctrl Pts',(5.09978736043104,4.8149381673483,78.0141488742897));
#141494=CARTESIAN_POINT('Ctrl Pts',(4.97004642619015,4.94532760128331,78.0225184537697));
#141495=CARTESIAN_POINT('Ctrl Pts',(4.84010538236574,5.07591814503361,78.0309009423064));
#141496=CARTESIAN_POINT('Ctrl Pts',(4.70514512454138,5.20125277945567,78.039283430843));
#141497=CARTESIAN_POINT('Ctrl Pts',(4.56563102380178,5.32096231118006,78.0476659193797));
#141498=CARTESIAN_POINT('Ctrl Pts',(4.51997972397395,5.36013323151019,78.0504088069836));
#141499=CARTESIAN_POINT('Ctrl Pts',(4.47384107816586,5.39870221087662,78.0531516945875));
#141500=CARTESIAN_POINT('Ctrl Pts',(4.42723205493097,5.43665732728225,78.0558945821914));
#141501=CARTESIAN_POINT('Ctrl Pts',(4.28466589499671,5.55275319928838,78.0642844373241));
#141502=CARTESIAN_POINT('Ctrl Pts',(4.13740883337362,5.66333692192329,78.072674292457));
#141503=CARTESIAN_POINT('Ctrl Pts',(3.98591391741904,5.76802538182914,78.0810641475897));
#141504=CARTESIAN_POINT('Ctrl Pts',(3.83455879884903,5.87261723669187,78.0894462606818));
#141505=CARTESIAN_POINT('Ctrl Pts',(3.67897389092021,5.97132448761054,78.0978283737739));
#141506=CARTESIAN_POINT('Ctrl Pts',(3.51964451587166,6.063804832314,78.106210486866));
#141507=CARTESIAN_POINT('Ctrl Pts',(3.36043874664933,6.15621343187057,78.1145860972149));
#141508=CARTESIAN_POINT('Ctrl Pts',(3.19749458510357,6.24240459184611,78.1229617075637));
#141509=CARTESIAN_POINT('Ctrl Pts',(3.03132585956824,6.32207957049047,78.1313373179126));
#141510=CARTESIAN_POINT('Ctrl Pts',(2.8652616566293,6.40170443238987,78.1397076598781));
#141511=CARTESIAN_POINT('Ctrl Pts',(2.6959772295971,6.4748211437882,78.1480780018437));
#141512=CARTESIAN_POINT('Ctrl Pts',(2.52401090989317,6.5411769192738,78.1564483438093));
#141513=CARTESIAN_POINT('Ctrl Pts',(2.35212755122628,6.60750068300292,78.1648146477036));
#141514=CARTESIAN_POINT('Ctrl Pts',(2.17756518610174,6.66706989695353,78.1731809515979));
#141515=CARTESIAN_POINT('Ctrl Pts',(2.0008824450884,6.71967975452976,78.1815472554922));
#141516=CARTESIAN_POINT('Ctrl Pts',(1.82424911728582,6.77227489860332,78.1899112195658));
#141517=CARTESIAN_POINT('Ctrl Pts',(1.64549691034441,6.81791447217705,78.1982751836394));
#141518=CARTESIAN_POINT('Ctrl Pts',(1.46520048149888,6.85644325518089,78.206639147713));
#141519=CARTESIAN_POINT('Ctrl Pts',(1.28493179727746,6.89496610924532,78.2150018247116));
#141520=CARTESIAN_POINT('Ctrl Pts',(1.10311968624668,6.9263802857582,78.2233645017101));
#141521=CARTESIAN_POINT('Ctrl Pts',(0.920350300449677,6.95058140639776,
78.2317271787086));
#141522=CARTESIAN_POINT('Ctrl Pts',(0.737584677540096,6.97478202878049,
78.2400896835349));
#141523=CARTESIAN_POINT('Ctrl Pts',(0.553862145020714,6.99176984866395,
78.2484521883612));
#141524=CARTESIAN_POINT('Ctrl Pts',(0.369775734515736,7.00149216015153,
78.2568146931876));
#141525=CARTESIAN_POINT('Ctrl Pts',(0.185668576605704,7.01121556738939,
78.2651781405075));
#141526=CARTESIAN_POINT('Ctrl Pts',(0.00119778715327035,7.01367181686934,
78.2735415878275));
#141527=CARTESIAN_POINT('Ctrl Pts',(-0.183041394468293,7.00886027899052,
78.2819050351475));
#141528=CARTESIAN_POINT('Ctrl Pts',(-0.367389061298113,7.00404590794297,
78.2902734071003));
#141529=CARTESIAN_POINT('Ctrl Pts',(-0.551504518869215,6.99195520575042,
78.2986417790531));
#141530=CARTESIAN_POINT('Ctrl Pts',(-0.734794400028367,6.97263965454884,
78.3070101510059));
#141531=CARTESIAN_POINT('Ctrl Pts',(-0.918139199626124,6.95331831590332,
78.3153810303416));
#141532=CARTESIAN_POINT('Ctrl Pts',(-1.10065760321633,6.92676785149604,
78.3237519096774));
#141533=CARTESIAN_POINT('Ctrl Pts',(-1.28176354146575,6.8930913809603,78.3321227890131));
#141534=CARTESIAN_POINT('Ctrl Pts',(-1.46302292881792,6.8593863767153,78.3405007609044));
#141535=CARTESIAN_POINT('Ctrl Pts',(-1.64286713708827,6.81854336718499,
78.3488787327957));
#141536=CARTESIAN_POINT('Ctrl Pts',(-1.82072128776991,6.77071639893162,
78.357256704687));
#141537=CARTESIAN_POINT('Ctrl Pts',(-1.93374904880257,6.74032197114941,
78.3625809740461));
#141538=CARTESIAN_POINT('Ctrl Pts',(-2.04597335456123,6.70710794305258,
78.3679052434052));
#141539=CARTESIAN_POINT('Ctrl Pts',(-2.15725019586244,6.67112420473128,
78.3732295127643));
#141540=CARTESIAN_POINT('Ctrl Pts',(-2.32158279427306,6.61798375655067,
78.3810923439535));
#141541=CARTESIAN_POINT('Ctrl Pts',(-2.48418984036486,6.55868970666489,
78.3889551751428));
#141542=CARTESIAN_POINT('Ctrl Pts',(-2.644556713752,6.49337711443354,78.396818006332));
#141543=CARTESIAN_POINT('Ctrl Pts',(-2.80480036636516,6.42811470630814,
78.4046747959733));
#141544=CARTESIAN_POINT('Ctrl Pts',(-2.96280691845336,6.35684309511312,
78.4125315856147));
#141545=CARTESIAN_POINT('Ctrl Pts',(-3.11807649192569,6.27974725231839,
78.420388375256));
#141546=CARTESIAN_POINT('Ctrl Pts',(-3.2732585007094,6.2026948879291,78.4282407340399));
#141547=CARTESIAN_POINT('Ctrl Pts',(-3.42570626087676,6.11982499477659,
78.4360930928239));
#141548=CARTESIAN_POINT('Ctrl Pts',(-3.5749397274467,6.03137069890612,78.4439454516078));
#141549=CARTESIAN_POINT('Ctrl Pts',(-3.72413795825315,5.94293728812747,
78.4517959563582));
#141550=CARTESIAN_POINT('Ctrl Pts',(-3.8701230739579,5.84892228586717,78.4596464611085));
#141551=CARTESIAN_POINT('Ctrl Pts',(-4.01243957350114,5.74960478915742,
78.4674969658589));
#141552=CARTESIAN_POINT('Ctrl Pts',(-4.15473317880556,5.65030326950232,
78.4753462077105));
#141553=CARTESIAN_POINT('Ctrl Pts',(-4.29335903163953,5.54570117428883,
78.4831954495621));
#141554=CARTESIAN_POINT('Ctrl Pts',(-4.42789097194043,5.43612068511254,
78.4910446914137));
#141555=CARTESIAN_POINT('Ctrl Pts',(-4.56246823868513,5.3265032761247,78.4988965778285));
#141556=CARTESIAN_POINT('Ctrl Pts',(-4.69294854171612,5.21190436399478,
78.5067484642433));
#141557=CARTESIAN_POINT('Ctrl Pts',(-4.81893900703761,5.09268626649546,
78.5146003506581));
#141558=CARTESIAN_POINT('Ctrl Pts',(-4.91145223755515,5.00514590137596,
78.5203658931223));
#141559=CARTESIAN_POINT('Ctrl Pts',(-5.00154533075462,4.91511581917966,
78.5261314355865));
#141560=CARTESIAN_POINT('Ctrl Pts',(-5.08907563104056,4.822751889124,78.5318969780506));
#141561=CARTESIAN_POINT('Ctrl Pts',(-5.23565883552319,4.66807401412599,
78.5415522824106));
#141562=CARTESIAN_POINT('Ctrl Pts',(-5.37497948782232,4.50692938614718,
78.5512075867705));
#141563=CARTESIAN_POINT('Ctrl Pts',(-5.50656696612014,4.33997083056263,
78.5608628911305));
#141564=CARTESIAN_POINT('Ctrl Pts',(-5.63888341436198,4.17208735590149,
78.5705716840652));
#141565=CARTESIAN_POINT('Ctrl Pts',(-5.76338078438032,3.9983254299945,78.580280477));
#141566=CARTESIAN_POINT('Ctrl Pts',(-5.87962792320045,3.8193719440795,78.5899892699348));
#141567=CARTESIAN_POINT('Ctrl Pts',(-5.99643445312336,3.63955731879496,
78.5997447824055));
#141568=CARTESIAN_POINT('Ctrl Pts',(-6.10491115573157,3.45450109818367,
78.6095002948763));
#141569=CARTESIAN_POINT('Ctrl Pts',(-6.20466818990649,3.26492254359312,
78.6192558073471));
#141570=CARTESIAN_POINT('Ctrl Pts',(-6.30452399889252,3.0751562770675,78.629020979276));
#141571=CARTESIAN_POINT('Ctrl Pts',(-6.39564286188399,2.88085875906164,
78.638786151205));
#141572=CARTESIAN_POINT('Ctrl Pts',(-6.47768131128054,2.6827730787353,78.6485513231339));
#141573=CARTESIAN_POINT('Ctrl Pts',(-6.55960790311294,2.48495748373914,
78.6583031804725));
#141574=CARTESIAN_POINT('Ctrl Pts',(-6.63247881191435,2.28336408462234,
78.6680550378112));
#141575=CARTESIAN_POINT('Ctrl Pts',(-6.69599944080937,2.07875396600478,
78.6778068951498));
#141576=CARTESIAN_POINT('Ctrl Pts',(-6.72369903538854,1.98952913572375,
78.6820594112123));
#141577=CARTESIAN_POINT('Ctrl Pts',(-6.74962119971282,1.89973091567733,
78.6863119272747));
#141578=CARTESIAN_POINT('Ctrl Pts',(-6.7737443574246,1.80942364933102,78.6905644433372));
#141579=CARTESIAN_POINT('Ctrl Pts',(-6.81931324488843,1.63883231520851,
78.6985974889361));
#141580=CARTESIAN_POINT('Ctrl Pts',(-6.85848122771586,1.46634030115257,
78.706630534535));
#141581=CARTESIAN_POINT('Ctrl Pts',(-6.89109073719558,1.29247631089987,
78.7146635801339));
#141582=CARTESIAN_POINT('Ctrl Pts',(-6.92367928402718,1.11872408711358,
78.7226914617818));
#141583=CARTESIAN_POINT('Ctrl Pts',(-6.94971768234668,0.943602001475774,
78.7307193434298));
#141584=CARTESIAN_POINT('Ctrl Pts',(-6.96909872353735,0.767651968075435,
78.7387472250777));
#141585=CARTESIAN_POINT('Ctrl Pts',(-6.98847101399679,0.591781377850374,
78.7467714820579));
#141586=CARTESIAN_POINT('Ctrl Pts',(-7.00119189229259,0.415083947803786,
78.7547957390381));
#141587=CARTESIAN_POINT('Ctrl Pts',(-7.00720559944598,0.238109742750817,
78.7628199960183));
#141588=CARTESIAN_POINT('Ctrl Pts',(-7.01321857948092,0.061156935682018,
78.7708432827841));
#141589=CARTESIAN_POINT('Ctrl Pts',(-7.01252598353081,-0.116072213854308,
78.7788665695499));
#141590=CARTESIAN_POINT('Ctrl Pts',(-7.00512407177398,-0.293024404363847,
78.7868898563157));
#141591=CARTESIAN_POINT('Ctrl Pts',(-6.99772276653778,-0.469962095219859,
78.7949124856447));
#141592=CARTESIAN_POINT('Ctrl Pts',(-6.98361325991897,-0.646622506097364,
78.8029351149737));
#141593=CARTESIAN_POINT('Ctrl Pts',(-6.96284389521981,-0.822454529624714,
78.8109577443027));
#141594=CARTESIAN_POINT('Ctrl Pts',(-6.94206672271815,-0.998352653474978,
78.8189833895692));
#141595=CARTESIAN_POINT('Ctrl Pts',(-6.91462473672402,-1.17342140394086,
78.8270090348357));
#141596=CARTESIAN_POINT('Ctrl Pts',(-6.88061795612284,-1.34711658900777,
78.8350346801022));
#141597=CARTESIAN_POINT('Ctrl Pts',(-6.8605654860123,-1.44953785457088,
78.8397670896093));
#141598=CARTESIAN_POINT('Ctrl Pts',(-6.8382314103516,-1.55148170122819,
78.8444994991165));
#141599=CARTESIAN_POINT('Ctrl Pts',(-6.8136444928177,-1.65283855472792,
78.8492319086236));
#141600=CARTESIAN_POINT('Ctrl Pts',(-6.76828810714639,-1.83981524798053,
78.8579619574581));
#141601=CARTESIAN_POINT('Ctrl Pts',(-6.71524003955458,-2.02488717757136,
78.8666920062926));
#141602=CARTESIAN_POINT('Ctrl Pts',(-6.65468693636532,-2.20743478759142,
78.8754220551271));
#141603=CARTESIAN_POINT('Ctrl Pts',(-6.59411632417112,-2.39003518147947,
78.884154628266));
#141604=CARTESIAN_POINT('Ctrl Pts',(-6.52603643101028,-2.57010953884597,
78.8928872014049));
#141605=CARTESIAN_POINT('Ctrl Pts',(-6.45068313217834,-2.74705545825523,
78.9016197745439));
#141606=CARTESIAN_POINT('Ctrl Pts',(-6.37425931944732,-2.92651517691482,
78.9104764078244));
#141607=CARTESIAN_POINT('Ctrl Pts',(-6.29035397887403,-3.10275662457441,
78.9193330411049));
#141608=CARTESIAN_POINT('Ctrl Pts',(-6.19926304083474,-3.27517393630329,
78.9281896743854));
#141609=CARTESIAN_POINT('Ctrl Pts',(-6.1093908935877,-3.44528431567993,
78.936927806492));
#141610=CARTESIAN_POINT('Ctrl Pts',(-6.01252439060037,-3.61167202221359,
78.9456659385985));
#141611=CARTESIAN_POINT('Ctrl Pts',(-5.9089937192203,-3.77378056976225,
78.9544040707051));
#141612=CARTESIAN_POINT('Ctrl Pts',(-5.8033570188948,-3.93918674195573,
78.9633199545726));
#141613=CARTESIAN_POINT('Ctrl Pts',(-5.69078227620538,-4.10013754471713,
78.97223583844));
#141614=CARTESIAN_POINT('Ctrl Pts',(-5.57166689362883,-4.25607267195245,
78.9811517223075));
#141615=CARTESIAN_POINT('Ctrl Pts',(-5.45255151105233,-4.41200779918771,
78.990067606175));
#141616=CARTESIAN_POINT('Ctrl Pts',(-5.32689567699746,-4.56292701427,78.9989834900425));
#141617=CARTESIAN_POINT('Ctrl Pts',(-5.19514124450711,-4.70830479176116,
79.0078993739099));
#141618=CARTESIAN_POINT('Ctrl Pts',(-5.06597581991057,-4.85082585918653,
79.0166400584063));
#141619=CARTESIAN_POINT('Ctrl Pts',(-4.93093553144405,-4.98803638596009,
79.0253807429026));
#141620=CARTESIAN_POINT('Ctrl Pts',(-4.79047193705433,-5.11947313527427,
79.034121427399));
#141621=CARTESIAN_POINT('Ctrl Pts',(-4.65003361439863,-5.25088623693381,
79.042860539301));
#141622=CARTESIAN_POINT('Ctrl Pts',(-4.50417413430033,-5.37652744868928,
79.051599651203));
#141623=CARTESIAN_POINT('Ctrl Pts',(-4.35338084659093,-5.49597141250164,
79.060338763105));
#141624=CARTESIAN_POINT('Ctrl Pts',(-4.20063381481317,-5.61696294477241,
79.0691911027793));
#141625=CARTESIAN_POINT('Ctrl Pts',(-4.04282444449079,-5.7315953265149,
79.0780434424536));
#141626=CARTESIAN_POINT('Ctrl Pts',(-3.88049376689191,-5.83946869908667,
79.0868957821279));
#141627=CARTESIAN_POINT('Ctrl Pts',(-3.72032155380397,-5.94590771032999,
79.0956304147778));
#141628=CARTESIAN_POINT('Ctrl Pts',(-3.55574776548765,-6.04576619744464,
79.1043650474277));
#141629=CARTESIAN_POINT('Ctrl Pts',(-3.3873219776571,-6.13870315149554,
79.1130996800776));
#141630=CARTESIAN_POINT('Ctrl Pts',(-3.21549165655506,-6.23351871900755,
79.1220108732641));
#141631=CARTESIAN_POINT('Ctrl Pts',(-3.03965219366928,-6.32112979232783,
79.1309220664505));
#141632=CARTESIAN_POINT('Ctrl Pts',(-2.86041524350073,-6.40122263300135,
79.139833259637));
#141633=CARTESIAN_POINT('Ctrl Pts',(-2.68117829333212,-6.48131547367489,
79.1487444528235));
#141634=CARTESIAN_POINT('Ctrl Pts',(-2.49854412713904,-6.5538899457306,
79.15765564601));
#141635=CARTESIAN_POINT('Ctrl Pts',(-2.31314879546303,-6.61868334433277,
79.1665668391964));
#141636=CARTESIAN_POINT('Ctrl Pts',(-2.14617667780427,-6.67703805519365,
79.1745925040487));
#141637=CARTESIAN_POINT('Ctrl Pts',(-1.9768879904652,-6.7291076329979,79.182618168901));
#141638=CARTESIAN_POINT('Ctrl Pts',(-1.80580461755494,-6.77471004882993,
79.1906438337533));
#141639=CARTESIAN_POINT('Ctrl Pts',(-1.63477554231082,-6.82029799157374,
79.1986669514565));
#141640=CARTESIAN_POINT('Ctrl Pts',(-1.4619532692763,-6.8594227644161,79.2066900691596));
#141641=CARTESIAN_POINT('Ctrl Pts',(-1.28787484801487,-6.89195218630764,
79.2147131868628));
#141642=CARTESIAN_POINT('Ctrl Pts',(-1.11381837956589,-6.92447750595439,
79.2227352927805));
#141643=CARTESIAN_POINT('Ctrl Pts',(-0.93850643876666,-6.95040906463028,
79.2307573986983));
#141644=CARTESIAN_POINT('Ctrl Pts',(-0.762486221034689,-6.96966579724109,
79.2387795046161));
#141645=CARTESIAN_POINT('Ctrl Pts',(-0.586400593594999,-6.98892968571881,
79.2468045915755));
#141646=CARTESIAN_POINT('Ctrl Pts',(-0.409606527847007,-7.00151375021534,
79.254829678535));
#141647=CARTESIAN_POINT('Ctrl Pts',(-0.232656750421843,-7.00738877178819,
79.2628547654944));
#141648=CARTESIAN_POINT('Ctrl Pts',(-0.0556721236238324,-7.01326495041713,
79.2708814329546));
#141649=CARTESIAN_POINT('Ctrl Pts',(0.12146790929119,-7.01242945049088,
79.2789081004147));
#141650=CARTESIAN_POINT('Ctrl Pts',(0.29821087019992,-7.00490519845876,
79.2869347678748));
#141651=CARTESIAN_POINT('Ctrl Pts',(0.475095719735005,-6.99737490598362,
79.2949678791153));
#141652=CARTESIAN_POINT('Ctrl Pts',(0.651582494832487,-6.98314516162781,
79.3030009903559));
#141653=CARTESIAN_POINT('Ctrl Pts',(0.827123457383149,-6.96229081184825,
79.3110341015964));
#141654=CARTESIAN_POINT('Ctrl Pts',(0.930558569403216,-6.95000267138114,
79.3157675025585));
#141655=CARTESIAN_POINT('Ctrl Pts',(1.03366543804422,-6.93541544974835,
79.3205009035206));
#141656=CARTESIAN_POINT('Ctrl Pts',(1.1363337643828,-6.91855274883582,79.3252343044827));
#141657=CARTESIAN_POINT('Ctrl Pts',(1.34783371186954,-6.88381506015738,
79.334985257777));
#141658=CARTESIAN_POINT('Ctrl Pts',(1.55759675624886,-6.83939833325074,
79.3447362110712));
#141659=CARTESIAN_POINT('Ctrl Pts',(1.7648298584535,-6.7854994019019,79.3544871643655));
#141660=CARTESIAN_POINT('Ctrl Pts',(1.97236151882041,-6.73152281903059,
79.3642521657373));
#141661=CARTESIAN_POINT('Ctrl Pts',(2.17735590883776,-6.66803671563266,
79.3740171671091));
#141662=CARTESIAN_POINT('Ctrl Pts',(2.3790326926166,-6.59528847056453,79.3837821684809));
#141663=CARTESIAN_POINT('Ctrl Pts',(2.58037332298278,-6.52266148174805,
79.3935308936186));
#141664=CARTESIAN_POINT('Ctrl Pts',(2.77840736319922,-6.44080321855899,
79.4032796187564));
#141665=CARTESIAN_POINT('Ctrl Pts',(2.97237492974255,-6.35000896373682,
79.4130283438942));
#141666=CARTESIAN_POINT('Ctrl Pts',(3.16581013052874,-6.25946390393769,
79.4227503125616));
#141667=CARTESIAN_POINT('Ctrl Pts',(3.35520110237369,-6.16003183124972,
79.432472281229));
#141668=CARTESIAN_POINT('Ctrl Pts',(3.53981127429961,-6.05205442018175,
79.4421942498964));
#141669=CARTESIAN_POINT('Ctrl Pts',(3.72319992893165,-5.94479146744286,
79.4518518908362));
#141670=CARTESIAN_POINT('Ctrl Pts',(3.90187078627441,-5.82909588572984,
79.461509531776));
#141671=CARTESIAN_POINT('Ctrl Pts',(4.0751194034755,-5.70535085774026,79.4711671727158));
#141672=CARTESIAN_POINT('Ctrl Pts',(4.15126813530641,-5.65096065766813,
79.4754120384003));
#141673=CARTESIAN_POINT('Ctrl Pts',(4.2263695763594,-5.59501601050443,79.4796569040848));
#141674=CARTESIAN_POINT('Ctrl Pts',(4.30036504556434,-5.53755244105087,
79.4839017697693));
#141675=CARTESIAN_POINT('Ctrl Pts',(4.43723653858589,-5.43126046628587,
79.4917536167832));
#141676=CARTESIAN_POINT('Ctrl Pts',(4.57026540768275,-5.31981216424357,
79.499605463797));
#141677=CARTESIAN_POINT('Ctrl Pts',(4.69902863801117,-5.20353307106344,
79.5074573108108));
#141678=CARTESIAN_POINT('Ctrl Pts',(4.82775535212855,-5.08728695369399,
79.5153069311043));
#141679=CARTESIAN_POINT('Ctrl Pts',(4.95221855094749,-4.96621302570767,
79.5231565513978));
#141680=CARTESIAN_POINT('Ctrl Pts',(5.07202870601448,-4.8406767468883,79.5310061716913));
#141681=CARTESIAN_POINT('Ctrl Pts',(5.19182929577332,-4.71515049053481,
79.538855165293));
#141682=CARTESIAN_POINT('Ctrl Pts',(5.30697731848026,-4.5851628690408,79.5467041588948));
#141683=CARTESIAN_POINT('Ctrl Pts',(5.41712068376836,-4.45111559723954,
79.5545531524965));
#141684=CARTESIAN_POINT('Ctrl Pts',(5.52731981141706,-4.31700046122976,
79.5624061198139));
#141685=CARTESIAN_POINT('Ctrl Pts',(5.63250897667486,-4.17882186347203,
79.5702590871312));
#141686=CARTESIAN_POINT('Ctrl Pts',(5.73237671782133,-4.03701420947214,
79.5781120544486));
#141687=CARTESIAN_POINT('Ctrl Pts',(5.83226982201799,-3.8951705410936,79.5859670161557));
#141688=CARTESIAN_POINT('Ctrl Pts',(5.92683860173875,-3.74969630017751,
79.5938219778629));
#141689=CARTESIAN_POINT('Ctrl Pts',(6.01581578436125,-3.60105359736982,
79.6016769395701));
#141690=CARTESIAN_POINT('Ctrl Pts',(6.10488128427494,-3.45226335425481,
79.6095396979833));
#141691=CARTESIAN_POINT('Ctrl Pts',(6.18834391851647,-3.3002987021646,79.6174024563965));
#141692=CARTESIAN_POINT('Ctrl Pts',(6.26598283969305,-3.14564550055665,
79.6252652148098));
#141693=CARTESIAN_POINT('Ctrl Pts',(6.3229376382212,-3.032194130988,79.6310332215584));
#141694=CARTESIAN_POINT('Ctrl Pts',(6.37675939458197,-2.91729641314543,
79.636801228307));
#141695=CARTESIAN_POINT('Ctrl Pts',(6.42737773349409,-2.80115012690938,
79.6425692350556));
#141696=CARTESIAN_POINT('Ctrl Pts',(6.5095962779528,-2.61249560359139,79.651938114586));
#141697=CARTESIAN_POINT('Ctrl Pts',(6.58350384587159,-2.42022175213591,
79.6613069941165));
#141698=CARTESIAN_POINT('Ctrl Pts',(6.64882690551553,-2.22502299830648,
79.6706758736469));
#141699=CARTESIAN_POINT('Ctrl Pts',(6.71403384970503,-2.03017122136595,
79.680028099461));
#141700=CARTESIAN_POINT('Ctrl Pts',(6.77068672594478,-1.83240506785728,
79.6893803252751));
#141701=CARTESIAN_POINT('Ctrl Pts',(6.81856188813345,-1.63243387008294,
79.6987325510892));
#141702=CARTESIAN_POINT('Ctrl Pts',(6.86635127364715,-1.43282095546948,
79.7080680207652));
#141703=CARTESIAN_POINT('Ctrl Pts',(6.90539431044331,-1.23101102657837,
79.7174034904411));
#141704=CARTESIAN_POINT('Ctrl Pts',(6.93551768568856,-1.02772612791602,
79.726738960117));
#141705=CARTESIAN_POINT('Ctrl Pts',(6.96552096875996,-0.825251660528144,
79.7360372122886));
#141706=CARTESIAN_POINT('Ctrl Pts',(6.98667551784331,-0.621314102134208,
79.7453354644603));
#141707=CARTESIAN_POINT('Ctrl Pts',(6.99885966834505,-0.416641218931813,
79.7546337166319));
#141708=CARTESIAN_POINT('Ctrl Pts',(7.00711527886316,-0.277961086320631,
79.7609339300458));
#141709=CARTESIAN_POINT('Ctrl Pts',(7.01125359746706,-0.138943660978469,
79.7672341434597));
#141710=CARTESIAN_POINT('Ctrl Pts',(7.01124999765299,0.000181413712756845,
79.7735343568736));
#141711=CARTESIAN_POINT('Ctrl Pts',(7.01124999765297,0.000181414525455699,
79.7735343569104));
#141712=CARTESIAN_POINT('Ctrl Pts',(7.0112451663169,0.186901331078262,79.7819898802984));
#141713=CARTESIAN_POINT('Ctrl Pts',(7.00377706110129,0.373576221296077,
79.7904454036863));
#141714=CARTESIAN_POINT('Ctrl Pts',(6.98888240313398,0.559597460380375,
79.7989009270743));
#141715=CARTESIAN_POINT('Ctrl Pts',(6.97397616886368,0.745763277355162,
79.8073630221943));
#141716=CARTESIAN_POINT('Ctrl Pts',(6.95163187211473,0.93127411459491,79.8158251173143));
#141717=CARTESIAN_POINT('Ctrl Pts',(6.92193813567668,1.11552633692123,79.8242872124343));
#141718=CARTESIAN_POINT('Ctrl Pts',(6.89223239538575,1.29985304420077,79.8327527284018));
#141719=CARTESIAN_POINT('Ctrl Pts',(6.85517134370744,1.48291981239697,79.8412182443693));
#141720=CARTESIAN_POINT('Ctrl Pts',(6.81089471507894,1.66413333077905,79.8496837603369));
#141721=CARTESIAN_POINT('Ctrl Pts',(6.76657913587012,1.84550626445363,79.858156723501));
#141722=CARTESIAN_POINT('Ctrl Pts',(6.71503537560351,2.02502238667251,79.8666296866652));
#141723=CARTESIAN_POINT('Ctrl Pts',(6.65645336339179,2.20210244618414,79.8751026498293));
#141724=CARTESIAN_POINT('Ctrl Pts',(6.62948841720056,2.28361132742592,79.8790027035689));
#141725=CARTESIAN_POINT('Ctrl Pts',(6.60103295687948,2.36460432385478,79.8829027573086));
#141726=CARTESIAN_POINT('Ctrl Pts',(6.57110895151811,2.44502632087645,79.8868028110482));
#141727=CARTESIAN_POINT('',(7.01125,-8.5868812060852E-16,79.2264656430895));
#141728=CARTESIAN_POINT('Ctrl Pts',(6.57110895151812,2.44502632087642,79.3399816340719));
#141729=CARTESIAN_POINT('Ctrl Pts',(6.58708418927795,2.40209221135377,79.3378986371194));
#141730=CARTESIAN_POINT('Ctrl Pts',(6.60263458483066,2.35901238930181,79.3358156401668));
#141731=CARTESIAN_POINT('Ctrl Pts',(6.6177575476705,2.31579610560822,79.3337326432143));
#141732=CARTESIAN_POINT('Ctrl Pts',(6.69106165165094,2.10631791095325,79.3236359295732));
#141733=CARTESIAN_POINT('Ctrl Pts',(6.75435454450706,1.89353185207257,79.3135392159322));
#141734=CARTESIAN_POINT('Ctrl Pts',(6.80741833042684,1.67829742211227,79.3034425022911));
#141735=CARTESIAN_POINT('Ctrl Pts',(6.86056137941765,1.46274148961281,79.2933307068665));
#141736=CARTESIAN_POINT('Ctrl Pts',(6.90344478033023,1.24472979699255,79.283218911442));
#141737=CARTESIAN_POINT('Ctrl Pts',(6.9359012343375,1.02513444484885,79.2731071160174));
#141738=CARTESIAN_POINT('Ctrl Pts',(6.96825526148659,0.806232096998995,
79.26302723164));
#141739=CARTESIAN_POINT('Ctrl Pts',(6.99024806641698,0.585755995141008,
79.2529473472627));
#141740=CARTESIAN_POINT('Ctrl Pts',(7.00176464561119,0.364579771749844,
79.2428674628853));
#141741=CARTESIAN_POINT('Ctrl Pts',(7.00801117416039,0.244615017414701,
79.2374001896201));
#141742=CARTESIAN_POINT('Ctrl Pts',(7.01117655918056,0.12444446885573,79.2319329163549));
#141743=CARTESIAN_POINT('Ctrl Pts',(7.01124873670978,0.00420885798236834,
79.2264656430896));
#141744=CARTESIAN_POINT('Ctrl Pts',(7.01125,-8.58630487052188E-16,79.2264656430895));
#141745=CARTESIAN_POINT('Ctrl Pts',(7.01125,-0.191009525814093,79.2177938341507));
#141746=CARTESIAN_POINT('Ctrl Pts',(7.00344006572044,-0.382018909627989,
79.209122025212));
#141747=CARTESIAN_POINT('Ctrl Pts',(6.98784625534326,-0.572390840409932,
79.2004502162732));
#141748=CARTESIAN_POINT('Ctrl Pts',(6.9722524678609,-0.762762491687932,
79.1917784200664));
#141749=CARTESIAN_POINT('Ctrl Pts',(6.94887485033552,-0.952496408755896,
79.1831066238596));
#141750=CARTESIAN_POINT('Ctrl Pts',(6.91779140296556,-1.14095953808881,
79.1744348276528));
#141751=CARTESIAN_POINT('Ctrl Pts',(6.88670800059848,-1.32942239456319,
79.165763044001));
#141752=CARTESIAN_POINT('Ctrl Pts',(6.8479188369279,-1.51661418677304,79.1570912603493));
#141753=CARTESIAN_POINT('Ctrl Pts',(6.8015533329142,-1.70191034488418,79.1484194766976));
#141754=CARTESIAN_POINT('Ctrl Pts',(6.75518789508329,-1.88720623850088,
79.1397477054241));
#141755=CARTESIAN_POINT('Ctrl Pts',(6.70124620748731,-2.07060622793265,
79.1310759341506));
#141756=CARTESIAN_POINT('Ctrl Pts',(6.63990824732713,-2.25149839652999,
79.1224041628771));
#141757=CARTESIAN_POINT('Ctrl Pts',(6.57857037347114,-2.43239031060713,
79.1137324038051));
#141758=CARTESIAN_POINT('Ctrl Pts',(6.50983633907366,-2.61077414195939,
79.105060644733));
#141759=CARTESIAN_POINT('Ctrl Pts',(6.43393547556444,-2.7860547120926,79.0963888856609));
#141760=CARTESIAN_POINT('Ctrl Pts',(6.35803471730222,-2.96133503917517,
79.0877171386134));
#141761=CARTESIAN_POINT('Ctrl Pts',(6.27496726266411,-3.13351185304295,
79.079045391566));
#141762=CARTESIAN_POINT('Ctrl Pts',(6.18501026583621,-3.30201068653642,
79.0703736445185));
#141763=CARTESIAN_POINT('Ctrl Pts',(6.09151188669053,-3.47714289831664,
79.0613605124455));
#141764=CARTESIAN_POINT('Ctrl Pts',(5.99057066119403,-3.64830137930616,
79.0523473803725));
#141765=CARTESIAN_POINT('Ctrl Pts',(5.88255038916835,-3.8148692613765,79.0433342482995));
#141766=CARTESIAN_POINT('Ctrl Pts',(5.77621793389306,-3.97883452028952,
79.0344619464151));
#141767=CARTESIAN_POINT('Ctrl Pts',(5.66302622906641,-4.13835132493379,
79.0255896445307));
#141768=CARTESIAN_POINT('Ctrl Pts',(5.54337059053176,-4.29286257158642,
79.0167173426464));
#141769=CARTESIAN_POINT('Ctrl Pts',(5.42558457134922,-4.44495958001011,
79.0079836704789));
#141770=CARTESIAN_POINT('Ctrl Pts',(5.30153533575225,-4.59220608123771,
78.9992499983115));
#141771=CARTESIAN_POINT('Ctrl Pts',(5.17164269972606,-4.73410375349655,
78.9905163261441));
#141772=CARTESIAN_POINT('Ctrl Pts',(5.04265587431879,-4.8750118976169,78.9818435585301));
#141773=CARTESIAN_POINT('Ctrl Pts',(4.90790710164428,-5.01064538261667,
78.9731707909161));
#141774=CARTESIAN_POINT('Ctrl Pts',(4.76784607609543,-5.14055156157016,
78.9644980233021));
#141775=CARTESIAN_POINT('Ctrl Pts',(4.62778576967683,-5.27045707353252,
78.9558253002177));
#141776=CARTESIAN_POINT('Ctrl Pts',(4.48241347330112,-5.39463514506226,
78.9471525771332));
#141777=CARTESIAN_POINT('Ctrl Pts',(4.33221433005818,-5.512671363408,78.9384798540487));
#141778=CARTESIAN_POINT('Ctrl Pts',(4.18201594573821,-5.6307069853429,78.9298071747856));
#141779=CARTESIAN_POINT('Ctrl Pts',(4.0269909867681,-5.74260064062323,78.9211344955224));
#141780=CARTESIAN_POINT('Ctrl Pts',(3.86765680432281,-5.84797891638432,
78.9124618162593));
#141781=CARTESIAN_POINT('Ctrl Pts',(3.70832341395226,-5.95335666829377,
78.9037891801094));
#141782=CARTESIAN_POINT('Ctrl Pts',(3.5446810799691,-6.05221894875703,78.8951165439595));
#141783=CARTESIAN_POINT('Ctrl Pts',(3.37727590613261,-6.14423583664854,
78.8864439078096));
#141784=CARTESIAN_POINT('Ctrl Pts',(3.20987155082895,-6.23625227462061,
78.8777713140648));
#141785=CARTESIAN_POINT('Ctrl Pts',(3.0387046414846,-6.32142325013534,78.86909872032));
#141786=CARTESIAN_POINT('Ctrl Pts',(2.86434638713337,-6.39946453517918,
78.8604261265752));
#141787=CARTESIAN_POINT('Ctrl Pts',(2.68998897108135,-6.47750544500735,
78.8517535745275));
#141788=CARTESIAN_POINT('Ctrl Pts',(2.51244050005896,-6.54841661688554,
78.8430810224798));
#141789=CARTESIAN_POINT('Ctrl Pts',(2.33229347361379,-6.61196141212564,
78.8344084704321));
#141790=CARTESIAN_POINT('Ctrl Pts',(2.15214729859692,-6.67550590703419,
78.8257359593735));
#141791=CARTESIAN_POINT('Ctrl Pts',(1.96940286067094,-6.73168400046285,
78.8170634483148));
#141792=CARTESIAN_POINT('Ctrl Pts',(1.7846699931603,-6.78030822146112,78.8083909372561));
#141793=CARTESIAN_POINT('Ctrl Pts',(1.59993798367519,-6.82893221661531,
78.7997184664786));
#141794=CARTESIAN_POINT('Ctrl Pts',(1.4132178378394,-6.87000233723,78.791045995701));
#141795=CARTESIAN_POINT('Ctrl Pts',(1.22513265046155,-6.90338153018309,
78.7823735249234));
#141796=CARTESIAN_POINT('Ctrl Pts',(1.03704832133025,-6.93676057082447,
78.7737010937189));
#141797=CARTESIAN_POINT('Ctrl Pts',(0.847599242854621,-6.96244870438779,
78.7650286625144));
#141798=CARTESIAN_POINT('Ctrl Pts',(0.657417610669254,-6.98036020902087,
78.75635623131));
#141799=CARTESIAN_POINT('Ctrl Pts',(0.467236830776379,-6.99827163338416,
78.7476838389707));
#141800=CARTESIAN_POINT('Ctrl Pts',(0.276323786589392,-7.00840647191844,
78.7390114466314));
#141801=CARTESIAN_POINT('Ctrl Pts',(0.0853155533234384,-7.01073090475317,
78.7303390542921));
#141802=CARTESIAN_POINT('Ctrl Pts',(-0.105691839532995,-7.01305532736071,
78.7216667001102));
#141803=CARTESIAN_POINT('Ctrl Pts',(-0.296794136559777,-7.00756940957919,
78.7129943459282));
#141804=CARTESIAN_POINT('Ctrl Pts',(-0.487353636612654,-6.99429145770895,
78.7043219917463));
#141805=CARTESIAN_POINT('Ctrl Pts',(-0.677912313780389,-6.98101356317634,
78.6956496750138));
#141806=CARTESIAN_POINT('Ctrl Pts',(-0.867927915266441,-6.95994372163514,
78.6869773582813));
#141807=CARTESIAN_POINT('Ctrl Pts',(-1.05676637165921,-6.93115224174381,
78.6783050415488));
#141808=CARTESIAN_POINT('Ctrl Pts',(-1.245604028008,-6.90236088383214,78.669632761558));
#141809=CARTESIAN_POINT('Ctrl Pts',(-1.4332642684094,-6.86584799585212,
78.6609604815671));
#141810=CARTESIAN_POINT('Ctrl Pts',(-1.61912088843568,-6.82173541784869,
78.6522882015763));
#141811=CARTESIAN_POINT('Ctrl Pts',(-1.80497673621616,-6.77762302313577,
78.6436159576193));
#141812=CARTESIAN_POINT('Ctrl Pts',(-1.98902870222326,-6.72591106719035,
78.6349437136623));
#141813=CARTESIAN_POINT('Ctrl Pts',(-2.17066262759744,-6.6667721064734,
78.6262714697053));
#141814=CARTESIAN_POINT('Ctrl Pts',(-2.35229581309165,-6.60763338665712,
78.6175992610744));
#141815=CARTESIAN_POINT('Ctrl Pts',(-2.53151070755275,-6.54106781055663,
78.6089270524435));
#141816=CARTESIAN_POINT('Ctrl Pts',(-2.70770929770338,-6.46729749753564,
78.6002548438127));
#141817=CARTESIAN_POINT('Ctrl Pts',(-2.88390718449131,-6.39352747899649,
78.5915826698002));
#141818=CARTESIAN_POINT('Ctrl Pts',(-3.05708852903999,-6.31255289079275,
78.5829104957876));
#141819=CARTESIAN_POINT('Ctrl Pts',(-3.22667545573402,-6.22464393084967,
78.5742383217751));
#141820=CARTESIAN_POINT('Ctrl Pts',(-3.39626171929477,-6.13673531465571,
78.5655661816733));
#141821=CARTESIAN_POINT('Ctrl Pts',(-3.56225334093939,-6.04189251170987,
78.5568940415715));
#141822=CARTESIAN_POINT('Ctrl Pts',(-3.72409644021767,-5.94043199325252,
78.5482219014696));
#141823=CARTESIAN_POINT('Ctrl Pts',(-3.88593891984732,-5.83897186325703,
78.5395497945708));
#141824=CARTESIAN_POINT('Ctrl Pts',(-4.04363266822696,-5.73089421932905,
78.530877687672));
#141825=CARTESIAN_POINT('Ctrl Pts',(-4.19665149725545,-5.6165596919363,
78.5222055807732));
#141826=CARTESIAN_POINT('Ctrl Pts',(-4.34966975290526,-5.50222559296783,
78.5135335063697));
#141827=CARTESIAN_POINT('Ctrl Pts',(-4.49801289671559,-5.38163482746919,
78.5048614319663));
#141828=CARTESIAN_POINT('Ctrl Pts',(-4.64118594512765,-5.2551897763306,
78.4961893575628));
#141829=CARTESIAN_POINT('Ctrl Pts',(-4.78435846873431,-5.12874518868039,
78.4875173149472));
#141830=CARTESIAN_POINT('Ctrl Pts',(-4.9223607219674,-4.99644654635617,
78.4788452723314));
#141831=CARTESIAN_POINT('Ctrl Pts',(-5.05473222957746,-4.85873529323948,
78.4701732297158));
#141832=CARTESIAN_POINT('Ctrl Pts',(-5.18710326277472,-4.72102453367296,
78.4615012181802));
#141833=CARTESIAN_POINT('Ctrl Pts',(-5.31384339389808,-4.57790140690643,
78.4528292066447));
#141834=CARTESIAN_POINT('Ctrl Pts',(-5.43452972930466,-4.4298434717046,
78.4441571951092));
#141835=CARTESIAN_POINT('Ctrl Pts',(-5.55521564202289,-4.28178605505662,
78.4354852139463));
#141836=CARTESIAN_POINT('Ctrl Pts',(-5.66984762199742,-4.1287940847157,
78.4268132327833));
#141837=CARTESIAN_POINT('Ctrl Pts',(-5.77804317951531,-3.97137804523274,
78.4181412516204));
#141838=CARTESIAN_POINT('Ctrl Pts',(-5.88623836691802,-3.81396254423831,
78.4094693001226));
#141839=CARTESIAN_POINT('Ctrl Pts',(-5.98799701504367,-3.65212323845438,
78.4007973486247));
#141840=CARTESIAN_POINT('Ctrl Pts',(-6.08297959063027,-3.486400129428,78.3921253971269));
#141841=CARTESIAN_POINT('Ctrl Pts',(-6.17796184904904,-3.32067757378774,
78.3834534745867));
#141842=CARTESIAN_POINT('Ctrl Pts',(-6.26616793897602,-3.15107148727402,
78.3747815520464));
#141843=CARTESIAN_POINT('Ctrl Pts',(-6.34730354929188,-2.97814778270769,
78.3661096295061));
#141844=CARTESIAN_POINT('Ctrl Pts',(-6.42843889529631,-2.80522464146629,
78.357437735216));
#141845=CARTESIAN_POINT('Ctrl Pts',(-6.50250368714091,-2.62898416091975,
78.3487658409258));
#141846=CARTESIAN_POINT('Ctrl Pts',(-6.56925079959966,-2.45001438658209,
78.3400939466356));
#141847=CARTESIAN_POINT('Ctrl Pts',(-6.63599770006415,-2.27104518066701,
78.3314220798881));
#141848=CARTESIAN_POINT('Ctrl Pts',(-6.69542686840661,-2.08934696441408,
78.3227502131406));
#141849=CARTESIAN_POINT('Ctrl Pts',(-6.7473400140075,-1.90552598981838,
78.314078346393));
#141850=CARTESIAN_POINT('Ctrl Pts',(-6.79925299896266,-1.72170558405843,
78.3054065064807));
#141851=CARTESIAN_POINT('Ctrl Pts',(-6.84364993053112,-1.53576270641729,
78.2967346665683));
#141852=CARTESIAN_POINT('Ctrl Pts',(-6.88038267538234,-1.34831776773821,
78.288062826656));
#141853=CARTESIAN_POINT('Ctrl Pts',(-6.91711530955977,-1.16087339382071,
78.2793910128714));
#141854=CARTESIAN_POINT('Ctrl Pts',(-6.94618374861324,-0.971927246623025,
78.2707191990868));
#141855=CARTESIAN_POINT('Ctrl Pts',(-6.96749100433623,-0.78210975380297,
78.2620473853023));
#141856=CARTESIAN_POINT('Ctrl Pts',(-6.98879819759952,-0.592292817410386,
78.2533755969381));
#141857=CARTESIAN_POINT('Ctrl Pts',(-7.00234422137931,-0.401604822732526,
78.2447038085739));
#141858=CARTESIAN_POINT('Ctrl Pts',(-7.00808387899837,-0.21068200545643,
78.2360320202097));
#141859=CARTESIAN_POINT('Ctrl Pts',(-7.01382352026046,-0.0197597322755547,
78.2273602565586));
#141860=CARTESIAN_POINT('Ctrl Pts',(-7.01175683134613,0.171397078298468,
78.2186884929074));
#141861=CARTESIAN_POINT('Ctrl Pts',(-7.00189070777997,0.362150629993181,
78.2100167292563));
#141862=CARTESIAN_POINT('Ctrl Pts',(-6.99157808297303,0.561536923508558,
78.2009525163109));
#141863=CARTESIAN_POINT('Ctrl Pts',(-6.97274368607599,0.760482277939237,
78.1918883033655));
#141864=CARTESIAN_POINT('Ctrl Pts',(-6.94545616842894,0.95826153785511,
78.1828240904202));
#141865=CARTESIAN_POINT('Ctrl Pts',(-6.91902138570836,1.1498601958986,78.1740431341294));
#141866=CARTESIAN_POINT('Ctrl Pts',(-6.88465388689399,1.3403642279907,78.1652621778385));
#141867=CARTESIAN_POINT('Ctrl Pts',(-6.84247124235356,1.5291219245255,78.1564812215477));
#141868=CARTESIAN_POINT('Ctrl Pts',(-6.80080846652437,1.7155533273558,78.1478084838022));
#141869=CARTESIAN_POINT('Ctrl Pts',(-6.75152215882668,1.90028091508163,
78.1391357460567));
#141870=CARTESIAN_POINT('Ctrl Pts',(-6.69477680034086,2.08268820424897,
78.1304630083112));
#141871=CARTESIAN_POINT('Ctrl Pts',(-6.63803201373298,2.26509365512142,
78.1217903579693));
#141872=CARTESIAN_POINT('Ctrl Pts',(-6.57382841116829,2.44517858291205,
78.1131177076274));
#141873=CARTESIAN_POINT('Ctrl Pts',(-6.50238025226108,2.62234201001799,
78.1044450572855));
#141874=CARTESIAN_POINT('Ctrl Pts',(-6.43093279007886,2.79950370951906,
78.0957724915147));
#141875=CARTESIAN_POINT('Ctrl Pts',(-6.35224101919167,2.97374370183801,
78.087099925744));
#141876=CARTESIAN_POINT('Ctrl Pts',(-6.26656754386633,3.14448052636062,
78.0784273599732));
#141877=CARTESIAN_POINT('Ctrl Pts',(-6.18089487601409,3.31521574168748,
78.0697548759414));
#141878=CARTESIAN_POINT('Ctrl Pts',(-6.08824076282435,3.48244760135076,
78.0610823919096));
#141879=CARTESIAN_POINT('Ctrl Pts',(-5.98891439682134,3.64561804225924,
78.0524099078778));
#141880=CARTESIAN_POINT('Ctrl Pts',(-5.88958893454527,3.80878699855161,
78.0437375027532));
#141881=CARTESIAN_POINT('Ctrl Pts',(-5.78359148866223,3.96789436736006,
78.0350650976285));
#141882=CARTESIAN_POINT('Ctrl Pts',(-5.67127577279528,4.1224092071755,78.0263926925039));
#141883=CARTESIAN_POINT('Ctrl Pts',(-5.55896104217726,4.27692269156547,
78.0177203634547));
#141884=CARTESIAN_POINT('Ctrl Pts',(-5.44032831952208,4.42684349778465,
78.0090480344056));
#141885=CARTESIAN_POINT('Ctrl Pts',(-5.31577347545041,4.57167134866428,
78.0003757053565));
#141886=CARTESIAN_POINT('Ctrl Pts',(-5.19121968333579,4.71649797636645,
77.9917034495515));
#141887=CARTESIAN_POINT('Ctrl Pts',(-5.06074405512509,4.85623151942303,
77.9830311937466));
#141888=CARTESIAN_POINT('Ctrl Pts',(-4.92478197319156,4.99040570284897,
77.9743589379416));
#141889=CARTESIAN_POINT('Ctrl Pts',(-4.78882099518222,5.12457879686728,
77.9656867525498));
#141890=CARTESIAN_POINT('Ctrl Pts',(-4.64737385478172,5.25319242205071,
77.9570145671579));
#141891=CARTESIAN_POINT('Ctrl Pts',(-4.50091253739826,5.3758174162811,77.9483423817661));
#141892=CARTESIAN_POINT('Ctrl Pts',(-4.35445236138621,5.49844145489627,
77.9396702639565));
#141893=CARTESIAN_POINT('Ctrl Pts',(-4.20297830438142,5.61507677359828,
77.9309981461469));
#141894=CARTESIAN_POINT('Ctrl Pts',(-4.04699580206287,5.72533418593059,
77.9223260283373));
#141895=CARTESIAN_POINT('Ctrl Pts',(-3.89101446441063,5.83559077500971,
77.9136539752794));
#141896=CARTESIAN_POINT('Ctrl Pts',(-3.73052498075555,5.93946938906078,
77.9049819222214));
#141897=CARTESIAN_POINT('Ctrl Pts',(-3.56606286128741,6.0366234131215,77.8963098691635));
#141898=CARTESIAN_POINT('Ctrl Pts',(-3.40160191613153,6.13377674347135,
77.8876378780268));
#141899=CARTESIAN_POINT('Ctrl Pts',(-3.23316863647579,6.22420543545029,
77.8789658868901));
#141900=CARTESIAN_POINT('Ctrl Pts',(-3.06132503080019,6.30760775716882,
77.8702938957534));
#141901=CARTESIAN_POINT('Ctrl Pts',(-2.8894825960697,6.39100951058258,77.8616219637077));
#141902=CARTESIAN_POINT('Ctrl Pts',(-2.71423013734018,6.46738486553112,
77.8529500316621));
#141903=CARTESIAN_POINT('Ctrl Pts',(-2.53615240857015,6.53647898512677,
77.8442780996165));
#141904=CARTESIAN_POINT('Ctrl Pts',(-2.35807583511879,6.60557265645903,
77.8356062238319));
#141905=CARTESIAN_POINT('Ctrl Pts',(-2.17717429308822,6.66738508423251,
77.8269343480474));
#141906=CARTESIAN_POINT('Ctrl Pts',(-1.99405137755703,6.72171002544464,
77.8182624722629));
#141907=CARTESIAN_POINT('Ctrl Pts',(-1.81092959032806,6.77603463193649,
77.8095906499096));
#141908=CARTESIAN_POINT('Ctrl Pts',(-1.62558672926414,6.82287176341229,
77.8009188275564));
#141909=CARTESIAN_POINT('Ctrl Pts',(-1.43864120071127,6.8620651452836,77.7922470052032));
#141910=CARTESIAN_POINT('Ctrl Pts',(-1.25169676302043,6.90125829845422,
77.7835752334516));
#141911=CARTESIAN_POINT('Ctrl Pts',(-1.06314995450863,6.93280773300164,
77.7749034617001));
#141912=CARTESIAN_POINT('Ctrl Pts',(-0.873629864329032,6.95660818378126,
77.7662316899485));
#141913=CARTESIAN_POINT('Ctrl Pts',(-0.679495509716173,6.98098810649668,
77.7573487857101));
#141914=CARTESIAN_POINT('Ctrl Pts',(-0.484340182091174,6.99723686027452,
77.7484658814716));
#141915=CARTESIAN_POINT('Ctrl Pts',(-0.288847078975853,7.00529756166482,
77.7395829772331));
#141916=CARTESIAN_POINT('Ctrl Pts',(-0.0979805524013863,7.01316749698021,
77.7309102974768));
#141917=CARTESIAN_POINT('Ctrl Pts',(0.0932076478821179,7.01323255451612,
77.7222376177204));
#141918=CARTESIAN_POINT('Ctrl Pts',(0.28407948621932,7.00549251716176,77.7135649379641));
#141919=CARTESIAN_POINT('Ctrl Pts',(0.474947621910944,6.99775262995324,
77.7048924264455));
#141920=CARTESIAN_POINT('Ctrl Pts',(0.665499124046535,6.98220796234756,
77.696219914927));
#141921=CARTESIAN_POINT('Ctrl Pts',(0.855098106414399,6.95891038819344,
77.6875474034084));
#141922=CARTESIAN_POINT('Ctrl Pts',(1.04469365841084,6.93561323555704,77.6788750487997));
#141923=CARTESIAN_POINT('Ctrl Pts',(1.2333364431492,6.90456349171748,77.6702026941909));
#141924=CARTESIAN_POINT('Ctrl Pts',(1.4203969667229,6.86586476850691,77.6615303395822));
#141925=CARTESIAN_POINT('Ctrl Pts',(1.60745435008764,6.82716669493675,77.6528581305574));
#141926=CARTESIAN_POINT('Ctrl Pts',(1.79292924725751,6.78081995649478,77.6441859215326));
#141927=CARTESIAN_POINT('Ctrl Pts',(1.97620275620699,6.72697920532388,77.6355137125077));
#141928=CARTESIAN_POINT('Ctrl Pts',(2.15947342778097,6.6731392876964,77.626841637743));
#141929=CARTESIAN_POINT('Ctrl Pts',(2.34054250680043,6.61180566956937,77.6181695629782));
#141930=CARTESIAN_POINT('Ctrl Pts',(2.51880581148603,6.54318300573385,77.6094974882134));
#141931=CARTESIAN_POINT('Ctrl Pts',(2.69706658905484,6.47456131471483,77.6008255363868));
#141932=CARTESIAN_POINT('Ctrl Pts',(2.87252140681634,6.39865088680259,77.5921535845601));
#141933=CARTESIAN_POINT('Ctrl Pts',(3.04458483294514,6.31570500874609,77.5834816327334));
#141934=CARTESIAN_POINT('Ctrl Pts',(3.21664604442449,6.23276019829615,77.5748097925244));
#141935=CARTESIAN_POINT('Ctrl Pts',(3.38531569578518,6.14278024223941,77.5661379523155));
#141936=CARTESIAN_POINT('Ctrl Pts',(3.55003100941986,6.04606536473576,77.5574661121066));
#141937=CARTESIAN_POINT('Ctrl Pts',(3.72225670715806,5.94494066119623,77.548398869373));
#141938=CARTESIAN_POINT('Ctrl Pts',(3.89015872998388,5.83645264819801,77.5393316266395));
#141939=CARTESIAN_POINT('Ctrl Pts',(4.05312466659611,5.72099702844969,77.5302643839059));
#141940=CARTESIAN_POINT('Ctrl Pts',(4.20899688867782,5.6105670553148,77.5215918275275));
#141941=CARTESIAN_POINT('Ctrl Pts',(4.36035338103661,5.4937633625381,77.5129192711491));
#141942=CARTESIAN_POINT('Ctrl Pts',(4.50668904924836,5.37097573778591,77.5042467147706));
#141943=CARTESIAN_POINT('Ctrl Pts',(4.65301950883883,5.24819248349408,77.4955744670802));
#141944=CARTESIAN_POINT('Ctrl Pts',(4.794329284268,5.11942590604149,77.4869022193897));
#141945=CARTESIAN_POINT('Ctrl Pts',(4.93014684172369,4.98510568408955,77.4782299716993));
#141946=CARTESIAN_POINT('Ctrl Pts',(5.06596027419711,4.85078954164356,77.469557987398));
#141947=CARTESIAN_POINT('Ctrl Pts',(5.19628162053286,4.71092029195721,77.4608860030966));
#141948=CARTESIAN_POINT('Ctrl Pts',(5.32067604038009,4.56596463365905,77.4522140187953));
#141949=CARTESIAN_POINT('Ctrl Pts',(5.44506733164208,4.42101262107213,77.443542252599));
#141950=CARTESIAN_POINT('Ctrl Pts',(5.56353180975496,4.27097467138821,77.4348704864026));
#141951=CARTESIAN_POINT('Ctrl Pts',(5.67567421678027,4.11635138775539,77.4261987202063));
#141952=CARTESIAN_POINT('Ctrl Pts',(5.78782406005978,3.9617178509269,77.4175263789781));
#141953=CARTESIAN_POINT('Ctrl Pts',(5.89365082654157,3.80249860162573,77.4088540377499));
#141954=CARTESIAN_POINT('Ctrl Pts',(5.99280137735851,3.63922494688497,77.4001816965217));
#141955=CARTESIAN_POINT('Ctrl Pts',(6.09194609290756,3.47596090122362,77.3915098656833));
#141956=CARTESIAN_POINT('Ctrl Pts',(6.18441523160385,3.30864317036959,77.3828380348449));
#141957=CARTESIAN_POINT('Ctrl Pts',(6.26990026462871,3.1378300199515,77.3741662040066));
#141958=CARTESIAN_POINT('Ctrl Pts',(6.35538670852299,2.96701405038435,77.3654942300458));
#141959=CARTESIAN_POINT('Ctrl Pts',(6.43388868896941,2.79270279979814,77.3568222560851));
#141960=CARTESIAN_POINT('Ctrl Pts',(6.50514427077197,2.61547788729758,77.3481502821244));
#141961=CARTESIAN_POINT('Ctrl Pts',(6.52787183386155,2.55895052090738,77.3453842835834));
#141962=CARTESIAN_POINT('Ctrl Pts',(6.5498625512969,2.50212689664082,77.3426182850423));
#141963=CARTESIAN_POINT('Ctrl Pts',(6.57110895151816,2.4450263208763,77.3398522865014));
#141964=CARTESIAN_POINT('Origin',(0.,0.,50.));
#141965=CARTESIAN_POINT('',(6.57110895151811,2.44502632087644,75.339916226746));
#141966=CARTESIAN_POINT('',(6.57110895151814,2.44502632087635,75.8870038120088));
#141967=CARTESIAN_POINT('',(6.57110895151814,2.44502632087636,50.));
#141968=CARTESIAN_POINT('',(7.01124789938016,-0.00542733243554445,77.7735343569458));
#141969=CARTESIAN_POINT('Ctrl Pts',(6.57110895151814,2.44502632087635,75.8870038120088));
#141970=CARTESIAN_POINT('Ctrl Pts',(6.50691177316196,2.61755888208302,75.895378926296));
#141971=CARTESIAN_POINT('Ctrl Pts',(6.43587702619422,2.78766482296899,75.9037540405832));
#141972=CARTESIAN_POINT('Ctrl Pts',(6.35821200936702,2.954787066176,75.9121291548703));
#141973=CARTESIAN_POINT('Ctrl Pts',(6.28059487615379,3.12180627178249,75.9204991055619));
#141974=CARTESIAN_POINT('Ctrl Pts',(6.19635576211538,3.28584515032049,75.9288690562535));
#141975=CARTESIAN_POINT('Ctrl Pts',(6.10575007356766,3.44636657969353,75.9372390069451));
#141976=CARTESIAN_POINT('Ctrl Pts',(6.0151869665541,3.6068125695568,75.9456050240498));
#141977=CARTESIAN_POINT('Ctrl Pts',(5.91826341307935,3.76374412102792,75.9539710411546));
#141978=CARTESIAN_POINT('Ctrl Pts',(5.81528096216037,3.91664829843517,75.9623370582594));
#141979=CARTESIAN_POINT('Ctrl Pts',(5.71232566496845,4.06951215908689,75.9707008694685));
#141980=CARTESIAN_POINT('Ctrl Pts',(5.6033148379879,4.21835048985813,75.9790646806775));
#141981=CARTESIAN_POINT('Ctrl Pts',(5.4885938955949,4.36267849053061,75.9874284918866));
#141982=CARTESIAN_POINT('Ctrl Pts',(5.37388930617439,4.50698591787292,75.9957911108707));
#141983=CARTESIAN_POINT('Ctrl Pts',(5.25347642868758,4.6467840397992,76.0041537298548));
#141984=CARTESIAN_POINT('Ctrl Pts',(5.12774183317567,4.78162004500569,76.0125163488389));
#141985=CARTESIAN_POINT('Ctrl Pts',(5.00200840094346,4.91645480272745,76.0208788904531));
#141986=CARTESIAN_POINT('Ctrl Pts',(4.87095357332457,5.04632729521203,76.0292414320674));
#141987=CARTESIAN_POINT('Ctrl Pts',(4.73500203658974,5.17082027109733,76.0376039736816));
#141988=CARTESIAN_POINT('Ctrl Pts',(4.5990336361189,5.29532868937284,76.0459675526045));
#141989=CARTESIAN_POINT('Ctrl Pts',(4.45816755827911,5.41445603912424,76.0543311315273));
#141990=CARTESIAN_POINT('Ctrl Pts',(4.31286325154248,5.52782390602256,76.0626947104501));
#141991=CARTESIAN_POINT('Ctrl Pts',(4.16747266331511,5.64125909059903,76.0710632556542));
#141992=CARTESIAN_POINT('Ctrl Pts',(4.01763883908727,5.74892775566056,76.0794318008583));
#141993=CARTESIAN_POINT('Ctrl Pts',(3.8638528494694,5.85049294676502,76.0878003460624));
#141994=CARTESIAN_POINT('Ctrl Pts',(3.71001917849709,5.9520896281625,76.0961714859343));
#141995=CARTESIAN_POINT('Ctrl Pts',(3.55223117598703,6.04757888555163,76.1045426258063));
#141996=CARTESIAN_POINT('Ctrl Pts',(3.39100704846998,6.13666829474487,76.1129137656783));
#141997=CARTESIAN_POINT('Ctrl Pts',(3.2296486081688,6.225831922647,76.1212918793892));
#141998=CARTESIAN_POINT('Ctrl Pts',(3.06484861387916,6.30858489553324,76.1296699931002));
#141999=CARTESIAN_POINT('Ctrl Pts',(2.89714890824418,6.38468125797675,76.1380481068111));
#142000=CARTESIAN_POINT('Ctrl Pts',(2.80482730357157,6.42657362900944,76.1426604041255));
#142001=CARTESIAN_POINT('Ctrl Pts',(2.71162725246564,6.46644942872256,76.1472727014399));
#142002=CARTESIAN_POINT('Ctrl Pts',(2.61764153474929,6.50427393012129,76.1518849987543));
#142003=CARTESIAN_POINT('Ctrl Pts',(2.45741902907857,6.56875539110389,76.1597478299436));
#142004=CARTESIAN_POINT('Ctrl Pts',(2.29457898084834,6.62740651627268,76.1676106611329));
#142005=CARTESIAN_POINT('Ctrl Pts',(2.12960305163939,6.68000130276546,76.1754734923222));
#142006=CARTESIAN_POINT('Ctrl Pts',(1.96475388465543,6.73255567710726,76.1833302819636));
#142007=CARTESIAN_POINT('Ctrl Pts',(1.7977724612511,6.77906285186163,76.191187071605));
#142008=CARTESIAN_POINT('Ctrl Pts',(1.62916110100275,6.81934459236953,76.1990438612465));
#142009=CARTESIAN_POINT('Ctrl Pts',(1.46064482958017,6.85960361588256,76.2068962200304));
#142010=CARTESIAN_POINT('Ctrl Pts',(1.2905008195074,6.89364410071723,76.2147485788144));
#142011=CARTESIAN_POINT('Ctrl Pts',(1.11924701355265,6.92133749250486,76.2226009375983));
#142012=CARTESIAN_POINT('Ctrl Pts',(0.948033642619447,6.94902434555961,
76.2304514423488));
#142013=CARTESIAN_POINT('Ctrl Pts',(0.775711372021637,6.97036701910394,
76.2383019470992));
#142014=CARTESIAN_POINT('Ctrl Pts',(0.602808751726681,6.98528798055898,
76.2461524518497));
#142015=CARTESIAN_POINT('Ctrl Pts',(0.42993394601388,7.00020654170159,76.2540016937013));
#142016=CARTESIAN_POINT('Ctrl Pts',(0.256479356831333,7.00870541744972,
76.261850935553));
#142017=CARTESIAN_POINT('Ctrl Pts',(0.0829786088306314,7.01075895413446,
76.2697001774047));
#142018=CARTESIAN_POINT('Ctrl Pts',(-0.0905805949680287,7.0128131826959,
76.2775520638195));
#142019=CARTESIAN_POINT('Ctrl Pts',(-0.264185606812616,7.00841773011404,
76.2854039502344));
#142020=CARTESIAN_POINT('Ctrl Pts',(-0.43730264539801,6.9975990853169,76.2932558366493));
#142021=CARTESIAN_POINT('Ctrl Pts',(-0.564420332083106,6.98965508909955,
76.2990213791131));
#142022=CARTESIAN_POINT('Ctrl Pts',(-0.691274897770224,6.97824893703673,
76.3047869215769));
#142023=CARTESIAN_POINT('Ctrl Pts',(-0.817656948322948,6.96340891211763,
76.3105524640407));
#142024=CARTESIAN_POINT('Ctrl Pts',(-1.02930349699573,6.93855696484656,
76.3202077684005));
#142025=CARTESIAN_POINT('Ctrl Pts',(-1.23951683000672,6.90408683421318,
76.3298630727602));
#142026=CARTESIAN_POINT('Ctrl Pts',(-1.44751734984712,6.86019825401508,
76.3395183771199));
#142027=CARTESIAN_POINT('Ctrl Pts',(-1.65667015354632,6.81606653931623,
76.3492271700545));
#142028=CARTESIAN_POINT('Ctrl Pts',(-1.86358552416067,6.76241179639644,
76.358935962989));
#142029=CARTESIAN_POINT('Ctrl Pts',(-2.06749234383549,6.69948520191527,
76.3686447559236));
#142030=CARTESIAN_POINT('Ctrl Pts',(-2.27238038044039,6.63625579931833,
76.3784002683941));
#142031=CARTESIAN_POINT('Ctrl Pts',(-2.47423080736855,6.56366513227131,
76.3881557808646));
#142032=CARTESIAN_POINT('Ctrl Pts',(-2.67228348793353,6.4820156990413,76.3979112933351));
#142033=CARTESIAN_POINT('Ctrl Pts',(-2.87053227112194,6.40028542031092,
76.4076764652639));
#142034=CARTESIAN_POINT('Ctrl Pts',(-3.06497575519559,6.30947845915102,
76.4174416371926));
#142035=CARTESIAN_POINT('Ctrl Pts',(-3.25487414386932,6.20994531941071,
76.4272068091213));
#142036=CARTESIAN_POINT('Ctrl Pts',(-3.44451361039866,6.11054789084815,
76.4369586664596));
#142037=CARTESIAN_POINT('Ctrl Pts',(-3.62962033378246,6.00244808107711,
76.446710523798));
#142038=CARTESIAN_POINT('Ctrl Pts',(-3.80948051215684,5.88604152126004,
76.4564623811363));
#142039=CARTESIAN_POINT('Ctrl Pts',(-3.88791257603977,5.8352798306041,76.4607148971999));
#142040=CARTESIAN_POINT('Ctrl Pts',(-3.9653472594436,5.78293913193116,76.4649674132635));
#142041=CARTESIAN_POINT('Ctrl Pts',(-4.04172677262675,5.72905500566474,
76.4692199293271));
#142042=CARTESIAN_POINT('Ctrl Pts',(-4.18600844094889,5.62726734939678,
76.477252974926));
#142043=CARTESIAN_POINT('Ctrl Pts',(-4.3265931194642,5.51991943857155,76.4852860205249));
#142044=CARTESIAN_POINT('Ctrl Pts',(-4.46302109857391,5.40731626929516,
76.4933190661238));
#142045=CARTESIAN_POINT('Ctrl Pts',(-4.59936137652575,5.29478548567155,
76.5013469477717));
#142046=CARTESIAN_POINT('Ctrl Pts',(-4.7315499923933,5.17700640051699,76.5093748294196));
#142047=CARTESIAN_POINT('Ctrl Pts',(-4.85915744024665,5.05432641737706,
76.5174027110675));
#142048=CARTESIAN_POINT('Ctrl Pts',(-4.98670727207932,4.93170182545892,
76.5254269680476));
#142049=CARTESIAN_POINT('Ctrl Pts',(-5.10967979069723,4.8041809950259,76.5334512250278));
#142050=CARTESIAN_POINT('Ctrl Pts',(-5.22767977197113,4.67215055025241,
76.541475482008));
#142051=CARTESIAN_POINT('Ctrl Pts',(-5.34566548584541,4.54013606930449,
76.5494987687738));
#142052=CARTESIAN_POINT('Ctrl Pts',(-5.45867961004383,4.40361332809949,
76.5575220555395));
#142053=CARTESIAN_POINT('Ctrl Pts',(-5.56636478781921,4.26300476324229,
76.5655453423053));
#142054=CARTESIAN_POINT('Ctrl Pts',(-5.67404114175487,4.12240772000269,
76.5735679716343));
#142055=CARTESIAN_POINT('Ctrl Pts',(-5.77638919931279,3.97772581352337,
76.5815906009633));
#142056=CARTESIAN_POINT('Ctrl Pts',(-5.87309299960993,3.82941316397603,
76.5896132302923));
#142057=CARTESIAN_POINT('Ctrl Pts',(-5.96983315365138,3.68104475943121,
76.5976388755588));
#142058=CARTESIAN_POINT('Ctrl Pts',(-6.0609246138721,3.52904319411107,76.6056645208253));
#142059=CARTESIAN_POINT('Ctrl Pts',(-6.14609552710443,3.37389038562413,
76.6136901660917));
#142060=CARTESIAN_POINT('Ctrl Pts',(-6.19631748759975,3.28240283520521,
76.618422575599));
#142061=CARTESIAN_POINT('Ctrl Pts',(-6.24448173017626,3.18982009089237,
76.6231549851063));
#142062=CARTESIAN_POINT('Ctrl Pts',(-6.29054013873538,3.09624471343256,
76.6278873946135));
#142063=CARTESIAN_POINT('Ctrl Pts',(-6.37550576889593,2.9236227935245,76.6366174434481));
#142064=CARTESIAN_POINT('Ctrl Pts',(-6.45334528794706,2.74753552575064,
76.6453474922826));
#142065=CARTESIAN_POINT('Ctrl Pts',(-6.52380507287336,2.56857819301883,
76.6540775411171));
#142066=CARTESIAN_POINT('Ctrl Pts',(-6.59428523133428,2.38956911455122,
76.6628101142562));
#142067=CARTESIAN_POINT('Ctrl Pts',(-6.65738129601282,2.20768856953147,
76.6715426873952));
#142068=CARTESIAN_POINT('Ctrl Pts',(-6.71288843299128,2.02355020909092,
76.6802752605343));
#142069=CARTESIAN_POINT('Ctrl Pts',(-6.76918413745766,1.83679586929658,
76.6891318938148));
#142070=CARTESIAN_POINT('Ctrl Pts',(-6.81767356152349,1.64771935091506,
76.6979885270952));
#142071=CARTESIAN_POINT('Ctrl Pts',(-6.85819576343266,1.45697544005871,
76.7068451603757));
#142072=CARTESIAN_POINT('Ctrl Pts',(-6.89817578093152,1.26878367024989,
76.7155832924824));
#142073=CARTESIAN_POINT('Ctrl Pts',(-6.93040041898706,1.07896912657834,
76.724321424589));
#142074=CARTESIAN_POINT('Ctrl Pts',(-6.95476667447427,0.888170628945882,
76.7330595566956));
#142075=CARTESIAN_POINT('Ctrl Pts',(-6.97962859021963,0.693490893482653,
76.741975440563));
#142076=CARTESIAN_POINT('Ctrl Pts',(-6.99630894588668,0.497787037273467,
76.7508913244304));
#142077=CARTESIAN_POINT('Ctrl Pts',(-7.00475389972484,0.301743876142743,
76.7598072082978));
#142078=CARTESIAN_POINT('Ctrl Pts',(-7.013198853563,0.105700715012085,76.7687230921652));
#142079=CARTESIAN_POINT('Ctrl Pts',(-7.0134083986347,-0.0906814486463031,
76.7776389760326));
#142080=CARTESIAN_POINT('Ctrl Pts',(-7.005385105977,-0.286716025808756,
76.7865548598999));
#142081=CARTESIAN_POINT('Ctrl Pts',(-6.99751947304752,-0.478898473991935,
76.7952955443963));
#142082=CARTESIAN_POINT('Ctrl Pts',(-6.9817407183158,-0.670767280903081,
76.8040362288926));
#142083=CARTESIAN_POINT('Ctrl Pts',(-6.95809877101564,-0.861677465929471,
76.8127769133889));
#142084=CARTESIAN_POINT('Ctrl Pts',(-6.93446107729452,-1.05255330304236,
76.8215160252909));
#142085=CARTESIAN_POINT('Ctrl Pts',(-6.9029630499438,-1.24247059108854,
76.8302551371929));
#142086=CARTESIAN_POINT('Ctrl Pts',(-6.86370636760534,-1.43079050241251,
76.8389942490949));
#142087=CARTESIAN_POINT('Ctrl Pts',(-6.82394105844773,-1.62155036922371,
76.8478465887692));
#142088=CARTESIAN_POINT('Ctrl Pts',(-6.77621467986333,-1.8106708945318,
76.8566989284435));
#142089=CARTESIAN_POINT('Ctrl Pts',(-6.72068646462178,-1.99749843723333,
76.8655512681178));
#142090=CARTESIAN_POINT('Ctrl Pts',(-6.66589659214933,-2.18184178762613,
76.8742859007677));
#142091=CARTESIAN_POINT('Ctrl Pts',(-6.60351116548221,-2.3639524896423,
76.8830205334175));
#142092=CARTESIAN_POINT('Ctrl Pts',(-6.53373368134623,-2.54321661360998,
76.8917551660674));
#142093=CARTESIAN_POINT('Ctrl Pts',(-6.46254572575269,-2.72610435532991,
76.9006663592539));
#142094=CARTESIAN_POINT('Ctrl Pts',(-6.38366377114332,-2.90602893428911,
76.9095775524404));
#142095=CARTESIAN_POINT('Ctrl Pts',(-6.2973564506595,-3.08235758727588,
76.9184887456269));
#142096=CARTESIAN_POINT('Ctrl Pts',(-6.21104913017568,-3.25868624026265,
76.9273999388134));
#142097=CARTESIAN_POINT('Ctrl Pts',(-6.11731656498037,-3.43141868908865,
76.9363111319999));
#142098=CARTESIAN_POINT('Ctrl Pts',(-6.01647881569091,-3.59994572498566,
76.9452223251864));
#142099=CARTESIAN_POINT('Ctrl Pts',(-5.92566157457395,-3.7517257930815,
76.9532479900388));
#142100=CARTESIAN_POINT('Ctrl Pts',(-5.82903892466044,-3.90016421168517,
76.9612736548911));
#142101=CARTESIAN_POINT('Ctrl Pts',(-5.72689495486187,-4.04478685946215,
76.9692993197434));
#142102=CARTESIAN_POINT('Ctrl Pts',(-5.62478340305396,-4.189363607558,76.9773224374466));
#142103=CARTESIAN_POINT('Ctrl Pts',(-5.51715423131131,-4.330126696814,76.9853455551497));
#142104=CARTESIAN_POINT('Ctrl Pts',(-5.40433510896873,-4.46663056368758,
76.9933686728529));
#142105=CARTESIAN_POINT('Ctrl Pts',(-5.29153021410495,-4.60311721622875,
77.0013907787707));
#142106=CARTESIAN_POINT('Ctrl Pts',(-5.17353690624581,-4.73534543418048,
77.0094128846885));
#142107=CARTESIAN_POINT('Ctrl Pts',(-5.05072339346041,-4.86290240137018,
77.0174349906062));
#142108=CARTESIAN_POINT('Ctrl Pts',(-4.92786424275859,-4.99050676915997,
77.0254600775657));
#142109=CARTESIAN_POINT('Ctrl Pts',(-4.80018156119482,-5.11343615210699,
77.0334851645252));
#142110=CARTESIAN_POINT('Ctrl Pts',(-4.66808102020432,-5.23131399853882,
77.0415102514846));
#142111=CARTESIAN_POINT('Ctrl Pts',(-4.53595446267337,-5.34921506042259,
77.0495369189448));
#142112=CARTESIAN_POINT('Ctrl Pts',(-4.39940859175142,-5.46206236635242,
77.057563586405));
#142113=CARTESIAN_POINT('Ctrl Pts',(-4.25888229620412,-5.56951956182749,
77.0655902538652));
#142114=CARTESIAN_POINT('Ctrl Pts',(-4.11824318664188,-5.67706302356049,
77.0736233651057));
#142115=CARTESIAN_POINT('Ctrl Pts',(-3.97361756707955,-5.77920751717179,
77.0816564763462));
#142116=CARTESIAN_POINT('Ctrl Pts',(-3.82547395057441,-5.87565958986535,
77.0896895875867));
#142117=CARTESIAN_POINT('Ctrl Pts',(-3.73818235011123,-5.93249265491422,
77.0944229885488));
#142118=CARTESIAN_POINT('Ctrl Pts',(-3.64966982055057,-5.98735015673688,
77.0991563895108));
#142119=CARTESIAN_POINT('Ctrl Pts',(-3.56003617203288,-6.04017955166214,
77.1038897904728));
#142120=CARTESIAN_POINT('Ctrl Pts',(-3.37538806651773,-6.1490097493589,
77.113640743767));
#142121=CARTESIAN_POINT('Ctrl Pts',(-3.18587248217892,-6.2492954597494,
77.1233916970612));
#142122=CARTESIAN_POINT('Ctrl Pts',(-2.99222443154484,-6.34067973594047,
77.1331426503554));
#142123=CARTESIAN_POINT('Ctrl Pts',(-2.79829739456617,-6.43219566832475,
77.142907651727));
#142124=CARTESIAN_POINT('Ctrl Pts',(-2.60022601729286,-6.51478449787616,
77.1526726530986));
#142125=CARTESIAN_POINT('Ctrl Pts',(-2.39876794143145,-6.58813622549358,
77.1624376544703));
#142126=CARTESIAN_POINT('Ctrl Pts',(-2.19764565444117,-6.66136569097924,
77.1721863796079));
#142127=CARTESIAN_POINT('Ctrl Pts',(-1.99314798639645,-6.72538881258191,
77.1819351047455));
#142128=CARTESIAN_POINT('Ctrl Pts',(-1.7860475661107,-6.7799454757461,77.1916838298831));
#142129=CARTESIAN_POINT('Ctrl Pts',(-1.57951555617596,-6.83435240202412,
77.2014057985502));
#142130=CARTESIAN_POINT('Ctrl Pts',(-1.37039509353772,-6.87934472802349,
77.2111277672174));
#142131=CARTESIAN_POINT('Ctrl Pts',(-1.15947062925996,-6.91471289515216,
77.2208497358845));
#142132=CARTESIAN_POINT('Ctrl Pts',(-0.949941797071313,-6.94984704035668,
77.2305073768243));
#142133=CARTESIAN_POINT('Ctrl Pts',(-0.738632798804169,-6.97548393062048,
77.240165017764));
#142134=CARTESIAN_POINT('Ctrl Pts',(-0.52633001027022,-6.99146646153645,
77.2498226587038));
#142135=CARTESIAN_POINT('Ctrl Pts',(-0.433015625573714,-6.99849133411874,
77.2540675243889));
#142136=CARTESIAN_POINT('Ctrl Pts',(-0.339509473258997,-7.00365170974024,
77.2583123900741));
#142137=CARTESIAN_POINT('Ctrl Pts',(-0.245879369247421,-7.00693726946934,
77.2625572557593));
#142138=CARTESIAN_POINT('Ctrl Pts',(-0.0726891420112815,-7.01301466137325,
77.2704091027732));
#142139=CARTESIAN_POINT('Ctrl Pts',(0.100854183990988,-7.01267108832776,
77.2782609497872));
#142140=CARTESIAN_POINT('Ctrl Pts',(0.274217249885417,-7.00588548738597,
77.2861127968011));
#142141=CARTESIAN_POINT('Ctrl Pts',(0.447531151415979,-6.99910181078574,
77.2939624170948));
#142142=CARTESIAN_POINT('Ctrl Pts',(0.620664513729673,-6.98587975522444,
77.3018120373884));
#142143=CARTESIAN_POINT('Ctrl Pts',(0.793084111274112,-6.9662503655083,
77.309661657682));
#142144=CARTESIAN_POINT('Ctrl Pts',(0.965489943318995,-6.94662254294786,
77.3175106512839));
#142145=CARTESIAN_POINT('Ctrl Pts',(1.13718174510511,-6.92058844846989,
77.3253596448858));
#142146=CARTESIAN_POINT('Ctrl Pts',(1.3076318089385,-6.88823094958003,77.3332086384876));
#142147=CARTESIAN_POINT('Ctrl Pts',(1.47816816664811,-6.85585706903597,
77.3410616058051));
#142148=CARTESIAN_POINT('Ctrl Pts',(1.64746115506012,-6.81715345885096,
77.3489145731226));
#142149=CARTESIAN_POINT('Ctrl Pts',(1.81499331769497,-6.77225411655695,
77.35676754044));
#142150=CARTESIAN_POINT('Ctrl Pts',(1.98256802787003,-6.72734337133864,
77.3646225021474));
#142151=CARTESIAN_POINT('Ctrl Pts',(2.14838065677686,-6.6762338715936,77.3724774638547));
#142152=CARTESIAN_POINT('Ctrl Pts',(2.31192992701016,-6.61910919800352,
77.380332425562));
#142153=CARTESIAN_POINT('Ctrl Pts',(2.47564153356501,-6.56192782339994,
77.3881951839754));
#142154=CARTESIAN_POINT('Ctrl Pts',(2.6370849394132,-6.49871948922789,77.3960579423888));
#142155=CARTESIAN_POINT('Ctrl Pts',(2.79577929786902,-6.42971575422328,
77.4039207008022));
#142156=CARTESIAN_POINT('Ctrl Pts',(2.91219520209637,-6.37909560437175,
77.40968870755));
#142157=CARTESIAN_POINT('Ctrl Pts',(3.02713214894396,-6.32535767299892,
77.4154567142979));
#142158=CARTESIAN_POINT('Ctrl Pts',(3.1404093910841,-6.26860873072254,77.4212247210457));
#142159=CARTESIAN_POINT('Ctrl Pts',(3.30494530485699,-6.18618053158314,
77.4296027874867));
#142160=CARTESIAN_POINT('Ctrl Pts',(3.46634321095442,-6.09721571817509,
77.4379808539277));
#142161=CARTESIAN_POINT('Ctrl Pts',(3.62407068942216,-6.00197785738761,
77.4463589203687));
#142162=CARTESIAN_POINT('Ctrl Pts',(3.78169031571435,-5.90680511911766,
77.4547312579875));
#142163=CARTESIAN_POINT('Ctrl Pts',(3.93564423765779,-5.80536805470691,
77.4631035956062));
#142164=CARTESIAN_POINT('Ctrl Pts',(4.08542477426931,-5.69797604209482,
77.4714759332249));
#142165=CARTESIAN_POINT('Ctrl Pts',(4.23512485814405,-5.59064171375545,
77.4798437737475));
#142166=CARTESIAN_POINT('Ctrl Pts',(4.3806557598339,-5.47735900608948,77.4882116142701));
#142167=CARTESIAN_POINT('Ctrl Pts',(4.52153854894201,-5.3584807280545,77.4965794547927));
#142168=CARTESIAN_POINT('Ctrl Pts',(4.66236630293313,-5.23964888919054,
77.5049440264626));
#142169=CARTESIAN_POINT('Ctrl Pts',(4.79854931437359,-5.11522605058764,
77.5133085981325));
#142170=CARTESIAN_POINT('Ctrl Pts',(4.92964118259504,-4.9856057178003,77.5216731698024));
#142171=CARTESIAN_POINT('Ctrl Pts',(5.06070102915595,-4.85601704722321,
77.5300356982679));
#142172=CARTESIAN_POINT('Ctrl Pts',(5.18667197933735,-4.72123364552564,
77.5383982267335));
#142173=CARTESIAN_POINT('Ctrl Pts',(5.30714367761709,-4.58168664878219,
77.5467607551991));
#142174=CARTESIAN_POINT('Ctrl Pts',(5.42762498991515,-4.44212851575194,
77.5551239510205));
#142175=CARTESIAN_POINT('Ctrl Pts',(5.54260595418539,-4.2978062730279,77.563487146842));
#142176=CARTESIAN_POINT('Ctrl Pts',(5.65171528838159,-4.14918556605677,
77.5718503426635));
#142177=CARTESIAN_POINT('Ctrl Pts',(5.76083206361579,-4.00055472345117,
77.5802141088382));
#142178=CARTESIAN_POINT('Ctrl Pts',(5.86407621553605,-3.84762509699095,
77.5885778750129));
#142179=CARTESIAN_POINT('Ctrl Pts',(5.9611186444202,-3.69089299081481,77.5969416411876));
#142180=CARTESIAN_POINT('Ctrl Pts',(6.05818062944185,-3.53412929974686,
77.6053070928411));
#142181=CARTESIAN_POINT('Ctrl Pts',(6.14903822626462,-3.37356188052684,
77.6136725444947));
#142182=CARTESIAN_POINT('Ctrl Pts',(6.23340709661391,-3.20971377701867,
77.6220379961482));
#142183=CARTESIAN_POINT('Ctrl Pts',(6.31780422193185,-3.04581080110305,
77.6304062493751));
#142184=CARTESIAN_POINT('Ctrl Pts',(6.39570813717459,-2.87862524226243,
77.6387745026019));
#142185=CARTESIAN_POINT('Ctrl Pts',(6.46688147404923,-2.70870274542978,
77.6471427558287));
#142186=CARTESIAN_POINT('Ctrl Pts',(6.53812079876125,-2.53862270620021,
77.6555187676202));
#142187=CARTESIAN_POINT('Ctrl Pts',(6.60261694815901,-2.36580096180234,
77.6638947794116));
#142188=CARTESIAN_POINT('Ctrl Pts',(6.66018109501871,-2.19080221472762,
77.6722707912031));
#142189=CARTESIAN_POINT('Ctrl Pts',(6.7177734720473,-2.01571764610502,77.6806509106942));
#142190=CARTESIAN_POINT('Ctrl Pts',(6.76842697074315,-1.8384542599116,77.6890310301853));
#142191=CARTESIAN_POINT('Ctrl Pts',(6.81200310361949,-1.65959039488016,
77.6974111496765));
#142192=CARTESIAN_POINT('Ctrl Pts',(6.85562902774758,-1.48052215522559,
77.7058008445157));
#142193=CARTESIAN_POINT('Ctrl Pts',(6.89216135548311,-1.29985010354622,
77.7141905393549));
#142194=CARTESIAN_POINT('Ctrl Pts',(6.92151277629054,-1.11816253297399,
77.7225802341941));
#142195=CARTESIAN_POINT('Ctrl Pts',(6.94014748685212,-1.00281222974806,
77.7279067066689));
#142196=CARTESIAN_POINT('Ctrl Pts',(6.95588878622549,-0.88705273944197,
77.7332331791438));
#142197=CARTESIAN_POINT('Ctrl Pts',(6.96872520897279,-0.771035358675027,
77.7385596516186));
#142198=CARTESIAN_POINT('Ctrl Pts',(6.99682073277446,-0.51710409239379,
77.7502178867158));
#142199=CARTESIAN_POINT('Ctrl Pts',(7.01104969501972,-0.261475717699596,
77.7618761218131));
#142200=CARTESIAN_POINT('Ctrl Pts',(7.01124789937955,-0.00542733321403496,
77.7735343569104));
#142201=CARTESIAN_POINT('Ctrl Pts',(7.01124789938016,-0.00542733243554912,
77.7735343569458));
#142202=CARTESIAN_POINT('Ctrl Pts',(7.01138511916316,0.171838741963074,
77.781605525113));
#142203=CARTESIAN_POINT('Ctrl Pts',(7.00479546290913,0.349352178619966,
77.7896766932801));
#142204=CARTESIAN_POINT('Ctrl Pts',(6.99144932896976,0.526557540016621,
77.7977478614472));
#142205=CARTESIAN_POINT('Ctrl Pts',(6.9781197110538,0.703543607353173,77.8058090414333));
#142206=CARTESIAN_POINT('Ctrl Pts',(6.9580503022769,0.880222000904489,77.8138702214194));
#142207=CARTESIAN_POINT('Ctrl Pts',(6.93126350620007,1.05603634886262,77.8219314014055));
#142208=CARTESIAN_POINT('Ctrl Pts',(6.90449585387803,1.23172504734945,77.8299868202974));
#142209=CARTESIAN_POINT('Ctrl Pts',(6.87102042328743,1.40655057346108,77.8380422391893));
#142210=CARTESIAN_POINT('Ctrl Pts',(6.83091153713191,1.57996016860493,77.8460976580813));
#142211=CARTESIAN_POINT('Ctrl Pts',(6.79082655032157,1.75326643562958,77.8541482770585));
#142212=CARTESIAN_POINT('Ctrl Pts',(6.74411606152931,1.92515810053984,77.8621988960356));
#142213=CARTESIAN_POINT('Ctrl Pts',(6.69090572305961,2.0950912074724,77.8702495150127));
#142214=CARTESIAN_POINT('Ctrl Pts',(6.65406888747181,2.21273372020634,77.8758228553855));
#142215=CARTESIAN_POINT('Ctrl Pts',(6.61411799969896,2.32943773228563,77.8813961957583));
#142216=CARTESIAN_POINT('Ctrl Pts',(6.57110895151815,2.44502632087633,77.886969536131));
#142217=CARTESIAN_POINT('',(7.01124999865213,-0.000137478976900538,77.2264656430895));
#142218=CARTESIAN_POINT('Ctrl Pts',(6.57110895151816,2.4450263208763,77.3398522865014));
#142219=CARTESIAN_POINT('Ctrl Pts',(6.637719246809,2.26600840850797,77.3311805125692));
#142220=CARTESIAN_POINT('Ctrl Pts',(6.69700989700475,2.08426710051949,77.3225087386371));
#142221=CARTESIAN_POINT('Ctrl Pts',(6.74878307789424,1.90040877971777,77.313836964705));
#142222=CARTESIAN_POINT('Ctrl Pts',(6.8005597878953,1.71653792623955,77.3051645996627));
#142223=CARTESIAN_POINT('Ctrl Pts',(6.84481792613571,1.53055004459464,77.2964922346203));
#142224=CARTESIAN_POINT('Ctrl Pts',(6.88140980451094,1.34306577086931,77.287819869578));
#142225=CARTESIAN_POINT('Ctrl Pts',(6.91799949925379,1.15559268532967,77.2791480220618));
#142226=CARTESIAN_POINT('Ctrl Pts',(6.94692379517685,0.966623665171066,
77.2704761745457));
#142227=CARTESIAN_POINT('Ctrl Pts',(6.96808618426385,0.776789219268177,
77.2618043270296));
#142228=CARTESIAN_POINT('Ctrl Pts',(6.98924897510674,0.586951169466541,
77.2531323148834));
#142229=CARTESIAN_POINT('Ctrl Pts',(7.00264953276855,0.396247943319841,
77.2444603027372));
#142230=CARTESIAN_POINT('Ctrl Pts',(7.00824314361837,0.205315860142578,
77.235788290591));
#142231=CARTESIAN_POINT('Ctrl Pts',(7.01024757124656,0.136896809746853,
77.2326807414238));
#142232=CARTESIAN_POINT('Ctrl Pts',(7.01125,0.0684484052931081,77.2295731922567));
#142233=CARTESIAN_POINT('Ctrl Pts',(7.01125,8.58630487052188E-16,77.2264656430895));
#142234=CARTESIAN_POINT('Ctrl Pts',(7.01124999865213,-0.000137478976900539,
77.2264656430895));
#142235=CARTESIAN_POINT('Ctrl Pts',(7.01124653751549,-0.176650970735805,
77.2184682469791));
#142236=CARTESIAN_POINT('Ctrl Pts',(7.00457294202628,-0.353199053916174,
77.2104708508687));
#142237=CARTESIAN_POINT('Ctrl Pts',(6.99124740153013,-0.529231833035602,
77.2024734547584));
#142238=CARTESIAN_POINT('Ctrl Pts',(6.97791746639215,-0.705322666161424,
77.1944734211796));
#142239=CARTESIAN_POINT('Ctrl Pts',(6.95793122676564,-0.880897487063261,
77.1864733876009));
#142240=CARTESIAN_POINT('Ctrl Pts',(6.93135887638516,-1.05541019952274,
77.1784733540221));
#142241=CARTESIAN_POINT('Ctrl Pts',(6.9047823209948,-1.22995052819495,77.1704720544575));
#142242=CARTESIAN_POINT('Ctrl Pts',(6.87161764258769,-1.40342804999125,
77.1624707548929));
#142243=CARTESIAN_POINT('Ctrl Pts',(6.8319863010249,-1.57530623851623,77.1544694553283));
#142244=CARTESIAN_POINT('Ctrl Pts',(6.79232266651492,-1.74732447915767,
77.1464616360363));
#142245=CARTESIAN_POINT('Ctrl Pts',(6.74618193427857,-1.91774042548032,
77.1384538167442));
#142246=CARTESIAN_POINT('Ctrl Pts',(6.69373582543948,-2.08603146230541,
77.1304459974522));
#142247=CARTESIAN_POINT('Ctrl Pts',(6.65431331897053,-2.21253187644019,
77.1244267080362));
#142248=CARTESIAN_POINT('Ctrl Pts',(6.6113292075835,-2.33783196150945,77.1184074186203));
#142249=CARTESIAN_POINT('Ctrl Pts',(6.56487433029689,-2.46171720347991,
77.1123881292043));
#142250=CARTESIAN_POINT('Ctrl Pts',(6.48961971012751,-2.6624052124388,77.1026371759106));
#142251=CARTESIAN_POINT('Ctrl Pts',(6.40520950385572,-2.85950492702172,
77.0928862226169));
#142252=CARTESIAN_POINT('Ctrl Pts',(6.31199119298207,-3.05227681284264,
77.0831352693232));
#142253=CARTESIAN_POINT('Ctrl Pts',(6.21863858364407,-3.24532642272864,
77.073370267952));
#142254=CARTESIAN_POINT('Ctrl Pts',(6.11645250333443,-3.43403569713888,
77.0636052665808));
#142255=CARTESIAN_POINT('Ctrl Pts',(6.0058275377292,-3.61768740351534,77.0538402652096));
#142256=CARTESIAN_POINT('Ctrl Pts',(5.895386961021,-3.80103300054849,77.0440915400724));
#142257=CARTESIAN_POINT('Ctrl Pts',(5.77653563054599,-3.97933784505743,
77.0343428149353));
#142258=CARTESIAN_POINT('Ctrl Pts',(5.64971113665204,-4.15191409290822,
77.0245940897981));
#142259=CARTESIAN_POINT('Ctrl Pts',(5.52323472681706,-4.32401668587588,
77.0148721211314));
#142260=CARTESIAN_POINT('Ctrl Pts',(5.38882886352657,-4.49042203795991,
77.0051501524646));
#142261=CARTESIAN_POINT('Ctrl Pts',(5.24697210171365,-4.65047420445901,
76.9954281837979));
#142262=CARTESIAN_POINT('Ctrl Pts',(5.10605396904297,-4.80946734757541,
76.9857705428585));
#142263=CARTESIAN_POINT('Ctrl Pts',(4.95778322259031,-4.96219104787508,
76.9761129019192));
#142264=CARTESIAN_POINT('Ctrl Pts',(4.80267287525534,-5.10802895604426,
76.9664552609799));
#142265=CARTESIAN_POINT('Ctrl Pts',(4.73449653744279,-5.17212973761073,
76.9622103952926));
#142266=CARTESIAN_POINT('Ctrl Pts',(4.6649994254643,-5.23490060213245,76.9579655296053));
#142267=CARTESIAN_POINT('Ctrl Pts',(4.59422781015657,-5.29629090882327,
76.953720663918));
#142268=CARTESIAN_POINT('Ctrl Pts',(4.46331957011717,-5.40984627942531,
76.945868816904));
#142269=CARTESIAN_POINT('Ctrl Pts',(4.32810190270061,-5.51862856870583,
76.93801696989));
#142270=CARTESIAN_POINT('Ctrl Pts',(4.1889764798803,-5.62228624435911,76.9301651228759));
#142271=CARTESIAN_POINT('Ctrl Pts',(4.04989051190508,-5.72591452353364,
76.9223155025823));
#142272=CARTESIAN_POINT('Ctrl Pts',(3.90689929853329,-5.82442085225462,
76.9144658822886));
#142273=CARTESIAN_POINT('Ctrl Pts',(3.76043715101642,-5.91749431734037,
76.9066162619949));
#142274=CARTESIAN_POINT('Ctrl Pts',(3.613986696629,-6.01056035170019,76.8987672683931));
#142275=CARTESIAN_POINT('Ctrl Pts',(3.46406618210344,-6.09819418192818,
76.8909182747912));
#142276=CARTESIAN_POINT('Ctrl Pts',(3.31113819014348,-6.18012867570518,
76.8830692811893));
#142277=CARTESIAN_POINT('Ctrl Pts',(3.15813277521908,-6.26210465051724,
76.8752163138718));
#142278=CARTESIAN_POINT('Ctrl Pts',(3.00211717731695,-6.3383753433048,76.8673633465543));
#142279=CARTESIAN_POINT('Ctrl Pts',(2.84357813319388,-6.40871983807388,
76.8595103792368));
#142280=CARTESIAN_POINT('Ctrl Pts',(2.68499882548059,-6.47908219798101,
76.8516554175295));
#142281=CARTESIAN_POINT('Ctrl Pts',(2.52389514901132,-6.54351521977476,
76.8438004558221));
#142282=CARTESIAN_POINT('Ctrl Pts',(2.36077241121885,-6.60184672534344,
76.8359454941148));
#142283=CARTESIAN_POINT('Ctrl Pts',(2.19748776047387,-6.66023612980727,
76.8280827357014));
#142284=CARTESIAN_POINT('Ctrl Pts',(2.03218040928632,-6.71251180717497,
76.8202199772879));
#142285=CARTESIAN_POINT('Ctrl Pts',(1.86536991975555,-6.75855174020079,
76.8123572188745));
#142286=CARTESIAN_POINT('Ctrl Pts',(1.74300013823561,-6.79232597443157,
76.8065892121269));
#142287=CARTESIAN_POINT('Ctrl Pts',(1.61982173542334,-6.8227455092496,76.8008212053792));
#142288=CARTESIAN_POINT('Ctrl Pts',(1.49604240872743,-6.84977982666516,
76.7950531986315));
#142289=CARTESIAN_POINT('Ctrl Pts',(1.31625215042021,-6.88904734444093,
76.7866751321905));
#142290=CARTESIAN_POINT('Ctrl Pts',(1.13479557452042,-6.92125810630842,
76.7782970657495));
#142291=CARTESIAN_POINT('Ctrl Pts',(0.952252475682059,-6.94628258747493,
76.7699189993085));
#142292=CARTESIAN_POINT('Ctrl Pts',(0.769834197645653,-6.97128995719856,
76.7615466616898));
#142293=CARTESIAN_POINT('Ctrl Pts',(0.586331202536263,-6.98912079856636,
76.7531743240711));
#142294=CARTESIAN_POINT('Ctrl Pts',(0.402332826543463,-6.99969676908833,
76.7448019864524));
#142295=CARTESIAN_POINT('Ctrl Pts',(0.21843328297071,-7.01026705886037,
76.7364341459298));
#142296=CARTESIAN_POINT('Ctrl Pts',(0.0340392165169123,-7.01359022894083,
76.7280663054072));
#142297=CARTESIAN_POINT('Ctrl Pts',(-0.150255111326989,-7.00963978846418,
76.7196984648847));
#142298=CARTESIAN_POINT('Ctrl Pts',(-0.334477445565594,-7.00569089120622,
76.7113338932148));
#142299=CARTESIAN_POINT('Ctrl Pts',(-0.518599790738046,-6.99447405657724,
76.7029693215449));
#142300=CARTESIAN_POINT('Ctrl Pts',(-0.702027618129939,-6.97601489289428,
76.694604749875));
#142301=CARTESIAN_POINT('Ctrl Pts',(-0.885410639816613,-6.95756023821009,
76.6862422214094));
#142302=CARTESIAN_POINT('Ctrl Pts',(-1.06809915534184,-6.93186681574628,
76.6778796929438));
#142303=CARTESIAN_POINT('Ctrl Pts',(-1.24950303009345,-6.89901215684444,
76.6695171644783));
#142304=CARTESIAN_POINT('Ctrl Pts',(-1.43092138144191,-6.866154876038,76.6611539686568));
#142305=CARTESIAN_POINT('Ctrl Pts',(-1.61105456271462,-6.82613526966803,
76.6527907728353));
#142306=CARTESIAN_POINT('Ctrl Pts',(-1.78932115041994,-6.77908226702995,
76.6444275770138));
#142307=CARTESIAN_POINT('Ctrl Pts',(-1.96759989554915,-6.73202605547142,
76.6360638108391));
#142308=CARTESIAN_POINT('Ctrl Pts',(-2.14401147528783,-6.6779355748947,
76.6277000446644));
#142309=CARTESIAN_POINT('Ctrl Pts',(-2.31798801533611,-6.6169901105607,
76.6193362784898));
#142310=CARTESIAN_POINT('Ctrl Pts',(-2.49199961540088,-6.55603236440421,
76.6109708268362));
#142311=CARTESIAN_POINT('Ctrl Pts',(-2.66357488698875,-6.48821698860404,
76.6026053751826));
#142312=CARTESIAN_POINT('Ctrl Pts',(-2.83216397389218,-6.41377219641353,
76.5942399235291));
#142313=CARTESIAN_POINT('Ctrl Pts',(-3.00080952094936,-6.33930247280848,
76.5858716703022));
#142314=CARTESIAN_POINT('Ctrl Pts',(-3.16646658851368,-6.25819903847252,
76.5775034170754));
#142315=CARTESIAN_POINT('Ctrl Pts',(-3.32860765713012,-6.17073720291139,
76.5691351638485));
#142316=CARTESIAN_POINT('Ctrl Pts',(-3.49089905364909,-6.08319427775093,
76.5607591520571));
#142317=CARTESIAN_POINT('Ctrl Pts',(-3.6496676474343,-5.98928132735913,
76.5523831402656));
#142318=CARTESIAN_POINT('Ctrl Pts',(-3.80441170459272,-5.88931898817324,
76.5440071284742));
#142319=CARTESIAN_POINT('Ctrl Pts',(-3.95923165014872,-5.78930762622113,
76.535627008983));
#142320=CARTESIAN_POINT('Ctrl Pts',(-4.11002285072763,-5.68324114309494,
76.5272468894919));
#142321=CARTESIAN_POINT('Ctrl Pts',(-4.25631416380471,-5.57148241507549,
76.5188667700008));
#142322=CARTESIAN_POINT('Ctrl Pts',(-4.40277263323834,-5.45959598855232,
76.5104770751616));
#142323=CARTESIAN_POINT('Ctrl Pts',(-4.54472068365802,-5.3420045253851,
76.5020873803224));
#142324=CARTESIAN_POINT('Ctrl Pts',(-4.68172072875001,-5.21911080362282,
76.4936976854832));
#142325=CARTESIAN_POINT('Ctrl Pts',(-4.76869969320849,-5.14108770041762,
76.4883712130083));
#142326=CARTESIAN_POINT('Ctrl Pts',(-4.85368495392375,-5.06092814975111,
76.4830447405335));
#142327=CARTESIAN_POINT('Ctrl Pts',(-4.93657252139308,-4.97874264282929,
76.4777182680587));
#142328=CARTESIAN_POINT('Ctrl Pts',(-5.06699760217106,-4.84942226697167,
76.4693369676537));
#142329=CARTESIAN_POINT('Ctrl Pts',(-5.19249008304766,-4.71482309815668,
76.4609556672488));
#142330=CARTESIAN_POINT('Ctrl Pts',(-5.31261214948045,-4.57534465496237,
76.4525743668439));
#142331=CARTESIAN_POINT('Ctrl Pts',(-5.43258197877855,-4.43604298027674,
76.4442036885103));
#142332=CARTESIAN_POINT('Ctrl Pts',(-5.54719474562804,-4.29187460107287,
76.4358330101767));
#142333=CARTESIAN_POINT('Ctrl Pts',(-5.65604866498148,-4.14327648870568,
76.4274623318431));
#142334=CARTESIAN_POINT('Ctrl Pts',(-5.76477905382583,-3.99484700968288,
76.4191011527923));
#142335=CARTESIAN_POINT('Ctrl Pts',(-5.86776342830509,-3.84199807954641,
76.4107399737414));
#142336=CARTESIAN_POINT('Ctrl Pts',(-5.96463929270948,-3.68520076391587,
76.4023787946905));
#142337=CARTESIAN_POINT('Ctrl Pts',(-6.06138944925228,-3.52860691129825,
76.3940284652558));
#142338=CARTESIAN_POINT('Ctrl Pts',(-6.15204673458512,-3.36807516996693,
76.385678135821));
#142339=CARTESIAN_POINT('Ctrl Pts',(-6.23629115844991,-3.2041066070809,
76.3773278063863));
#142340=CARTESIAN_POINT('Ctrl Pts',(-6.32047076126999,-3.04026420819551,
76.3689839020305));
#142341=CARTESIAN_POINT('Ctrl Pts',(-6.39824718671091,-2.87299054781785,
76.3606399976748));
#142342=CARTESIAN_POINT('Ctrl Pts',(-6.46934513066078,-2.70281337552108,
76.352296093319));
#142343=CARTESIAN_POINT('Ctrl Pts',(-6.54038596829858,-2.53277289059061,
76.3439588908393));
#142344=CARTESIAN_POINT('Ctrl Pts',(-6.60475889663115,-2.35983384627065,
76.3356216883595));
#142345=CARTESIAN_POINT('Ctrl Pts',(-6.66223566239757,-2.18454630099204,
76.3272844858798));
#142346=CARTESIAN_POINT('Ctrl Pts',(-6.68115669642255,-2.12684260865401,
76.3245399248439));
#142347=CARTESIAN_POINT('Ctrl Pts',(-6.69933078348043,-2.0688845826821,
76.321795363808));
#142348=CARTESIAN_POINT('Ctrl Pts',(-6.7167509220829,-2.01069232186293,
76.3190508027721));
#142349=CARTESIAN_POINT('Ctrl Pts',(-6.76967542231036,-1.83389715442817,
76.3107124924702));
#142350=CARTESIAN_POINT('Ctrl Pts',(-6.81559374010485,-1.65508383051262,
76.3023741821684));
#142351=CARTESIAN_POINT('Ctrl Pts',(-6.85437739255984,-1.47483460864757,
76.2940358718665));
#142352=CARTESIAN_POINT('Ctrl Pts',(-6.89318544637291,-1.29447198008848,
76.2856923153827));
#142353=CARTESIAN_POINT('Ctrl Pts',(-6.92484981227638,-1.11267197191921,
76.277348758899));
#142354=CARTESIAN_POINT('Ctrl Pts',(-6.94929344594752,-0.930025356971954,
76.2690052024152));
#142355=CARTESIAN_POINT('Ctrl Pts',(-6.97375567622863,-0.747239785276085,
76.26065529819));
#142356=CARTESIAN_POINT('Ctrl Pts',(-6.99098617312171,-0.563606646431596,
76.2523053939649));
#142357=CARTESIAN_POINT('Ctrl Pts',(-7.0009598519598,-0.379720573247087,
76.2439554897397));
#142358=CARTESIAN_POINT('Ctrl Pts',(-7.01094849057808,-0.195558684560555,
76.2355930612761));
#142359=CARTESIAN_POINT('Ctrl Pts',(-7.01365854234673,-0.0111434308617165,
76.2272306328125));
#142360=CARTESIAN_POINT('Ctrl Pts',(-7.00911703962843,0.172930296045726,
76.2188682043489));
#142361=CARTESIAN_POINT('Ctrl Pts',(-7.0045716533062,0.357161431082704,
76.2104986248689));
#142362=CARTESIAN_POINT('Ctrl Pts',(-6.99276236071144,0.541050130409365,
76.202129045389));
#142363=CARTESIAN_POINT('Ctrl Pts',(-6.97376799027683,0.724007306793444,
76.1937594659091));
#142364=CARTESIAN_POINT('Ctrl Pts',(-6.95474432334008,0.907246672330727,
76.1853769773726));
#142365=CARTESIAN_POINT('Ctrl Pts',(-6.92851347978127,1.08955132016771,
76.1769944888361));
#142366=CARTESIAN_POINT('Ctrl Pts',(-6.89520548792931,1.27034162402465,
76.1686120002996));
#142367=CARTESIAN_POINT('Ctrl Pts',(-6.88430656721078,1.32949917387554,
76.165869112695));
#142368=CARTESIAN_POINT('Ctrl Pts',(-6.87265029112176,1.38849469943314,
76.1631262250904));
#142369=CARTESIAN_POINT('Ctrl Pts',(-6.86024236830199,1.44730826386583,
76.1603833374859));
#142370=CARTESIAN_POINT('Ctrl Pts',(-6.82228941872304,1.62720527627431,
76.1519934823531));
#142371=CARTESIAN_POINT('Ctrl Pts',(-6.77722367749001,1.80576193640422,
76.1436036272203));
#142372=CARTESIAN_POINT('Ctrl Pts',(-6.72515683921795,1.98239553329299,
76.1352137720875));
#142373=CARTESIAN_POINT('Ctrl Pts',(-6.67313804749433,2.15886613517478,
76.1268316589955));
#142374=CARTESIAN_POINT('Ctrl Pts',(-6.61413113025583,2.3334168976397,76.1184495459034));
#142375=CARTESIAN_POINT('Ctrl Pts',(-6.54829853369401,2.50547657664582,
76.1100674328113));
#142376=CARTESIAN_POINT('Ctrl Pts',(-6.48251700927431,2.67740277380803,
76.1016918224624));
#142377=CARTESIAN_POINT('Ctrl Pts',(-6.40992047975667,2.8468414345137,76.0933162121136));
#142378=CARTESIAN_POINT('Ctrl Pts',(-6.33072093878141,3.01323728866059,
76.0849406017647));
#142379=CARTESIAN_POINT('Ctrl Pts',(-6.25157121549357,3.17952847734418,
76.0765702597991));
#142380=CARTESIAN_POINT('Ctrl Pts',(-6.16582690315319,3.34278037969969,
76.0681999178336));
#142381=CARTESIAN_POINT('Ctrl Pts',(-6.07374793431603,3.50245807867729,
76.059829575868));
#142382=CARTESIAN_POINT('Ctrl Pts',(-5.98171338677479,3.6620587449686,76.0514632719737));
#142383=CARTESIAN_POINT('Ctrl Pts',(-5.88335044082332,3.8180883621323,76.0430969680794));
#142384=CARTESIAN_POINT('Ctrl Pts',(-5.77896496849459,3.97003658111765,
76.0347306641851));
#142385=CARTESIAN_POINT('Ctrl Pts',(-5.67460868985666,4.12194230444509,
76.0263667001115));
#142386=CARTESIAN_POINT('Ctrl Pts',(-5.56423342811717,4.26976863416483,
76.0180027360379));
#142387=CARTESIAN_POINT('Ctrl Pts',(-5.44818868140137,4.41303372458788,
76.0096387719642));
#142388=CARTESIAN_POINT('Ctrl Pts',(-5.33216179204368,4.55627676889428,
76.0012760949657));
#142389=CARTESIAN_POINT('Ctrl Pts',(-5.21046736398403,4.69495971803615,
75.9929134179672));
#142390=CARTESIAN_POINT('Ctrl Pts',(-5.08349578478998,4.82863305382823,
75.9845507409687));
#142391=CARTESIAN_POINT('Ctrl Pts',(-4.95652681970868,4.96230363753063,
75.9761882361424));
#142392=CARTESIAN_POINT('Ctrl Pts',(-4.82428114676611,5.09096457553284,
75.9678257313161));
#142393=CARTESIAN_POINT('Ctrl Pts',(-4.68718697469538,5.21420222342268,
75.9594632264898));
#142394=CARTESIAN_POINT('Ctrl Pts',(-4.55007735146583,5.3374537607758,75.9510997791698));
#142395=CARTESIAN_POINT('Ctrl Pts',(-4.40811838440878,5.45528057009708,
75.9427363318498));
#142396=CARTESIAN_POINT('Ctrl Pts',(-4.26177272292003,5.56730813056676,
75.9343728845299));
#142397=CARTESIAN_POINT('Ctrl Pts',(-4.11534088899297,5.67940165601243,
75.9260045125771));
#142398=CARTESIAN_POINT('Ctrl Pts',(-3.96451745982751,5.78568890835623,
75.9176361406243));
#142399=CARTESIAN_POINT('Ctrl Pts',(-3.80979637388745,5.88583708167446,
75.9092677686715));
#142400=CARTESIAN_POINT('Ctrl Pts',(-3.65502892946641,5.98601526200278,
75.9008968893357));
#142401=CARTESIAN_POINT('Ctrl Pts',(-3.49636177845906,6.08005052134992,
75.89252601));
#142402=CARTESIAN_POINT('Ctrl Pts',(-3.33431562974891,6.16765480905929,
75.8841551306643));
#142403=CARTESIAN_POINT('Ctrl Pts',(-3.17213218108927,6.25533332293431,
75.875777158773));
#142404=CARTESIAN_POINT('Ctrl Pts',(-3.00656430586399,6.33656982562424,
75.8673991868817));
#142405=CARTESIAN_POINT('Ctrl Pts',(-2.8381560084519,6.41112291523009,75.8590212149904));
#142406=CARTESIAN_POINT('Ctrl Pts',(-2.7311311640895,6.45850201076407,75.8536969456313));
#142407=CARTESIAN_POINT('Ctrl Pts',(-2.62295958428094,6.50318283201099,
75.8483726762721));
#142408=CARTESIAN_POINT('Ctrl Pts',(-2.51378464525668,6.54511369800187,
75.843048406913));
#142409=CARTESIAN_POINT('Ctrl Pts',(-2.35255611646706,6.60703680869931,
75.8351855757237));
#142410=CARTESIAN_POINT('Ctrl Pts',(-2.18880317525655,6.66308866001884,
75.8273227445343));
#142411=CARTESIAN_POINT('Ctrl Pts',(-2.0230110193665,6.71305094409552,75.819459913345));
#142412=CARTESIAN_POINT('Ctrl Pts',(-1.85734625286391,6.76297483875184,
75.8116031237035));
#142413=CARTESIAN_POINT('Ctrl Pts',(-1.68964575031866,6.80681836178648,
75.8037463340621));
#142414=CARTESIAN_POINT('Ctrl Pts',(-1.52041460454805,6.84441129628962,
75.7958895444206));
#142415=CARTESIAN_POINT('Ctrl Pts',(-1.35127889713284,6.88198303015723,
75.7880371856366));
#142416=CARTESIAN_POINT('Ctrl Pts',(-1.1806146346543,6.91331110517551,75.7801848268526));
#142417=CARTESIAN_POINT('Ctrl Pts',(-1.00894174040602,6.93827522709834,
75.7723324680686));
#142418=CARTESIAN_POINT('Ctrl Pts',(-0.837309380130855,6.96323345470074,
75.7644819633181));
#142419=CARTESIAN_POINT('Ctrl Pts',(-0.664669237816469,6.98183065663988,
75.7566314585676));
#142420=CARTESIAN_POINT('Ctrl Pts',(-0.491551030523516,6.99399772282572,
75.7487809538171));
#142421=CARTESIAN_POINT('Ctrl Pts',(-0.318460672493938,7.00616283171408,
75.7409317119654));
#142422=CARTESIAN_POINT('Ctrl Pts',(-0.144892783383574,7.01189984029959,
75.7330824701137));
#142423=CARTESIAN_POINT('Ctrl Pts',(0.0286186714364771,7.01119159160162,
75.725233228262));
#142424=CARTESIAN_POINT('Ctrl Pts',(0.202188585661757,7.0104831042808,75.7173813418471));
#142425=CARTESIAN_POINT('Ctrl Pts',(0.375701645758201,7.0033250237297,75.7095294554322));
#142426=CARTESIAN_POINT('Ctrl Pts',(0.548624559648844,6.98975233145282,
75.7016775690173));
#142427=CARTESIAN_POINT('Ctrl Pts',(0.675599702981625,6.9797860724505,75.6959120265537));
#142428=CARTESIAN_POINT('Ctrl Pts',(0.802256653232083,6.96636228413978,
75.6901464840901));
#142429=CARTESIAN_POINT('Ctrl Pts',(0.928386492955239,6.94951257874956,
75.6843809416265));
#142430=CARTESIAN_POINT('Ctrl Pts',(1.13961067507704,6.92129510659661,75.6747256372668));
#142431=CARTESIAN_POINT('Ctrl Pts',(1.34924873524208,6.88348348125227,75.6650703329071));
#142432=CARTESIAN_POINT('Ctrl Pts',(1.55652435376117,6.83628981967912,75.6554150285474));
#142433=CARTESIAN_POINT('Ctrl Pts',(1.76494824032233,6.78883471407431,75.6457062356129));
#142434=CARTESIAN_POINT('Ctrl Pts',(1.97098340391546,6.73189339869494,75.6359974426784));
#142435=CARTESIAN_POINT('Ctrl Pts',(2.17386282222187,6.66572929188259,75.6262886497439));
#142436=CARTESIAN_POINT('Ctrl Pts',(2.37771851351549,6.59924679777033,75.6165331372734));
#142437=CARTESIAN_POINT('Ctrl Pts',(2.57838798132566,6.52345257317632,75.6067776248029));
#142438=CARTESIAN_POINT('Ctrl Pts',(2.77511599997138,6.43866117676671,75.5970221123325));
#142439=CARTESIAN_POINT('Ctrl Pts',(2.97203880962188,6.35378582382962,75.5872569404038));
#142440=CARTESIAN_POINT('Ctrl Pts',(3.16501233314907,6.25989550531329,75.5774917684751));
#142441=CARTESIAN_POINT('Ctrl Pts',(3.35330244677766,6.15735245563667,75.5677265965464));
#142442=CARTESIAN_POINT('Ctrl Pts',(3.54133583110839,6.05494922108171,75.557974739208));
#142443=CARTESIAN_POINT('Ctrl Pts',(3.7246985350011,5.94391685311914,75.5482228818697));
#142444=CARTESIAN_POINT('Ctrl Pts',(3.90268314407793,5.82466229402444,75.5384710245314));
#142445=CARTESIAN_POINT('Ctrl Pts',(3.98029732391505,5.77265866941902,75.5342185084676));
#142446=CARTESIAN_POINT('Ctrl Pts',(4.05688911733023,5.71909211162802,75.5299659924039));
#142447=CARTESIAN_POINT('Ctrl Pts',(4.13240130821834,5.66399911637841,75.5257134763401));
#142448=CARTESIAN_POINT('Ctrl Pts',(4.27504459599869,5.55992789445191,75.5176804307412));
#142449=CARTESIAN_POINT('Ctrl Pts',(4.41390286247982,5.45035596546751,75.5096473851423));
#142450=CARTESIAN_POINT('Ctrl Pts',(4.5485213107685,5.33559560386512,75.5016143395435));
#142451=CARTESIAN_POINT('Ctrl Pts',(4.68305322113534,5.22090901464186,75.4935864578956));
#142452=CARTESIAN_POINT('Ctrl Pts',(4.81335046072279,5.10104086866301,75.4855585762478));
#142453=CARTESIAN_POINT('Ctrl Pts',(4.93898910745856,4.97634536169926,75.4775306945999));
#142454=CARTESIAN_POINT('Ctrl Pts',(5.06457102710724,4.85170615598569,75.4695064376198));
#142455=CARTESIAN_POINT('Ctrl Pts',(5.18549828237782,4.72224418681249,75.4614821806396));
#142456=CARTESIAN_POINT('Ctrl Pts',(5.30138185291129,4.58835231996442,75.4534579236594));
#142457=CARTESIAN_POINT('Ctrl Pts',(5.4172514119404,4.45447664200721,75.4454346368937));
#142458=CARTESIAN_POINT('Ctrl Pts',(5.52807825533282,4.31617240520348,75.4374113501279));
#142459=CARTESIAN_POINT('Ctrl Pts',(5.63351179532338,4.17386768051557,75.4293880633622));
#142460=CARTESIAN_POINT('Ctrl Pts',(5.73893669597605,4.03157461643016,75.4213654340332));
#142461=CARTESIAN_POINT('Ctrl Pts',(5.83896895847622,3.88528201440496,75.4133428047042));
#142462=CARTESIAN_POINT('Ctrl Pts',(5.93329988997063,3.73544896607818,75.4053201753752));
#142463=CARTESIAN_POINT('Ctrl Pts',(6.02766628317955,3.58555959119234,75.3972945301088));
#142464=CARTESIAN_POINT('Ctrl Pts',(6.11632687090332,3.43212742321844,75.3892688848423));
#142465=CARTESIAN_POINT('Ctrl Pts',(6.19901750485473,3.27563864566967,75.3812432395759));
#142466=CARTESIAN_POINT('Ctrl Pts',(6.24777694154722,3.18336332647866,75.3765108300685));
#142467=CARTESIAN_POINT('Ctrl Pts',(6.29446148932598,3.09002570380226,75.371778420561));
#142468=CARTESIAN_POINT('Ctrl Pts',(6.33902467059603,2.99572909123554,75.3670460110536));
#142469=CARTESIAN_POINT('Ctrl Pts',(6.42418139636258,2.81553569955649,75.3580027496178));
#142470=CARTESIAN_POINT('Ctrl Pts',(6.50163293414364,2.63174597938776,75.3489594881819));
#142471=CARTESIAN_POINT('Ctrl Pts',(6.57110895151811,2.44502632087644,75.339916226746));
#142472=CARTESIAN_POINT('Origin',(0.,0.,50.));
#142473=CARTESIAN_POINT('',(6.57110895151811,2.44502632087643,73.339830038482));
#142474=CARTESIAN_POINT('',(6.57110895151812,2.44502632087642,73.8869619471141));
#142475=CARTESIAN_POINT('',(6.57110895151814,2.44502632087636,50.));
#142476=CARTESIAN_POINT('',(7.01124707280511,0.0064067606328066,75.7735343568825));
#142477=CARTESIAN_POINT('Ctrl Pts',(6.57110895151812,2.44502632087642,73.8869619471141));
#142478=CARTESIAN_POINT('Ctrl Pts',(6.50275899109119,2.62871965495729,73.8958758490847));
#142479=CARTESIAN_POINT('Ctrl Pts',(6.42672848959599,2.80947512617339,73.9047897510554));
#142480=CARTESIAN_POINT('Ctrl Pts',(6.34329324847321,2.98667998392432,73.913703653026));
#142481=CARTESIAN_POINT('Ctrl Pts',(6.2907616291823,3.09824984335786,73.9193159302655));
#142482=CARTESIAN_POINT('Ctrl Pts',(6.23529565958854,3.20841264439689,73.9249282075049));
#142483=CARTESIAN_POINT('Ctrl Pts',(6.17697358078328,3.31702034133128,73.9305404847443));
#142484=CARTESIAN_POINT('Ctrl Pts',(6.09526402854701,3.46918032032569,73.9384033159336));
#142485=CARTESIAN_POINT('Ctrl Pts',(6.00780935259603,3.61854067465666,73.946266147123));
#142486=CARTESIAN_POINT('Ctrl Pts',(5.91483458550851,3.76461928866285,73.9541289783124));
#142487=CARTESIAN_POINT('Ctrl Pts',(5.82193125725678,3.91058566053664,73.9619857679538));
#142488=CARTESIAN_POINT('Ctrl Pts',(5.72351647602113,4.05327498704915,73.9698425575953));
#142489=CARTESIAN_POINT('Ctrl Pts',(5.61986173966912,4.19222859461447,73.9776993472368));
#142490=CARTESIAN_POINT('Ctrl Pts',(5.51626545968203,4.33110383892233,73.9855517060208));
#142491=CARTESIAN_POINT('Ctrl Pts',(5.40743533018594,4.46624725047326,73.9934040648048));
#142492=CARTESIAN_POINT('Ctrl Pts',(5.2936866735676,4.5972282915462,74.0012564235888));
#142493=CARTESIAN_POINT('Ctrl Pts',(5.17996487433408,4.72817840646733,74.0091069283393));
#142494=CARTESIAN_POINT('Ctrl Pts',(5.06132710273039,4.85496781378237,74.0169574330898));
#142495=CARTESIAN_POINT('Ctrl Pts',(4.93812951377572,4.97719835526747,74.0248079378403));
#142496=CARTESIAN_POINT('Ctrl Pts',(4.81495174343018,5.09940923371089,74.032657179692));
#142497=CARTESIAN_POINT('Ctrl Pts',(4.68721588893935,5.21706243968238,74.0405064215437));
#142498=CARTESIAN_POINT('Ctrl Pts',(4.55531523914614,5.32979639709651,74.0483556633954));
#142499=CARTESIAN_POINT('Ctrl Pts',(4.4233701494424,5.44256833678737,74.0562075498104));
#142500=CARTESIAN_POINT('Ctrl Pts',(4.28725775191128,5.5504174692811,74.0640594362253));
#142501=CARTESIAN_POINT('Ctrl Pts',(4.14740486202403,5.65302215394204,74.0719113226402));
#142502=CARTESIAN_POINT('Ctrl Pts',(4.04471262570295,5.72836349678697,74.0776768651037));
#142503=CARTESIAN_POINT('Ctrl Pts',(3.9400043080111,5.80087797358243,74.0834424075672));
#142504=CARTESIAN_POINT('Ctrl Pts',(3.83345880483194,5.87045314725844,74.0892079500307));
#142505=CARTESIAN_POINT('Ctrl Pts',(3.65503166326317,5.98696767854079,74.0988632543904));
#142506=CARTESIAN_POINT('Ctrl Pts',(3.47154285547476,6.09517901204123,74.1085185587502));
#142507=CARTESIAN_POINT('Ctrl Pts',(3.28371893133776,6.19474103917783,74.1181738631099));
#142508=CARTESIAN_POINT('Ctrl Pts',(3.09485449789795,6.29485462126632,74.1278826560444));
#142509=CARTESIAN_POINT('Ctrl Pts',(2.90160685091477,6.38622282672841,74.1375914489789));
#142510=CARTESIAN_POINT('Ctrl Pts',(2.70472898750889,6.46854447821371,74.1473002419134));
#142511=CARTESIAN_POINT('Ctrl Pts',(2.50690373110709,6.55126226847603,74.1570557543839));
#142512=CARTESIAN_POINT('Ctrl Pts',(2.30541328557382,6.62484623515333,74.1668112668544));
#142513=CARTESIAN_POINT('Ctrl Pts',(2.10103509689751,6.68904164167819,74.1765667793249));
#142514=CARTESIAN_POINT('Ctrl Pts',(1.89645454237132,6.75330061153182,74.1863319512536));
#142515=CARTESIAN_POINT('Ctrl Pts',(1.68898056535691,6.80815242604585,74.1960971231823));
#142516=CARTESIAN_POINT('Ctrl Pts',(1.47940575007312,6.85339223955193,74.205862295111));
#142517=CARTESIAN_POINT('Ctrl Pts',(1.27011668529535,6.89857036959865,74.2156141524493));
#142518=CARTESIAN_POINT('Ctrl Pts',(1.05873254434566,6.93416268434599,74.2253660097876));
#142519=CARTESIAN_POINT('Ctrl Pts',(0.846054864409197,6.96001564142708,
74.2351178671259));
#142520=CARTESIAN_POINT('Ctrl Pts',(0.753311993082726,6.97128940307755,
74.2393703831896));
#142521=CARTESIAN_POINT('Ctrl Pts',(0.660323296795574,6.98071178572122,
74.2436228992534));
#142522=CARTESIAN_POINT('Ctrl Pts',(0.567155942729901,6.98827308418369,
74.2478754153171));
#142523=CARTESIAN_POINT('Ctrl Pts',(0.391161874201906,7.00255645300005,
74.2559084609159));
#142524=CARTESIAN_POINT('Ctrl Pts',(0.214444101747809,7.0102020196953,74.2639415065147));
#142525=CARTESIAN_POINT('Ctrl Pts',(0.037550999544158,7.01114944106409,
74.2719745521135));
#142526=CARTESIAN_POINT('Ctrl Pts',(-0.139228388962058,7.01209625339394,
74.2800024337614));
#142527=CARTESIAN_POINT('Ctrl Pts',(-0.316182517833347,7.00635348929289,
74.2880303154091));
#142528=CARTESIAN_POINT('Ctrl Pts',(-0.492759034395258,6.99391271725076,
74.296058197057));
#142529=CARTESIAN_POINT('Ctrl Pts',(-0.669255824920555,6.98147756233975,
74.3040824540371));
#142530=CARTESIAN_POINT('Ctrl Pts',(-0.845374977708918,6.96235044675942,
74.3121067110173));
#142531=CARTESIAN_POINT('Ctrl Pts',(-1.0205653345377,6.93657501656545,74.3201309679974));
#142532=CARTESIAN_POINT('Ctrl Pts',(-1.19573450906741,6.9108027028836,74.3281542547631));
#142533=CARTESIAN_POINT('Ctrl Pts',(-1.36997474774586,6.87838372141755,
74.3361775415289));
#142534=CARTESIAN_POINT('Ctrl Pts',(-1.54274102340186,6.83941347611131,
74.3442008282946));
#142535=CARTESIAN_POINT('Ctrl Pts',(-1.71549314240272,6.80044642406904,
74.3522234576236));
#142536=CARTESIAN_POINT('Ctrl Pts',(-1.88677118218473,6.7549292620711,74.3602460869525));
#142537=CARTESIAN_POINT('Ctrl Pts',(-2.05604160109687,6.70300824235351,
74.3682687162814));
#142538=CARTESIAN_POINT('Ctrl Pts',(-2.22537565363579,6.65106770402887,
74.3762943615479));
#142539=CARTESIAN_POINT('Ctrl Pts',(-2.39270022781168,6.59271860925155,
74.3843200068143));
#142540=CARTESIAN_POINT('Ctrl Pts',(-2.55749783942897,6.52815681213435,
74.3923456520807));
#142541=CARTESIAN_POINT('Ctrl Pts',(-2.65467255350605,6.4900872423536,74.3970780615883));
#142542=CARTESIAN_POINT('Ctrl Pts',(-2.75096898407742,6.44985844336226,
74.401810471096));
#142543=CARTESIAN_POINT('Ctrl Pts',(-2.84628447904245,6.40751833605352,
74.4065428806036));
#142544=CARTESIAN_POINT('Ctrl Pts',(-3.02211645732264,6.32941199215401,
74.4152729294383));
#142545=CARTESIAN_POINT('Ctrl Pts',(-3.1946970624525,6.24407939971055,74.4240029782731));
#142546=CARTESIAN_POINT('Ctrl Pts',(-3.36345017752929,6.15181513585854,
74.4327330271079));
#142547=CARTESIAN_POINT('Ctrl Pts',(-3.53225208777979,6.05952419367955,
74.4414656002472));
#142548=CARTESIAN_POINT('Ctrl Pts',(-3.69722405853467,5.96029771081409,
74.4501981733864));
#142549=CARTESIAN_POINT('Ctrl Pts',(-3.85781566581852,5.85447562562739,
74.4589307465257));
#142550=CARTESIAN_POINT('Ctrl Pts',(-4.02068873323303,5.74715016879892,
74.4677873798061));
#142551=CARTESIAN_POINT('Ctrl Pts',(-4.17905578647582,5.63304043873274,
74.4766440130864));
#142552=CARTESIAN_POINT('Ctrl Pts',(-4.33237374851898,5.51254607832385,
74.4855006463668));
#142553=CARTESIAN_POINT('Ctrl Pts',(-4.4836403262669,5.3936639245691,74.4942387784736));
#142554=CARTESIAN_POINT('Ctrl Pts',(-4.62999188267125,5.26856712114457,
74.5029769105805));
#142555=CARTESIAN_POINT('Ctrl Pts',(-4.77094005591142,5.13768017157549,
74.5117150426874));
#142556=CARTESIAN_POINT('Ctrl Pts',(-4.9147554078106,5.00413070953874,74.5206309265545));
#142557=CARTESIAN_POINT('Ctrl Pts',(-5.05294497011473,4.86455320967521,
74.5295468104216));
#142558=CARTESIAN_POINT('Ctrl Pts',(-5.18502865945245,4.71943898818034,
74.5384626942887));
#142559=CARTESIAN_POINT('Ctrl Pts',(-5.31711234879022,4.57432476668543,
74.5473785781558));
#142560=CARTESIAN_POINT('Ctrl Pts',(-5.44308996609929,4.42367405129665,
74.5562944620229));
#142561=CARTESIAN_POINT('Ctrl Pts',(-5.56252360649307,4.26801566183951,
74.56521034589));
#142562=CARTESIAN_POINT('Ctrl Pts',(-5.67961034567175,4.1154159990707,74.5739510303861));
#142563=CARTESIAN_POINT('Ctrl Pts',(-5.79042033806903,3.95798743193976,
74.5826917148821));
#142564=CARTESIAN_POINT('Ctrl Pts',(-5.89457869846284,3.79625717386587,
74.5914323993782));
#142565=CARTESIAN_POINT('Ctrl Pts',(-5.99871831903719,3.63455601375231,
74.6001715112799));
#142566=CARTESIAN_POINT('Ctrl Pts',(-6.09620854939378,3.46855493842968,
74.6089106231816));
#142567=CARTESIAN_POINT('Ctrl Pts',(-6.18671818026086,3.29880959143291,
74.6176497350833));
#142568=CARTESIAN_POINT('Ctrl Pts',(-6.27840049366468,3.12686494915442,
74.6265020747577));
#142569=CARTESIAN_POINT('Ctrl Pts',(-6.36291990525096,2.95107857490478,
74.6353544144322));
#142570=CARTESIAN_POINT('Ctrl Pts',(-6.43997990603593,2.77205435955961,
74.6442067541066));
#142571=CARTESIAN_POINT('Ctrl Pts',(-6.51601526206472,2.59541057792342,
74.6529413867562));
#142572=CARTESIAN_POINT('Ctrl Pts',(-6.58478824835034,2.41561478930709,
74.6616760194057));
#142573=CARTESIAN_POINT('Ctrl Pts',(-6.64606178442928,2.23326875231099,
74.6704106520553));
#142574=CARTESIAN_POINT('Ctrl Pts',(-6.70857389445685,2.04723680022803,
74.6793218452422));
#142575=CARTESIAN_POINT('Ctrl Pts',(-6.7632800266812,1.8585506693742,74.688233038429));
#142576=CARTESIAN_POINT('Ctrl Pts',(-6.80998104714929,1.66786831013946,
74.6971442316159));
#142577=CARTESIAN_POINT('Ctrl Pts',(-6.8566820676174,1.47718595090465,74.7060554248027));
#142578=CARTESIAN_POINT('Ctrl Pts',(-6.89537789113214,1.28450765451162,
74.7149666179896));
#142579=CARTESIAN_POINT('Ctrl Pts',(-6.92592396116717,1.09050623410895,
74.7238778111764));
#142580=CARTESIAN_POINT('Ctrl Pts',(-6.95343458915171,0.915783237040895,
74.7319034760289));
#142581=CARTESIAN_POINT('Ctrl Pts',(-6.97434683907087,0.739906637123656,
74.7399291408814));
#142582=CARTESIAN_POINT('Ctrl Pts',(-6.98857508167542,0.563422479393069,
74.7479548057339));
#142583=CARTESIAN_POINT('Ctrl Pts',(-7.00279880858477,0.386994333405122,
74.7559779234372));
#142584=CARTESIAN_POINT('Ctrl Pts',(-7.01034272214564,0.209959378448671,
74.7640010411405));
#142585=CARTESIAN_POINT('Ctrl Pts',(-7.01117295096855,0.0328696532836382,
74.7720241588438));
#142586=CARTESIAN_POINT('Ctrl Pts',(-7.01200307509234,-0.144197739317557,
74.7800462647618));
#142587=CARTESIAN_POINT('Ctrl Pts',(-7.00612119978994,-0.321319521904239,
74.7880683706797));
#142588=CARTESIAN_POINT('Ctrl Pts',(-6.99354556022944,-0.497942827536565,
74.7960904765977));
#142589=CARTESIAN_POINT('Ctrl Pts',(-6.98096524751879,-0.67463176698591,
74.8041155635573));
#142590=CARTESIAN_POINT('Ctrl Pts',(-6.96168622452595,-0.850821493238382,
74.812140650517));
#142591=CARTESIAN_POINT('Ctrl Pts',(-6.93577872499585,-1.02596298198083,
74.8201657374766));
#142592=CARTESIAN_POINT('Ctrl Pts',(-6.90986612311346,-1.20113896396232,
74.8281924049369));
#142593=CARTESIAN_POINT('Ctrl Pts',(-6.87732250638558,-1.37526593583321,
74.8362190723972));
#142594=CARTESIAN_POINT('Ctrl Pts',(-6.83826936652441,-1.5478044557869,
74.8442457398576));
#142595=CARTESIAN_POINT('Ctrl Pts',(-6.79918487494009,-1.72048148905682,
74.8522788510982));
#142596=CARTESIAN_POINT('Ctrl Pts',(-6.75358051291989,-1.8915671681038,
74.8603119623389));
#142597=CARTESIAN_POINT('Ctrl Pts',(-6.70162800407903,-2.06053601216861,
74.8683450735796));
#142598=CARTESIAN_POINT('Ctrl Pts',(-6.6710156985963,-2.16009859320625,
74.8730784745407));
#142599=CARTESIAN_POINT('Ctrl Pts',(-6.63820025694383,-2.25892652539235,
74.8778118755017));
#142600=CARTESIAN_POINT('Ctrl Pts',(-6.60322465143507,-2.35691551931336,
74.8825452764628));
#142601=CARTESIAN_POINT('Ctrl Pts',(-6.53117381556781,-2.55877589642768,
74.8922962297567));
#142602=CARTESIAN_POINT('Ctrl Pts',(-6.44991144028724,-2.75719415863265,
74.9020471830505));
#142603=CARTESIAN_POINT('Ctrl Pts',(-6.35977319227492,-2.95142533453267,
74.9117981363444));
#142604=CARTESIAN_POINT('Ctrl Pts',(-6.269505083206,-3.14593633688021,74.9215631377158));
#142605=CARTESIAN_POINT('Ctrl Pts',(-6.17033553918559,-3.33624815153717,
74.9313281390871));
#142606=CARTESIAN_POINT('Ctrl Pts',(-6.06264768007091,-3.52163735637712,
74.9410931404585));
#142607=CARTESIAN_POINT('Ctrl Pts',(-5.95513931430501,-3.70671755582428,
74.9508418655959));
#142608=CARTESIAN_POINT('Ctrl Pts',(-5.83914102905413,-3.88689151107827,
74.9605905907332));
#142609=CARTESIAN_POINT('Ctrl Pts',(-5.71507941116065,-4.06146450022989,
74.9703393158706));
#142610=CARTESIAN_POINT('Ctrl Pts',(-5.59135829430299,-4.23555835421754,
74.9800612845376));
#142611=CARTESIAN_POINT('Ctrl Pts',(-5.45961804830347,-4.40408189819558,
74.9897832532045));
#142612=CARTESIAN_POINT('Ctrl Pts',(-5.32032672712792,-4.56637165363358,
74.9995052218715));
#142613=CARTESIAN_POINT('Ctrl Pts',(-5.18195706024321,-4.72758758014818,
75.0091628628111));
#142614=CARTESIAN_POINT('Ctrl Pts',(-5.03613592336463,-4.88265188593332,
75.0188205037506));
#142615=CARTESIAN_POINT('Ctrl Pts',(-4.8833664542797,-5.03094013438003,
75.0284781446902));
#142616=CARTESIAN_POINT('Ctrl Pts',(-4.81621901306715,-5.09611792484255,
75.0327230103765));
#142617=CARTESIAN_POINT('Ctrl Pts',(-4.7477297973699,-5.15998698883543,
75.0369678760629));
#142618=CARTESIAN_POINT('Ctrl Pts',(-4.67794426613898,-5.22249595551757,
75.0412127417492));
#142619=CARTESIAN_POINT('Ctrl Pts',(-4.54886001342036,-5.33812054287909,
75.0490645887632));
#142620=CARTESIAN_POINT('Ctrl Pts',(-4.41539090845857,-5.44904124456751,
75.0569164357772));
#142621=CARTESIAN_POINT('Ctrl Pts',(-4.27793297717984,-5.55490017959434,
75.0647682827911));
#142622=CARTESIAN_POINT('Ctrl Pts',(-4.14051402785882,-5.66072909388326,
75.0726179030848));
#142623=CARTESIAN_POINT('Ctrl Pts',(-3.99910880429848,-5.76149886439636,
75.0804675233784));
#142624=CARTESIAN_POINT('Ctrl Pts',(-3.85414661408296,-5.85689170462053,
75.0883171436721));
#142625=CARTESIAN_POINT('Ctrl Pts',(-3.70919599724444,-5.95227692894638,
75.0961661372739));
#142626=CARTESIAN_POINT('Ctrl Pts',(-3.56068929814396,-6.04228586849202,
75.1040151308758));
#142627=CARTESIAN_POINT('Ctrl Pts',(-3.40908478907484,-6.12664406207824,
75.1118641244776));
#142628=CARTESIAN_POINT('Ctrl Pts',(-3.25740352708227,-6.21104496374759,
75.1197170917951));
#142629=CARTESIAN_POINT('Ctrl Pts',(-3.10262165528774,-6.28978921769999,
75.1275700591125));
#142630=CARTESIAN_POINT('Ctrl Pts',(-2.94522233258021,-6.36264818877885,
75.13542302643));
#142631=CARTESIAN_POINT('Ctrl Pts',(-2.78778303573294,-6.43552566358849,
75.1432779881373));
#142632=CARTESIAN_POINT('Ctrl Pts',(-2.62772531557513,-6.50251473051098,
75.1511329498446));
#142633=CARTESIAN_POINT('Ctrl Pts',(-2.46555167505598,-6.56343519051789,
75.158987911552));
#142634=CARTESIAN_POINT('Ctrl Pts',(-2.30321706364293,-6.62441611917355,
75.1668506699654));
#142635=CARTESIAN_POINT('Ctrl Pts',(-2.1387626988558,-6.67931628951148,
75.1747134283787));
#142636=CARTESIAN_POINT('Ctrl Pts',(-1.97270613489017,-6.72800543013059,
75.1825761867921));
#142637=CARTESIAN_POINT('Ctrl Pts',(-1.85088942234223,-6.76372308503902,
75.18834419354));
#142638=CARTESIAN_POINT('Ctrl Pts',(-1.72821079584976,-6.79609933591651,
75.1941122002878));
#142639=CARTESIAN_POINT('Ctrl Pts',(-1.60487744077161,-6.82510036282269,
75.1998802070357));
#142640=CARTESIAN_POINT('Ctrl Pts',(-1.42573495907739,-6.86722453862543,
75.2082582734767));
#142641=CARTESIAN_POINT('Ctrl Pts',(-1.24481405199275,-6.90231937438806,
75.2166363399177));
#142642=CARTESIAN_POINT('Ctrl Pts',(-1.06269237914407,-6.9302461334219,
75.2250144063587));
#142643=CARTESIAN_POINT('Ctrl Pts',(-0.88069523893112,-6.95815379646976,
75.2333867439775));
#142644=CARTESIAN_POINT('Ctrl Pts',(-0.69749929381418,-6.97890310515552,
75.2417590815962));
#142645=CARTESIAN_POINT('Ctrl Pts',(-0.513692558389837,-6.99240634674179,
75.250131419215));
#142646=CARTESIAN_POINT('Ctrl Pts',(-0.329984552447882,-7.00590233523122,
75.2584992597376));
#142647=CARTESIAN_POINT('Ctrl Pts',(-0.145666737463464,-7.0121599931371,
75.2668671002602));
#142648=CARTESIAN_POINT('Ctrl Pts',(0.038667121992827,-7.01114337438458,
75.2752349407828));
#142649=CARTESIAN_POINT('Ctrl Pts',(0.222928972401273,-7.0101271527688,
75.2835995124528));
#142650=CARTESIAN_POINT('Ctrl Pts',(0.40720652655978,-7.00184232297566,
75.2919640841227));
#142651=CARTESIAN_POINT('Ctrl Pts',(0.590904923471322,-6.98630502725993,
75.3003286557926));
#142652=CARTESIAN_POINT('Ctrl Pts',(0.77455844858733,-6.9707715268215,75.3086911842583));
#142653=CARTESIAN_POINT('Ctrl Pts',(0.957632771390947,-6.94798912146856,
75.317053712724));
#142654=CARTESIAN_POINT('Ctrl Pts',(1.1395365979978,-6.91802593984177,75.3254162411897));
#142655=CARTESIAN_POINT('Ctrl Pts',(1.32145494109673,-6.88806036705973,
75.3337794370112));
#142656=CARTESIAN_POINT('Ctrl Pts',(1.50220227609893,-6.85091292059187,
75.3421426328327));
#142657=CARTESIAN_POINT('Ctrl Pts',(1.68119520106125,-6.80670325917243,
75.3505058286542));
#142658=CARTESIAN_POINT('Ctrl Pts',(1.8602003329826,-6.76249058274263,75.3588695948289));
#142659=CARTESIAN_POINT('Ctrl Pts',(2.03745049700454,-6.71121480962025,
75.3672333610036));
#142660=CARTESIAN_POINT('Ctrl Pts',(2.21237503716852,-6.65304616378194,
75.3755971271783));
#142661=CARTESIAN_POINT('Ctrl Pts',(2.3873348283923,-6.59486579570951,75.3839625788319));
#142662=CARTESIAN_POINT('Ctrl Pts',(2.55996774924811,-6.52978988885687,
75.3923280304855));
#142663=CARTESIAN_POINT('Ctrl Pts',(2.72972038082471,-6.45803787578009,
75.4006934821391));
#142664=CARTESIAN_POINT('Ctrl Pts',(2.89952986222396,-6.38626183309517,
75.409061735366));
#142665=CARTESIAN_POINT('Ctrl Pts',(3.06645682817716,-6.30780535386422,
75.4174299885929));
#142666=CARTESIAN_POINT('Ctrl Pts',(3.22996944408843,-6.22293531645276,
75.4257982418199));
#142667=CARTESIAN_POINT('Ctrl Pts',(3.39363365952154,-6.13798659240899,
75.4341742536114));
#142668=CARTESIAN_POINT('Ctrl Pts',(3.55387690700227,-6.0466125793586,75.4425502654029));
#142669=CARTESIAN_POINT('Ctrl Pts',(3.71019241278406,-5.94912588727282,
75.4509262771944));
#142670=CARTESIAN_POINT('Ctrl Pts',(3.86658457762135,-5.85159138650868,
75.4593063966855));
#142671=CARTESIAN_POINT('Ctrl Pts',(4.01904488418193,-5.74793840807308,
75.4676865161767));
#142672=CARTESIAN_POINT('Ctrl Pts',(4.16709647390175,-5.63852228333768,
75.4760666356679));
#142673=CARTESIAN_POINT('Ctrl Pts',(4.31531723131679,-5.52898113681984,
75.4844563305071));
#142674=CARTESIAN_POINT('Ctrl Pts',(4.45911894531299,-5.41366388624698,
75.4928460253463));
#142675=CARTESIAN_POINT('Ctrl Pts',(4.59805767418991,-5.29296629380192,
75.5012357201855));
#142676=CARTESIAN_POINT('Ctrl Pts',(4.68626747551973,-5.21633747520954,
75.5065621926599));
#142677=CARTESIAN_POINT('Ctrl Pts',(4.77251783043358,-5.13754074699948,
75.5118886651343));
#142678=CARTESIAN_POINT('Ctrl Pts',(4.85670300396802,-5.05668493123193,
75.5172151376086));
#142679=CARTESIAN_POINT('Ctrl Pts',(4.98916989127781,-4.92945684835293,
75.5255964380134));
#142680=CARTESIAN_POINT('Ctrl Pts',(5.11678882345246,-4.79687213146762,
75.5339777384181));
#142681=CARTESIAN_POINT('Ctrl Pts',(5.23911568247115,-4.65932328006813,
75.5423590388229));
#142682=CARTESIAN_POINT('Ctrl Pts',(5.36128751010322,-4.52194875170229,
75.5507297171563));
#142683=CARTESIAN_POINT('Ctrl Pts',(5.47818041481491,-4.37962286960814,
75.5591003954898));
#142684=CARTESIAN_POINT('Ctrl Pts',(5.5893857073991,-4.23277615477391,75.5674710738232));
#142685=CARTESIAN_POINT('Ctrl Pts',(5.70046480106886,-4.08609608574916,
75.5758322528738));
#142686=CARTESIAN_POINT('Ctrl Pts',(5.80586895046219,-3.93490566899011,
75.5841934319245));
#142687=CARTESIAN_POINT('Ctrl Pts',(5.90522820807114,-3.77967014077961,
75.5925546109751));
#142688=CARTESIAN_POINT('Ctrl Pts',(6.00445853532294,-3.62463604897852,
75.6009049404097));
#142689=CARTESIAN_POINT('Ctrl Pts',(6.09765944060215,-3.46556759009271,
75.6092552698443));
#142690=CARTESIAN_POINT('Ctrl Pts',(6.18450299894852,-3.30296067468216,
75.6176055992788));
#142691=CARTESIAN_POINT('Ctrl Pts',(6.27127973637222,-3.14047887556491,
75.6259495036344));
#142692=CARTESIAN_POINT('Ctrl Pts',(6.35170872122839,-2.97446433341784,
75.6342934079901));
#142693=CARTESIAN_POINT('Ctrl Pts',(6.42550628435155,-2.80544034908225,
75.6426373123457));
#142694=CARTESIAN_POINT('Ctrl Pts',(6.49924457281158,-2.63655212586543,
75.6509745148253));
#142695=CARTESIAN_POINT('Ctrl Pts',(6.56636193155825,-2.46465958063462,
75.6593117173048));
#142696=CARTESIAN_POINT('Ctrl Pts',(6.62662138123789,-2.29030906914783,
75.6676489197844));
#142697=CARTESIAN_POINT('Ctrl Pts',(6.64645845945428,-2.23291384314066,
75.6703934808212));
#142698=CARTESIAN_POINT('Ctrl Pts',(6.66555273342515,-2.17525242693332,
75.6731380418581));
#142699=CARTESIAN_POINT('Ctrl Pts',(6.68389688264667,-2.11734480532722,
75.6758826028949));
#142700=CARTESIAN_POINT('Ctrl Pts',(6.73828743675348,-1.94564822849889,
75.6840202490606));
#142701=CARTESIAN_POINT('Ctrl Pts',(6.7860549329571,-1.77186261854291,75.6921578952262));
#142702=CARTESIAN_POINT('Ctrl Pts',(6.82705109833968,-1.5965587565633,75.7002955413919));
#142703=CARTESIAN_POINT('Ctrl Pts',(6.86695367326183,-1.42593120099797,
75.7082161123229));
#142704=CARTESIAN_POINT('Ctrl Pts',(6.90044152218364,-1.25386574377441,
75.716136683254));
#142705=CARTESIAN_POINT('Ctrl Pts',(6.92742985515551,-1.08089877620435,
75.724057254185));
#142706=CARTESIAN_POINT('Ctrl Pts',(6.95552767229749,-0.900821176322602,
75.7323034379679));
#142707=CARTESIAN_POINT('Ctrl Pts',(6.97658018198766,-0.719766819359412,
75.7405496217509));
#142708=CARTESIAN_POINT('Ctrl Pts',(6.99055149854564,-0.538345900589294,
75.7487958055338));
#142709=CARTESIAN_POINT('Ctrl Pts',(7.00452281510362,-0.356924981819176,
75.7570419893167));
#142710=CARTESIAN_POINT('Ctrl Pts',(7.01141296534025,-0.175137957217851,
75.7652881730996));
#142711=CARTESIAN_POINT('Ctrl Pts',(7.01124707280511,0.00640676063271148,
75.7735343568825));
#142712=CARTESIAN_POINT('Ctrl Pts',(7.01124707280455,0.00640676124637189,
75.7735343569104));
#142713=CARTESIAN_POINT('Ctrl Pts',(7.01104249227247,0.23028971888088,75.7837036421222));
#142714=CARTESIAN_POINT('Ctrl Pts',(7.00010998406542,0.453798136459291,
75.7938729273341));
#142715=CARTESIAN_POINT('Ctrl Pts',(6.97858319956023,0.676020036179168,
75.8040422125459));
#142716=CARTESIAN_POINT('Ctrl Pts',(6.95705641505505,0.898241935899045,
75.8142114977577));
#142717=CARTESIAN_POINT('Ctrl Pts',(6.92493548555935,1.11917735600817,75.8243807829695));
#142718=CARTESIAN_POINT('Ctrl Pts',(6.8824094301673,1.33793385413639,75.8345500681813));
#142719=CARTESIAN_POINT('Ctrl Pts',(6.84585080011827,1.5259935698133,75.8432923588192));
#142720=CARTESIAN_POINT('Ctrl Pts',(6.80154666212197,1.71272100934492,75.8520346494571));
#142721=CARTESIAN_POINT('Ctrl Pts',(6.74961410355704,1.89745514191085,75.860776940095));
#142722=CARTESIAN_POINT('Ctrl Pts',(6.69768154499209,2.08218927447684,75.8695192307329));
#142723=CARTESIAN_POINT('Ctrl Pts',(6.6381206211002,2.26492969856719,75.8782615213709));
#142724=CARTESIAN_POINT('Ctrl Pts',(6.57110895151814,2.44502632087635,75.8870038120088));
#142725=CARTESIAN_POINT('',(7.01124999042383,-0.000366444890689146,75.2264656430566));
#142726=CARTESIAN_POINT('Ctrl Pts',(6.57110895151811,2.44502632087644,75.339916226746));
#142727=CARTESIAN_POINT('Ctrl Pts',(6.63820287688893,2.26470863274675,75.3311830274232));
#142728=CARTESIAN_POINT('Ctrl Pts',(6.69785902018697,2.08165885386196,75.3224498281004));
#142729=CARTESIAN_POINT('Ctrl Pts',(6.74988410723788,1.89649442428854,75.3137166287776));
#142730=CARTESIAN_POINT('Ctrl Pts',(6.80193302667208,1.71124517198998,75.3049794288281));
#142731=CARTESIAN_POINT('Ctrl Pts',(6.84634382896498,1.52387959651581,75.2962422288786));
#142732=CARTESIAN_POINT('Ctrl Pts',(6.88297349805567,1.3350289837915,75.287505028929));
#142733=CARTESIAN_POINT('Ctrl Pts',(6.91960826284139,1.1461520993275,75.2787666135138));
#142734=CARTESIAN_POINT('Ctrl Pts',(6.94845968467338,0.955790034550496,
75.2700281980986));
#142735=CARTESIAN_POINT('Ctrl Pts',(6.96943605429437,0.76458331632448,75.2612897826833));
#142736=CARTESIAN_POINT('Ctrl Pts',(6.9904174952856,0.573330370840038,75.2525492546175));
#142737=CARTESIAN_POINT('Ctrl Pts',(7.00352005089385,0.38123263605352,75.2438087265516));
#142738=CARTESIAN_POINT('Ctrl Pts',(7.00870385634683,0.188936011731862,
75.2350681984858));
#142739=CARTESIAN_POINT('Ctrl Pts',(7.01040451536259,0.125848962879511,
75.2322006800204));
#142740=CARTESIAN_POINT('Ctrl Pts',(7.01125328872049,0.0627405290793296,
75.2293331615549));
#142741=CARTESIAN_POINT('Ctrl Pts',(7.01124999042387,-0.000366444165664637,
75.2264656430895));
#142742=CARTESIAN_POINT('Ctrl Pts',(7.01124999042383,-0.000366444890591926,
75.2264656430566));
#142743=CARTESIAN_POINT('Ctrl Pts',(7.01124305565536,-0.133050503537697,
75.2204366106267));
#142744=CARTESIAN_POINT('Ctrl Pts',(7.00746885027525,-0.26572305004299,
75.2144075781969));
#142745=CARTESIAN_POINT('Ctrl Pts',(6.99993417826155,-0.39818094191683,
75.2083785457671));
#142746=CARTESIAN_POINT('Ctrl Pts',(6.98901066912309,-0.590213851871724,
75.1996378612723));
#142747=CARTESIAN_POINT('Ctrl Pts',(6.97018003265678,-0.781807211055622,
75.1908971767776));
#142748=CARTESIAN_POINT('Ctrl Pts',(6.94350245760761,-0.972316915258118,
75.1821564922828));
#142749=CARTESIAN_POINT('Ctrl Pts',(6.91682968229739,-1.16279234359993,
75.1734173803823));
#142750=CARTESIAN_POINT('Ctrl Pts',(6.88231282582201,-1.35218423527349,
75.1646782684819));
#142751=CARTESIAN_POINT('Ctrl Pts',(6.84006372184559,-1.5398554619158,75.1559391565815));
#142752=CARTESIAN_POINT('Ctrl Pts',(6.79726721990968,-1.72995823945147,
75.1470868169064));
#142753=CARTESIAN_POINT('Ctrl Pts',(6.74653674960314,-1.91829517075989,
75.1382344772314));
#142754=CARTESIAN_POINT('Ctrl Pts',(6.68804192720558,-2.1042152319666,75.1293821375563));
#142755=CARTESIAN_POINT('Ctrl Pts',(6.63032489371786,-2.28766316733728,
75.120647504908));
#142756=CARTESIAN_POINT('Ctrl Pts',(6.56504880416474,-2.46875784249007,
75.1119128722598));
#142757=CARTESIAN_POINT('Ctrl Pts',(6.49242690110756,-2.64688864447957,
75.1031782396115));
#142758=CARTESIAN_POINT('Ctrl Pts',(6.41833702991177,-2.8286201554951,75.094267046423));
#142759=CARTESIAN_POINT('Ctrl Pts',(6.3366012975286,-3.00726641754748,75.0853558532346));
#142760=CARTESIAN_POINT('Ctrl Pts',(6.24749837444822,-3.18219902328042,
75.0764446600462));
#142761=CARTESIAN_POINT('Ctrl Pts',(6.15839545136785,-3.35713162901335,
75.0675334668577));
#142762=CARTESIAN_POINT('Ctrl Pts',(6.06192546316565,-3.52835030220223,
75.0586222736693));
#142763=CARTESIAN_POINT('Ctrl Pts',(5.95841812638889,-3.69525100549615,
75.0497110804809));
#142764=CARTESIAN_POINT('Ctrl Pts',(5.86519658161795,-3.8455663538465,75.0416854156281));
#142765=CARTESIAN_POINT('Ctrl Pts',(5.76622355082883,-3.99244807420047,
75.0336597507752));
#142766=CARTESIAN_POINT('Ctrl Pts',(5.66179063329981,-4.13542662698524,
75.0256340859224));
#142767=CARTESIAN_POINT('Ctrl Pts',(5.55739086021743,-4.27835980188414,
75.0176109682188));
#142768=CARTESIAN_POINT('Ctrl Pts',(5.44753486626134,-4.41739197982342,
75.0095878505151));
#142769=CARTESIAN_POINT('Ctrl Pts',(5.33255737107235,-4.55208286905258,
75.0015647328115));
#142770=CARTESIAN_POINT('Ctrl Pts',(5.21759437555166,-4.68675677258193,
74.9935426268932));
#142771=CARTESIAN_POINT('Ctrl Pts',(5.09751140366893,-4.81709019956761,
74.985520520975));
#142772=CARTESIAN_POINT('Ctrl Pts',(4.97268318744038,-4.94267624671572,
74.9774984150567));
#142773=CARTESIAN_POINT('Ctrl Pts',(4.84780858462505,-5.06830896206314,
74.9694733280968));
#142774=CARTESIAN_POINT('Ctrl Pts',(4.71818547138304,-5.189190511028,74.9614482411368));
#142775=CARTESIAN_POINT('Ctrl Pts',(4.58422546114696,-5.30495084650857,
74.9534231541769));
#142776=CARTESIAN_POINT('Ctrl Pts',(4.45023906815718,-5.42073398040796,
74.9453964867162));
#142777=CARTESIAN_POINT('Ctrl Pts',(4.31191435971892,-5.53139365852342,
74.9373698192556));
#142778=CARTESIAN_POINT('Ctrl Pts',(4.16969552258898,-5.63660055453652,
74.9293431517949));
#142779=CARTESIAN_POINT('Ctrl Pts',(4.02736251267753,-5.74189191027517,
74.9213100405539));
#142780=CARTESIAN_POINT('Ctrl Pts',(3.88112943045361,-5.84172153050869,
74.9132769293129));
#142781=CARTESIAN_POINT('Ctrl Pts',(3.73146940036782,-5.93580345670396,
74.9052438180719));
#142782=CARTESIAN_POINT('Ctrl Pts',(3.64328427399438,-5.99123994529901,
74.9005104171127));
#142783=CARTESIAN_POINT('Ctrl Pts',(3.55390981724565,-6.04468168800366,
74.8957770161535));
#142784=CARTESIAN_POINT('Ctrl Pts',(3.46344666392992,-6.09607773643125,
74.8910436151943));
#142785=CARTESIAN_POINT('Ctrl Pts',(3.27708975261288,-6.20195519579238,
74.8812926619006));
#142786=CARTESIAN_POINT('Ctrl Pts',(3.08600197742468,-6.29921177698256,
74.8715417086069));
#142787=CARTESIAN_POINT('Ctrl Pts',(2.89092393913194,-6.3875022771545,74.8617907553132));
#142788=CARTESIAN_POINT('Ctrl Pts',(2.69556485432981,-6.4759199763546,74.8520257539421));
#142789=CARTESIAN_POINT('Ctrl Pts',(2.49620404248284,-6.55534574016212,
74.842260752571));
#142790=CARTESIAN_POINT('Ctrl Pts',(2.2936039834245,-6.62548166775211,74.8324957511999));
#142791=CARTESIAN_POINT('Ctrl Pts',(2.09134161668606,-6.6955006932829,74.8227470260628));
#142792=CARTESIAN_POINT('Ctrl Pts',(1.88585082927563,-6.75626081688636,
74.8129983009257));
#142793=CARTESIAN_POINT('Ctrl Pts',(1.67790829224755,-6.80751425450633,
74.8032495757885));
#142794=CARTESIAN_POINT('Ctrl Pts',(1.47053647685398,-6.85862702131354,
74.7935276071218));
#142795=CARTESIAN_POINT('Ctrl Pts',(1.2607263841683,-6.90028518132652,74.7838056384552));
#142796=CARTESIAN_POINT('Ctrl Pts',(1.04926570132366,-6.93229168821724,
74.7740836697885));
#142797=CARTESIAN_POINT('Ctrl Pts',(0.839204198585687,-6.96408641641168,
74.7644260288492));
#142798=CARTESIAN_POINT('Ctrl Pts',(0.627513918363548,-6.98635675871692,
74.7547683879098));
#142799=CARTESIAN_POINT('Ctrl Pts',(0.414983637407091,-6.99895814698048,
74.7451107469705));
#142800=CARTESIAN_POINT('Ctrl Pts',(0.321569261902796,-7.00449689096477,
74.740865881283));
#142801=CARTESIAN_POINT('Ctrl Pts',(0.227992819344614,-7.00816832190245,
74.7366210155955));
#142802=CARTESIAN_POINT('Ctrl Pts',(0.1343222813047,-7.00996320156141,74.732376149908));
#142803=CARTESIAN_POINT('Ctrl Pts',(-0.0389427377908712,-7.01328324076362,
74.724524302894));
#142804=CARTESIAN_POINT('Ctrl Pts',(-0.212458611612996,-7.01017750829806,
74.71667245588));
#142805=CARTESIAN_POINT('Ctrl Pts',(-0.385691713602764,-7.00063343309434,
74.7088206088661));
#142806=CARTESIAN_POINT('Ctrl Pts',(-0.558875688085379,-6.99109206451318,
74.7009709885724));
#142807=CARTESIAN_POINT('Ctrl Pts',(-0.731776669740262,-6.97511600610928,
74.6931213682788));
#142808=CARTESIAN_POINT('Ctrl Pts',(-0.903861994686435,-6.9527447858426,
74.6852717479852));
#142809=CARTESIAN_POINT('Ctrl Pts',(-1.07593358082064,-6.9303753516317,
74.6774227543833));
#142810=CARTESIAN_POINT('Ctrl Pts',(-1.24718926169736,-6.9016118218864,
74.6695737607814));
#142811=CARTESIAN_POINT('Ctrl Pts',(-1.41710271543123,-6.86654545287639,
74.6617247671796));
#142812=CARTESIAN_POINT('Ctrl Pts',(-1.58710219137103,-6.83146133079063,
74.6538717998621));
#142813=CARTESIAN_POINT('Ctrl Pts',(-1.75575770835422,-6.79006807097766,
74.6460188325446));
#142814=CARTESIAN_POINT('Ctrl Pts',(-1.92255400822254,-6.74250789009308,
74.6381658652272));
#142815=CARTESIAN_POINT('Ctrl Pts',(-2.08939266874659,-6.6949356305206,
74.6303109035198));
#142816=CARTESIAN_POINT('Ctrl Pts',(-2.25437080871741,-6.64119344782468,
74.6224559418125));
#142817=CARTESIAN_POINT('Ctrl Pts',(-2.41699013619184,-6.58147287801533,
74.6146009801052));
#142818=CARTESIAN_POINT('Ctrl Pts',(-2.57977087694202,-6.52169303054844,
74.6067382216918));
#142819=CARTESIAN_POINT('Ctrl Pts',(-2.74018777618854,-6.45592308880591,
74.5988754632784));
#142820=CARTESIAN_POINT('Ctrl Pts',(-2.89776373376264,-6.3844022355887,
74.591012704865));
#142821=CARTESIAN_POINT('Ctrl Pts',(-3.01335919515147,-6.33193556393495,
74.5852446981172));
#142822=CARTESIAN_POINT('Ctrl Pts',(-3.12742626232804,-6.27637504553682,
74.5794766913693));
#142823=CARTESIAN_POINT('Ctrl Pts',(-3.23978591027583,-6.21783031435229,
74.5737086846215));
#142824=CARTESIAN_POINT('Ctrl Pts',(-3.40298901265608,-6.13279372041624,
74.5653306181805));
#142825=CARTESIAN_POINT('Ctrl Pts',(-3.56295046482632,-6.0412712863507,
74.5569525517394));
#142826=CARTESIAN_POINT('Ctrl Pts',(-3.71914210934023,-5.94353501992142,
74.5485744852984));
#142827=CARTESIAN_POINT('Ctrl Pts',(-3.87522695186342,-5.84586558438987,
74.5402021476796));
#142828=CARTESIAN_POINT('Ctrl Pts',(-4.02754684822451,-5.74199096145036,
74.5318298100608));
#142829=CARTESIAN_POINT('Ctrl Pts',(-4.17559910596613,-5.63222857035782,
74.5234574724421));
#142830=CARTESIAN_POINT('Ctrl Pts',(-4.32357183929446,-5.52252513675695,
74.5150896319195));
#142831=CARTESIAN_POINT('Ctrl Pts',(-4.46728124117143,-5.40694043614627,
74.5067217913969));
#142832=CARTESIAN_POINT('Ctrl Pts',(-4.60625405735394,-5.2858348556884,
74.4983539508742));
#142833=CARTESIAN_POINT('Ctrl Pts',(-4.74517258454004,-5.1647765844857,
74.4899893792043));
#142834=CARTESIAN_POINT('Ctrl Pts',(-4.87935796838435,-5.03820194984778,
74.4816248075344));
#142835=CARTESIAN_POINT('Ctrl Pts',(-5.00837012799905,-4.90651151261941,
74.4732602358644));
#142836=CARTESIAN_POINT('Ctrl Pts',(-5.13735077396163,-4.77485324326295,
74.4648977073988));
#142837=CARTESIAN_POINT('Ctrl Pts',(-5.26116048622779,-4.63808189826811,
74.4565351789332));
#142838=CARTESIAN_POINT('Ctrl Pts',(-5.37939582343618,-4.49663509052017,
74.4481726504676));
#142839=CARTESIAN_POINT('Ctrl Pts',(-5.4976405961943,-4.35517699487457,
74.4398094546461));
#142840=CARTESIAN_POINT('Ctrl Pts',(-5.61030988971596,-4.20904293933965,
74.4314462588245));
#142841=CARTESIAN_POINT('Ctrl Pts',(-5.71703988043465,-4.05870441988817,
74.423083063003));
#142842=CARTESIAN_POINT('Ctrl Pts',(-5.82377714992473,-3.90835564765107,
74.4147192968283));
#142843=CARTESIAN_POINT('Ctrl Pts',(-5.92457411841075,-3.75380210773928,
74.4063555306535));
#142844=CARTESIAN_POINT('Ctrl Pts',(-6.01910962728595,-3.59554527953878,
74.3979917644788));
#142845=CARTESIAN_POINT('Ctrl Pts',(-6.11366418710039,-3.43725655918205,
74.3896263128252));
#142846=CARTESIAN_POINT('Ctrl Pts',(-6.20195460260811,-3.27526334467866,
74.3812608611716));
#142847=CARTESIAN_POINT('Ctrl Pts',(-6.28370489658267,-3.11009313930677,
74.3728954095181));
#142848=CARTESIAN_POINT('Ctrl Pts',(-6.36548256856999,-2.94486761875777,
74.3645271562912));
#142849=CARTESIAN_POINT('Ctrl Pts',(-6.44071560577069,-2.77646328030718,
74.3561589030643));
#142850=CARTESIAN_POINT('Ctrl Pts',(-6.50917535472009,-2.60542947784135,
74.3477906498374));
#142851=CARTESIAN_POINT('Ctrl Pts',(-6.5776985756236,-2.43423710264003,
74.3394146380459));
#142852=CARTESIAN_POINT('Ctrl Pts',(-6.63943583704861,-2.26041069735044,
74.3310386262544));
#142853=CARTESIAN_POINT('Ctrl Pts',(-6.69420732378028,-2.08451789839918,
74.3226626144629));
#142854=CARTESIAN_POINT('Ctrl Pts',(-6.74900567112578,-1.90853883944601,
74.3142824949717));
#142855=CARTESIAN_POINT('Ctrl Pts',(-6.79683133996748,-1.73049168160572,
74.3059023754806));
#142856=CARTESIAN_POINT('Ctrl Pts',(-6.837555065492,-1.55095689458627,74.2975222559894));
#142857=CARTESIAN_POINT('Ctrl Pts',(-6.87832532303154,-1.37121696633039,
74.2891325611502));
#142858=CARTESIAN_POINT('Ctrl Pts',(-6.91197735568421,-1.18998633446477,
74.2807428663109));
#142859=CARTESIAN_POINT('Ctrl Pts',(-6.93843322754421,-1.00785460727745,
74.2723531714717));
#142860=CARTESIAN_POINT('Ctrl Pts',(-6.95522960404522,-0.892222316691677,
74.2670266989973));
#142861=CARTESIAN_POINT('Ctrl Pts',(-6.96912642305545,-0.776226943848889,
74.2617002265229));
#142862=CARTESIAN_POINT('Ctrl Pts',(-6.9801146287026,-0.660019948692465,
74.2563737540485));
#142863=CARTESIAN_POINT('Ctrl Pts',(-6.99740476826138,-0.477166148128354,
74.2479924536438));
#142864=CARTESIAN_POINT('Ctrl Pts',(-7.00752560932667,-0.293419399647785,
74.239611153239));
#142865=CARTESIAN_POINT('Ctrl Pts',(-7.01039695250091,-0.10936695509142,
74.2312298528342));
#142866=CARTESIAN_POINT('Ctrl Pts',(-7.01326465666801,0.0744522299348578,
74.2228591745008));
#142867=CARTESIAN_POINT('Ctrl Pts',(-7.00890116796128,0.258576013983379,
74.2144884961673));
#142868=CARTESIAN_POINT('Ctrl Pts',(-6.99727794591041,0.442411471569036,
74.2061178178339));
#142869=CARTESIAN_POINT('Ctrl Pts',(-6.98566791422094,0.626038307473389,
74.1977566387832));
#142870=CARTESIAN_POINT('Ctrl Pts',(-6.96681459007466,0.809377144052614,
74.1893954597325));
#142871=CARTESIAN_POINT('Ctrl Pts',(-6.94074144317346,0.991834049382468,
74.1810342806818));
#142872=CARTESIAN_POINT('Ctrl Pts',(-6.91470212925596,1.17405419535501,
74.1726839512472));
#142873=CARTESIAN_POINT('Ctrl Pts',(-6.88146172532469,1.35539436990032,
74.1643336218126));
#142874=CARTESIAN_POINT('Ctrl Pts',(-6.84109555853296,1.53526483758362,
74.155983292378));
#142875=CARTESIAN_POINT('Ctrl Pts',(-6.80076045109191,1.7149969057017,74.1476393880224));
#142876=CARTESIAN_POINT('Ctrl Pts',(-6.75331057855019,1.89326120219734,
74.1392954836668));
#142877=CARTESIAN_POINT('Ctrl Pts',(-6.69887267340664,2.06947613370769,
74.1309515793112));
#142878=CARTESIAN_POINT('Ctrl Pts',(-6.644478493128,2.24554952828614,74.1226143768316));
#142879=CARTESIAN_POINT('Ctrl Pts',(-6.58310757067069,2.41957652857064,
74.114277174352));
#142880=CARTESIAN_POINT('Ctrl Pts',(-6.51493705751346,2.59098855635022,
74.1059399718724));
#142881=CARTESIAN_POINT('Ctrl Pts',(-6.49249570086895,2.64741644973706,
74.1031954108357));
#142882=CARTESIAN_POINT('Ctrl Pts',(-6.46931788326026,2.70356107537436,
74.100450849799));
#142883=CARTESIAN_POINT('Ctrl Pts',(-6.44541110559441,2.75940251546966,
74.0977062887623));
#142884=CARTESIAN_POINT('Ctrl Pts',(-6.3727794068148,2.92905560352325,74.0893679784603));
#142885=CARTESIAN_POINT('Ctrl Pts',(-6.29347528529295,3.09576958922796,
74.0810296681583));
#142886=CARTESIAN_POINT('Ctrl Pts',(-6.20777312730868,3.25901509084634,
74.0726913578563));
#142887=CARTESIAN_POINT('Ctrl Pts',(-6.12201704843473,3.42236330099496,
74.0643478013724));
#142888=CARTESIAN_POINT('Ctrl Pts',(-6.02985505618335,3.58223838418103,
74.0560042448885));
#142889=CARTESIAN_POINT('Ctrl Pts',(-5.9316064869784,3.7381373765735,74.0476606884046));
#142890=CARTESIAN_POINT('Ctrl Pts',(-5.83328317069005,3.89415497624015,
74.0393107841793));
#142891=CARTESIAN_POINT('Ctrl Pts',(-5.72886421532385,4.04619017435708,
74.030960879954));
#142892=CARTESIAN_POINT('Ctrl Pts',(-5.61871132563447,4.19377033249163,
74.0226109757286));
#142893=CARTESIAN_POINT('Ctrl Pts',(-5.50839321476202,4.34157184994224,
74.0142485472649));
#142894=CARTESIAN_POINT('Ctrl Pts',(-5.3923241792621,4.48490471141038,74.0058861188011));
#142895=CARTESIAN_POINT('Ctrl Pts',(-5.27090610600303,4.6233294695706,73.9975236903374));
#142896=CARTESIAN_POINT('Ctrl Pts',(-5.14938420373964,4.76187259976909,
73.9891541108573));
#142897=CARTESIAN_POINT('Ctrl Pts',(-5.02250436216349,4.89549901532504,
73.9807845313772));
#142898=CARTESIAN_POINT('Ctrl Pts',(-4.89070451905666,5.02380691008111,
73.9724149518972));
#142899=CARTESIAN_POINT('Ctrl Pts',(-4.7587013907501,5.15231270413205,73.9640324633605));
#142900=CARTESIAN_POINT('Ctrl Pts',(-4.62176333995414,5.27548336631318,
73.9556499748238));
#142901=CARTESIAN_POINT('Ctrl Pts',(-4.48036155506989,5.3929571571033,73.9472674862872));
#142902=CARTESIAN_POINT('Ctrl Pts',(-4.43409257406062,5.43139650636332,
73.9445245986834));
#142903=CARTESIAN_POINT('Ctrl Pts',(-4.38734588960136,5.46922623406694,
73.9417817110796));
#142904=CARTESIAN_POINT('Ctrl Pts',(-4.34013865785259,5.50643468980733,
73.9390388234758));
#142905=CARTESIAN_POINT('Ctrl Pts',(-4.19574271722301,5.62024670053062,
73.930648968343));
#142906=CARTESIAN_POINT('Ctrl Pts',(-4.04674420327156,5.72847259738453,
73.9222591132102));
#142907=CARTESIAN_POINT('Ctrl Pts',(-3.89360220379064,5.83073652647217,
73.9138692580775));
#142908=CARTESIAN_POINT('Ctrl Pts',(-3.74060152159998,5.93290608783965,
73.9054871449854));
#142909=CARTESIAN_POINT('Ctrl Pts',(-3.58346524818031,6.0291244672418,73.8971050318933));
#142910=CARTESIAN_POINT('Ctrl Pts',(-3.42268409254751,6.1190571304019,73.8887229188012));
#142911=CARTESIAN_POINT('Ctrl Pts',(-3.26202766901513,6.20892002487592,
73.8803473084524));
#142912=CARTESIAN_POINT('Ctrl Pts',(-3.09773228662066,6.29250676523242,
73.8719716981035));
#142913=CARTESIAN_POINT('Ctrl Pts',(-2.93031646353258,6.36952682591493,
73.8635960877547));
#142914=CARTESIAN_POINT('Ctrl Pts',(-2.76300594748313,6.44649843983563,
73.8552257457891));
#142915=CARTESIAN_POINT('Ctrl Pts',(-2.59257920226384,6.51691147297106,
73.8468554038236));
#142916=CARTESIAN_POINT('Ctrl Pts',(-2.41957851456268,6.58052174028524,
73.838485061858));
#142917=CARTESIAN_POINT('Ctrl Pts',(-2.24666128690485,6.64410132034761,
73.8301187579637));
#142918=CARTESIAN_POINT('Ctrl Pts',(-2.0711729009687,6.70088456585241,73.8217524540694));
#142919=CARTESIAN_POINT('Ctrl Pts',(-1.89367517636312,6.75067558759315,
73.813386150175));
#142920=CARTESIAN_POINT('Ctrl Pts',(-1.71622709289637,6.80045268418061,
73.8050221861015));
#142921=CARTESIAN_POINT('Ctrl Pts',(-1.53677110706267,6.84324136622197,
73.7966582220278));
#142922=CARTESIAN_POINT('Ctrl Pts',(-1.35588427386249,6.87889557984364,
73.7882942579542));
#142923=CARTESIAN_POINT('Ctrl Pts',(-1.17502527613985,6.91454430687436,
73.7799315809557));
#142924=CARTESIAN_POINT('Ctrl Pts',(-0.992736192412884,6.94306069089118,
73.7715689039572));
#142925=CARTESIAN_POINT('Ctrl Pts',(-0.809604761811532,6.96434969628551,
73.7632062269587));
#142926=CARTESIAN_POINT('Ctrl Pts',(-0.626477101551507,6.98563826337814,
73.7548437221324));
#142927=CARTESIAN_POINT('Ctrl Pts',(-0.442507455494422,6.99969971100225,
73.7464812173061));
#142928=CARTESIAN_POINT('Ctrl Pts',(-0.258289619035452,7.00649077892767,
73.7381187124798));
#142929=CARTESIAN_POINT('Ctrl Pts',(-0.0740510203588375,7.01328261223843,
73.7297552651598));
#142930=CARTESIAN_POINT('Ctrl Pts',(0.110435496055611,7.0128024206199,73.7213918178398));
#142931=CARTESIAN_POINT('Ctrl Pts',(0.29457475621586,7.00505904868049,73.7130283705199));
#142932=CARTESIAN_POINT('Ctrl Pts',(0.478822442747335,6.99731111722607,
73.7046599985671));
#142933=CARTESIAN_POINT('Ctrl Pts',(0.662722135685751,6.98229147231949,
73.6962916266143));
#142934=CARTESIAN_POINT('Ctrl Pts',(0.845681362458587,6.96006103390554,
73.6879232546615));
#142935=CARTESIAN_POINT('Ctrl Pts',(1.0286954085976,6.93782393467121,73.6795523753258));
#142936=CARTESIAN_POINT('Ctrl Pts',(1.2107681010083,6.90837177876362,73.67118149599));
#142937=CARTESIAN_POINT('Ctrl Pts',(1.39131508590212,6.87181700092786,73.6628106166543));
#142938=CARTESIAN_POINT('Ctrl Pts',(1.57201504630374,6.83523125062416,73.654432644763));
#142939=CARTESIAN_POINT('Ctrl Pts',(1.75118639480659,6.79153092394869,73.6460546728717));
#142940=CARTESIAN_POINT('Ctrl Pts',(1.92825677760947,6.74087919800549,73.6376767009805));
#142941=CARTESIAN_POINT('Ctrl Pts',(2.04078644777437,6.70868961370886,73.6323524316213));
#142942=CARTESIAN_POINT('Ctrl Pts',(2.15246788626534,6.67369357447061,73.6270281622621));
#142943=CARTESIAN_POINT('Ctrl Pts',(2.26315789621714,6.63594325618371,73.6217038929029));
#142944=CARTESIAN_POINT('Ctrl Pts',(2.42662386757941,6.58019393923369,73.6138410617136));
#142945=CARTESIAN_POINT('Ctrl Pts',(2.58826656138551,6.51831926484873,73.6059782305243));
#142946=CARTESIAN_POINT('Ctrl Pts',(2.74757357211221,6.45046246623686,73.598115399335));
#142947=CARTESIAN_POINT('Ctrl Pts',(2.90675817642966,6.38265780661764,73.5902586096936));
#142948=CARTESIAN_POINT('Ctrl Pts',(3.06361031810684,6.30888031196602,73.5824018200522));
#142949=CARTESIAN_POINT('Ctrl Pts',(3.2176331264742,6.22932288663189,73.5745450304108));
#142950=CARTESIAN_POINT('Ctrl Pts',(3.37156907326855,6.14981032791968,73.5666926716268));
#142951=CARTESIAN_POINT('Ctrl Pts',(3.52267852309253,6.06452449706037,73.5588403128428));
#142952=CARTESIAN_POINT('Ctrl Pts',(3.67048520232653,5.97370613120548,73.5509879540589));
#142953=CARTESIAN_POINT('Ctrl Pts',(3.81825698267898,5.88290920862642,73.5431374493084));
#142954=CARTESIAN_POINT('Ctrl Pts',(3.96272721553292,5.78658254317437,73.535286944558));
#142955=CARTESIAN_POINT('Ctrl Pts',(4.10344489977822,5.68501244651093,73.5274364398075));
#142956=CARTESIAN_POINT('Ctrl Pts',(4.24413994698325,5.58345868927477,73.5195871979559));
#142957=CARTESIAN_POINT('Ctrl Pts',(4.38108333970336,5.47666340572829,73.5117379561042));
#142958=CARTESIAN_POINT('Ctrl Pts',(4.51385409986448,5.36495551963263,73.5038887142526));
#142959=CARTESIAN_POINT('Ctrl Pts',(4.64666959309339,5.25320999696372,73.4960368278377));
#142960=CARTESIAN_POINT('Ctrl Pts',(4.77530935348191,5.13654881152433,73.4881849414228));
#142961=CARTESIAN_POINT('Ctrl Pts',(4.89938632363381,5.01534048837065,73.4803330550079));
#142962=CARTESIAN_POINT('Ctrl Pts',(4.99049449845879,4.92633872533108,73.4745675125441));
#142963=CARTESIAN_POINT('Ctrl Pts',(5.07914321494787,4.83488608072522,73.4688019700803));
#142964=CARTESIAN_POINT('Ctrl Pts',(5.16519231646955,4.74114067460395,73.4630364276165));
#142965=CARTESIAN_POINT('Ctrl Pts',(5.3091382818708,4.58432006000798,73.4533916252729));
#142966=CARTESIAN_POINT('Ctrl Pts',(5.44573570756597,4.42116291705853,73.4437468229294));
#142967=CARTESIAN_POINT('Ctrl Pts',(5.57452589644171,4.25232731482429,73.4341020205858));
#142968=CARTESIAN_POINT('Ctrl Pts',(5.70432389576355,4.08217053832135,73.4243817456256));
#142969=CARTESIAN_POINT('Ctrl Pts',(5.82619199054581,3.90624614694125,73.4146614706654));
#142970=CARTESIAN_POINT('Ctrl Pts',(5.93970849948159,3.72525026054441,73.4049411957052));
#142971=CARTESIAN_POINT('Ctrl Pts',(6.05356126387142,3.54371823315333,73.3951921276162));
#142972=CARTESIAN_POINT('Ctrl Pts',(6.1590129034956,3.35708467698042,73.3854430595271));
#142973=CARTESIAN_POINT('Ctrl Pts',(6.25568581308494,3.16607352575203,73.375693991438));
#142974=CARTESIAN_POINT('Ctrl Pts',(6.35251836848934,2.9747469383683,73.3659288237206));
#142975=CARTESIAN_POINT('Ctrl Pts',(6.44054316953447,2.77902832587818,73.3561636560031));
#142976=CARTESIAN_POINT('Ctrl Pts',(6.51942859313609,2.57966613760379,73.3463984882856));
#142977=CARTESIAN_POINT('Ctrl Pts',(6.53711577681312,2.53496642653839,73.3442090050178));
#142978=CARTESIAN_POINT('Ctrl Pts',(6.55434369867958,2.49008362846496,73.3420195217499));
#142979=CARTESIAN_POINT('Ctrl Pts',(6.57110895151812,2.44502632087643,73.339830038482));
#142980=CARTESIAN_POINT('Origin',(0.,0.,50.));
#142981=CARTESIAN_POINT('',(6.57110895151817,2.44502632087629,71.3398522865014));
#142982=CARTESIAN_POINT('',(6.57110895151816,2.44502632087631,71.8867112926201));
#142983=CARTESIAN_POINT('',(6.57110895151814,2.44502632087636,50.));
#142984=CARTESIAN_POINT('',(7.0112497650765,-0.00181499715760335,73.7735343569104));
#142985=CARTESIAN_POINT('Ctrl Pts',(6.57110895151816,2.44502632087631,71.8867112926201));
#142986=CARTESIAN_POINT('Ctrl Pts',(6.49663749355182,2.64517143174769,71.896403236564));
#142987=CARTESIAN_POINT('Ctrl Pts',(6.41310542934644,2.84167750050844,71.9060951805078));
#142988=CARTESIAN_POINT('Ctrl Pts',(6.32088104020746,3.03382422662321,71.9157871244517));
#142989=CARTESIAN_POINT('Ctrl Pts',(6.22811547998219,3.22709846633247,71.9255359405514));
#142990=CARTESIAN_POINT('Ctrl Pts',(6.12655532786914,3.41596202306511,71.935284756651));
#142991=CARTESIAN_POINT('Ctrl Pts',(6.01661860960486,3.59971208141103,71.9450335727507));
#142992=CARTESIAN_POINT('Ctrl Pts',(5.90651695262479,3.78373782106823,71.9547970150575));
#142993=CARTESIAN_POINT('Ctrl Pts',(5.78801361952856,3.96263468803567,71.9645604573643));
#142994=CARTESIAN_POINT('Ctrl Pts',(5.6615710320532,4.13572726512714,71.9743238996711));
#142995=CARTESIAN_POINT('Ctrl Pts',(5.53523478523948,4.30867426801344,71.9840791307341));
#142996=CARTESIAN_POINT('Ctrl Pts',(5.40097266211013,4.47582671490287,71.9938343617971));
#142997=CARTESIAN_POINT('Ctrl Pts',(5.25928775646086,4.63654169152407,72.00358959286));
#142998=CARTESIAN_POINT('Ctrl Pts',(5.148221290281,4.76252578583319,72.0112366956757));
#142999=CARTESIAN_POINT('Ctrl Pts',(5.03259437926697,4.88455467989839,72.0188837984914));
#143000=CARTESIAN_POINT('Ctrl Pts',(4.91266726452391,5.00233214716648,72.0265309013071));
#143001=CARTESIAN_POINT('Ctrl Pts',(4.78668753017622,5.12605374315723,72.0345639469058));
#143002=CARTESIAN_POINT('Ctrl Pts',(4.65589946607834,5.24514239954313,72.0425969925046));
#143003=CARTESIAN_POINT('Ctrl Pts',(4.52068546131911,5.35920045550808,72.0506300381033));
#143004=CARTESIAN_POINT('Ctrl Pts',(4.38555837732815,5.4731851905632,72.058657919751));
#143005=CARTESIAN_POINT('Ctrl Pts',(4.24601129507244,5.58214552691228,72.0666858013987));
#143006=CARTESIAN_POINT('Ctrl Pts',(4.10246291680207,5.68572111334735,72.0747136830464));
#143007=CARTESIAN_POINT('Ctrl Pts',(3.95897935203999,5.78924993438382,72.0827379400264));
#143008=CARTESIAN_POINT('Ctrl Pts',(3.81149838510998,5.88739863239531,72.0907621970064));
#143009=CARTESIAN_POINT('Ctrl Pts',(3.66047116582932,5.97984760730841,72.0987864539863));
#143010=CARTESIAN_POINT('Ctrl Pts',(3.50946220727736,6.07228540419905,72.106809740752));
#143011=CARTESIAN_POINT('Ctrl Pts',(3.35490815886445,6.15902465282508,72.1148330275176));
#143012=CARTESIAN_POINT('Ctrl Pts',(3.19728862277623,6.23978942154026,72.1228563142832));
#143013=CARTESIAN_POINT('Ctrl Pts',(3.03968200220254,6.32054757230331,72.130878943612));
#143014=CARTESIAN_POINT('Ctrl Pts',(2.87901072243325,6.39533205468025,72.1389015729409));
#143015=CARTESIAN_POINT('Ctrl Pts',(2.71577814403288,6.46391333751415,72.1469242022697));
#143016=CARTESIAN_POINT('Ctrl Pts',(2.55248420180427,6.53252040202779,72.154949847536));
#143017=CARTESIAN_POINT('Ctrl Pts',(2.38662737680296,6.59491946920017,72.1629754928023));
#143018=CARTESIAN_POINT('Ctrl Pts',(2.21873047903218,6.65092938046358,72.1710011380686));
#143019=CARTESIAN_POINT('Ctrl Pts',(2.11972823696198,6.68395623722421,72.1757335475769));
#143020=CARTESIAN_POINT('Ctrl Pts',(2.02001699363196,6.71476251525016,72.1804659570852));
#143021=CARTESIAN_POINT('Ctrl Pts',(1.91970626837374,6.7433192424552,72.1851983665935));
#143022=CARTESIAN_POINT('Ctrl Pts',(1.73465940617335,6.79599888115189,72.1939284154283));
#143023=CARTESIAN_POINT('Ctrl Pts',(1.54747933220094,6.84104703880505,72.2026584642631));
#143024=CARTESIAN_POINT('Ctrl Pts',(1.35879712463329,6.87832079337598,72.2113885130979));
#143025=CARTESIAN_POINT('Ctrl Pts',(1.17006035937003,6.91560532569952,72.2201210862372));
#143026=CARTESIAN_POINT('Ctrl Pts',(0.979820862286258,6.94511091476385,
72.2288536593765));
#143027=CARTESIAN_POINT('Ctrl Pts',(0.788719045880268,6.96674592827711,
72.2375862325158));
#143028=CARTESIAN_POINT('Ctrl Pts',(0.594902323120467,6.98868830169284,
72.2464428657961));
#143029=CARTESIAN_POINT('Ctrl Pts',(0.400198881060796,7.00253473439962,
72.2552994990765));
#143030=CARTESIAN_POINT('Ctrl Pts',(0.205281742183532,7.00824414306652,
72.2641561323568));
#143031=CARTESIAN_POINT('Ctrl Pts',(0.0129725818632786,7.01387716021924,
72.2728942644637));
#143032=CARTESIAN_POINT('Ctrl Pts',(-0.179544313973932,7.01158956178464,
72.2816323965706));
#143033=CARTESIAN_POINT('Ctrl Pts',(-0.371622006413891,7.0013944073198,
72.2903705286775));
#143034=CARTESIAN_POINT('Ctrl Pts',(-0.567606958151783,6.99099186223312,
72.2992864125446));
#143035=CARTESIAN_POINT('Ctrl Pts',(-0.763134350480073,6.97235661479577,
72.3082022964117));
#143036=CARTESIAN_POINT('Ctrl Pts',(-0.957520795727762,6.9455583280431,
72.3171181802788));
#143037=CARTESIAN_POINT('Ctrl Pts',(-1.15190724097545,6.91876004129044,
72.3260340641458));
#143038=CARTESIAN_POINT('Ctrl Pts',(-1.34515244039453,6.88379876254866,
72.3349499480129));
#143039=CARTESIAN_POINT('Ctrl Pts',(-1.53658136398455,6.84079997327472,
72.34386583188));
#143040=CARTESIAN_POINT('Ctrl Pts',(-1.72424866085302,6.79864612107556,
72.3526065163761));
#143041=CARTESIAN_POINT('Ctrl Pts',(-1.91019033201575,6.74876322731733,
72.3613472008722));
#143042=CARTESIAN_POINT('Ctrl Pts',(-2.0937807640309,6.69131591502555,72.3700878853683));
#143043=CARTESIAN_POINT('Ctrl Pts',(-2.27733816507752,6.63387893845956,
72.3788269972701));
#143044=CARTESIAN_POINT('Ctrl Pts',(-2.45854491058638,6.56888034304456,
72.3875661091718));
#143045=CARTESIAN_POINT('Ctrl Pts',(-2.63679070771567,6.49653456284228,
72.3963052210736));
#143046=CARTESIAN_POINT('Ctrl Pts',(-2.81734593569057,6.42325143893238,
72.405157560748));
#143047=CARTESIAN_POINT('Ctrl Pts',(-2.9948626811838,6.34242950270267,72.4140099004224));
#143048=CARTESIAN_POINT('Ctrl Pts',(-3.16872638395628,6.25434246472956,
72.4228622400968));
#143049=CARTESIAN_POINT('Ctrl Pts',(-3.34027827087986,6.16742669486601,
72.4315968727465));
#143050=CARTESIAN_POINT('Ctrl Pts',(-3.50827341436658,6.07343796675173,
72.4403315053962));
#143051=CARTESIAN_POINT('Ctrl Pts',(-3.67214425031528,5.97268642801348,
72.4490661380458));
#143052=CARTESIAN_POINT('Ctrl Pts',(-3.83932754644016,5.86989831298131,
72.4579773312326));
#143053=CARTESIAN_POINT('Ctrl Pts',(-4.00221776424444,5.76007120420412,
72.4668885244193));
#143054=CARTESIAN_POINT('Ctrl Pts',(-4.16024047493172,5.64358270544872,
72.4757997176061));
#143055=CARTESIAN_POINT('Ctrl Pts',(-4.318263185619,5.52709420669332,72.4847109107928));
#143056=CARTESIAN_POINT('Ctrl Pts',(-4.47141813719525,5.40394448698109,
72.4936221039796));
#143057=CARTESIAN_POINT('Ctrl Pts',(-4.61916328400746,5.27455752818921,
72.5025332971663));
#143058=CARTESIAN_POINT('Ctrl Pts',(-4.75222661313086,5.15802808642092,
72.5105589620188));
#143059=CARTESIAN_POINT('Ctrl Pts',(-4.88096269756898,5.03638549043432,
72.5185846268712));
#143060=CARTESIAN_POINT('Ctrl Pts',(-5.00495595374574,4.90999414088907,
72.5266102917237));
#143061=CARTESIAN_POINT('Ctrl Pts',(-5.12890985750446,4.78364290485789,
72.534633409427));
#143062=CARTESIAN_POINT('Ctrl Pts',(-5.24812367342293,4.65254617720194,
72.5426565271303));
#143063=CARTESIAN_POINT('Ctrl Pts',(-5.36221771831549,4.51710612050275,
72.5506796448336));
#143064=CARTESIAN_POINT('Ctrl Pts',(-5.47629737495057,4.38168314397993,
72.5587017507515));
#143065=CARTESIAN_POINT('Ctrl Pts',(-5.58525831096701,4.24191821008803,
72.5667238566694));
#143066=CARTESIAN_POINT('Ctrl Pts',(-5.68876032072863,4.09824750055478,
72.5747459625874));
#143067=CARTESIAN_POINT('Ctrl Pts',(-5.79230079218675,3.95452340250049,
72.582771049547));
#143068=CARTESIAN_POINT('Ctrl Pts',(-5.89037806807313,3.80689092531865,
72.5907961365066));
#143069=CARTESIAN_POINT('Ctrl Pts',(-5.98269432985107,3.65581661439244,
72.5988212234662));
#143070=CARTESIAN_POINT('Ctrl Pts',(-6.07502877285522,3.50471255013602,
72.6068478909265));
#143071=CARTESIAN_POINT('Ctrl Pts',(-6.16159975781812,3.35016561912344,
72.6148745583869));
#143072=CARTESIAN_POINT('Ctrl Pts',(-6.24215496203757,3.19266784874496,
72.6229012258472));
#143073=CARTESIAN_POINT('Ctrl Pts',(-6.3227748356905,3.0350436397126,72.6309343370879));
#143074=CARTESIAN_POINT('Ctrl Pts',(-6.39736912436822,2.87446419050912,
72.6389674483285));
#143075=CARTESIAN_POINT('Ctrl Pts',(-6.46573301858888,2.71144299125568,
72.6470005595691));
#143076=CARTESIAN_POINT('Ctrl Pts',(-6.50601550851415,2.61538497859571,
72.6517339605304));
#143077=CARTESIAN_POINT('Ctrl Pts',(-6.54413573015642,2.51847954998675,
72.6564673614917));
#143078=CARTESIAN_POINT('Ctrl Pts',(-6.5800598628589,2.42083431149125,72.6612007624529));
#143079=CARTESIAN_POINT('Ctrl Pts',(-6.65406469426367,2.21968208125696,
72.6709517157469));
#143080=CARTESIAN_POINT('Ctrl Pts',(-6.71879150752435,2.01527117142247,
72.680702669041));
#143081=CARTESIAN_POINT('Ctrl Pts',(-6.77402074923543,1.80838863395782,
72.690453622335));
#143082=CARTESIAN_POINT('Ctrl Pts',(-6.82932955902953,1.60120804338932,
72.7002186237063));
#143083=CARTESIAN_POINT('Ctrl Pts',(-6.87511341721585,1.39154873978261,
72.7099836250777));
#143084=CARTESIAN_POINT('Ctrl Pts',(-6.91120301163148,1.18021163124076,
72.7197486264491));
#143085=CARTESIAN_POINT('Ctrl Pts',(-6.94723245217097,0.969226777869918,
72.7294973515865));
#143086=CARTESIAN_POINT('Ctrl Pts',(-6.97359991649599,0.756569746106266,
72.7392460767239));
#143087=CARTESIAN_POINT('Ctrl Pts',(-6.99018785445205,0.543047255744024,
72.7489948018613));
#143088=CARTESIAN_POINT('Ctrl Pts',(-7.00673026495013,0.330110801827794,
72.7587167705281));
#143089=CARTESIAN_POINT('Ctrl Pts',(-7.01354672967137,0.11631367112125,
72.7684387391949));
#143090=CARTESIAN_POINT('Ctrl Pts',(-7.01057155428257,-0.0975348388223232,
72.7781607078618));
#143091=CARTESIAN_POINT('Ctrl Pts',(-7.00761606485217,-0.309968369034859,
72.7878183488014));
#143092=CARTESIAN_POINT('Ctrl Pts',(-6.99499805624747,-0.522452553737243,
72.797475989741));
#143093=CARTESIAN_POINT('Ctrl Pts',(-6.97270378508319,-0.734185595055159,
72.8071336306806));
#143094=CARTESIAN_POINT('Ctrl Pts',(-6.96290468535936,-0.827249556259204,
72.8113784963668));
#143095=CARTESIAN_POINT('Ctrl Pts',(-6.95123688691363,-0.920168297538873,
72.815623362053));
#143096=CARTESIAN_POINT('Ctrl Pts',(-6.93770238185834,-1.0128732513287,
72.8198682277392));
#143097=CARTESIAN_POINT('Ctrl Pts',(-6.91266722857916,-1.18435220223127,
72.8277200747532));
#143098=CARTESIAN_POINT('Ctrl Pts',(-6.88125167260411,-1.35502869998371,
72.8355719217671));
#143099=CARTESIAN_POINT('Ctrl Pts',(-6.84353050352245,-1.5243742355005,
72.8434237687811));
#143100=CARTESIAN_POINT('Ctrl Pts',(-6.80582003185933,-1.69367174599276,
72.8512733890747));
#143101=CARTESIAN_POINT('Ctrl Pts',(-6.7618075870222,-1.86163867309074,
72.8591230093683));
#143102=CARTESIAN_POINT('Ctrl Pts',(-6.71161920016452,-2.027755970151,72.866972629662));
#143103=CARTESIAN_POINT('Ctrl Pts',(-6.66143482020766,-2.1938600048696,
72.8748216232638));
#143104=CARTESIAN_POINT('Ctrl Pts',(-6.60507559083961,-2.35811433857433,
72.8826706168656));
#143105=CARTESIAN_POINT('Ctrl Pts',(-6.54271754008799,-2.52001463351406,
72.8905196104675));
#143106=CARTESIAN_POINT('Ctrl Pts',(-6.48032791928116,-2.68199689383255,
72.8983725777849));
#143107=CARTESIAN_POINT('Ctrl Pts',(-6.41193354624365,-2.84162237771152,
72.9062255451024));
#143108=CARTESIAN_POINT('Ctrl Pts',(-6.33775891676812,-2.99840598909256,
72.9140785124199));
#143109=CARTESIAN_POINT('Ctrl Pts',(-6.26356544942902,-3.15522941824288,
72.9219334741272));
#143110=CARTESIAN_POINT('Ctrl Pts',(-6.1835889769201,-3.30920919845494,
72.9297884358345));
#143111=CARTESIAN_POINT('Ctrl Pts',(-6.09809987938691,-3.45988503039066,
72.9376433975418));
#143112=CARTESIAN_POINT('Ctrl Pts',(-6.01252592677857,-3.61071042068424,
72.9455061559552));
#143113=CARTESIAN_POINT('Ctrl Pts',(-5.92142862103154,-3.75822498839262,
72.9533689143686));
#143114=CARTESIAN_POINT('Ctrl Pts',(-5.82512188612499,-3.90199712638127,
72.9612316727819));
#143115=CARTESIAN_POINT('Ctrl Pts',(-5.75447264732019,-4.00746630379749,
72.9669996795299));
#143116=CARTESIAN_POINT('Ctrl Pts',(-5.681020872031,-4.11092210946462,72.9727676862778));
#143117=CARTESIAN_POINT('Ctrl Pts',(-5.60490397254818,-4.21220583792075,
72.9785356930257));
#143118=CARTESIAN_POINT('Ctrl Pts',(-5.49434369253786,-4.35932109688012,
72.9869137594667));
#143119=CARTESIAN_POINT('Ctrl Pts',(-5.3779144051963,-4.50217851939186,
72.9952918259078));
#143120=CARTESIAN_POINT('Ctrl Pts',(-5.25597076081091,-4.64030149063623,
73.0036698923488));
#143121=CARTESIAN_POINT('Ctrl Pts',(-5.13411050004045,-4.77833001503422,
73.0120422299675));
#143122=CARTESIAN_POINT('Ctrl Pts',(-5.0067436166585,-4.91163029686378,
73.0204145675863));
#143123=CARTESIAN_POINT('Ctrl Pts',(-4.87426540130468,-5.03975826405832,
73.0287869052051));
#143124=CARTESIAN_POINT('Ctrl Pts',(-4.74185834496281,-5.16781740892216,
73.0371547457277));
#143125=CARTESIAN_POINT('Ctrl Pts',(-4.60434566665396,-5.29070955068605,
73.0455225862503));
#143126=CARTESIAN_POINT('Ctrl Pts',(-4.46216023742459,-5.40802668059681,
73.0538904267729));
#143127=CARTESIAN_POINT('Ctrl Pts',(-4.32003035218113,-5.52529798119126,
73.0622549984428));
#143128=CARTESIAN_POINT('Ctrl Pts',(-4.17323160927016,-5.63699840398013,
73.0706195701128));
#143129=CARTESIAN_POINT('Ctrl Pts',(-4.02223109316965,-5.7427592319058,
73.0789841417828));
#143130=CARTESIAN_POINT('Ctrl Pts',(-3.87126746179388,-5.84849422575403,
73.0873466702483));
#143131=CARTESIAN_POINT('Ctrl Pts',(-3.71610437327186,-5.94829233005877,
73.0957091987138));
#143132=CARTESIAN_POINT('Ctrl Pts',(-3.55723947947013,-6.0418270289871,
73.1040717271793));
#143133=CARTESIAN_POINT('Ctrl Pts',(-3.39836190775218,-6.13536919227743,
73.1124349230008));
#143134=CARTESIAN_POINT('Ctrl Pts',(-3.23578222071624,-6.22264677962249,
73.1207981188223));
#143135=CARTESIAN_POINT('Ctrl Pts',(-3.07002502461947,-6.30337789686691,
73.1291613146439));
#143136=CARTESIAN_POINT('Ctrl Pts',(-2.90425652421417,-6.3841145198117,
73.1375250808185));
#143137=CARTESIAN_POINT('Ctrl Pts',(-2.73531037817286,-6.45830363823736,
73.1458888469932));
#143138=CARTESIAN_POINT('Ctrl Pts',(-2.56373380198725,-6.5257103486937,
73.1542526131679));
#143139=CARTESIAN_POINT('Ctrl Pts',(-2.39212264942908,-6.59313064305283,
73.1626180648215));
#143140=CARTESIAN_POINT('Ctrl Pts',(-2.21788031573932,-6.65376568379617,
73.1709835164751));
#143141=CARTESIAN_POINT('Ctrl Pts',(-2.04157230816635,-6.70742939381611,
73.1793489681286));
#143142=CARTESIAN_POINT('Ctrl Pts',(-1.86520525538916,-6.76111107570676,
73.1877172213555));
#143143=CARTESIAN_POINT('Ctrl Pts',(-1.68677146369094,-6.80781667574779,
73.1960854745823));
#143144=CARTESIAN_POINT('Ctrl Pts',(-1.50685026482488,-6.84741037487145,
73.2044537278092));
#143145=CARTESIAN_POINT('Ctrl Pts',(-1.32676225333829,-6.887040783003,73.2128297396006));
#143146=CARTESIAN_POINT('Ctrl Pts',(-1.14518440038569,-6.91954604320939,
73.2212057513921));
#143147=CARTESIAN_POINT('Ctrl Pts',(-0.962706094649794,-6.94484150559422,
73.2295817631836));
#143148=CARTESIAN_POINT('Ctrl Pts',(-0.780138299297698,-6.97014937318639,
73.2379618826748));
#143149=CARTESIAN_POINT('Ctrl Pts',(-0.596669496899309,-6.98824035330358,
73.2463420021659));
#143150=CARTESIAN_POINT('Ctrl Pts',(-0.41289347728538,-6.9990817639827,
73.2547221216571));
#143151=CARTESIAN_POINT('Ctrl Pts',(-0.228907470289866,-7.00993556234682,
73.2631118164963));
#143152=CARTESIAN_POINT('Ctrl Pts',(-0.0446138732872293,-7.01352322616916,
73.2715015113355));
#143153=CARTESIAN_POINT('Ctrl Pts',(0.139392894994874,-7.00986420576925,
73.2798912061747));
#143154=CARTESIAN_POINT('Ctrl Pts',(0.25621561681979,-7.00754115686012,
73.2852176786493));
#143155=CARTESIAN_POINT('Ctrl Pts',(0.372922769238492,-7.00229819252731,
73.2905441511239));
#143156=CARTESIAN_POINT('Ctrl Pts',(0.489363448128481,-6.99415112634377,
73.2958706235985));
#143157=CARTESIAN_POINT('Ctrl Pts',(0.672584954252464,-6.98133157091975,
73.3042519240034));
#143158=CARTESIAN_POINT('Ctrl Pts',(0.855515982900771,-6.96129316380664,
73.3126332244083));
#143159=CARTESIAN_POINT('Ctrl Pts',(1.0375640702819,-6.93405273722086,73.3210145248132));
#143160=CARTESIAN_POINT('Ctrl Pts',(1.21938143836258,-6.90684683388801,
73.3293852031467));
#143161=CARTESIAN_POINT('Ctrl Pts',(1.40031777380758,-6.8724571493474,73.3377558814803));
#143162=CARTESIAN_POINT('Ctrl Pts',(1.57978345622159,-6.83095240753063,
73.3461265598139));
#143163=CARTESIAN_POINT('Ctrl Pts',(1.75904547590016,-6.7894947664695,73.3544877388648));
#143164=CARTESIAN_POINT('Ctrl Pts',(1.93683985164169,-6.74093823461438,
73.3628489179157));
#143165=CARTESIAN_POINT('Ctrl Pts',(2.11258446832033,-6.68540301154027,
73.3712100969666));
#143166=CARTESIAN_POINT('Ctrl Pts',(2.28810103562714,-6.62993985196931,
73.3795604264014));
#143167=CARTESIAN_POINT('Ctrl Pts',(2.46157283818407,-6.56751616194294,
73.3879107558361));
#143168=CARTESIAN_POINT('Ctrl Pts',(2.63243037418638,-6.49830261588063,
73.3962610852709));
#143169=CARTESIAN_POINT('Ctrl Pts',(2.80315644553242,-6.42914232550287,
73.4046049896265));
#143170=CARTESIAN_POINT('Ctrl Pts',(2.97127195653029,-6.35320271284023,
73.4129488939821));
#143171=CARTESIAN_POINT('Ctrl Pts',(3.13622383738162,-6.27070383643968,
73.4212927983377));
#143172=CARTESIAN_POINT('Ctrl Pts',(3.30104322785578,-6.18827122365004,
73.4296300008175));
#143173=CARTESIAN_POINT('Ctrl Pts',(3.46270376374544,-6.09929000041611,
73.4379672032972));
#143174=CARTESIAN_POINT('Ctrl Pts',(3.62067345368134,-6.00402784006764,
73.4463044057769));
#143175=CARTESIAN_POINT('Ctrl Pts',(3.6726762036358,-5.97266806271583,73.449048966813));
#143176=CARTESIAN_POINT('Ctrl Pts',(3.72427915896821,-5.94062800628213,
73.451793527849));
#143177=CARTESIAN_POINT('Ctrl Pts',(3.77546389517341,-5.90791832532763,
73.454538088885));
#143178=CARTESIAN_POINT('Ctrl Pts',(3.93096935035945,-5.8085423354734,73.4628763991868));
#143179=CARTESIAN_POINT('Ctrl Pts',(4.08248496435823,-5.70306382850212,
73.4712147094886));
#143180=CARTESIAN_POINT('Ctrl Pts',(4.22953330314882,-5.59184000129251,
73.4795530197905));
#143181=CARTESIAN_POINT('Ctrl Pts',(4.3766741597659,-5.48054619582384,73.4878965762743));
#143182=CARTESIAN_POINT('Ctrl Pts',(4.51934187364946,-5.36350005768225,
73.496240132758));
#143183=CARTESIAN_POINT('Ctrl Pts',(4.6570924182614,-5.24109881325207,73.5045836892418));
#143184=CARTESIAN_POINT('Ctrl Pts',(4.79494776288413,-5.11860444649141,
73.5129335934668));
#143185=CARTESIAN_POINT('Ctrl Pts',(4.92787823158848,-4.99074706424958,
73.5212834976919));
#143186=CARTESIAN_POINT('Ctrl Pts',(5.05547663844316,-4.85796073683758,
73.5296334019169));
#143187=CARTESIAN_POINT('Ctrl Pts',(5.18326643346779,-4.72497523975861,
73.5379958303805));
#143188=CARTESIAN_POINT('Ctrl Pts',(5.30570795750625,-4.58704626032255,
73.546358258844));
#143189=CARTESIAN_POINT('Ctrl Pts',(5.42243333521388,-4.44464208768955,
73.5547206873076));
#143190=CARTESIAN_POINT('Ctrl Pts',(5.53925852903079,-4.30211614007721,
73.5630902667875));
#143191=CARTESIAN_POINT('Ctrl Pts',(5.65035762644575,-4.15510762439005,
73.5714598462673));
#143192=CARTESIAN_POINT('Ctrl Pts',(5.75540577794039,-4.00411424584144,
73.5798294257471));
#143193=CARTESIAN_POINT('Ctrl Pts',(5.86061595341033,-3.85288797840247,
73.5882119142836));
#143194=CARTESIAN_POINT('Ctrl Pts',(5.95975635712508,-3.69766484182881,
73.5965944028201));
#143195=CARTESIAN_POINT('Ctrl Pts',(6.0525471007111,-3.53896879841764,73.6049768913566));
#143196=CARTESIAN_POINT('Ctrl Pts',(6.08290975248512,-3.48704085261408,
73.6077197789615));
#143197=CARTESIAN_POINT('Ctrl Pts',(6.11259292135486,-3.43474123220562,
73.6104626665664));
#143198=CARTESIAN_POINT('Ctrl Pts',(6.14158791671023,-3.38208876640145,
73.6132055541713));
#143199=CARTESIAN_POINT('Ctrl Pts',(6.23397316448646,-3.21432494924165,
73.6219450744885));
#143200=CARTESIAN_POINT('Ctrl Pts',(6.31953798906509,-3.04266953665,73.6306845948056));
#143201=CARTESIAN_POINT('Ctrl Pts',(6.39796990775004,-2.86768331968942,
73.6394241151227));
#143202=CARTESIAN_POINT('Ctrl Pts',(6.47630853837843,-2.69290523386191,
73.6481532405281));
#143203=CARTESIAN_POINT('Ctrl Pts',(6.54753107721928,-2.51480449984745,
73.6568823659336));
#143204=CARTESIAN_POINT('Ctrl Pts',(6.61137137601919,-2.33396552906296,
73.665611491339));
#143205=CARTESIAN_POINT('Ctrl Pts',(6.67714570110341,-2.1476480857572,73.67460506347));
#143206=CARTESIAN_POINT('Ctrl Pts',(6.73508331753212,-1.95842413667652,
73.6835986356009));
#143207=CARTESIAN_POINT('Ctrl Pts',(6.78494573670534,-1.76695724692594,
73.6925922077319));
#143208=CARTESIAN_POINT('Ctrl Pts',(6.83320011183776,-1.5816650914979,73.7012957405845));
#143209=CARTESIAN_POINT('Ctrl Pts',(6.87389189068418,-1.39427269803777,
73.7099992734372));
#143210=CARTESIAN_POINT('Ctrl Pts',(6.90685442182102,-1.20539975040292,
73.7187028062899));
#143211=CARTESIAN_POINT('Ctrl Pts',(6.9414646336589,-1.00708571010822,73.72784139806));
#143212=CARTESIAN_POINT('Ctrl Pts',(6.96755298493941,-0.807139581817272,
73.73697998983));
#143213=CARTESIAN_POINT('Ctrl Pts',(6.98498622485248,-0.606295308509952,
73.7461185816001));
#143214=CARTESIAN_POINT('Ctrl Pts',(7.0015461796038,-0.415511948984274,
73.7547993929099));
#143215=CARTESIAN_POINT('Ctrl Pts',(7.01029680999461,-0.223918551223194,
73.7634802042197));
#143216=CARTESIAN_POINT('Ctrl Pts',(7.01117626839302,-0.0321542535674641,
73.7721610155295));
#143217=CARTESIAN_POINT('Ctrl Pts',(7.01122264641647,-0.0220416102536277,
73.7726187959898));
#143218=CARTESIAN_POINT('Ctrl Pts',(7.01124714700305,-0.0119284933641162,
73.7730765764501));
#143219=CARTESIAN_POINT('Ctrl Pts',(7.0112497650765,-0.00181499715760335,
73.7735343569104));
#143220=CARTESIAN_POINT('Ctrl Pts',(7.01124976619934,-0.00181065449666946,
73.773534553478));
#143221=CARTESIAN_POINT('Ctrl Pts',(7.01130032134908,0.193949929554239,
73.7823955219703));
#143222=CARTESIAN_POINT('Ctrl Pts',(7.00314781087931,0.38956846135378,73.7912564904627));
#143223=CARTESIAN_POINT('Ctrl Pts',(6.98685399846189,0.584378102496293,
73.8001174589551));
#143224=CARTESIAN_POINT('Ctrl Pts',(6.97052503348697,0.7796080293851,73.8089975442567));
#143225=CARTESIAN_POINT('Ctrl Pts',(6.94601965073969,0.974025329710912,
73.8178776295584));
#143226=CARTESIAN_POINT('Ctrl Pts',(6.91345145316409,1.16696853738365,73.82675771486));
#143227=CARTESIAN_POINT('Ctrl Pts',(6.88084931454048,1.36011282141808,73.8356470545701));
#143228=CARTESIAN_POINT('Ctrl Pts',(6.840167620754,1.55177970339379,73.8445363942802));
#143229=CARTESIAN_POINT('Ctrl Pts',(6.79157087268327,1.74131893799506,73.8534257339902));
#143230=CARTESIAN_POINT('Ctrl Pts',(6.7429094431003,1.93111044635558,73.8623269052725));
#143231=CARTESIAN_POINT('Ctrl Pts',(6.6863119604482,2.11876840904201,73.8712280765548));
#143232=CARTESIAN_POINT('Ctrl Pts',(6.62199304558498,2.30365680315539,73.8801292478371));
#143233=CARTESIAN_POINT('Ctrl Pts',(6.60553559337101,2.35096468945151,73.8824068142628));
#143234=CARTESIAN_POINT('Ctrl Pts',(6.58857286076634,2.39809134540819,73.8846843806884));
#143235=CARTESIAN_POINT('Ctrl Pts',(6.57110895151812,2.44502632087642,73.8869619471141));
#143236=CARTESIAN_POINT('',(7.01125,-1.99357674465772E-12,73.2264656430894));
#143237=CARTESIAN_POINT('Ctrl Pts',(6.57110895151812,2.44502632087643,73.339830038482));
#143238=CARTESIAN_POINT('Ctrl Pts',(6.64576037121474,2.24439755544203,73.330080824681));
#143239=CARTESIAN_POINT('Ctrl Pts',(6.71123467403681,2.04030721866428,73.3203316108801));
#143240=CARTESIAN_POINT('Ctrl Pts',(6.76726039322619,1.83352483832973,73.3105823970792));
#143241=CARTESIAN_POINT('Ctrl Pts',(6.77916262307297,1.78959552417517,73.3085112521628));
#143242=CARTESIAN_POINT('Ctrl Pts',(6.79063859508601,1.74554478499926,73.3064401072465));
#143243=CARTESIAN_POINT('Ctrl Pts',(6.80168598724614,1.70138011431884,73.3043689623301));
#143244=CARTESIAN_POINT('Ctrl Pts',(6.8449702867887,1.52834046774678,73.2962541008627));
#143245=CARTESIAN_POINT('Ctrl Pts',(6.88169100112489,1.35347215331281,73.2881392393953));
#143246=CARTESIAN_POINT('Ctrl Pts',(6.9116968681817,1.1773160004295,73.2800243779279));
#143247=CARTESIAN_POINT('Ctrl Pts',(6.94168248721581,1.00127871809161,73.2719149923863));
#143248=CARTESIAN_POINT('Ctrl Pts',(6.96496221977511,0.823955678815036,
73.2638056068446));
#143249=CARTESIAN_POINT('Ctrl Pts',(6.98143534720025,0.645900189938756,
73.2556962213029));
#143250=CARTESIAN_POINT('Ctrl Pts',(6.99789894399179,0.46794771620836,73.2475915274983));
#143251=CARTESIAN_POINT('Ctrl Pts',(7.00756374903666,0.289263992916175,
73.2394868336937));
#143252=CARTESIAN_POINT('Ctrl Pts',(7.01038060736404,0.11040970244574,73.2313821398891));
#143253=CARTESIAN_POINT('Ctrl Pts',(7.01095019807634,0.0742439706740013,
73.2297433076226));
#143254=CARTESIAN_POINT('Ctrl Pts',(7.01123995951458,0.0380712819471819,
73.228104475356));
#143255=CARTESIAN_POINT('Ctrl Pts',(7.01124974356013,0.00189629324868483,
73.2264656430895));
#143256=CARTESIAN_POINT('Ctrl Pts',(7.01125,-8.58630487052188E-16,73.2264656430895));
#143257=CARTESIAN_POINT('Ctrl Pts',(7.01125,-0.191009525814159,73.2177938341507));
#143258=CARTESIAN_POINT('Ctrl Pts',(7.00344006572044,-0.38201890962812,
73.209122025212));
#143259=CARTESIAN_POINT('Ctrl Pts',(6.98784625534325,-0.572390840410128,
73.2004502162732));
#143260=CARTESIAN_POINT('Ctrl Pts',(6.97225246786088,-0.762762491688126,
73.1917784200664));
#143261=CARTESIAN_POINT('Ctrl Pts',(6.94887485033549,-0.952496408756088,
73.1831066238596));
#143262=CARTESIAN_POINT('Ctrl Pts',(6.91779140296553,-1.140959538089,73.1744348276527));
#143263=CARTESIAN_POINT('Ctrl Pts',(6.88670800059844,-1.32942239456338,
73.165763044001));
#143264=CARTESIAN_POINT('Ctrl Pts',(6.84791883692786,-1.51661418677323,
73.1570912603493));
#143265=CARTESIAN_POINT('Ctrl Pts',(6.80155333291415,-1.70191034488437,
73.1484194766976));
#143266=CARTESIAN_POINT('Ctrl Pts',(6.75518789508331,-1.88720623850081,
73.1397477054241));
#143267=CARTESIAN_POINT('Ctrl Pts',(6.7012462074874,-2.07060622793232,73.1310759341506));
#143268=CARTESIAN_POINT('Ctrl Pts',(6.63990824732733,-2.25149839652942,
73.1224041628772));
#143269=CARTESIAN_POINT('Ctrl Pts',(6.57857037347141,-2.43239031060637,
73.1137324038051));
#143270=CARTESIAN_POINT('Ctrl Pts',(6.50983633907402,-2.61077414195845,
73.105060644733));
#143271=CARTESIAN_POINT('Ctrl Pts',(6.43393547556492,-2.78605471209149,
73.096388885661));
#143272=CARTESIAN_POINT('Ctrl Pts',(6.35803471730284,-2.96133503917383,
73.0877171386135));
#143273=CARTESIAN_POINT('Ctrl Pts',(6.27496726266488,-3.13351185304139,
73.0790453915661));
#143274=CARTESIAN_POINT('Ctrl Pts',(6.18501026583716,-3.30201068653465,
73.0703736445186));
#143275=CARTESIAN_POINT('Ctrl Pts',(6.09151188669153,-3.47714289831489,
73.0613605124456));
#143276=CARTESIAN_POINT('Ctrl Pts',(5.99057066119507,-3.64830137930445,
73.0523473803726));
#143277=CARTESIAN_POINT('Ctrl Pts',(5.88255038916944,-3.81486926137482,
73.0433342482996));
#143278=CARTESIAN_POINT('Ctrl Pts',(5.7762179338942,-3.97883452028786,73.0344619464152));
#143279=CARTESIAN_POINT('Ctrl Pts',(5.66302622906759,-4.13835132493216,
73.0255896445308));
#143280=CARTESIAN_POINT('Ctrl Pts',(5.54337059053299,-4.29286257158483,
73.0167173426465));
#143281=CARTESIAN_POINT('Ctrl Pts',(5.4255845713505,-4.44495958000855,73.007983670479));
#143282=CARTESIAN_POINT('Ctrl Pts',(5.30153533575357,-4.59220608123619,
72.9992499983116));
#143283=CARTESIAN_POINT('Ctrl Pts',(5.17164269972743,-4.73410375349506,
72.9905163261442));
#143284=CARTESIAN_POINT('Ctrl Pts',(5.04265587432023,-4.8750118976154,72.9818435585302));
#143285=CARTESIAN_POINT('Ctrl Pts',(4.90790710164581,-5.01064538261517,
72.9731707909162));
#143286=CARTESIAN_POINT('Ctrl Pts',(4.76784607609706,-5.14055156156865,
72.9644980233022));
#143287=CARTESIAN_POINT('Ctrl Pts',(4.62778576967854,-5.27045707353101,
72.9558253002178));
#143288=CARTESIAN_POINT('Ctrl Pts',(4.48241347330293,-5.39463514506075,
72.9471525771333));
#143289=CARTESIAN_POINT('Ctrl Pts',(4.33221433006009,-5.5126713634065,72.9384798540488));
#143290=CARTESIAN_POINT('Ctrl Pts',(4.18201594574026,-5.63070698534137,
72.9298071747857));
#143291=CARTESIAN_POINT('Ctrl Pts',(4.0269909867703,-5.74260064062169,72.9211344955226));
#143292=CARTESIAN_POINT('Ctrl Pts',(3.86765680432516,-5.84797891638276,
72.9124618162595));
#143293=CARTESIAN_POINT('Ctrl Pts',(3.70832341395466,-5.95335666829228,
72.9037891801095));
#143294=CARTESIAN_POINT('Ctrl Pts',(3.54468107997153,-6.0522189487556,72.8951165439596));
#143295=CARTESIAN_POINT('Ctrl Pts',(3.37727590613509,-6.14423583664718,
72.8864439078097));
#143296=CARTESIAN_POINT('Ctrl Pts',(3.20987155083152,-6.23625227461928,
72.877771314065));
#143297=CARTESIAN_POINT('Ctrl Pts',(3.03870464148727,-6.32142325013406,
72.8690987203202));
#143298=CARTESIAN_POINT('Ctrl Pts',(2.86434638713613,-6.39946453517794,
72.8604261265754));
#143299=CARTESIAN_POINT('Ctrl Pts',(2.68998897108409,-6.47750544500621,
72.8517535745277));
#143300=CARTESIAN_POINT('Ctrl Pts',(2.51244050006166,-6.5484166168845,72.84308102248));
#143301=CARTESIAN_POINT('Ctrl Pts',(2.33229347361646,-6.6119614121247,72.8344084704323));
#143302=CARTESIAN_POINT('Ctrl Pts',(2.15214729859961,-6.67550590703332,
72.8257359593736));
#143303=CARTESIAN_POINT('Ctrl Pts',(1.96940286067366,-6.73168400046206,
72.8170634483149));
#143304=CARTESIAN_POINT('Ctrl Pts',(1.78466999316304,-6.7803082214604,72.8083909372563));
#143305=CARTESIAN_POINT('Ctrl Pts',(1.59993798367808,-6.82893221661463,
72.7997184664787));
#143306=CARTESIAN_POINT('Ctrl Pts',(1.41321783784243,-6.87000233722938,
72.7910459957011));
#143307=CARTESIAN_POINT('Ctrl Pts',(1.22513265046473,-6.90338153018253,
72.7823735249235));
#143308=CARTESIAN_POINT('Ctrl Pts',(1.03704832133351,-6.93676057082398,
72.773701093719));
#143309=CARTESIAN_POINT('Ctrl Pts',(0.847599242857963,-6.96244870438738,
72.7650286625146));
#143310=CARTESIAN_POINT('Ctrl Pts',(0.657417610672671,-6.98036020902055,
72.7563562313101));
#143311=CARTESIAN_POINT('Ctrl Pts',(0.467236830779674,-6.99827163338395,
72.7476838389708));
#143312=CARTESIAN_POINT('Ctrl Pts',(0.276323786592565,-7.00840647191832,
72.7390114466316));
#143313=CARTESIAN_POINT('Ctrl Pts',(0.0853155533264802,-7.01073090475313,
72.7303390542923));
#143314=CARTESIAN_POINT('Ctrl Pts',(-0.105691839529951,-7.01305532736075,
72.7216667001103));
#143315=CARTESIAN_POINT('Ctrl Pts',(-0.296794136556739,-7.00756940957932,
72.7129943459284));
#143316=CARTESIAN_POINT('Ctrl Pts',(-0.48735363660962,-6.99429145770917,
72.7043219917464));
#143317=CARTESIAN_POINT('Ctrl Pts',(-0.677912313777361,-6.98101356317664,
72.6956496750139));
#143318=CARTESIAN_POINT('Ctrl Pts',(-0.867927915263419,-6.95994372163552,
72.6869773582814));
#143319=CARTESIAN_POINT('Ctrl Pts',(-1.0567663716562,-6.93115224174427,
72.678305041549));
#143320=CARTESIAN_POINT('Ctrl Pts',(-1.2456040280048,-6.90236088383271,
72.6696327615581));
#143321=CARTESIAN_POINT('Ctrl Pts',(-1.43326426840602,-6.86584799585282,
72.6609604815673));
#143322=CARTESIAN_POINT('Ctrl Pts',(-1.61912088843213,-6.82173541784953,
72.6522882015764));
#143323=CARTESIAN_POINT('Ctrl Pts',(-1.80497673621251,-6.77762302313673,
72.6436159576195));
#143324=CARTESIAN_POINT('Ctrl Pts',(-1.98902870221951,-6.72591106719145,
72.6349437136625));
#143325=CARTESIAN_POINT('Ctrl Pts',(-2.17066262759359,-6.66677210647466,
72.6262714697055));
#143326=CARTESIAN_POINT('Ctrl Pts',(-2.35229581308771,-6.60763338665851,
72.6175992610746));
#143327=CARTESIAN_POINT('Ctrl Pts',(-2.53151070754872,-6.54106781055818,
72.6089270524437));
#143328=CARTESIAN_POINT('Ctrl Pts',(-2.70770929769928,-6.46729749753735,
72.6002548438129));
#143329=CARTESIAN_POINT('Ctrl Pts',(-2.88390718448732,-6.39352747899829,
72.5915826698004));
#143330=CARTESIAN_POINT('Ctrl Pts',(-3.05708852903611,-6.31255289079463,
72.5829104957879));
#143331=CARTESIAN_POINT('Ctrl Pts',(-3.22667545573025,-6.22464393085163,
72.5742383217753));
#143332=CARTESIAN_POINT('Ctrl Pts',(-3.39626171929099,-6.1367353146578,
72.5655661816735));
#143333=CARTESIAN_POINT('Ctrl Pts',(-3.56225334093561,-6.04189251171209,
72.5568940415717));
#143334=CARTESIAN_POINT('Ctrl Pts',(-3.72409644021389,-5.94043199325489,
72.5482219014698));
#143335=CARTESIAN_POINT('Ctrl Pts',(-3.88593891984383,-5.83897186325936,
72.539549794571));
#143336=CARTESIAN_POINT('Ctrl Pts',(-4.04363266822376,-5.73089421933132,
72.5308776876722));
#143337=CARTESIAN_POINT('Ctrl Pts',(-4.19665149725252,-5.61655969193849,
72.5222055807734));
#143338=CARTESIAN_POINT('Ctrl Pts',(-4.34966975290223,-5.50222559297022,
72.5135335063699));
#143339=CARTESIAN_POINT('Ctrl Pts',(-4.49801289671247,-5.38163482747179,
72.5048614319665));
#143340=CARTESIAN_POINT('Ctrl Pts',(-4.64118594512446,-5.25518977633341,
72.496189357563));
#143341=CARTESIAN_POINT('Ctrl Pts',(-4.78435846873139,-5.12874518868312,
72.4875173149473));
#143342=CARTESIAN_POINT('Ctrl Pts',(-4.92236072196475,-4.9964465463588,
72.4788452723316));
#143343=CARTESIAN_POINT('Ctrl Pts',(-5.05473222957506,-4.85873529324198,
72.4701732297159));
#143344=CARTESIAN_POINT('Ctrl Pts',(-5.18710326277225,-4.72102453367566,
72.4615012181804));
#143345=CARTESIAN_POINT('Ctrl Pts',(-5.31384339389555,-4.57790140690936,
72.4528292066449));
#143346=CARTESIAN_POINT('Ctrl Pts',(-5.43452972930209,-4.42984347170775,
72.4441571951094));
#143347=CARTESIAN_POINT('Ctrl Pts',(-5.55521564202016,-4.28178605506015,
72.4354852139465));
#143348=CARTESIAN_POINT('Ctrl Pts',(-5.66984762199455,-4.12879408471962,
72.4268132327835));
#143349=CARTESIAN_POINT('Ctrl Pts',(-5.77804317951233,-3.97137804523707,
72.4181412516206));
#143350=CARTESIAN_POINT('Ctrl Pts',(-5.88623836691534,-3.81396254424245,
72.4094693001228));
#143351=CARTESIAN_POINT('Ctrl Pts',(-5.98799701504128,-3.65212323845831,
72.400797348625));
#143352=CARTESIAN_POINT('Ctrl Pts',(-6.08297959062815,-3.4864001294317,
72.3921253971271));
#143353=CARTESIAN_POINT('Ctrl Pts',(-6.17796184904699,-3.32067757379155,
72.3834534745869));
#143354=CARTESIAN_POINT('Ctrl Pts',(-6.26616793897404,-3.15107148727796,
72.3747815520466));
#143355=CARTESIAN_POINT('Ctrl Pts',(-6.34730354928998,-2.97814778271174,
72.3661096295063));
#143356=CARTESIAN_POINT('Ctrl Pts',(-6.42843889529457,-2.80522464147027,
72.3574377352162));
#143357=CARTESIAN_POINT('Ctrl Pts',(-6.50250368713934,-2.62898416092365,
72.348765840926));
#143358=CARTESIAN_POINT('Ctrl Pts',(-6.56925079959824,-2.45001438658591,
72.3400939466358));
#143359=CARTESIAN_POINT('Ctrl Pts',(-6.6359977000629,-2.27104518067068,
72.3314220798883));
#143360=CARTESIAN_POINT('Ctrl Pts',(-6.69542686840552,-2.08934696441759,
72.3227502131407));
#143361=CARTESIAN_POINT('Ctrl Pts',(-6.74734001400655,-1.90552598982173,
72.3140783463932));
#143362=CARTESIAN_POINT('Ctrl Pts',(-6.79925299896168,-1.72170558406226,
72.3054065064808));
#143363=CARTESIAN_POINT('Ctrl Pts',(-6.84364993053014,-1.53576270642159,
72.2967346665685));
#143364=CARTESIAN_POINT('Ctrl Pts',(-6.8803826753814,-1.348317767743,72.2880628266562));
#143365=CARTESIAN_POINT('Ctrl Pts',(-6.917115309559,-1.16087339382533,72.2793910128716));
#143366=CARTESIAN_POINT('Ctrl Pts',(-6.94618374861263,-0.971927246627463,
72.270719199087));
#143367=CARTESIAN_POINT('Ctrl Pts',(-6.96749100433575,-0.782109753807224,
72.2620473853025));
#143368=CARTESIAN_POINT('Ctrl Pts',(-6.98879819759914,-0.592292817414787,
72.2533755969383));
#143369=CARTESIAN_POINT('Ctrl Pts',(-7.00234422137905,-0.401604822737071,
72.2447038085741));
#143370=CARTESIAN_POINT('Ctrl Pts',(-7.00808387899823,-0.210682005461113,
72.23603202021));
#143371=CARTESIAN_POINT('Ctrl Pts',(-7.01382352026043,-0.0197597322806402,
72.2273602565588));
#143372=CARTESIAN_POINT('Ctrl Pts',(-7.01175683134626,0.171397078292984,
72.2186884929077));
#143373=CARTESIAN_POINT('Ctrl Pts',(-7.00189070778028,0.362150629987307,
72.2100167292565));
#143374=CARTESIAN_POINT('Ctrl Pts',(-6.99157808297349,0.561536923502758,
72.2009525163112));
#143375=CARTESIAN_POINT('Ctrl Pts',(-6.97274368607662,0.76048227793352,
72.1918883033658));
#143376=CARTESIAN_POINT('Ctrl Pts',(-6.94545616842971,0.958261537849481,
72.1828240904204));
#143377=CARTESIAN_POINT('Ctrl Pts',(-6.91902138570928,1.14986019589306,
72.1740431341296));
#143378=CARTESIAN_POINT('Ctrl Pts',(-6.88465388689505,1.34036422798524,
72.1652621778388));
#143379=CARTESIAN_POINT('Ctrl Pts',(-6.84247124235475,1.52912192452015,
72.156481221548));
#143380=CARTESIAN_POINT('Ctrl Pts',(-6.80080846652573,1.71555332735041,
72.1478084838025));
#143381=CARTESIAN_POINT('Ctrl Pts',(-6.7515221588282,1.90028091507621,72.139135746057));
#143382=CARTESIAN_POINT('Ctrl Pts',(-6.69477680034255,2.08268820424354,
72.1304630083115));
#143383=CARTESIAN_POINT('Ctrl Pts',(-6.63803201373481,2.26509365511603,
72.1217903579696));
#143384=CARTESIAN_POINT('Ctrl Pts',(-6.57382841117027,2.44517858290671,
72.1131177076277));
#143385=CARTESIAN_POINT('Ctrl Pts',(-6.5023802522632,2.62234201001271,72.1044450572858));
#143386=CARTESIAN_POINT('Ctrl Pts',(-6.43093279008113,2.79950370951384,
72.095772491515));
#143387=CARTESIAN_POINT('Ctrl Pts',(-6.35224101919408,2.97374370183285,
72.0870999257442));
#143388=CARTESIAN_POINT('Ctrl Pts',(-6.26656754386888,3.14448052635553,
72.0784273599734));
#143389=CARTESIAN_POINT('Ctrl Pts',(-6.18089487601678,3.31521574168246,
72.0697548759417));
#143390=CARTESIAN_POINT('Ctrl Pts',(-6.08824076282718,3.48244760134581,
72.0610823919099));
#143391=CARTESIAN_POINT('Ctrl Pts',(-5.98891439682431,3.64561804225437,
72.0524099078781));
#143392=CARTESIAN_POINT('Ctrl Pts',(-5.88958893454844,3.80878699854671,
72.0437375027534));
#143393=CARTESIAN_POINT('Ctrl Pts',(-5.7835914886656,3.96789436735514,72.0350650976288));
#143394=CARTESIAN_POINT('Ctrl Pts',(-5.67127577279886,4.12240920717057,
72.0263926925041));
#143395=CARTESIAN_POINT('Ctrl Pts',(-5.55896104218094,4.27692269156069,
72.017720363455));
#143396=CARTESIAN_POINT('Ctrl Pts',(-5.44032831952585,4.42684349778002,
72.0090480344059));
#143397=CARTESIAN_POINT('Ctrl Pts',(-5.31577347545426,4.5716713486598,72.0003757053567));
#143398=CARTESIAN_POINT('Ctrl Pts',(-5.19121968333993,4.71649797636188,
71.9917034495518));
#143399=CARTESIAN_POINT('Ctrl Pts',(-5.06074405512955,4.85623151941838,
71.9830311937469));
#143400=CARTESIAN_POINT('Ctrl Pts',(-4.92478197319633,4.99040570284426,
71.9743589379419));
#143401=CARTESIAN_POINT('Ctrl Pts',(-4.78882099518712,5.1245787968627,71.9656867525501));
#143402=CARTESIAN_POINT('Ctrl Pts',(-4.64737385478674,5.25319242204627,
71.9570145671583));
#143403=CARTESIAN_POINT('Ctrl Pts',(-4.5009125374034,5.37581741627679,71.9483423817664));
#143404=CARTESIAN_POINT('Ctrl Pts',(-4.35445236139157,5.49844145489202,
71.9396702639568));
#143405=CARTESIAN_POINT('Ctrl Pts',(-4.20297830438701,5.6150767735941,71.9309981461472));
#143406=CARTESIAN_POINT('Ctrl Pts',(-4.04699580206867,5.72533418592649,
71.9223260283377));
#143407=CARTESIAN_POINT('Ctrl Pts',(-3.89101446441665,5.83559077500569,
71.9136539752797));
#143408=CARTESIAN_POINT('Ctrl Pts',(-3.73052498076179,5.93946938905685,
71.9049819222218));
#143409=CARTESIAN_POINT('Ctrl Pts',(-3.56606286129387,6.03662341311769,
71.8963098691638));
#143410=CARTESIAN_POINT('Ctrl Pts',(-3.40160191613826,6.13377674346761,
71.8876378780271));
#143411=CARTESIAN_POINT('Ctrl Pts',(-3.2331686364828,6.22420543544664,71.8789658868904));
#143412=CARTESIAN_POINT('Ctrl Pts',(-3.06132503080748,6.30760775716528,
71.8702938957537));
#143413=CARTESIAN_POINT('Ctrl Pts',(-2.88948259607709,6.39100951057923,
71.8616219637081));
#143414=CARTESIAN_POINT('Ctrl Pts',(-2.71423013734766,6.46738486552798,
71.8529500316625));
#143415=CARTESIAN_POINT('Ctrl Pts',(-2.53615240857771,6.53647898512383,
71.8442780996169));
#143416=CARTESIAN_POINT('Ctrl Pts',(-2.35807583512656,6.60557265645625,
71.8356062238323));
#143417=CARTESIAN_POINT('Ctrl Pts',(-2.17717429309618,6.66738508422991,
71.8269343480478));
#143418=CARTESIAN_POINT('Ctrl Pts',(-1.99405137756518,6.72171002544222,
71.8182624722632));
#143419=CARTESIAN_POINT('Ctrl Pts',(-1.8109295903359,6.77603463193441,71.80959064991));
#143420=CARTESIAN_POINT('Ctrl Pts',(-1.62558672927165,6.82287176341051,
71.8009188275567));
#143421=CARTESIAN_POINT('Ctrl Pts',(-1.43864120071842,6.8620651452821,71.7922470052035));
#143422=CARTESIAN_POINT('Ctrl Pts',(-1.25169676302724,6.90125829845299,
71.7835752334519));
#143423=CARTESIAN_POINT('Ctrl Pts',(-1.06314995451508,6.93280773300066,
71.7749034617004));
#143424=CARTESIAN_POINT('Ctrl Pts',(-0.873629864335108,6.9566081837805,
71.7662316899488));
#143425=CARTESIAN_POINT('Ctrl Pts',(-0.67949550972214,6.98098810649611,
71.7573487857103));
#143426=CARTESIAN_POINT('Ctrl Pts',(-0.484340182097022,6.99723686027412,
71.7484658814718));
#143427=CARTESIAN_POINT('Ctrl Pts',(-0.288847078981576,7.00529756166459,
71.7395829772334));
#143428=CARTESIAN_POINT('Ctrl Pts',(-0.0979805524071825,7.01316749698012,
71.730910297477));
#143429=CARTESIAN_POINT('Ctrl Pts',(0.0932076478762551,7.0132325545162,
71.7222376177207));
#143430=CARTESIAN_POINT('Ctrl Pts',(0.284079486213397,7.005492517162,71.7135649379643));
#143431=CARTESIAN_POINT('Ctrl Pts',(0.474947621905027,6.99775262995365,
71.7048924264458));
#143432=CARTESIAN_POINT('Ctrl Pts',(0.665499124040627,6.98220796234813,
71.6962199149273));
#143433=CARTESIAN_POINT('Ctrl Pts',(0.855098106408511,6.95891038819416,
71.6875474034087));
#143434=CARTESIAN_POINT('Ctrl Pts',(1.0446936584049,6.93561323555793,71.6788750488));
#143435=CARTESIAN_POINT('Ctrl Pts',(1.23333644314323,6.90456349171855,71.6702026941912));
#143436=CARTESIAN_POINT('Ctrl Pts',(1.4203969667169,6.86586476850815,71.6615303395825));
#143437=CARTESIAN_POINT('Ctrl Pts',(1.60745435008166,6.82716669493816,71.6528581305576));
#143438=CARTESIAN_POINT('Ctrl Pts',(1.79292924725158,6.78081995649635,71.6441859215328));
#143439=CARTESIAN_POINT('Ctrl Pts',(1.9762027562011,6.72697920532561,71.635513712508));
#143440=CARTESIAN_POINT('Ctrl Pts',(2.15947342777526,6.67313928769825,71.6268416377432));
#143441=CARTESIAN_POINT('Ctrl Pts',(2.3405425067949,6.61180566957133,71.6181695629785));
#143442=CARTESIAN_POINT('Ctrl Pts',(2.51880581148067,6.54318300573591,71.6094974882137));
#143443=CARTESIAN_POINT('Ctrl Pts',(2.69706658904941,6.47456131471709,71.600825536387));
#143444=CARTESIAN_POINT('Ctrl Pts',(2.87252140681086,6.39865088680505,71.5921535845603));
#143445=CARTESIAN_POINT('Ctrl Pts',(3.04458483293961,6.31570500874875,71.5834816327337));
#143446=CARTESIAN_POINT('Ctrl Pts',(3.21664604441903,6.23276019829896,71.5748097925247));
#143447=CARTESIAN_POINT('Ctrl Pts',(3.3853156957798,6.14278024224237,71.5661379523158));
#143448=CARTESIAN_POINT('Ctrl Pts',(3.55003100941456,6.04606536473888,71.5574661121068));
#143449=CARTESIAN_POINT('Ctrl Pts',(3.72225670715308,5.94494066119936,71.5483988693733));
#143450=CARTESIAN_POINT('Ctrl Pts',(3.89015872997921,5.83645264820113,71.5393316266397));
#143451=CARTESIAN_POINT('Ctrl Pts',(4.05312466659174,5.72099702845279,71.5302643839061));
#143452=CARTESIAN_POINT('Ctrl Pts',(4.20899688867359,5.61056705531797,71.5215918275277));
#143453=CARTESIAN_POINT('Ctrl Pts',(4.36035338103252,5.49376336254134,71.5129192711493));
#143454=CARTESIAN_POINT('Ctrl Pts',(4.50668904924442,5.37097573778922,71.5042467147709));
#143455=CARTESIAN_POINT('Ctrl Pts',(4.65301950883502,5.24819248349745,71.4955744670804));
#143456=CARTESIAN_POINT('Ctrl Pts',(4.79432928426434,5.11942590604493,71.48690221939));
#143457=CARTESIAN_POINT('Ctrl Pts',(4.93014684172017,4.98510568409303,71.4782299716995));
#143458=CARTESIAN_POINT('Ctrl Pts',(5.06596027419377,4.85078954164705,71.4695579873982));
#143459=CARTESIAN_POINT('Ctrl Pts',(5.19628162052971,4.71092029196069,71.4608860030969));
#143460=CARTESIAN_POINT('Ctrl Pts',(5.32067604037713,4.56596463366251,71.4522140187955));
#143461=CARTESIAN_POINT('Ctrl Pts',(5.44506733163951,4.42101262107531,71.4435422525992));
#143462=CARTESIAN_POINT('Ctrl Pts',(5.56353180975275,4.2709746713911,71.4348704864028));
#143463=CARTESIAN_POINT('Ctrl Pts',(5.67567421677841,4.11635138775795,71.4261987202064));
#143464=CARTESIAN_POINT('Ctrl Pts',(5.78782406005803,3.96171785092946,71.4175263789782));
#143465=CARTESIAN_POINT('Ctrl Pts',(5.89365082653992,3.80249860162828,71.40885403775));
#143466=CARTESIAN_POINT('Ctrl Pts',(5.99280137735697,3.63922494688751,71.4001816965218));
#143467=CARTESIAN_POINT('Ctrl Pts',(6.09194609290613,3.47596090122614,71.3915098656834));
#143468=CARTESIAN_POINT('Ctrl Pts',(6.18441523160251,3.3086431703721,71.3828380348451));
#143469=CARTESIAN_POINT('Ctrl Pts',(6.26990026462747,3.13783001995398,71.3741662040067));
#143470=CARTESIAN_POINT('Ctrl Pts',(6.35538670852191,2.96701405038669,71.365494230046));
#143471=CARTESIAN_POINT('Ctrl Pts',(6.43388868896847,2.79270279980033,71.3568222560852));
#143472=CARTESIAN_POINT('Ctrl Pts',(6.50514427077116,2.6154778872996,71.3481502821245));
#143473=CARTESIAN_POINT('Ctrl Pts',(6.52787183386102,2.55895052090873,71.3453842835834));
#143474=CARTESIAN_POINT('Ctrl Pts',(6.54986255129665,2.5021268966415,71.3426182850424));
#143475=CARTESIAN_POINT('Ctrl Pts',(6.57110895151817,2.44502632087629,71.3398522865014));
#143476=CARTESIAN_POINT('Origin',(0.,0.,50.));
#143477=CARTESIAN_POINT('',(6.57110895151815,2.44502632087633,69.3398494195812));
#143478=CARTESIAN_POINT('',(6.57110895151813,2.44502632087638,69.887000105296));
#143479=CARTESIAN_POINT('',(6.57110895151814,2.44502632087636,50.));
#143480=CARTESIAN_POINT('',(7.01124919374723,-0.00336239182316637,71.7735343569455));
#143481=CARTESIAN_POINT('Ctrl Pts',(6.57110895151813,2.44502632087638,69.887000105296));
#143482=CARTESIAN_POINT('Ctrl Pts',(6.50935707499648,2.61098703267723,69.8950229664158));
#143483=CARTESIAN_POINT('Ctrl Pts',(6.4413031944783,2.77463542245891,69.9030458275357));
#143484=CARTESIAN_POINT('Ctrl Pts',(6.36715806475345,2.93545988576665,69.9110686886556));
#143485=CARTESIAN_POINT('Ctrl Pts',(6.29301396543497,3.09628211407184,69.9190914382805));
#143486=CARTESIAN_POINT('Ctrl Pts',(6.21277894391802,3.25428016343137,69.9271141879055));
#143487=CARTESIAN_POINT('Ctrl Pts',(6.12671087069771,3.40896472105162,69.9351369375304));
#143488=CARTESIAN_POINT('Ctrl Pts',(6.04061153883583,3.563705457798,69.9431626008985));
#143489=CARTESIAN_POINT('Ctrl Pts',(5.94867510931066,3.71512998294193,69.9511882642665));
#143490=CARTESIAN_POINT('Ctrl Pts',(5.85120427308608,3.86277557167372,69.9592139276345));
#143491=CARTESIAN_POINT('Ctrl Pts',(5.8324204731663,3.89122864856521,69.9607605692842));
#143492=CARTESIAN_POINT('Ctrl Pts',(5.8134312644223,3.91954147243274,69.9623072109338));
#143493=CARTESIAN_POINT('Ctrl Pts',(5.79423899333395,3.94771086208556,69.9638538525834));
#143494=CARTESIAN_POINT('Ctrl Pts',(5.68590784636475,4.10671352917298,69.9725839014183));
#143495=CARTESIAN_POINT('Ctrl Pts',(5.57104950672155,4.26122332956056,69.9813139502533));
#143496=CARTESIAN_POINT('Ctrl Pts',(5.45005695875983,4.41072621104207,69.9900439990882));
#143497=CARTESIAN_POINT('Ctrl Pts',(5.32902942565171,4.56027232146855,69.9987765722276));
#143498=CARTESIAN_POINT('Ctrl Pts',(5.20186431613109,4.70480841024443,70.0075091453671));
#143499=CARTESIAN_POINT('Ctrl Pts',(5.0689946415254,4.84385382590007,70.0162417185065));
#143500=CARTESIAN_POINT('Ctrl Pts',(4.93423734109838,4.98487460363671,70.0250983517868));
#143501=CARTESIAN_POINT('Ctrl Pts',(4.79361235559935,5.1202473021447,70.0339549850671));
#143502=CARTESIAN_POINT('Ctrl Pts',(4.64761012010458,5.24950918981971,70.0428116183474));
#143503=CARTESIAN_POINT('Ctrl Pts',(4.50356138495889,5.37704156190312,70.0515497504545));
#143504=CARTESIAN_POINT('Ctrl Pts',(4.35427862401281,5.49862546533893,70.0602878825615));
#143505=CARTESIAN_POINT('Ctrl Pts',(4.200266932895,5.61385645122217,70.0690260146685));
#143506=CARTESIAN_POINT('Ctrl Pts',(4.04312232403179,5.73143147474227,70.0779418985354));
#143507=CARTESIAN_POINT('Ctrl Pts',(3.88105456657115,5.84239216862962,70.0868577824024));
#143508=CARTESIAN_POINT('Ctrl Pts',(3.71463300631888,5.94635419318984,70.0957736662693));
#143509=CARTESIAN_POINT('Ctrl Pts',(3.54821144606662,6.05031621775005,70.1046895501362));
#143510=CARTESIAN_POINT('Ctrl Pts',(3.37743634272625,6.1472794179211,70.1136054340031));
#143511=CARTESIAN_POINT('Ctrl Pts',(3.20290638631624,6.23690766670428,70.1225213178701));
#143512=CARTESIAN_POINT('Ctrl Pts',(3.03180598765053,6.3247746977513,70.1312620023661));
#143513=CARTESIAN_POINT('Ctrl Pts',(2.85707876118995,6.40560170126693,70.1400026868622));
#143514=CARTESIAN_POINT('Ctrl Pts',(2.67931053117118,6.47911426354369,70.1487433713582));
#143515=CARTESIAN_POINT('Ctrl Pts',(2.50157428460959,6.55261359968949,70.1574824832599));
#143516=CARTESIAN_POINT('Ctrl Pts',(2.32079838006797,6.61880101813621,70.1662215951617));
#143517=CARTESIAN_POINT('Ctrl Pts',(2.13758879099239,6.67745016627782,70.1749607070634));
#143518=CARTESIAN_POINT('Ctrl Pts',(1.95200545800082,6.73685919854604,70.1838130467378));
#143519=CARTESIAN_POINT('Ctrl Pts',(1.76392520167813,6.78853315221968,70.1926653864122));
#143520=CARTESIAN_POINT('Ctrl Pts',(1.57399524889274,6.83228845402206,70.2015177260866));
#143521=CARTESIAN_POINT('Ctrl Pts',(1.38659074028235,6.87546195411048,70.2102523587363));
#143522=CARTESIAN_POINT('Ctrl Pts',(1.19738569639967,6.91092602912153,70.2189869913858));
#143523=CARTESIAN_POINT('Ctrl Pts',(1.00701460405256,6.93855519180506,70.2277216240355));
#143524=CARTESIAN_POINT('Ctrl Pts',(0.812795379370071,6.96674284618504,
70.2366328172223));
#143525=CARTESIAN_POINT('Ctrl Pts',(0.617362747750107,6.98677540412073,
70.2455440104091));
#143526=CARTESIAN_POINT('Ctrl Pts',(0.421399684128626,6.99857477410339,
70.2544552035959));
#143527=CARTESIAN_POINT('Ctrl Pts',(0.225436620507078,7.01037414408606,
70.2633663967828));
#143528=CARTESIAN_POINT('Ctrl Pts',(0.0289434266559483,7.01394029444692,
70.2722775899696));
#143529=CARTESIAN_POINT('Ctrl Pts',(-0.167392073520737,7.00925149043908,
70.2811887831564));
#143530=CARTESIAN_POINT('Ctrl Pts',(-0.34421720681212,7.00502862502291,
70.2892144480088));
#143531=CARTESIAN_POINT('Ctrl Pts',(-0.520995680480194,6.994107460158,70.2972401128612));
#143532=CARTESIAN_POINT('Ctrl Pts',(-0.697174942038089,6.97650153462996,
70.3052657777136));
#143533=CARTESIAN_POINT('Ctrl Pts',(-0.873298288620175,6.9589011967908,
70.3132888954168));
#143534=CARTESIAN_POINT('Ctrl Pts',(-1.0488224373931,6.93462035856031,70.3213120131201));
#143535=CARTESIAN_POINT('Ctrl Pts',(-1.22319820765153,6.90372455326095,
70.3293351308233));
#143536=CARTESIAN_POINT('Ctrl Pts',(-1.39755198759958,6.87283264419297,
70.3373572367412));
#143537=CARTESIAN_POINT('Ctrl Pts',(-1.57075731675607,6.83532749421412,
70.3453793426591));
#143538=CARTESIAN_POINT('Ctrl Pts',(-1.7422735306847,6.79132604921715,70.353401448577));
#143539=CARTESIAN_POINT('Ctrl Pts',(-1.91385348061782,6.74730825313459,
70.3614265355366));
#143540=CARTESIAN_POINT('Ctrl Pts',(-2.08374270526499,6.69678942780533,
70.3694516224961));
#143541=CARTESIAN_POINT('Ctrl Pts',(-2.25141363242581,6.63993698902537,
70.3774767094557));
#143542=CARTESIAN_POINT('Ctrl Pts',(-2.41911758153682,6.58307335344204,
70.385503376916));
#143543=CARTESIAN_POINT('Ctrl Pts',(-2.58460201849845,6.51987374548574,
70.3935300443762));
#143544=CARTESIAN_POINT('Ctrl Pts',(-2.747357977816,6.4505542943402,70.4015567118365));
#143545=CARTESIAN_POINT('Ctrl Pts',(-2.91024459704388,6.38117919378367,
70.4095898230771));
#143546=CARTESIAN_POINT('Ctrl Pts',(-3.07039803027828,6.30567458973282,
70.4176229343178));
#143547=CARTESIAN_POINT('Ctrl Pts',(-3.22733204274851,6.22430353118714,
70.4256560455584));
#143548=CARTESIAN_POINT('Ctrl Pts',(-3.31980326383186,6.17635674752869,
70.4303894465199));
#143549=CARTESIAN_POINT('Ctrl Pts',(-3.41115718157247,6.12637399944037,
70.4351228474814));
#143550=CARTESIAN_POINT('Ctrl Pts',(-3.50129888771257,6.07441624038086,
70.4398562484429));
#143551=CARTESIAN_POINT('Ctrl Pts',(-3.68699360776641,5.96738163968023,
70.4496072017372));
#143552=CARTESIAN_POINT('Ctrl Pts',(-3.86765228367227,5.85190080474336,
70.4593581550316));
#143553=CARTESIAN_POINT('Ctrl Pts',(-4.04260209641249,5.72843738314222,
70.469109108326));
#143554=CARTESIAN_POINT('Ctrl Pts',(-4.21780395717759,5.60479608932122,
70.4788741096978));
#143555=CARTESIAN_POINT('Ctrl Pts',(-4.38728047141502,5.47314922690004,
70.4886391110696));
#143556=CARTESIAN_POINT('Ctrl Pts',(-4.55038851878558,5.33400327058434,
70.4984041124415));
#143557=CARTESIAN_POINT('Ctrl Pts',(-4.71322469883662,5.19508924174724,
70.5081528375793));
#143558=CARTESIAN_POINT('Ctrl Pts',(-4.86971359808391,5.04870112491487,
70.5179015627171));
#143559=CARTESIAN_POINT('Ctrl Pts',(-5.01924811638757,4.89538301960529,
70.5276502878549));
#143560=CARTESIAN_POINT('Ctrl Pts',(-5.1683722204212,4.74248571304497,70.5373722565224));
#143561=CARTESIAN_POINT('Ctrl Pts',(-5.31058001986225,4.58269641717835,
70.5470942251898));
#143562=CARTESIAN_POINT('Ctrl Pts',(-5.44530257869364,4.41659443338105,
70.5568161938572));
#143563=CARTESIAN_POINT('Ctrl Pts',(-5.57913371353883,4.25159150302954,
70.5664738347971));
#143564=CARTESIAN_POINT('Ctrl Pts',(-5.70557828430508,4.08035916550015,
70.5761314757369));
#143565=CARTESIAN_POINT('Ctrl Pts',(-5.82411204847887,3.90350424737355,
70.5857891166768));
#143566=CARTESIAN_POINT('Ctrl Pts',(-5.87621171868739,3.825770422135,70.590033982361));
#143567=CARTESIAN_POINT('Ctrl Pts',(-5.9267835374794,3.74695087419612,70.5942788480452));
#143568=CARTESIAN_POINT('Ctrl Pts',(-5.97578510504719,3.66709952698262,
70.5985237137293));
#143569=CARTESIAN_POINT('Ctrl Pts',(-6.06642467779315,3.51939625229435,
70.6063755607432));
#143570=CARTESIAN_POINT('Ctrl Pts',(-6.15165117836031,3.36822136138251,
70.614227407757));
#143571=CARTESIAN_POINT('Ctrl Pts',(-6.23118342980272,3.21402856655819,
70.6220792547708));
#143572=CARTESIAN_POINT('Ctrl Pts',(-6.31069312654178,3.05987949956354,
70.6299288750643));
#143573=CARTESIAN_POINT('Ctrl Pts',(-6.38451161166049,2.90271456978279,
70.6377784953578));
#143574=CARTESIAN_POINT('Ctrl Pts',(-6.45240311453084,2.74301305321223,
70.6456281156512));
#143575=CARTESIAN_POINT('Ctrl Pts',(-6.52028919713257,2.58332428676625,
70.6534771092529));
#143576=CARTESIAN_POINT('Ctrl Pts',(-6.58224909093422,2.42109968803214,
70.6613261028546));
#143577=CARTESIAN_POINT('Ctrl Pts',(-6.63809483719363,2.25683927095469,
70.6691750964562));
#143578=CARTESIAN_POINT('Ctrl Pts',(-6.69396885651942,2.09249569363698,
70.6770280637736));
#143579=CARTESIAN_POINT('Ctrl Pts',(-6.74372242056195,1.92611460026772,
70.6848810310909));
#143580=CARTESIAN_POINT('Ctrl Pts',(-6.78721711243595,1.75821228273398,
70.6927339984082));
#143581=CARTESIAN_POINT('Ctrl Pts',(-6.83072285050017,1.59026732365346,
70.7005889601154));
#143582=CARTESIAN_POINT('Ctrl Pts',(-6.86796646776411,1.42080074334621,
70.7084439218225));
#143583=CARTESIAN_POINT('Ctrl Pts',(-6.89886066457496,1.25033919129185,
70.7162988835297));
#143584=CARTESIAN_POINT('Ctrl Pts',(-6.92978552645864,1.0797084418979,70.724161641943));
#143585=CARTESIAN_POINT('Ctrl Pts',(-6.95434832651003,0.908081125735139,
70.7320244003562));
#143586=CARTESIAN_POINT('Ctrl Pts',(-6.97251358095588,0.73598975936209,
70.7398871587695));
#143587=CARTESIAN_POINT('Ctrl Pts',(-6.985839350963,0.609746002340369,70.7456551655182));
#143588=CARTESIAN_POINT('Ctrl Pts',(-6.99572338168467,0.483252631127725,
70.751423172267));
#143589=CARTESIAN_POINT('Ctrl Pts',(-7.00216950191017,0.356719538319783,
70.7571911790158));
#143590=CARTESIAN_POINT('Ctrl Pts',(-7.01153253248355,0.172929417276306,
70.7655692454568));
#143591=CARTESIAN_POINT('Ctrl Pts',(-7.01366137701738,-0.0113515913451885,
70.7739473118978));
#143592=CARTESIAN_POINT('Ctrl Pts',(-7.00852298676297,-0.195530321216453,
70.7823253783389));
#143593=CARTESIAN_POINT('Ctrl Pts',(-7.00338811007876,-0.379583111860833,
70.7906977159576));
#143594=CARTESIAN_POINT('Ctrl Pts',(-6.99099591495639,-0.563533435639649,
70.7990700535764));
#143595=CARTESIAN_POINT('Ctrl Pts',(-6.97136540613591,-0.746787075833213,
70.8074423911951));
#143596=CARTESIAN_POINT('Ctrl Pts',(-6.95174544159702,-0.929942283632423,
70.8158102317177));
#143597=CARTESIAN_POINT('Ctrl Pts',(-6.92489495053787,-1.11240122787188,
70.8241780722404));
#143598=CARTESIAN_POINT('Ctrl Pts',(-6.89088489724594,-1.29357330499971,
70.832545912763));
#143599=CARTESIAN_POINT('Ctrl Pts',(-6.85688812980171,-1.4746746082124,
70.8409104844329));
#143600=CARTESIAN_POINT('Ctrl Pts',(-6.81573743799092,-1.65448972419131,
70.8492750561028));
#143601=CARTESIAN_POINT('Ctrl Pts',(-6.76755522877475,-1.83243629847905,
70.8576396277727));
#143602=CARTESIAN_POINT('Ctrl Pts',(-6.71938478897124,-2.01033940596234,
70.8660021562383));
#143603=CARTESIAN_POINT('Ctrl Pts',(-6.66418634327739,-2.18637456511051,
70.8743646847039));
#143604=CARTESIAN_POINT('Ctrl Pts',(-6.60213280590181,-2.35997224045857,
70.8827272131695));
#143605=CARTESIAN_POINT('Ctrl Pts',(-6.54007431646009,-2.53358376944347,
70.8910904089911));
#143606=CARTESIAN_POINT('Ctrl Pts',(-6.47115974733332,-2.70475711448229,
70.8994536048126));
#143607=CARTESIAN_POINT('Ctrl Pts',(-6.39561129658583,-2.8729397323097,
70.9078168006341));
#143608=CARTESIAN_POINT('Ctrl Pts',(-6.32005769358556,-3.04113381985424,
70.9161805668088));
#143609=CARTESIAN_POINT('Ctrl Pts',(-6.2378694413764,-3.20633647344641,
70.9245443329835));
#143610=CARTESIAN_POINT('Ctrl Pts',(-6.14931620337863,-3.3680167448166,
70.9329080991582));
#143611=CARTESIAN_POINT('Ctrl Pts',(-6.06074511999784,-3.52972959824066,
70.9412735508118));
#143612=CARTESIAN_POINT('Ctrl Pts',(-5.96580665108144,-3.68791836565289,
70.9496390024653));
#143613=CARTESIAN_POINT('Ctrl Pts',(-5.8648157864291,-3.84207786929834,
70.9580044541189));
#143614=CARTESIAN_POINT('Ctrl Pts',(-5.76379110013426,-3.99628900065919,
70.9663727073458));
#143615=CARTESIAN_POINT('Ctrl Pts',(-5.65671015643478,-4.14646790261302,
70.9747409605727));
#143616=CARTESIAN_POINT('Ctrl Pts',(-5.5439307587409,-4.2921391292439,70.9831092137996));
#143617=CARTESIAN_POINT('Ctrl Pts',(-5.43104679845622,-4.43794541388337,
70.9914852255911));
#143618=CARTESIAN_POINT('Ctrl Pts',(-5.31245402809057,-4.57923541155135,
70.9998612373825));
#143619=CARTESIAN_POINT('Ctrl Pts',(-5.18855075560524,-4.71556652153358,
71.008237249174));
#143620=CARTESIAN_POINT('Ctrl Pts',(-5.0645867194242,-4.85196448997658,
71.0166173686652));
#143621=CARTESIAN_POINT('Ctrl Pts',(-4.93530721340399,-4.98339848230032,
71.0249974881563));
#143622=CARTESIAN_POINT('Ctrl Pts',(-4.80114721921409,-5.10946297979864,
71.0333776076475));
#143623=CARTESIAN_POINT('Ctrl Pts',(-4.66683393023635,-5.23567152195436,
71.0417673024866));
#143624=CARTESIAN_POINT('Ctrl Pts',(-4.52762925404168,-5.35649808920436,
71.0501569973259));
#143625=CARTESIAN_POINT('Ctrl Pts',(-4.38400205491484,-5.47157678781926,
71.0585466921651));
#143626=CARTESIAN_POINT('Ctrl Pts',(-4.29281562472936,-5.54463826768434,
71.0638731646395));
#143627=CARTESIAN_POINT('Ctrl Pts',(-4.19984721973291,-5.61538375356384,
71.069199637114));
#143628=CARTESIAN_POINT('Ctrl Pts',(-4.10522283754347,-5.68372870716148,
71.0745261095884));
#143629=CARTESIAN_POINT('Ctrl Pts',(-3.95632966733252,-5.79127072301,71.0829074099934));
#143630=CARTESIAN_POINT('Ctrl Pts',(-3.80303460730352,-5.89308390277214,
71.0912887103984));
#143631=CARTESIAN_POINT('Ctrl Pts',(-3.64580334336631,-5.988801594977,71.0996700108033));
#143632=CARTESIAN_POINT('Ctrl Pts',(-3.48877134704022,-6.08439797901839,
71.1080406891369));
#143633=CARTESIAN_POINT('Ctrl Pts',(-3.32781336609375,-6.17391410190532,
71.1164113674705));
#143634=CARTESIAN_POINT('Ctrl Pts',(-3.16342614885192,-6.25702497703661,
71.124782045804));
#143635=CARTESIAN_POINT('Ctrl Pts',(-2.9992254828764,-6.34004153559474,
71.1331432248549));
#143636=CARTESIAN_POINT('Ctrl Pts',(-2.83160362760783,-6.41666718709266,
71.1415044039059));
#143637=CARTESIAN_POINT('Ctrl Pts',(-2.66108454776913,-6.48662127706901,
71.1498655829568));
#143638=CARTESIAN_POINT('Ctrl Pts',(-2.49078673655147,-6.55648459336161,
71.1582159123916));
#143639=CARTESIAN_POINT('Ctrl Pts',(-2.31759950116911,-6.61969349194116,
71.1665662418264));
#143640=CARTESIAN_POINT('Ctrl Pts',(-2.14206945952485,-6.67601415464879,
71.1749165712612));
#143641=CARTESIAN_POINT('Ctrl Pts',(-1.96667447774646,-6.73229148197587,
71.183260475617));
#143642=CARTESIAN_POINT('Ctrl Pts',(-1.78894059271763,-6.78169103585769,
71.1916043799728));
#143643=CARTESIAN_POINT('Ctrl Pts',(-1.60943344468846,-6.82402744349832,
71.1999482843287));
#143644=CARTESIAN_POINT('Ctrl Pts',(-1.43007047792197,-6.86632984627186,
71.2082854868084));
#143645=CARTESIAN_POINT('Ctrl Pts',(-1.24893740668833,-6.90158034212509,
71.2166226892882));
#143646=CARTESIAN_POINT('Ctrl Pts',(-1.06661419242548,-6.92964362193443,
71.2249598917679));
#143647=CARTESIAN_POINT('Ctrl Pts',(-1.00659439669826,-6.93888189874083,
71.2277044528036));
#143648=CARTESIAN_POINT('Ctrl Pts',(-0.946445732503702,-6.94734171020637,
71.2304490138393));
#143649=CARTESIAN_POINT('Ctrl Pts',(-0.886189172522259,-6.95501943297101,
71.233193574875));
#143650=CARTESIAN_POINT('Ctrl Pts',(-0.703122413099019,-6.97834528872355,
71.2415318851769));
#143651=CARTESIAN_POINT('Ctrl Pts',(-0.519209392211515,-6.99442936365933,
71.2498701954787));
#143652=CARTESIAN_POINT('Ctrl Pts',(-0.335045536714064,-7.003240039498,
71.2582085057805));
#143653=CARTESIAN_POINT('Ctrl Pts',(-0.150765811567265,-7.01205625871498,
71.2665520622643));
#143654=CARTESIAN_POINT('Ctrl Pts',(0.033764735698275,-7.01358993542551,
71.2748956187481));
#143655=CARTESIAN_POINT('Ctrl Pts',(0.217950683141193,-7.00786158983026,
71.2832391752318));
#143656=CARTESIAN_POINT('Ctrl Pts',(0.402276758448518,-7.0021288861347,
71.2915890794569));
#143657=CARTESIAN_POINT('Ctrl Pts',(0.586257383867467,-6.98912314990522,
71.299938983682));
#143658=CARTESIAN_POINT('Ctrl Pts',(0.769301819284021,-6.96891679340099,
71.3082888879071));
#143659=CARTESIAN_POINT('Ctrl Pts',(0.952620807809685,-6.94868012885713,
71.3166513163707));
#143660=CARTESIAN_POINT('Ctrl Pts',(1.13500047431318,-6.92122129742962,
71.3250137448343));
#143661=CARTESIAN_POINT('Ctrl Pts',(1.31585833880889,-6.88666417031404,
71.3333761732979));
#143662=CARTESIAN_POINT('Ctrl Pts',(1.49687086143248,-6.8520774921441,71.3417457527778));
#143663=CARTESIAN_POINT('Ctrl Pts',(1.67635866712909,-6.81038048101128,
71.3501153322576));
#143664=CARTESIAN_POINT('Ctrl Pts',(1.85375346567542,-6.76174715964716,
71.3584849117375));
#143665=CARTESIAN_POINT('Ctrl Pts',(2.03142187408473,-6.71303882731031,
71.366867400274));
#143666=CARTESIAN_POINT('Ctrl Pts',(2.20699051269871,-6.65737290495638,
71.3752498888104));
#143667=CARTESIAN_POINT('Ctrl Pts',(2.37990879088698,-6.59497238125823,
71.3836323773469));
#143668=CARTESIAN_POINT('Ctrl Pts',(2.43649048495389,-6.57455390740749,
71.3863752649517));
#143669=CARTESIAN_POINT('Ctrl Pts',(2.49278858440483,-6.55341473034262,
71.3891181525565));
#143670=CARTESIAN_POINT('Ctrl Pts',(2.54878435310448,-6.53156373955501,
71.3918610401613));
#143671=CARTESIAN_POINT('Ctrl Pts',(2.72006238382453,-6.46472664171179,
71.4002508952942));
#143672=CARTESIAN_POINT('Ctrl Pts',(2.8888558835757,-6.3910913488721,71.408640750427));
#143673=CARTESIAN_POINT('Ctrl Pts',(3.05460822287005,-6.31086326640617,
71.4170306055598));
#143674=CARTESIAN_POINT('Ctrl Pts',(3.22020760822928,-6.23070921729006,
71.4254127186519));
#143675=CARTESIAN_POINT('Ctrl Pts',(3.38277113310771,-6.14397464898929,
71.433794831744));
#143676=CARTESIAN_POINT('Ctrl Pts',(3.54176177336686,-6.05091316275628,
71.4421769448361));
#143677=CARTESIAN_POINT('Ctrl Pts',(3.70062907058682,-5.95792387251245,
71.450552555185));
#143678=CARTESIAN_POINT('Ctrl Pts',(3.85592872663196,-5.85861761554745,
71.4589281655339));
#143679=CARTESIAN_POINT('Ctrl Pts',(4.00714757241335,-5.75329426462803,
71.4673037758828));
#143680=CARTESIAN_POINT('Ctrl Pts',(4.15827129929455,-5.64803716366082,
71.4756741178484));
#143681=CARTESIAN_POINT('Ctrl Pts',(4.30531906500941,-5.53677070276705,
71.484044459814));
#143682=CARTESIAN_POINT('Ctrl Pts',(4.44780561295396,-5.4198387237883,71.4924148017796));
#143683=CARTESIAN_POINT('Ctrl Pts',(4.59022342167176,-5.30296315584578,
71.5007811056739));
#143684=CARTESIAN_POINT('Ctrl Pts',(4.72808414701667,-5.18042772841354,
71.5091474095682));
#143685=CARTESIAN_POINT('Ctrl Pts',(4.86093427647319,-5.05261759114106,
71.5175137134626));
#143686=CARTESIAN_POINT('Ctrl Pts',(4.99374725147239,-4.92484319878136,
71.5258776775362));
#143687=CARTESIAN_POINT('Ctrl Pts',(5.12155218716623,-4.79179726470219,
71.5342416416099));
#143688=CARTESIAN_POINT('Ctrl Pts',(5.24393081960761,-4.65390332104884,
71.5426056056835));
#143689=CARTESIAN_POINT('Ctrl Pts',(5.36629062001084,-4.51603059698226,
71.550968282682));
#143690=CARTESIAN_POINT('Ctrl Pts',(5.48322556392833,-4.37331159651445,
71.5593309596806));
#143691=CARTESIAN_POINT('Ctrl Pts',(5.59435596157596,-4.22620490957071,
71.5676936366791));
#143692=CARTESIAN_POINT('Ctrl Pts',(5.70548407125212,-4.07910125128437,
71.5760561415055));
#143693=CARTESIAN_POINT('Ctrl Pts',(5.8108076751712,-3.92761034912387,71.5844186463318));
#143694=CARTESIAN_POINT('Ctrl Pts',(5.90998865498239,-3.77222224431163,
71.5927811511581));
#143695=CARTESIAN_POINT('Ctrl Pts',(6.00918081295636,-3.61681662652934,
71.6011445984781));
#143696=CARTESIAN_POINT('Ctrl Pts',(6.1022287902082,-3.45751320769643,71.609508045798));
#143697=CARTESIAN_POINT('Ctrl Pts',(6.18883869360879,-3.29482961425787,
71.6178714931179));
#143698=CARTESIAN_POINT('Ctrl Pts',(6.27549959535505,-3.13205022814655,
71.6262398650708));
#143699=CARTESIAN_POINT('Ctrl Pts',(6.35571469263457,-2.96588698021059,
71.6346082370236));
#143700=CARTESIAN_POINT('Ctrl Pts',(6.42923635906474,-2.79688154947254,
71.6429766089764));
#143701=CARTESIAN_POINT('Ctrl Pts',(6.50278005450727,-2.62782548029141,
71.6513474883121));
#143702=CARTESIAN_POINT('Ctrl Pts',(6.56962619384954,-2.45592583379929,
71.6597183676478));
#143703=CARTESIAN_POINT('Ctrl Pts',(6.6295756786435,-2.28174338689489,71.6680892469836));
#143704=CARTESIAN_POINT('Ctrl Pts',(6.68957595798786,-2.1074133570862,71.6764672188748));
#143705=CARTESIAN_POINT('Ctrl Pts',(6.74266780455232,-1.93079697476473,
71.6848451907661));
#143706=CARTESIAN_POINT('Ctrl Pts',(6.7887019480829,-1.75247037709501,71.6932231626574));
#143707=CARTESIAN_POINT('Ctrl Pts',(6.81795702115392,-1.63914237215731,
71.6985474320164));
#143708=CARTESIAN_POINT('Ctrl Pts',(6.84436271219509,-1.52512392652085,
71.7038717013753));
#143709=CARTESIAN_POINT('Ctrl Pts',(6.86789146169496,-1.41056493394581,
71.7091959707343));
#143710=CARTESIAN_POINT('Ctrl Pts',(6.90680224734189,-1.22111243439664,
71.7180010074727));
#143711=CARTESIAN_POINT('Ctrl Pts',(6.93790954719751,-1.02985490893788,
71.726806044211));
#143712=CARTESIAN_POINT('Ctrl Pts',(6.96105872276573,-0.83742941237284,
71.7356110809493));
#143713=CARTESIAN_POINT('Ctrl Pts',(6.9841432039996,-0.645541681801989,
71.744391510505));
#143714=CARTESIAN_POINT('Ctrl Pts',(6.99931389611826,-0.452492746218981,
71.7531719400608));
#143715=CARTESIAN_POINT('Ctrl Pts',(7.00646718374247,-0.258928881432433,
71.7619523696164));
#143716=CARTESIAN_POINT('Ctrl Pts',(7.00961240899781,-0.173820888013127,
71.7658130320478));
#143717=CARTESIAN_POINT('Ctrl Pts',(7.01120830977235,-0.088613512133081,
71.7696736944791));
#143718=CARTESIAN_POINT('Ctrl Pts',(7.01124919374686,-0.00336239259829206,
71.7735343569104));
#143719=CARTESIAN_POINT('Ctrl Pts',(7.01124919374723,-0.0033623918231733,
71.7735343569455));
#143720=CARTESIAN_POINT('Ctrl Pts',(7.01133243824314,0.170218777619445,
71.7813951135351));
#143721=CARTESIAN_POINT('Ctrl Pts',(7.00496446246303,0.343967021436137,
71.7892558701247));
#143722=CARTESIAN_POINT('Ctrl Pts',(6.99213931214681,0.517314606435117,
71.7971166267143));
#143723=CARTESIAN_POINT('Ctrl Pts',(6.97984637489561,0.683468681241118,
71.8046511807055));
#143724=CARTESIAN_POINT('Ctrl Pts',(6.96162145167992,0.849254241414303,
71.8121857346967));
#143725=CARTESIAN_POINT('Ctrl Pts',(6.93751249916818,1.01417300614109,71.8197202886879));
#143726=CARTESIAN_POINT('Ctrl Pts',(6.91340523989911,1.17908018813785,71.8272543135052));
#143727=CARTESIAN_POINT('Ctrl Pts',(6.88341483877573,1.34312029690996,71.8347883383225));
#143728=CARTESIAN_POINT('Ctrl Pts',(6.84764077591688,1.50580289762654,71.8423223631399));
#143729=CARTESIAN_POINT('Ctrl Pts',(6.81185484725353,1.66853945810565,71.849858886898));
#143730=CARTESIAN_POINT('Ctrl Pts',(6.77028152667085,1.82991722015094,71.8573954106561));
#143731=CARTESIAN_POINT('Ctrl Pts',(6.72307070525294,1.98945893515542,71.8649319344142));
#143732=CARTESIAN_POINT('Ctrl Pts',(6.71694946583844,2.01014472296447,71.8659091016164));
#143733=CARTESIAN_POINT('Ctrl Pts',(6.71073352178202,2.03079966839776,71.8668862688185));
#143734=CARTESIAN_POINT('Ctrl Pts',(6.70442326004344,2.05142275328333,71.8678634360207));
#143735=CARTESIAN_POINT('Ctrl Pts',(6.66385193369962,2.18401723854725,71.8741460548872));
#143736=CARTESIAN_POINT('Ctrl Pts',(6.61938366189032,2.31528604824613,71.8804286737536));
#143737=CARTESIAN_POINT('Ctrl Pts',(6.57110895151816,2.44502632087631,71.8867112926201));
#143738=CARTESIAN_POINT('',(7.01124849188977,-0.00459863821984105,71.2264656430896));
#143739=CARTESIAN_POINT('Ctrl Pts',(6.57110895151817,2.44502632087629,71.3398522865014));
#143740=CARTESIAN_POINT('Ctrl Pts',(6.63771924680903,2.2660084085079,71.3311805125692));
#143741=CARTESIAN_POINT('Ctrl Pts',(6.69700989700479,2.08426710051935,71.3225087386371));
#143742=CARTESIAN_POINT('Ctrl Pts',(6.7487830778943,1.90040877971757,71.313836964705));
#143743=CARTESIAN_POINT('Ctrl Pts',(6.80055978789537,1.71653792623928,71.3051645996627));
#143744=CARTESIAN_POINT('Ctrl Pts',(6.84481792613578,1.53055004459431,71.2964922346203));
#143745=CARTESIAN_POINT('Ctrl Pts',(6.88140980451101,1.34306577086891,71.2878198695779));
#143746=CARTESIAN_POINT('Ctrl Pts',(6.91799949925382,1.15559268532947,71.2791480220618));
#143747=CARTESIAN_POINT('Ctrl Pts',(6.94692379517685,0.966623665171059,
71.2704761745457));
#143748=CARTESIAN_POINT('Ctrl Pts',(6.96808618426383,0.776789219268369,
71.2618043270296));
#143749=CARTESIAN_POINT('Ctrl Pts',(6.98924897510675,0.586951169466536,
71.2531323148834));
#143750=CARTESIAN_POINT('Ctrl Pts',(7.00264953276857,0.396247943319635,
71.2444603027372));
#143751=CARTESIAN_POINT('Ctrl Pts',(7.00824314361838,0.205315860142174,
71.235788290591));
#143752=CARTESIAN_POINT('Ctrl Pts',(7.01024757124657,0.136896809746581,
71.2326807414238));
#143753=CARTESIAN_POINT('Ctrl Pts',(7.01125,0.068448405292975,71.2295731922567));
#143754=CARTESIAN_POINT('Ctrl Pts',(7.01125,8.58630487052188E-16,71.2264656430895));
#143755=CARTESIAN_POINT('Ctrl Pts',(7.01124849188977,-0.00459863821984105,
71.2264656430896));
#143756=CARTESIAN_POINT('Ctrl Pts',(7.01110776524495,-0.219155519857082,
71.2167319929736));
#143757=CARTESIAN_POINT('Ctrl Pts',(7.00111426117045,-0.433432367386418,
71.2069983428576));
#143758=CARTESIAN_POINT('Ctrl Pts',(6.98136890923631,-0.646617905450055,
71.1972646927415));
#143759=CARTESIAN_POINT('Ctrl Pts',(6.96148781764589,-0.861268990025962,
71.1874641285322));
#143760=CARTESIAN_POINT('Ctrl Pts',(6.93172037097155,-1.07481368090438,
71.1776635643229));
#143761=CARTESIAN_POINT('Ctrl Pts',(6.89222048842957,-1.28643822291304,
71.1678630001136));
#143762=CARTESIAN_POINT('Ctrl Pts',(6.85264754105462,-1.49845421701776,
71.1580443073292));
#143763=CARTESIAN_POINT('Ctrl Pts',(6.80330615487526,-1.70854293642341,
71.1482256145448));
#143764=CARTESIAN_POINT('Ctrl Pts',(6.74440143903495,-1.9159007781311,71.1384069217604));
#143765=CARTESIAN_POINT('Ctrl Pts',(6.68553901871984,-2.1231097300819,71.1285952791206));
#143766=CARTESIAN_POINT('Ctrl Pts',(6.61712701506897,-2.32759170868229,
71.1187836364809));
#143767=CARTESIAN_POINT('Ctrl Pts',(6.5394198817576,-2.52855970318547,71.1089719938411));
#143768=CARTESIAN_POINT('Ctrl Pts',(6.47091931044857,-2.70571747302802,
71.1003228120008));
#143769=CARTESIAN_POINT('Ctrl Pts',(6.39519636928296,-2.88014479004352,
71.0916736301604));
#143770=CARTESIAN_POINT('Ctrl Pts',(6.31245749192088,-3.05131233655159,
71.0830244483201));
#143771=CARTESIAN_POINT('Ctrl Pts',(6.2356126311098,-3.21028652989516,71.0749914027212));
#143772=CARTESIAN_POINT('Ctrl Pts',(6.15267817287989,-3.366521933789,71.0669583571223));
#143773=CARTESIAN_POINT('Ctrl Pts',(6.06387990035083,-3.51951518204158,
71.0589253115234));
#143774=CARTESIAN_POINT('Ctrl Pts',(5.97513871077037,-3.67241008034347,
71.0508974298755));
#143775=CARTESIAN_POINT('Ctrl Pts',(5.88054139338673,-3.82206665590438,
71.0428695482276));
#143776=CARTESIAN_POINT('Ctrl Pts',(5.78036050395399,-3.96800441114029,
71.0348416665797));
#143777=CARTESIAN_POINT('Ctrl Pts',(5.68022484718038,-4.1138762740411,71.0268174095995));
#143778=CARTESIAN_POINT('Ctrl Pts',(5.57451084506208,-4.25603235827843,
71.0187931526193));
#143779=CARTESIAN_POINT('Ctrl Pts',(5.46353534834988,-4.39401957890851,
71.0107688956392));
#143780=CARTESIAN_POINT('Ctrl Pts',(5.35257326970559,-4.53199011547815,
71.0027456088734));
#143781=CARTESIAN_POINT('Ctrl Pts',(5.23635118719689,-4.66579250212281,
70.9947223221076));
#143782=CARTESIAN_POINT('Ctrl Pts',(5.11522747004122,-4.79500516081429,
70.9866990353418));
#143783=CARTESIAN_POINT('Ctrl Pts',(4.9941136778938,-4.92420723168092,70.9786764060128));
#143784=CARTESIAN_POINT('Ctrl Pts',(4.86809930481864,-5.04882005897734,
70.9706537766838));
#143785=CARTESIAN_POINT('Ctrl Pts',(4.73758074165986,-5.16845772728709,
70.9626311473548));
#143786=CARTESIAN_POINT('Ctrl Pts',(4.60701311281319,-5.2881403708429,70.9546055020883));
#143787=CARTESIAN_POINT('Ctrl Pts',(4.4719381837576,-5.40284387351634,70.9465798568218));
#143788=CARTESIAN_POINT('Ctrl Pts',(4.33278697616236,-5.51222129288165,
70.9385542115554));
#143789=CARTESIAN_POINT('Ctrl Pts',(4.25073494471767,-5.57671688446291,
70.9338218020481));
#143790=CARTESIAN_POINT('Ctrl Pts',(4.16726621785939,-5.63936136102783,
70.9290893925408));
#143791=CARTESIAN_POINT('Ctrl Pts',(4.08247411608701,-5.70009049524476,
70.9243569830336));
#143792=CARTESIAN_POINT('Ctrl Pts',(3.92605502595589,-5.81211974938641,
70.9156269341991));
#143793=CARTESIAN_POINT('Ctrl Pts',(3.76505279120063,-5.91768488094815,
70.9068968853646));
#143794=CARTESIAN_POINT('Ctrl Pts',(3.60001325395888,-6.01643840937647,
70.8981668365301));
#143795=CARTESIAN_POINT('Ctrl Pts',(3.43492599532925,-6.1152204925106,70.8894342633911));
#143796=CARTESIAN_POINT('Ctrl Pts',(3.26579933911061,-6.20718690045705,
70.8807016902521));
#143797=CARTESIAN_POINT('Ctrl Pts',(3.09320522068632,-6.29203528480403,
70.8719691171131));
#143798=CARTESIAN_POINT('Ctrl Pts',(2.91815912729324,-6.37808907589638,
70.8631124838326));
#143799=CARTESIAN_POINT('Ctrl Pts',(2.73954655925391,-6.45682092833281,
70.8542558505521));
#143800=CARTESIAN_POINT('Ctrl Pts',(2.55798720585462,-6.52796507475217,
70.8453992172716));
#143801=CARTESIAN_POINT('Ctrl Pts',(2.37885710472599,-6.59815731714677,
70.836661085165));
#143802=CARTESIAN_POINT('Ctrl Pts',(2.19685885117257,-6.66096355879762,
70.8279229530584));
#143803=CARTESIAN_POINT('Ctrl Pts',(2.01260584970456,-6.71617780111836,
70.8191848209518));
#143804=CARTESIAN_POINT('Ctrl Pts',(1.82460475939467,-6.77251521583741,
70.8102689370844));
#143805=CARTESIAN_POINT('Ctrl Pts',(1.63425648872507,-6.82094836000331,
70.801353053217));
#143806=CARTESIAN_POINT('Ctrl Pts',(1.4422278526844,-6.86131222022736,70.7924371693495));
#143807=CARTESIAN_POINT('Ctrl Pts',(1.25019921664367,-6.90167608045143,
70.7835212854821));
#143808=CARTESIAN_POINT('Ctrl Pts',(1.05649051242816,-6.93397060047979,
70.7746054016147));
#143809=CARTESIAN_POINT('Ctrl Pts',(0.861779521941969,-6.95808613183694,
70.7656895177473));
#143810=CARTESIAN_POINT('Ctrl Pts',(0.670894651622895,-6.98172778690884,
70.7569488332509));
#143811=CARTESIAN_POINT('Ctrl Pts',(0.479026245871978,-6.99751141897496,
70.7482081487545));
#143812=CARTESIAN_POINT('Ctrl Pts',(0.286818775441527,-7.00538089989076,
70.7394674642582));
#143813=CARTESIAN_POINT('Ctrl Pts',(0.0946458863275725,-7.01324896495623,
70.7307283523562));
#143814=CARTESIAN_POINT('Ctrl Pts',(-0.0978656721700958,-7.01320571128641,
70.7219892404541));
#143815=CARTESIAN_POINT('Ctrl Pts',(-0.290069043990111,-7.00524707003391,
70.7132501285521));
#143816=CARTESIAN_POINT('Ctrl Pts',(-0.484762687116275,-6.9971853131297,
70.7043977888778));
#143817=CARTESIAN_POINT('Ctrl Pts',(-0.679139816189818,-6.98100161767388,
70.6955454492035));
#143818=CARTESIAN_POINT('Ctrl Pts',(-0.872529556747008,-6.95674627502706,
70.6866931095292));
#143819=CARTESIAN_POINT('Ctrl Pts',(-1.06334784933147,-6.9328134487221,
70.6779584768794));
#143820=CARTESIAN_POINT('Ctrl Pts',(-1.25320457133843,-6.90102234370466,
70.6692238442294));
#143821=CARTESIAN_POINT('Ctrl Pts',(-1.44146079355278,-6.86147340905364,
70.6604892115796));
#143822=CARTESIAN_POINT('Ctrl Pts',(-1.63352239842513,-6.82112503824964,
70.6515780183931));
#143823=CARTESIAN_POINT('Ctrl Pts',(-1.82391782122646,-6.77270190480472,
70.6426668252066));
#143824=CARTESIAN_POINT('Ctrl Pts',(-2.0119789093691,-6.71636564153218,
70.6337556320201));
#143825=CARTESIAN_POINT('Ctrl Pts',(-2.20003999751181,-6.66002937825962,
70.6248444388336));
#143826=CARTESIAN_POINT('Ctrl Pts',(-2.38576645674874,-6.59578005923957,
70.6159332456472));
#143827=CARTESIAN_POINT('Ctrl Pts',(-2.56850496940922,-6.52383390228631,
70.6070220524607));
#143828=CARTESIAN_POINT('Ctrl Pts',(-2.73308428303562,-6.45903722118699,
70.5989963876084));
#143829=CARTESIAN_POINT('Ctrl Pts',(-2.89531542892063,-6.38796714380799,
70.5909707227561));
#143830=CARTESIAN_POINT('Ctrl Pts',(-3.05468423894261,-6.31082647225034,
70.5829450579037));
#143831=CARTESIAN_POINT('Ctrl Pts',(-3.21400246921343,-6.23371028324966,
70.5749219402006));
#143832=CARTESIAN_POINT('Ctrl Pts',(-3.37045984267261,-6.15052749538354,
70.5668988224974));
#143833=CARTESIAN_POINT('Ctrl Pts',(-3.52356324438916,-6.06152857167973,
70.5588757047943));
#143834=CARTESIAN_POINT('Ctrl Pts',(-3.67664733842679,-5.97254087151913,
70.5508535988765));
#143835=CARTESIAN_POINT('Ctrl Pts',(-3.8263779866911,-5.87773868118234,
70.5428314929587));
#143836=CARTESIAN_POINT('Ctrl Pts',(-3.97228775771086,-5.77741780836737,
70.5348093870409));
#143837=CARTESIAN_POINT('Ctrl Pts',(-4.11825174929443,-5.67705965597716,
70.5267843000814));
#143838=CARTESIAN_POINT('Ctrl Pts',(-4.26039172317582,-5.57117892974228,
70.518759213122));
#143839=CARTESIAN_POINT('Ctrl Pts',(-4.39826990370491,-5.46011432267344,
70.5107341261625));
#143840=CARTESIAN_POINT('Ctrl Pts',(-4.53617523865164,-5.34902784198606,
70.5027074587024));
#143841=CARTESIAN_POINT('Ctrl Pts',(-4.66981682820477,-5.23275568339619,
70.4946807912422));
#143842=CARTESIAN_POINT('Ctrl Pts',(-4.79879112613414,-5.11167587883233,
70.486654123782));
#143843=CARTESIAN_POINT('Ctrl Pts',(-4.92786896417546,-4.99049887182797,
70.4786210125415));
#143844=CARTESIAN_POINT('Ctrl Pts',(-5.05227176628368,-4.86450676796228,
70.470587901301));
#143845=CARTESIAN_POINT('Ctrl Pts',(-5.17163347091825,-4.73411383523655,
70.4625547900605));
#143846=CARTESIAN_POINT('Ctrl Pts',(-5.24196572334579,-4.65728158248588,
70.4578213890985));
#143847=CARTESIAN_POINT('Ctrl Pts',(-5.31054845581264,-4.57892201253535,
70.4530879881364));
#143848=CARTESIAN_POINT('Ctrl Pts',(-5.37731352235196,-4.49912500880236,
70.4483545871744));
#143849=CARTESIAN_POINT('Ctrl Pts',(-5.51485163727971,-4.33474069767678,
70.4386036338801));
#143850=CARTESIAN_POINT('Ctrl Pts',(-5.64475541595421,-4.16415819944512,
70.4288526805858));
#143851=CARTESIAN_POINT('Ctrl Pts',(-5.76655261146557,-3.98804432544318,
70.4191017272915));
#143852=CARTESIAN_POINT('Ctrl Pts',(-5.88852527868578,-3.81167672636744,
70.4093367259198));
#143853=CARTESIAN_POINT('Ctrl Pts',(-6.00236797922327,-3.62976184298234,
70.3995717245481));
#143854=CARTESIAN_POINT('Ctrl Pts',(-6.10765108553284,-3.44299648270072,
70.3898067231763));
#143855=CARTESIAN_POINT('Ctrl Pts',(-6.21275870671831,-3.25654242157788,
70.3800579980386));
#143856=CARTESIAN_POINT('Ctrl Pts',(-6.30933522913878,-3.06525407469387,
70.3703092729009));
#143857=CARTESIAN_POINT('Ctrl Pts',(-6.39699779057307,-2.8698511860205,
70.3605605477632));
#143858=CARTESIAN_POINT('Ctrl Pts',(-6.48441975226722,-2.67498460250943,
70.3508385790959));
#143859=CARTESIAN_POINT('Ctrl Pts',(-6.56297657773471,-2.47602605791691,
70.3411166104286));
#143860=CARTESIAN_POINT('Ctrl Pts',(-6.63233334959338,-2.27371522015654,
70.3313946417614));
#143861=CARTESIAN_POINT('Ctrl Pts',(-6.70123120580752,-2.07274302036933,
70.3217370008216));
#143862=CARTESIAN_POINT('Ctrl Pts',(-6.76105031225179,-1.86846277806501,
70.3120793598817));
#143863=CARTESIAN_POINT('Ctrl Pts',(-6.8115071862928,-1.66162463076999,
70.3024217189419));
#143864=CARTESIAN_POINT('Ctrl Pts',(-6.83368471955457,-1.570712144045,70.2981768532572));
#143865=CARTESIAN_POINT('Ctrl Pts',(-6.85405414701907,-1.47930581811492,
70.2939319875726));
#143866=CARTESIAN_POINT('Ctrl Pts',(-6.87259420767557,-1.38747087145073,
70.2896871218879));
#143867=CARTESIAN_POINT('Ctrl Pts',(-6.90688827743327,-1.21760119704961,
70.281835274874));
#143868=CARTESIAN_POINT('Ctrl Pts',(-6.9349053693729,-1.04633401805478,
70.2739834278602));
#143869=CARTESIAN_POINT('Ctrl Pts',(-6.95653755564075,-0.874192083846496,
70.2661315808463));
#143870=CARTESIAN_POINT('Ctrl Pts',(-6.97816360719546,-0.702098967699072,
70.2582819605528));
#143871=CARTESIAN_POINT('Ctrl Pts',(-6.99340830736989,-0.529131967912636,
70.2504323402592));
#143872=CARTESIAN_POINT('Ctrl Pts',(-7.00221515756051,-0.35582221646467,
70.2425827199657));
#143873=CARTESIAN_POINT('Ctrl Pts',(-7.01102130463679,-0.182526301583597,
70.2347337263639));
#143874=CARTESIAN_POINT('Ctrl Pts',(-7.01339060631139,-0.0088880705264088,
70.2268847327622));
#143875=CARTESIAN_POINT('Ctrl Pts',(-7.00931859181253,0.164558320881367,
70.2190357391604));
#143876=CARTESIAN_POINT('Ctrl Pts',(-7.00524451577196,0.33809252311822,
70.2111827718431));
#143877=CARTESIAN_POINT('Ctrl Pts',(-6.99472261678196,0.511434309793231,
70.2033298045257));
#143878=CARTESIAN_POINT('Ctrl Pts',(-6.97780054194339,0.684051284155319,
70.1954768372083));
#143879=CARTESIAN_POINT('Ctrl Pts',(-6.9608741694664,0.856712097428874,
70.1876218755011));
#143880=CARTESIAN_POINT('Ctrl Pts',(-6.93754443420151,1.02864735361808,
70.1797669137939));
#143881=CARTESIAN_POINT('Ctrl Pts',(-6.90791054361484,1.19933251599168,
70.1719119520867));
#143882=CARTESIAN_POINT('Ctrl Pts',(-6.87824723891469,1.3701870976564,70.1640491936734));
#143883=CARTESIAN_POINT('Ctrl Pts',(-6.84226736039791,1.53978873426941,
70.1561864352601));
#143884=CARTESIAN_POINT('Ctrl Pts',(-6.80012078706763,1.70762520588995,
70.1483236768468));
#143885=CARTESIAN_POINT('Ctrl Pts',(-6.76920266563841,1.8307476331666,70.1425556700984));
#143886=CARTESIAN_POINT('Ctrl Pts',(-6.73496700950947,1.95292040784015,
70.13678766335));
#143887=CARTESIAN_POINT('Ctrl Pts',(-6.69748962124314,2.07394776593829,
70.1310196566016));
#143888=CARTESIAN_POINT('Ctrl Pts',(-6.64305347672589,2.24974077235465,
70.1226415901605));
#143889=CARTESIAN_POINT('Ctrl Pts',(-6.58165583125923,2.42350599110936,
70.1142635237195));
#143890=CARTESIAN_POINT('Ctrl Pts',(-6.5134697150402,2.59467509213661,70.1058854572784));
#143891=CARTESIAN_POINT('Ctrl Pts',(-6.44533022367726,2.76572714976642,
70.0975131196597));
#143892=CARTESIAN_POINT('Ctrl Pts',(-6.3704116373528,2.93418632446898,70.0891407820409));
#143893=CARTESIAN_POINT('Ctrl Pts',(-6.28893622386487,3.09950120739777,
70.0807684444221));
#143894=CARTESIAN_POINT('Ctrl Pts',(-6.20750457387338,3.26472729351068,
70.0724006038995));
#143895=CARTESIAN_POINT('Ctrl Pts',(-6.11952326408433,3.42681216119099,
70.0640327633769));
#143896=CARTESIAN_POINT('Ctrl Pts',(-6.02526210732681,3.5852256693982,70.0556649228543));
#143897=CARTESIAN_POINT('Ctrl Pts',(-5.93103777319206,3.74357729420554,
70.0473003511843));
#143898=CARTESIAN_POINT('Ctrl Pts',(-5.83053865193824,3.89826013746391,
70.0389357795144));
#143899=CARTESIAN_POINT('Ctrl Pts',(-5.72408002124428,4.04876950108204,
70.0305712078444));
#143900=CARTESIAN_POINT('Ctrl Pts',(-5.61764739507809,4.19924209995032,
70.0222086793788));
#143901=CARTESIAN_POINT('Ctrl Pts',(-5.50525835252381,4.34554298435232,
70.0138461509132));
#143902=CARTESIAN_POINT('Ctrl Pts',(-5.3872711856394,4.48719686829979,70.0054836224476));
#143903=CARTESIAN_POINT('Ctrl Pts',(-5.26927460300992,4.62886205667041,
69.9971204266261));
#143904=CARTESIAN_POINT('Ctrl Pts',(-5.14567920921771,4.76587924728211,
69.9887572308046));
#143905=CARTESIAN_POINT('Ctrl Pts',(-5.01688372631032,4.89780606385988,
69.980394034983));
#143906=CARTESIAN_POINT('Ctrl Pts',(-4.88807945980912,5.02974187758216,
69.9720302688083));
#143907=CARTESIAN_POINT('Ctrl Pts',(-4.75407462659041,5.15658638960114,
69.9636665026336));
#143908=CARTESIAN_POINT('Ctrl Pts',(-4.61530508773046,5.27793382960315,
69.9553027364589));
#143909=CARTESIAN_POINT('Ctrl Pts',(-4.4765075838224,5.39930572372546,69.9469372848053));
#143910=CARTESIAN_POINT('Ctrl Pts',(-4.33294370714164,5.51517812047347,
69.9385718331517));
#143911=CARTESIAN_POINT('Ctrl Pts',(-4.18508301290906,5.62518504029513,
69.9302063814981));
#143912=CARTESIAN_POINT('Ctrl Pts',(-4.03717280042067,5.73522880121796,
69.9218381282712));
#143913=CARTESIAN_POINT('Ctrl Pts',(-3.88496316466333,5.8394029720958,69.9134698750443));
#143914=CARTESIAN_POINT('Ctrl Pts',(-3.7289536328293,5.9373842192256,69.9051016218174));
#143915=CARTESIAN_POINT('Ctrl Pts',(-3.5727994579021,6.03545630895002,69.8967256100259));
#143916=CARTESIAN_POINT('Ctrl Pts',(-3.41283862551568,6.12732382620423,
69.8883495982344));
#143917=CARTESIAN_POINT('Ctrl Pts',(-3.24959739565233,6.21270821209798,
69.8799735864429));
#143918=CARTESIAN_POINT('Ctrl Pts',(-3.08627611027292,6.29813447154954,
69.8715934669517));
#143919=CARTESIAN_POINT('Ctrl Pts',(-2.91967151344542,6.37707111279513,
69.8632133474606));
#143920=CARTESIAN_POINT('Ctrl Pts',(-2.75033154337589,6.44928701206665,
69.8548332279694));
#143921=CARTESIAN_POINT('Ctrl Pts',(-2.58079808093965,6.52158542715094,
69.8464435331302));
#143922=CARTESIAN_POINT('Ctrl Pts',(-2.4085233048815,6.58714763243901,69.8380538382909));
#143923=CARTESIAN_POINT('Ctrl Pts',(-2.23407333606647,6.64579136684088,
69.8296641434517));
#143924=CARTESIAN_POINT('Ctrl Pts',(-2.12331806130904,6.68302326181112,
69.8243376709773));
#143925=CARTESIAN_POINT('Ctrl Pts',(-2.0116863307701,6.71746748972255,69.8190111985029));
#143926=CARTESIAN_POINT('Ctrl Pts',(-1.89932553437109,6.74908801816853,
69.8136847260286));
#143927=CARTESIAN_POINT('Ctrl Pts',(-1.72252379684623,6.79884348938155,
69.8053034256237));
#143928=CARTESIAN_POINT('Ctrl Pts',(-1.54355969267545,6.84170545877321,
69.7969221252188));
#143929=CARTESIAN_POINT('Ctrl Pts',(-1.36299661902977,6.87748986033519,
69.788540824814));
#143930=CARTESIAN_POINT('Ctrl Pts',(-1.18266238264729,6.91322891040668,
69.7801701464804));
#143931=CARTESIAN_POINT('Ctrl Pts',(-1.00073353410874,6.94190820531124,
69.7717994681469));
#143932=CARTESIAN_POINT('Ctrl Pts',(-0.817788303417419,6.96339348689227,
69.7634287898134));
#143933=CARTESIAN_POINT('Ctrl Pts',(-0.635050684152917,6.98485438636753,
69.7550676107626));
#143934=CARTESIAN_POINT('Ctrl Pts',(-0.451299305063117,6.99913750622476,
69.7467064317118));
#143935=CARTESIAN_POINT('Ctrl Pts',(-0.267122700122726,7.00615957751314,
69.738345252661));
#143936=CARTESIAN_POINT('Ctrl Pts',(-0.083185086052544,7.01317253683572,
69.7299949232263));
#143937=CARTESIAN_POINT('Ctrl Pts',(0.101176327415832,7.01294322847672,
69.7216445937916));
#143938=CARTESIAN_POINT('Ctrl Pts',(0.285367848509045,7.00544015416143,
69.7132942643569));
#143939=CARTESIAN_POINT('Ctrl Pts',(0.469417645245128,6.99794285301299,
69.7049503600011));
#143940=CARTESIAN_POINT('Ctrl Pts',(0.653297484122077,6.98318295244684,
69.6966064556454));
#143941=CARTESIAN_POINT('Ctrl Pts',(0.836412478332128,6.96118098662794,
69.6882625512897));
#143942=CARTESIAN_POINT('Ctrl Pts',(1.01938039343656,6.93919669292523,69.67992534881));
#143943=CARTESIAN_POINT('Ctrl Pts',(1.20158436469483,6.90998197386602,69.6715881463303));
#143944=CARTESIAN_POINT('Ctrl Pts',(1.38243328120704,6.87360929828799,69.6632509438506));
#143945=CARTESIAN_POINT('Ctrl Pts',(1.44196774626208,6.8616356142598,69.6605063828145));
#143946=CARTESIAN_POINT('Ctrl Pts',(1.50135540542364,6.84888664744526,69.6577618217784));
#143947=CARTESIAN_POINT('Ctrl Pts',(1.56057531963105,6.83536621069116,69.6550172607423));
#143948=CARTESIAN_POINT('Ctrl Pts',(1.74049262305989,6.79428947907926,69.6466789504403));
#143949=CARTESIAN_POINT('Ctrl Pts',(1.91871320861347,6.74612185920721,69.6383406401384));
#143950=CARTESIAN_POINT('Ctrl Pts',(2.09466711578936,6.69103850209597,69.6300023298365));
#143951=CARTESIAN_POINT('Ctrl Pts',(2.27073172719304,6.63592048840557,69.6216587733527));
#143952=CARTESIAN_POINT('Ctrl Pts',(2.44452650296482,6.57387815645998,69.6133152168689));
#143953=CARTESIAN_POINT('Ctrl Pts',(2.61549942395125,6.50513561163875,69.604971660385));
#143954=CARTESIAN_POINT('Ctrl Pts',(2.78660242039094,6.43634076778897,69.5966217561598));
#143955=CARTESIAN_POINT('Ctrl Pts',(2.95487897611539,6.36083566531887,69.5882718519346));
#143956=CARTESIAN_POINT('Ctrl Pts',(3.1197993199902,6.27889152362809,69.5799219477093));
#143957=CARTESIAN_POINT('Ctrl Pts',(3.28496703217679,6.19682447178861,69.5715595192457));
#143958=CARTESIAN_POINT('Ctrl Pts',(3.44676817917903,6.10829922676386,69.563197090782));
#143959=CARTESIAN_POINT('Ctrl Pts',(3.6046984487669,6.0136324842775,69.5548346623183));
#143960=CARTESIAN_POINT('Ctrl Pts',(3.76276377026411,5.91888478882146,69.5464650828383));
#143961=CARTESIAN_POINT('Ctrl Pts',(3.91695133627263,5.8179852961546,69.5380955033583));
#143962=CARTESIAN_POINT('Ctrl Pts',(4.06678741139398,5.7112929108064,69.5297259238783));
#143963=CARTESIAN_POINT('Ctrl Pts',(4.2168545904053,5.60443596545312,69.5213434353418));
#143964=CARTESIAN_POINT('Ctrl Pts',(4.36255660796857,5.49176847300213,69.5129609468052));
#143965=CARTESIAN_POINT('Ctrl Pts',(4.50345319324468,5.37368922610476,69.5045784582686));
#143966=CARTESIAN_POINT('Ctrl Pts',(4.54955686467315,5.33505176167785,69.5018355706643));
#143967=CARTESIAN_POINT('Ctrl Pts',(4.59514631446448,5.29583514689353,69.49909268306));
#143968=CARTESIAN_POINT('Ctrl Pts',(4.64020700827323,5.25605417427104,69.4963497954557));
#143969=CARTESIAN_POINT('Ctrl Pts',(4.77570749191783,5.13643016108832,69.4881017511947));
#143970=CARTESIAN_POINT('Ctrl Pts',(4.9067250793169,5.01143441045634,69.4798537069337));
#143971=CARTESIAN_POINT('Ctrl Pts',(5.03281608802424,4.88143306689997,69.4716056626726));
#143972=CARTESIAN_POINT('Ctrl Pts',(5.15879061092155,4.75155182161201,69.463365238147));
#143973=CARTESIAN_POINT('Ctrl Pts',(5.2798473828122,4.61667444192376,69.4551248136213));
#143974=CARTESIAN_POINT('Ctrl Pts',(5.39557698681743,4.47720622060523,69.4468843890957));
#143975=CARTESIAN_POINT('Ctrl Pts',(5.51121869203085,4.33784392800091,69.4386502233261));
#143976=CARTESIAN_POINT('Ctrl Pts',(5.62154107133063,4.19389800584841,69.4304160575564));
#143977=CARTESIAN_POINT('Ctrl Pts',(5.72617252610861,4.04580953132238,69.4221818917868));
#143978=CARTESIAN_POINT('Ctrl Pts',(5.83073393570096,3.89782019414189,69.4139532383526));
#143979=CARTESIAN_POINT('Ctrl Pts',(5.9296118174176,3.74569411481522,69.4057245849184));
#143980=CARTESIAN_POINT('Ctrl Pts',(6.0224756756318,3.58990435790751,69.3974959314841));
#143981=CARTESIAN_POINT('Ctrl Pts',(6.11530333231547,3.43417533321306,69.3892704858625));
#143982=CARTESIAN_POINT('Ctrl Pts',(6.20212146096078,3.27478577326012,69.3810450402407));
#143983=CARTESIAN_POINT('Ctrl Pts',(6.28264339172886,3.11223690853792,69.3728195946191));
#143984=CARTESIAN_POINT('Ctrl Pts',(6.36314952543434,2.94971993319751,69.3645957626929));
#143985=CARTESIAN_POINT('Ctrl Pts',(6.43736176921313,2.78404519728397,69.3563719307667));
#143986=CARTESIAN_POINT('Ctrl Pts',(6.50503971704048,2.6157379154315,69.3481480988406));
#143987=CARTESIAN_POINT('Ctrl Pts',(6.52780435145871,2.55912488468372,69.3453818724208));
#143988=CARTESIAN_POINT('Ctrl Pts',(6.54983007321618,2.5022141828206,69.342615646001));
#143989=CARTESIAN_POINT('Ctrl Pts',(6.57110895151815,2.44502632087633,69.3398494195812));
#143990=CARTESIAN_POINT('Origin',(0.,0.,50.));
#143991=CARTESIAN_POINT('',(6.57110895151817,2.44502632087627,67.3401074818243));
#143992=CARTESIAN_POINT('',(6.57110895151815,2.44502632087632,67.8869083240903));
#143993=CARTESIAN_POINT('',(6.57110895151814,2.44502632087636,50.));
#143994=CARTESIAN_POINT('',(7.01124997488654,-0.000593425248588222,69.773534356871));
#143995=CARTESIAN_POINT('Ctrl Pts',(6.57110895151815,2.44502632087632,67.8869083240903));
#143996=CARTESIAN_POINT('Ctrl Pts',(6.53460574947235,2.543130179994,67.8916644840135));
#143997=CARTESIAN_POINT('Ctrl Pts',(6.49590744269728,2.64041041299079,67.8964206439368));
#143998=CARTESIAN_POINT('Ctrl Pts',(6.45505378653798,2.73676947794323,67.90117680386));
#143999=CARTESIAN_POINT('Ctrl Pts',(6.37997453672858,2.91385439491506,67.9099174883563));
#144000=CARTESIAN_POINT('Ctrl Pts',(6.29760020324618,3.0878574907195,67.9186581728526));
#144001=CARTESIAN_POINT('Ctrl Pts',(6.20820478069396,3.25819274498436,67.9273988573489));
#144002=CARTESIAN_POINT('Ctrl Pts',(6.11882544186321,3.42849735310753,67.9361379692509));
#144003=CARTESIAN_POINT('Ctrl Pts',(6.02242766387985,3.59513519522477,67.9448770811528));
#144004=CARTESIAN_POINT('Ctrl Pts',(5.91933170363533,3.75754424389623,67.9536161930548));
#144005=CARTESIAN_POINT('Ctrl Pts',(5.81489998684652,3.92205753553803,67.9624685327291));
#144006=CARTESIAN_POINT('Ctrl Pts',(5.70359544243341,4.08223143696591,67.9713208724034));
#144007=CARTESIAN_POINT('Ctrl Pts',(5.58579740979659,4.23751033735727,67.9801732120777));
#144008=CARTESIAN_POINT('Ctrl Pts',(5.46956570385057,4.39072453869758,67.9889078447276));
#144009=CARTESIAN_POINT('Ctrl Pts',(5.34701230226013,4.53917289001124,67.9976424773774));
#144010=CARTESIAN_POINT('Ctrl Pts',(5.21854397657135,4.68235254194842,68.0063771100272));
#144011=CARTESIAN_POINT('Ctrl Pts',(5.08747881167492,4.82842640560585,68.0152883032138));
#144012=CARTESIAN_POINT('Ctrl Pts',(4.95025722690546,4.96901606934448,68.0241994964003));
#144013=CARTESIAN_POINT('Ctrl Pts',(4.80735358883626,5.10362400989759,68.0331106895868));
#144014=CARTESIAN_POINT('Ctrl Pts',(4.66444995076705,5.23823195045071,68.0420218827733));
#144015=CARTESIAN_POINT('Ctrl Pts',(4.51586447081349,5.3668579501655,68.0509330759599));
#144016=CARTESIAN_POINT('Ctrl Pts',(4.3621113449029,5.48904465068098,68.0598442691464));
#144017=CARTESIAN_POINT('Ctrl Pts',(4.22363706511551,5.59908934247682,68.0678699339987));
#144018=CARTESIAN_POINT('Ctrl Pts',(4.08090719246255,5.7039610929444,68.075895598851));
#144019=CARTESIAN_POINT('Ctrl Pts',(3.93435465838549,5.80331629196104,68.0839212637033));
#144020=CARTESIAN_POINT('Ctrl Pts',(3.78784863648837,5.90263995807431,68.0919443814064));
#144021=CARTESIAN_POINT('Ctrl Pts',(3.63752267162726,5.99645035299509,68.0999674991095));
#144022=CARTESIAN_POINT('Ctrl Pts',(3.48384041783224,6.0844459489405,68.1079906168126));
#144023=CARTESIAN_POINT('Ctrl Pts',(3.33017754471416,6.17243044787129,68.1160127227304));
#144024=CARTESIAN_POINT('Ctrl Pts',(3.17315954406012,6.25460142688896,68.1240348286482));
#144025=CARTESIAN_POINT('Ctrl Pts',(3.01327646962929,6.330702289642,68.132056934566));
#144026=CARTESIAN_POINT('Ctrl Pts',(2.85333398210773,6.4068314317328,68.1400820215254));
#144027=CARTESIAN_POINT('Ctrl Pts',(2.69052462394261,6.47688579103166,68.1481071084848));
#144028=CARTESIAN_POINT('Ctrl Pts',(2.5253607311898,6.54065591052339,68.1561321954443));
#144029=CARTESIAN_POINT('Ctrl Pts',(2.36016431023493,6.604438589221,68.1641588629044));
#144030=CARTESIAN_POINT('Ctrl Pts',(2.19261277603009,6.6619344386964,68.1721855303646));
#144031=CARTESIAN_POINT('Ctrl Pts',(2.02323538748915,6.71298332556485,68.1802121978247));
#144032=CARTESIAN_POINT('Ctrl Pts',(1.85372202337752,6.76407319429979,68.1882453090652));
#144033=CARTESIAN_POINT('Ctrl Pts',(1.68238023097071,6.80870566659897,68.1962784203057));
#144034=CARTESIAN_POINT('Ctrl Pts',(1.5097518764689,6.84677119772515,68.2043115315462));
#144035=CARTESIAN_POINT('Ctrl Pts',(1.40803297891685,6.8692007914733,68.2090449325084));
#144036=CARTESIAN_POINT('Ctrl Pts',(1.30586757527244,6.88935131737869,68.2137783334706));
#144037=CARTESIAN_POINT('Ctrl Pts',(1.20336758864791,6.90720877121082,68.2185117344328));
#144038=CARTESIAN_POINT('Ctrl Pts',(0.992214426209671,6.94399568186245,
68.2282626877271));
#144039=CARTESIAN_POINT('Ctrl Pts',(0.779516735548898,6.97107099913281,
68.2380136410215));
#144040=CARTESIAN_POINT('Ctrl Pts',(0.566088162918322,6.98835966120117,
68.2477645943159));
#144041=CARTESIAN_POINT('Ctrl Pts',(0.352352106390719,7.00567323083052,
68.2575295956877));
#144042=CARTESIAN_POINT('Ctrl Pts',(0.137883100145668,7.01317193896387,
68.2672945970595));
#144043=CARTESIAN_POINT('Ctrl Pts',(-0.076500574440827,7.01083263418906,
68.2770595984314));
#144044=CARTESIAN_POINT('Ctrl Pts',(-0.290526915861115,7.0084972285506,
68.2868083235692));
#144045=CARTESIAN_POINT('Ctrl Pts',(-0.504468171976303,6.99635658321835,
68.296557048707));
#144046=CARTESIAN_POINT('Ctrl Pts',(-0.717509613025243,6.97443951280075,
68.3063057738448));
#144047=CARTESIAN_POINT('Ctrl Pts',(-0.9299663379256,6.95258259624307,68.3160277425122));
#144048=CARTESIAN_POINT('Ctrl Pts',(-1.14152813827517,6.92100282537907,
68.3257497111796));
#144049=CARTESIAN_POINT('Ctrl Pts',(-1.35138703438341,6.8797804940129,68.3354716798469));
#144050=CARTESIAN_POINT('Ctrl Pts',(-1.55985734898668,6.83883092004701,
68.3451293207868));
#144051=CARTESIAN_POINT('Ctrl Pts',(-1.76664716884618,6.78836594907956,
68.3547869617267));
#144052=CARTESIAN_POINT('Ctrl Pts',(-1.97096519591468,6.72851564306668,
68.3644446026666));
#144053=CARTESIAN_POINT('Ctrl Pts',(-2.06077000302823,6.7022093730606,68.3686894683508));
#144054=CARTESIAN_POINT('Ctrl Pts',(-2.15009729759262,6.67409061705496,
68.3729343340351));
#144055=CARTESIAN_POINT('Ctrl Pts',(-2.2388799771677,6.64417361380161,68.3771791997193));
#144056=CARTESIAN_POINT('Ctrl Pts',(-2.40310378761465,6.58883529449278,
68.3850310467332));
#144057=CARTESIAN_POINT('Ctrl Pts',(-2.56539553606999,6.52736341128697,
68.392882893747));
#144058=CARTESIAN_POINT('Ctrl Pts',(-2.7252486497801,6.45992618838418,68.4007347407609));
#144059=CARTESIAN_POINT('Ctrl Pts',(-2.88505643043961,6.39250809013256,
68.4085843610544));
#144060=CARTESIAN_POINT('Ctrl Pts',(-3.04242660089788,6.31912816543598,
68.416433981348));
#144061=CARTESIAN_POINT('Ctrl Pts',(-3.19687107404595,6.24000335724496,
68.4242836016415));
#144062=CARTESIAN_POINT('Ctrl Pts',(-3.35130321677823,6.16088486615784,
68.4321325952432));
#144063=CARTESIAN_POINT('Ctrl Pts',(-3.50280978803219,6.07602257923392,
68.439981588845));
#144064=CARTESIAN_POINT('Ctrl Pts',(-3.65092612509082,5.98567999408833,
68.4478305824467));
#144065=CARTESIAN_POINT('Ctrl Pts',(-3.79911744911363,5.89529167113739,
68.4556835497641));
#144066=CARTESIAN_POINT('Ctrl Pts',(-3.9439147834452,5.79941770524224,68.4635365170815));
#144067=CARTESIAN_POINT('Ctrl Pts',(-4.08488107546139,5.69836583257318,
68.4713894843988));
#144068=CARTESIAN_POINT('Ctrl Pts',(-4.22588316817927,5.59728829612382,
68.4792444461061));
#144069=CARTESIAN_POINT('Ctrl Pts',(-4.36305197862399,5.49103046672035,
68.4870994078133));
#144070=CARTESIAN_POINT('Ctrl Pts',(-4.49598306686708,5.37994078266151,
68.4949543695205));
#144071=CARTESIAN_POINT('Ctrl Pts',(-4.62904610032678,5.2687408328054,68.5028171279338));
#144072=CARTESIAN_POINT('Ctrl Pts',(-4.7578627272447,5.15269970462525,68.510679886347));
#144073=CARTESIAN_POINT('Ctrl Pts',(-4.88206453376931,5.03220353827346,
68.5185426447603));
#144074=CARTESIAN_POINT('Ctrl Pts',(-4.97317719685091,4.94380927965001,
68.5243106515088));
#144075=CARTESIAN_POINT('Ctrl Pts',(-5.061807165531,4.85301833476021,68.5300786582572));
#144076=CARTESIAN_POINT('Ctrl Pts',(-5.14782290711444,4.75999431506886,
68.5358466650056));
#144077=CARTESIAN_POINT('Ctrl Pts',(-5.27276131814438,4.62487633556995,
68.5442247314466));
#144078=CARTESIAN_POINT('Ctrl Pts',(-5.3924597185564,4.48474669896059,68.5526027978877));
#144079=CARTESIAN_POINT('Ctrl Pts',(-5.50651270748239,4.34003967318675,
68.5609808643287));
#144080=CARTESIAN_POINT('Ctrl Pts',(-5.6204877083297,4.19543159635777,68.5693532019474));
#144081=CARTESIAN_POINT('Ctrl Pts',(-5.72882479108253,4.04625262793844,
68.5777255395661));
#144082=CARTESIAN_POINT('Ctrl Pts',(-5.83115784931043,3.89297119163826,
68.5860978771849));
#144083=CARTESIAN_POINT('Ctrl Pts',(-5.93343594061958,3.7397720885391,68.5944657177075));
#144084=CARTESIAN_POINT('Ctrl Pts',(-6.02971625560652,3.5824751840913,68.60283355823));
#144085=CARTESIAN_POINT('Ctrl Pts',(-6.11967489796486,3.42157941683643,
68.6112013987526));
#144086=CARTESIAN_POINT('Ctrl Pts',(-6.20959839845501,3.2607465026627,68.6195659704225));
#144087=CARTESIAN_POINT('Ctrl Pts',(-6.29320499072813,3.09631781569016,
68.6279305420924));
#144088=CARTESIAN_POINT('Ctrl Pts',(-6.37021556185153,2.92881891861627,
68.6362951137623));
#144089=CARTESIAN_POINT('Ctrl Pts',(-6.44720732169097,2.76136093630604,
68.6446576422279));
#144090=CARTESIAN_POINT('Ctrl Pts',(-6.51760613671815,2.59083453803991,
68.6530201706935));
#144091=CARTESIAN_POINT('Ctrl Pts',(-6.58117988695038,2.41778780253763,
68.661382699159));
#144092=CARTESIAN_POINT('Ctrl Pts',(-6.6447587105668,2.24472725736442,68.6697458949806));
#144093=CARTESIAN_POINT('Ctrl Pts',(-6.70151126222094,2.06914627954993,
68.6781090908021));
#144094=CARTESIAN_POINT('Ctrl Pts',(-6.75125414920358,1.89161147579558,
68.6864722866236));
#144095=CARTESIAN_POINT('Ctrl Pts',(-6.80100042855138,1.71406456452352,
68.6948360527983));
#144096=CARTESIAN_POINT('Ctrl Pts',(-6.84373600107298,1.53456387818423,
68.7031998189729));
#144097=CARTESIAN_POINT('Ctrl Pts',(-6.87932775394974,1.35368985230621,
68.7115635851476));
#144098=CARTESIAN_POINT('Ctrl Pts',(-6.91492667933058,1.17277937641989,
68.7199290368012));
#144099=CARTESIAN_POINT('Ctrl Pts',(-6.94337885093542,0.99049533173565,
68.7282944884548));
#144100=CARTESIAN_POINT('Ctrl Pts',(-6.96460246864185,0.807427406203142,
68.7366599401083));
#144101=CARTESIAN_POINT('Ctrl Pts',(-6.98583319409612,0.624298171582286,
68.7450281933352));
#144102=CARTESIAN_POINT('Ctrl Pts',(-6.99983050060367,0.440384859106724,
68.753396446562));
#144103=CARTESIAN_POINT('Ctrl Pts',(-7.00656450931252,0.256281757724323,
68.7617646997889));
#144104=CARTESIAN_POINT('Ctrl Pts',(-7.01330476140815,0.0720079665017409,
68.7701407115804));
#144105=CARTESIAN_POINT('Ctrl Pts',(-7.01276824690758,-0.11245563634756,
68.7785167233719));
#144106=CARTESIAN_POINT('Ctrl Pts',(-7.00497722994805,-0.296514030712585,
68.7868927351633));
#144107=CARTESIAN_POINT('Ctrl Pts',(-6.99718239217753,-0.480662689588405,
68.7952728546545));
#144108=CARTESIAN_POINT('Ctrl Pts',(-6.98212597764238,-0.664405415692843,
68.8036529741456));
#144109=CARTESIAN_POINT('Ctrl Pts',(-6.95988216650146,-0.847152165147994,
68.8120330936368));
#144110=CARTESIAN_POINT('Ctrl Pts',(-6.93761293898861,-1.03010772591359,
68.820422788476));
#144111=CARTESIAN_POINT('Ctrl Pts',(-6.90813995078051,-1.21206471037406,
68.8288124833152));
#144112=CARTESIAN_POINT('Ctrl Pts',(-6.87158878422862,-1.39244179158893,
68.8372021781544));
#144113=CARTESIAN_POINT('Ctrl Pts',(-6.84838307933848,-1.50696008773349,
68.8425286506291));
#144114=CARTESIAN_POINT('Ctrl Pts',(-6.82232535479691,-1.62084179431044,
68.8478551231038));
#144115=CARTESIAN_POINT('Ctrl Pts',(-6.7934581919395,-1.73394127838003,
68.8531815955785));
#144116=CARTESIAN_POINT('Ctrl Pts',(-6.74803519108956,-1.91190535425393,
68.8615628959834));
#144117=CARTESIAN_POINT('Ctrl Pts',(-6.69556204792654,-2.08829092126212,
68.8699441963883));
#144118=CARTESIAN_POINT('Ctrl Pts',(-6.63616141893687,-2.26251810695821,
68.8783254967933));
#144119=CARTESIAN_POINT('Ctrl Pts',(-6.57683607154881,-2.4365244852015,
68.8866961751268));
#144120=CARTESIAN_POINT('Ctrl Pts',(-6.51060083998907,-2.60837762595666,
68.8950668534604));
#144121=CARTESIAN_POINT('Ctrl Pts',(-6.43762892445178,-2.7775097467987,
68.903437531794));
#144122=CARTESIAN_POINT('Ctrl Pts',(-6.36473981951007,-2.94644993172191,
68.9117987108449));
#144123=CARTESIAN_POINT('Ctrl Pts',(-6.28512939688618,-3.11267495222198,
68.9201598898957));
#144124=CARTESIAN_POINT('Ctrl Pts',(-6.19902015630381,-3.2756336279015,
68.9285210689466));
#144125=CARTESIAN_POINT('Ctrl Pts',(-6.11302265261846,-3.43838084547686,
68.9368713983813));
#144126=CARTESIAN_POINT('Ctrl Pts',(-6.02054330380782,-3.59786988397885,
68.9452217278161));
#144127=CARTESIAN_POINT('Ctrl Pts',(-5.92185200977182,-3.75357101129864,
68.9535720572508));
#144128=CARTESIAN_POINT('Ctrl Pts',(-5.82323665278288,-3.90915233591497,
68.9619159616066));
#144129=CARTESIAN_POINT('Ctrl Pts',(-5.71841905034829,-4.06095128199274,
68.9702598659623));
#144130=CARTESIAN_POINT('Ctrl Pts',(-5.60771474562165,-4.20846312734679,
68.9786037703181));
#144131=CARTESIAN_POINT('Ctrl Pts',(-5.49709935928305,-4.35585649026659,
68.9869409727978));
#144132=CARTESIAN_POINT('Ctrl Pts',(-5.38060689654618,-4.49896935858342,
68.9952781752776));
#144133=CARTESIAN_POINT('Ctrl Pts',(-5.25859597100946,-4.63732627450162,
69.0036153777573));
#144134=CARTESIAN_POINT('Ctrl Pts',(-5.21843064780921,-4.68287260750744,
69.0063599387932));
#144135=CARTESIAN_POINT('Ctrl Pts',(-5.17766763597248,-4.72790378649475,
69.0091044998292));
#144136=CARTESIAN_POINT('Ctrl Pts',(-5.1363207172274,-4.77240359276964,
69.0118490608651));
#144137=CARTESIAN_POINT('Ctrl Pts',(-5.01070374824256,-4.90759941761767,
69.020187371167));
#144138=CARTESIAN_POINT('Ctrl Pts',(-4.87979739535122,-5.0377770788816,
69.028525681469));
#144139=CARTESIAN_POINT('Ctrl Pts',(-4.7440385786251,-5.16253082576916,
69.0368639917709));
#144140=CARTESIAN_POINT('Ctrl Pts',(-4.60819434705807,-5.2873630634811,
69.0452075482548));
#144141=CARTESIAN_POINT('Ctrl Pts',(-4.46749180331283,-5.40676435837665,
69.0535511047386));
#144142=CARTESIAN_POINT('Ctrl Pts',(-4.32240126739949,-5.52036899546428,
69.0618946612225));
#144143=CARTESIAN_POINT('Ctrl Pts',(-4.17720034723872,-5.63406006246472,
69.0702445654477));
#144144=CARTESIAN_POINT('Ctrl Pts',(-4.02760503364756,-5.74194547323626,
69.078594469673));
#144145=CARTESIAN_POINT('Ctrl Pts',(-3.87411529769811,-5.84370235575371,
69.0869443738982));
#144146=CARTESIAN_POINT('Ctrl Pts',(-3.72039533850314,-5.94561186606483,
69.0953068023619));
#144147=CARTESIAN_POINT('Ctrl Pts',(-3.56276955743051,-6.04137429773488,
69.1036692308256));
#144148=CARTESIAN_POINT('Ctrl Pts',(-3.40176455165533,-6.13071158166825,
69.1120316592893));
#144149=CARTESIAN_POINT('Ctrl Pts',(-3.24062186465198,-6.22012526115785,
69.1204012387693));
#144150=CARTESIAN_POINT('Ctrl Pts',(-3.0760944791062,-6.30310268301348,
69.1287708182493));
#144151=CARTESIAN_POINT('Ctrl Pts',(-2.9087302278244,-6.37941337618442,
69.1371403977293));
#144152=CARTESIAN_POINT('Ctrl Pts',(-2.7411078375766,-6.4558417693019,69.1455228862659));
#144153=CARTESIAN_POINT('Ctrl Pts',(-2.57064014066444,-6.52558276217499,
69.1539053748025));
#144154=CARTESIAN_POINT('Ctrl Pts',(-2.39789275105042,-6.58845482013498,
69.1622878633391));
#144155=CARTESIAN_POINT('Ctrl Pts',(-2.34136697454129,-6.60902758771692,
69.1650307509432));
#144156=CARTESIAN_POINT('Ctrl Pts',(-2.28459721093394,-6.62886529793762,
69.1677736385473));
#144157=CARTESIAN_POINT('Ctrl Pts',(-2.22760354135047,-6.64796277253888,
69.1705165261514));
#144158=CARTESIAN_POINT('Ctrl Pts',(-2.05327316391249,-6.70637750490621,
69.1789063812842));
#144159=CARTESIAN_POINT('Ctrl Pts',(-1.87649502487395,-6.75798071670235,
69.1872962364169));
#144160=CARTESIAN_POINT('Ctrl Pts',(-1.6978281097713,-6.80257350362129,
69.1956860915497));
#144161=CARTESIAN_POINT('Ctrl Pts',(-1.51932606599329,-6.84712514094158,
69.2040682046418));
#144162=CARTESIAN_POINT('Ctrl Pts',(-1.33893903809474,-6.88467917035178,
69.2124503177338));
#144163=CARTESIAN_POINT('Ctrl Pts',(-1.15724183614579,-6.91508625363227,
69.2208324308259));
#144164=CARTESIAN_POINT('Ctrl Pts',(-0.975685592715808,-6.94546974746075,
69.2292080411748));
#144165=CARTESIAN_POINT('Ctrl Pts',(-0.792821524716646,-6.96871729517089,
69.2375836515236));
#144166=CARTESIAN_POINT('Ctrl Pts',(-0.609235770882665,-6.98473036974063,
69.2459592618725));
#144167=CARTESIAN_POINT('Ctrl Pts',(-0.425765495213908,-7.00073337184867,
69.2543296038381));
#144168=CARTESIAN_POINT('Ctrl Pts',(-0.241574765487565,-7.00951094579591,
69.2626999458037));
#144169=CARTESIAN_POINT('Ctrl Pts',(-0.0572564586363296,-7.01101620740135,
69.2710702877692));
#144170=CARTESIAN_POINT('Ctrl Pts',(0.126972928256298,-7.01252074282934,
69.2794365916636));
#144171=CARTESIAN_POINT('Ctrl Pts',(0.311329441413336,-7.00675995946025,
69.2878028955579));
#144172=CARTESIAN_POINT('Ctrl Pts',(0.495218112664075,-6.99373902740083,
69.2961691994522));
#144173=CARTESIAN_POINT('Ctrl Pts',(0.679055355407793,-6.98072173693113,
69.3045331635258));
#144174=CARTESIAN_POINT('Ctrl Pts',(0.86242468949627,-6.96044836823186,
69.3128971275994));
#144175=CARTESIAN_POINT('Ctrl Pts',(1.04473362047737,-6.93297614482729,
69.321261091673));
#144176=CARTESIAN_POINT('Ctrl Pts',(1.22701449714345,-6.90550814894139,
69.3296237686716));
#144177=CARTESIAN_POINT('Ctrl Pts',(1.40823497115293,-6.87084355600873,
69.3379864456701));
#144178=CARTESIAN_POINT('Ctrl Pts',(1.58780970526545,-6.82909122082616,
69.3463491226686));
#144179=CARTESIAN_POINT('Ctrl Pts',(1.76738074226206,-6.78733974524793,
69.3547116274949));
#144180=CARTESIAN_POINT('Ctrl Pts',(1.94530578690506,-6.7385008932111,69.3630741323212));
#144181=CARTESIAN_POINT('Ctrl Pts',(2.12101127108758,-6.68273430194703,
69.3714366371475));
#144182=CARTESIAN_POINT('Ctrl Pts',(2.29673655810607,-6.62696142552537,
69.3798000844674));
#144183=CARTESIAN_POINT('Ctrl Pts',(2.47024147285186,-6.56425935313681,
69.3881635317874));
#144184=CARTESIAN_POINT('Ctrl Pts',(2.64096873085647,-6.49483723623144,
69.3965269791074));
#144185=CARTESIAN_POINT('Ctrl Pts',(2.81179651786845,-6.42537424163269,
69.4048953510602));
#144186=CARTESIAN_POINT('Ctrl Pts',(2.97984307476608,-6.34918341862338,
69.413263723013));
#144187=CARTESIAN_POINT('Ctrl Pts',(3.14457123150028,-6.26652202840785,
69.4216320949658));
#144188=CARTESIAN_POINT('Ctrl Pts',(3.30934874509559,-6.18383587067936,
69.4300029743015));
#144189=CARTESIAN_POINT('Ctrl Pts',(3.47080558452627,-6.09467543208481,
69.4383738536373));
#144190=CARTESIAN_POINT('Ctrl Pts',(3.62842960467726,-5.99934372797572,
69.446744732973));
#144191=CARTESIAN_POINT('Ctrl Pts',(3.78618717795604,-5.90393125034462,
69.4551227048643));
#144192=CARTESIAN_POINT('Ctrl Pts',(3.94010516419902,-5.80233723385321,
69.4635006767556));
#144193=CARTESIAN_POINT('Ctrl Pts',(4.08969983616813,-5.69490841125179,
69.4718786486469));
#144194=CARTESIAN_POINT('Ctrl Pts',(4.18476846836167,-5.62663651969011,
69.477202918006));
#144195=CARTESIAN_POINT('Ctrl Pts',(4.2780916519057,-5.55600897634522,69.4825271873652));
#144196=CARTESIAN_POINT('Ctrl Pts',(4.36955219335629,-5.48312321510608,
69.4878514567244));
#144197=CARTESIAN_POINT('Ctrl Pts',(4.50462026549706,-5.37548620464293,
69.4957142879136));
#144198=CARTESIAN_POINT('Ctrl Pts',(4.63590515167311,-5.26269828661825,
69.5035771191028));
#144199=CARTESIAN_POINT('Ctrl Pts',(4.76297282760539,-5.14506719159164,
69.5114399502921));
#144200=CARTESIAN_POINT('Ctrl Pts',(4.88994286880163,-5.02752648053427,
69.5192967399334));
#144201=CARTESIAN_POINT('Ctrl Pts',(5.0127018657146,-4.90515025023536,69.5271535295747));
#144202=CARTESIAN_POINT('Ctrl Pts',(5.13084717804576,-4.77828774751373,
69.5350103192161));
#144203=CARTESIAN_POINT('Ctrl Pts',(5.24892586201304,-4.65149678923875,
69.542862678));
#144204=CARTESIAN_POINT('Ctrl Pts',(5.36239577814006,-4.52022486952671,
69.5507150367839));
#144205=CARTESIAN_POINT('Ctrl Pts',(5.47088981512386,-4.38485931282567,
69.5585673955677));
#144206=CARTESIAN_POINT('Ctrl Pts',(5.57935823539993,-4.24952571751164,
69.5664179003181));
#144207=CARTESIAN_POINT('Ctrl Pts',(5.68285287002074,-4.11010070088217,
69.5742684050685));
#144208=CARTESIAN_POINT('Ctrl Pts',(5.78104577593687,-3.96700596155621,
69.5821189098188));
#144209=CARTESIAN_POINT('Ctrl Pts',(5.87922288570915,-3.82393424166394,
69.5899681516704));
#144210=CARTESIAN_POINT('Ctrl Pts',(5.97209975122079,-3.67719429056144,
69.597817393522));
#144211=CARTESIAN_POINT('Ctrl Pts',(6.05939107001222,-3.52723778942619,
69.6056666353736));
#144212=CARTESIAN_POINT('Ctrl Pts',(6.14671179895765,-3.37723076501036,
69.6135185217884));
#144213=CARTESIAN_POINT('Ctrl Pts',(6.2284430301337,-3.22400535592021,69.6213704082032));
#144214=CARTESIAN_POINT('Ctrl Pts',(6.30434475481217,-3.06803907650673,
69.629222294618));
#144215=CARTESIAN_POINT('Ctrl Pts',(6.36007844651651,-2.9535149788011,69.6349878370822));
#144216=CARTESIAN_POINT('Ctrl Pts',(6.41266993518779,-2.83751361474837,
69.6407533795464));
#144217=CARTESIAN_POINT('Ctrl Pts',(6.4620406373389,-2.72023112324682,69.6465189220106));
#144218=CARTESIAN_POINT('Ctrl Pts',(6.54286855733576,-2.52822048886078,
69.6559580586793));
#144219=CARTESIAN_POINT('Ctrl Pts',(6.61503119340741,-2.33285131357872,
69.665397195348));
#144220=CARTESIAN_POINT('Ctrl Pts',(6.67832305966802,-2.13486010623796,
69.6748363320168));
#144221=CARTESIAN_POINT('Ctrl Pts',(6.74199387910535,-1.93568344804203,
69.6843319844914));
#144222=CARTESIAN_POINT('Ctrl Pts',(6.79668738743301,-1.73385338414025,
69.6938276369659));
#144223=CARTESIAN_POINT('Ctrl Pts',(6.84224674383686,-1.53012615785559,
69.7033232894405));
#144224=CARTESIAN_POINT('Ctrl Pts',(6.88791457833146,-1.32591385139671,
69.7128415513269));
#144225=CARTESIAN_POINT('Ctrl Pts',(6.9244047295736,-1.11979545018396,69.7223598132133));
#144226=CARTESIAN_POINT('Ctrl Pts',(6.95161148449768,-0.912537303949778,
69.7318780750997));
#144227=CARTESIAN_POINT('Ctrl Pts',(6.97886808837653,-0.704899413715052,
69.7414137766039));
#144228=CARTESIAN_POINT('Ctrl Pts',(6.99680725098884,-0.49611770472743,
69.7509494781081));
#144229=CARTESIAN_POINT('Ctrl Pts',(7.00537487861924,-0.286965803730128,
69.7604851796122));
#144230=CARTESIAN_POINT('Ctrl Pts',(7.00928301589988,-0.191560823861168,
69.7648349053651));
#144231=CARTESIAN_POINT('Ctrl Pts',(7.01124189309494,-0.0960788486770531,
69.7691846311181));
#144232=CARTESIAN_POINT('Ctrl Pts',(7.01124997488654,-0.00059342524868163,
69.773534356871));
#144233=CARTESIAN_POINT('Ctrl Pts',(7.01124997488661,-0.000593424381606831,
69.7735343569105));
#144234=CARTESIAN_POINT('Ctrl Pts',(7.01126957801824,0.231015623752868,
69.784085033706));
#144235=CARTESIAN_POINT('Ctrl Pts',(6.99981027861164,0.462672585231173,
69.7946357105016));
#144236=CARTESIAN_POINT('Ctrl Pts',(6.97687299454425,0.693447748932259,
69.8051863872972));
#144237=CARTESIAN_POINT('Ctrl Pts',(6.95940918677021,0.869153516278404,
69.8132193780777));
#144238=CARTESIAN_POINT('Ctrl Pts',(6.9352853685406,1.04438262091616,69.8212523688583));
#144239=CARTESIAN_POINT('Ctrl Pts',(6.90454037206146,1.21858475826403,69.8292853596388));
#144240=CARTESIAN_POINT('Ctrl Pts',(6.8738143646981,1.39267930267211,69.8373133889814));
#144241=CARTESIAN_POINT('Ctrl Pts',(6.83647538110482,1.56574778262201,69.845341418324));
#144242=CARTESIAN_POINT('Ctrl Pts',(6.79261404458961,1.73724523419812,69.8533694476666));
#144243=CARTESIAN_POINT('Ctrl Pts',(6.74877309020606,1.90866299181328,69.8613937464263));
#144244=CARTESIAN_POINT('Ctrl Pts',(6.69841590921792,2.07851082043406,69.869418045186));
#144245=CARTESIAN_POINT('Ctrl Pts',(6.64168414458086,2.24625427904394,69.8774423439457));
#144246=CARTESIAN_POINT('Ctrl Pts',(6.61915969795449,2.31285415663549,69.8806282643958));
#144247=CARTESIAN_POINT('Ctrl Pts',(6.5956309472628,2.37912244721619,69.8838141848459));
#144248=CARTESIAN_POINT('Ctrl Pts',(6.57110895151813,2.44502632087638,69.887000105296));
#144249=CARTESIAN_POINT('',(7.01124999898235,-0.000119457234741844,69.2264656431203));
#144250=CARTESIAN_POINT('Ctrl Pts',(6.57110895151815,2.44502632087633,69.3398494195812));
#144251=CARTESIAN_POINT('Ctrl Pts',(6.63437020280986,2.27500910220762,69.3316255394411));
#144252=CARTESIAN_POINT('Ctrl Pts',(6.69102680977921,2.10254104764004,69.323401659301));
#144253=CARTESIAN_POINT('Ctrl Pts',(6.74090331182414,1.92817247753887,69.3151777791609));
#144254=CARTESIAN_POINT('Ctrl Pts',(6.79080539628015,1.75371447116496,69.3069496808685));
#144255=CARTESIAN_POINT('Ctrl Pts',(6.8339203313287,1.57735433361791,69.2987215825761));
#144256=CARTESIAN_POINT('Ctrl Pts',(6.8701229150204,1.39965627745229,69.2904934842837));
#144257=CARTESIAN_POINT('Ctrl Pts',(6.90633538304412,1.22190970467799,69.2822631394871));
#144258=CARTESIAN_POINT('Ctrl Pts',(6.93563167566411,1.04282482491902,69.2740327946906));
#144259=CARTESIAN_POINT('Ctrl Pts',(6.95793805352408,0.86297427877169,69.265802449894));
#144260=CARTESIAN_POINT('Ctrl Pts',(6.98026350914649,0.682969913567984,
69.2575650660091));
#144261=CARTESIAN_POINT('Ctrl Pts',(6.99558707148393,0.502198917429808,
69.2493276821243));
#144262=CARTESIAN_POINT('Ctrl Pts',(7.00388696177219,0.321238212573748,
69.2410902982394));
#144263=CARTESIAN_POINT('Ctrl Pts',(7.00879883811094,0.214145639834064,
69.2362154131997));
#144264=CARTESIAN_POINT('Ctrl Pts',(7.01125182384951,0.106986653807984,
69.23134052816));
#144265=CARTESIAN_POINT('Ctrl Pts',(7.01124999898235,-0.000119457234834394,
69.2264656431203));
#144266=CARTESIAN_POINT('Ctrl Pts',(7.01124999898234,-0.000119457912646379,
69.2264656430895));
#144267=CARTESIAN_POINT('Ctrl Pts',(7.0112440780319,-0.347633178973828,
69.2106487170207));
#144268=CARTESIAN_POINT('Ctrl Pts',(6.98539996000994,-0.694636108609602,
69.1948317909518));
#144269=CARTESIAN_POINT('Ctrl Pts',(6.93395267227689,-1.03823258527373,
69.1790148648829));
#144270=CARTESIAN_POINT('Ctrl Pts',(6.90837745387949,-1.20903954747671,
69.1711520336937));
#144271=CARTESIAN_POINT('Ctrl Pts',(6.87644938733158,-1.37914961289592,
69.1632892025045));
#144272=CARTESIAN_POINT('Ctrl Pts',(6.83821763069403,-1.54803300926221,
69.1554263713153));
#144273=CARTESIAN_POINT('Ctrl Pts',(6.8000152501149,-1.71678664103078,69.1475695816739));
#144274=CARTESIAN_POINT('Ctrl Pts',(6.75551889518727,-1.88431510865091,
69.1397127920326));
#144275=CARTESIAN_POINT('Ctrl Pts',(6.70482937411485,-2.05009502865275,
69.1318560023913));
#144276=CARTESIAN_POINT('Ctrl Pts',(6.6541684395327,-2.2157814566276,69.1240036436074));
#144277=CARTESIAN_POINT('Ctrl Pts',(6.59732139762873,-2.37972093508718,
69.1161512848235));
#144278=CARTESIAN_POINT('Ctrl Pts',(6.53443980464629,-2.5414017789311,69.1082989260396));
#144279=CARTESIAN_POINT('Ctrl Pts',(6.47157305874174,-2.70304444804109,
69.1004484212893));
#144280=CARTESIAN_POINT('Ctrl Pts',(6.40267472777406,-2.86242918585216,
69.0925979165389));
#144281=CARTESIAN_POINT('Ctrl Pts',(6.32794573150476,-3.01906100992191,
69.0847474117886));
#144282=CARTESIAN_POINT('Ctrl Pts',(6.25322875677584,-3.17566763686751,
69.076898169937));
#144283=CARTESIAN_POINT('Ctrl Pts',(6.17268315097053,-3.32952188861905,
69.0690489280854));
#144284=CARTESIAN_POINT('Ctrl Pts',(6.08655713355269,-3.48015068962522,
69.0611996862339));
#144285=CARTESIAN_POINT('Ctrl Pts',(6.00040209859372,-3.63083024042291,
69.0533477998191));
#144286=CARTESIAN_POINT('Ctrl Pts',(5.9086630860813,-3.77828183832323,69.0454959134044));
#144287=CARTESIAN_POINT('Ctrl Pts',(5.81163335102251,-3.92205868846744,
69.0376440269896));
#144288=CARTESIAN_POINT('Ctrl Pts',(5.74038562426792,-4.02763223998237,
69.0318784845252));
#144289=CARTESIAN_POINT('Ctrl Pts',(5.66628620282106,-4.13122498531178,
69.0261129420608));
#144290=CARTESIAN_POINT('Ctrl Pts',(5.58946555198211,-4.23267071784534,
69.0203473995965));
#144291=CARTESIAN_POINT('Ctrl Pts',(5.46081733378235,-4.402557494277,69.0106920952363));
#144292=CARTESIAN_POINT('Ctrl Pts',(5.32460260861429,-4.5663359541943,69.0010367908762));
#144293=CARTESIAN_POINT('Ctrl Pts',(5.18138853131843,-4.72343513240331,
68.991381486516));
#144294=CARTESIAN_POINT('Ctrl Pts',(5.03738107490166,-4.88140461058741,
68.9816726935811));
#144295=CARTESIAN_POINT('Ctrl Pts',(4.88629657357506,-5.03262060014217,
68.9719639006461));
#144296=CARTESIAN_POINT('Ctrl Pts',(4.72874223922069,-5.17654550810771,
68.9622551077112));
#144297=CARTESIAN_POINT('Ctrl Pts',(4.57042974003007,-5.32116299495232,
68.9524995952402));
#144298=CARTESIAN_POINT('Ctrl Pts',(4.40558503934989,-5.45841904930235,
68.9427440827692));
#144299=CARTESIAN_POINT('Ctrl Pts',(4.23485403427872,-5.58781154575325,
68.9329885702982));
#144300=CARTESIAN_POINT('Ctrl Pts',(4.06395397924646,-5.71733216068197,
68.923223398369));
#144301=CARTESIAN_POINT('Ctrl Pts',(3.88715599910566,-5.83897362941886,
68.9134582264398));
#144302=CARTESIAN_POINT('Ctrl Pts',(3.70513707572406,-5.95227568351761,
68.9036930545106));
#144303=CARTESIAN_POINT('Ctrl Pts',(3.52336633101492,-6.06542325283614,
68.8939411971718));
#144304=CARTESIAN_POINT('Ctrl Pts',(3.33638890290019,-6.17025411324706,
68.8841893398329));
#144305=CARTESIAN_POINT('Ctrl Pts',(3.14490751207708,-6.26635326988362,
68.8744374824941));
#144306=CARTESIAN_POINT('Ctrl Pts',(3.0614077579646,-6.30825946199491,68.8701849664327));
#144307=CARTESIAN_POINT('Ctrl Pts',(2.97705189743213,-6.34850579991736,
68.8659324503714));
#144308=CARTESIAN_POINT('Ctrl Pts',(2.89189988375889,-6.38706048388579,
68.86167993431));
#144309=CARTESIAN_POINT('Ctrl Pts',(2.73104687373215,-6.45989066956701,
68.8536468887113));
#144310=CARTESIAN_POINT('Ctrl Pts',(2.56727285395838,-6.52671653460162,
68.8456138431125));
#144311=CARTESIAN_POINT('Ctrl Pts',(2.40107367693294,-6.58729624052538,
68.8375807975138));
#144312=CARTESIAN_POINT('Ctrl Pts',(2.23498133913767,-6.64783700348166,
68.8295529158661));
#144313=CARTESIAN_POINT('Ctrl Pts',(2.06646729025432,-6.7021394748109,68.8215250342184));
#144314=CARTESIAN_POINT('Ctrl Pts',(1.89604864416291,-6.75000934084302,
68.8134971525706));
#144315=CARTESIAN_POINT('Ctrl Pts',(1.72570694377035,-6.79785759315868,
68.8054728955906));
#144316=CARTESIAN_POINT('Ctrl Pts',(1.55346271059627,-6.83927892421513,
68.7974486386106));
#144317=CARTESIAN_POINT('Ctrl Pts',(1.37984950630213,-6.87412844675293,
68.7894243816306));
#144318=CARTESIAN_POINT('Ctrl Pts',(1.20625729361261,-6.90897375562851,
68.781401094865));
#144319=CARTESIAN_POINT('Ctrl Pts',(1.03129679716905,-6.93724875903058,
68.7733778080994));
#144320=CARTESIAN_POINT('Ctrl Pts',(0.855513271464657,-6.95885936090448,
68.7653545213337));
#144321=CARTESIAN_POINT('Ctrl Pts',(0.679744149652203,-6.98046819198232,
68.7573318920049));
#144322=CARTESIAN_POINT('Ctrl Pts',(0.503152497308208,-6.99541366853733,
68.7493092626761));
#144323=CARTESIAN_POINT('Ctrl Pts',(0.326289914393268,-7.00365343619066,
68.7412866333472));
#144324=CARTESIAN_POINT('Ctrl Pts',(0.149360843738384,-7.01189630141003,
68.7332609880809));
#144325=CARTESIAN_POINT('Ctrl Pts',(-0.0278389943924678,-7.01342840779972,
68.7252353428146));
#144326=CARTESIAN_POINT('Ctrl Pts',(-0.204756378946018,-7.0082595120173,
68.7172096975483));
#144327=CARTESIAN_POINT('Ctrl Pts',(-0.309077649702985,-7.0052116160867,
68.7124772880401));
#144328=CARTESIAN_POINT('Ctrl Pts',(-0.41330071978238,-6.9998347698926,
68.7077448785319));
#144329=CARTESIAN_POINT('Ctrl Pts',(-0.517312787693255,-6.9921394467065,
68.7030124690237));
#144330=CARTESIAN_POINT('Ctrl Pts',(-0.709187652006125,-6.9779436026873,
68.694282420189));
#144331=CARTESIAN_POINT('Ctrl Pts',(-0.900440130699388,-6.95584821871191,
68.6855523713543));
#144332=CARTESIAN_POINT('Ctrl Pts',(-1.09042849719825,-6.92593620061562,
68.6768223225197));
#144333=CARTESIAN_POINT('Ctrl Pts',(-1.28047179907019,-6.89601553342201,
68.6680897493805));
#144334=CARTESIAN_POINT('Ctrl Pts',(-1.46924998854195,-6.85827376325209,
68.6593571762413));
#144335=CARTESIAN_POINT('Ctrl Pts',(-1.65613021921969,-6.81284516626405,
68.6506246031021));
#144336=CARTESIAN_POINT('Ctrl Pts',(-1.84566538189065,-6.76677118353823,
68.6417679698217));
#144337=CARTESIAN_POINT('Ctrl Pts',(-2.03324796605526,-6.71279037058421,
68.6329113365413));
#144338=CARTESIAN_POINT('Ctrl Pts',(-2.21823189569369,-6.65109568563159,
68.6240547032609));
#144339=CARTESIAN_POINT('Ctrl Pts',(-2.4007407524607,-6.59022647152575,
68.6153165711541));
#144340=CARTESIAN_POINT('Ctrl Pts',(-2.58071980633433,-6.52184863553274,
68.6065784390473));
#144341=CARTESIAN_POINT('Ctrl Pts',(-2.75756609906633,-6.44619700069584,
68.5978403069405));
#144342=CARTESIAN_POINT('Ctrl Pts',(-2.93800981278901,-6.36900645444081,
68.5889244230733));
#144343=CARTESIAN_POINT('Ctrl Pts',(-3.11519167258863,-6.28424312418007,
68.5800085392061));
#144344=CARTESIAN_POINT('Ctrl Pts',(-3.28849396901101,-6.19220752060832,
68.5710926553389));
#144345=CARTESIAN_POINT('Ctrl Pts',(-3.46179626543339,-6.10017191703656,
68.5621767714717));
#144346=CARTESIAN_POINT('Ctrl Pts',(-3.63121873424672,-6.00086418736691,
68.5532608876044));
#144347=CARTESIAN_POINT('Ctrl Pts',(-3.7961707162443,-5.89463437845209,
68.5443450037372));
#144348=CARTESIAN_POINT('Ctrl Pts',(-3.95788135011537,-5.79049201212472,
68.5356043192409));
#144349=CARTESIAN_POINT('Ctrl Pts',(-4.11531273401089,-5.67968602162188,
68.5268636347445));
#144350=CARTESIAN_POINT('Ctrl Pts',(-4.2679340745156,-5.56258620590177,
68.5181229502482));
#144351=CARTESIAN_POINT('Ctrl Pts',(-4.42052795590595,-5.44550745838367,
68.5093838383461));
#144352=CARTESIAN_POINT('Ctrl Pts',(-4.56831330504335,-5.3221373136714,
68.5006447264441));
#144353=CARTESIAN_POINT('Ctrl Pts',(-4.71079085001859,-5.19288707078068,
68.4919056145421));
#144354=CARTESIAN_POINT('Ctrl Pts',(-4.85511439664656,-5.06196220497283,
68.4830532748678));
#144355=CARTESIAN_POINT('Ctrl Pts',(-4.99399141363427,-4.92500398339401,
68.4742009351935));
#144356=CARTESIAN_POINT('Ctrl Pts',(-5.1269390145189,-4.782480831525,68.4653485955192));
#144357=CARTESIAN_POINT('Ctrl Pts',(-5.25811884924494,-4.64185276917254,
68.4566139628694));
#144358=CARTESIAN_POINT('Ctrl Pts',(-5.38352579063847,-4.49580706297155,
68.4478793302195));
#144359=CARTESIAN_POINT('Ctrl Pts',(-5.5027336149339,-4.34483018374441,
68.4391446975696));
#144360=CARTESIAN_POINT('Ctrl Pts',(-5.62435108806826,-4.19080148083132,
68.4302335043831));
#144361=CARTESIAN_POINT('Ctrl Pts',(-5.73951596195329,-4.03164034016135,
68.4213223111966));
#144362=CARTESIAN_POINT('Ctrl Pts',(-5.84781877346933,-3.86789893290397,
68.4124111180101));
#144363=CARTESIAN_POINT('Ctrl Pts',(-5.95612158498537,-3.70415752564659,
68.4034999248236));
#144364=CARTESIAN_POINT('Ctrl Pts',(-6.05756215566655,-3.53583609719769,
68.3945887316371));
#144365=CARTESIAN_POINT('Ctrl Pts',(-6.15177738397906,-3.36351922552314,
68.3856775384507));
#144366=CARTESIAN_POINT('Ctrl Pts',(-6.23663020117123,-3.20832592744157,
68.3776518735984));
#144367=CARTESIAN_POINT('Ctrl Pts',(-6.31566086756942,-3.04982023554966,
68.3696262087461));
#144368=CARTESIAN_POINT('Ctrl Pts',(-6.38860452752145,-2.88848727769959,
68.3616005438938));
#144369=CARTESIAN_POINT('Ctrl Pts',(-6.46152503694502,-2.72720552297309,
68.3535774261907));
#144370=CARTESIAN_POINT('Ctrl Pts',(-6.52836223524753,-2.56309862235754,
68.3455543084876));
#144371=CARTESIAN_POINT('Ctrl Pts',(-6.58889796677334,-2.39667481022148,
68.3375311907845));
#144372=CARTESIAN_POINT('Ctrl Pts',(-6.64942606421354,-2.23027198558481,
68.3295090848668));
#144373=CARTESIAN_POINT('Ctrl Pts',(-6.70365415305433,-2.06155317601521,
68.3214869789491));
#144374=CARTESIAN_POINT('Ctrl Pts',(-6.75141284885911,-1.89104497745563,
68.3134648730313));
#144375=CARTESIAN_POINT('Ctrl Pts',(-6.79918929195661,-1.72047341747335,
68.3054397860719));
#144376=CARTESIAN_POINT('Ctrl Pts',(-6.84049143763795,-1.54811149266162,
68.2974146991125));
#144377=CARTESIAN_POINT('Ctrl Pts',(-6.8752001470764,-1.37449972722464,
68.2893896121531));
#144378=CARTESIAN_POINT('Ctrl Pts',(-6.9099156922215,-1.20085376981924,
68.281362944693));
#144379=CARTESIAN_POINT('Ctrl Pts',(-6.9380351509861,-1.0259578425942,68.2733362772328));
#144380=CARTESIAN_POINT('Ctrl Pts',(-6.95949086974734,-0.850360744862719,
68.2653096097727));
#144381=CARTESIAN_POINT('Ctrl Pts',(-6.98096381308399,-0.674622678399933,
68.2572764985322));
#144382=CARTESIAN_POINT('Ctrl Pts',(-6.9957622966471,-0.498182682104386,
68.2492433872918));
#144383=CARTESIAN_POINT('Ctrl Pts',(-7.00387066355044,-0.321593362427602,
68.2412102760513));
#144384=CARTESIAN_POINT('Ctrl Pts',(-7.00864840788313,-0.217540520300971,
68.236476875089));
#144385=CARTESIAN_POINT('Ctrl Pts',(-7.01110433567618,-0.113435852704417,
68.2317434741267));
#144386=CARTESIAN_POINT('Ctrl Pts',(-7.01124370937301,-0.00939203265251101,
68.2270100731644));
#144387=CARTESIAN_POINT('Ctrl Pts',(-7.01153082352607,0.204941474686562,
68.21725911987));
#144388=CARTESIAN_POINT('Ctrl Pts',(-7.00198517742497,0.419142924397046,
68.2075081665757));
#144389=CARTESIAN_POINT('Ctrl Pts',(-6.98267138124,0.632397773645563,68.1977572132813));
#144390=CARTESIAN_POINT('Ctrl Pts',(-6.96332975990841,0.845959856510448,
68.1879922119095));
#144391=CARTESIAN_POINT('Ctrl Pts',(-6.93419184213086,1.05857257252489,
68.1782272105376));
#144392=CARTESIAN_POINT('Ctrl Pts',(-6.89537417949339,1.26942565252004,
68.1684622091658));
#144393=CARTESIAN_POINT('Ctrl Pts',(-6.85662121785671,1.47992728411851,
68.158713484028));
#144394=CARTESIAN_POINT('Ctrl Pts',(-6.80822076379539,1.68867510418824,
68.1489647588902));
#144395=CARTESIAN_POINT('Ctrl Pts',(-6.75033997079495,1.89487119382507,
68.1392160337524));
#144396=CARTESIAN_POINT('Ctrl Pts',(-6.69261803812816,2.10050135514788,
68.1294940650851));
#144397=CARTESIAN_POINT('Ctrl Pts',(-6.62546772170094,2.30359372895432,
68.1197720964178));
#144398=CARTESIAN_POINT('Ctrl Pts',(-6.54910575244425,2.50336581541763,
68.1100501277504));
#144399=CARTESIAN_POINT('Ctrl Pts',(-6.47324905039368,2.70181606216193,
68.1003924868106));
#144400=CARTESIAN_POINT('Ctrl Pts',(-6.38830218448537,2.89698976137551,
68.0907348458707));
#144401=CARTESIAN_POINT('Ctrl Pts',(-6.294528085565,3.08812932736527,68.0810772049308));
#144402=CARTESIAN_POINT('Ctrl Pts',(-6.25331114065465,3.17214174713031,
68.0768323392465));
#144403=CARTESIAN_POINT('Ctrl Pts',(-6.21038951750221,3.2553749391852,68.0725874735622));
#144404=CARTESIAN_POINT('Ctrl Pts',(-6.1657886753124,3.33776520652508,68.0683426078779));
#144405=CARTESIAN_POINT('Ctrl Pts',(-6.08328924762513,3.49016479291883,
68.060490760864));
#144406=CARTESIAN_POINT('Ctrl Pts',(-5.995074925503,3.63961591340362,68.0526389138501));
#144407=CARTESIAN_POINT('Ctrl Pts',(-5.90139775178321,3.78564804726325,
68.0447870668363));
#144408=CARTESIAN_POINT('Ctrl Pts',(-5.80774714415255,3.93163876759031,
68.0369374465428));
#144409=CARTESIAN_POINT('Ctrl Pts',(-5.70863697235295,4.07421210922336,
68.0290878262492));
#144410=CARTESIAN_POINT('Ctrl Pts',(-5.60436413782013,4.21292406449672,
68.0212382059557));
#144411=CARTESIAN_POINT('Ctrl Pts',(-5.50009962813947,4.35162494539464,
68.0133892123539));
#144412=CARTESIAN_POINT('Ctrl Pts',(-5.39067350606146,4.48646474916962,
68.0055402187522));
#144413=CARTESIAN_POINT('Ctrl Pts',(-5.2764245580144,4.61703047922392,67.9976912251504));
#144414=CARTESIAN_POINT('Ctrl Pts',(-5.16211776907036,4.74766231088414,
67.989838257833));
#144415=CARTESIAN_POINT('Ctrl Pts',(-5.04298352713535,4.8740154579152,67.9819852905157));
#144416=CARTESIAN_POINT('Ctrl Pts',(-4.91939950847617,4.99571166486863,
67.9741323231983));
#144417=CARTESIAN_POINT('Ctrl Pts',(-4.79578410362873,5.11743877856957,
67.9662773614911));
#144418=CARTESIAN_POINT('Ctrl Pts',(-4.66771695223548,5.23450633856139,
67.9584223997839));
#144419=CARTESIAN_POINT('Ctrl Pts',(-4.53561028362952,5.34657515775605,
67.9505674380766));
#144420=CARTESIAN_POINT('Ctrl Pts',(-4.40337248811236,5.45875521462144,
67.9427046796633));
#144421=CARTESIAN_POINT('Ctrl Pts',(-4.26708746699851,5.565926385278,67.93484192125));
#144422=CARTESIAN_POINT('Ctrl Pts',(-4.12719846490059,5.66779140352062,
67.9269791628367));
#144423=CARTESIAN_POINT('Ctrl Pts',(-4.02457790024451,5.74251811923086,
67.9212111560883));
#144424=CARTESIAN_POINT('Ctrl Pts',(-3.9200185028237,5.81439022392368,67.9154431493399));
#144425=CARTESIAN_POINT('Ctrl Pts',(-3.81370389557039,5.88330597193544,
67.9096751425916));
#144426=CARTESIAN_POINT('Ctrl Pts',(-3.65928125321348,5.98340653368255,
67.9012970761505));
#144427=CARTESIAN_POINT('Ctrl Pts',(-3.5008126218529,6.07749008693282,67.8929190097095));
#144428=CARTESIAN_POINT('Ctrl Pts',(-3.33879497014616,6.16523111568631,
67.8845409432685));
#144429=CARTESIAN_POINT('Ctrl Pts',(-3.17688810418469,6.25291214816682,
67.8761686056498));
#144430=CARTESIAN_POINT('Ctrl Pts',(-3.01143734429132,6.33425914669018,
67.867796268031));
#144431=CARTESIAN_POINT('Ctrl Pts',(-2.84296662347438,6.40899113280013,
67.8594239304123));
#144432=CARTESIAN_POINT('Ctrl Pts',(-2.67458639459219,6.48368297756102,
67.8510560898897));
#144433=CARTESIAN_POINT('Ctrl Pts',(-2.50318973898364,6.55176676159969,
67.8426882493671));
#144434=CARTESIAN_POINT('Ctrl Pts',(-2.32932346968877,6.61300829698989,
67.8343204088445));
#144435=CARTESIAN_POINT('Ctrl Pts',(-2.15552512033324,6.6742259086979,67.8259558371746));
#144436=CARTESIAN_POINT('Ctrl Pts',(-1.97925939070828,6.72860649283184,
67.8175912655047));
#144437=CARTESIAN_POINT('Ctrl Pts',(-1.80109170179253,6.77596452501296,
67.8092266938348));
#144438=CARTESIAN_POINT('Ctrl Pts',(-1.62296753369368,6.82331098910191,
67.8008641653693));
#144439=CARTESIAN_POINT('Ctrl Pts',(-1.44294265029347,6.86363823819778,
67.7925016369037));
#144440=CARTESIAN_POINT('Ctrl Pts',(-1.26159665607423,6.89681088909087,
67.7841391084381));
#144441=CARTESIAN_POINT('Ctrl Pts',(-1.08023618987751,6.92998618726524,
67.7757759126166));
#144442=CARTESIAN_POINT('Ctrl Pts',(-0.897554724448007,6.95600568145761,
67.7674127167951));
#144443=CARTESIAN_POINT('Ctrl Pts',(-0.714141822617488,6.97478515939298,
67.7590495209736));
#144444=CARTESIAN_POINT('Ctrl Pts',(-0.530716412394702,6.99356591805111,
67.7506857547989));
#144445=CARTESIAN_POINT('Ctrl Pts',(-0.346559793393782,7.00510564218792,
67.7423219886242));
#144446=CARTESIAN_POINT('Ctrl Pts',(-0.162266591864389,7.00937202006462,
67.7339582224495));
#144447=CARTESIAN_POINT('Ctrl Pts',(0.0220637487109107,7.01363925770827,
67.725592770796));
#144448=CARTESIAN_POINT('Ctrl Pts',(0.206530398000816,7.01063021878269,
67.7172273191424));
#144449=CARTESIAN_POINT('Ctrl Pts',(0.390538351783021,7.0003647303756,67.7088618674888));
#144450=CARTESIAN_POINT('Ctrl Pts',(0.574607929467187,6.99009580407662,
67.700493614262));
#144451=CARTESIAN_POINT('Ctrl Pts',(0.758218177186079,6.97256560077398,
67.6921253610351));
#144452=CARTESIAN_POINT('Ctrl Pts',(0.940778399858321,6.94784589386236,
67.6837571078082));
#144453=CARTESIAN_POINT('Ctrl Pts',(1.12350788190187,6.9231032682558,67.6753810960168));
#144454=CARTESIAN_POINT('Ctrl Pts',(1.30518506736229,6.89115786315449,67.6670050842253));
#144455=CARTESIAN_POINT('Ctrl Pts',(1.48522742135716,6.85213295765259,67.6586290724339));
#144456=CARTESIAN_POINT('Ctrl Pts',(1.6653580703472,6.8130889138548,67.6502489529427));
#144457=CARTESIAN_POINT('Ctrl Pts',(1.84385196931342,6.76695852206363,67.6418688334516));
#144458=CARTESIAN_POINT('Ctrl Pts',(2.02014032892689,6.71391537137185,67.6334887139604));
#144459=CARTESIAN_POINT('Ctrl Pts',(2.19663012032212,6.66081161216129,67.6250990191212));
#144460=CARTESIAN_POINT('Ctrl Pts',(2.37090902365704,6.60077941180021,67.616709324282));
#144461=CARTESIAN_POINT('Ctrl Pts',(2.54242559369602,6.53404152596381,67.6083196294428));
#144462=CARTESIAN_POINT('Ctrl Pts',(2.65131850419885,6.49167079392387,67.6029931569681));
#144463=CARTESIAN_POINT('Ctrl Pts',(2.75909838700588,6.44659813077486,67.5976666844934));
#144464=CARTESIAN_POINT('Ctrl Pts',(2.86562898909334,6.39889029905717,67.5923402120187));
#144465=CARTESIAN_POINT('Ctrl Pts',(3.03325681081882,6.32382116630678,67.5839589116137));
#144466=CARTESIAN_POINT('Ctrl Pts',(3.19812844818391,6.24207373701859,67.5755776112088));
#144467=CARTESIAN_POINT('Ctrl Pts',(3.35969339088097,6.15386763602945,67.5671963108038));
#144468=CARTESIAN_POINT('Ctrl Pts',(3.52105357366497,6.06577332336066,67.5588256324701));
#144469=CARTESIAN_POINT('Ctrl Pts',(3.67911512826064,5.97123680741788,67.5504549541365));
#144470=CARTESIAN_POINT('Ctrl Pts',(3.8333480660444,5.87052545919475,67.5420842758028));
#144471=CARTESIAN_POINT('Ctrl Pts',(3.98740597592415,5.76992840106064,67.5337230967519));
#144472=CARTESIAN_POINT('Ctrl Pts',(4.13764365602719,5.66317065516584,67.525361917701));
#144473=CARTESIAN_POINT('Ctrl Pts',(4.28355587359808,5.55056534420265,67.51700073865));
#144474=CARTESIAN_POINT('Ctrl Pts',(4.42927875285473,5.43810615191344,67.5086504092152));
#144475=CARTESIAN_POINT('Ctrl Pts',(4.57068710673427,5.3198147286725,67.5003000797804));
#144476=CARTESIAN_POINT('Ctrl Pts',(4.70730491031947,5.19604725188121,67.4919497503456));
#144477=CARTESIAN_POINT('Ctrl Pts',(4.843817594677,5.07237500675979,67.4836058459898));
#144478=CARTESIAN_POINT('Ctrl Pts',(4.9755468325591,4.94323532386597,67.475261941634));
#144479=CARTESIAN_POINT('Ctrl Pts',(5.10204901725726,4.80902509746043,67.4669180372781));
#144480=CARTESIAN_POINT('Ctrl Pts',(5.22844959461181,4.67492266954565,67.4585808347983));
#144481=CARTESIAN_POINT('Ctrl Pts',(5.34963126781095,4.53575805826245,67.4502436323185));
#144482=CARTESIAN_POINT('Ctrl Pts',(5.46518660247705,4.3919656149161,67.4419064298387));
#144483=CARTESIAN_POINT('Ctrl Pts',(5.50322678079105,4.3446299362916,67.4391618688032));
#144484=CARTESIAN_POINT('Ctrl Pts',(5.5406575368392,4.29679303928106,67.4364173077677));
#144485=CARTESIAN_POINT('Ctrl Pts',(5.57746523610609,4.24847126652965,67.4336727467322));
#144486=CARTESIAN_POINT('Ctrl Pts',(5.68930934225374,4.10164042438266,67.4253331063335));
#144487=CARTESIAN_POINT('Ctrl Pts',(5.79530587865598,3.95045074942612,67.4169934659349));
#144488=CARTESIAN_POINT('Ctrl Pts',(5.89512928401661,3.79540212457519,67.4086538255363));
#144489=CARTESIAN_POINT('Ctrl Pts',(5.9950015738718,3.64027757090143,67.4003101011345));
#144490=CARTESIAN_POINT('Ctrl Pts',(6.08869453208299,3.4812905776173,67.3919663767327));
#144491=CARTESIAN_POINT('Ctrl Pts',(6.17592787990105,3.31896691528567,67.3836226523309));
#144492=CARTESIAN_POINT('Ctrl Pts',(6.26326419102146,3.15645165901962,67.3752690796607));
#144493=CARTESIAN_POINT('Ctrl Pts',(6.34412550537733,2.99059215515047,67.3669155069906));
#144494=CARTESIAN_POINT('Ctrl Pts',(6.41827853250221,2.82193678910802,67.3585619343204));
#144495=CARTESIAN_POINT('Ctrl Pts',(6.47288405162372,2.69774072898136,67.3524104501551));
#144496=CARTESIAN_POINT('Ctrl Pts',(6.52385286119279,2.57202901017231,67.3462589659897));
#144497=CARTESIAN_POINT('Ctrl Pts',(6.57110895151817,2.44502632087627,67.3401074818243));
#144498=CARTESIAN_POINT('Origin',(0.,0.,50.));
#144499=CARTESIAN_POINT('',(6.57110895151811,2.44502632087645,65.3396321383564));
#144500=CARTESIAN_POINT('',(6.57110895151813,2.4450263208764,65.8869025478802));
#144501=CARTESIAN_POINT('',(6.57110895151814,2.44502632087636,50.));
#144502=CARTESIAN_POINT('',(7.01124987764386,0.00130986217660699,67.7735343569348));
#144503=CARTESIAN_POINT('Ctrl Pts',(6.57110895151813,2.44502632087639,65.8869025478802));
#144504=CARTESIAN_POINT('Ctrl Pts',(6.50935958509336,2.61098028668847,65.89492465128));
#144505=CARTESIAN_POINT('Ctrl Pts',(6.44131154789099,2.77461454209502,65.9029467546797));
#144506=CARTESIAN_POINT('Ctrl Pts',(6.36717722856169,2.93541831815935,65.9109688580794));
#144507=CARTESIAN_POINT('Ctrl Pts',(6.29301524881048,3.0962820920807,65.9189939546242));
#144508=CARTESIAN_POINT('Ctrl Pts',(6.21276260144777,3.25431294251536,65.9270190511689));
#144509=CARTESIAN_POINT('Ctrl Pts',(6.12667896086201,3.40902206989494,65.9350441477136));
#144510=CARTESIAN_POINT('Ctrl Pts',(6.04057820932657,3.56376194899547,65.9430708394165));
#144511=CARTESIAN_POINT('Ctrl Pts',(5.94864434153738,3.71517847367931,65.9510975311194));
#144512=CARTESIAN_POINT('Ctrl Pts',(5.85118159661041,3.8628099210274,65.9591242228222));
#144513=CARTESIAN_POINT('Ctrl Pts',(5.75364074662331,4.01055967781855,65.9671573469854));
#144514=CARTESIAN_POINT('Ctrl Pts',(5.65056238001352,4.15451799840591,65.9751904711486));
#144515=CARTESIAN_POINT('Ctrl Pts',(5.5422927899449,4.29425397397788,65.9832235953118));
#144516=CARTESIAN_POINT('Ctrl Pts',(5.47964922627976,4.37510363339291,65.9878714703488));
#144517=CARTESIAN_POINT('Ctrl Pts',(5.41526857342077,4.45454041626961,65.9925193453858));
#144518=CARTESIAN_POINT('Ctrl Pts',(5.34922373629437,4.53248629138191,65.9971672204228));
#144519=CARTESIAN_POINT('Ctrl Pts',(5.21066576797148,4.69601189859992,66.0069181737171));
#144520=CARTESIAN_POINT('Ctrl Pts',(5.06469993486289,4.85307034626018,66.0166691270113));
#144521=CARTESIAN_POINT('Ctrl Pts',(4.91190287584107,5.00308271976431,66.0264200803056));
#144522=CARTESIAN_POINT('Ctrl Pts',(4.75888568398996,5.15331121423581,66.0361850816774));
#144523=CARTESIAN_POINT('Ctrl Pts',(4.59901760757246,5.29647330211476,66.0459500830492));
#144524=CARTESIAN_POINT('Ctrl Pts',(4.43291210196411,5.43202695674093,66.055715084421));
#144525=CARTESIAN_POINT('Ctrl Pts',(4.26708345981833,5.56735467151011,66.0654638095587));
#144526=CARTESIAN_POINT('Ctrl Pts',(4.0950381962377,5.69509927458982,66.0752125346964));
#144527=CARTESIAN_POINT('Ctrl Pts',(3.91742033283823,5.81476091497885,66.0849612598342));
#144528=CARTESIAN_POINT('Ctrl Pts',(3.74028996160147,5.93409413056448,66.0946832285015));
#144529=CARTESIAN_POINT('Ctrl Pts',(3.55761755688491,6.04538864907153,66.1044051971689));
#144530=CARTESIAN_POINT('Ctrl Pts',(3.37007493883061,6.14818847053064,66.1141271658362));
#144531=CARTESIAN_POINT('Ctrl Pts',(3.18377324129821,6.25030809242007,66.123784806776));
#144532=CARTESIAN_POINT('Ctrl Pts',(2.99266559430891,6.34404501232882,66.1334424477159));
#144533=CARTESIAN_POINT('Ctrl Pts',(2.79744289471133,6.42899213044542,66.1431000886557));
#144534=CARTESIAN_POINT('Ctrl Pts',(2.71163579714709,6.46632931340138,66.1473449543402));
#144535=CARTESIAN_POINT('Ctrl Pts',(2.62503412976144,6.50196891497991,66.1515898200247));
#144536=CARTESIAN_POINT('Ctrl Pts',(2.53769853712627,6.53587887717996,66.1558346857093));
#144537=CARTESIAN_POINT('Ctrl Pts',(2.37615144395389,6.59860308454738,66.1636865327232));
#144538=CARTESIAN_POINT('Ctrl Pts',(2.21215820691028,6.65538003626358,66.1715383797372));
#144539=CARTESIAN_POINT('Ctrl Pts',(2.04621555630563,6.70601434979324,66.1793902267511));
#144540=CARTESIAN_POINT('Ctrl Pts',(1.88031996569481,6.75663430384103,66.1872398470447));
#144541=CARTESIAN_POINT('Ctrl Pts',(1.71247642570905,6.80111497362372,66.1950894673383));
#144542=CARTESIAN_POINT('Ctrl Pts',(1.5431986859047,6.83931022679349,66.202939087632));
#144543=CARTESIAN_POINT('Ctrl Pts',(1.3739344607627,6.87750243056084,66.2107880812338));
#144544=CARTESIAN_POINT('Ctrl Pts',(1.20323663601939,6.90941013345104,66.2186370748357));
#144545=CARTESIAN_POINT('Ctrl Pts',(1.03163080196702,6.93493795580991,66.2264860684375));
#144546=CARTESIAN_POINT('Ctrl Pts',(0.859938088906338,6.96047870215765,
66.234339035755));
#144547=CARTESIAN_POINT('Ctrl Pts',(0.687336825839987,6.97963305817717,
66.2421920030724));
#144548=CARTESIAN_POINT('Ctrl Pts',(0.514359746088131,6.99235730023174,
66.2500449703899));
#144549=CARTESIAN_POINT('Ctrl Pts',(0.341338735969675,7.0050847738163,66.2578999320972));
#144550=CARTESIAN_POINT('Ctrl Pts',(0.167942100275611,7.01137886621324,
66.2657548938045));
#144551=CARTESIAN_POINT('Ctrl Pts',(-0.00529639140698661,7.0112479995175,
66.2736098555118));
#144552=CARTESIAN_POINT('Ctrl Pts',(-0.178706836773275,7.01111700292562,
66.2814726139252));
#144553=CARTESIAN_POINT('Ctrl Pts',(-0.351958443592178,7.004548324577,66.2893353723386));
#144554=CARTESIAN_POINT('Ctrl Pts',(-0.524520949046105,6.99160241550618,
66.297198130752));
#144555=CARTESIAN_POINT('Ctrl Pts',(-0.651110326916408,6.98210548237502,
66.3029661374999));
#144556=CARTESIAN_POINT('Ctrl Pts',(-0.777328949270345,6.96917774512625,
66.3087341442478));
#144557=CARTESIAN_POINT('Ctrl Pts',(-0.902971002041689,6.95286055749516,
66.3145021509957));
#144558=CARTESIAN_POINT('Ctrl Pts',(-1.08546688179807,6.92915973881061,
66.3228802174367));
#144559=CARTESIAN_POINT('Ctrl Pts',(-1.26715024106887,6.89825376719719,
66.3312582838777));
#144560=CARTESIAN_POINT('Ctrl Pts',(-1.44743158371718,6.86021635030252,
66.3396363503187));
#144561=CARTESIAN_POINT('Ctrl Pts',(-1.62758965212568,6.82220494294152,
66.3480086879374));
#144562=CARTESIAN_POINT('Ctrl Pts',(-1.80634729462278,6.77707188004004,
66.3563810255562));
#144563=CARTESIAN_POINT('Ctrl Pts',(-1.98312330321772,6.72494226939792,
66.3647533631749));
#144564=CARTESIAN_POINT('Ctrl Pts',(-2.15980435879701,6.67284065952228,
66.3731212036975));
#144565=CARTESIAN_POINT('Ctrl Pts',(-2.33450558821077,6.61375008798852,
66.3814890442201));
#144566=CARTESIAN_POINT('Ctrl Pts',(-2.50665864296525,6.54784613519191,
66.3898568847427));
#144567=CARTESIAN_POINT('Ctrl Pts',(-2.67874444703872,6.48196792742615,
66.3982214564126));
#144568=CARTESIAN_POINT('Ctrl Pts',(-2.84828375495011,6.40928176337826,
66.4065860280825));
#144569=CARTESIAN_POINT('Ctrl Pts',(-3.01472554613026,6.33001235733467,
66.4149505997524));
#144570=CARTESIAN_POINT('Ctrl Pts',(-3.18112668076413,6.25076231433838,
66.423313128218));
#144571=CARTESIAN_POINT('Ctrl Pts',(-3.3444315112613,6.16493237784235,66.4316756566835));
#144572=CARTESIAN_POINT('Ctrl Pts',(-3.50411067349051,6.07279465735751,
66.440038185149));
#144573=CARTESIAN_POINT('Ctrl Pts',(-3.66380257861672,5.98064958399416,
66.4484013809706));
#144574=CARTESIAN_POINT('Ctrl Pts',(-3.81986794971852,5.88219587998925,
66.456764576792));
#144575=CARTESIAN_POINT('Ctrl Pts',(-3.9718029657698,5.77775109913903,66.4651277726135));
#144576=CARTESIAN_POINT('Ctrl Pts',(-4.12374834348467,5.67329919536407,
66.4734915387882));
#144577=CARTESIAN_POINT('Ctrl Pts',(-4.27156253337539,5.56285558612425,
66.4818553049629));
#144578=CARTESIAN_POINT('Ctrl Pts',(-4.41477146026289,5.44678065614435,
66.4902190711376));
#144579=CARTESIAN_POINT('Ctrl Pts',(-4.55800924683019,5.3306823345688,66.4985845227911));
#144580=CARTESIAN_POINT('Ctrl Pts',(-4.69663966440762,5.20895063640654,
66.5069499744447));
#144581=CARTESIAN_POINT('Ctrl Pts',(-4.83022210864495,5.08198592517311,
66.5153154260982));
#144582=CARTESIAN_POINT('Ctrl Pts',(-4.96384928938052,4.95497869370722,
66.523683679325));
#144583=CARTESIAN_POINT('Ctrl Pts',(-5.09242488754069,4.82273518100134,
66.5320519325519));
#144584=CARTESIAN_POINT('Ctrl Pts',(-5.21554521691631,4.68569254783126,
66.5404201857787));
#144585=CARTESIAN_POINT('Ctrl Pts',(-5.33877969640249,4.54852285658876,
66.5487961975702));
#144586=CARTESIAN_POINT('Ctrl Pts',(-5.45654858012949,4.40654539834418,
66.5571722093616));
#144587=CARTESIAN_POINT('Ctrl Pts',(-5.56848774956643,4.26023130186948,
66.5655482211531));
#144588=CARTESIAN_POINT('Ctrl Pts',(-5.68048181535481,4.11384545115451,
66.5739283406442));
#144589=CARTESIAN_POINT('Ctrl Pts',(-5.78664027107147,3.96311898601142,
66.5823084601353));
#144590=CARTESIAN_POINT('Ctrl Pts',(-5.88664204816884,3.8085524755779,66.5906885796264));
#144591=CARTESIAN_POINT('Ctrl Pts',(-5.98675808996436,3.65380935332637,
66.5990782744656));
#144592=CARTESIAN_POINT('Ctrl Pts',(-6.08070322303536,3.49521769780813,
66.6074679693048));
#144593=CARTESIAN_POINT('Ctrl Pts',(-6.16820143086034,3.33330431716525,
66.615857664144));
#144594=CARTESIAN_POINT('Ctrl Pts',(-6.22375253307756,3.2305083058867,66.6211841366189));
#144595=CARTESIAN_POINT('Ctrl Pts',(-6.27670596914462,3.12637386532603,
66.6265106090938));
#144596=CARTESIAN_POINT('Ctrl Pts',(-6.32700113053064,3.02104009519306,
66.6318370815687));
#144597=CARTESIAN_POINT('Ctrl Pts',(-6.40614147312554,2.85529551011944,
66.6402183819735));
#144598=CARTESIAN_POINT('Ctrl Pts',(-6.47885731027143,2.68624609122133,
66.6485996823783));
#144599=CARTESIAN_POINT('Ctrl Pts',(-6.54487131078168,2.51441565533761,
66.6569809827832));
#144600=CARTESIAN_POINT('Ctrl Pts',(-6.61080164821007,2.34280298937716,
66.6653516611167));
#144601=CARTESIAN_POINT('Ctrl Pts',(-6.67004695930758,2.1684166338342,66.6737223394502));
#144602=CARTESIAN_POINT('Ctrl Pts',(-6.72237646680039,1.99180350464306,
66.6820930177837));
#144603=CARTESIAN_POINT('Ctrl Pts',(-6.77464658928657,1.81539080103108,
66.6904541968345));
#144604=CARTESIAN_POINT('Ctrl Pts',(-6.82001645807766,1.63675667261268,
66.6988153758852));
#144605=CARTESIAN_POINT('Ctrl Pts',(-6.8583037852352,1.45646687292523,66.707176554936));
#144606=CARTESIAN_POINT('Ctrl Pts',(-6.89654143006947,1.27641102051942,
66.7155268843706));
#144607=CARTESIAN_POINT('Ctrl Pts',(-6.92771479682103,1.0947041011038,66.7238772138053));
#144608=CARTESIAN_POINT('Ctrl Pts',(-6.95169173340486,0.911925767927725,
66.73222754324));
#144609=CARTESIAN_POINT('Ctrl Pts',(-6.97565022117037,0.729288071744552,
66.7405714475957));
#144610=CARTESIAN_POINT('Ctrl Pts',(-6.992423271009,0.545580928145699,66.7489153519514));
#144611=CARTESIAN_POINT('Ctrl Pts',(-7.00192979954241,0.361394029806848,
66.7572592563071));
#144612=CARTESIAN_POINT('Ctrl Pts',(-7.01142869237278,0.177355071534034,
66.7655964587868));
#144613=CARTESIAN_POINT('Ctrl Pts',(-7.01367268715592,-0.00716254670140126,
66.7739336612664));
#144614=CARTESIAN_POINT('Ctrl Pts',(-7.00863251950259,-0.191564007764597,
66.7822708637461));
#144615=CARTESIAN_POINT('Ctrl Pts',(-7.00697332413204,-0.252267950879734,
66.7850154247824));
#144616=CARTESIAN_POINT('Ctrl Pts',(-7.00452516988018,-0.312959274449869,
66.7877599858186));
#144617=CARTESIAN_POINT('Ctrl Pts',(-7.00128824767291,-0.373616695956113,
66.7905045468549));
#144618=CARTESIAN_POINT('Ctrl Pts',(-6.99145408423809,-0.557901321421504,
66.7988428571569));
#144619=CARTESIAN_POINT('Ctrl Pts',(-6.97434365674271,-0.74172169567443,
66.8071811674588));
#144620=CARTESIAN_POINT('Ctrl Pts',(-6.95003248498663,-0.92448635475627,
66.8155194777608));
#144621=CARTESIAN_POINT('Ctrl Pts',(-6.92570601746616,-1.10736600316041,
66.8238630342447));
#144622=CARTESIAN_POINT('Ctrl Pts',(-6.89416981231439,-1.28918828673419,
66.8322065907285));
#144623=CARTESIAN_POINT('Ctrl Pts',(-6.85555068412153,-1.46937108313076,
66.8405501472124));
#144624=CARTESIAN_POINT('Ctrl Pts',(-6.8169021746639,-1.64969096181517,
66.8489000514378));
#144625=CARTESIAN_POINT('Ctrl Pts',(-6.77116006214231,-1.8283685453243,
66.8572499556632));
#144626=CARTESIAN_POINT('Ctrl Pts',(-6.71850137597255,-2.00483561010748,
66.8655998598885));
#144627=CARTESIAN_POINT('Ctrl Pts',(-6.66576370567079,-2.18156736242755,
66.8739622883523));
#144628=CARTESIAN_POINT('Ctrl Pts',(-6.60608882428118,-2.3560816561386,
66.882324716816));
#144629=CARTESIAN_POINT('Ctrl Pts',(-6.53970290913463,-2.52782760938242,
66.8906871452797));
#144630=CARTESIAN_POINT('Ctrl Pts',(-6.47326022498118,-2.69972042882796,
66.8990567247597));
#144631=CARTESIAN_POINT('Ctrl Pts',(-6.40009518637036,-2.86883988441289,
66.9074263042397));
#144632=CARTESIAN_POINT('Ctrl Pts',(-6.32048077042347,-3.03465803562892,
66.9157958837197));
#144633=CARTESIAN_POINT('Ctrl Pts',(-6.2407435589398,-3.20073194114075,
66.9241783722564));
#144634=CARTESIAN_POINT('Ctrl Pts',(-6.15453724534981,-3.36349407824554,
66.932560860793));
#144635=CARTESIAN_POINT('Ctrl Pts',(-6.06217981160715,-3.52244268856751,
66.9409433493296));
#144636=CARTESIAN_POINT('Ctrl Pts',(-6.03195894592561,-3.57445327838308,
66.9436862369336));
#144637=CARTESIAN_POINT('Ctrl Pts',(-6.00107981223195,-3.62605579681705,
66.9464291245375));
#144638=CARTESIAN_POINT('Ctrl Pts',(-5.96955451152231,-3.67723340250027,
66.9491720121414));
#144639=CARTESIAN_POINT('Ctrl Pts',(-5.87312595003348,-3.83377379340497,
66.9575618672742));
#144640=CARTESIAN_POINT('Ctrl Pts',(-5.7704540065582,-3.98665241824442,
66.965951722407));
#144641=CARTESIAN_POINT('Ctrl Pts',(-5.66184044539661,-4.13535842864572,
66.9743415775398));
#144642=CARTESIAN_POINT('Ctrl Pts',(-5.55332711130674,-4.28392721522512,
66.9827236906319));
#144643=CARTESIAN_POINT('Ctrl Pts',(-5.43888328252094,-4.42833079901718,
66.991105803724));
#144644=CARTESIAN_POINT('Ctrl Pts',(-5.31885462928421,-4.56808625083217,
66.9994879168161));
#144645=CARTESIAN_POINT('Ctrl Pts',(-5.1989190928432,-4.70773328203671,
67.007863527165));
#144646=CARTESIAN_POINT('Ctrl Pts',(-5.07340758332469,-4.84273912197751,
67.0162391375138));
#144647=CARTESIAN_POINT('Ctrl Pts',(-4.94270702263624,-4.97265259704339,
67.0246147478627));
#144648=CARTESIAN_POINT('Ctrl Pts',(-4.81208867454096,-5.10248435460465,
67.0329850898283));
#144649=CARTESIAN_POINT('Ctrl Pts',(-4.67628801592457,-5.22722990298623,
67.0413554317939));
#144650=CARTESIAN_POINT('Ctrl Pts',(-4.5357302285449,-5.34647340368996,
67.0497257737595));
#144651=CARTESIAN_POINT('Ctrl Pts',(-4.39524024990849,-5.46565937821832,
67.0580920776538));
#144652=CARTESIAN_POINT('Ctrl Pts',(-4.2499979692602,-5.57934838595602,
67.066458381548));
#144653=CARTESIAN_POINT('Ctrl Pts',(-4.10046352380986,-5.68716321661378,
67.0748246854423));
#144654=CARTESIAN_POINT('Ctrl Pts',(-3.95097089895209,-5.79494789448573,
67.0831886495159));
#144655=CARTESIAN_POINT('Ctrl Pts',(-3.7971887683768,-5.89686147787002,
67.0915526135896));
#144656=CARTESIAN_POINT('Ctrl Pts',(-3.63960871915088,-5.99256830866207,
67.0999165776632));
#144657=CARTESIAN_POINT('Ctrl Pts',(-3.48205291887605,-6.0882604117632,
67.1082792546617));
#144658=CARTESIAN_POINT('Ctrl Pts',(-3.32070064602507,-6.1777474960226,
67.1166419316602));
#144659=CARTESIAN_POINT('Ctrl Pts',(-3.15607107101373,-6.26073813197855,
67.1250046086588));
#144660=CARTESIAN_POINT('Ctrl Pts',(-2.99144488542432,-6.34372705930905,
67.1333671134851));
#144661=CARTESIAN_POINT('Ctrl Pts',(-2.82354182586683,-6.42021965745362,
67.1417296183114));
#144662=CARTESIAN_POINT('Ctrl Pts',(-2.6529045611805,-6.48997102857692,
67.1500921231377));
#144663=CARTESIAN_POINT('Ctrl Pts',(-2.48224806486999,-6.55973026100858,
67.1584555704577));
#144664=CARTESIAN_POINT('Ctrl Pts',(-2.30885705345781,-6.62274662780782,
67.1668190177777));
#144665=CARTESIAN_POINT('Ctrl Pts',(-2.13329341539538,-6.67882368133272,
67.1751824650977));
#144666=CARTESIAN_POINT('Ctrl Pts',(-1.9576264005297,-6.73493375460244,
67.1835508370505));
#144667=CARTESIAN_POINT('Ctrl Pts',(-1.77978451577,-6.78409624865235,67.1919192090033));
#144668=CARTESIAN_POINT('Ctrl Pts',(-1.60034502805046,-6.82616454194405,
67.2002875809561));
#144669=CARTESIAN_POINT('Ctrl Pts',(-1.42085177557134,-6.86824543999573,
67.2086584602918));
#144670=CARTESIAN_POINT('Ctrl Pts',(-1.23976028690113,-6.90322782899852,
67.2170293396275));
#144671=CARTESIAN_POINT('Ctrl Pts',(-1.05765792792164,-6.93101625088302,
67.2254002189633));
#144672=CARTESIAN_POINT('Ctrl Pts',(-0.875401275582062,-6.95882821759697,
67.2337781908546));
#144673=CARTESIAN_POINT('Ctrl Pts',(-0.692132367456765,-6.9794339932566,
67.2421561627458));
#144674=CARTESIAN_POINT('Ctrl Pts',(-0.508444758336789,-6.99278989318425,
67.2505341346371));
#144675=CARTESIAN_POINT('Ctrl Pts',(-0.391709786965803,-7.00127767634588,
67.2558584039962));
#144676=CARTESIAN_POINT('Ctrl Pts',(-0.274805793216936,-7.00683849559469,
67.2611826733552));
#144677=CARTESIAN_POINT('Ctrl Pts',(-0.157885183101471,-7.00947207936925,
67.2665069427143));
#144678=CARTESIAN_POINT('Ctrl Pts',(0.0147820803068757,-7.01336133125443,
67.2743697739035));
#144679=CARTESIAN_POINT('Ctrl Pts',(0.187844607511428,-7.01087185981264,
67.2822326050927));
#144680=CARTESIAN_POINT('Ctrl Pts',(0.360771993992302,-7.00196187727774,
67.2900954362819));
#144681=CARTESIAN_POINT('Ctrl Pts',(0.533566508602851,-6.99305874088831,
67.2979522259233));
#144682=CARTESIAN_POINT('Ctrl Pts',(0.706225710680853,-6.97774492350471,
67.3058090155646));
#144683=CARTESIAN_POINT('Ctrl Pts',(0.878216694423301,-6.95603062098897,
67.3136658052059));
#144684=CARTESIAN_POINT('Ctrl Pts',(1.05011068339125,-6.93432856431211,
67.3215181639898));
#144685=CARTESIAN_POINT('Ctrl Pts',(1.22133682656196,-6.906233250375,67.3293705227736));
#144686=CARTESIAN_POINT('Ctrl Pts',(1.39136510248672,-6.87180687403845,
67.3372228815574));
#144687=CARTESIAN_POINT('Ctrl Pts',(1.56135323275291,-6.83738862617079,
67.3450733863078));
#144688=CARTESIAN_POINT('Ctrl Pts',(1.73014368366044,-6.79664235836967,
67.3529238910581));
#144689=CARTESIAN_POINT('Ctrl Pts',(1.8972144850932,-6.74968175250156,67.3607743958085));
#144690=CARTESIAN_POINT('Ctrl Pts',(2.06425841009959,-6.70272870111488,
67.3686236376601));
#144691=CARTESIAN_POINT('Ctrl Pts',(2.22958286985326,-6.64956340788821,
67.3764728795116));
#144692=CARTESIAN_POINT('Ctrl Pts',(2.39267942526589,-6.59034989438416,
67.3843221213632));
#144693=CARTESIAN_POINT('Ctrl Pts',(2.55583093110067,-6.5311164306883,67.392174007778));
#144694=CARTESIAN_POINT('Ctrl Pts',(2.71675267432883,-6.46583080672162,
67.4000258941928));
#144695=CARTESIAN_POINT('Ctrl Pts',(2.87495444240738,-6.39470589758295,
67.4078777806076));
#144696=CARTESIAN_POINT('Ctrl Pts',(2.99112003161824,-6.3424797620725,67.413643323072));
#144697=CARTESIAN_POINT('Ctrl Pts',(3.10581943797929,-6.28710623659363,
67.4194088655363));
#144698=CARTESIAN_POINT('Ctrl Pts',(3.21886666312054,-6.2286855730203,67.4251744080006));
#144699=CARTESIAN_POINT('Ctrl Pts',(3.4081819569637,-6.13085101691265,67.4348297123607));
#144700=CARTESIAN_POINT('Ctrl Pts',(3.59276685959877,-6.02452017000506,
67.4444850167208));
#144701=CARTESIAN_POINT('Ctrl Pts',(3.77196215332629,-5.91015465756812,
67.4541403210809));
#144702=CARTESIAN_POINT('Ctrl Pts',(3.95215015535748,-5.79515558165141,
67.4638491140155));
#144703=CARTESIAN_POINT('Ctrl Pts',(4.12688865790131,-5.67203264405174,
67.4735579069501));
#144704=CARTESIAN_POINT('Ctrl Pts',(4.29554450564503,-5.54129262559945,
67.4832666998846));
#144705=CARTESIAN_POINT('Ctrl Pts',(4.4650119396528,-5.40992347507401,67.4930222123554));
#144706=CARTESIAN_POINT('Ctrl Pts',(4.62833801801298,-5.27086380470448,
67.5027777248262));
#144707=CARTESIAN_POINT('Ctrl Pts',(4.78491794614872,-5.1246645559611,67.5125332372969));
#144708=CARTESIAN_POINT('Ctrl Pts',(4.94165291250443,-4.97832054746749,
67.522298409226));
#144709=CARTESIAN_POINT('Ctrl Pts',(5.09162834726075,-4.82482285475868,
67.5320635811551));
#144710=CARTESIAN_POINT('Ctrl Pts',(5.234275407092,-4.66476017874573,67.5418287530842));
#144711=CARTESIAN_POINT('Ctrl Pts',(5.37672797089282,-4.50491574456084,
67.5515806104229));
#144712=CARTESIAN_POINT('Ctrl Pts',(5.51187210511577,-4.33852424567191,
67.5613324677615));
#144713=CARTESIAN_POINT('Ctrl Pts',(5.63917919487846,-4.16620745649445,
67.5710843251002));
#144714=CARTESIAN_POINT('Ctrl Pts',(5.69469430602751,-4.09106485664502,
67.5753368411625));
#144715=CARTESIAN_POINT('Ctrl Pts',(5.74871962059691,-4.01479596185866,
67.5795893572248));
#144716=CARTESIAN_POINT('Ctrl Pts',(5.80121359253968,-3.93745443354369,
67.5838418732872));
#144717=CARTESIAN_POINT('Ctrl Pts',(5.90037523334362,-3.79135550892132,
67.5918749188861));
#144718=CARTESIAN_POINT('Ctrl Pts',(5.99411776632083,-3.64135563124401,
67.5999079644851));
#144719=CARTESIAN_POINT('Ctrl Pts',(6.08211843569535,-3.48790222005646,
67.607941010084));
#144720=CARTESIAN_POINT('Ctrl Pts',(6.17006253485096,-3.33454745463064,
67.6159688917319));
#144721=CARTESIAN_POINT('Ctrl Pts',(6.25227193601276,-3.17774389145165,
67.6239967733799));
#144722=CARTESIAN_POINT('Ctrl Pts',(6.32846709274347,-3.01796799495339,
67.6320246550278));
#144723=CARTESIAN_POINT('Ctrl Pts',(6.40462784661007,-2.85826423884688,
67.640048912008));
#144724=CARTESIAN_POINT('Ctrl Pts',(6.47477960543809,-2.69559115175709,
67.6480731689882));
#144725=CARTESIAN_POINT('Ctrl Pts',(6.53868872578647,-2.53044982360309,
67.6560974259685));
#144726=CARTESIAN_POINT('Ctrl Pts',(6.60259011887134,-2.36532846271748,
67.6641207127343));
#144727=CARTESIAN_POINT('Ctrl Pts',(6.66025023749395,-2.19773979408075,
67.6721439995002));
#144728=CARTESIAN_POINT('Ctrl Pts',(6.71148349589809,-2.02820508006157,
67.680167286266));
#144729=CARTESIAN_POINT('Ctrl Pts',(6.76271255619354,-1.85868425790052,
67.6881899155951));
#144730=CARTESIAN_POINT('Ctrl Pts',(6.80751570303843,-1.68721806011946,
67.6962125449241));
#144731=CARTESIAN_POINT('Ctrl Pts',(6.84575725567681,-1.5143428141766,67.7042351742532));
#144732=CARTESIAN_POINT('Ctrl Pts',(6.88401318441651,-1.34140257944856,
67.7122608195197));
#144733=CARTESIAN_POINT('Ctrl Pts',(6.91570251502456,-1.16705259719756,
67.7202864647862));
#144734=CARTESIAN_POINT('Ctrl Pts',(6.94074064033649,-0.991839667527716,
67.7283121100528));
#144735=CARTESIAN_POINT('Ctrl Pts',(6.95550464476575,-0.888523447264298,
67.7330445195597));
#144736=CARTESIAN_POINT('Ctrl Pts',(6.96795700030494,-0.784907340178289,
67.7377769290667));
#144737=CARTESIAN_POINT('Ctrl Pts',(6.97808881553933,-0.681104283458026,
67.7425093385737));
#144738=CARTESIAN_POINT('Ctrl Pts',(6.99876795306016,-0.46924119324748,
67.752168234313));
#144739=CARTESIAN_POINT('Ctrl Pts',(7.00978401744958,-0.256539865705297,
67.7618271300524));
#144740=CARTESIAN_POINT('Ctrl Pts',(7.01111315913122,-0.0438044787334321,
67.7714860257919));
#144741=CARTESIAN_POINT('Ctrl Pts',(7.01120711473929,-0.0287664410901019,
67.7721688028314));
#144742=CARTESIAN_POINT('Ctrl Pts',(7.01125268710357,-0.0137282329925991,
67.772851579871));
#144743=CARTESIAN_POINT('Ctrl Pts',(7.01124987764396,0.00130986164159499,
67.7735343569105));
#144744=CARTESIAN_POINT('Ctrl Pts',(7.01124987764386,0.00130986217660248,
67.7735343569348));
#144745=CARTESIAN_POINT('Ctrl Pts',(7.01121431270823,0.191676951975715,
67.7821776246599));
#144746=CARTESIAN_POINT('Ctrl Pts',(7.00342123474153,0.382030764535196,
67.7908208923851));
#144747=CARTESIAN_POINT('Ctrl Pts',(6.98789966165083,0.571738472730573,
67.7994641601102));
#144748=CARTESIAN_POINT('Ctrl Pts',(6.97237406338665,0.761495377384949,
67.8081096692739));
#144749=CARTESIAN_POINT('Ctrl Pts',(6.94911598735449,0.950605554743249,
67.8167551784376));
#144750=CARTESIAN_POINT('Ctrl Pts',(6.91820640209675,1.13844048614214,67.8254006876012));
#144751=CARTESIAN_POINT('Ctrl Pts',(6.88729488458905,1.32628715966041,67.8340467372214));
#144752=CARTESIAN_POINT('Ctrl Pts',(6.84873095327239,1.51285814355938,67.8426927868415));
#144753=CARTESIAN_POINT('Ctrl Pts',(6.80264692888082,1.69753389465082,67.8513388364616));
#144754=CARTESIAN_POINT('Ctrl Pts',(6.7565525050491,1.88225132014994,67.8599868371716));
#144755=CARTESIAN_POINT('Ctrl Pts',(6.70293466818401,2.06507237817528,67.8686348378817));
#144756=CARTESIAN_POINT('Ctrl Pts',(6.64197623980495,2.24539043205553,67.8772828385918));
#144757=CARTESIAN_POINT('Ctrl Pts',(6.61936005031205,2.31229024204057,67.8804913337579));
#144758=CARTESIAN_POINT('Ctrl Pts',(6.59573393242823,2.37884567034198,67.8836998289241));
#144759=CARTESIAN_POINT('Ctrl Pts',(6.57110895151815,2.44502632087632,67.8869083240903));
#144760=CARTESIAN_POINT('',(7.0112494081677,0.00288079295883046,67.2264656430621));
#144761=CARTESIAN_POINT('Ctrl Pts',(6.57110895151817,2.44502632087627,67.3401074818243));
#144762=CARTESIAN_POINT('Ctrl Pts',(6.6353893413515,2.27227012539716,67.3317398873517));
#144763=CARTESIAN_POINT('Ctrl Pts',(6.69279811250386,2.09712499354561,67.3233722928791));
#144764=CARTESIAN_POINT('Ctrl Pts',(6.74318804242022,1.92016707269471,67.3150046984065));
#144765=CARTESIAN_POINT('Ctrl Pts',(6.79366014580145,1.74292057741006,67.3066234584648));
#144766=CARTESIAN_POINT('Ctrl Pts',(6.83709045258875,1.56385570257469,67.2982422185232));
#144767=CARTESIAN_POINT('Ctrl Pts',(6.8733827515476,1.38355921927034,67.2898609785815));
#144768=CARTESIAN_POINT('Ctrl Pts',(6.89482537839213,1.27703441032229,67.2849090795362));
#144769=CARTESIAN_POINT('Ctrl Pts',(6.91377724198473,1.1700797930562,67.279957180491));
#144770=CARTESIAN_POINT('Ctrl Pts',(6.93022702928659,1.06281695745107,67.2750052814458));
#144771=CARTESIAN_POINT('Ctrl Pts',(6.97711648270191,0.757068582654123,
67.26089009349));
#144772=CARTESIAN_POINT('Ctrl Pts',(7.0037476227958,0.448352346246154,67.2467749055342));
#144773=CARTESIAN_POINT('Ctrl Pts',(7.00987641219841,0.13877769346808,67.2326597175784));
#144774=CARTESIAN_POINT('Ctrl Pts',(7.01077289755884,0.0934948282978932,
67.2305950260821));
#144775=CARTESIAN_POINT('Ctrl Pts',(7.01123078995113,0.048193640652253,
67.2285303345859));
#144776=CARTESIAN_POINT('Ctrl Pts',(7.01124940816745,0.00288079356271242,
67.2264656430896));
#144777=CARTESIAN_POINT('Ctrl Pts',(7.0112494081677,0.00288079295891919,
67.2264656430621));
#144778=CARTESIAN_POINT('Ctrl Pts',(7.01132401095931,-0.178686846915374,
67.2181924669956));
#144779=CARTESIAN_POINT('Ctrl Pts',(7.00434137349408,-0.360424500685907,
67.2099192909291));
#144780=CARTESIAN_POINT('Ctrl Pts',(6.99028831897533,-0.541752508159516,
67.2016461148625));
#144781=CARTESIAN_POINT('Ctrl Pts',(6.97624724392217,-0.722925943356717,
67.1933799912292));
#144782=CARTESIAN_POINT('Ctrl Pts',(6.95514778939696,-0.903690088920113,
67.1851138675959));
#144783=CARTESIAN_POINT('Ctrl Pts',(6.92702882887233,-1.08346581232248,
67.1768477439626));
#144784=CARTESIAN_POINT('Ctrl Pts',(6.89892893047013,-1.26311966397767,
67.1685872240165));
#144785=CARTESIAN_POINT('Ctrl Pts',(6.86381906325825,-1.44178609232468,
67.1603267040704));
#144786=CARTESIAN_POINT('Ctrl Pts',(6.821789904695,-1.61889130540051,67.1520661841243));
#144787=CARTESIAN_POINT('Ctrl Pts',(6.77978178839405,-1.79590784921733,
67.1438097998791));
#144788=CARTESIAN_POINT('Ctrl Pts',(6.7308613651662,-1.97136440397714,67.1355534156339));
#144789=CARTESIAN_POINT('Ctrl Pts',(6.67517041976566,-2.14469728157275,
67.1272970313887));
#144790=CARTESIAN_POINT('Ctrl Pts',(6.61949475681673,-2.31798259396192,
67.1190429128222));
#144791=CARTESIAN_POINT('Ctrl Pts',(6.5570523783293,-2.4891450653505,67.1107887942558));
#144792=CARTESIAN_POINT('Ctrl Pts',(6.48803506528663,-2.65763570756247,
67.1025346756894));
#144793=CARTESIAN_POINT('Ctrl Pts',(6.41902577227563,-2.82610677062502,
67.0942815162778));
#144794=CARTESIAN_POINT('Ctrl Pts',(6.34344319710818,-2.99190630719308,
67.0860283568662));
#144795=CARTESIAN_POINT('Ctrl Pts',(6.26152754535116,-3.15450461424748,
67.0777751974547));
#144796=CARTESIAN_POINT('Ctrl Pts',(6.17960845368729,-3.31710974933804,
67.0695216914659));
#144797=CARTESIAN_POINT('Ctrl Pts',(6.09135590981829,-3.47651308214818,
67.0612681854771));
#144798=CARTESIAN_POINT('Ctrl Pts',(5.99705654282694,-3.63220860973549,
67.0530146794883));
#144799=CARTESIAN_POINT('Ctrl Pts',(5.90270291679597,-3.78799372318184,
67.0447564245035));
#144800=CARTESIAN_POINT('Ctrl Pts',(5.80229569107786,-3.94006647478785,
67.0364981695188));
#144801=CARTESIAN_POINT('Ctrl Pts',(5.69616588633061,-4.087948233271,67.0282399145341));
#144802=CARTESIAN_POINT('Ctrl Pts',(5.59000606981233,-4.23587181029405,
67.0199793242501));
#144803=CARTESIAN_POINT('Ctrl Pts',(5.47812065295235,-4.37960175772584,
67.0117187339661));
#144804=CARTESIAN_POINT('Ctrl Pts',(5.36088184160279,-4.51869145249745,
67.0034581436821));
#144805=CARTESIAN_POINT('Ctrl Pts',(5.24353078727498,-4.65791431001103,
66.9951896448118));
#144806=CARTESIAN_POINT('Ctrl Pts',(5.12081632178934,-4.79248777969411,
66.9869211459415));
#144807=CARTESIAN_POINT('Ctrl Pts',(4.99314929103177,-4.92200027630728,
66.9786526470712));
#144808=CARTESIAN_POINT('Ctrl Pts',(4.88515921543913,-5.03155138136907,
66.9716585483385));
#144809=CARTESIAN_POINT('Ctrl Pts',(4.77362630084601,-5.13748190703201,
66.9646644496056));
#144810=CARTESIAN_POINT('Ctrl Pts',(4.65881814937934,-5.23956486871894,
66.9576703508729));
#144811=CARTESIAN_POINT('Ctrl Pts',(4.5297497520606,-5.35432748870857,66.9498075196836));
#144812=CARTESIAN_POINT('Ctrl Pts',(4.3962500321622,-5.46448492412578,66.9419446884944));
#144813=CARTESIAN_POINT('Ctrl Pts',(4.2586961446527,-5.56966190266701,66.9340818573052));
#144814=CARTESIAN_POINT('Ctrl Pts',(4.12124794914882,-5.67475806658345,
66.9262250676638));
#144815=CARTESIAN_POINT('Ctrl Pts',(3.97975208176395,-5.7748811537224,66.9183682780225));
#144816=CARTESIAN_POINT('Ctrl Pts',(3.83462126203656,-5.86969388803515,
66.9105114883811));
#144817=CARTESIAN_POINT('Ctrl Pts',(3.68957228922128,-5.964453152454,66.9026591295972));
#144818=CARTESIAN_POINT('Ctrl Pts',(3.54089276006501,-6.05390781348886,
66.8948067708133));
#144819=CARTESIAN_POINT('Ctrl Pts',(3.38902686433104,-6.13776209015489,
66.8869544120294));
#144820=CARTESIAN_POINT('Ctrl Pts',(3.23719682590718,-6.2215965678477,66.879103907279));
#144821=CARTESIAN_POINT('Ctrl Pts',(3.08218224765762,-6.29983310143366,
66.8712534025286));
#144822=CARTESIAN_POINT('Ctrl Pts',(2.92445452040377,-6.37222036032888,
66.8634028977782));
#144823=CARTESIAN_POINT('Ctrl Pts',(2.76675216656987,-6.4445959743957,66.8555536559266));
#144824=CARTESIAN_POINT('Ctrl Pts',(2.60633788060554,-6.51112403054878,
66.847704414075));
#144825=CARTESIAN_POINT('Ctrl Pts',(2.44370533555261,-6.57160032225726,
66.8398551722234));
#144826=CARTESIAN_POINT('Ctrl Pts',(2.28101799641227,-6.63209698961203,
66.8320032858086));
#144827=CARTESIAN_POINT('Ctrl Pts',(2.11611126326507,-6.68653768673339,
66.8241513993938));
#144828=CARTESIAN_POINT('Ctrl Pts',(1.94949655074439,-6.7347672388239,66.816299512979));
#144829=CARTESIAN_POINT('Ctrl Pts',(1.82715344114728,-6.77018159862419,
66.8105339705149));
#144830=CARTESIAN_POINT('Ctrl Pts',(1.70388980937451,-6.80224806435733,
66.8047684280507));
#144831=CARTESIAN_POINT('Ctrl Pts',(1.57991231257096,-6.83092260584811,
66.7990028855866));
#144832=CARTESIAN_POINT('Ctrl Pts',(1.37229256596841,-6.87894261909045,
66.7893475812265));
#144833=CARTESIAN_POINT('Ctrl Pts',(1.16277658245736,-6.91742492590395,
66.7796922768665));
#144834=CARTESIAN_POINT('Ctrl Pts',(0.952165633350585,-6.94629449196952,
66.7700369725065));
#144835=CARTESIAN_POINT('Ctrl Pts',(0.740387939095827,-6.97532399001524,
66.7603281795716));
#144836=CARTESIAN_POINT('Ctrl Pts',(0.52750316800487,-6.99463399454545,
66.7506193866367));
#144837=CARTESIAN_POINT('Ctrl Pts',(0.314321967060732,-7.00420075836802,
66.7409105937018));
#144838=CARTESIAN_POINT('Ctrl Pts',(0.100114920075997,-7.01381355827043,
66.731155081231));
#144839=CARTESIAN_POINT('Ctrl Pts',(-0.11439137222014,-7.01358914327683,
66.7213995687601));
#144840=CARTESIAN_POINT('Ctrl Pts',(-0.328379282896417,-7.00355578324785,
66.7116440562892));
#144841=CARTESIAN_POINT('Ctrl Pts',(-0.542579074524512,-6.99351248864889,
66.7018788843602));
#144842=CARTESIAN_POINT('Ctrl Pts',(-0.756259420085494,-6.97364083502745,
66.6921137124312));
#144843=CARTESIAN_POINT('Ctrl Pts',(-0.968605641946421,-6.94402114576918,
66.6823485405021));
#144844=CARTESIAN_POINT('Ctrl Pts',(-1.18066233455172,-6.91444184228519,
66.6725966831635));
#144845=CARTESIAN_POINT('Ctrl Pts',(-1.39138850150225,-6.8751410728307,
66.6628448258248));
#144846=CARTESIAN_POINT('Ctrl Pts',(-1.59997870808713,-6.82625041264733,
66.6530929684862));
#144847=CARTESIAN_POINT('Ctrl Pts',(-1.69093914496475,-6.8049305439808,
66.6488404524241));
#144848=CARTESIAN_POINT('Ctrl Pts',(-1.78149348873842,-6.78178773194605,
66.644587936362));
#144849=CARTESIAN_POINT('Ctrl Pts',(-1.87157533319683,-6.75683597067956,
66.6403354203));
#144850=CARTESIAN_POINT('Ctrl Pts',(-2.04174084311913,-6.70970184276623,
66.6323023747012));
#144851=CARTESIAN_POINT('Ctrl Pts',(-2.21030233969986,-6.65608610196948,
66.6242693291025));
#144852=CARTESIAN_POINT('Ctrl Pts',(-2.37672416113031,-6.59612074058681,
66.6162362835037));
#144853=CARTESIAN_POINT('Ctrl Pts',(-2.54303900020586,-6.5361939272474,
66.608208401856));
#144854=CARTESIAN_POINT('Ctrl Pts',(-2.70721655860214,-6.46992574194944,
66.6001805202082));
#144855=CARTESIAN_POINT('Ctrl Pts',(-2.86873529756915,-6.39749828878295,
66.5921526385605));
#144856=CARTESIAN_POINT('Ctrl Pts',(-3.03018110923428,-6.32510353732511,
66.5841283815804));
#144857=CARTESIAN_POINT('Ctrl Pts',(-3.18897015798354,-6.24655520490433,
66.5761041246003));
#144858=CARTESIAN_POINT('Ctrl Pts',(-3.34459994239156,-6.16208388354576,
66.5680798676202));
#144859=CARTESIAN_POINT('Ctrl Pts',(-3.50021090957254,-6.07762277563083,
66.5600565808546));
#144860=CARTESIAN_POINT('Ctrl Pts',(-3.65266304760336,-5.98724027321399,
66.552033294089));
#144861=CARTESIAN_POINT('Ctrl Pts',(-3.80147741768659,-5.89121345779619,
66.5440100073233));
#144862=CARTESIAN_POINT('Ctrl Pts',(-3.95027959375968,-5.79519451091931,
66.5359873779945));
#144863=CARTESIAN_POINT('Ctrl Pts',(-4.0954442897418,-5.69353237446911,
66.5279647486656));
#144864=CARTESIAN_POINT('Ctrl Pts',(-4.23652084418538,-5.586547923296,66.5199421193367));
#144865=CARTESIAN_POINT('Ctrl Pts',(-4.37765043336989,-5.4795232535857,
66.5119164740704));
#144866=CARTESIAN_POINT('Ctrl Pts',(-4.51468852043737,-5.36717249623786,
66.5038908288041));
#144867=CARTESIAN_POINT('Ctrl Pts',(-4.64721658537029,-5.24985757627379,
66.4958651835377));
#144868=CARTESIAN_POINT('Ctrl Pts',(-4.72536320832142,-5.18068155064017,
66.4911327740297));
#144869=CARTESIAN_POINT('Ctrl Pts',(-4.80194233615778,-5.10978023901075,
66.4864003645217));
#144870=CARTESIAN_POINT('Ctrl Pts',(-4.87687406826176,-5.0372339517652,
66.4816679550137));
#144871=CARTESIAN_POINT('Ctrl Pts',(-5.01510337395312,-4.90340516341523,
66.472937906179));
#144872=CARTESIAN_POINT('Ctrl Pts',(-5.14779378229524,-4.76390974365538,
66.4642078573442));
#144873=CARTESIAN_POINT('Ctrl Pts',(-5.2745056821904,-4.6192224855533,66.4554778085094));
#144874=CARTESIAN_POINT('Ctrl Pts',(-5.40125422098924,-4.47449339095032,
66.4467452353702));
#144875=CARTESIAN_POINT('Ctrl Pts',(-5.52202062029474,-4.32456966756031,
66.4380126622309));
#144876=CARTESIAN_POINT('Ctrl Pts',(-5.63640499890855,-4.16995986201052,
66.4292800890917));
#144877=CARTESIAN_POINT('Ctrl Pts',(-5.75241439021074,-4.01315357737142,
66.4204234558113));
#144878=CARTESIAN_POINT('Ctrl Pts',(-5.86185887282661,-3.85152728225305,
66.4115668225309));
#144879=CARTESIAN_POINT('Ctrl Pts',(-5.96436600367793,-3.68564305605834,
66.4027101892506));
#144880=CARTESIAN_POINT('Ctrl Pts',(-6.06550159582862,-3.52197834995123,
66.3939720571437));
#144881=CARTESIAN_POINT('Ctrl Pts',(-6.1598841996382,-3.35416919529334,
66.3852339250369));
#144882=CARTESIAN_POINT('Ctrl Pts',(-6.2472013001056,-3.18278219148891,
66.37649579293));
#144883=CARTESIAN_POINT('Ctrl Pts',(-6.33629461179553,-3.00790881997501,
66.3675799090629));
#144884=CARTESIAN_POINT('Ctrl Pts',(-6.41803174922114,-2.82931074057956,
66.3586640251958));
#144885=CARTESIAN_POINT('Ctrl Pts',(-6.49213095549625,-2.64761443929954,
66.3497481413286));
#144886=CARTESIAN_POINT('Ctrl Pts',(-6.56623016177137,-2.46591813801946,
66.3408322574615));
#144887=CARTESIAN_POINT('Ctrl Pts',(-6.63269132833057,-2.28112389717326,
66.3319163735943));
#144888=CARTESIAN_POINT('Ctrl Pts',(-6.69128520431793,-2.09387890695139,
66.3230004897271));
#144889=CARTESIAN_POINT('Ctrl Pts',(-6.74872769583538,-1.9103133281045,
66.314259805231));
#144890=CARTESIAN_POINT('Ctrl Pts',(-6.79861531624834,-1.72437292503407,
66.3055191207349));
#144891=CARTESIAN_POINT('Ctrl Pts',(-6.84077743512908,-1.53668169948391,
66.2967784362388));
#144892=CARTESIAN_POINT('Ctrl Pts',(-6.88293196834461,-1.34902424270155,
66.288039324337));
#144893=CARTESIAN_POINT('Ctrl Pts',(-6.91736371586907,-1.15961685956442,
66.2793002124351));
#144894=CARTESIAN_POINT('Ctrl Pts',(-6.9439528378881,-0.96909522116552,
66.2705611005333));
#144895=CARTESIAN_POINT('Ctrl Pts',(-6.97088646025153,-0.776105100731107,
66.2617087608589));
#144896=CARTESIAN_POINT('Ctrl Pts',(-6.98977275376875,-0.581971929368133,
66.2528564211845));
#144897=CARTESIAN_POINT('Ctrl Pts',(-7.00054105897644,-0.387364742955533,
66.2440040815102));
#144898=CARTESIAN_POINT('Ctrl Pts',(-7.01116618111459,-0.195345192551464,
66.2352694488605));
#144899=CARTESIAN_POINT('Ctrl Pts',(-7.01388785773911,-0.00286443578903975,
66.2265348162108));
#144900=CARTESIAN_POINT('Ctrl Pts',(-7.00869049695713,0.189430938241047,
66.2178001835612));
#144901=CARTESIAN_POINT('Ctrl Pts',(-7.00338807751408,0.385613341740791,
66.2088889903744));
#144902=CARTESIAN_POINT('Ctrl Pts',(-6.98984304867728,0.581602497237557,
66.1999777971877));
#144903=CARTESIAN_POINT('Ctrl Pts',(-6.968094780042,0.776712108088613,66.191066604001));
#144904=CARTESIAN_POINT('Ctrl Pts',(-6.94634651140671,0.971821718939736,
66.1821554108142));
#144905=CARTESIAN_POINT('Ctrl Pts',(-6.91639502316282,1.16605148238852,
66.1732442176275));
#144906=CARTESIAN_POINT('Ctrl Pts',(-6.87833604413355,1.35871992201237,
66.1643330244408));
#144907=CARTESIAN_POINT('Ctrl Pts',(-6.84405908436909,1.53224240005331,
66.1563073595883));
#144908=CARTESIAN_POINT('Ctrl Pts',(-6.80318963512189,1.70457808618064,
66.1482816947359));
#144909=CARTESIAN_POINT('Ctrl Pts',(-6.7558351447834,1.87518480662827,66.1402560298835));
#144910=CARTESIAN_POINT('Ctrl Pts',(-6.70849568359854,2.04573738068782,
66.1322329121802));
#144911=CARTESIAN_POINT('Ctrl Pts',(-6.65467537691532,2.21456172874354,
66.1242097944769));
#144912=CARTESIAN_POINT('Ctrl Pts',(-6.59453233375239,2.38112785494484,
66.1161866767736));
#144913=CARTESIAN_POINT('Ctrl Pts',(-6.53439687515367,2.54767297569959,
66.1081645708557));
#144914=CARTESIAN_POINT('Ctrl Pts',(-6.46794039332366,2.71196009736767,
66.1001424649378));
#144915=CARTESIAN_POINT('Ctrl Pts',(-6.39537020826617,2.8734763722226,66.0921203590199));
#144916=CARTESIAN_POINT('Ctrl Pts',(-6.32277305588252,3.03505266707143,
66.0840952720603));
#144917=CARTESIAN_POINT('Ctrl Pts',(-6.24405780942596,3.19385572226692,
66.0760701851007));
#144918=CARTESIAN_POINT('Ctrl Pts',(-6.15947929163983,3.34939418676873,
66.0680450981411));
#144919=CARTESIAN_POINT('Ctrl Pts',(-6.07488411653789,3.50496328379273,
66.0600184306808));
#144920=CARTESIAN_POINT('Ctrl Pts',(-5.9844235525224,3.65726619144901,66.0519917632205));
#144921=CARTESIAN_POINT('Ctrl Pts',(-5.8883972550324,3.8058381901267,66.0439650957602));
#144922=CARTESIAN_POINT('Ctrl Pts',(-5.79229386796916,3.9545294618814,66.0359319845196));
#144923=CARTESIAN_POINT('Ctrl Pts',(-5.69061603016253,4.09948353981285,
66.0278988732789));
#144924=CARTESIAN_POINT('Ctrl Pts',(-5.5837057600017,4.24026609403512,66.0198657620383));
#144925=CARTESIAN_POINT('Ctrl Pts',(-5.52071034510035,4.32322028918178,
66.0151323610769));
#144926=CARTESIAN_POINT('Ctrl Pts',(-5.4558990038931,4.40472675176677,66.0103989601156));
#144927=CARTESIAN_POINT('Ctrl Pts',(-5.38934796350171,4.48470234138231,
66.0056655591543));
#144928=CARTESIAN_POINT('Ctrl Pts',(-5.25225074908404,4.64945454500257,
65.9959146058604));
#144929=CARTESIAN_POINT('Ctrl Pts',(-5.10768840989514,4.80780577013776,
65.9861636525664));
#144930=CARTESIAN_POINT('Ctrl Pts',(-4.95623241002525,4.9591719934194,65.9764126992725));
#144931=CARTESIAN_POINT('Ctrl Pts',(-4.80455820937429,5.11075628814208,
65.9666476979011));
#144932=CARTESIAN_POINT('Ctrl Pts',(-4.64597050922282,5.25533542432872,
65.9568826965296));
#144933=CARTESIAN_POINT('Ctrl Pts',(-4.48107791698386,5.3923619374463,65.9471176951582));
#144934=CARTESIAN_POINT('Ctrl Pts',(-4.31646016653066,5.5291600557582,65.9373689700207));
#144935=CARTESIAN_POINT('Ctrl Pts',(-4.1455585562666,5.65843068638659,65.9276202448833));
#144936=CARTESIAN_POINT('Ctrl Pts',(-3.96901263396953,5.77966826676846,
65.9178715197458));
#144937=CARTESIAN_POINT('Ctrl Pts',(-3.79295126177409,5.90057309700163,
65.9081495510788));
#144938=CARTESIAN_POINT('Ctrl Pts',(-3.61127653660829,6.01348886882795,
65.8984275824118));
#144939=CARTESIAN_POINT('Ctrl Pts',(-3.42465619391963,6.11795362159177,
65.8887056137449));
#144940=CARTESIAN_POINT('Ctrl Pts',(-3.23927066929506,6.22172715837178,
65.8790479728053));
#144941=CARTESIAN_POINT('Ctrl Pts',(-3.04900478516365,6.31716109481636,
65.8693903318656));
#144942=CARTESIAN_POINT('Ctrl Pts',(-2.85454578810235,6.40384219872157,
65.8597326909261));
#144943=CARTESIAN_POINT('Ctrl Pts',(-2.7690743640634,6.44194152814324,65.85548782524));
#144944=CARTESIAN_POINT('Ctrl Pts',(-2.68279329434385,6.47835041454282,
65.851242959554));
#144945=CARTESIAN_POINT('Ctrl Pts',(-2.5957629358197,6.51303626149315,65.846998093868));
#144946=CARTESIAN_POINT('Ctrl Pts',(-2.43478044279259,6.57719564460395,
65.839146246854));
#144947=CARTESIAN_POINT('Ctrl Pts',(-2.27129897621767,6.63542977659541,
65.8312943998401));
#144948=CARTESIAN_POINT('Ctrl Pts',(-2.10581350796261,6.68753886210631,
65.8234425528261));
#144949=CARTESIAN_POINT('Ctrl Pts',(-1.94037497004867,6.73963316990179,
65.8155929325325));
#144950=CARTESIAN_POINT('Ctrl Pts',(-1.77293392443038,6.7856057719751,65.8077433122389));
#144951=CARTESIAN_POINT('Ctrl Pts',(-1.60400279984087,6.8253059697425,65.7998936919453));
#144952=CARTESIAN_POINT('Ctrl Pts',(-1.43508516224169,6.86500299795673,
65.7920446983435));
#144953=CARTESIAN_POINT('Ctrl Pts',(-1.26467805401425,6.89842853222309,
65.7841957047417));
#144954=CARTESIAN_POINT('Ctrl Pts',(-1.09330619582332,6.92548251926711,
65.7763467111399));
#144955=CARTESIAN_POINT('Ctrl Pts',(-0.921847577077617,6.95255020295276,
65.7684937438224));
#144956=CARTESIAN_POINT('Ctrl Pts',(-0.749423609760433,6.97323983468869,
65.760640776505));
#144957=CARTESIAN_POINT('Ctrl Pts',(-0.576566616985063,6.98750295160427,
65.7527878091875));
#144958=CARTESIAN_POINT('Ctrl Pts',(-0.403665724341947,7.00176969087227,
65.7449328474802));
#144959=CARTESIAN_POINT('Ctrl Pts',(-0.230331968266925,7.00960664652595,
65.7370778857729));
#144960=CARTESIAN_POINT('Ctrl Pts',(-0.0570991721608681,7.01101749013926,
65.7292229240656));
#144961=CARTESIAN_POINT('Ctrl Pts',(0.116305571975743,7.01242973413278,
65.7213601656523));
#144962=CARTESIAN_POINT('Ctrl Pts',(0.289608774858064,7.00740313774478,
65.7134974072389));
#144963=CARTESIAN_POINT('Ctrl Pts',(0.462279656693552,6.99599343063637,
65.7056346488255));
#144964=CARTESIAN_POINT('Ctrl Pts',(0.588948537924436,6.98762343322146,
65.6998666420775));
#144965=CARTESIAN_POINT('Ctrl Pts',(0.715277210151469,6.97581946807508,
65.6940986353295));
#144966=CARTESIAN_POINT('Ctrl Pts',(0.841059499438371,6.96062105568925,
65.6883306285815));
#144967=CARTESIAN_POINT('Ctrl Pts',(1.02375907362194,6.93854526515546,65.6799525621405));
#144968=CARTESIAN_POINT('Ctrl Pts',(1.20571028047177,6.90925737613356,65.6715744956995));
#144969=CARTESIAN_POINT('Ctrl Pts',(1.38632299124672,6.8728258472364,65.6631964292585));
#144970=CARTESIAN_POINT('Ctrl Pts',(1.56681220119583,6.83641922978588,65.6548240916397));
#144971=CARTESIAN_POINT('Ctrl Pts',(1.74596441859612,6.79287877596949,65.646451754021));
#144972=CARTESIAN_POINT('Ctrl Pts',(1.92319734509794,6.74232441627576,65.6380794164023));
#144973=CARTESIAN_POINT('Ctrl Pts',(2.10033507315695,6.69179721122206,65.6297115758797));
#144974=CARTESIAN_POINT('Ctrl Pts',(2.27555525047154,6.63426370216071,65.6213437353571));
#144975=CARTESIAN_POINT('Ctrl Pts',(2.44828798850789,6.56989440461778,65.6129758948345));
#144976=CARTESIAN_POINT('Ctrl Pts',(2.62095324941255,6.50555025260092,65.6046113231646));
#144977=CARTESIAN_POINT('Ctrl Pts',(2.79113270119106,6.4343757518059,65.5962467514946));
#144978=CARTESIAN_POINT('Ctrl Pts',(2.95827334528979,6.35659070391102,65.5878821798247));
#144979=CARTESIAN_POINT('Ctrl Pts',(3.12537316213467,6.27882465648077,65.5795196513592));
#144980=CARTESIAN_POINT('Ctrl Pts',(3.28943535404691,6.19445142110524,65.5711571228936));
#144981=CARTESIAN_POINT('Ctrl Pts',(3.44992815626778,6.10373838553806,65.5627945944281));
#144982=CARTESIAN_POINT('Ctrl Pts',(3.61043376631636,6.01301811078685,65.5544313986066));
#144983=CARTESIAN_POINT('Ctrl Pts',(3.76736912848605,5.91595718152013,65.5460682027851));
#144984=CARTESIAN_POINT('Ctrl Pts',(3.92022761568842,5.81286865529352,65.5377050069636));
#144985=CARTESIAN_POINT('Ctrl Pts',(4.07309652753306,5.70977309863617,65.5293412407889));
#144986=CARTESIAN_POINT('Ctrl Pts',(4.22188773726402,5.60064930901317,65.5209774746142));
#144987=CARTESIAN_POINT('Ctrl Pts',(4.36612398129579,5.4858534379305,65.5126137084395));
#144988=CARTESIAN_POINT('Ctrl Pts',(4.51038929203538,5.37103443300884,65.5042482567859));
#144989=CARTESIAN_POINT('Ctrl Pts',(4.65009754946804,5.25054127212033,65.4958828051323));
#144990=CARTESIAN_POINT('Ctrl Pts',(4.78480460372754,5.12477038184617,65.4875173534787));
#144991=CARTESIAN_POINT('Ctrl Pts',(4.91955677111448,4.99895737114831,65.4791491002518));
#144992=CARTESIAN_POINT('Ctrl Pts',(5.04930415532039,4.8678633309057,65.4707808470249));
#144993=CARTESIAN_POINT('Ctrl Pts',(5.17363919568747,4.73192181204913,65.462412593798));
#144994=CARTESIAN_POINT('Ctrl Pts',(5.29808951237505,4.59585425601068,65.4540365820066));
#144995=CARTESIAN_POINT('Ctrl Pts',(5.41711723560646,4.45493048325975,65.4456605702151));
#144996=CARTESIAN_POINT('Ctrl Pts',(5.53035406854319,4.30961836350364,65.4372845584236));
#144997=CARTESIAN_POINT('Ctrl Pts',(5.6436464342218,4.16423498088871,65.4289044389325));
#144998=CARTESIAN_POINT('Ctrl Pts',(5.75114204944297,4.01445922275958,65.4205243194413));
#144999=CARTESIAN_POINT('Ctrl Pts',(5.85251540364741,3.86078878113913,65.4121441999502));
#145000=CARTESIAN_POINT('Ctrl Pts',(5.95400458975026,3.70694275157331,65.403754505111));
#145001=CARTESIAN_POINT('Ctrl Pts',(6.04935736083194,3.54919342423773,65.3953648102718));
#145002=CARTESIAN_POINT('Ctrl Pts',(6.13829302306579,3.38806513005312,65.3869751154326));
#145003=CARTESIAN_POINT('Ctrl Pts',(6.19475674027863,3.2857675566241,65.381648642958));
#145004=CARTESIAN_POINT('Ctrl Pts',(6.24863480532168,3.18210848944696,65.3763221704833));
#145005=CARTESIAN_POINT('Ctrl Pts',(6.29986537417107,3.07722648334834,65.3709956980087));
#145006=CARTESIAN_POINT('Ctrl Pts',(6.38141373562198,2.91027624377222,65.3625170667466));
#145007=CARTESIAN_POINT('Ctrl Pts',(6.45641141732215,2.73989902163659,65.3540384354846));
#145008=CARTESIAN_POINT('Ctrl Pts',(6.52457226502016,2.56662878520243,65.3455598042225));
#145009=CARTESIAN_POINT('Ctrl Pts',(6.54045669722058,2.52624930906705,65.3435839156005));
#145010=CARTESIAN_POINT('Ctrl Pts',(6.55597001641838,2.48571283255154,65.3416080269784));
#145011=CARTESIAN_POINT('Ctrl Pts',(6.57110895151811,2.44502632087645,65.3396321383564));
#145012=CARTESIAN_POINT('Origin',(0.,0.,50.));
#145013=CARTESIAN_POINT('',(6.57110895151814,2.44502632087636,63.3399907370491));
#145014=CARTESIAN_POINT('',(6.57110895151817,2.44502632087628,63.8871110093167));
#145015=CARTESIAN_POINT('',(6.57110895151814,2.44502632087636,50.));
#145016=CARTESIAN_POINT('',(7.01124989960866,-0.00118648116582599,65.7735343569499));
#145017=CARTESIAN_POINT('Ctrl Pts',(6.57110895151817,2.44502632087628,63.8871110093167));
#145018=CARTESIAN_POINT('Ctrl Pts',(6.49699556480479,2.64420910050587,63.8967749832153));
#145019=CARTESIAN_POINT('Ctrl Pts',(6.41376271381867,2.84017939726017,63.9064389571139));
#145020=CARTESIAN_POINT('Ctrl Pts',(6.32167067777122,3.03217849149875,63.9161029310125));
#145021=CARTESIAN_POINT('Ctrl Pts',(6.26326411714714,3.15394805180726,63.9222320112414));
#145022=CARTESIAN_POINT('Ctrl Pts',(6.2012950942145,3.27412045456893,63.9283610914703));
#145023=CARTESIAN_POINT('Ctrl Pts',(6.13584066416528,3.39250437088529,63.9344901716992));
#145024=CARTESIAN_POINT('Ctrl Pts',(6.05198825043598,3.54416373332095,63.9423420187132));
#145025=CARTESIAN_POINT('Ctrl Pts',(5.96244740792769,3.69282388792006,63.9501938657272));
#145026=CARTESIAN_POINT('Ctrl Pts',(5.86747435681217,3.83801657560928,63.9580457127412));
#145027=CARTESIAN_POINT('Ctrl Pts',(5.77252823928607,3.9831680878262,63.9658953330348));
#145028=CARTESIAN_POINT('Ctrl Pts',(5.67215318614176,4.12485377025659,63.9737449533285));
#145029=CARTESIAN_POINT('Ctrl Pts',(5.56665003842499,4.26263227503887,63.9815945736221));
#145030=CARTESIAN_POINT('Ctrl Pts',(5.46115531378514,4.40039977996978,63.989443567224));
#145031=CARTESIAN_POINT('Ctrl Pts',(5.3505335421151,4.53426042582434,63.9972925608259));
#145032=CARTESIAN_POINT('Ctrl Pts',(5.23512717181703,4.6638042473289,64.0051415544278));
#145033=CARTESIAN_POINT('Ctrl Pts',(5.11966237465312,4.79341365307686,64.0129945217452));
#145034=CARTESIAN_POINT('Ctrl Pts',(4.99940839305648,4.91870158257157,64.0208474890627));
#145035=CARTESIAN_POINT('Ctrl Pts',(4.87474625455506,5.03929315640611,64.0287004563802));
#145036=CARTESIAN_POINT('Ctrl Pts',(4.75005245605922,5.15991535644842,64.0365554180875));
#145037=CARTESIAN_POINT('Ctrl Pts',(4.62094855417452,5.27583856977249,64.0444103797949));
#145038=CARTESIAN_POINT('Ctrl Pts',(4.48784978044503,5.38672729128359,64.0522653415022));
#145039=CARTESIAN_POINT('Ctrl Pts',(4.35461889505698,5.49772607911991,64.0601280999156));
#145040=CARTESIAN_POINT('Ctrl Pts',(4.21738552003268,5.60368016153394,64.067990858329));
#145041=CARTESIAN_POINT('Ctrl Pts',(4.07659552790009,5.70429622866879,64.0758536167424));
#145042=CARTESIAN_POINT('Ctrl Pts',(3.97331400989568,5.77810673175863,64.0816216234902));
#145043=CARTESIAN_POINT('Ctrl Pts',(3.86811914000701,5.8490454825764,64.0873896302379));
#145044=CARTESIAN_POINT('Ctrl Pts',(3.76119543936221,5.91701237360722,64.0931576369857));
#145045=CARTESIAN_POINT('Ctrl Pts',(3.60588808496837,6.01573471457292,64.1015357034267));
#145046=CARTESIAN_POINT('Ctrl Pts',(3.44658844908732,6.10840427875473,64.1099137698677));
#145047=CARTESIAN_POINT('Ctrl Pts',(3.28379637756845,6.19469998572718,64.1182918363087));
#145048=CARTESIAN_POINT('Ctrl Pts',(3.12111562133356,6.28093668472069,64.1266641739275));
#145049=CARTESIAN_POINT('Ctrl Pts',(2.95494748011205,6.36080806232983,64.1350365115462));
#145050=CARTESIAN_POINT('Ctrl Pts',(2.78581836668239,6.43403781387358,64.143408849165));
#145051=CARTESIAN_POINT('Ctrl Pts',(2.61678009883506,6.50722823097462,64.1517766896876));
#145052=CARTESIAN_POINT('Ctrl Pts',(2.4447843309715,6.57378400487815,64.1601445302101));
#145053=CARTESIAN_POINT('Ctrl Pts',(2.27037993859189,6.63347582319703,64.1685123707327));
#145054=CARTESIAN_POINT('Ctrl Pts',(2.09604367636636,6.69314432322258,64.1768769424027));
#145055=CARTESIAN_POINT('Ctrl Pts',(1.9193009764892,6.74595410840701,64.1852415140726));
#145056=CARTESIAN_POINT('Ctrl Pts',(1.74071888858968,6.79172469358168,64.1936060857425));
#145057=CARTESIAN_POINT('Ctrl Pts',(1.56218042273221,6.83748409842793,64.2019686142081));
#145058=CARTESIAN_POINT('Ctrl Pts',(1.38180378309591,6.8762076511627,64.2103311426736));
#145059=CARTESIAN_POINT('Ctrl Pts',(1.20016975602968,6.90776513202437,64.2186936711392));
#145060=CARTESIAN_POINT('Ctrl Pts',(1.01852123399991,6.93932513127173,64.2270568669607));
#145061=CARTESIAN_POINT('Ctrl Pts',(0.835615446852659,6.96371785390755,
64.2354200627822));
#145062=CARTESIAN_POINT('Ctrl Pts',(0.652042683505307,6.98086433770111,
64.2437832586038));
#145063=CARTESIAN_POINT('Ctrl Pts',(0.468457400863388,6.99801199085052,
64.2521470247785));
#145064=CARTESIAN_POINT('Ctrl Pts',(0.284205378697097,7.00791238895935,
64.2605107909532));
#145065=CARTESIAN_POINT('Ctrl Pts',(0.0998815072616129,7.01053851333884,
64.2688745571279));
#145066=CARTESIAN_POINT('Ctrl Pts',(-0.0844795094002239,7.01316516693891,
64.2772400087814));
#145067=CARTESIAN_POINT('Ctrl Pts',(-0.268912075450465,7.00851461905334,
64.285605460435));
#145068=CARTESIAN_POINT('Ctrl Pts',(-0.452821386676459,6.99661199111888,
64.2939709120886));
#145069=CARTESIAN_POINT('Ctrl Pts',(-0.636792288769149,6.98470537701773,
64.3023391653154));
#145070=CARTESIAN_POINT('Ctrl Pts',(-0.820239258643475,6.96554186118294,
64.3107074185423));
#145071=CARTESIAN_POINT('Ctrl Pts',(-1.00257226334398,6.93919847095278,
64.3190756717692));
#145072=CARTESIAN_POINT('Ctrl Pts',(-1.18507431675252,6.91283065664157,
64.3274516835606));
#145073=CARTESIAN_POINT('Ctrl Pts',(-1.36646001539432,6.87926971279002,
64.3358276953521));
#145074=CARTESIAN_POINT('Ctrl Pts',(-1.54614794455558,6.838644097776,64.3442037071436));
#145075=CARTESIAN_POINT('Ctrl Pts',(-1.7259239948975,6.79799855945842,64.3525838266348));
#145076=CARTESIAN_POINT('Ctrl Pts',(-1.90400029633763,6.75028151973062,
64.3609639461259));
#145077=CARTESIAN_POINT('Ctrl Pts',(-2.07980962689622,6.6956716226507,64.3693440656171));
#145078=CARTESIAN_POINT('Ctrl Pts',(-2.25581984188537,6.64099932684573,
64.3777337604563));
#145079=CARTESIAN_POINT('Ctrl Pts',(-2.42955759793582,6.57941853965959,
64.3861234552955));
#145080=CARTESIAN_POINT('Ctrl Pts',(-2.60047345402352,6.51115691543515,
64.3945131501347));
#145081=CARTESIAN_POINT('Ctrl Pts',(-2.70898498160349,6.46781878818801,
64.3998396226093));
#145082=CARTESIAN_POINT('Ctrl Pts',(-2.81635948020824,6.42178874201956,
64.405166095084));
#145083=CARTESIAN_POINT('Ctrl Pts',(-2.92246129635095,6.37313474938595,
64.4104925675586));
#145084=CARTESIAN_POINT('Ctrl Pts',(-3.08941441566581,6.29657681538813,
64.4188738679634));
#145085=CARTESIAN_POINT('Ctrl Pts',(-3.25355202745307,6.21336537748386,
64.4272551683682));
#145086=CARTESIAN_POINT('Ctrl Pts',(-3.41432559771735,6.1237249509814,64.435636468773));
#145087=CARTESIAN_POINT('Ctrl Pts',(-3.57489541101686,6.03419813059712,
64.4440071471065));
#145088=CARTESIAN_POINT('Ctrl Pts',(-3.73210939551151,5.9382587176033,64.45237782544));
#145089=CARTESIAN_POINT('Ctrl Pts',(-3.88543996298573,5.83617878894517,
64.4607485037735));
#145090=CARTESIAN_POINT('Ctrl Pts',(-4.03859652659142,5.73421470347981,
64.4691096828242));
#145091=CARTESIAN_POINT('Ctrl Pts',(-4.18787818575637,5.62612417167076,
64.4774708618749));
#145092=CARTESIAN_POINT('Ctrl Pts',(-4.33278251431195,5.51222480003969,
64.4858320409257));
#145093=CARTESIAN_POINT('Ctrl Pts',(-4.47749881240839,5.39847322627882,
64.4941823703603));
#145094=CARTESIAN_POINT('Ctrl Pts',(-4.61784885308061,5.27892804887209,
64.502532699795));
#145095=CARTESIAN_POINT('Ctrl Pts',(-4.75335979999926,5.15394966741537,
64.5108830292296));
#145096=CARTESIAN_POINT('Ctrl Pts',(-4.88876647935039,5.0290674493471,64.5192269335852));
#145097=CARTESIAN_POINT('Ctrl Pts',(-5.01934124516012,4.89876057944643,
64.5275708379409));
#145098=CARTESIAN_POINT('Ctrl Pts',(-5.14464404037652,4.76342988405606,
64.5359147422965));
#145099=CARTESIAN_POINT('Ctrl Pts',(-5.26984619160639,4.62820788712418,
64.5442519447762));
#145100=CARTESIAN_POINT('Ctrl Pts',(-5.38978459534836,4.48797035199404,
64.5525891472558));
#145101=CARTESIAN_POINT('Ctrl Pts',(-5.50405569879128,4.3431552386604,64.5609263497354));
#145102=CARTESIAN_POINT('Ctrl Pts',(-5.54167311528961,4.29548290270325,
64.5636709107719));
#145103=CARTESIAN_POINT('Ctrl Pts',(-5.5786766731508,4.24731479165283,64.5664154718084));
#145104=CARTESIAN_POINT('Ctrl Pts',(-5.61505288383781,4.19866736884511,
64.5691600328449));
#145105=CARTESIAN_POINT('Ctrl Pts',(-5.72556823703457,4.05087058044496,
64.5774983431469));
#145106=CARTESIAN_POINT('Ctrl Pts',(-5.83019934000538,3.89876854557725,
64.5858366534489));
#145107=CARTESIAN_POINT('Ctrl Pts',(-5.92862524299052,3.74286378200912,
64.5941749637509));
#145108=CARTESIAN_POINT('Ctrl Pts',(-6.02711307221399,3.58686092845398,
64.6025185202348));
#145109=CARTESIAN_POINT('Ctrl Pts',(-6.11938773932444,3.42705085102124,
64.6108620767187));
#145110=CARTESIAN_POINT('Ctrl Pts',(-6.20517366433518,3.26396175803901,
64.6192056332026));
#145111=CARTESIAN_POINT('Ctrl Pts',(-6.29102485490372,3.10074858758575,
64.6275555374279));
#145112=CARTESIAN_POINT('Ctrl Pts',(-6.3703773040939,2.93425171520219,64.6359054416531));
#145113=CARTESIAN_POINT('Ctrl Pts',(-6.44300289214442,2.76502084880361,
64.6442553458784));
#145114=CARTESIAN_POINT('Ctrl Pts',(-6.5157374132027,2.59553614862856,64.6526177743421));
#145115=CARTESIAN_POINT('Ctrl Pts',(-6.58172478121225,2.4233095611296,64.6609802028059));
#145116=CARTESIAN_POINT('Ctrl Pts',(-6.64078572321868,2.24890896676476,
64.6693426312696));
#145117=CARTESIAN_POINT('Ctrl Pts',(-6.69989717038178,2.07435923611729,
64.6777122107497));
#145118=CARTESIAN_POINT('Ctrl Pts',(-6.75207028099807,1.89763210276973,
64.6860817902297));
#145119=CARTESIAN_POINT('Ctrl Pts',(-6.79717641354589,1.71930781584782,
64.6944513697098));
#145120=CARTESIAN_POINT('Ctrl Pts',(-6.84235211680747,1.54070848544023,
64.7028338582464));
#145121=CARTESIAN_POINT('Ctrl Pts',(-6.88043899302143,1.36050739876751,
64.711216346783));
#145122=CARTESIAN_POINT('Ctrl Pts',(-6.91135973018643,1.17929353532417,
64.7195988353197));
#145123=CARTESIAN_POINT('Ctrl Pts',(-6.92147750205127,1.11999738985123,
64.7223417229236));
#145124=CARTESIAN_POINT('Ctrl Pts',(-6.93082840628621,1.06059283281779,
64.7250846105275));
#145125=CARTESIAN_POINT('Ctrl Pts',(-6.9394109443965,1.00110054804204,64.7278274981314));
#145126=CARTESIAN_POINT('Ctrl Pts',(-6.96566293201509,0.819127487944456,
64.7362173532642));
#145127=CARTESIAN_POINT('Ctrl Pts',(-6.98477516963699,0.635966017425455,
64.744607208397));
#145128=CARTESIAN_POINT('Ctrl Pts',(-6.99665206940565,0.452201705195453,
64.7529970635297));
#145129=CARTESIAN_POINT('Ctrl Pts',(-7.0085180093377,0.268606968096569,
64.7613791766218));
#145130=CARTESIAN_POINT('Ctrl Pts',(-7.01316190024731,0.0844108247160268,
64.7697612897139));
#145131=CARTESIAN_POINT('Ctrl Pts',(-7.0105397529384,-0.0997944636261545,
64.778143402806));
#145132=CARTESIAN_POINT('Ctrl Pts',(-7.00791963986005,-0.283856847705757,
64.7865190131549));
#145133=CARTESIAN_POINT('Ctrl Pts',(-6.99804473149794,-0.467928035088668,
64.7948946235037));
#145134=CARTESIAN_POINT('Ctrl Pts',(-6.98092305719585,-0.651413718009799,
64.8032702338526));
#145135=CARTESIAN_POINT('Ctrl Pts',(-6.96381215268117,-0.834783985711531,
64.8116405758181));
#145136=CARTESIAN_POINT('Ctrl Pts',(-6.93946360157776,-1.01756915682932,
64.8200109177837));
#145137=CARTESIAN_POINT('Ctrl Pts',(-6.90793744792476,-1.19917754234256,
64.8283812597493));
#145138=CARTESIAN_POINT('Ctrl Pts',(-6.87642650331046,-1.38069831523444,
64.8367475636436));
#145139=CARTESIAN_POINT('Ctrl Pts',(-6.83774491738015,-1.5610431113291,
64.8451138675379));
#145140=CARTESIAN_POINT('Ctrl Pts',(-6.79200432150243,-1.73962750587371,
64.8534801714322));
#145141=CARTESIAN_POINT('Ctrl Pts',(-6.74627651798734,-1.91816195536857,
64.8618441355058));
#145142=CARTESIAN_POINT('Ctrl Pts',(-6.69349372114037,-2.09493666656742,
64.8702080995794));
#145143=CARTESIAN_POINT('Ctrl Pts',(-6.63381833132686,-2.26937896999415,
64.878572063653));
#145144=CARTESIAN_POINT('Ctrl Pts',(-6.57415212456416,-2.44379442964924,
64.8869347406516));
#145145=CARTESIAN_POINT('Ctrl Pts',(-6.507595545918,-2.61587788626935,64.8952974176501));
#145146=CARTESIAN_POINT('Ctrl Pts',(-6.43436051072568,-2.78507295784401,
64.9036600946486));
#145147=CARTESIAN_POINT('Ctrl Pts',(-6.36112698330889,-2.95426454600137,
64.9120225994749));
#145148=CARTESIAN_POINT('Ctrl Pts',(-6.28121540443332,-3.12056756624219,
64.9203851043012));
#145149=CARTESIAN_POINT('Ctrl Pts',(-6.19488554340462,-3.28344630938537,
64.9287476091275));
#145150=CARTESIAN_POINT('Ctrl Pts',(-6.10854595259397,-3.44634340973008,
64.9371110564475));
#145151=CARTESIAN_POINT('Ctrl Pts',(-6.01578679181504,-3.60581517341989,
64.9454745037674));
#145152=CARTESIAN_POINT('Ctrl Pts',(-5.91691362818464,-3.76135077852397,
64.9538379510874));
#145153=CARTESIAN_POINT('Ctrl Pts',(-5.81798224525687,-3.91697796736334,
64.9622063230402));
#145154=CARTESIAN_POINT('Ctrl Pts',(-5.71292984131665,-4.06866408809416,
64.970574694993));
#145155=CARTESIAN_POINT('Ctrl Pts',(-5.60210571352749,-4.2159267233863,
64.9789430669458));
#145156=CARTESIAN_POINT('Ctrl Pts',(-5.49124837993321,-4.36323348241272,
64.9873139462815));
#145157=CARTESIAN_POINT('Ctrl Pts',(-5.37461607608116,-4.50611385372882,
64.9956848256173));
#145158=CARTESIAN_POINT('Ctrl Pts',(-5.25259863229461,-4.644118233908,65.004055704953));
#145159=CARTESIAN_POINT('Ctrl Pts',(-5.13047780444739,-4.78223954370618,
65.0124336768443));
#145160=CARTESIAN_POINT('Ctrl Pts',(-5.00296294133329,-4.91547636429601,
65.0208116487355));
#145161=CARTESIAN_POINT('Ctrl Pts',(-4.87048179501422,-5.04341487951716,
65.0291896206268));
#145162=CARTESIAN_POINT('Ctrl Pts',(-4.78628894772784,-5.12472084774993,
65.034513889986));
#145163=CARTESIAN_POINT('Ctrl Pts',(-4.700091096312,-5.20388774030555,65.0398381593451));
#145164=CARTESIAN_POINT('Ctrl Pts',(-4.61200508624651,-5.28081770627773,
65.0451624287043));
#145165=CARTESIAN_POINT('Ctrl Pts',(-4.48192049048981,-5.39442716046491,
65.0530252598936));
#145166=CARTESIAN_POINT('Ctrl Pts',(-4.34744573065318,-5.50339217667704,
65.0608880910829));
#145167=CARTESIAN_POINT('Ctrl Pts',(-4.20896128643903,-5.60734085389478,
65.0687509222722));
#145168=CARTESIAN_POINT('Ctrl Pts',(-4.07058324924061,-5.71120966027509,
65.0766077119136));
#145169=CARTESIAN_POINT('Ctrl Pts',(-3.92820195745968,-5.81006956527485,
65.084464501555));
#145170=CARTESIAN_POINT('Ctrl Pts',(-3.78223311581931,-5.90358697912547,
65.0923212911965));
#145171=CARTESIAN_POINT('Ctrl Pts',(-3.63634659369579,-5.99705165358157,
65.1001736499804));
#145172=CARTESIAN_POINT('Ctrl Pts',(-3.48687686637413,-6.08517962522453,
65.1080260087644));
#145173=CARTESIAN_POINT('Ctrl Pts',(-3.33427073827808,-6.16767907777006,
65.1158783675484));
#145174=CARTESIAN_POINT('Ctrl Pts',(-3.18170064226957,-6.2501590512322,
65.1237288722988));
#145175=CARTESIAN_POINT('Ctrl Pts',(-3.02599595044965,-6.32701296201912,
65.1315793770493));
#145176=CARTESIAN_POINT('Ctrl Pts',(-2.86763027164455,-6.39799368455829,
65.1394298817997));
#145177=CARTESIAN_POINT('Ctrl Pts',(-2.70929006888577,-6.4689629885364,
65.1472791236514));
#145178=CARTESIAN_POINT('Ctrl Pts',(-2.54829008068934,-6.53406083180514,
65.1551283655031));
#145179=CARTESIAN_POINT('Ctrl Pts',(-2.38512577784746,-6.59308740927553,
65.1629776073547));
#145180=CARTESIAN_POINT('Ctrl Pts',(-2.22190650175832,-6.65213387395521,
65.1708294937696));
#145181=CARTESIAN_POINT('Ctrl Pts',(-2.05652181357907,-6.70510485711426,
65.1786813801845));
#145182=CARTESIAN_POINT('Ctrl Pts',(-1.88948448864171,-6.75184974134366,
65.1865332665994));
#145183=CARTESIAN_POINT('Ctrl Pts',(-1.76683106001611,-6.78617392801027,
65.1922988090632));
#145184=CARTESIAN_POINT('Ctrl Pts',(-1.64328693965486,-6.81714216116263,
65.198064351527));
#145185=CARTESIAN_POINT('Ctrl Pts',(-1.51905916835793,-6.84471225147761,
65.2038298939908));
#145186=CARTESIAN_POINT('Ctrl Pts',(-1.31102029789007,-6.89088268815167,
65.2134851983505));
#145187=CARTESIAN_POINT('Ctrl Pts',(-1.1011701447253,-6.9274989208654,65.2231405027102));
#145188=CARTESIAN_POINT('Ctrl Pts',(-0.890310616200778,-6.95449304904248,
65.2327958070699));
#145189=CARTESIAN_POINT('Ctrl Pts',(-0.678282965444561,-6.98163671962568,
65.2425046000045));
#145190=CARTESIAN_POINT('Ctrl Pts',(-0.46523477859497,-6.9990514293502,
65.2522133929391));
#145191=CARTESIAN_POINT('Ctrl Pts',(-0.251976881867445,-7.00672064617281,
65.2619221858737));
#145192=CARTESIAN_POINT('Ctrl Pts',(-0.0376927700335318,-7.01442676791796,
65.2716776983442));
#145193=CARTESIAN_POINT('Ctrl Pts',(0.176803030718485,-7.01229340123862,
65.2814332108148));
#145194=CARTESIAN_POINT('Ctrl Pts',(0.390693177417793,-7.0003560912013,
65.2911887232853));
#145195=CARTESIAN_POINT('Ctrl Pts',(0.604795108269136,-6.9884069613905,
65.3009538952141));
#145196=CARTESIAN_POINT('Ctrl Pts',(0.818290147891335,-6.96663448447612,
65.3107190671429));
#145197=CARTESIAN_POINT('Ctrl Pts',(1.03036436573623,-6.93512623074166,
65.3204842390716));
#145198=CARTESIAN_POINT('Ctrl Pts',(1.24214942519621,-6.90366093779636,
65.33023609641));
#145199=CARTESIAN_POINT('Ctrl Pts',(1.45251749723369,-6.86248640462504,
65.3399879537484));
#145200=CARTESIAN_POINT('Ctrl Pts',(1.66066434996332,-6.81174136908184,
65.3497398110867));
#145201=CARTESIAN_POINT('Ctrl Pts',(1.75143145248323,-6.78961285845041,
65.3539923271502));
#145202=CARTESIAN_POINT('Ctrl Pts',(1.84177625502004,-6.76566509059098,
65.3582448432137));
#145203=CARTESIAN_POINT('Ctrl Pts',(1.93163247853033,-6.73991265005614,
65.3624973592771));
#145204=CARTESIAN_POINT('Ctrl Pts',(2.10137178816044,-6.69126603096945,
65.370530404876));
#145205=CARTESIAN_POINT('Ctrl Pts',(2.26944946600706,-6.63615233030069,
65.3785634504749));
#145206=CARTESIAN_POINT('Ctrl Pts',(2.4353310461155,-6.5747083021474,65.3865964960738));
#145207=CARTESIAN_POINT('Ctrl Pts',(2.60110599115723,-6.51330377258123,
65.3946243777217));
#145208=CARTESIAN_POINT('Ctrl Pts',(2.76468730624415,-6.44557714252209,
65.4026522593695));
#145209=CARTESIAN_POINT('Ctrl Pts',(2.925555093882,-6.37171515019002,65.4106801410174));
#145210=CARTESIAN_POINT('Ctrl Pts',(3.08635024812813,-6.29788650727552,
65.4187043979976));
#145211=CARTESIAN_POINT('Ctrl Pts',(3.24443398196679,-6.21792817046698,
65.4267286549777));
#145212=CARTESIAN_POINT('Ctrl Pts',(3.39930586598422,-6.13207519458016,
65.4347529119579));
#145213=CARTESIAN_POINT('Ctrl Pts',(3.55415902441318,-6.04623259919271,
65.4427761987237));
#145214=CARTESIAN_POINT('Ctrl Pts',(3.70580078238414,-5.95449695522676,
65.4507994854895));
#145215=CARTESIAN_POINT('Ctrl Pts',(3.853754685903,-5.85714959544151,65.4588227722552));
#145216=CARTESIAN_POINT('Ctrl Pts',(4.00169646591944,-5.75981021240392,
65.4668454015842));
#145217=CARTESIAN_POINT('Ctrl Pts',(4.14595068932674,-5.65686023436843,
65.4748680309132));
#145218=CARTESIAN_POINT('Ctrl Pts',(4.28606956809203,-5.54862453406026,
65.4828906602422));
#145219=CARTESIAN_POINT('Ctrl Pts',(4.42624112158021,-5.44034814483443,
65.4909163055087));
#145220=CARTESIAN_POINT('Ctrl Pts',(4.56227393640459,-5.32678229047758,
65.4989419507751));
#145221=CARTESIAN_POINT('Ctrl Pts',(4.69375273000823,-5.2082926062233,65.5069675960416));
#145222=CARTESIAN_POINT('Ctrl Pts',(4.77128063863112,-5.13842386798926,
65.5117000055489));
#145223=CARTESIAN_POINT('Ctrl Pts',(4.84722576033643,-5.06684386172466,
65.5164324150562));
#145224=CARTESIAN_POINT('Ctrl Pts',(4.92150891237859,-4.99363360569016,
65.5211648245635));
#145225=CARTESIAN_POINT('Ctrl Pts',(5.058541758735,-4.85857996982404,65.529894873398));
#145226=CARTESIAN_POINT('Ctrl Pts',(5.18998549790365,-4.71790921937674,
65.5386249222326));
#145227=CARTESIAN_POINT('Ctrl Pts',(5.31540476153175,-4.57210004085493,
65.5473549710671));
#145228=CARTESIAN_POINT('Ctrl Pts',(5.44086029029623,-4.42624870142743,
65.5560875442061));
#145229=CARTESIAN_POINT('Ctrl Pts',(5.56028768778448,-4.27525617590496,
65.5648201173452));
#145230=CARTESIAN_POINT('Ctrl Pts',(5.67329161435357,-4.11963454944798,
65.5735526904842));
#145231=CARTESIAN_POINT('Ctrl Pts',(5.78790094209027,-3.9618020693649,65.5824093237647));
#145232=CARTESIAN_POINT('Ctrl Pts',(5.89590272628379,-3.79920819291018,
65.5912659570452));
#145233=CARTESIAN_POINT('Ctrl Pts',(5.99692954073015,-3.63241829171946,
65.6001225903256));
#145234=CARTESIAN_POINT('Ctrl Pts',(6.09660462300902,-3.46786002849424,
65.6088607224323));
#145235=CARTESIAN_POINT('Ctrl Pts',(6.18949010158144,-3.2992175778555,65.6175988545389));
#145236=CARTESIAN_POINT('Ctrl Pts',(6.27527851617244,-3.12706029794192,
65.6263369866456));
#145237=CARTESIAN_POINT('Ctrl Pts',(6.36281204534399,-2.95140098129346,
65.635252870513));
#145238=CARTESIAN_POINT('Ctrl Pts',(6.44295654417856,-2.77208256922448,
65.6441687543804));
#145239=CARTESIAN_POINT('Ctrl Pts',(6.51543584224807,-2.58973403036861,
65.6530846382478));
#145240=CARTESIAN_POINT('Ctrl Pts',(6.58791514031757,-2.40738549151275,
65.6620005221152));
#145241=CARTESIAN_POINT('Ctrl Pts',(6.65272913157334,-2.22200710914342,
65.6709164059825));
#145242=CARTESIAN_POINT('Ctrl Pts',(6.70965433379166,-2.03424808799978,
65.6798322898499));
#145243=CARTESIAN_POINT('Ctrl Pts',(6.76495279891978,-1.85185460886237,
65.6884933867616));
#145244=CARTESIAN_POINT('Ctrl Pts',(6.81281612486858,-1.66718451891293,
65.6971544836732));
#145245=CARTESIAN_POINT('Ctrl Pts',(6.85308001335165,-1.48085140817713,
65.7058155805848));
#145246=CARTESIAN_POINT('Ctrl Pts',(6.89333506400459,-1.29455919712691,
65.7144747764058));
#145247=CARTESIAN_POINT('Ctrl Pts',(6.92599394708081,-1.10660497444136,
65.7231339722267));
#145248=CARTESIAN_POINT('Ctrl Pts',(6.95094321879162,-0.917613715914716,
65.7317931680476));
#145249=CARTESIAN_POINT('Ctrl Pts',(6.97588795116692,-0.728656842950113,
65.7404507883919));
#145250=CARTESIAN_POINT('Ctrl Pts',(6.9931258345822,-0.538663595112505,
65.7491084087362));
#145251=CARTESIAN_POINT('Ctrl Pts',(7.00259503583784,-0.34826617199953,
65.7577660290805));
#145252=CARTESIAN_POINT('Ctrl Pts',(7.00834386225704,-0.232674401734254,
65.7630221383572));
#145253=CARTESIAN_POINT('Ctrl Pts',(7.01123031221653,-0.116933788902505,
65.7682782476338));
#145254=CARTESIAN_POINT('Ctrl Pts',(7.01124989960851,-0.00118648203415713,
65.7735343569105));
#145255=CARTESIAN_POINT('Ctrl Pts',(7.01124989960866,-0.00118648116572791,
65.77353435695));
#145256=CARTESIAN_POINT('Ctrl Pts',(7.0112840123165,0.200395074739239,65.7826882173262));
#145257=CARTESIAN_POINT('Ctrl Pts',(7.00262022694374,0.401968333003894,
65.7918420777024));
#145258=CARTESIAN_POINT('Ctrl Pts',(6.98528696966447,0.60282046575725,65.8009959380786));
#145259=CARTESIAN_POINT('Ctrl Pts',(6.96796416523818,0.803551474259107,
65.8101442782024));
#145260=CARTESIAN_POINT('Ctrl Pts',(6.94198235287763,1.00356203563452,65.8192926183262));
#145261=CARTESIAN_POINT('Ctrl Pts',(6.90742184975187,1.20214389823782,65.8284409584499));
#145262=CARTESIAN_POINT('Ctrl Pts',(6.89475517763354,1.27492557427682,65.8317938906788));
#145263=CARTESIAN_POINT('Ctrl Pts',(6.88093665414608,1.34751538295692,65.8351468229076));
#145264=CARTESIAN_POINT('Ctrl Pts',(6.86597197759889,1.41987864457733,65.8384997551364));
#145265=CARTESIAN_POINT('Ctrl Pts',(6.82996706766942,1.59398415956331,65.8465668872604));
#145266=CARTESIAN_POINT('Ctrl Pts',(6.7873122578682,1.76683134930017,65.8546340193843));
#145267=CARTESIAN_POINT('Ctrl Pts',(6.73812170080834,1.93787061167553,65.8627011515083));
#145268=CARTESIAN_POINT('Ctrl Pts',(6.68893114374847,2.10890987405096,65.8707682836323));
#145269=CARTESIAN_POINT('Ctrl Pts',(6.63320492220022,2.27814084184561,65.8788354157562));
#145270=CARTESIAN_POINT('Ctrl Pts',(6.57110895151813,2.44502632087639,65.8869025478802));
#145271=CARTESIAN_POINT('',(7.01124984252467,0.00148600060135456,65.226465643127));
#145272=CARTESIAN_POINT('Ctrl Pts',(6.57110895151811,2.44502632087645,65.3396321383564));
#145273=CARTESIAN_POINT('Ctrl Pts',(6.6359526070107,2.27075632573637,65.3311689379889));
#145274=CARTESIAN_POINT('Ctrl Pts',(6.69392407376079,2.09373197228993,65.3227057376215));
#145275=CARTESIAN_POINT('Ctrl Pts',(6.74479490719116,1.91451514029745,65.314242537254));
#145276=CARTESIAN_POINT('Ctrl Pts',(6.79557866611771,1.73560506987483,65.3057938231633));
#145277=CARTESIAN_POINT('Ctrl Pts',(6.8392859518127,1.55451030828681,65.2973451090727));
#145278=CARTESIAN_POINT('Ctrl Pts',(6.87573731344327,1.37181010312068,65.288896394982));
#145279=CARTESIAN_POINT('Ctrl Pts',(6.91215146763154,1.18929638776006,65.2804563048501));
#145280=CARTESIAN_POINT('Ctrl Pts',(6.94132439855923,1.00518080182279,65.2720162147183));
#145281=CARTESIAN_POINT('Ctrl Pts',(6.96312671381785,0.820056662564405,
65.2635761245864));
#145282=CARTESIAN_POINT('Ctrl Pts',(6.98490210623169,0.635161126021161,
65.2551464567989));
#145283=CARTESIAN_POINT('Ctrl Pts',(6.99932500152693,0.44925983156964,65.2467167890113));
#145284=CARTESIAN_POINT('Ctrl Pts',(7.00631723022827,0.262955189921164,
65.2382871212238));
#145285=CARTESIAN_POINT('Ctrl Pts',(7.0095857844396,0.17586610186922,65.2343466285248));
#145286=CARTESIAN_POINT('Ctrl Pts',(7.01123136026748,0.0886890089352705,
65.2304061358259));
#145287=CARTESIAN_POINT('Ctrl Pts',(7.01124984252467,0.00148600060139123,
65.2264656431269));
#145288=CARTESIAN_POINT('Ctrl Pts',(7.01124984252485,0.00148599977491322,
65.2264656430896));
#145289=CARTESIAN_POINT('Ctrl Pts',(7.01127194560764,-0.102800850311695,
65.2217531729671));
#145290=CARTESIAN_POINT('Ctrl Pts',(7.00896671320105,-0.207099752355944,
65.2170407028447));
#145291=CARTESIAN_POINT('Ctrl Pts',(7.00433593370117,-0.311295182041935,
65.2123282327223));
#145292=CARTESIAN_POINT('Ctrl Pts',(6.99614216792538,-0.495660027264679,
65.2039899224206));
#145293=CARTESIAN_POINT('Ctrl Pts',(6.98066829470659,-0.679625393476375,
65.195651612119));
#145294=CARTESIAN_POINT('Ctrl Pts',(6.95798456722586,-0.862599168065245,
65.1873133018173));
#145295=CARTESIAN_POINT('Ctrl Pts',(6.93528656791354,-1.04568806354407,
65.1789697453337));
#145296=CARTESIAN_POINT('Ctrl Pts',(6.90536970664401,-1.22778379784101,
65.17062618885));
#145297=CARTESIAN_POINT('Ctrl Pts',(6.86835561249141,-1.40830314309731,
65.1622826323664));
#145298=CARTESIAN_POINT('Ctrl Pts',(6.8313133581775,-1.58895982668374,65.1539327281414));
#145299=CARTESIAN_POINT('Ctrl Pts',(6.78716316639149,-1.76803740838765,
65.1455828239164));
#145300=CARTESIAN_POINT('Ctrl Pts',(6.73607700273446,-1.94496611171812,
65.1372329196913));
#145301=CARTESIAN_POINT('Ctrl Pts',(6.68491421361207,-2.12216019501178,
65.1288704912278));
#145302=CARTESIAN_POINT('Ctrl Pts',(6.62679475423575,-2.29719864398295,
65.1205080627642));
#145303=CARTESIAN_POINT('Ctrl Pts',(6.56193989050479,-2.46952858576328,
65.1121456343007));
#145304=CARTESIAN_POINT('Ctrl Pts',(6.49702956702429,-2.64200589313594,
65.1037760548208));
#145305=CARTESIAN_POINT('Ctrl Pts',(6.42537247423215,-2.81176977086986,
65.095406475341));
#145306=CARTESIAN_POINT('Ctrl Pts',(6.34723688012722,-2.97828987005176,
65.0870368958611));
#145307=CARTESIAN_POINT('Ctrl Pts',(6.26898077138835,-3.14506680619798,
65.0786544073246));
#145308=CARTESIAN_POINT('Ctrl Pts',(6.18422634422477,-3.30858967570553,
65.0702719187882));
#145309=CARTESIAN_POINT('Ctrl Pts',(6.09328710268872,-3.46835391024436,
65.0618894302517));
#145310=CARTESIAN_POINT('Ctrl Pts',(6.06353029271894,-3.52063138569762,
65.0591465426463));
#145311=CARTESIAN_POINT('Ctrl Pts',(6.03311160924494,-3.57250666406741,
65.0564036550409));
#145312=CARTESIAN_POINT('Ctrl Pts',(6.00204300290693,-3.62396279696081,
65.0536607674355));
#145313=CARTESIAN_POINT('Ctrl Pts',(5.90701136331527,-3.78135513772773,
65.0452709123027));
#145314=CARTESIAN_POINT('Ctrl Pts',(5.80570400173806,-3.93514141930128,
65.0368810571698));
#145315=CARTESIAN_POINT('Ctrl Pts',(5.69841812432148,-4.08480812804034,
65.028491202037));
#145316=CARTESIAN_POINT('Ctrl Pts',(5.59123124880834,-4.23433672643904,
65.0201090889448));
#145317=CARTESIAN_POINT('Ctrl Pts',(5.47807704596437,-4.37975306437344,
65.0117269758526));
#145318=CARTESIAN_POINT('Ctrl Pts',(5.35929687460376,-4.52057115554688,
65.0033448627605));
#145319=CARTESIAN_POINT('Ctrl Pts',(5.24060885148161,-4.66128000172684,
64.9949692524116));
#145320=CARTESIAN_POINT('Ctrl Pts',(5.11630377263338,-4.79739746281312,
64.9865936420627));
#145321=CARTESIAN_POINT('Ctrl Pts',(4.98676452950537,-4.92846893971821,
64.9782180317138));
#145322=CARTESIAN_POINT('Ctrl Pts',(4.85730676848496,-5.0594579707179,64.9698476897481));
#145323=CARTESIAN_POINT('Ctrl Pts',(4.72262163834821,-5.18540711300072,
64.9614773477826));
#145324=CARTESIAN_POINT('Ctrl Pts',(4.58313060333516,-5.30589676070621,
64.953107005817));
#145325=CARTESIAN_POINT('Ctrl Pts',(4.44370686243555,-5.42632828106309,
64.9447407019226));
#145326=CARTESIAN_POINT('Ctrl Pts',(4.29948208843632,-5.54130534457375,
64.9363743980283));
#145327=CARTESIAN_POINT('Ctrl Pts',(4.15091304341011,-5.65044666097715,
64.928008094134));
#145328=CARTESIAN_POINT('Ctrl Pts',(4.00238554898131,-5.75955745361366,
64.9196441300604));
#145329=CARTESIAN_POINT('Ctrl Pts',(3.84951646993777,-5.86283555794911,
64.9112801659868));
#145330=CARTESIAN_POINT('Ctrl Pts',(3.69279438675011,-5.95994095437923,
64.9029162019131));
#145331=CARTESIAN_POINT('Ctrl Pts',(3.53609642048622,-6.05703140790282,
64.8945535249146));
#145332=CARTESIAN_POINT('Ctrl Pts',(3.3755469115246,-6.14795087433382,64.886190847916));
#145333=CARTESIAN_POINT('Ctrl Pts',(3.21166241619738,-6.23240331548635,
64.8778281709175));
#145334=CARTESIAN_POINT('Ctrl Pts',(3.04778129495275,-6.31685401791727,
64.8694656660912));
#145335=CARTESIAN_POINT('Ctrl Pts',(2.88056561657793,-6.39483781037193,
64.8611031612649));
#145336=CARTESIAN_POINT('Ctrl Pts',(2.71055584899794,-6.46610497532812,
64.8527406564386));
#145337=CARTESIAN_POINT('Ctrl Pts',(2.54052692051615,-6.53738017242957,
64.8443772091186));
#145338=CARTESIAN_POINT('Ctrl Pts',(2.3677035782861,-6.60193710624488,64.8360137617986));
#145339=CARTESIAN_POINT('Ctrl Pts',(2.19264594025775,-6.65957433648512,
64.8276503144786));
#145340=CARTESIAN_POINT('Ctrl Pts',(2.01748522337276,-6.71724550514621,
64.8192819425258));
#145341=CARTESIAN_POINT('Ctrl Pts',(1.8400878939732,-6.76798872457742,64.810913570573));
#145342=CARTESIAN_POINT('Ctrl Pts',(1.66102989130136,-6.81165224176216,
64.8025451986202));
#145343=CARTESIAN_POINT('Ctrl Pts',(1.48191823817219,-6.8553288416778,64.7941743192844));
#145344=CARTESIAN_POINT('Ctrl Pts',(1.30114524022368,-6.89192143686218,
64.7858034399486));
#145345=CARTESIAN_POINT('Ctrl Pts',(1.11929739056601,-6.9213293458679,64.7774325606129));
#145346=CARTESIAN_POINT('Ctrl Pts',(0.937295463191772,-6.95076217187691,
64.7690545887216));
#145347=CARTESIAN_POINT('Ctrl Pts',(0.754217189902066,-6.97299810058511,
64.7606766168303));
#145348=CARTESIAN_POINT('Ctrl Pts',(0.570655713219298,-6.98798816680954,
64.752298644939));
#145349=CARTESIAN_POINT('Ctrl Pts',(0.454000900049228,-6.99751447595904,
64.7469743755804));
#145350=CARTESIAN_POINT('Ctrl Pts',(0.337151023200128,-7.0041154412878,
64.7416501062217));
#145351=CARTESIAN_POINT('Ctrl Pts',(0.220258480231267,-7.00778943493497,
64.7363258368631));
#145352=CARTESIAN_POINT('Ctrl Pts',(0.0476326661061011,-7.01321515438915,
64.7284630056738));
#145353=CARTESIAN_POINT('Ctrl Pts',(-0.125445162475985,-7.01226592069183,
64.7206001744845));
#145354=CARTESIAN_POINT('Ctrl Pts',(-0.298444993881777,-7.00489522749105,
64.7127373432952));
#145355=CARTESIAN_POINT('Ctrl Pts',(-0.471311897752816,-6.99753019769508,
64.7048805536537));
#145356=CARTESIAN_POINT('Ctrl Pts',(-0.644100545164281,-6.98375353657632,
64.6970237640123));
#145357=CARTESIAN_POINT('Ctrl Pts',(-0.816277960679824,-6.96357069709272,
64.6891669743709));
#145358=CARTESIAN_POINT('Ctrl Pts',(-0.988358276283166,-6.94339923977522,
64.6813146155869));
#145359=CARTESIAN_POINT('Ctrl Pts',(-1.15982766819099,-6.91682883499378,
64.6734622568029));
#145360=CARTESIAN_POINT('Ctrl Pts',(-1.33015558245117,-6.88391695831479,
64.6656098980189));
#145361=CARTESIAN_POINT('Ctrl Pts',(-1.50044328030389,-6.85101285251381,
64.6577593932684));
#145362=CARTESIAN_POINT('Ctrl Pts',(-1.66958966131295,-6.81177031883289,
64.6499088885179));
#145363=CARTESIAN_POINT('Ctrl Pts',(-1.83707176434058,-6.76629838945657,
64.6420583837674));
#145364=CARTESIAN_POINT('Ctrl Pts',(-2.00452692477618,-6.72083377508061,
64.6342091419158));
#145365=CARTESIAN_POINT('Ctrl Pts',(-2.1703179727901,-6.6691418627927,64.6263599000641));
#145366=CARTESIAN_POINT('Ctrl Pts',(-2.33393502974738,-6.61138214289706,
64.6185106582124));
#145367=CARTESIAN_POINT('Ctrl Pts',(-2.4976072124939,-6.55360296262116,
64.6106587717975));
#145368=CARTESIAN_POINT('Ctrl Pts',(-2.65910358105503,-6.48975201836282,
64.6028068853825));
#145369=CARTESIAN_POINT('Ctrl Pts',(-2.81793204785603,-6.42003781423178,
64.5949549989676));
#145370=CARTESIAN_POINT('Ctrl Pts',(-2.93455781412435,-6.36884754185601,
64.5891894565039));
#145371=CARTESIAN_POINT('Ctrl Pts',(-3.04974546524054,-6.31449695611502,
64.5834239140402));
#145372=CARTESIAN_POINT('Ctrl Pts',(-3.16330811802645,-6.25708464965338,
64.5776583715764));
#145373=CARTESIAN_POINT('Ctrl Pts',(-3.35348657624183,-6.16093874554134,
64.5680030672169));
#145374=CARTESIAN_POINT('Ctrl Pts',(-3.53901044179996,-6.05625478980657,
64.5583477628573));
#145375=CARTESIAN_POINT('Ctrl Pts',(-3.71921641495434,-5.9434885228487,
64.5486924584977));
#145376=CARTESIAN_POINT('Ctrl Pts',(-3.90042069539488,-5.83009755192588,
64.5389836655633));
#145377=CARTESIAN_POINT('Ctrl Pts',(-4.07624798900836,-5.70853454417221,
64.5292748726288));
#145378=CARTESIAN_POINT('Ctrl Pts',(-4.246060655549,-5.57930062569663,64.5195660796944));
#145379=CARTESIAN_POINT('Ctrl Pts',(-4.41669047506078,-5.44944482263136,
64.5098105672239));
#145380=CARTESIAN_POINT('Ctrl Pts',(-4.58124762253423,-5.31184415036341,
64.5000550547534));
#145381=CARTESIAN_POINT('Ctrl Pts',(-4.73912242433671,-5.16704414628412,
64.4902995422829));
#145382=CARTESIAN_POINT('Ctrl Pts',(-4.89715354648244,-5.02210076792291,
64.4805343703541));
#145383=CARTESIAN_POINT('Ctrl Pts',(-5.04848906764465,-4.86994383338251,
64.4707691984254));
#145384=CARTESIAN_POINT('Ctrl Pts',(-5.19255492798473,-4.7111569579416,
64.4610040264967));
#145385=CARTESIAN_POINT('Ctrl Pts',(-5.3364243577922,-4.55258658480346,
64.4512521691583));
#145386=CARTESIAN_POINT('Ctrl Pts',(-5.47304391187152,-4.38740436615538,
64.44150031182));
#145387=CARTESIAN_POINT('Ctrl Pts',(-5.60187946290261,-4.21622734747665,
64.4317484544817));
#145388=CARTESIAN_POINT('Ctrl Pts',(-5.65806109388263,-4.14158177008204,
64.4274959384178));
#145389=CARTESIAN_POINT('Ctrl Pts',(-5.7127630105389,-4.06579668417115,
64.423243422354));
#145390=CARTESIAN_POINT('Ctrl Pts',(-5.76594319091945,-3.98892537929573,
64.4189909062902));
#145391=CARTESIAN_POINT('Ctrl Pts',(-5.86640108632526,-3.8437147115315,
64.4109578606913));
#145392=CARTESIAN_POINT('Ctrl Pts',(-5.96147480433731,-3.69455501880349,
64.4029248150925));
#145393=CARTESIAN_POINT('Ctrl Pts',(-6.05083762023003,-3.54189083063114,
64.3948917694936));
#145394=CARTESIAN_POINT('Ctrl Pts',(-6.14014299026379,-3.38932478087729,
64.3868638878458));
#145395=CARTESIAN_POINT('Ctrl Pts',(-6.22374458135831,-3.23325903501766,
64.378836006198));
#145396=CARTESIAN_POINT('Ctrl Pts',(-6.30135861793588,-3.0741675508445,
64.3708081245502));
#145397=CARTESIAN_POINT('Ctrl Pts',(-6.37893761101054,-2.91514789804532,
64.3627838675701));
#145398=CARTESIAN_POINT('Ctrl Pts',(-6.45053427203421,-2.75310555586578,
64.35475961059));
#145399=CARTESIAN_POINT('Ctrl Pts',(-6.5159105074575,-2.58853951511369,
64.3467353536099));
#145400=CARTESIAN_POINT('Ctrl Pts',(-6.58127883822837,-2.42399337207126,
64.3387120668441));
#145401=CARTESIAN_POINT('Ctrl Pts',(-6.64042809905632,-2.25692447587121,
64.3306887800784));
#145402=CARTESIAN_POINT('Ctrl Pts',(-6.69316807265263,-2.08785241665293,
64.3226654933127));
#145403=CARTESIAN_POINT('Ctrl Pts',(-6.74590372467866,-1.9187942113814,
64.3146428639837));
#145404=CARTESIAN_POINT('Ctrl Pts',(-6.79223103024297,-1.74773352125313,
64.3066202346547));
#145405=CARTESIAN_POINT('Ctrl Pts',(-6.83200954101177,-1.57520544502113,
64.2985976053257));
#145406=CARTESIAN_POINT('Ctrl Pts',(-6.87180300566862,-1.40261251051544,
64.2905719600593));
#145407=CARTESIAN_POINT('Ctrl Pts',(-6.90504267802685,-1.22855144604104,
64.2825463147929));
#145408=CARTESIAN_POINT('Ctrl Pts',(-6.93163908812218,-1.05356827710248,
64.2745206695265));
#145409=CARTESIAN_POINT('Ctrl Pts',(-6.94732195221921,-0.950387537751055,
64.2697882600188));
#145410=CARTESIAN_POINT('Ctrl Pts',(-6.96069592775564,-0.846886351344504,
64.2650558505112));
#145411=CARTESIAN_POINT('Ctrl Pts',(-6.97175111860442,-0.743177571471341,
64.2603234410035));
#145412=CARTESIAN_POINT('Ctrl Pts',(-6.99214503333888,-0.551862193665758,
64.2515933921688));
#145413=CARTESIAN_POINT('Ctrl Pts',(-7.00465564836291,-0.359744518498557,
64.2428633433341));
#145414=CARTESIAN_POINT('Ctrl Pts',(-7.00924961118251,-0.167470745618054,
64.2341332944993));
#145415=CARTESIAN_POINT('Ctrl Pts',(-7.01384490235223,0.0248586234652346,
64.22540072136));
#145416=CARTESIAN_POINT('Ctrl Pts',(-7.01051896558698,0.21734390649135,
64.2166681482206));
#145417=CARTESIAN_POINT('Ctrl Pts',(-6.99929057855394,0.409338441226893,
64.2079355750813));
#145418=CARTESIAN_POINT('Ctrl Pts',(-6.98790267435951,0.604060564804206,
64.199078941801));
#145419=CARTESIAN_POINT('Ctrl Pts',(-6.9683860917018,0.798277600745668,
64.1902223085207));
#145420=CARTESIAN_POINT('Ctrl Pts',(-6.94081497261681,0.991319362465166,
64.1813656752403));
#145421=CARTESIAN_POINT('Ctrl Pts',(-6.91361275330025,1.18177823805019,
64.1726275431335));
#145422=CARTESIAN_POINT('Ctrl Pts',(-6.87857025954122,1.3710928225916,64.1638894110266));
#145423=CARTESIAN_POINT('Ctrl Pts',(-6.83581054283176,1.55862785327678,
64.1551512789198));
#145424=CARTESIAN_POINT('Ctrl Pts',(-6.79218100465246,1.74997773608423,
64.1462353950527));
#145425=CARTESIAN_POINT('Ctrl Pts',(-6.74051697392506,1.93947460024544,
64.1373195111856));
#145426=CARTESIAN_POINT('Ctrl Pts',(-6.68100348636698,2.12645690707625,
64.1284036273185));
#145427=CARTESIAN_POINT('Ctrl Pts',(-6.62148999880889,2.31343921390706,
64.1194877434514));
#145428=CARTESIAN_POINT('Ctrl Pts',(-6.55412715193585,2.49790667708451,
64.1105718595843));
#145429=CARTESIAN_POINT('Ctrl Pts',(-6.47915356094306,2.67921550014532,
64.1016559757172));
#145430=CARTESIAN_POINT('Ctrl Pts',(-6.40565321995918,2.85696155901605,
64.0929152912211));
#145431=CARTESIAN_POINT('Ctrl Pts',(-6.32483065806716,3.03169084005782,
64.0841746067251));
#145432=CARTESIAN_POINT('Ctrl Pts',(-6.23695464383602,3.20281490773855,
64.075433922229));
#145433=CARTESIAN_POINT('Ctrl Pts',(-6.14909443995983,3.37390818735642,
64.0666948103273));
#145434=CARTESIAN_POINT('Ctrl Pts',(-6.05418344312836,3.54139730552184,
64.0579556984256));
#145435=CARTESIAN_POINT('Ctrl Pts',(-5.95253689588775,3.70471740698194,
64.0492165865238));
#145436=CARTESIAN_POINT('Ctrl Pts',(-5.84957337132991,3.87015355541964,
64.0403642468494));
#145437=CARTESIAN_POINT('Ctrl Pts',(-5.73969867367886,4.03131164898845,
64.031511907175));
#145438=CARTESIAN_POINT('Ctrl Pts',(-5.62328718275385,4.18763272300429,
64.0226595675006));
#145439=CARTESIAN_POINT('Ctrl Pts',(-5.50842358207695,4.34187524047797,
64.013924934851));
#145440=CARTESIAN_POINT('Ctrl Pts',(-5.38719612325943,4.49140835545715,
64.0051903022014));
#145441=CARTESIAN_POINT('Ctrl Pts',(-5.26000708672101,4.63572561851376,
63.9964556695518));
#145442=CARTESIAN_POINT('Ctrl Pts',(-5.13024707032258,4.78296008879882,
63.987544476365));
#145443=CARTESIAN_POINT('Ctrl Pts',(-4.99428207218218,4.9247653643007,63.9786332831781));
#145444=CARTESIAN_POINT('Ctrl Pts',(-4.85258201246857,5.06063971991353,
63.9697220899913));
#145445=CARTESIAN_POINT('Ctrl Pts',(-4.71088195275502,5.19651407552631,
63.9608108968044));
#145446=CARTESIAN_POINT('Ctrl Pts',(-4.56344704093831,5.32645729172441,
63.9518997036176));
#145447=CARTESIAN_POINT('Ctrl Pts',(-4.41078738240452,5.4500074522629,63.9429885104308));
#145448=CARTESIAN_POINT('Ctrl Pts',(-4.27329790931198,5.56128011352838,
63.9349628455783));
#145449=CARTESIAN_POINT('Ctrl Pts',(-4.13150697620337,5.66741791020393,
63.9269371807258));
#145450=CARTESIAN_POINT('Ctrl Pts',(-3.98584443947909,5.76807339297738,
63.9189115158734));
#145451=CARTESIAN_POINT('Ctrl Pts',(-3.8402281324701,5.86869693017022,63.91088839817));
#145452=CARTESIAN_POINT('Ctrl Pts',(-3.6907429693899,5.96384140939698,63.9028652804667));
#145453=CARTESIAN_POINT('Ctrl Pts',(-3.53784990251516,6.05320118860867,
63.8948421627633));
#145454=CARTESIAN_POINT('Ctrl Pts',(-3.384976116794,6.1425496987703,63.8868200568453));
#145455=CARTESIAN_POINT('Ctrl Pts',(-3.22869560001304,6.2261147775928,63.8787979509273));
#145456=CARTESIAN_POINT('Ctrl Pts',(-3.06949610299193,6.3036354777396,63.8707758450093));
#145457=CARTESIAN_POINT('Ctrl Pts',(-2.91023744690084,6.38118498484001,
63.8627507580497));
#145458=CARTESIAN_POINT('Ctrl Pts',(-2.74805797224509,6.45268546291316,
63.8547256710901));
#145459=CARTESIAN_POINT('Ctrl Pts',(-2.58346813076676,6.51792290379478,
63.8467005841305));
#145460=CARTESIAN_POINT('Ctrl Pts',(-2.41884587414272,6.58317319286394,
63.8386739166702));
#145461=CARTESIAN_POINT('Ctrl Pts',(-2.25181264901268,6.6421578605787,63.8306472492099));
#145462=CARTESIAN_POINT('Ctrl Pts',(-2.08289626825347,6.69471206985004,
63.8226205817495));
#145463=CARTESIAN_POINT('Ctrl Pts',(-1.9138442820195,6.74730846945523,63.8145874705089));
#145464=CARTESIAN_POINT('Ctrl Pts',(-1.74290647344521,6.7934640001079,63.8065543592682));
#145465=CARTESIAN_POINT('Ctrl Pts',(-1.57062371239913,6.83306429916693,
63.7985212480275));
#145466=CARTESIAN_POINT('Ctrl Pts',(-1.46910845109101,6.85639823392887,
63.7937878470665));
#145467=CARTESIAN_POINT('Ctrl Pts',(-1.3671264192136,6.87745716470111,63.7890544461054));
#145468=CARTESIAN_POINT('Ctrl Pts',(-1.26478941081879,6.89622609176792,
63.7843210451443));
#145469=CARTESIAN_POINT('Ctrl Pts',(-1.05397198856531,6.9348906656572,63.7745700918503));
#145470=CARTESIAN_POINT('Ctrl Pts',(-0.841523672655311,6.96385777599663,
63.7648191385563));
#145471=CARTESIAN_POINT('Ctrl Pts',(-0.628257409121949,6.9830451230379,
63.7550681852622));
#145472=CARTESIAN_POINT('Ctrl Pts',(-0.414683895533134,7.0022601130516,
63.745303183891));
#145473=CARTESIAN_POINT('Ctrl Pts',(-0.200290115638335,7.01166715299209,
63.7355381825197));
#145474=CARTESIAN_POINT('Ctrl Pts',(0.0141058876221566,7.01123581021452,
63.7257731811485));
#145475=CARTESIAN_POINT('Ctrl Pts',(0.228144537171048,7.01080518639597,
63.7160244560111));
#145476=CARTESIAN_POINT('Ctrl Pts',(0.442185364769944,7.00056895396792,
63.7062757308736));
#145477=CARTESIAN_POINT('Ctrl Pts',(0.655413416490399,6.98054867585524,
63.6965270057362));
#145478=CARTESIAN_POINT('Ctrl Pts',(0.868056239884947,6.96058334564342,
63.6868050370694));
#145479=CARTESIAN_POINT('Ctrl Pts',(1.07989070097927,6.93088758192718,63.6770830684026));
#145480=CARTESIAN_POINT('Ctrl Pts',(1.29010813751828,6.8915344848596,63.6673610997357));
#145481=CARTESIAN_POINT('Ctrl Pts',(1.49893462018888,6.85244177695623,63.6577034587962));
#145482=CARTESIAN_POINT('Ctrl Pts',(1.70616535524532,6.80381909359534,63.6480458178566));
#145483=CARTESIAN_POINT('Ctrl Pts',(1.91100791851239,6.74578944956652,63.638388176917));
#145484=CARTESIAN_POINT('Ctrl Pts',(2.00104327739133,6.72028342317033,63.6341433112307));
#145485=CARTESIAN_POINT('Ctrl Pts',(2.09061727252663,6.69296073300884,63.6298984455443));
#145486=CARTESIAN_POINT('Ctrl Pts',(2.17966267742007,6.66383502010381,63.625653579858));
#145487=CARTESIAN_POINT('Ctrl Pts',(2.34437245817196,6.60996037275317,63.617801732844));
#145488=CARTESIAN_POINT('Ctrl Pts',(2.50720483800169,6.54993521035113,63.60994988583));
#145489=CARTESIAN_POINT('Ctrl Pts',(2.66765176713443,6.48392324228199,63.6020980388161));
#145490=CARTESIAN_POINT('Ctrl Pts',(2.82805319481588,6.41792999467305,63.5942484185224));
#145491=CARTESIAN_POINT('Ctrl Pts',(2.98607016503819,6.3459534636276,63.5863987982287));
#145492=CARTESIAN_POINT('Ctrl Pts',(3.14121267937534,6.26820623986094,63.5785491779351));
#145493=CARTESIAN_POINT('Ctrl Pts',(3.2963428075658,6.19046522321631,63.5707001843333));
#145494=CARTESIAN_POINT('Ctrl Pts',(3.44859859601861,6.10695460258495,63.5628511907314));
#145495=CARTESIAN_POINT('Ctrl Pts',(3.5975130554672,6.01793372996439,63.5550021971296));
#145496=CARTESIAN_POINT('Ctrl Pts',(3.7465029059468,5.9288677886823,63.5471492298121));
#145497=CARTESIAN_POINT('Ctrl Pts',(3.89214771963935,5.83428621747869,63.5392962624946));
#145498=CARTESIAN_POINT('Ctrl Pts',(4.03400772258457,5.73449285086554,63.5314432951772));
#145499=CARTESIAN_POINT('Ctrl Pts',(4.17590375320397,5.63467414009039,63.5235883334698));
#145500=CARTESIAN_POINT('Ctrl Pts',(4.31401275444233,5.52964122788591,63.5157333717625));
#145501=CARTESIAN_POINT('Ctrl Pts',(4.44792720152231,5.41973893951156,63.5078784100552));
#145502=CARTESIAN_POINT('Ctrl Pts',(4.58197456988463,5.30972756392952,63.5000156516418));
#145503=CARTESIAN_POINT('Ctrl Pts',(4.71181878306663,5.19483741159344,63.4921528932284));
#145504=CARTESIAN_POINT('Ctrl Pts',(4.8370880054203,5.07545132873118,63.484290134815));
#145505=CARTESIAN_POINT('Ctrl Pts',(4.92898370942698,4.98787141143711,63.4785221280672));
#145506=CARTESIAN_POINT('Ctrl Pts',(5.01841814622961,4.89787280848837,63.4727541213193));
#145507=CARTESIAN_POINT('Ctrl Pts',(5.10525833231068,4.80561795431892,63.4669861145715));
#145508=CARTESIAN_POINT('Ctrl Pts',(5.23025327460224,4.67282931471073,63.4586838330689));
#145509=CARTESIAN_POINT('Ctrl Pts',(5.35016368603412,4.53505539088394,63.4503815515662));
#145510=CARTESIAN_POINT('Ctrl Pts',(5.46458333403442,4.39271619250473,63.4420792700636));
#145511=CARTESIAN_POINT('Ctrl Pts',(5.58182955935114,4.24686070337994,63.4335718923124));
#145512=CARTESIAN_POINT('Ctrl Pts',(5.69330995865957,4.09621169834653,63.4250645145612));
#145513=CARTESIAN_POINT('Ctrl Pts',(5.79862868272004,3.94126019978845,63.41655713681));
#145514=CARTESIAN_POINT('Ctrl Pts',(5.90126312236804,3.7902579884628,63.4082665887032));
#145515=CARTESIAN_POINT('Ctrl Pts',(5.9980459315389,3.63517021859697,63.3999760405964));
#145516=CARTESIAN_POINT('Ctrl Pts',(6.08865238761097,3.4764836638965,63.3916854924896));
#145517=CARTESIAN_POINT('Ctrl Pts',(6.18281340341766,3.3115717157504,63.3830696999162));
#145518=CARTESIAN_POINT('Ctrl Pts',(6.27030342472347,3.14277320211189,63.3744539073428));
#145519=CARTESIAN_POINT('Ctrl Pts',(6.35080850537203,2.97066623682201,63.3658381147693));
#145520=CARTESIAN_POINT('Ctrl Pts',(6.43131358602062,2.79855927153207,63.3572223221959));
#145521=CARTESIAN_POINT('Ctrl Pts',(6.50483353961304,2.62314422035117,63.3486065296225));
#145522=CARTESIAN_POINT('Ctrl Pts',(6.57110895151814,2.44502632087636,63.3399907370491));
#145523=CARTESIAN_POINT('Origin',(0.,0.,50.));
#145524=CARTESIAN_POINT('',(6.57110895151815,2.44502632087632,61.3398717892601));
#145525=CARTESIAN_POINT('',(6.57110895151817,2.44502632087627,61.8868156729052));
#145526=CARTESIAN_POINT('',(6.57110895151814,2.44502632087636,50.));
#145527=CARTESIAN_POINT('',(7.01124948002266,0.00270025590217394,63.773534356882));
#145528=CARTESIAN_POINT('Ctrl Pts',(6.57110895151817,2.44502632087627,61.8868156729052));
#145529=CARTESIAN_POINT('Ctrl Pts',(6.50691218988431,2.61755776212454,61.8951901719231));
#145530=CARTESIAN_POINT('Ctrl Pts',(6.43587838748572,2.78766143545089,61.903564670941));
#145531=CARTESIAN_POINT('Ctrl Pts',(6.35821510578084,2.95478040319757,61.9119391699589));
#145532=CARTESIAN_POINT('Ctrl Pts',(6.28059813039113,3.12179972715606,61.9203086757267));
#145533=CARTESIAN_POINT('Ctrl Pts',(6.1963596950319,3.28583759643497,61.9286781814945));
#145534=CARTESIAN_POINT('Ctrl Pts',(6.10575546037758,3.44635703614257,61.9370476872623));
#145535=CARTESIAN_POINT('Ctrl Pts',(6.01519196982608,3.60680429135921,61.9454134293207));
#145536=CARTESIAN_POINT('Ctrl Pts',(5.91826854952778,3.76373598624047,61.9537791713792));
#145537=CARTESIAN_POINT('Ctrl Pts',(5.81528699583377,3.91663933986609,61.9621449134376));
#145538=CARTESIAN_POINT('Ctrl Pts',(5.71233667388179,4.0694963217103,61.9705081183747));
#145539=CARTESIAN_POINT('Ctrl Pts',(5.60333206608359,4.21832712642698,61.9788713233118));
#145540=CARTESIAN_POINT('Ctrl Pts',(5.48861876500483,4.36264720266685,61.9872345282489));
#145541=CARTESIAN_POINT('Ctrl Pts',(5.37322158177889,4.5078276666969,61.9956475918031));
#145542=CARTESIAN_POINT('Ctrl Pts',(5.25204759730724,4.64844315984357,62.0040606553572));
#145543=CARTESIAN_POINT('Ctrl Pts',(5.12549076997958,4.78403291474402,62.0124737189114));
#145544=CARTESIAN_POINT('Ctrl Pts',(4.99968093332064,4.91882236290619,62.0208371250895));
#145545=CARTESIAN_POINT('Ctrl Pts',(4.86855187424113,5.04864501876509,62.0292005312675));
#145546=CARTESIAN_POINT('Ctrl Pts',(4.73252882630589,5.17308394197154,62.0375639374456));
#145547=CARTESIAN_POINT('Ctrl Pts',(4.59648557025939,5.29754135230678,62.0459285861237));
#145548=CARTESIAN_POINT('Ctrl Pts',(4.45554711813616,5.41661321313302,62.0542932348018));
#145549=CARTESIAN_POINT('Ctrl Pts',(4.31017345618164,5.52992145876659,62.0626578834799));
#145550=CARTESIAN_POINT('Ctrl Pts',(4.16475881112236,5.64326164776349,62.0710248902831));
#145551=CARTESIAN_POINT('Ctrl Pts',(4.01490672227784,5.75083477951493,62.0793918970863));
#145552=CARTESIAN_POINT('Ctrl Pts',(3.86110828640053,5.85230461982193,62.0877589038894));
#145553=CARTESIAN_POINT('Ctrl Pts',(3.70580092859063,5.95476998434649,62.0962079996943));
#145554=CARTESIAN_POINT('Ctrl Pts',(3.54646965994457,6.0510114686339,62.1046570954993));
#145555=CARTESIAN_POINT('Ctrl Pts',(3.38364764720855,6.1407292044219,62.1131061913042));
#145556=CARTESIAN_POINT('Ctrl Pts',(3.22218795096895,6.22969628033639,62.1214845943176));
#145557=CARTESIAN_POINT('Ctrl Pts',(3.05729601733866,6.312248251256,62.1298629973311));
#145558=CARTESIAN_POINT('Ctrl Pts',(2.88951408629364,6.38814017595189,62.1382414003445));
#145559=CARTESIAN_POINT('Ctrl Pts',(2.71960866470156,6.46499260803786,62.1467258425452));
#145560=CARTESIAN_POINT('Ctrl Pts',(2.54673991877884,6.53501513325592,62.1552102847459));
#145561=CARTESIAN_POINT('Ctrl Pts',(2.37148933148852,6.59800461602871,62.1636947269465));
#145562=CARTESIAN_POINT('Ctrl Pts',(2.19623874419813,6.66099409880152,62.1721791691472));
#145563=CARTESIAN_POINT('Ctrl Pts',(2.0186066570039,6.71695046741193,62.1806636113479));
#145564=CARTESIAN_POINT('Ctrl Pts',(1.83918801382947,6.76572346554942,62.1891480535485));
#145565=CARTESIAN_POINT('Ctrl Pts',(1.66195048764615,6.81390355085988,62.1975293539535));
#145566=CARTESIAN_POINT('Ctrl Pts',(1.48261202793872,6.85517116373265,62.2059106543584));
#145567=CARTESIAN_POINT('Ctrl Pts',(1.30173764763051,6.88934725930123,62.2142919547633));
#145568=CARTESIAN_POINT('Ctrl Pts',(1.12109249912092,6.92348004167176,62.222662633097));
#145569=CARTESIAN_POINT('Ctrl Pts',(0.938915628636189,6.95053915747266,
62.2310333114306));
#145570=CARTESIAN_POINT('Ctrl Pts',(0.755786438088463,6.97039549971891,
62.2394039897642));
#145571=CARTESIAN_POINT('Ctrl Pts',(0.572865067730339,6.99022930842586,
62.2477651688151));
#145572=CARTESIAN_POINT('Ctrl Pts',(0.388993855063862,7.00287659997775,
62.256126347866));
#145573=CARTESIAN_POINT('Ctrl Pts',(0.204762051795161,7.00825934627455,
62.2644875269168));
#145574=CARTESIAN_POINT('Ctrl Pts',(0.0207693110235397,7.01363510782308,
62.2728378563516));
#145575=CARTESIAN_POINT('Ctrl Pts',(-0.163582761091555,7.01176511695458,
62.2811881857864));
#145576=CARTESIAN_POINT('Ctrl Pts',(-0.347700215973515,7.00262316009594,
62.2895385152211));
#145577=CARTESIAN_POINT('Ctrl Pts',(-0.531676003487666,6.99348823742623,
62.2978824195769));
#145578=CARTESIAN_POINT('Ctrl Pts',(-0.715417207661931,6.97709251544554,
62.3062263239327));
#145579=CARTESIAN_POINT('Ctrl Pts',(-0.898329147986046,6.95346182159496,
62.3145702282885));
#145580=CARTESIAN_POINT('Ctrl Pts',(-1.08109417229915,6.92985010806502,
62.3229074307683));
#145581=CARTESIAN_POINT('Ctrl Pts',(-1.26303093713436,6.89901505408378,
62.331244633248));
#145582=CARTESIAN_POINT('Ctrl Pts',(-1.44354899992312,6.86103438610542,
62.3395818357278));
#145583=CARTESIAN_POINT('Ctrl Pts',(-1.50297454974923,6.84853135985692,
62.3423263967635));
#145584=CARTESIAN_POINT('Ctrl Pts',(-1.56224640000419,6.83525438799622,
62.3450709577992));
#145585=CARTESIAN_POINT('Ctrl Pts',(-1.62134364638829,6.82120746956258,
62.3478155188349));
#145586=CARTESIAN_POINT('Ctrl Pts',(-1.80088827007231,6.77853122255614,
62.3561538291368));
#145587=CARTESIAN_POINT('Ctrl Pts',(-1.97867313897258,6.72877946772584,
62.3644921394386));
#145588=CARTESIAN_POINT('Ctrl Pts',(-2.1541298738823,6.6721324214188,62.3728304497405));
#145589=CARTESIAN_POINT('Ctrl Pts',(-2.32969700021576,6.61544973471245,
62.3811740062242));
#145590=CARTESIAN_POINT('Ctrl Pts',(-2.50293275906428,6.55186320395057,
62.3895175627079));
#145591=CARTESIAN_POINT('Ctrl Pts',(-2.67328714752016,6.4816018382344,62.3978611191917));
#145592=CARTESIAN_POINT('Ctrl Pts',(-2.84377114085238,6.41128701797739,
62.4062110234168));
#145593=CARTESIAN_POINT('Ctrl Pts',(-3.01136908864337,6.3342873582309,62.414560927642));
#145594=CARTESIAN_POINT('Ctrl Pts',(-3.17555365440632,6.25087878225827,
62.4229108318672));
#145595=CARTESIAN_POINT('Ctrl Pts',(-3.3399844848681,6.167345099594,62.4312732603307));
#145596=CARTESIAN_POINT('Ctrl Pts',(-3.50099140991984,6.07738343963517,
62.4396356887943));
#145597=CARTESIAN_POINT('Ctrl Pts',(-3.65807295567938,5.9813149736013,62.4479981172579));
#145598=CARTESIAN_POINT('Ctrl Pts',(-3.81528882757404,5.88516435593284,
62.4563676967378));
#145599=CARTESIAN_POINT('Ctrl Pts',(-3.96857235071375,5.78289669405816,
62.4647372762177));
#145600=CARTESIAN_POINT('Ctrl Pts',(-4.11745300246685,5.67487509421809,
62.4731068556977));
#145601=CARTESIAN_POINT('Ctrl Pts',(-4.26656328448577,5.56668688422153,
62.4814893442342));
#145602=CARTESIAN_POINT('Ctrl Pts',(-4.41125686798621,5.45272720420105,
62.4898718327707));
#145603=CARTESIAN_POINT('Ctrl Pts',(-4.55109704854791,5.33339874912785,
62.4982543213072));
#145604=CARTESIAN_POINT('Ctrl Pts',(-4.59685504705112,5.29435252330993,
62.5009972089119));
#145605=CARTESIAN_POINT('Ctrl Pts',(-4.64209369023455,5.25473174629258,
62.5037400965166));
#145606=CARTESIAN_POINT('Ctrl Pts',(-4.68679857597168,5.21455133935508,
62.5064829841214));
#145607=CARTESIAN_POINT('Ctrl Pts',(-4.82354042219802,5.09164882129327,
62.5148728392542));
#145608=CARTESIAN_POINT('Ctrl Pts',(-4.95556165108419,4.96325958096101,
62.523262694387));
#145609=CARTESIAN_POINT('Ctrl Pts',(-5.08241371095019,4.82977198563717,
62.5316525495197));
#145610=CARTESIAN_POINT('Ctrl Pts',(-5.20914871351373,4.69640757079486,
62.5400346626118));
#145611=CARTESIAN_POINT('Ctrl Pts',(-5.33072383076614,4.5579544168971,62.5484167757039));
#145612=CARTESIAN_POINT('Ctrl Pts',(-5.44672584142539,4.41483908776401,
62.556798888796));
#145613=CARTESIAN_POINT('Ctrl Pts',(-5.56263785911027,4.27183478579391,
62.5651744991449));
#145614=CARTESIAN_POINT('Ctrl Pts',(-5.67298518379294,4.12417577396186,
62.5735501094938));
#145615=CARTESIAN_POINT('Ctrl Pts',(-5.77739322365019,3.97232351424464,
62.5819257198426));
#145616=CARTESIAN_POINT('Ctrl Pts',(-5.88173558929987,3.82056677185385,
62.5902960618082));
#145617=CARTESIAN_POINT('Ctrl Pts',(-5.98014593340554,3.66462231092458,
62.5986664037738));
#145618=CARTESIAN_POINT('Ctrl Pts',(-6.07229127951136,3.50498290712956,
62.6070367457394));
#145619=CARTESIAN_POINT('Ctrl Pts',(-6.16439217229915,3.34542051754617,
62.6154030496337));
#145620=CARTESIAN_POINT('Ctrl Pts',(-6.25023393020028,3.18216702395701,
62.623769353528));
#145621=CARTESIAN_POINT('Ctrl Pts',(-6.32952784024959,3.01574267503137,
62.6321356574223));
#145622=CARTESIAN_POINT('Ctrl Pts',(-6.40879957401472,2.84936487033156,
62.640499621496));
#145623=CARTESIAN_POINT('Ctrl Pts',(-6.48152696887035,2.6798182743762,62.6488635855696));
#145624=CARTESIAN_POINT('Ctrl Pts',(-6.5474678242823,2.50764663628831,62.6572275496432));
#145625=CARTESIAN_POINT('Ctrl Pts',(-6.61339853249239,2.33550149255439,
62.6655902266417));
#145626=CARTESIAN_POINT('Ctrl Pts',(-6.67254466594148,2.1607324189128,62.6739529036403));
#145627=CARTESIAN_POINT('Ctrl Pts',(-6.72471247731919,1.98390238164271,
62.6823155806388));
#145628=CARTESIAN_POINT('Ctrl Pts',(-6.77687921465701,1.8070759849799,62.6906780854651));
#145629=CARTESIAN_POINT('Ctrl Pts',(-6.82206782379463,1.62818902462807,
62.6990405902914));
#145630=CARTESIAN_POINT('Ctrl Pts',(-6.86013454488729,1.44781925271909,
62.7074030951177));
#145631=CARTESIAN_POINT('Ctrl Pts',(-6.89820555627872,1.26742915228726,
62.7157665424377));
#145632=CARTESIAN_POINT('Ctrl Pts',(-6.92915301199316,1.08555622877291,
62.7241299897576));
#145633=CARTESIAN_POINT('Ctrl Pts',(-6.95288426097044,0.902788466945334,
62.7324934370776));
#145634=CARTESIAN_POINT('Ctrl Pts',(-6.97662948357404,0.719913086323296,
62.7408618090304));
#145635=CARTESIAN_POINT('Ctrl Pts',(-6.99314996540047,0.536142140642771,
62.7492301809832));
#145636=CARTESIAN_POINT('Ctrl Pts',(-7.00240482998677,0.352069821879175,
62.757598552936));
#145637=CARTESIAN_POINT('Ctrl Pts',(-7.01166246757238,0.167942350238086,
62.7659694322718));
#145638=CARTESIAN_POINT('Ctrl Pts',(-7.01365013587316,-0.0164863459675034,
62.7743403116075));
#145639=CARTESIAN_POINT('Ctrl Pts',(-7.00837910332975,-0.200621301239111,
62.7827111909433));
#145640=CARTESIAN_POINT('Ctrl Pts',(-7.00310360469747,-0.384912272067153,
62.7910891628346));
#145641=CARTESIAN_POINT('Ctrl Pts',(-6.99055713077681,-0.568908676021576,
62.7994671347259));
#145642=CARTESIAN_POINT('Ctrl Pts',(-6.97080299477925,-0.752018730136862,
62.8078451066172));
#145643=CARTESIAN_POINT('Ctrl Pts',(-6.95824908049424,-0.868386660598136,
62.8131693759762));
#145644=CARTESIAN_POINT('Ctrl Pts',(-6.94278524829728,-0.984396730672524,
62.8184936453352));
#145645=CARTESIAN_POINT('Ctrl Pts',(-6.92443852335641,-1.09989894933928,
62.8238179146942));
#145646=CARTESIAN_POINT('Ctrl Pts',(-6.8973442515681,-1.27047154552732,
62.8316807458835));
#145647=CARTESIAN_POINT('Ctrl Pts',(-6.86390358510918,-1.44029073648694,
62.8395435770729));
#145648=CARTESIAN_POINT('Ctrl Pts',(-6.82417039470791,-1.60882720840124,
62.8474064082622));
#145649=CARTESIAN_POINT('Ctrl Pts',(-6.78446773401874,-1.7772341822834,
62.8552631979036));
#145650=CARTESIAN_POINT('Ctrl Pts',(-6.73848225135099,-1.94436002842866,
62.8631199875451));
#145651=CARTESIAN_POINT('Ctrl Pts',(-6.68631940867443,-2.10968228121764,
62.8709767771865));
#145652=CARTESIAN_POINT('Ctrl Pts',(-6.63418598337189,-2.27491130008196,
62.8788291359706));
#145653=CARTESIAN_POINT('Ctrl Pts',(-6.57588224238199,-2.43833838644849,
62.8866814947546));
#145654=CARTESIAN_POINT('Ctrl Pts',(-6.51156428959697,-2.59945322422727,
62.8945338535386));
#145655=CARTESIAN_POINT('Ctrl Pts',(-6.44726152303103,-2.76053002091305,
62.9023843582891));
#145656=CARTESIAN_POINT('Ctrl Pts',(-6.3769475043088,-2.91929529869549,
62.9102348630396));
#145657=CARTESIAN_POINT('Ctrl Pts',(-6.30082755024359,-3.07525588278299,
62.91808536779));
#145658=CARTESIAN_POINT('Ctrl Pts',(-6.22471984147991,-3.23119137772794,
62.9259346096417));
#145659=CARTESIAN_POINT('Ctrl Pts',(-6.14280822672519,-3.38432273560712,
62.9337838514934));
#145660=CARTESIAN_POINT('Ctrl Pts',(-6.05534512566555,-3.5341791085878,
62.9416330933451));
#145661=CARTESIAN_POINT('Ctrl Pts',(-5.9678525565752,-3.68408597111377,
62.94948497976));
#145662=CARTESIAN_POINT('Ctrl Pts',(-5.87480495764768,-3.83071531495389,
62.957336866175));
#145663=CARTESIAN_POINT('Ctrl Pts',(-5.77649954844859,-3.9736229727131,
62.9651887525899));
#145664=CARTESIAN_POINT('Ctrl Pts',(-5.70431511006091,-4.07855828706345,
62.9709542950535));
#145665=CARTESIAN_POINT('Ctrl Pts',(-5.6292967177402,-4.1814874955188,62.9767198375172));
#145666=CARTESIAN_POINT('Ctrl Pts',(-5.55157631074634,-4.28224555910332,
62.9824853799808));
#145667=CARTESIAN_POINT('Ctrl Pts',(-5.4214213098565,-4.45098072613015,
62.9921406843405));
#145668=CARTESIAN_POINT('Ctrl Pts',(-5.28375446150655,-4.61354048174883,
63.0017959887003));
#145669=CARTESIAN_POINT('Ctrl Pts',(-5.13914797928086,-4.76935893066914,
63.01145129306));
#145670=CARTESIAN_POINT('Ctrl Pts',(-4.99374040427196,-4.92604058456477,
63.0211600859945));
#145671=CARTESIAN_POINT('Ctrl Pts',(-4.84131616607317,-5.07590603636646,
63.030868878929));
#145672=CARTESIAN_POINT('Ctrl Pts',(-4.68248723673392,-5.21842311817698,
63.0405776718636));
#145673=CARTESIAN_POINT('Ctrl Pts',(-4.52289400910047,-5.36162600428635,
63.0503331843341));
#145674=CARTESIAN_POINT('Ctrl Pts',(-4.35683435041004,-5.49740961724818,
63.0600886968046));
#145675=CARTESIAN_POINT('Ctrl Pts',(-4.18495860075941,-5.6252775995883,
63.0698442092751));
#145676=CARTESIAN_POINT('Ctrl Pts',(-4.01291266767407,-5.75327219090302,
63.0796093812038));
#145677=CARTESIAN_POINT('Ctrl Pts',(-3.83503916209638,-5.87333546050407,
63.0893745531325));
#145678=CARTESIAN_POINT('Ctrl Pts',(-3.65201913516281,-5.98501318285137,
63.0991397250612));
#145679=CARTESIAN_POINT('Ctrl Pts',(-3.46924865188348,-6.09653863515807,
63.1088915823995));
#145680=CARTESIAN_POINT('Ctrl Pts',(-3.28134570445317,-6.19970137194527,
63.1186434397378));
#145681=CARTESIAN_POINT('Ctrl Pts',(-3.08901667891444,-6.29409266851771,
63.1283952970762));
#145682=CARTESIAN_POINT('Ctrl Pts',(-3.00514729462933,-6.3352541099758,
63.1326478131398));
#145683=CARTESIAN_POINT('Ctrl Pts',(-2.92043660940189,-6.37474814420639,
63.1369003292034));
#145684=CARTESIAN_POINT('Ctrl Pts',(-2.83494485713366,-6.41254350624707,
63.141152845267));
#145685=CARTESIAN_POINT('Ctrl Pts',(-2.6734500775664,-6.4839393251358,63.1491858908659));
#145686=CARTESIAN_POINT('Ctrl Pts',(-2.50908783830633,-6.54930506614085,
63.1572189364648));
#145687=CARTESIAN_POINT('Ctrl Pts',(-2.34235612441156,-6.60840331312577,
63.1652519820637));
#145688=CARTESIAN_POINT('Ctrl Pts',(-2.17573159208224,-6.66746356948204,
63.1732798637116));
#145689=CARTESIAN_POINT('Ctrl Pts',(-2.00674096113006,-6.72026422965895,
63.1813077453595));
#145690=CARTESIAN_POINT('Ctrl Pts',(-1.83590305421743,-6.76661558964414,
63.1893356270073));
#145691=CARTESIAN_POINT('Ctrl Pts',(-1.66514228230398,-6.81294602153334,
63.1973598839875));
#145692=CARTESIAN_POINT('Ctrl Pts',(-1.49253624819078,-6.85283285541565,
63.2053841409677));
#145693=CARTESIAN_POINT('Ctrl Pts',(-1.31861978180878,-6.88613595810616,
63.2134083979479));
#145694=CARTESIAN_POINT('Ctrl Pts',(-1.14472434369888,-6.91943503411236,
63.2214316847137));
#145695=CARTESIAN_POINT('Ctrl Pts',(-0.969519147282888,-6.94615188802948,
63.2294549714794));
#145696=CARTESIAN_POINT('Ctrl Pts',(-0.793550262853192,-6.96619727992437,
63.2374782582452));
#145697=CARTESIAN_POINT('Ctrl Pts',(-0.617595797503796,-6.98624102927821,
63.2455008875742));
#145698=CARTESIAN_POINT('Ctrl Pts',(-0.4408781335326,-6.99961436801203,
63.2535235169032));
#145699=CARTESIAN_POINT('Ctrl Pts',(-0.263949225982252,-7.0062798522899,
63.2615461462322));
#145700=CARTESIAN_POINT('Ctrl Pts',(-0.0869538057588191,-7.01294784231532,
63.2695717914987));
#145701=CARTESIAN_POINT('Ctrl Pts',(0.0902526500143067,-7.01290292960822,
63.2775974367652));
#145702=CARTESIAN_POINT('Ctrl Pts',(0.267117029018896,-7.00615979373209,
63.2856230820317));
#145703=CARTESIAN_POINT('Ctrl Pts',(0.371407044452844,-7.00218362991351,
63.290355491539));
#145704=CARTESIAN_POINT('Ctrl Pts',(0.475578137019581,-6.99587948197759,
63.2950879010463));
#145705=CARTESIAN_POINT('Ctrl Pts',(0.579517602900145,-6.98725882663788,
63.2998203105537));
#145706=CARTESIAN_POINT('Ctrl Pts',(0.771258535625853,-6.97135598856246,
63.3085503593882));
#145707=CARTESIAN_POINT('Ctrl Pts',(0.962306806828307,-6.94755946216096,
63.3172804082228));
#145708=CARTESIAN_POINT('Ctrl Pts',(1.15202145315067,-6.91595786091707,
63.3260104570573));
#145709=CARTESIAN_POINT('Ctrl Pts',(1.3417909556994,-6.88434712203081,63.3347430301963));
#145710=CARTESIAN_POINT('Ctrl Pts',(1.53022579343208,-6.84492684852486,
63.3434756033354));
#145711=CARTESIAN_POINT('Ctrl Pts',(1.71669433998222,-6.79783694314397,
63.3522081764744));
#145712=CARTESIAN_POINT('Ctrl Pts',(1.90581196989943,-6.75007805048663,
63.3610648097549));
#145713=CARTESIAN_POINT('Ctrl Pts',(2.09290673320342,-6.69443001733442,
63.3699214430354));
#145714=CARTESIAN_POINT('Ctrl Pts',(2.27733429665622,-6.63109154391442,
63.3787780763158));
#145715=CARTESIAN_POINT('Ctrl Pts',(2.45929423137669,-6.56860053512469,
63.3875162084224));
#145716=CARTESIAN_POINT('Ctrl Pts',(2.63865764173921,-6.49862371531824,
63.3962543405291));
#145717=CARTESIAN_POINT('Ctrl Pts',(2.81482368313845,-6.42140126415901,
63.4049924726357));
#145718=CARTESIAN_POINT('Ctrl Pts',(2.99457330780912,-6.34260794791162,
63.4139083565031));
#145719=CARTESIAN_POINT('Ctrl Pts',(3.17099381508166,-6.25627117582712,
63.4228242403704));
#145720=CARTESIAN_POINT('Ctrl Pts',(3.34347019430442,-6.16269694389542,
63.4317401242378));
#145721=CARTESIAN_POINT('Ctrl Pts',(3.51594657352718,-6.06912271196373,
63.4406560081052));
#145722=CARTESIAN_POINT('Ctrl Pts',(3.68447856178892,-5.9683111697436,63.4495718919725));
#145723=CARTESIAN_POINT('Ctrl Pts',(3.84847863845254,-5.86061760669253,
63.4584877758399));
#145724=CARTESIAN_POINT('Ctrl Pts',(4.00925607216609,-5.75504024937012,
63.4672284603362));
#145725=CARTESIAN_POINT('Ctrl Pts',(4.16569512362393,-5.64283761417378,
63.4759691448325));
#145726=CARTESIAN_POINT('Ctrl Pts',(4.3172683113901,-5.52438420911932,63.4847098293288));
#145727=CARTESIAN_POINT('Ctrl Pts',(4.46881422862211,-5.40595211579999,
63.4934489412307));
#145728=CARTESIAN_POINT('Ctrl Pts',(4.61549581484821,-5.28127166710137,
63.5021880531327));
#145729=CARTESIAN_POINT('Ctrl Pts',(4.75681747821264,-5.15075858893336,
63.5109271650346));
#145730=CARTESIAN_POINT('Ctrl Pts',(4.89997016712154,-5.01855452599823,
63.519779504709));
#145731=CARTESIAN_POINT('Ctrl Pts',(5.03762284929539,-4.8803658166327,63.5286318443833));
#145732=CARTESIAN_POINT('Ctrl Pts',(5.16929682606274,-4.73666516513018,
63.5374841840576));
#145733=CARTESIAN_POINT('Ctrl Pts',(5.2992199716851,-4.594875260021,63.5462188167074));
#145734=CARTESIAN_POINT('Ctrl Pts',(5.42332223922286,-4.44771930043756,
63.5549534493572));
#145735=CARTESIAN_POINT('Ctrl Pts',(5.54118175104932,-4.29568753104064,
63.5636880820071));
#145736=CARTESIAN_POINT('Ctrl Pts',(5.66142365713336,-4.14058261456575,
63.5725992751936));
#145737=CARTESIAN_POINT('Ctrl Pts',(5.77516754427281,-3.98040288733585,
63.5815104683802));
#145738=CARTESIAN_POINT('Ctrl Pts',(5.88200887951174,-3.81570414259872,
63.5904216615667));
#145739=CARTESIAN_POINT('Ctrl Pts',(5.98885021475063,-3.65100539786166,
63.5993328547533));
#145740=CARTESIAN_POINT('Ctrl Pts',(6.08878882181403,-3.48178788259178,
63.6082440479399));
#145741=CARTESIAN_POINT('Ctrl Pts',(6.18146681589444,-3.30863938296332,
63.6171552411264));
#145742=CARTESIAN_POINT('Ctrl Pts',(6.26488837546854,-3.15278450047213,
63.6251764077546));
#145743=CARTESIAN_POINT('Ctrl Pts',(6.34246548234576,-2.99367208680069,
63.6331975743829));
#145744=CARTESIAN_POINT('Ctrl Pts',(6.41393773392161,-2.8317890648628,63.6412187410111));
#145745=CARTESIAN_POINT('Ctrl Pts',(6.48538716206193,-2.66995773748654,
63.6492373462176));
#145746=CARTESIAN_POINT('Ctrl Pts',(6.55073546808279,-2.50535789862939,
63.6572559514241));
#145747=CARTESIAN_POINT('Ctrl Pts',(6.60976914815376,-2.33849917053966,
63.6652745566305));
#145748=CARTESIAN_POINT('Ctrl Pts',(6.66879529367676,-2.17166173885381,
63.6732921384117));
#145749=CARTESIAN_POINT('Ctrl Pts',(6.72150829684188,-2.00256633831411,
63.6813097201928));
#145750=CARTESIAN_POINT('Ctrl Pts',(6.76774358430884,-1.83174052189346,
63.6893273019739));
#145751=CARTESIAN_POINT('Ctrl Pts',(6.81399538839174,-1.66085368142483,
63.697347747873));
#145752=CARTESIAN_POINT('Ctrl Pts',(6.85376475567758,-1.48823554410405,
63.7053681937721));
#145753=CARTESIAN_POINT('Ctrl Pts',(6.88693748412361,-1.31442711942242,
63.7133886396712));
#145754=CARTESIAN_POINT('Ctrl Pts',(6.92011674764756,-1.14058445421699,
63.7214106656104));
#145755=CARTESIAN_POINT('Ctrl Pts',(6.9466967234212,-0.965551396643878,
63.7294326915495));
#145756=CARTESIAN_POINT('Ctrl Pts',(6.96661476310131,-0.789876765729247,
63.7374547174887));
#145757=CARTESIAN_POINT('Ctrl Pts',(6.98654811079227,-0.614067120064253,
63.7454829087565));
#145758=CARTESIAN_POINT('Ctrl Pts',(6.99980926583188,-0.437615281936497,
63.7535111000242));
#145759=CARTESIAN_POINT('Ctrl Pts',(7.00638760501589,-0.261073343678946,
63.761539291292));
#145760=CARTESIAN_POINT('Ctrl Pts',(7.00966387681666,-0.173148510710257,
63.7655376464887));
#145761=CARTESIAN_POINT('Ctrl Pts',(7.01128333372664,-0.0852013256471142,
63.7695360016853));
#145762=CARTESIAN_POINT('Ctrl Pts',(7.01124948002266,0.00270025590207967,
63.773534356882));
#145763=CARTESIAN_POINT('Ctrl Pts',(7.01124948002242,0.00270025652918008,
63.7735343569105));
#145764=CARTESIAN_POINT('Ctrl Pts',(7.01124302160633,0.0194696138023747,
63.7742971400779));
#145765=CARTESIAN_POINT('Ctrl Pts',(7.01117640060358,0.0362375540536934,
63.7750599232454));
#145766=CARTESIAN_POINT('Ctrl Pts',(7.01104964859508,0.0530036549197061,
63.7758227064129));
#145767=CARTESIAN_POINT('Ctrl Pts',(7.00942846247404,0.267445779739449,
63.7855788712198));
#145768=CARTESIAN_POINT('Ctrl Pts',(6.99796556449339,0.481668111792948,
63.7953350360268));
#145769=CARTESIAN_POINT('Ctrl Pts',(6.97673294021471,0.694855411882936,
63.8050912008337));
#145770=CARTESIAN_POINT('Ctrl Pts',(6.95548118222794,0.908234824992813,
63.8148561573758));
#145771=CARTESIAN_POINT('Ctrl Pts',(6.9244421066821,1.12057730384373,63.8246211139179));
#145772=CARTESIAN_POINT('Ctrl Pts',(6.88373949701866,1.33107366425954,63.83438607046));
#145773=CARTESIAN_POINT('Ctrl Pts',(6.84311081382055,1.54118770884795,63.8441332913157));
#145774=CARTESIAN_POINT('Ctrl Pts',(6.79285368022903,1.74946229878537,63.8538805121713));
#145775=CARTESIAN_POINT('Ctrl Pts',(6.73314228653791,1.95510140702088,63.863627733027));
#145776=CARTESIAN_POINT('Ctrl Pts',(6.68518950162099,2.12024523164395,63.8714554917902));
#145777=CARTESIAN_POINT('Ctrl Pts',(6.63114033388791,2.28368950797833,63.8792832505535));
#145778=CARTESIAN_POINT('Ctrl Pts',(6.57110895151817,2.44502632087628,63.8871110093167));
#145779=CARTESIAN_POINT('',(7.01124858877574,-0.00444847055471408,63.2264656430603));
#145780=CARTESIAN_POINT('Ctrl Pts',(6.57110895151814,2.44502632087636,63.3399907370491));
#145781=CARTESIAN_POINT('Ctrl Pts',(6.63484048754942,2.27374519259836,63.331705647918));
#145782=CARTESIAN_POINT('Ctrl Pts',(6.69187315219911,2.09996518305276,63.3234205587869));
#145783=CARTESIAN_POINT('Ctrl Pts',(6.7420259826953,1.92424328273777,63.3151354696559));
#145784=CARTESIAN_POINT('Ctrl Pts',(6.79219731414985,1.74845656008818,63.306847324225));
#145785=CARTESIAN_POINT('Ctrl Pts',(6.83548364555182,1.5707268398795,63.298559178794));
#145786=CARTESIAN_POINT('Ctrl Pts',(6.87175418446422,1.39162530546065,63.2902710333631));
#145787=CARTESIAN_POINT('Ctrl Pts',(6.90803158763612,1.21248987578013,63.281981319387));
#145788=CARTESIAN_POINT('Ctrl Pts',(6.93729048961663,1.03198244662936,63.2736916054108));
#145789=CARTESIAN_POINT('Ctrl Pts',(6.95945146872979,0.850683147179211,
63.2654018914347));
#145790=CARTESIAN_POINT('Ctrl Pts',(6.98162775056118,0.669258655963964,
63.2571064532007));
#145791=CARTESIAN_POINT('Ctrl Pts',(6.99669628152373,0.487041538204856,
63.2488110149668));
#145792=CARTESIAN_POINT('Ctrl Pts',(7.00462955623186,0.304616714024459,
63.2405155767329));
#145793=CARTESIAN_POINT('Ctrl Pts',(7.00910840272075,0.201626106321506,
63.2358322655185));
#145794=CARTESIAN_POINT('Ctrl Pts',(7.01131395111323,0.0985693323568585,
63.231148954304));
#145795=CARTESIAN_POINT('Ctrl Pts',(7.01124858877614,-0.00444846991103996,
63.2264656430896));
#145796=CARTESIAN_POINT('Ctrl Pts',(7.01124858877573,-0.00444847055461616,
63.2264656430603));
#145797=CARTESIAN_POINT('Ctrl Pts',(7.01109817222254,-0.241520478426499,
63.2156880690037));
#145798=CARTESIAN_POINT('Ctrl Pts',(6.99891979679981,-0.478179014153952,
63.204910494947));
#145799=CARTESIAN_POINT('Ctrl Pts',(6.97486124731762,-0.713398306114453,
63.1941329208903));
#145800=CARTESIAN_POINT('Ctrl Pts',(6.95038805171756,-0.952671573412448,
63.1831695966808));
#145801=CARTESIAN_POINT('Ctrl Pts',(6.91362159641276,-1.19045596327219,
63.1722062724713));
#145802=CARTESIAN_POINT('Ctrl Pts',(6.86476735118868,-1.42569133284663,
63.1612429482619));
#145803=CARTESIAN_POINT('Ctrl Pts',(6.84754912786283,-1.50859784606554,
63.1573790268408));
#145804=CARTESIAN_POINT('Ctrl Pts',(6.82882987787831,-1.59118788006927,
63.1535151054197));
#145805=CARTESIAN_POINT('Ctrl Pts',(6.80862007451927,-1.67341544254653,
63.1496511839986));
#145806=CARTESIAN_POINT('Ctrl Pts',(6.76478263203099,-1.85177670499975,
63.1412698835937));
#145807=CARTESIAN_POINT('Ctrl Pts',(6.71388127875477,-2.0286222625827,63.1328885831888));
#145808=CARTESIAN_POINT('Ctrl Pts',(6.65603350584824,-2.20337117425222,
63.1245072827839));
#145809=CARTESIAN_POINT('Ctrl Pts',(6.59825904652563,-2.37789861725739,
63.1161366044503));
#145810=CARTESIAN_POINT('Ctrl Pts',(6.53355581430722,-2.5503344013266,63.1077659261167));
#145811=CARTESIAN_POINT('Ctrl Pts',(6.46209194964979,-2.72010922515463,
63.0993952477831));
#145812=CARTESIAN_POINT('Ctrl Pts',(6.39070918420901,-2.88969138370652,
63.0910340687323));
#145813=CARTESIAN_POINT('Ctrl Pts',(6.31258120412595,-3.05661830052571,
63.0826728896814));
#145814=CARTESIAN_POINT('Ctrl Pts',(6.22792559518153,-3.22033683694466,
63.0743117106306));
#145815=CARTESIAN_POINT('Ctrl Pts',(6.14337983687574,-3.38384292925029,
63.0659613811959));
#145816=CARTESIAN_POINT('Ctrl Pts',(6.05232349453927,-3.54414865553281,
63.0576110517611));
#145817=CARTESIAN_POINT('Ctrl Pts',(5.95502174312746,-3.70072190273455,
63.0492607223264));
#145818=CARTESIAN_POINT('Ctrl Pts',(5.85779485959307,-3.85717467618828,
63.0409168179707));
#145819=CARTESIAN_POINT('Ctrl Pts',(5.75433231561575,-4.00990041666434,
63.0325729136149));
#145820=CARTESIAN_POINT('Ctrl Pts',(5.64494515016839,-4.15839161384427,
63.0242290092592));
#145821=CARTESIAN_POINT('Ctrl Pts',(5.53564584517409,-4.30676354196915,
63.0158918067795));
#145822=CARTESIAN_POINT('Ctrl Pts',(5.42043160301229,-4.45090744699308,
63.0075546042997));
#145823=CARTESIAN_POINT('Ctrl Pts',(5.29965679182837,-4.59034469853055,
62.99921740182));
#145824=CARTESIAN_POINT('Ctrl Pts',(5.25989839064931,-4.63624667205952,
62.996472840784));
#145825=CARTESIAN_POINT('Ctrl Pts',(5.21953773998056,-4.68163883099359,
62.993728279748));
#145826=CARTESIAN_POINT('Ctrl Pts',(5.17858847666912,-4.72650483463307,
62.9909837187121));
#145827=CARTESIAN_POINT('Ctrl Pts',(5.05417963326997,-4.86281321161849,
62.9826454084102));
#145828=CARTESIAN_POINT('Ctrl Pts',(4.92443695716898,-4.99415069566876,
62.9743070981084));
#145829=CARTESIAN_POINT('Ctrl Pts',(4.78979374022895,-5.12010766376681,
62.9659687878066));
#145830=CARTESIAN_POINT('Ctrl Pts',(4.65506581034569,-5.24614387971507,
62.9576252313229));
#145831=CARTESIAN_POINT('Ctrl Pts',(4.5154314289632,-5.36679260359573,62.9492816748391));
#145832=CARTESIAN_POINT('Ctrl Pts',(4.37135764285154,-5.48168394937025,
62.9409381183554));
#145833=CARTESIAN_POINT('Ctrl Pts',(4.22717424603034,-5.5966627039807,62.9325882141302));
#145834=CARTESIAN_POINT('Ctrl Pts',(4.07854496339126,-5.70587513938718,
62.924238309905));
#145835=CARTESIAN_POINT('Ctrl Pts',(3.92596687286556,-5.8089939469466,62.9158884056798));
#145836=CARTESIAN_POINT('Ctrl Pts',(3.7731599264961,-5.91226742508571,62.9075259772162));
#145837=CARTESIAN_POINT('Ctrl Pts',(3.61639260808626,-6.00942882717345,
62.8991635487527));
#145838=CARTESIAN_POINT('Ctrl Pts',(3.45618901933156,-6.10019540876782,
62.8908011202891));
#145839=CARTESIAN_POINT('Ctrl Pts',(3.29584843466955,-6.19103960816273,
62.8824315408092));
#145840=CARTESIAN_POINT('Ctrl Pts',(3.13206600716901,-6.27547792632041,
62.8740619613293));
#145841=CARTESIAN_POINT('Ctrl Pts',(2.96538749690621,-6.35327502597616,
62.8656923818495));
#145842=CARTESIAN_POINT('Ctrl Pts',(2.79845190534932,-6.43119211817938,
62.857309893313));
#145843=CARTESIAN_POINT('Ctrl Pts',(2.6286116064732,-6.50244739625811,62.8489274047765));
#145844=CARTESIAN_POINT('Ctrl Pts',(2.45643057630671,-6.56685429915157,
62.84054491624));
#145845=CARTESIAN_POINT('Ctrl Pts',(2.40009012187456,-6.58792929315107,
62.8378020286353));
#145846=CARTESIAN_POINT('Ctrl Pts',(2.34349914849372,-6.60827143021681,
62.8350591410305));
#145847=CARTESIAN_POINT('Ctrl Pts',(2.28667769040812,-6.62787535358729,
62.8323162534258));
#145848=CARTESIAN_POINT('Ctrl Pts',(2.11287406792426,-6.68783919491554,
62.823926398293));
#145849=CARTESIAN_POINT('Ctrl Pts',(1.93656216285547,-6.74101356882585,
62.8155365431602));
#145850=CARTESIAN_POINT('Ctrl Pts',(1.75829916848905,-6.78719460429644,
62.8071466880274));
#145851=CARTESIAN_POINT('Ctrl Pts',(1.58020067271463,-6.83333302455495,
62.7987645749353));
#145852=CARTESIAN_POINT('Ctrl Pts',(1.40015499349829,-6.87249088908758,
62.7903824618432));
#145853=CARTESIAN_POINT('Ctrl Pts',(1.21873558913893,-6.90451375016852,
62.7820003487511));
#145854=CARTESIAN_POINT('Ctrl Pts',(1.0374569277867,-6.93651176829631,62.7736247384022));
#145855=CARTESIAN_POINT('Ctrl Pts',(0.854806988572278,-6.96138576163942,
62.7652491280533));
#145856=CARTESIAN_POINT('Ctrl Pts',(0.671371010195393,-6.97903199084008,
62.7568735177045));
#145857=CARTESIAN_POINT('Ctrl Pts',(0.488050415772942,-6.99666712030052,
62.7485031757389));
#145858=CARTESIAN_POINT('Ctrl Pts',(0.303945094410669,-7.00708351927796,
62.7401328337733));
#145859=CARTESIAN_POINT('Ctrl Pts',(0.119647482326063,-7.01022902924527,
62.7317624918077));
#145860=CARTESIAN_POINT('Ctrl Pts',(-0.064561219784228,-7.01337302173654,
62.7233961879134));
#145861=CARTESIAN_POINT('Ctrl Pts',(-0.248961699536415,-7.00925311447306,
62.7150298840191));
#145862=CARTESIAN_POINT('Ctrl Pts',(-0.432958966309935,-6.99786918254349,
62.7066635801247));
#145863=CARTESIAN_POINT('Ctrl Pts',(-0.616904774204914,-6.98648843438061,
62.6982996160511));
#145864=CARTESIAN_POINT('Ctrl Pts',(-0.800447266150583,-6.96784773125722,
62.6899356519775));
#145865=CARTESIAN_POINT('Ctrl Pts',(-0.982993461906868,-6.94199902163263,
62.6815716879039));
#145866=CARTESIAN_POINT('Ctrl Pts',(-1.1655115668371,-6.9161542896949,62.6732090109053));
#145867=CARTESIAN_POINT('Ctrl Pts',(-1.34703335593707,-6.88310380882911,
62.6648463339068));
#145868=CARTESIAN_POINT('Ctrl Pts',(-1.52697254641174,-6.84295122041688,
62.6564836569083));
#145869=CARTESIAN_POINT('Ctrl Pts',(-1.7069080322674,-6.80279945867305,
62.648121152082));
#145870=CARTESIAN_POINT('Ctrl Pts',(-1.8852606637958,-6.75554595291287,
62.6397586472557));
#145871=CARTESIAN_POINT('Ctrl Pts',(-2.06145547494011,-6.70134522967885,
62.6313961424294));
#145872=CARTESIAN_POINT('Ctrl Pts',(-2.23767014406945,-6.64713839776805,
62.6230326951094));
#145873=CARTESIAN_POINT('Ctrl Pts',(-2.41172619399862,-6.58598288447688,
62.6146692477894));
#145874=CARTESIAN_POINT('Ctrl Pts',(-2.58306450102135,-6.51808287351912,
62.6063058004694));
#145875=CARTESIAN_POINT('Ctrl Pts',(-2.75450369685442,-6.4501428811267,
62.5979374285166));
#145876=CARTESIAN_POINT('Ctrl Pts',(-2.92322164582076,-6.37545057568158,
62.5895690565638));
#145877=CARTESIAN_POINT('Ctrl Pts',(-3.08867890969278,-6.29425842775136,
62.581200684611));
#145878=CARTESIAN_POINT('Ctrl Pts',(-3.25418574888546,-6.21304195253158,
62.5728298052752));
#145879=CARTESIAN_POINT('Ctrl Pts',(-3.41642966212173,-6.12532190107686,
62.5644589259395));
#145880=CARTESIAN_POINT('Ctrl Pts',(-3.57489582793616,-6.03139671899508,
62.5560880466037));
#145881=CARTESIAN_POINT('Ctrl Pts',(-3.73349626041912,-5.9373919551223,
62.5477100747124));
#145882=CARTESIAN_POINT('Ctrl Pts',(-3.88831226941796,-5.83717172745508,
62.5393321028211));
#145883=CARTESIAN_POINT('Ctrl Pts',(-4.03885706116365,-5.73107845016874,
62.5309541309298));
#145884=CARTESIAN_POINT('Ctrl Pts',(-4.13452950220826,-5.66365530853291,
62.5256298615709));
#145885=CARTESIAN_POINT('Ctrl Pts',(-4.22847752742665,-5.59386107508764,
62.5203055922119));
#145886=CARTESIAN_POINT('Ctrl Pts',(-4.32058308092017,-5.52179213692134,
62.514981322853));
#145887=CARTESIAN_POINT('Ctrl Pts',(-4.45660370082002,-5.41536140312642,
62.5071184916636));
#145888=CARTESIAN_POINT('Ctrl Pts',(-4.58888712415343,-5.30374629795428,
62.4992556604743));
#145889=CARTESIAN_POINT('Ctrl Pts',(-4.71699660523524,-5.18725067725662,
62.491392829285));
#145890=CARTESIAN_POINT('Ctrl Pts',(-4.84500765109107,-5.07084456806625,
62.4835360396435));
#145891=CARTESIAN_POINT('Ctrl Pts',(-4.96885085226277,-4.94956565568039,
62.4756792500021));
#145892=CARTESIAN_POINT('Ctrl Pts',(-5.08812047633635,-4.82375958986212,
62.4678224603606));
#145893=CARTESIAN_POINT('Ctrl Pts',(-5.2073228379878,-4.69802447270971,
62.4599701015766));
#145894=CARTESIAN_POINT('Ctrl Pts',(-5.32195649182377,-4.56776755665584,
62.4521177427926));
#145895=CARTESIAN_POINT('Ctrl Pts',(-5.43165089415382,-4.43337288376897,
62.4442653840086));
#145896=CARTESIAN_POINT('Ctrl Pts',(-5.54131939635566,-4.29900994303236,
62.4364148792581));
#145897=CARTESIAN_POINT('Ctrl Pts',(-5.64605072073865,-4.16051147967919,
62.4285643745076));
#145898=CARTESIAN_POINT('Ctrl Pts',(-5.74551318440802,-4.01829625715845,
62.4207138697572));
#145899=CARTESIAN_POINT('Ctrl Pts',(-5.84495964770179,-3.87610391258475,
62.4128646279055));
#145900=CARTESIAN_POINT('Ctrl Pts',(-5.93913872139395,-3.73019631348123,
62.4050153860538));
#145901=CARTESIAN_POINT('Ctrl Pts',(-6.0277610946666,-3.58102258414042,
62.3971661442021));
#145902=CARTESIAN_POINT('Ctrl Pts',(-6.11641332655142,-3.4317985952504,
62.3893142577872));
#145903=CARTESIAN_POINT('Ctrl Pts',(-6.19950492345108,-3.27930660639255,
62.3814623713722));
#145904=CARTESIAN_POINT('Ctrl Pts',(-6.2767916365877,-3.12402197709343,
62.3736104849573));
#145905=CARTESIAN_POINT('Ctrl Pts',(-6.33354230807208,-3.00999840659495,
62.3678449424937));
#145906=CARTESIAN_POINT('Ctrl Pts',(-6.38716404762343,-2.89446966477233,
62.36207940003));
#145907=CARTESIAN_POINT('Ctrl Pts',(-6.43757652936332,-2.777631183417,62.3563138575664));
#145908=CARTESIAN_POINT('Ctrl Pts',(-6.52200013005579,-2.58196683690949,
62.3466585532067));
#145909=CARTESIAN_POINT('Ctrl Pts',(-6.59737977147073,-2.38272892650724,
62.337003248847));
#145910=CARTESIAN_POINT('Ctrl Pts',(-6.66349814332101,-2.18069233420431,
62.3273479444873));
#145911=CARTESIAN_POINT('Ctrl Pts',(-6.72998279854747,-1.97753649708229,
62.3176391515528));
#145912=CARTESIAN_POINT('Ctrl Pts',(-6.78710332592351,-1.77155094568032,
62.3079303586183));
#145913=CARTESIAN_POINT('Ctrl Pts',(-6.83469119427755,-1.56352897042712,
62.2982215656837));
#145914=CARTESIAN_POINT('Ctrl Pts',(-6.88250805949484,-1.3545059757657,
62.2884660532132));
#145915=CARTESIAN_POINT('Ctrl Pts',(-6.92070031476327,-1.14342695873469,
62.2787105407428));
#145916=CARTESIAN_POINT('Ctrl Pts',(-6.94914935517109,-0.931101391914558,
62.2689550282723));
#145917=CARTESIAN_POINT('Ctrl Pts',(-6.97762656450572,-0.718565590117578,
62.2591898563436));
#145918=CARTESIAN_POINT('Ctrl Pts',(-6.99634126819928,-0.504780809182639,
62.2494246844149));
#145919=CARTESIAN_POINT('Ctrl Pts',(-7.0052266015776,-0.290562941631536,
62.2396595124862));
#145920=CARTESIAN_POINT('Ctrl Pts',(-7.01409982000545,-0.0766371552824991,
62.2299076551478));
#145921=CARTESIAN_POINT('Ctrl Pts',(-7.0131704526151,0.137720499562426,
62.2201557978095));
#145922=CARTESIAN_POINT('Ctrl Pts',(-7.00242371330003,0.351694045888468,
62.2104039404712));
#145923=CARTESIAN_POINT('Ctrl Pts',(-6.99773735664163,0.445002008810862,
62.2061514244075));
#145924=CARTESIAN_POINT('Ctrl Pts',(-6.99118480248129,0.538236889438612,
62.2018989083438));
#145925=CARTESIAN_POINT('Ctrl Pts',(-6.9827679269484,0.631330848985552,
62.1976463922802));
#145926=CARTESIAN_POINT('Ctrl Pts',(-6.9668683644438,0.807186274533022,
62.1896133466813));
#145927=CARTESIAN_POINT('Ctrl Pts',(-6.94430472223171,0.982624320127165,
62.1815803010824));
#145928=CARTESIAN_POINT('Ctrl Pts',(-6.9151109345152,1.15709434613102,62.1735472554835));
#145929=CARTESIAN_POINT('Ctrl Pts',(-6.8859359136895,1.33145221608439,62.1655193738356));
#145930=CARTESIAN_POINT('Ctrl Pts',(-6.85013929144247,1.50484294507663,
62.1574914921877));
#145931=CARTESIAN_POINT('Ctrl Pts',(-6.80780683282828,1.67672081438639,
62.1494636105398));
#145932=CARTESIAN_POINT('Ctrl Pts',(-6.76549348773645,1.8485210791439,62.1414393535596));
#145933=CARTESIAN_POINT('Ctrl Pts',(-6.71665026952844,2.01880948909778,
62.1334150965794));
#145934=CARTESIAN_POINT('Ctrl Pts',(-6.66141405653127,2.18705037206455,
62.1253908395993));
#145935=CARTESIAN_POINT('Ctrl Pts',(-6.60618452215485,2.35527091299494,
62.1173675528335));
#145936=CARTESIAN_POINT('Ctrl Pts',(-6.54456363958376,2.52144406956844,
62.1093442660677));
#145937=CARTESIAN_POINT('Ctrl Pts',(-6.47673824463895,2.68504902616902,
62.1013209793019));
#145938=CARTESIAN_POINT('Ctrl Pts',(-6.40891840738025,2.84864057680276,
62.0932983499729));
#145939=CARTESIAN_POINT('Ctrl Pts',(-6.33489521456378,3.00966400948752,
62.0852757206439));
#145940=CARTESIAN_POINT('Ctrl Pts',(-6.25490365125662,3.16761848649686,
62.0772530913149));
#145941=CARTESIAN_POINT('Ctrl Pts',(-6.17488201681645,3.32563234314437,
62.0692274460484));
#145942=CARTESIAN_POINT('Ctrl Pts',(-6.08888769815882,3.48057461350168,
62.0612018007819));
#145943=CARTESIAN_POINT('Ctrl Pts',(-5.99720182272748,3.63196873058871,
62.0531761555154));
#145944=CARTESIAN_POINT('Ctrl Pts',(-5.94313824351753,3.72123992751572,
62.0484437460081));
#145945=CARTESIAN_POINT('Ctrl Pts',(-5.8870965657202,3.80927792588718,62.0437113365009));
#145946=CARTESIAN_POINT('Ctrl Pts',(-5.82914149318423,3.89598973496311,
62.0389789269936));
#145947=CARTESIAN_POINT('Ctrl Pts',(-5.72222965204512,4.05595017934109,
62.030248878159));
#145948=CARTESIAN_POINT('Ctrl Pts',(-5.60875089324011,4.21147602252567,
62.0215188293245));
#145949=CARTESIAN_POINT('Ctrl Pts',(-5.48909361084644,4.36204973537268,
62.0127887804899));
#145950=CARTESIAN_POINT('Ctrl Pts',(-5.36940172940039,4.51266698679647,
62.0040562073509));
#145951=CARTESIAN_POINT('Ctrl Pts',(-5.24352792879278,4.65832903523479,
61.9953236342118));
#145952=CARTESIAN_POINT('Ctrl Pts',(-5.11190092573161,4.79855139474449,
61.9865910610728));
#145953=CARTESIAN_POINT('Ctrl Pts',(-4.9784039509733,4.94076583671062,61.9777344277923));
#145954=CARTESIAN_POINT('Ctrl Pts',(-4.8389892594256,5.07738464152953,61.9688777945119));
#145955=CARTESIAN_POINT('Ctrl Pts',(-4.69414314874617,5.20794073138121,
61.9600211612314));
#145956=CARTESIAN_POINT('Ctrl Pts',(-4.55123506955074,5.3367499892926,61.9512830291248));
#145957=CARTESIAN_POINT('Ctrl Pts',(-4.40304023448336,5.45965759339595,
61.9425448970182));
#145958=CARTESIAN_POINT('Ctrl Pts',(-4.25006011984992,5.57625461579376,
61.9338067649115));
#145959=CARTESIAN_POINT('Ctrl Pts',(-4.09396807186477,5.69522346386043,
61.9248908810442));
#145960=CARTESIAN_POINT('Ctrl Pts',(-3.93289420718763,5.8076220569043,61.9159749971768));
#145961=CARTESIAN_POINT('Ctrl Pts',(-3.76740442871578,5.913061003659,61.9070591133094));
#145962=CARTESIAN_POINT('Ctrl Pts',(-3.60191465024387,6.01849995041373,
61.898143229442));
#145963=CARTESIAN_POINT('Ctrl Pts',(-3.43200921629051,6.1169790935122,61.8892273455747));
#145964=CARTESIAN_POINT('Ctrl Pts',(-3.25828380186393,6.20815699133093,
61.8803114617073));
#145965=CARTESIAN_POINT('Ctrl Pts',(-3.08797213573309,6.29754322041591,
61.8715707772111));
#145966=CARTESIAN_POINT('Ctrl Pts',(-2.91397113395657,6.37992197706101,
61.8628300927148));
#145967=CARTESIAN_POINT('Ctrl Pts',(-2.73686415547664,6.45501364498691,
61.8540894082186));
#145968=CARTESIAN_POINT('Ctrl Pts',(-2.55978904148388,6.53009180267447,
61.8453502963167));
#145969=CARTESIAN_POINT('Ctrl Pts',(-2.37960931877037,6.59788538310797,
61.8366111844148));
#145970=CARTESIAN_POINT('Ctrl Pts',(-2.1969289224011,6.65816264989205,61.8278720725129));
#145971=CARTESIAN_POINT('Ctrl Pts',(-2.0118816385748,6.71922089542115,61.8190197328385));
#145972=CARTESIAN_POINT('Ctrl Pts',(-1.82426869333963,6.77256658958781,
61.8101673931642));
#145973=CARTESIAN_POINT('Ctrl Pts',(-1.63473565425623,6.81801040650449,
61.8013150534898));
#145974=CARTESIAN_POINT('Ctrl Pts',(-1.44772278169457,6.86284997000673,
61.7925804208401));
#145975=CARTESIAN_POINT('Ctrl Pts',(-1.25884083650483,6.89999643726584,
61.7838457881903));
#145976=CARTESIAN_POINT('Ctrl Pts',(-1.06872316361794,6.92931867949847,
61.7751111555405));
#145977=CARTESIAN_POINT('Ctrl Pts',(-0.874762480986496,6.95923363707903,
61.7661999623539));
#145978=CARTESIAN_POINT('Ctrl Pts',(-0.679515864638774,6.98100461965456,
61.7572887691673));
#145979=CARTESIAN_POINT('Ctrl Pts',(-0.483665567503547,6.99454746079484,
61.7483775759807));
#145980=CARTESIAN_POINT('Ctrl Pts',(-0.287815270368321,7.00809030193511,
61.739466382794));
#145981=CARTESIAN_POINT('Ctrl Pts',(-0.0913615939237434,7.01340496728704,
61.7305551896074));
#145982=CARTESIAN_POINT('Ctrl Pts',(0.105007858588381,7.01046360179801,
61.7216439964208));
#145983=CARTESIAN_POINT('Ctrl Pts',(0.281863570289811,7.00781452741153,
61.7136183315683));
#145984=CARTESIAN_POINT('Ctrl Pts',(0.458732234539534,6.99846700358813,
61.7055926667158));
#145985=CARTESIAN_POINT('Ctrl Pts',(0.635061200245588,6.98242965123478,
61.6975670018633));
#145986=CARTESIAN_POINT('Ctrl Pts',(0.81133420346308,6.96639738874369,61.68954388416));
#145987=CARTESIAN_POINT('Ctrl Pts',(0.98706748452383,6.94367955795302,61.6815207664567));
#145988=CARTESIAN_POINT('Ctrl Pts',(1.16171130126777,6.91433680225419,61.6734976487534));
#145989=CARTESIAN_POINT('Ctrl Pts',(1.33633309389806,6.88499774693364,61.6654755428354));
#145990=CARTESIAN_POINT('Ctrl Pts',(1.50986533457572,6.84903549215138,61.6574534369174));
#145991=CARTESIAN_POINT('Ctrl Pts',(1.68176633953544,6.80656216762218,61.6494313309995));
#145992=CARTESIAN_POINT('Ctrl Pts',(1.85373122348923,6.76407305986213,61.6414062440398));
#145993=CARTESIAN_POINT('Ctrl Pts',(2.02406330386218,6.71506813398563,61.6333811570802));
#145994=CARTESIAN_POINT('Ctrl Pts',(2.19223353945854,6.65971010412414,61.6253560701206));
#145995=CARTESIAN_POINT('Ctrl Pts',(2.36043689534125,6.60434117177568,61.6173294026603));
#145996=CARTESIAN_POINT('Ctrl Pts',(2.52647721282525,6.54261676580371,61.6093027351999));
#145997=CARTESIAN_POINT('Ctrl Pts',(2.68984362316753,6.47474847738544,61.6012760677396));
#145998=CARTESIAN_POINT('Ctrl Pts',(2.85334118348836,6.40682570454437,61.5932429564989));
#145999=CARTESIAN_POINT('Ctrl Pts',(3.01416021447469,6.33274934743334,61.5852098452582));
#146000=CARTESIAN_POINT('Ctrl Pts',(3.17181215965281,6.25277811747535,61.5771767340175));
#146001=CARTESIAN_POINT('Ctrl Pts',(3.26470641275866,6.205656163677,61.5724433330564));
#146002=CARTESIAN_POINT('Ctrl Pts',(3.35650152547001,6.15648838283058,61.5677099320953));
#146003=CARTESIAN_POINT('Ctrl Pts',(3.44710205084303,6.10533488136186,61.5629765311343));
#146004=CARTESIAN_POINT('Ctrl Pts',(3.63374195280158,5.99995707632539,61.5532255778405));
#146005=CARTESIAN_POINT('Ctrl Pts',(3.8154211757974,5.88608855414379,61.5434746245467));
#146006=CARTESIAN_POINT('Ctrl Pts',(3.9914628013073,5.76418695639551,61.5337236712529));
#146007=CARTESIAN_POINT('Ctrl Pts',(4.16775804780412,5.64210973652695,61.5239586698816));
#146008=CARTESIAN_POINT('Ctrl Pts',(4.33839941862934,5.51197631337505,61.5141936685103));
#146009=CARTESIAN_POINT('Ctrl Pts',(4.5027393116297,5.37428741825411,61.5044286671391));
#146010=CARTESIAN_POINT('Ctrl Pts',(4.66680528407829,5.23682802199335,61.4946799420018));
#146011=CARTESIAN_POINT('Ctrl Pts',(4.8245907413907,5.09183834721426,61.4849312168646));
#146012=CARTESIAN_POINT('Ctrl Pts',(4.97548376535131,4.93985706910894,61.4751824917274));
#146013=CARTESIAN_POINT('Ctrl Pts',(5.12596264647027,4.78829292068092,61.4654605230606));
#146014=CARTESIAN_POINT('Ctrl Pts',(5.26958683091385,4.62977550544657,61.4557385543938));
#146015=CARTESIAN_POINT('Ctrl Pts',(5.40578224980526,4.46487903869639,61.4460165857269));
#146016=CARTESIAN_POINT('Ctrl Pts',(5.54107649918223,4.30107364879802,61.4363589447875));
#146017=CARTESIAN_POINT('Ctrl Pts',(5.66903991448771,4.13097336299275,61.4267013038482));
#146018=CARTESIAN_POINT('Ctrl Pts',(5.78914287362294,3.95518031842806,61.4170436629088));
#146019=CARTESIAN_POINT('Ctrl Pts',(5.8419322590775,3.8779132231244,61.4127987972218));
#146020=CARTESIAN_POINT('Ctrl Pts',(5.89320351581207,3.79954685127154,61.4085539315349));
#146021=CARTESIAN_POINT('Ctrl Pts',(5.94291376581599,3.7201347468304,61.404309065848));
#146022=CARTESIAN_POINT('Ctrl Pts',(6.03486251755945,3.57324665280332,61.3964573632072));
#146023=CARTESIAN_POINT('Ctrl Pts',(6.12142950456126,3.42283903687358,61.3886056605664));
#146024=CARTESIAN_POINT('Ctrl Pts',(6.20232953860754,3.26936306595281,61.3807539579256));
#146025=CARTESIAN_POINT('Ctrl Pts',(6.28321295025175,3.11591862949711,61.3729038685617));
#146026=CARTESIAN_POINT('Ctrl Pts',(6.35843154219062,2.95940742648086,61.3650537791978));
#146027=CARTESIAN_POINT('Ctrl Pts',(6.42774524540919,2.80030670152746,61.3572036898339));
#146028=CARTESIAN_POINT('Ctrl Pts',(6.47875690302238,2.68321597732042,61.3514263896426));
#146029=CARTESIAN_POINT('Ctrl Pts',(6.52657123496308,2.56472326869091,61.3456490894513));
#146030=CARTESIAN_POINT('Ctrl Pts',(6.57110895151815,2.44502632087632,61.3398717892601));
#146031=CARTESIAN_POINT('Origin',(0.,0.,50.));
#146032=CARTESIAN_POINT('',(6.57110895151816,2.4450263208763,59.3399667921338));
#146033=CARTESIAN_POINT('',(6.57110895151811,2.44502632087644,59.8868036378692));
#146034=CARTESIAN_POINT('',(6.57110895151814,2.44502632087636,50.));
#146035=CARTESIAN_POINT('',(7.01124996031773,0.000745952195652544,61.7735343568788));
#146036=CARTESIAN_POINT('Ctrl Pts',(6.57110895151811,2.44502632087643,59.8868036378692));
#146037=CARTESIAN_POINT('Ctrl Pts',(6.50640911017929,2.61890980955436,59.8952320262474));
#146038=CARTESIAN_POINT('Ctrl Pts',(6.43483843042466,2.79012927483976,59.9036604146256));
#146039=CARTESIAN_POINT('Ctrl Pts',(6.35665295223755,2.95813958550128,59.9120888030038));
#146040=CARTESIAN_POINT('Ctrl Pts',(6.27841693811276,3.12625849124703,59.9205226391521));
#146041=CARTESIAN_POINT('Ctrl Pts',(6.1935577387562,3.29116381664877,59.9289564753004));
#146042=CARTESIAN_POINT('Ctrl Pts',(6.102377161576,3.45233537484058,59.9373903114487));
#146043=CARTESIAN_POINT('Ctrl Pts',(6.01109044809208,3.61369454045911,59.9458339647777));
#146044=CARTESIAN_POINT('Ctrl Pts',(5.91346782168328,3.77131098065186,59.9542776181066));
#146045=CARTESIAN_POINT('Ctrl Pts',(5.80985483003942,3.9246927798705,59.9627212714355));
#146046=CARTESIAN_POINT('Ctrl Pts',(5.78906647449476,3.95546648233435,59.9644153608032));
#146047=CARTESIAN_POINT('Ctrl Pts',(5.76803711304307,3.98606982641891,59.9661094501708));
#146048=CARTESIAN_POINT('Ctrl Pts',(5.74676973213664,4.01649899891662,59.9678035395385));
#146049=CARTESIAN_POINT('Ctrl Pts',(5.64155196050998,4.16704361636331,59.9761848399435));
#146050=CARTESIAN_POINT('Ctrl Pts',(5.53029242921032,4.31362675215176,59.9845661403485));
#146051=CARTESIAN_POINT('Ctrl Pts',(5.41331025385377,4.45574894468053,59.9929474407534));
#146052=CARTESIAN_POINT('Ctrl Pts',(5.29647633627894,4.59769101813617,60.0013181190871));
#146053=CARTESIAN_POINT('Ctrl Pts',(5.17393443489199,4.73518316442958,60.0096887974208));
#146054=CARTESIAN_POINT('Ctrl Pts',(5.04604670722158,4.86775504632662,60.0180594757544));
#146055=CARTESIAN_POINT('Ctrl Pts',(4.918304110165,5.000176481899,60.0264206548054));
#146056=CARTESIAN_POINT('Ctrl Pts',(4.78522800431385,5.12768854753524,60.0347818338563));
#146057=CARTESIAN_POINT('Ctrl Pts',(4.64722083486221,5.24985381458594,60.0431430129072));
#146058=CARTESIAN_POINT('Ctrl Pts',(4.50939274599253,5.37186055779179,60.051493342342));
#146059=CARTESIAN_POINT('Ctrl Pts',(4.36664660046041,5.48853412504243,60.0598436717768));
#146060=CARTESIAN_POINT('Ctrl Pts',(4.21942164594463,5.59947386244761,60.0681940012116));
#146061=CARTESIAN_POINT('Ctrl Pts',(4.07230997222455,5.71032823836112,60.0765379055674));
#146062=CARTESIAN_POINT('Ctrl Pts',(3.92072661768556,5.81545738007573,60.0848818099233));
#146063=CARTESIAN_POINT('Ctrl Pts',(3.76514473326157,5.91450012258793,60.0932257142791));
#146064=CARTESIAN_POINT('Ctrl Pts',(3.60968781317767,6.01346331335153,60.1015629167589));
#146065=CARTESIAN_POINT('Ctrl Pts',(3.45023904397216,6.10634967915229,60.1099001192387));
#146066=CARTESIAN_POINT('Ctrl Pts',(3.28730157291819,6.19284061890742,60.1182373217184));
#146067=CARTESIAN_POINT('Ctrl Pts',(3.23366345685152,6.22131295885042,60.120981882754));
#146068=CARTESIAN_POINT('Ctrl Pts',(3.17964750749847,6.2490925814078,60.1237264437895));
#146069=CARTESIAN_POINT('Ctrl Pts',(3.125272337548,6.27616916427985,60.126471004825));
#146070=CARTESIAN_POINT('Ctrl Pts',(2.96007395649831,6.35843111691184,60.1348093151269));
#146071=CARTESIAN_POINT('Ctrl Pts',(2.79169365377402,6.43413296875797,60.1431476254287));
#146072=CARTESIAN_POINT('Ctrl Pts',(2.62068329858579,6.50304894730261,60.1514859357305));
#146073=CARTESIAN_POINT('Ctrl Pts',(2.4495653494853,6.57200828544228,60.1598294922142));
#146074=CARTESIAN_POINT('Ctrl Pts',(2.27581435123775,6.63417311187902,60.1681730486979));
#146075=CARTESIAN_POINT('Ctrl Pts',(2.09999932366907,6.68936689105101,60.1765166051816));
#146076=CARTESIAN_POINT('Ctrl Pts',(1.92405053679387,6.74460266140958,60.1848665094067));
#146077=CARTESIAN_POINT('Ctrl Pts',(1.74603490060753,6.79285670764081,60.1932164136319));
#146078=CARTESIAN_POINT('Ctrl Pts',(1.56653408797299,6.83400303729217,60.201566317857));
#146079=CARTESIAN_POINT('Ctrl Pts',(1.38676403740216,6.87521108339328,60.2099287463205));
#146080=CARTESIAN_POINT('Ctrl Pts',(1.20550467847311,6.90929003551477,60.2182911747841));
#146081=CARTESIAN_POINT('Ctrl Pts',(1.02334681551833,6.9361652126855,60.2266536032477));
#146082=CARTESIAN_POINT('Ctrl Pts',(0.841033182758529,6.9630633717964,60.2350231827276));
#146083=CARTESIAN_POINT('Ctrl Pts',(0.657819837930774,6.98274542983082,
60.2433927622075));
#146084=CARTESIAN_POINT('Ctrl Pts',(0.474300687196313,6.99518873373872,
60.2517623416874));
#146085=CARTESIAN_POINT('Ctrl Pts',(0.290498480531814,7.00765122992681,
60.2601448302239));
#146086=CARTESIAN_POINT('Ctrl Pts',(0.106389852311009,7.01285265196089,
60.2685273187603));
#146087=CARTESIAN_POINT('Ctrl Pts',(-0.077431893973664,7.01082240998128,
60.2769098072968));
#146088=CARTESIAN_POINT('Ctrl Pts',(-0.137581381466362,7.01015808153794,
60.2796526949017));
#146089=CARTESIAN_POINT('Ctrl Pts',(-0.197700200067954,7.00871986780067,
60.2823955825065));
#146090=CARTESIAN_POINT('Ctrl Pts',(-0.257767731965874,7.00650999848407,
60.2851384701114));
#146091=CARTESIAN_POINT('Ctrl Pts',(-0.441500339135086,6.99975052230428,
60.2935283252442));
#146092=CARTESIAN_POINT('Ctrl Pts',(-0.62512358458665,6.98575389272276,
60.301918180377));
#146093=CARTESIAN_POINT('Ctrl Pts',(-0.80804424770065,6.96453092865973,
60.3103080355098));
#146094=CARTESIAN_POINT('Ctrl Pts',(-0.990796114190584,6.94332754885046,
60.3186901486019));
#146095=CARTESIAN_POINT('Ctrl Pts',(-1.17284636583484,6.91491116563024,
60.3270722616939));
#146096=CARTESIAN_POINT('Ctrl Pts',(-1.35360443769803,6.8793445609843,60.335454374786));
#146097=CARTESIAN_POINT('Ctrl Pts',(-1.53422227960854,6.84380554848533,
60.3438299851349));
#146098=CARTESIAN_POINT('Ctrl Pts',(-1.71354961894826,6.80112743693797,
60.3522055954838));
#146099=CARTESIAN_POINT('Ctrl Pts',(-1.89100319271688,6.75142455246554,
60.3605812058327));
#146100=CARTESIAN_POINT('Ctrl Pts',(-2.06834514555234,6.70175293184556,
60.3689515477982));
#146101=CARTESIAN_POINT('Ctrl Pts',(-2.24381536716304,6.64506543719745,
60.3773218897638));
#146102=CARTESIAN_POINT('Ctrl Pts',(-2.41684248557271,6.58152709957429,
60.3856922317294));
#146103=CARTESIAN_POINT('Ctrl Pts',(-2.58978613118775,6.51801941450234,
60.3940585356237));
#146104=CARTESIAN_POINT('Ctrl Pts',(-2.7602887159284,6.44766759032323,60.4024248395181));
#146105=CARTESIAN_POINT('Ctrl Pts',(-2.92779525274036,6.37068611065802,
60.4107911434124));
#146106=CARTESIAN_POINT('Ctrl Pts',(-3.095254942669,6.29372616055497,60.419155107486));
#146107=CARTESIAN_POINT('Ctrl Pts',(-3.25971995648313,6.21014038788013,
60.4275190715596));
#146108=CARTESIAN_POINT('Ctrl Pts',(-3.42065596391864,6.12019111948376,
60.4358830356332));
#146109=CARTESIAN_POINT('Ctrl Pts',(-3.58156720597674,6.03025569278518,
60.4442457126318));
#146110=CARTESIAN_POINT('Ctrl Pts',(-3.7389502375947,5.93395888306578,60.4526083896303));
#146111=CARTESIAN_POINT('Ctrl Pts',(-3.89229561965895,5.83160881504271,
60.4609710666288));
#146112=CARTESIAN_POINT('Ctrl Pts',(-4.04563784462231,5.72926085422029,
60.4693335714551));
#146113=CARTESIAN_POINT('Ctrl Pts',(-4.19494231265859,5.62086006638129,
60.4776960762814));
#146114=CARTESIAN_POINT('Ctrl Pts',(-4.33972849283295,5.50675795464027,
60.4860585811077));
#146115=CARTESIAN_POINT('Ctrl Pts',(-4.48453099109167,5.39264298305391,
60.4944220284277));
#146116=CARTESIAN_POINT('Ctrl Pts',(-4.62481392844133,5.27282561030957,
60.5027854757477));
#146117=CARTESIAN_POINT('Ctrl Pts',(-4.76012946021177,5.14769794029564,
60.5111489230676));
#146118=CARTESIAN_POINT('Ctrl Pts',(-4.89552466957032,5.02249659159293,
60.5195172950204));
#146119=CARTESIAN_POINT('Ctrl Pts',(-5.02594638640059,4.8919789200875,60.5278856669733));
#146120=CARTESIAN_POINT('Ctrl Pts',(-5.15098254250197,4.75657496622727,
60.5362540389261));
#146121=CARTESIAN_POINT('Ctrl Pts',(-5.27605616270253,4.62113044180477,
60.5446249182618));
#146122=CARTESIAN_POINT('Ctrl Pts',(-5.39574078546182,4.4807969608252,60.5529957975974));
#146123=CARTESIAN_POINT('Ctrl Pts',(-5.50966388458844,4.33603856548369,
60.5613666769331));
#146124=CARTESIAN_POINT('Ctrl Pts',(-5.62368350952584,4.19115751791814,
60.5697446488244));
#146125=CARTESIAN_POINT('Ctrl Pts',(-5.73193165718387,4.0418443262551,60.5781226207157));
#146126=CARTESIAN_POINT('Ctrl Pts',(-5.83407780103488,3.88859393276954,
60.586500592607));
#146127=CARTESIAN_POINT('Ctrl Pts',(-5.89899250723227,3.79120205978547,
60.5918248619661));
#146128=CARTESIAN_POINT('Ctrl Pts',(-5.96144366641336,3.69222065152036,
60.5971491313251));
#146129=CARTESIAN_POINT('Ctrl Pts',(-6.02135593370052,3.59178218746482,
60.6024734006842));
#146130=CARTESIAN_POINT('Ctrl Pts',(-6.1098338096449,3.44345560319192,60.6103362318735));
#146131=CARTESIAN_POINT('Ctrl Pts',(-6.19295614891969,3.29164153103617,
60.6181990630628));
#146132=CARTESIAN_POINT('Ctrl Pts',(-6.27042519721603,3.13678089904576,
60.6260618942521));
#146133=CARTESIAN_POINT('Ctrl Pts',(-6.34783472077468,2.98203925700939,
60.6339186838935));
#146134=CARTESIAN_POINT('Ctrl Pts',(-6.41959942216613,2.82425604909458,
60.6417754735349));
#146135=CARTESIAN_POINT('Ctrl Pts',(-6.485465547011,2.66389999831701,60.6496322631763));
#146136=CARTESIAN_POINT('Ctrl Pts',(-6.5512945264794,2.50363438076118,60.6574846219603));
#146137=CARTESIAN_POINT('Ctrl Pts',(-6.61123140219648,2.34079915821796,
60.6653369807442));
#146138=CARTESIAN_POINT('Ctrl Pts',(-6.66506908723143,2.17588617003095,
60.6731893395282));
#146139=CARTESIAN_POINT('Ctrl Pts',(-6.71889406056072,2.01101211972483,
60.6810398442786));
#146140=CARTESIAN_POINT('Ctrl Pts',(-6.7666225831489,1.84406163967337,60.6888903490291));
#146141=CARTESIAN_POINT('Ctrl Pts',(-6.80809633639751,1.67554493727587,
60.6967408537795));
#146142=CARTESIAN_POINT('Ctrl Pts',(-6.84956341782639,1.5070553439045,60.7045900956312));
#146143=CARTESIAN_POINT('Ctrl Pts',(-6.88477764469766,1.33700040095018,
60.7124393374828));
#146144=CARTESIAN_POINT('Ctrl Pts',(-6.91363116893276,1.16590335039466,
60.7202885793345));
#146145=CARTESIAN_POINT('Ctrl Pts',(-6.94249441448492,0.994748653893899,
60.7281404657493));
#146146=CARTESIAN_POINT('Ctrl Pts',(-6.9649926132986,0.822551525024216,
60.7359923521642));
#146147=CARTESIAN_POINT('Ctrl Pts',(-6.98106940870049,0.649843422222746,
60.7438442385791));
#146148=CARTESIAN_POINT('Ctrl Pts',(-6.99287439946007,0.523026011992201,
60.7496097810429));
#146149=CARTESIAN_POINT('Ctrl Pts',(-7.00121818321514,0.39593328043947,
60.7553753235068));
#146150=CARTESIAN_POINT('Ctrl Pts',(-7.00609632877495,0.268776476698001,
60.7611408659707));
#146151=CARTESIAN_POINT('Ctrl Pts',(-7.0142655479574,0.0558324823935959,
60.7707961703308));
#146152=CARTESIAN_POINT('Ctrl Pts',(-7.01271064726126,-0.157182581790572,
60.780451474691));
#146153=CARTESIAN_POINT('Ctrl Pts',(-7.00150842649691,-0.369467611831974,
60.7901067790512));
#146154=CARTESIAN_POINT('Ctrl Pts',(-6.99024414753111,-0.582928661114273,
60.7998155719861));
#146155=CARTESIAN_POINT('Ctrl Pts',(-6.9692254208665,-0.79565152111639,
60.8095243649211));
#146156=CARTESIAN_POINT('Ctrl Pts',(-6.93858118164358,-1.00683551200857,
60.819233157856));
#146157=CARTESIAN_POINT('Ctrl Pts',(-6.90778947973966,-1.2190357381956,
60.8289886703269));
#146158=CARTESIAN_POINT('Ctrl Pts',(-6.86727943477904,-1.4296822099299,
60.8387441827978));
#146159=CARTESIAN_POINT('Ctrl Pts',(-6.81723238419103,-1.63797716175688,
60.8484996952686));
#146160=CARTESIAN_POINT('Ctrl Pts',(-6.7671357793234,-1.84647835763151,
60.8582648671977));
#146161=CARTESIAN_POINT('Ctrl Pts',(-6.70748330029079,-2.05262334166574,
60.8680300391268));
#146162=CARTESIAN_POINT('Ctrl Pts',(-6.6385068576747,-2.25562702216169,
60.8777952110558));
#146163=CARTESIAN_POINT('Ctrl Pts',(-6.56962446287299,-2.45835391174557,
60.8875470683946));
#146164=CARTESIAN_POINT('Ctrl Pts',(-6.49144352547867,-2.65794802224537,
60.8972989257333));
#146165=CARTESIAN_POINT('Ctrl Pts',(-6.40424455972472,-2.85364296675958,
60.907050783072));
#146166=CARTESIAN_POINT('Ctrl Pts',(-6.36621949541621,-2.93898013544801,
60.9113032991337));
#146167=CARTESIAN_POINT('Ctrl Pts',(-6.32648020592294,-3.02357604429839,
60.9155558151954));
#146168=CARTESIAN_POINT('Ctrl Pts',(-6.28505290906144,-3.1073680974095,
60.9198083312571));
#146169=CARTESIAN_POINT('Ctrl Pts',(-6.20679632874754,-3.2656521282474,
60.9278413768558));
#146170=CARTESIAN_POINT('Ctrl Pts',(-6.12247476553096,-3.42114328480263,
60.9358744224545));
#146171=CARTESIAN_POINT('Ctrl Pts',(-6.03231847320822,-3.57334023013354,
60.9439074680532));
#146172=CARTESIAN_POINT('Ctrl Pts',(-5.94222013682133,-3.72543933740822,
60.9519353497009));
#146173=CARTESIAN_POINT('Ctrl Pts',(-5.84629472340964,-3.87424813461167,
60.9599632313486));
#146174=CARTESIAN_POINT('Ctrl Pts',(-5.74481905403682,-4.0192885687489,
60.9679911129963));
#146175=CARTESIAN_POINT('Ctrl Pts',(-5.6433892019298,-4.16426351569925,
60.9760153699762));
#146176=CARTESIAN_POINT('Ctrl Pts',(-5.53641429329042,-4.30547318763866,
60.9840396269562));
#146177=CARTESIAN_POINT('Ctrl Pts',(-5.4242151984711,-4.44246733732226,
60.9920638839361));
#146178=CARTESIAN_POINT('Ctrl Pts',(-5.31202966966456,-4.57944492301854,
61.0000871707017));
#146179=CARTESIAN_POINT('Ctrl Pts',(-5.19462143899718,-4.71220771337947,
61.0081104574673));
#146180=CARTESIAN_POINT('Ctrl Pts',(-5.07235261325369,-4.84033733631433,
61.0161337442329));
#146181=CARTESIAN_POINT('Ctrl Pts',(-4.95009380634964,-4.9684564601697,
61.0241563735617));
#146182=CARTESIAN_POINT('Ctrl Pts',(-4.82297545373627,-5.09194291034018,
61.0321790028905));
#146183=CARTESIAN_POINT('Ctrl Pts',(-4.69139736494629,-5.21041431430122,
61.0402016322193));
#146184=CARTESIAN_POINT('Ctrl Pts',(-4.55976981216225,-5.32893025507591,
61.0482272774856));
#146185=CARTESIAN_POINT('Ctrl Pts',(-4.42367944863565,-5.44242714022515,
61.0562529227519));
#146186=CARTESIAN_POINT('Ctrl Pts',(-4.28356036651973,-5.55056187686268,
61.0642785680182));
#146187=CARTESIAN_POINT('Ctrl Pts',(-4.20093761725585,-5.61432470699975,
61.0690109775266));
#146188=CARTESIAN_POINT('Ctrl Pts',(-4.1169147023471,-5.67622388779455,
61.073743387035));
#146189=CARTESIAN_POINT('Ctrl Pts',(-4.03158551017731,-5.73619602494792,
61.0784757965434));
#146190=CARTESIAN_POINT('Ctrl Pts',(-3.8741756297881,-5.84682881890682,
61.0872058453782));
#146191=CARTESIAN_POINT('Ctrl Pts',(-3.71224031257441,-5.95095695938307,
61.095935894213));
#146192=CARTESIAN_POINT('Ctrl Pts',(-3.54632847140008,-6.04823783720822,
61.1046659430478));
#146193=CARTESIAN_POINT('Ctrl Pts',(-3.3803686566086,-6.14554684392132,
61.1133985161871));
#146194=CARTESIAN_POINT('Ctrl Pts',(-3.2104302590754,-6.23600449744522,
61.1221310893265));
#146195=CARTESIAN_POINT('Ctrl Pts',(-3.03708788223122,-6.31931355117819,
61.1308636624658));
#146196=CARTESIAN_POINT('Ctrl Pts',(-2.86128290022261,-6.40380614300324,
61.1397202957462));
#146197=CARTESIAN_POINT('Ctrl Pts',(-2.68197674508946,-6.48094534691311,
61.1485769290265));
#146198=CARTESIAN_POINT('Ctrl Pts',(-2.49979144672779,-6.5504709208855,
61.1574335623069));
#146199=CARTESIAN_POINT('Ctrl Pts',(-2.32004377573059,-6.61906624722997,
61.1661716944138));
#146200=CARTESIAN_POINT('Ctrl Pts',(-2.13749379628574,-6.68025034070188,
61.1749098265207));
#146201=CARTESIAN_POINT('Ctrl Pts',(-1.95275672186057,-6.73382266975663,
61.1836479586276));
#146202=CARTESIAN_POINT('Ctrl Pts',(-1.76426171155767,-6.78848477127875,
61.1925638424947));
#146203=CARTESIAN_POINT('Ctrl Pts',(-1.57348995649215,-6.83522202694157,
61.2014797263617));
#146204=CARTESIAN_POINT('Ctrl Pts',(-1.3811097137541,-6.87387536409223,
61.2103956102288));
#146205=CARTESIAN_POINT('Ctrl Pts',(-1.18872947101606,-6.91252870124289,
61.2193114940959));
#146206=CARTESIAN_POINT('Ctrl Pts',(-0.994741038290665,-6.94309806627461,
61.228227377963));
#146207=CARTESIAN_POINT('Ctrl Pts',(-0.799823146438977,-6.96547984685337,
61.23714326183));
#146208=CARTESIAN_POINT('Ctrl Pts',(-0.608735440416435,-6.98742181978806,
61.2458839463261));
#146209=CARTESIAN_POINT('Ctrl Pts',(-0.416734168987128,-7.0014973280946,
61.2546246308223));
#146210=CARTESIAN_POINT('Ctrl Pts',(-0.224464276884863,-7.00765598120388,
61.2633653153184));
#146211=CARTESIAN_POINT('Ctrl Pts',(-0.0322289773305222,-7.01381352626916,
61.2721044272201));
#146212=CARTESIAN_POINT('Ctrl Pts',(0.160274572823184,-7.01205705195798,
61.2808435391219));
#146213=CARTESIAN_POINT('Ctrl Pts',(0.352399506920261,-7.00238824616447,
61.2895826510236));
#146214=CARTESIAN_POINT('Ctrl Pts',(0.547013696058328,-6.99259416707588,
61.298434990698));
#146215=CARTESIAN_POINT('Ctrl Pts',(0.741239103930971,-6.97468128782271,
61.3072873303724));
#146216=CARTESIAN_POINT('Ctrl Pts',(0.934405330199851,-6.94870586810192,
61.3161396700468));
#146217=CARTESIAN_POINT('Ctrl Pts',(1.12500308049431,-6.92307583609599,
61.3248743026965));
#146218=CARTESIAN_POINT('Ctrl Pts',(1.31456936493636,-6.88959639389009,
61.3336089353461));
#146219=CARTESIAN_POINT('Ctrl Pts',(1.50246617354109,-6.84837367262219,
61.3423435679958));
#146220=CARTESIAN_POINT('Ctrl Pts',(1.69416109968256,-6.8063176815307,61.3512547611826));
#146221=CARTESIAN_POINT('Ctrl Pts',(1.8841180498202,-6.7562020754472,61.3601659543693));
#146222=CARTESIAN_POINT('Ctrl Pts',(2.07167033624739,-6.69819442688943,
61.3690771475561));
#146223=CARTESIAN_POINT('Ctrl Pts',(2.25922262267458,-6.64018677833167,
61.3779883407428));
#146224=CARTESIAN_POINT('Ctrl Pts',(2.44436995181516,-6.57428716399544,
61.3868995339296));
#146225=CARTESIAN_POINT('Ctrl Pts',(2.62646095606154,-6.50071760721724,
61.3958107271163));
#146226=CARTESIAN_POINT('Ctrl Pts',(2.79045710585923,-6.43445884773662,
61.4038363919688));
#146227=CARTESIAN_POINT('Ctrl Pts',(2.95204935192849,-6.36194783750196,
61.4118620568212));
#146228=CARTESIAN_POINT('Ctrl Pts',(3.11072535130985,-6.28339194633108,
61.4198877216737));
#146229=CARTESIAN_POINT('Ctrl Pts',(3.26935099082007,-6.20486098687369,
61.4279108393769));
#146230=CARTESIAN_POINT('Ctrl Pts',(3.42506189819082,-6.12028912847259,
61.4359339570802));
#146231=CARTESIAN_POINT('Ctrl Pts',(3.57736720696945,-6.02993121262586,
61.4439570747834));
#146232=CARTESIAN_POINT('Ctrl Pts',(3.72965330871607,-5.93958469170289,
61.4519791807013));
#146233=CARTESIAN_POINT('Ctrl Pts',(3.87853435246432,-5.84345375424984,
61.4600012866192));
#146234=CARTESIAN_POINT('Ctrl Pts',(4.02354555774109,-5.74183835607395,
61.4680233925371));
#146235=CARTESIAN_POINT('Ctrl Pts',(4.1686106496721,-5.64018519727249,61.4760484794967));
#146236=CARTESIAN_POINT('Ctrl Pts',(4.30980272816781,-5.53304371448372,
61.4840735664563));
#146237=CARTESIAN_POINT('Ctrl Pts',(4.44668704905208,-5.4207564832127,61.4920986534159));
#146238=CARTESIAN_POINT('Ctrl Pts',(4.58359832861805,-5.30844713753364,
61.5001253208762));
#146239=CARTESIAN_POINT('Ctrl Pts',(4.7161998826159,-5.19099026374683,61.5081519883365));
#146240=CARTESIAN_POINT('Ctrl Pts',(4.84409154502365,-5.06876747009866,
61.5161786557968));
#146241=CARTESIAN_POINT('Ctrl Pts',(4.97208587840775,-4.94644655642203,
61.5242117670375));
#146242=CARTESIAN_POINT('Ctrl Pts',(5.09536250989122,-4.81935234121083,
61.5322448782781));
#146243=CARTESIAN_POINT('Ctrl Pts',(5.21355907913378,-4.68790233376099,
61.5402779895188));
#146244=CARTESIAN_POINT('Ctrl Pts',(5.283204791451,-4.61044721419521,61.5450113904802));
#146245=CARTESIAN_POINT('Ctrl Pts',(5.35108746100097,-4.53148040745293,
61.5497447914415));
#146246=CARTESIAN_POINT('Ctrl Pts',(5.41713974441693,-4.45109239984506,
61.5544781924029));
#146247=CARTESIAN_POINT('Ctrl Pts',(5.5532095039421,-4.28549060232616,61.5642291456968));
#146248=CARTESIAN_POINT('Ctrl Pts',(5.68159006986931,-4.11375880356511,
61.5739800989907));
#146249=CARTESIAN_POINT('Ctrl Pts',(5.80181514815839,-3.93656799116945,
61.5837310522846));
#146250=CARTESIAN_POINT('Ctrl Pts',(5.92221343322642,-3.75912190216833,
61.593496053656));
#146251=CARTESIAN_POINT('Ctrl Pts',(6.03443270648752,-3.57620109972098,
61.6032610550274));
#146252=CARTESIAN_POINT('Ctrl Pts',(6.13804955852324,-3.38850618704064,
61.6130260563988));
#146253=CARTESIAN_POINT('Ctrl Pts',(6.24149370273561,-3.2011241228901,61.6227747815362));
#146254=CARTESIAN_POINT('Ctrl Pts',(6.33636406414719,-3.00898388541046,
61.6325235066736));
#146255=CARTESIAN_POINT('Ctrl Pts',(6.42228420093148,-2.81280859728597,
61.6422722318109));
#146256=CARTESIAN_POINT('Ctrl Pts',(6.50796852025351,-2.61717173426571,
61.6519942004776));
#146257=CARTESIAN_POINT('Ctrl Pts',(6.58475163872778,-2.41752196590726,
61.6617161691443));
#146258=CARTESIAN_POINT('Ctrl Pts',(6.65230523477775,-2.2146019113711,61.6714381378109));
#146259=CARTESIAN_POINT('Ctrl Pts',(6.71941184632809,-2.01302452583181,
61.6810957787504));
#146260=CARTESIAN_POINT('Ctrl Pts',(6.77741062828986,-1.80822002349115,
61.6907534196898));
#146261=CARTESIAN_POINT('Ctrl Pts',(6.82602478497098,-1.60094103497345,
61.7004110606292));
#146262=CARTESIAN_POINT('Ctrl Pts',(6.84739238052307,-1.50983478330803,
61.7046559263159));
#146263=CARTESIAN_POINT('Ctrl Pts',(6.86694754704264,-1.41825080290872,
61.7089007920025));
#146264=CARTESIAN_POINT('Ctrl Pts',(6.88466960476102,-1.32625449887257,
61.7131456576892));
#146265=CARTESIAN_POINT('Ctrl Pts',(6.91599476258385,-1.16364365599851,
61.720648798108));
#146266=CARTESIAN_POINT('Ctrl Pts',(6.941587348978,-0.999751854661091,61.7281519385268));
#146267=CARTESIAN_POINT('Ctrl Pts',(6.9613427933109,-0.835064713970333,
61.7356550789455));
#146268=CARTESIAN_POINT('Ctrl Pts',(6.98109422577986,-0.670411017346532,
61.7431566956538));
#146269=CARTESIAN_POINT('Ctrl Pts',(6.99501081379055,-0.504962703708429,
61.750658312362));
#146270=CARTESIAN_POINT('Ctrl Pts',(7.00303936527326,-0.33921410780379,
61.7581599290703));
#146271=CARTESIAN_POINT('Ctrl Pts',(7.00852415564041,-0.225981190988831,
61.7632847383398));
#146272=CARTESIAN_POINT('Ctrl Pts',(7.01126202048759,-0.112608316252692,
61.7684095476093));
#146273=CARTESIAN_POINT('Ctrl Pts',(7.01124996031773,0.000745952195671065,
61.7735343568789));
#146274=CARTESIAN_POINT('Ctrl Pts',(7.01124996031765,0.000745952895824991,
61.7735343569105));
#146275=CARTESIAN_POINT('Ctrl Pts',(7.01123049451363,0.183706054626861,
61.7818060844611));
#146276=CARTESIAN_POINT('Ctrl Pts',(7.00404513626102,0.366557650708819,
61.7900778120117));
#146277=CARTESIAN_POINT('Ctrl Pts',(6.98974513960821,0.548716179662563,
61.7983495395624));
#146278=CARTESIAN_POINT('Ctrl Pts',(6.97543598949126,0.730991308752774,
61.8066265618668));
#146279=CARTESIAN_POINT('Ctrl Pts',(6.95400315525616,0.912572151228788,
61.8149035841712));
#146280=CARTESIAN_POINT('Ctrl Pts',(6.9255494732271,1.0928819956353,61.8231806064756));
#146281=CARTESIAN_POINT('Ctrl Pts',(6.89705104070401,1.27347542213181,61.8314706464568));
#146282=CARTESIAN_POINT('Ctrl Pts',(6.86150975109376,1.45279352336208,61.839760686438));
#146283=CARTESIAN_POINT('Ctrl Pts',(6.81907938419261,1.63027081019669,61.8480507264193));
#146284=CARTESIAN_POINT('Ctrl Pts',(6.7785388798998,1.7998431998382,61.8559715252714));
#146285=CARTESIAN_POINT('Ctrl Pts',(6.73170975517686,1.96773496389655,61.8638923241236));
#146286=CARTESIAN_POINT('Ctrl Pts',(6.67876767326888,2.13346875510251,61.8718131229757));
#146287=CARTESIAN_POINT('Ctrl Pts',(6.64534233145582,2.23810590614353,61.8768139729522));
#146288=CARTESIAN_POINT('Ctrl Pts',(6.60944418485232,2.34199880220716,61.8818148229287));
#146289=CARTESIAN_POINT('Ctrl Pts',(6.57110895151817,2.44502632087627,61.8868156729052));
#146290=CARTESIAN_POINT('',(7.01124977383073,-0.00178085893519804,61.2264656430588));
#146291=CARTESIAN_POINT('Ctrl Pts',(6.57110895151815,2.44502632087632,61.3398717892601));
#146292=CARTESIAN_POINT('Ctrl Pts',(6.63164596423562,2.2823306055912,61.3320191079328));
#146293=CARTESIAN_POINT('Ctrl Pts',(6.68612743998776,2.11740963806755,61.3241664266055));
#146294=CARTESIAN_POINT('Ctrl Pts',(6.7343971179006,1.95077472326052,61.3163137452782));
#146295=CARTESIAN_POINT('Ctrl Pts',(6.78267671899837,1.78410555197722,61.3084594496122));
#146296=CARTESIAN_POINT('Ctrl Pts',(6.82474188414918,1.61572210142618,61.3006051539462));
#146297=CARTESIAN_POINT('Ctrl Pts',(6.86048707053804,1.4461478892148,61.2927508582802));
#146298=CARTESIAN_POINT('Ctrl Pts',(6.89626942910293,1.27639733319035,61.2848883947658));
#146299=CARTESIAN_POINT('Ctrl Pts',(6.92571861128505,1.10545391742226,61.2770259312515));
#146300=CARTESIAN_POINT('Ctrl Pts',(6.94878064777434,0.933849062545336,
61.2691634677372));
#146301=CARTESIAN_POINT('Ctrl Pts',(6.97177862027636,0.762720908468189,
61.2613228453453));
#146302=CARTESIAN_POINT('Ctrl Pts',(6.98842491556832,0.59093536336877,61.2534822229534));
#146303=CARTESIAN_POINT('Ctrl Pts',(6.99871765569726,0.419019973666483,
61.2456416005615));
#146304=CARTESIAN_POINT('Ctrl Pts',(7.00710870499223,0.27886774097779,61.2392496147375));
#146305=CARTESIAN_POINT('Ctrl Pts',(7.01128541614006,0.138543129239347,
61.2328576289136));
#146306=CARTESIAN_POINT('Ctrl Pts',(7.0112497738309,-0.00178085825863861,
61.2264656430896));
#146307=CARTESIAN_POINT('Ctrl Pts',(7.01124977383073,-0.00178085893530164,
61.2264656430588));
#146308=CARTESIAN_POINT('Ctrl Pts',(7.01120349318839,-0.183987959526845,
61.2181658133235));
#146309=CARTESIAN_POINT('Ctrl Pts',(7.00405009571344,-0.366345146885556,
61.2098659835883));
#146310=CARTESIAN_POINT('Ctrl Pts',(6.98978022374334,-0.548269081990379,
61.201566153853));
#146311=CARTESIAN_POINT('Ctrl Pts',(6.97552151841008,-0.730050655725633,
61.1932728190033));
#146312=CARTESIAN_POINT('Ctrl Pts',(6.9541574639881,-0.911399316733849,
61.1849794841536));
#146313=CARTESIAN_POINT('Ctrl Pts',(6.92573074867032,-1.09173264099891,
61.1766861493038));
#146314=CARTESIAN_POINT('Ctrl Pts',(6.89732149485793,-1.27195519301059,
61.1683979087504));
#146315=CARTESIAN_POINT('Ctrl Pts',(6.86185828029754,-1.45116331791928,
61.1601096681969));
#146316=CARTESIAN_POINT('Ctrl Pts',(6.81943556082566,-1.62878027807512,
61.1518214276435));
#146317=CARTESIAN_POINT('Ctrl Pts',(6.77703176659377,-1.80631800135883,
61.143536884565));
#146318=CARTESIAN_POINT('Ctrl Pts',(6.72767473546444,-1.98226564625203,
61.1352523414865));
#146319=CARTESIAN_POINT('Ctrl Pts',(6.6715099690144,-2.15605688604023,61.126967798408));
#146320=CARTESIAN_POINT('Ctrl Pts',(6.61535405140371,-2.32982074476984,
61.1186845605711));
#146321=CARTESIAN_POINT('Ctrl Pts',(6.55239263567478,-2.50142855213749,
61.1104013227342));
#146322=CARTESIAN_POINT('Ctrl Pts',(6.48282118364402,-2.67032883057432,
61.1021180848974));
#146323=CARTESIAN_POINT('Ctrl Pts',(6.41325469007457,-2.83921707123599,
61.0938354374192));
#146324=CARTESIAN_POINT('Ctrl Pts',(6.33707922764114,-3.00539785430112,
61.0855527899411));
#146325=CARTESIAN_POINT('Ctrl Pts',(6.25453861104882,-3.16833920617719,
61.0772701424629));
#146326=CARTESIAN_POINT('Ctrl Pts',(6.17199128110482,-3.33129381071169,
61.0689868213246));
#146327=CARTESIAN_POINT('Ctrl Pts',(6.08307791799497,-3.49100815671002,
61.0607035001863));
#146328=CARTESIAN_POINT('Ctrl Pts',(5.98808868764945,-3.64697414733703,
61.052420179048));
#146329=CARTESIAN_POINT('Ctrl Pts',(5.89307723454667,-3.80297662625159,
61.0441349200243));
#146330=CARTESIAN_POINT('Ctrl Pts',(5.79198725699891,-3.95522871267261,
61.0358496610007));
#146331=CARTESIAN_POINT('Ctrl Pts',(5.68515286692431,-4.10325035090503,
61.0275644019771));
#146332=CARTESIAN_POINT('Ctrl Pts',(5.57822405302862,-4.2514028156314,61.0192718201633));
#146333=CARTESIAN_POINT('Ctrl Pts',(5.46554087860769,-4.39531708486661,
61.0109792383496));
#146334=CARTESIAN_POINT('Ctrl Pts',(5.34747918397504,-4.53454440263337,
61.0026866565358));
#146335=CARTESIAN_POINT('Ctrl Pts',(5.22936597961448,-4.67383246458374,
60.99439045671));
#146336=CARTESIAN_POINT('Ctrl Pts',(5.10586980112438,-4.80842924463886,
60.9860942568842));
#146337=CARTESIAN_POINT('Ctrl Pts',(4.9774044478282,-4.93792178200911,60.9777980570584));
#146338=CARTESIAN_POINT('Ctrl Pts',(4.84877759344969,-5.06757711179307,
60.9694914276093));
#146339=CARTESIAN_POINT('Ctrl Pts',(4.71516932244074,-5.19211513814238,
60.9611847981601));
#146340=CARTESIAN_POINT('Ctrl Pts',(4.57702879684953,-5.31116126240864,
60.9528781687109));
#146341=CARTESIAN_POINT('Ctrl Pts',(4.44081952894491,-5.42854307606393,
60.9446876691368));
#146342=CARTESIAN_POINT('Ctrl Pts',(4.30020418609226,-5.54058539599169,
60.9364971695627));
#146343=CARTESIAN_POINT('Ctrl Pts',(4.15564160387625,-5.6469699328607,60.9283066699885));
#146344=CARTESIAN_POINT('Ctrl Pts',(4.00771138083155,-5.7558327383412,60.9199253695837));
#146345=CARTESIAN_POINT('Ctrl Pts',(3.85532845952543,-5.85900610843106,
60.9115440691789));
#146346=CARTESIAN_POINT('Ctrl Pts',(3.69895524447717,-5.95611926188981,
60.903162768774));
#146347=CARTESIAN_POINT('Ctrl Pts',(3.54278020958773,-6.05310933864281,
60.8947920904405));
#146348=CARTESIAN_POINT('Ctrl Pts',(3.3826252353439,-6.14405433361975,60.8864214121071));
#146349=CARTESIAN_POINT('Ctrl Pts',(3.21898415823916,-6.22862485236551,
60.8780507337736));
#146350=CARTESIAN_POINT('Ctrl Pts',(3.0555287856611,-6.31309939809258,60.8696895547228));
#146351=CARTESIAN_POINT('Ctrl Pts',(2.8885954845283,-6.39121373610326,60.8613283756721));
#146352=CARTESIAN_POINT('Ctrl Pts',(2.71870570118038,-6.46268256011924,
60.8529671966213));
#146353=CARTESIAN_POINT('Ctrl Pts',(2.54903636986627,-6.53405864490571,
60.8446168671866));
#146354=CARTESIAN_POINT('Ctrl Pts',(2.37641850900181,-6.59880628940873,
60.836266537752));
#146355=CARTESIAN_POINT('Ctrl Pts',(2.20139663402076,-6.65668682019983,
60.8279162083173));
#146356=CARTESIAN_POINT('Ctrl Pts',(2.02650942790268,-6.7145228153849,60.8195723039616));
#146357=CARTESIAN_POINT('Ctrl Pts',(1.84922220363346,-6.76550212413633,
60.8112283996059));
#146358=CARTESIAN_POINT('Ctrl Pts',(1.67009892937172,-6.80943434718417,
60.8028844952502));
#146359=CARTESIAN_POINT('Ctrl Pts',(1.49111952804158,-6.85333128359632,
60.7945472927706));
#146360=CARTESIAN_POINT('Ctrl Pts',(1.31030733514935,-6.89019234507178,
60.786210090291));
#146361=CARTESIAN_POINT('Ctrl Pts',(1.12824108500719,-6.91987706658159,
60.7778728878113));
#146362=CARTESIAN_POINT('Ctrl Pts',(1.06830588043472,-6.92964911304807,
60.7751283267749));
#146363=CARTESIAN_POINT('Ctrl Pts',(1.00823488468427,-6.93864387184233,
60.7723837657386));
#146364=CARTESIAN_POINT('Ctrl Pts',(0.948049037360293,-6.94685753310518,
60.7696392047022));
#146365=CARTESIAN_POINT('Ctrl Pts',(0.765197111634181,-6.97181163520646,
60.7613008944002));
#146366=CARTESIAN_POINT('Ctrl Pts',(0.581434511015953,-6.98953177441674,
60.7529625840983));
#146367=CARTESIAN_POINT('Ctrl Pts',(0.397356357399926,-6.99998103481244,
60.7446242737963));
#146368=CARTESIAN_POINT('Ctrl Pts',(0.213162388055935,-7.01043686952822,
60.7362807173124));
#146369=CARTESIAN_POINT('Ctrl Pts',(0.0286527968346948,-7.01361268227103,
60.7279371608286));
#146370=CARTESIAN_POINT('Ctrl Pts',(-0.15557683528507,-7.00952369357738,
60.7195936043447));
#146371=CARTESIAN_POINT('Ctrl Pts',(-0.33994662850615,-7.00543159399895,
60.7112437001194));
#146372=CARTESIAN_POINT('Ctrl Pts',(-0.524035710577234,-6.99406367562674,
60.7028937958941));
#146373=CARTESIAN_POINT('Ctrl Pts',(-0.707252720357442,-6.97548709066593,
60.6945438916689));
#146374=CARTESIAN_POINT('Ctrl Pts',(-0.89074454209414,-6.95688264220235,
60.6861814632051));
#146375=CARTESIAN_POINT('Ctrl Pts',(-1.07336135139443,-6.93104795352176,
60.6778190347414));
#146376=CARTESIAN_POINT('Ctrl Pts',(-1.2545195889691,-6.89810170723749,
60.6694566062777));
#146377=CARTESIAN_POINT('Ctrl Pts',(-1.43583274153234,-6.86512728742143,
60.6610870267977));
#146378=CARTESIAN_POINT('Ctrl Pts',(-1.61568451468976,-6.82502924726269,
60.6527174473177));
#146379=CARTESIAN_POINT('Ctrl Pts',(-1.79350509203785,-6.77797654520391,
60.6443478678377));
#146380=CARTESIAN_POINT('Ctrl Pts',(-1.97159993596103,-6.73085127008505,
60.635965379301));
#146381=CARTESIAN_POINT('Ctrl Pts',(-2.1476570110733,-6.67674999394005,
60.6275828907644));
#146382=CARTESIAN_POINT('Ctrl Pts',(-2.3211237640995,-6.61589079672818,
60.6192004022278));
#146383=CARTESIAN_POINT('Ctrl Pts',(-2.37788492810306,-6.59597667016615,
60.6164575146238));
#146384=CARTESIAN_POINT('Ctrl Pts',(-2.43436892249107,-6.57533934513027,
60.6137146270197));
#146385=CARTESIAN_POINT('Ctrl Pts',(-2.49055693275975,-6.553987544021,60.6109717394157));
#146386=CARTESIAN_POINT('Ctrl Pts',(-2.6624229857697,-6.48867735126354,
60.6025818842829));
#146387=CARTESIAN_POINT('Ctrl Pts',(-2.83186510552412,-6.41654712207527,
60.5941920291502));
#146388=CARTESIAN_POINT('Ctrl Pts',(-2.99832485660896,-6.33779730006734,
60.5858021740174));
#146389=CARTESIAN_POINT('Ctrl Pts',(-3.16463100096917,-6.25912014729113,
60.5774200609253));
#146390=CARTESIAN_POINT('Ctrl Pts',(-3.32795996722733,-6.17383571881712,
60.5690379478332));
#146391=CARTESIAN_POINT('Ctrl Pts',(-3.48777249563173,-6.08219282670443,
60.5606558347412));
#146392=CARTESIAN_POINT('Ctrl Pts',(-3.64746104338542,-5.99062103005285,
60.5522802243923));
#146393=CARTESIAN_POINT('Ctrl Pts',(-3.80363830796317,-5.89270076724273,
60.5439046140434));
#146394=CARTESIAN_POINT('Ctrl Pts',(-3.95578847193313,-5.78872733230897,
60.5355290036946));
#146395=CARTESIAN_POINT('Ctrl Pts',(-4.10784293119036,-5.6848192982099,
60.527158661729));
#146396=CARTESIAN_POINT('Ctrl Pts',(-4.25587506991755,-5.57486586886242,
60.5187883197634));
#146397=CARTESIAN_POINT('Ctrl Pts',(-4.39939659076748,-5.45920655403727,
60.5104179777979));
#146398=CARTESIAN_POINT('Ctrl Pts',(-4.54284887309268,-5.343603036282,60.5020516739036));
#146399=CARTESIAN_POINT('Ctrl Pts',(-4.68179462141666,-5.22229932821359,
60.4936853700093));
#146400=CARTESIAN_POINT('Ctrl Pts',(-4.81577691361216,-5.09567652827573,
60.485319066115));
#146401=CARTESIAN_POINT('Ctrl Pts',(-4.94972173471596,-4.96908914118586,
60.4769551020414));
#146402=CARTESIAN_POINT('Ctrl Pts',(-5.07870562797895,-4.83718585297373,
60.4685911379677));
#146403=CARTESIAN_POINT('Ctrl Pts',(-5.20230657686822,-4.70038645674733,
60.4602271738941));
#146404=CARTESIAN_POINT('Ctrl Pts',(-5.32588850562545,-4.56360811167468,
60.4518644968956));
#146405=CARTESIAN_POINT('Ctrl Pts',(-5.4440889212943,-4.42193540456727,
60.4435018198971));
#146406=CARTESIAN_POINT('Ctrl Pts',(-5.55652406798683,-4.2758235282087,
60.4351391428986));
#146407=CARTESIAN_POINT('Ctrl Pts',(-5.66895689984519,-4.12971466002662,
60.4267766380723));
#146408=CARTESIAN_POINT('Ctrl Pts',(-5.77562449929959,-3.97916706553816,
60.418414133246));
#146409=CARTESIAN_POINT('Ctrl Pts',(-5.87618440035397,-3.82466775753616,
60.4100516284197));
#146410=CARTESIAN_POINT('Ctrl Pts',(-5.97675563498276,-3.67015103673457,
60.4016881810997));
#146411=CARTESIAN_POINT('Ctrl Pts',(-6.07121761998422,-3.51168199019138,
60.3933247337797));
#146412=CARTESIAN_POINT('Ctrl Pts',(-6.15927186734285,-3.34977560840408,
60.3849612864598));
#146413=CARTESIAN_POINT('Ctrl Pts',(-6.247377963517,-3.18777389158897,60.376592914507));
#146414=CARTESIAN_POINT('Ctrl Pts',(-6.3290686245528,-3.02233108365956,
60.3682245425542));
#146415=CARTESIAN_POINT('Ctrl Pts',(-6.40409141329752,-2.85398663848115,
60.3598561706014));
#146416=CARTESIAN_POINT('Ctrl Pts',(-6.47913668083047,-2.68559175290729,
60.3514852912657));
#146417=CARTESIAN_POINT('Ctrl Pts',(-6.5475099633949,-2.51429379891878,
60.3431144119299));
#146418=CARTESIAN_POINT('Ctrl Pts',(-6.6090071798928,-2.34065175936649,
60.3347435325942));
#146419=CARTESIAN_POINT('Ctrl Pts',(-6.67055650231725,-2.16686259479172,
60.3263655607029));
#146420=CARTESIAN_POINT('Ctrl Pts',(-6.72521801252132,-1.9907256878751,
60.3179875888116));
#146421=CARTESIAN_POINT('Ctrl Pts',(-6.77283731893193,-1.81281582456216,
60.3096096169203));
#146422=CARTESIAN_POINT('Ctrl Pts',(-6.80309977592204,-1.69975265769871,
60.3042853475612));
#146423=CARTESIAN_POINT('Ctrl Pts',(-6.83051910817107,-1.58597371990945,
60.2989610782021));
#146424=CARTESIAN_POINT('Ctrl Pts',(-6.85506642330611,-1.47162865375785,
60.293636808843));
#146425=CARTESIAN_POINT('Ctrl Pts',(-6.89131766869568,-1.30276492958497,
60.2857739776537));
#146426=CARTESIAN_POINT('Ctrl Pts',(-6.92137795629609,-1.13231489320908,
60.2779111464644));
#146427=CARTESIAN_POINT('Ctrl Pts',(-6.94510661887924,-0.960791660507012,
60.2700483152751));
#146428=CARTESIAN_POINT('Ctrl Pts',(-6.96881704911733,-0.789400220768501,
60.2621915256337));
#146429=CARTESIAN_POINT('Ctrl Pts',(-6.9862054772162,-0.616937599792321,
60.2543347359923));
#146430=CARTESIAN_POINT('Ctrl Pts',(-6.99718182459544,-0.443929134041922,
60.2464779463509));
#146431=CARTESIAN_POINT('Ctrl Pts',(-7.00815198183436,-0.27101823687632,
60.2386255875669));
#146432=CARTESIAN_POINT('Ctrl Pts',(-7.01271722755956,-0.0975624866027649,
60.2307732287829));
#146433=CARTESIAN_POINT('Ctrl Pts',(-7.01083909849225,0.0759058466283117,
60.2229208699989));
#146434=CARTESIAN_POINT('Ctrl Pts',(-7.00896141287313,0.249333221961846,
60.2150703652485));
#146435=CARTESIAN_POINT('Ctrl Pts',(-7.00064337606927,0.422772793345405,
60.207219860498));
#146436=CARTESIAN_POINT('Ctrl Pts',(-6.98589860770976,0.595690528125873,
60.1993693557476));
#146437=CARTESIAN_POINT('Ctrl Pts',(-6.97115621131877,0.768580445892675,
60.1915201138959));
#146438=CARTESIAN_POINT('Ctrl Pts',(-6.94998917689306,0.940948314276102,
60.1836708720442));
#146439=CARTESIAN_POINT('Ctrl Pts',(-6.9224631093025,1.11226393578411,60.1758216301926));
#146440=CARTESIAN_POINT('Ctrl Pts',(-6.89492776764099,1.28363727687826,
60.1679697437777));
#146441=CARTESIAN_POINT('Ctrl Pts',(-6.86102917391458,1.45395728593272,
60.1601178573628));
#146442=CARTESIAN_POINT('Ctrl Pts',(-6.82088434045903,1.62270249170353,
60.1522659709479));
#146443=CARTESIAN_POINT('Ctrl Pts',(-6.79140648892611,1.74660999596832,
60.1465004284841));
#146444=CARTESIAN_POINT('Ctrl Pts',(-6.75856187735721,1.8696685699544,60.1407348860203));
#146445=CARTESIAN_POINT('Ctrl Pts',(-6.72241403827011,1.99167669579403,
60.1349693435565));
#146446=CARTESIAN_POINT('Ctrl Pts',(-6.66187881707922,2.19599842210773,
60.1253140391967));
#146447=CARTESIAN_POINT('Ctrl Pts',(-6.5921100323113,2.39726976123393,60.115658734837));
#146448=CARTESIAN_POINT('Ctrl Pts',(-6.513437275972,2.59475652315945,60.1060034304772));
#146449=CARTESIAN_POINT('Ctrl Pts',(-6.43432868732159,2.79333732469751,
60.0962946375426));
#146450=CARTESIAN_POINT('Ctrl Pts',(-6.34621726946916,2.98809147761485,
60.0865858446081));
#146451=CARTESIAN_POINT('Ctrl Pts',(-6.24948186149068,3.17830190910162,
60.0768770516735));
#146452=CARTESIAN_POINT('Ctrl Pts',(-6.15228095451501,3.36942764933584,
60.0671215392029));
#146453=CARTESIAN_POINT('Ctrl Pts',(-6.04637289996954,3.5559658056905,60.0573660267324));
#146454=CARTESIAN_POINT('Ctrl Pts',(-5.93218523847481,3.73721886687434,
60.0476105142618));
#146455=CARTESIAN_POINT('Ctrl Pts',(-5.81788451362779,3.91865139647398,
60.037845342333));
#146456=CARTESIAN_POINT('Ctrl Pts',(-5.6952878136832,4.09478833711091,60.0280801704043));
#146457=CARTESIAN_POINT('Ctrl Pts',(-5.56486651922017,4.26496039674021,
60.0183149984755));
#146458=CARTESIAN_POINT('Ctrl Pts',(-5.43462305123304,4.4349004306272,60.0085631411371));
#146459=CARTESIAN_POINT('Ctrl Pts',(-5.29657633465462,4.59889180831757,
59.9988112837987));
#146460=CARTESIAN_POINT('Ctrl Pts',(-5.15123779084723,4.75629853821723,
59.9890594264603));
#146461=CARTESIAN_POINT('Ctrl Pts',(-5.08785965981767,4.82493927240359,
59.9848069103969));
#146462=CARTESIAN_POINT('Ctrl Pts',(-5.0230954581525,4.89232827086292,59.9805543943335));
#146463=CARTESIAN_POINT('Ctrl Pts',(-4.95699008884031,4.95841464801392,
59.9763018782701));
#146464=CARTESIAN_POINT('Ctrl Pts',(-4.8321163815815,5.08325247888928,59.9682688326712));
#146465=CARTESIAN_POINT('Ctrl Pts',(-4.70239330495944,5.20350034449769,
59.9602357870723));
#146466=CARTESIAN_POINT('Ctrl Pts',(-4.56819969400882,5.31875719676672,
59.9522027414734));
#146467=CARTESIAN_POINT('Ctrl Pts',(-4.4340923478782,5.43393995749335,59.9441748598256));
#146468=CARTESIAN_POINT('Ctrl Pts',(-4.29552046477135,5.5441378534666,59.9361469781777));
#146469=CARTESIAN_POINT('Ctrl Pts',(-4.15289952347646,5.64898682158217,
59.9281190965298));
#146470=CARTESIAN_POINT('Ctrl Pts',(-4.01034297694249,5.75378844935505,
59.9200948395496));
#146471=CARTESIAN_POINT('Ctrl Pts',(-3.86374130708915,5.85324574132342,
59.9120705825695));
#146472=CARTESIAN_POINT('Ctrl Pts',(-3.71354280164434,5.94703509514241,
59.9040463255893));
#146473=CARTESIAN_POINT('Ctrl Pts',(-3.56336245672864,6.04081310887327,
59.8960230388235));
#146474=CARTESIAN_POINT('Ctrl Pts',(-3.40958644912039,6.12892434889666,
59.8879997520578));
#146475=CARTESIAN_POINT('Ctrl Pts',(-3.25269190640852,6.21108862635887,
59.879976465292));
#146476=CARTESIAN_POINT('Ctrl Pts',(-3.09581021980487,6.29324617119148,
59.871953835963));
#146477=CARTESIAN_POINT('Ctrl Pts',(-2.93581083376654,6.36945755758264,
59.863931206634));
#146478=CARTESIAN_POINT('Ctrl Pts',(-2.77319504625346,6.439488783897,59.855908577305));
#146479=CARTESIAN_POINT('Ctrl Pts',(-2.61051812678136,6.50954633696673,
59.8478829320385));
#146480=CARTESIAN_POINT('Ctrl Pts',(-2.44522317905844,6.57341894644921,
59.8398572867721));
#146481=CARTESIAN_POINT('Ctrl Pts',(-2.27783138019637,6.63092080829599,
59.8318316415056));
#146482=CARTESIAN_POINT('Ctrl Pts',(-2.17912697524418,6.66482741002804,
59.8270992319982));
#146483=CARTESIAN_POINT('Ctrl Pts',(-2.07969383546348,6.69651983059121,
59.8223668224909));
#146484=CARTESIAN_POINT('Ctrl Pts',(-1.97964121801694,6.72596812439878,
59.8176344129836));
#146485=CARTESIAN_POINT('Ctrl Pts',(-1.79507049670079,6.78029246861194,
59.8089043641491));
#146486=CARTESIAN_POINT('Ctrl Pts',(-1.60829873307994,6.82700461812528,
59.8001743153145));
#146487=CARTESIAN_POINT('Ctrl Pts',(-1.41995570843133,6.86595604039185,
59.79144426648));
#146488=CARTESIAN_POINT('Ctrl Pts',(-1.23155822416242,6.90491872551071,
59.7827116933409));
#146489=CARTESIAN_POINT('Ctrl Pts',(-1.04158884025968,6.93611614870944,
59.7739791202019));
#146490=CARTESIAN_POINT('Ctrl Pts',(-0.850687128395915,6.95945098208771,
59.7652465470628));
#146491=CARTESIAN_POINT('Ctrl Pts',(-0.657073352975061,6.98311732402396,
59.7563899137824));
#146492=CARTESIAN_POINT('Ctrl Pts',(-0.462500844984582,6.99869593704891,
59.7475332805019));
#146493=CARTESIAN_POINT('Ctrl Pts',(-0.267642234641472,7.00613975001471,
59.7386766472214));
#146494=CARTESIAN_POINT('Ctrl Pts',(-0.0753908197555502,7.01348396525006,
59.7299385151148));
#146495=CARTESIAN_POINT('Ctrl Pts',(0.117138810529907,7.01290972725822,
59.7212003830082));
#146496=CARTESIAN_POINT('Ctrl Pts',(0.309299626698119,7.00442433776141,
59.7124622509015));
#146497=CARTESIAN_POINT('Ctrl Pts',(0.505369393085973,6.99576633781364,
59.7035463670341));
#146498=CARTESIAN_POINT('Ctrl Pts',(0.701054883652899,6.97887188955907,
59.6946304831668));
#146499=CARTESIAN_POINT('Ctrl Pts',(0.895672117836021,6.9538045715875,59.6857145992994));
#146500=CARTESIAN_POINT('Ctrl Pts',(1.09028935201921,6.92873725361591,59.676798715432));
#146501=CARTESIAN_POINT('Ctrl Pts',(1.28383803066124,6.89549711059299,59.6678828315646));
#146502=CARTESIAN_POINT('Ctrl Pts',(1.4756420337927,6.85420361169729,59.6589669476973));
#146503=CARTESIAN_POINT('Ctrl Pts',(1.66367703979367,6.81372154048978,59.6502262632009));
#146504=CARTESIAN_POINT('Ctrl Pts',(1.850055271653,6.76549537689206,59.6414855787046));
#146505=CARTESIAN_POINT('Ctrl Pts',(2.03414967566964,6.70968416987514,59.6327448942083));
#146506=CARTESIAN_POINT('Ctrl Pts',(2.21821095804526,6.65388300422137,59.6240057823063));
#146507=CARTESIAN_POINT('Ctrl Pts',(2.39998897124958,6.59049959991576,59.6152666704043));
#146508=CARTESIAN_POINT('Ctrl Pts',(2.57887153829044,6.51974295133601,59.6065275585022));
#146509=CARTESIAN_POINT('Ctrl Pts',(2.76007178644062,6.44806954853875,59.5976752188279));
#146510=CARTESIAN_POINT('Ctrl Pts',(2.93830076275092,6.36883059152284,59.5888228791536));
#146511=CARTESIAN_POINT('Ctrl Pts',(3.11294149548016,6.28229431085633,59.5799705394793));
#146512=CARTESIAN_POINT('Ctrl Pts',(3.28526008042121,6.19690867832102,59.5712359068295));
#146513=CARTESIAN_POINT('Ctrl Pts',(3.45408500730464,6.10441871501682,59.5625012741796));
#146514=CARTESIAN_POINT('Ctrl Pts',(3.61884597440103,6.00512950535303,59.5537666415298));
#146515=CARTESIAN_POINT('Ctrl Pts',(3.78693739464137,5.90383327869782,59.5448554483432));
#146516=CARTESIAN_POINT('Ctrl Pts',(3.95079854883831,5.79546013155386,59.5359442551567));
#146517=CARTESIAN_POINT('Ctrl Pts',(4.10985167052522,5.68038254070807,59.5270330619702));
#146518=CARTESIAN_POINT('Ctrl Pts',(4.26890479221214,5.56530494986227,59.5181218687837));
#146519=CARTESIAN_POINT('Ctrl Pts',(4.42314962790079,5.44352308208674,59.5092106755972));
#146520=CARTESIAN_POINT('Ctrl Pts',(4.57204038025183,5.3154560786302,59.5002994824107));
#146521=CARTESIAN_POINT('Ctrl Pts',(4.70613547312816,5.20011542481706,59.4922738175583));
#146522=CARTESIAN_POINT('Ctrl Pts',(4.83594899628315,5.07962330972136,59.484248152706));
#146523=CARTESIAN_POINT('Ctrl Pts',(4.96106213967889,4.95434042116049,59.4762224878536));
#146524=CARTESIAN_POINT('Ctrl Pts',(5.08613557523176,4.82909729431546,59.4681993701504));
#146525=CARTESIAN_POINT('Ctrl Pts',(5.206511342309,4.69906668019786,59.4601762524472));
#146526=CARTESIAN_POINT('Ctrl Pts',(5.32180619378596,4.56464734654074,59.452153134744));
#146527=CARTESIAN_POINT('Ctrl Pts',(5.43708650557331,4.43024496433778,59.4441310288262));
#146528=CARTESIAN_POINT('Ctrl Pts',(5.5472869399191,4.29145524356305,59.4361089229083));
#146529=CARTESIAN_POINT('Ctrl Pts',(5.65206342293754,4.14871132107207,59.4280868169905));
#146530=CARTESIAN_POINT('Ctrl Pts',(5.75687884125086,4.0059143544575,59.420061730031));
#146531=CARTESIAN_POINT('Ctrl Pts',(5.85626606225826,3.85916054474957,59.4120366430715));
#146532=CARTESIAN_POINT('Ctrl Pts',(5.94992312727897,3.7089137684733,59.404011556112));
#146533=CARTESIAN_POINT('Ctrl Pts',(6.04359863759,3.55863740184624,59.3959848886518));
#146534=CARTESIAN_POINT('Ctrl Pts',(6.13154155727149,3.40486701393061,59.3879582211916));
#146535=CARTESIAN_POINT('Ctrl Pts',(6.21349519490292,3.24809236713157,59.3799315537313));
#146536=CARTESIAN_POINT('Ctrl Pts',(6.2955146246258,3.09119186219863,59.3718984424908));
#146537=CARTESIAN_POINT('Ctrl Pts',(6.37153500761923,2.93128261050024,59.3638653312502));
#146538=CARTESIAN_POINT('Ctrl Pts',(6.44134697279782,2.76887625915793,59.3558322200097));
#146539=CARTESIAN_POINT('Ctrl Pts',(6.48248271874028,2.67318053721156,59.3510988190479));
#146540=CARTESIAN_POINT('Ctrl Pts',(6.521463823452,2.57661819015167,59.3463654180861));
#146541=CARTESIAN_POINT('Ctrl Pts',(6.55825550999446,2.47929651879869,59.3416320171243));
#146542=CARTESIAN_POINT('Ctrl Pts',(6.56256998608823,2.46788383120762,59.3410769421275));
#146543=CARTESIAN_POINT('Ctrl Pts',(6.56685448137081,2.45646038464508,59.3405218671306));
#146544=CARTESIAN_POINT('Ctrl Pts',(6.57110895151816,2.4450263208763,59.3399667921338));
#146545=CARTESIAN_POINT('Origin',(0.,0.,50.));
#146546=CARTESIAN_POINT('',(6.57110895151816,2.4450263208763,57.3398522865015));
#146547=CARTESIAN_POINT('',(6.57110895151813,2.44502632087639,57.8870048219557));
#146548=CARTESIAN_POINT('',(6.57110895151814,2.44502632087636,50.));
#146549=CARTESIAN_POINT('',(7.01124999602994,-0.000235945344234768,59.7735343568684));
#146550=CARTESIAN_POINT('Ctrl Pts',(6.57110895151813,2.44502632087639,57.8870048219557));
#146551=CARTESIAN_POINT('Ctrl Pts',(6.52450546921719,2.57027509922486,57.8930453782421));
#146552=CARTESIAN_POINT('Ctrl Pts',(6.47430760150655,2.69422367287727,57.8990859345286));
#146553=CARTESIAN_POINT('Ctrl Pts',(6.42059905730801,2.816653032909,57.905126490815));
#146554=CARTESIAN_POINT('Ctrl Pts',(6.34646043726219,2.98565302986097,57.9134648011168));
#146555=CARTESIAN_POINT('Ctrl Pts',(6.26567581471899,3.15165466081322,57.9218031114186));
#146556=CARTESIAN_POINT('Ctrl Pts',(6.17852427623118,3.31413100684357,57.9301414217204));
#146557=CARTESIAN_POINT('Ctrl Pts',(6.09131790495256,3.47670957747773,57.9384849782041));
#146558=CARTESIAN_POINT('Ctrl Pts',(5.99773678244466,3.63575815039843,57.9468285346878));
#146559=CARTESIAN_POINT('Ctrl Pts',(5.8981047085228,3.79077662356954,57.9551720911715));
#146560=CARTESIAN_POINT('Ctrl Pts',(5.79839683495317,3.94591303411963,57.9635219953967));
#146561=CARTESIAN_POINT('Ctrl Pts',(5.69262900436559,4.09701295376717,57.9718718996218));
#146562=CARTESIAN_POINT('Ctrl Pts',(5.58116711335293,4.24360698172295,57.9802218038469));
#146563=CARTESIAN_POINT('Ctrl Pts',(5.46953803775208,4.3904208898725,57.9885842323105));
#146564=CARTESIAN_POINT('Ctrl Pts',(5.35219803326782,4.5327151396672,57.9969466607741));
#146565=CARTESIAN_POINT('Ctrl Pts',(5.22955288163711,4.6700538777043,58.0053090892377));
#146566=CARTESIAN_POINT('Ctrl Pts',(5.10680285168271,4.80751005908451,58.0136786687175));
#146567=CARTESIAN_POINT('Ctrl Pts',(4.97873885001579,4.9400020384957,58.0220482481974));
#146568=CARTESIAN_POINT('Ctrl Pts',(4.84580237287856,5.06713192304133,58.0304178276773));
#146569=CARTESIAN_POINT('Ctrl Pts',(4.71266085742252,5.19445788994418,58.0388003162137));
#146570=CARTESIAN_POINT('Ctrl Pts',(4.57463209395561,5.31640501878296,58.0471828047502));
#146571=CARTESIAN_POINT('Ctrl Pts',(4.43219047145647,5.43261577761859,58.0555652932867));
#146572=CARTESIAN_POINT('Ctrl Pts',(4.38558123852113,5.47064184214335,58.0583081808916));
#146573=CARTESIAN_POINT('Ctrl Pts',(4.33849974627091,5.50805405801524,58.0610510684965));
#146574=CARTESIAN_POINT('Ctrl Pts',(4.29096325386765,5.54484092796697,58.0637939561013));
#146575=CARTESIAN_POINT('Ctrl Pts',(4.14556018154534,5.65736340578731,58.0721838112342));
#146576=CARTESIAN_POINT('Ctrl Pts',(3.99560443078813,5.76425903116473,58.080573666367));
#146577=CARTESIAN_POINT('Ctrl Pts',(3.84155841605354,5.86515605065613,58.0889635214998));
#146578=CARTESIAN_POINT('Ctrl Pts',(3.68765455282126,5.96595996379276,58.097345634592));
#146579=CARTESIAN_POINT('Ctrl Pts',(3.52966822361311,6.06077612667109,58.1057277476842));
#146580=CARTESIAN_POINT('Ctrl Pts',(3.36809309514126,6.14927438523943,58.1141098607763));
#146581=CARTESIAN_POINT('Ctrl Pts',(3.20664331472488,6.23770398791544,58.1224854711252));
#146582=CARTESIAN_POINT('Ctrl Pts',(3.0416105730649,6.31982530074116,58.1308610814741));
#146583=CARTESIAN_POINT('Ctrl Pts',(2.87351595327708,6.39535242412505,58.139236691823));
#146584=CARTESIAN_POINT('Ctrl Pts',(2.70552706750145,6.47083203982669,58.1476070337886));
#146585=CARTESIAN_POINT('Ctrl Pts',(2.53448044288038,6.53972560213424,58.1559773757542));
#146586=CARTESIAN_POINT('Ctrl Pts',(2.36092051770871,6.60179376166524,58.1643477177198));
#146587=CARTESIAN_POINT('Ctrl Pts',(2.1874443223696,6.66383197789798,58.1727140216142));
#146588=CARTESIAN_POINT('Ctrl Pts',(2.01145755333925,6.71905124714059,58.1810803255087));
#146589=CARTESIAN_POINT('Ctrl Pts',(1.83352375125979,6.76726068775736,58.1894466294031));
#146590=CARTESIAN_POINT('Ctrl Pts',(1.65563971227895,6.81545664554445,58.1978105934767));
#146591=CARTESIAN_POINT('Ctrl Pts',(1.47581004259518,6.85664659655504,58.2061745575504));
#146592=CARTESIAN_POINT('Ctrl Pts',(1.29461307413814,6.89068962809751,58.214538521624));
#146593=CARTESIAN_POINT('Ctrl Pts',(1.11344398888363,6.92472742098311,58.2229011986226));
#146594=CARTESIAN_POINT('Ctrl Pts',(0.930908347273212,6.95162042649785,
58.2312638756212));
#146595=CARTESIAN_POINT('Ctrl Pts',(0.747594710914991,6.97127884327631,
58.2396265526197));
#146596=CARTESIAN_POINT('Ctrl Pts',(0.564284848649643,6.99093685532389,
58.247989057446));
#146597=CARTESIAN_POINT('Ctrl Pts',(0.380197350393221,7.00336054099226,
58.2563515622724));
#146598=CARTESIAN_POINT('Ctrl Pts',(0.195926373013485,7.0085119261408,58.2647140670987));
#146599=CARTESIAN_POINT('Ctrl Pts',(0.0116346274260749,7.01366389187472,
58.2730775144187));
#146600=CARTESIAN_POINT('Ctrl Pts',(-0.172840309989962,7.01154191434983,
58.2814409617387));
#146601=CARTESIAN_POINT('Ctrl Pts',(-0.356903367522352,7.00216013446931,
58.2898044090588));
#146602=CARTESIAN_POINT('Ctrl Pts',(-0.541074806555653,6.99277283033314,
58.2981727810116));
#146603=CARTESIAN_POINT('Ctrl Pts',(-0.724833552456556,6.97611719760979,
58.3065411529645));
#146604=CARTESIAN_POINT('Ctrl Pts',(-0.907587698260507,6.95225942643586,
58.3149095249173));
#146605=CARTESIAN_POINT('Ctrl Pts',(-1.09039660198301,6.92839450685012,
58.3232804042531));
#146606=CARTESIAN_POINT('Ctrl Pts',(-1.27219998014171,6.89732319371543,
58.3316512835889));
#146607=CARTESIAN_POINT('Ctrl Pts',(-1.45241450268126,6.85916311767705,
58.3400221629247));
#146608=CARTESIAN_POINT('Ctrl Pts',(-1.6327817190366,6.82097070901897,58.348400134816));
#146609=CARTESIAN_POINT('Ctrl Pts',(-1.81155706911948,6.77567760933404,
58.3567781067074));
#146610=CARTESIAN_POINT('Ctrl Pts',(-1.98816967395938,6.72345208282533,
58.3651560785987));
#146611=CARTESIAN_POINT('Ctrl Pts',(-2.10040842248689,6.69026233545797,
58.3704803479572));
#146612=CARTESIAN_POINT('Ctrl Pts',(-2.21177399738411,6.65427379297141,
58.3758046173158));
#146613=CARTESIAN_POINT('Ctrl Pts',(-2.32212367178652,6.61553990354746,
58.3811288866743));
#146614=CARTESIAN_POINT('Ctrl Pts',(-2.48508703881145,6.55833805793548,
58.3889917178636));
#146615=CARTESIAN_POINT('Ctrl Pts',(-2.64617268895316,6.49502732338538,
58.3968545490528));
#146616=CARTESIAN_POINT('Ctrl Pts',(-2.80486951165799,6.42575548749495,
58.4047173802421));
#146617=CARTESIAN_POINT('Ctrl Pts',(-2.96344439680265,6.35653687786648,
58.4125741698835));
#146618=CARTESIAN_POINT('Ctrl Pts',(-3.11963375748957,6.28136642706461,
58.4204309595249));
#146619=CARTESIAN_POINT('Ctrl Pts',(-3.27294245944308,6.20044145361237,
58.4282877491663));
#146620=CARTESIAN_POINT('Ctrl Pts',(-3.4261647025459,6.11956211801439,58.4361401079502));
#146621=CARTESIAN_POINT('Ctrl Pts',(-3.5765091823989,6.03293489279628,58.4439924667342));
#146622=CARTESIAN_POINT('Ctrl Pts',(-3.72350178664023,5.94080474408872,
58.4518448255181));
#146623=CARTESIAN_POINT('Ctrl Pts',(-3.87045968421232,5.84869634838441,
58.4596953302685));
#146624=CARTESIAN_POINT('Ctrl Pts',(-4.01406695406378,5.75108781031801,
58.467545835019));
#146625=CARTESIAN_POINT('Ctrl Pts',(-4.1538751609237,5.64826944381738,58.4753963397694));
#146626=CARTESIAN_POINT('Ctrl Pts',(-4.29366087704949,5.54546761755139,
58.483245581621));
#146627=CARTESIAN_POINT('Ctrl Pts',(-4.42964844122439,5.43745785971971,
58.4910948234726));
#146628=CARTESIAN_POINT('Ctrl Pts',(-4.56141981924342,5.32457282747765,
58.4989440653242));
#146629=CARTESIAN_POINT('Ctrl Pts',(-4.69323559361908,5.21164976205854,
58.5067959517391));
#146630=CARTESIAN_POINT('Ctrl Pts',(-4.82083205444636,5.09384838971931,
58.5146478381539));
#146631=CARTESIAN_POINT('Ctrl Pts',(-4.94382543927954,4.97154066547106,
58.5224997245688));
#146632=CARTESIAN_POINT('Ctrl Pts',(-5.03413795089466,4.88173162588922,
58.5282652670327));
#146633=CARTESIAN_POINT('Ctrl Pts',(-5.12196929038337,4.78949368930705,
58.5340308094967));
#146634=CARTESIAN_POINT('Ctrl Pts',(-5.20718071382556,4.6949862168129,58.5397963519606));
#146635=CARTESIAN_POINT('Ctrl Pts',(-5.34988059565328,4.53671864408659,
58.5494516563206));
#146636=CARTESIAN_POINT('Ctrl Pts',(-5.48515969510916,4.37216652306128,
58.5591069606805));
#146637=CARTESIAN_POINT('Ctrl Pts',(-5.61256373454069,4.20199415613809,
58.5687622650405));
#146638=CARTESIAN_POINT('Ctrl Pts',(-5.7406735684508,4.03087906622498,58.5784710579754));
#146639=CARTESIAN_POINT('Ctrl Pts',(-5.86082086347158,3.8540813582749,58.5881798509102));
#146640=CARTESIAN_POINT('Ctrl Pts',(-5.97259164395314,3.67229841067977,
58.5978886438451));
#146641=CARTESIAN_POINT('Ctrl Pts',(-6.0849002749202,3.48964070810666,58.6076441563158));
#146642=CARTESIAN_POINT('Ctrl Pts',(-6.18875157816082,3.30194972107997,
58.6173996687866));
#146643=CARTESIAN_POINT('Ctrl Pts',(-6.28377368039477,3.10995416301881,
58.6271551812574));
#146644=CARTESIAN_POINT('Ctrl Pts',(-6.37888986912822,2.91776849981838,
58.6369203531863));
#146645=CARTESIAN_POINT('Ctrl Pts',(-6.46515936333439,2.72126977955496,
58.6466855251152));
#146646=CARTESIAN_POINT('Ctrl Pts',(-6.54225724023705,2.5212093854073,58.6564506970442));
#146647=CARTESIAN_POINT('Ctrl Pts',(-6.61924999593386,2.32142176906782,
58.6662025543827));
#146648=CARTESIAN_POINT('Ctrl Pts',(-6.68709611430525,2.11808222018858,
58.6759544117213));
#146649=CARTESIAN_POINT('Ctrl Pts',(-6.74551997479243,1.91195889918595,
58.6857062690598));
#146650=CARTESIAN_POINT('Ctrl Pts',(-6.7709970092206,1.82207420307306,58.6899587851223));
#146651=CARTESIAN_POINT('Ctrl Pts',(-6.79468293256122,1.7316603990258,58.6942113011848));
#146652=CARTESIAN_POINT('Ctrl Pts',(-6.81655777172355,1.64078234609448,
58.6984638172473));
#146653=CARTESIAN_POINT('Ctrl Pts',(-6.85787956284092,1.46911279037727,
58.706496862846));
#146654=CARTESIAN_POINT('Ctrl Pts',(-6.89275525666476,1.2957019724591,58.7145299084448));
#146655=CARTESIAN_POINT('Ctrl Pts',(-6.9210404522921,1.12108234320073,58.7225629540435));
#146656=CARTESIAN_POINT('Ctrl Pts',(-6.94930746510654,0.946574966163909,
58.7305908356913));
#146657=CARTESIAN_POINT('Ctrl Pts',(-6.97099235446236,0.77086068490809,
58.738618717339));
#146658=CARTESIAN_POINT('Ctrl Pts',(-6.98600139184709,0.59448390693991,
58.7466465989868));
#146659=CARTESIAN_POINT('Ctrl Pts',(-7.0010036525035,0.418186764825464,
58.7546708559668));
#146660=CARTESIAN_POINT('Ctrl Pts',(-7.00933603181592,0.241228086079722,
58.7626951129468));
#146661=CARTESIAN_POINT('Ctrl Pts',(-7.01095643732032,0.0641591497509032,
58.7707193699269));
#146662=CARTESIAN_POINT('Ctrl Pts',(-7.01257664690119,-0.112888377140101,
58.7787426566925));
#146663=CARTESIAN_POINT('Ctrl Pts',(-7.00748648807325,-0.290045768790848,
58.7867659434582));
#146664=CARTESIAN_POINT('Ctrl Pts',(-6.9956959518272,-0.466759801277448,
58.7947892302238));
#146665=CARTESIAN_POINT('Ctrl Pts',(-6.98390638171043,-0.643459353625247,
58.8028118595527));
#146666=CARTESIAN_POINT('Ctrl Pts',(-6.96541755622063,-0.819715253609423,
58.8108344888815));
#146667=CARTESIAN_POINT('Ctrl Pts',(-6.94029147899009,-0.994977763147284,
58.8188571182104));
#146668=CARTESIAN_POINT('Ctrl Pts',(-6.91515595614323,-1.17030615891187,
58.8268827634767));
#146669=CARTESIAN_POINT('Ctrl Pts',(-6.88337825213684,-1.3446400555356,
58.8349084087431));
#146670=CARTESIAN_POINT('Ctrl Pts',(-6.84507185867646,-1.51743791044498,
58.8429340540095));
#146671=CARTESIAN_POINT('Ctrl Pts',(-6.82248407481442,-1.6193300554874,
58.8476664635175));
#146672=CARTESIAN_POINT('Ctrl Pts',(-6.79762723465024,-1.72068831271401,
58.8523988730255));
#146673=CARTESIAN_POINT('Ctrl Pts',(-6.77053281198699,-1.82140385535652,
58.8571312825335));
#146674=CARTESIAN_POINT('Ctrl Pts',(-6.72055073993723,-2.00719749899507,
58.8658613313682));
#146675=CARTESIAN_POINT('Ctrl Pts',(-6.66292661929621,-2.19089610356262,
58.874591380203));
#146676=CARTESIAN_POINT('Ctrl Pts',(-6.5978624126179,-2.37188493537608,
58.8833214290377));
#146677=CARTESIAN_POINT('Ctrl Pts',(-6.53277939254295,-2.55292610033632,
58.8920540021769));
#146678=CARTESIAN_POINT('Ctrl Pts',(-6.46025208497314,-2.73125567077547,
58.9007865753162));
#146679=CARTESIAN_POINT('Ctrl Pts',(-6.38053124060429,-2.90627728377262,
58.9095191484554));
#146680=CARTESIAN_POINT('Ctrl Pts',(-6.29967783438381,-3.08378535816713,
58.9183757817358));
#146681=CARTESIAN_POINT('Ctrl Pts',(-6.21142506240127,-3.2578905053806,
58.9272324150162));
#146682=CARTESIAN_POINT('Ctrl Pts',(-6.11608379788457,-3.42799439027456,
58.9360890482966));
#146683=CARTESIAN_POINT('Ctrl Pts',(-6.0220181932462,-3.59582229632339,
58.9448271804034));
#146684=CARTESIAN_POINT('Ctrl Pts',(-5.92105276120039,-3.75975511738309,
58.9535653125102));
#146685=CARTESIAN_POINT('Ctrl Pts',(-5.81353139610945,-3.91924473195406,
58.9623034446171));
#146686=CARTESIAN_POINT('Ctrl Pts',(-5.70382282307937,-4.08197869662147,
58.9712193284842));
#146687=CARTESIAN_POINT('Ctrl Pts',(-5.58728889986215,-4.24008650268444,
58.9801352123514));
#146688=CARTESIAN_POINT('Ctrl Pts',(-5.46434081004124,-4.3930178777485,
58.9890510962186));
#146689=CARTESIAN_POINT('Ctrl Pts',(-5.34139272022036,-4.5459492528125,
58.9979669800857));
#146690=CARTESIAN_POINT('Ctrl Pts',(-5.2120306580182,-4.69370396499874,
59.0068828639529));
#146691=CARTESIAN_POINT('Ctrl Pts',(-5.07670938084766,-4.83576761485841,
59.01579874782));
#146692=CARTESIAN_POINT('Ctrl Pts',(-4.94404720096971,-4.97503967809833,
59.0245394323161));
#146693=CARTESIAN_POINT('Ctrl Pts',(-4.80564374230496,-5.10885705661865,
59.0332801168122));
#146694=CARTESIAN_POINT('Ctrl Pts',(-4.66196191854767,-5.23676786123954,
59.0420208013083));
#146695=CARTESIAN_POINT('Ctrl Pts',(-4.51830594553702,-5.36465565258208,
59.0507599132101));
#146696=CARTESIAN_POINT('Ctrl Pts',(-4.36937370841492,-5.48663881031182,
59.0594990251118));
#146697=CARTESIAN_POINT('Ctrl Pts',(-4.21566296181306,-5.60230420049621,
59.0682381370136));
#146698=CARTESIAN_POINT('Ctrl Pts',(-4.05996067125789,-5.71946820228404,
59.077090476688));
#146699=CARTESIAN_POINT('Ctrl Pts',(-3.89935539732758,-5.83014939441803,
59.0859428163624));
#146700=CARTESIAN_POINT('Ctrl Pts',(-3.7343979268174,-5.93396146656531,
59.0947951560368));
#146701=CARTESIAN_POINT('Ctrl Pts',(-3.57163384853754,-6.0363931793281,
59.1035297886865));
#146702=CARTESIAN_POINT('Ctrl Pts',(-3.40463283991887,-6.13213717322749,
59.1122644213361));
#146703=CARTESIAN_POINT('Ctrl Pts',(-3.23395276927096,-6.22086618153973,
59.1209990539858));
#146704=CARTESIAN_POINT('Ctrl Pts',(-3.05982259761068,-6.31138874454317,
59.1299102471725));
#146705=CARTESIAN_POINT('Ctrl Pts',(-2.8818632914545,-6.39460954862002,
59.1388214403593));
#146706=CARTESIAN_POINT('Ctrl Pts',(-2.70069410209234,-6.47023012955673,
59.1477326335461));
#146707=CARTESIAN_POINT('Ctrl Pts',(-2.51952491273025,-6.5458507104934,
59.1566438267328));
#146708=CARTESIAN_POINT('Ctrl Pts',(-2.33514611471098,-6.61387093909174,
59.1655550199196));
#146709=CARTESIAN_POINT('Ctrl Pts',(-2.14820008150133,-6.67404397440845,
59.1744662131063));
#146710=CARTESIAN_POINT('Ctrl Pts',(-1.97983135953765,-6.72823745944264,
59.1824918779587));
#146711=CARTESIAN_POINT('Ctrl Pts',(-1.80930274092148,-6.7760902631983,
59.1905175428111));
#146712=CARTESIAN_POINT('Ctrl Pts',(-1.63714046594313,-6.81743336287723,
59.1985432076635));
#146713=CARTESIAN_POINT('Ctrl Pts',(-1.46503283104772,-6.85876334127046,
59.2065663253668));
#146714=CARTESIAN_POINT('Ctrl Pts',(-1.2912929280533,-6.89358764334637,
59.21458944307));
#146715=CARTESIAN_POINT('Ctrl Pts',(-1.11646092110653,-6.92178745514061,
59.2226125607733));
#146716=CARTESIAN_POINT('Ctrl Pts',(-0.941650962006826,-6.94998371069164,
59.2306346666911));
#146717=CARTESIAN_POINT('Ctrl Pts',(-0.76574953516945,-6.9715570822227,
59.2386567726089));
#146718=CARTESIAN_POINT('Ctrl Pts',(-0.589305679076254,-6.98644010774504,
59.2466788785268));
#146719=CARTESIAN_POINT('Ctrl Pts',(-0.41279625584923,-7.00132866385001,
59.2547039654863));
#146720=CARTESIAN_POINT('Ctrl Pts',(-0.23574436605913,-7.00952187356466,
59.2627290524459));
#146721=CARTESIAN_POINT('Ctrl Pts',(-0.0587032911843279,-7.01100424233962,
59.2707541394054));
#146722=CARTESIAN_POINT('Ctrl Pts',(0.11837265104363,-7.01248690305969,
59.2787808068656));
#146723=CARTESIAN_POINT('Ctrl Pts',(0.295437407489505,-7.00725609560233,
59.2868074743259));
#146724=CARTESIAN_POINT('Ctrl Pts',(0.47193923904547,-6.99534844858705,
59.2948341417861));
#146725=CARTESIAN_POINT('Ctrl Pts',(0.648582765650722,-6.98343124215465,
59.3028672530267));
#146726=CARTESIAN_POINT('Ctrl Pts',(0.824662099738474,-6.96482652455851,
59.3109003642673));
#146727=CARTESIAN_POINT('Ctrl Pts',(0.999631529102146,-6.93962271081973,
59.3189334755079));
#146728=CARTESIAN_POINT('Ctrl Pts',(1.1027298729944,-6.92477170818637,59.3236668764696));
#146729=CARTESIAN_POINT('Ctrl Pts',(1.20544302502316,-6.90763047736603,
59.3284002774312));
#146730=CARTESIAN_POINT('Ctrl Pts',(1.30766130588673,-6.88822534994222,
59.3331336783929));
#146731=CARTESIAN_POINT('Ctrl Pts',(1.51823414571167,-6.84825018352115,
59.3428846316872));
#146732=CARTESIAN_POINT('Ctrl Pts',(1.72683044093882,-6.79864205883776,
59.3526355849815));
#146733=CARTESIAN_POINT('Ctrl Pts',(1.93266228093756,-6.73961742759492,
59.3623865382758));
#146734=CARTESIAN_POINT('Ctrl Pts',(2.138790660315,-6.68050776029802,59.3721515396476));
#146735=CARTESIAN_POINT('Ctrl Pts',(2.34214658072248,-6.61195446061038,
59.3819165410193));
#146736=CARTESIAN_POINT('Ctrl Pts',(2.54195608502505,-6.5342241945241,59.3916815423911));
#146737=CARTESIAN_POINT('Ctrl Pts',(2.74143254828437,-6.45662348868572,
59.4014302675289));
#146738=CARTESIAN_POINT('Ctrl Pts',(2.93737437407866,-6.36987640088767,
59.4111789926666));
#146739=CARTESIAN_POINT('Ctrl Pts',(3.12902924003106,-6.27429697874835,
59.4209277178044));
#146740=CARTESIAN_POINT('Ctrl Pts',(3.32015808768823,-6.17897988506306,
59.4306496864717));
#146741=CARTESIAN_POINT('Ctrl Pts',(3.50702342874798,-6.0748788687175,59.4403716551389));
#146742=CARTESIAN_POINT('Ctrl Pts',(3.68889739736921,-5.96235377633554,
59.4500936238061));
#146743=CARTESIAN_POINT('Ctrl Pts',(3.86956795344513,-5.85057323309858,
59.459751264746));
#146744=CARTESIAN_POINT('Ctrl Pts',(4.04531291709129,-5.73047972517395,
59.4694089056859));
#146745=CARTESIAN_POINT('Ctrl Pts',(4.21543757068625,-5.6024737973637,59.4790665466259));
#146746=CARTESIAN_POINT('Ctrl Pts',(4.2902132129599,-5.54621078512777,59.4833114123103));
#146747=CARTESIAN_POINT('Ctrl Pts',(4.36390331477806,-5.48841979198442,
59.4875562779948));
#146748=CARTESIAN_POINT('Ctrl Pts',(4.43645009465427,-5.42913778791275,
59.4918011436793));
#146749=CARTESIAN_POINT('Ctrl Pts',(4.57064190642679,-5.31948220367514,
59.4996529906931));
#146750=CARTESIAN_POINT('Ctrl Pts',(4.70086432802666,-5.20476723100868,
59.5075048377069));
#146751=CARTESIAN_POINT('Ctrl Pts',(4.82670255273915,-5.08532880253395,
59.5153566847208));
#146752=CARTESIAN_POINT('Ctrl Pts',(4.95250509074879,-4.96592424583161,
59.5232063050143));
#146753=CARTESIAN_POINT('Ctrl Pts',(5.07392562864606,-4.84179916023225,
59.5310559253078));
#146754=CARTESIAN_POINT('Ctrl Pts',(5.19058382646348,-4.71332855877413,
59.5389055456013));
#146755=CARTESIAN_POINT('Ctrl Pts',(5.30723271061473,-4.58486821405163,
59.5467545392029));
#146756=CARTESIAN_POINT('Ctrl Pts',(5.41911975569858,-4.45206332703062,
59.5546035328045));
#146757=CARTESIAN_POINT('Ctrl Pts',(5.52590294794162,-4.31532422564402,
59.5624525264062));
#146758=CARTESIAN_POINT('Ctrl Pts',(5.63274020138915,-4.17851589725299,
59.5703054937235));
#146759=CARTESIAN_POINT('Ctrl Pts',(5.73446820407984,-4.0377696758671,59.5781584610409));
#146760=CARTESIAN_POINT('Ctrl Pts',(5.83078636956512,-3.89352756186387,
59.5860114283582));
#146761=CARTESIAN_POINT('Ctrl Pts',(5.92712899662768,-3.74924881521091,
59.5938663900654));
#146762=CARTESIAN_POINT('Ctrl Pts',(6.01805884938787,-3.60147273208194,
59.6017213517725));
#146763=CARTESIAN_POINT('Ctrl Pts',(6.10332020436586,-3.45066791295244,
59.6095763134797));
#146764=CARTESIAN_POINT('Ctrl Pts',(6.18866618836593,-3.29971340743369,
59.617439071893));
#146765=CARTESIAN_POINT('Ctrl Pts',(6.26833226190828,-3.14572450028115,
59.6253018303062));
#146766=CARTESIAN_POINT('Ctrl Pts',(6.3421097017522,-2.98919238147038,59.6331645887195));
#146767=CARTESIAN_POINT('Ctrl Pts',(6.39623177298422,-2.87436266520077,
59.6389325954682));
#146768=CARTESIAN_POINT('Ctrl Pts',(6.44718587697957,-2.75816478953243,
59.6447006022169));
#146769=CARTESIAN_POINT('Ctrl Pts',(6.49490656785004,-2.64079821974311,
59.6504686089657));
#146770=CARTESIAN_POINT('Ctrl Pts',(6.57394014154451,-2.44641923499858,
59.6600214083516));
#146771=CARTESIAN_POINT('Ctrl Pts',(6.64423617990191,-2.2485090433388,59.6695742077376));
#146772=CARTESIAN_POINT('Ctrl Pts',(6.70553042679575,-2.04780083450916,
59.6791270071235));
#146773=CARTESIAN_POINT('Ctrl Pts',(6.76670447562403,-1.84748621463226,
59.6886610734625));
#146774=CARTESIAN_POINT('Ctrl Pts',(6.81891197121808,-1.64438463374801,
59.6981951398015));
#146775=CARTESIAN_POINT('Ctrl Pts',(6.86193910720774,-1.43924224905782,
59.7077292061405));
#146776=CARTESIAN_POINT('Ctrl Pts',(6.90486689029431,-1.23457355361042,
59.717241257601));
#146777=CARTESIAN_POINT('Ctrl Pts',(6.93865661190477,-1.0278735591232,59.7267533090615));
#146778=CARTESIAN_POINT('Ctrl Pts',(6.96314526809213,-0.819899102296261,
59.736265360522));
#146779=CARTESIAN_POINT('Ctrl Pts',(6.98751355114625,-0.612946936639984,
59.7457306558262));
#146780=CARTESIAN_POINT('Ctrl Pts',(7.00267193531367,-0.404732904770793,
59.7551959511303));
#146781=CARTESIAN_POINT('Ctrl Pts',(7.00850939139864,-0.196017022671853,
59.7646612464345));
#146782=CARTESIAN_POINT('Ctrl Pts',(7.01033347227623,-0.130797748411864,
59.7676189499124));
#146783=CARTESIAN_POINT('Ctrl Pts',(7.01124779874313,-0.0655295714675496,
59.7705766533904));
#146784=CARTESIAN_POINT('Ctrl Pts',(7.01124999602994,-0.000235945344329035,
59.7735343568684));
#146785=CARTESIAN_POINT('Ctrl Pts',(7.01124999602997,-0.000235944414836881,
59.7735343569105));
#146786=CARTESIAN_POINT('Ctrl Pts',(7.01125624018264,0.185313331802434,
59.7819394612398));
#146787=CARTESIAN_POINT('Ctrl Pts',(7.0038924388928,0.370844036264387,59.790344565569));
#146788=CARTESIAN_POINT('Ctrl Pts',(6.98918905231667,0.555754400321562,
59.7987496698983));
#146789=CARTESIAN_POINT('Ctrl Pts',(6.97447793728878,0.740761957690168,
59.8071591921515));
#146790=CARTESIAN_POINT('Ctrl Pts',(6.95241955274104,0.925148202345302,
59.8155687144047));
#146791=CARTESIAN_POINT('Ctrl Pts',(6.92309629813099,1.10831593388573,59.8239782366579));
#146792=CARTESIAN_POINT('Ctrl Pts',(6.89376518002966,1.29153278473029,59.8323900140566));
#146793=CARTESIAN_POINT('Ctrl Pts',(6.85716536206296,1.47353015410552,59.8408017914553));
#146794=CARTESIAN_POINT('Ctrl Pts',(6.81343045669716,1.65372064577168,59.849213568854));
#146795=CARTESIAN_POINT('Ctrl Pts',(6.76966412479619,1.83404061668966,59.8576313906928));
#146796=CARTESIAN_POINT('Ctrl Pts',(6.71875254183586,2.01255080428954,59.8660492125316));
#146797=CARTESIAN_POINT('Ctrl Pts',(6.66087961695624,2.18867752099686,59.8744670343705));
#146798=CARTESIAN_POINT('Ctrl Pts',(6.63260803866194,2.27471741394277,59.8785792355367));
#146799=CARTESIAN_POINT('Ctrl Pts',(6.60267593100112,2.3601887632264,59.882691436703));
#146800=CARTESIAN_POINT('Ctrl Pts',(6.57110895151811,2.44502632087643,59.8868036378692));
#146801=CARTESIAN_POINT('',(7.01125,-8.5868812060852E-16,59.2264656430896));
#146802=CARTESIAN_POINT('Ctrl Pts',(6.57110895151816,2.4450263208763,59.3399667921338));
#146803=CARTESIAN_POINT('Ctrl Pts',(6.64787822596452,2.23870573356451,59.3299508081697));
#146804=CARTESIAN_POINT('Ctrl Pts',(6.71486704351225,2.02892736619064,59.3199348242056));
#146805=CARTESIAN_POINT('Ctrl Pts',(6.77184227450777,1.81652932034951,59.3099188402415));
#146806=CARTESIAN_POINT('Ctrl Pts',(6.82887754402312,1.60390745682371,59.2998923017813));
#146807=CARTESIAN_POINT('Ctrl Pts',(6.87587814593312,1.38866035124284,59.2898657633211));
#146808=CARTESIAN_POINT('Ctrl Pts',(6.91266147369141,1.17163898562759,59.2798392248609));
#146809=CARTESIAN_POINT('Ctrl Pts',(6.94931701083637,0.95537158369946,59.2698475200489));
#146810=CARTESIAN_POINT('Ctrl Pts',(6.97582616014358,0.737342184747944,
59.259855815237));
#146811=CARTESIAN_POINT('Ctrl Pts',(6.99205864969101,0.518403705408438,
59.249864110425));
#146812=CARTESIAN_POINT('Ctrl Pts',(7.00472967309146,0.347501109915278,
59.2420646213132));
#146813=CARTESIAN_POINT('Ctrl Pts',(7.01113979294834,0.176044788858334,
59.2342651322014));
#146814=CARTESIAN_POINT('Ctrl Pts',(7.01124859079596,0.00444528533067366,
59.2264656430896));
#146815=CARTESIAN_POINT('Ctrl Pts',(7.01125,-8.58630487052188E-16,59.2264656430896));
#146816=CARTESIAN_POINT('Ctrl Pts',(7.01125,-0.191009525814462,59.2177938341508));
#146817=CARTESIAN_POINT('Ctrl Pts',(7.00344006572041,-0.382018909628726,
59.209122025212));
#146818=CARTESIAN_POINT('Ctrl Pts',(6.98784625534317,-0.572390840411034,
59.2004502162733));
#146819=CARTESIAN_POINT('Ctrl Pts',(6.97225246786074,-0.762762491689531,
59.1917784200664));
#146820=CARTESIAN_POINT('Ctrl Pts',(6.94887485033525,-0.952496408757991,
59.1831066238596));
#146821=CARTESIAN_POINT('Ctrl Pts',(6.91779140296513,-1.14095953809139,
59.1744348276527));
#146822=CARTESIAN_POINT('Ctrl Pts',(6.88670800059787,-1.32942239456645,
59.165763044001));
#146823=CARTESIAN_POINT('Ctrl Pts',(6.84791883692705,-1.51661418677696,
59.1570912603492));
#146824=CARTESIAN_POINT('Ctrl Pts',(6.80155333291305,-1.70191034488875,
59.1484194766975));
#146825=CARTESIAN_POINT('Ctrl Pts',(6.75518789508205,-1.88720623850532,
59.139747705424));
#146826=CARTESIAN_POINT('Ctrl Pts',(6.70124620748597,-2.07060622793696,
59.1310759341505));
#146827=CARTESIAN_POINT('Ctrl Pts',(6.63990824732571,-2.25149839653418,
59.122404162877));
#146828=CARTESIAN_POINT('Ctrl Pts',(6.57857037346951,-2.43239031061157,
59.113732403805));
#146829=CARTESIAN_POINT('Ctrl Pts',(6.50983633907179,-2.61077414196406,
59.1050606447329));
#146830=CARTESIAN_POINT('Ctrl Pts',(6.43393547556233,-2.78605471209748,
59.0963888856608));
#146831=CARTESIAN_POINT('Ctrl Pts',(6.35803471730007,-2.96133503917979,
59.0877171386133));
#146832=CARTESIAN_POINT('Ctrl Pts',(6.27496726266193,-3.1335118530473,59.0790453915658));
#146833=CARTESIAN_POINT('Ctrl Pts',(6.18501026583403,-3.30201068654051,
59.0703736445184));
#146834=CARTESIAN_POINT('Ctrl Pts',(6.09151188668825,-3.47714289832064,
59.0613605124454));
#146835=CARTESIAN_POINT('Ctrl Pts',(5.99057066119165,-3.64830137931007,
59.0523473803724));
#146836=CARTESIAN_POINT('Ctrl Pts',(5.88255038916588,-3.81486926138032,
59.0433342482994));
#146837=CARTESIAN_POINT('Ctrl Pts',(5.77621793389049,-3.97883452029324,
59.034461946415));
#146838=CARTESIAN_POINT('Ctrl Pts',(5.66302622906376,-4.13835132493741,
59.0255896445306));
#146839=CARTESIAN_POINT('Ctrl Pts',(5.54337059052903,-4.29286257158994,
59.0167173426463));
#146840=CARTESIAN_POINT('Ctrl Pts',(5.42558457134642,-4.44495958001353,
59.0079836704789));
#146841=CARTESIAN_POINT('Ctrl Pts',(5.30153533574937,-4.59220608124103,
58.9992499983114));
#146842=CARTESIAN_POINT('Ctrl Pts',(5.17164269972312,-4.73410375349976,
58.990516326144));
#146843=CARTESIAN_POINT('Ctrl Pts',(5.04265587431577,-4.87501189762002,
58.98184355853));
#146844=CARTESIAN_POINT('Ctrl Pts',(4.9079071016412,-5.01064538261968,58.973170790916));
#146845=CARTESIAN_POINT('Ctrl Pts',(4.7678460760923,-5.14055156157307,58.964498023302));
#146846=CARTESIAN_POINT('Ctrl Pts',(4.62778576967364,-5.27045707353532,
58.9558253002176));
#146847=CARTESIAN_POINT('Ctrl Pts',(4.48241347329788,-5.39463514506495,
58.9471525771331));
#146848=CARTESIAN_POINT('Ctrl Pts',(4.3322143300549,-5.51267136341058,58.9384798540486));
#146849=CARTESIAN_POINT('Ctrl Pts',(4.18201594573482,-5.63070698534541,
58.9298071747855));
#146850=CARTESIAN_POINT('Ctrl Pts',(4.02699098676462,-5.74260064062568,
58.9211344955223));
#146851=CARTESIAN_POINT('Ctrl Pts',(3.86765680431923,-5.84797891638668,
58.9124618162592));
#146852=CARTESIAN_POINT('Ctrl Pts',(3.70832341394854,-5.9533566682961,58.9037891801093));
#146853=CARTESIAN_POINT('Ctrl Pts',(3.54468107996522,-6.0522189487593,58.8951165439594));
#146854=CARTESIAN_POINT('Ctrl Pts',(3.37727590612859,-6.14423583665075,
58.8864439078095));
#146855=CARTESIAN_POINT('Ctrl Pts',(3.20987155082483,-6.23625227462273,
58.8777713140647));
#146856=CARTESIAN_POINT('Ctrl Pts',(3.0387046414804,-6.32142325013736,58.8690987203199));
#146857=CARTESIAN_POINT('Ctrl Pts',(2.86434638712907,-6.3994645351811,58.8604261265751));
#146858=CARTESIAN_POINT('Ctrl Pts',(2.68998897107704,-6.47750544500914,
58.8517535745274));
#146859=CARTESIAN_POINT('Ctrl Pts',(2.51244050005463,-6.5484166168872,58.8430810224797));
#146860=CARTESIAN_POINT('Ctrl Pts',(2.33229347360944,-6.61196141212718,
58.834408470432));
#146861=CARTESIAN_POINT('Ctrl Pts',(2.15214729859244,-6.67550590703564,
58.8257359593733));
#146862=CARTESIAN_POINT('Ctrl Pts',(1.96940286066631,-6.73168400046421,
58.8170634483147));
#146863=CARTESIAN_POINT('Ctrl Pts',(1.78466999315554,-6.78030822146237,
58.808390937256));
#146864=CARTESIAN_POINT('Ctrl Pts',(1.59993798367062,-6.82893221661638,
58.7997184664784));
#146865=CARTESIAN_POINT('Ctrl Pts',(1.41321783783503,-6.8700023372309,58.7910459957009));
#146866=CARTESIAN_POINT('Ctrl Pts',(1.22513265045738,-6.90338153018383,
58.7823735249233));
#146867=CARTESIAN_POINT('Ctrl Pts',(1.03704832132596,-6.93676057082511,
58.7737010937188));
#146868=CARTESIAN_POINT('Ctrl Pts',(0.847599242850215,-6.96244870438833,
58.7650286625143));
#146869=CARTESIAN_POINT('Ctrl Pts',(0.657417610664734,-6.9803602090213,
58.7563562313098));
#146870=CARTESIAN_POINT('Ctrl Pts',(0.467236830771745,-6.99827163338448,
58.7476838389706));
#146871=CARTESIAN_POINT('Ctrl Pts',(0.276323786584655,-7.00840647191863,
58.7390114466313));
#146872=CARTESIAN_POINT('Ctrl Pts',(0.0853155533185971,-7.01073090475322,
58.730339054292));
#146873=CARTESIAN_POINT('Ctrl Pts',(-0.105691839537741,-7.01305532736064,
58.7216667001101));
#146874=CARTESIAN_POINT('Ctrl Pts',(-0.296794136564428,-7.00756940957899,
58.7129943459281));
#146875=CARTESIAN_POINT('Ctrl Pts',(-0.487353636617199,-6.99429145770864,
58.7043219917462));
#146876=CARTESIAN_POINT('Ctrl Pts',(-0.677912313784896,-6.9810135631759,
58.6956496750137));
#146877=CARTESIAN_POINT('Ctrl Pts',(-0.867927915270903,-6.95994372163458,
58.6869773582812));
#146878=CARTESIAN_POINT('Ctrl Pts',(-1.05676637166362,-6.93115224174314,
58.6783050415487));
#146879=CARTESIAN_POINT('Ctrl Pts',(-1.24560402801224,-6.90236088383137,
58.6696327615579));
#146880=CARTESIAN_POINT('Ctrl Pts',(-1.43326426841345,-6.86584799585127,
58.660960481567));
#146881=CARTESIAN_POINT('Ctrl Pts',(-1.61912088843955,-6.82173541784777,
58.6522882015762));
#146882=CARTESIAN_POINT('Ctrl Pts',(-1.80497673622004,-6.77762302313473,
58.6436159576192));
#146883=CARTESIAN_POINT('Ctrl Pts',(-1.98902870222715,-6.7259110671892,
58.6349437136622));
#146884=CARTESIAN_POINT('Ctrl Pts',(-2.17066262760132,-6.66677210647214,
58.6262714697052));
#146885=CARTESIAN_POINT('Ctrl Pts',(-2.35229581309554,-6.60763338665573,
58.6175992610743));
#146886=CARTESIAN_POINT('Ctrl Pts',(-2.53151070755663,-6.54106781055513,
58.6089270524435));
#146887=CARTESIAN_POINT('Ctrl Pts',(-2.70770929770725,-6.46729749753402,
58.6002548438126));
#146888=CARTESIAN_POINT('Ctrl Pts',(-2.88390718449518,-6.39352747899475,
58.5915826698001));
#146889=CARTESIAN_POINT('Ctrl Pts',(-3.05708852904383,-6.31255289079089,
58.5829104957876));
#146890=CARTESIAN_POINT('Ctrl Pts',(-3.22667545573784,-6.22464393084769,
58.574238321775));
#146891=CARTESIAN_POINT('Ctrl Pts',(-3.39626171929845,-6.13673531465368,
58.5655661816732));
#146892=CARTESIAN_POINT('Ctrl Pts',(-3.56225334094293,-6.04189251170778,
58.5568940415714));
#146893=CARTESIAN_POINT('Ctrl Pts',(-3.72409644022107,-5.94043199325039,
58.5482219014696));
#146894=CARTESIAN_POINT('Ctrl Pts',(-3.88593891985092,-5.83897186325464,
58.5395497945707));
#146895=CARTESIAN_POINT('Ctrl Pts',(-4.04363266823074,-5.7308942193264,
58.5308776876719));
#146896=CARTESIAN_POINT('Ctrl Pts',(-4.19665149725939,-5.61655969193336,
58.5222055807731));
#146897=CARTESIAN_POINT('Ctrl Pts',(-4.34966975290894,-5.50222559296491,
58.5135335063696));
#146898=CARTESIAN_POINT('Ctrl Pts',(-4.49801289671901,-5.38163482746632,
58.5048614319662));
#146899=CARTESIAN_POINT('Ctrl Pts',(-4.64118594513082,-5.2551897763278,
58.4961893575627));
#146900=CARTESIAN_POINT('Ctrl Pts',(-4.78435846873758,-5.12874518867735,
58.487517314947));
#146901=CARTESIAN_POINT('Ctrl Pts',(-4.92236072197075,-4.99644654635288,
58.4788452723313));
#146902=CARTESIAN_POINT('Ctrl Pts',(-5.05473222958088,-4.85873529323592,
58.4701732297156));
#146903=CARTESIAN_POINT('Ctrl Pts',(-5.18710326277798,-4.72102453366937,
58.4615012181801));
#146904=CARTESIAN_POINT('Ctrl Pts',(-5.31384339390117,-4.57790140690284,
58.4528292066446));
#146905=CARTESIAN_POINT('Ctrl Pts',(-5.43452972930759,-4.429843471701,58.4441571951091));
#146906=CARTESIAN_POINT('Ctrl Pts',(-5.55521564202563,-4.28178605505306,
58.4354852139461));
#146907=CARTESIAN_POINT('Ctrl Pts',(-5.66984762199996,-4.1287940847122,
58.4268132327832));
#146908=CARTESIAN_POINT('Ctrl Pts',(-5.77804317951767,-3.97137804522931,
58.4181412516203));
#146909=CARTESIAN_POINT('Ctrl Pts',(-5.88623836692049,-3.81396254423451,
58.4094693001225));
#146910=CARTESIAN_POINT('Ctrl Pts',(-5.98799701504623,-3.65212323845021,
58.4007973486246));
#146911=CARTESIAN_POINT('Ctrl Pts',(-6.08297959063289,-3.48640012942344,
58.3921253971268));
#146912=CARTESIAN_POINT('Ctrl Pts',(-6.17796184905169,-3.32067757378284,
58.3834534745865));
#146913=CARTESIAN_POINT('Ctrl Pts',(-6.26616793897866,-3.15107148726879,
58.3747815520462));
#146914=CARTESIAN_POINT('Ctrl Pts',(-6.3473035492945,-2.97814778270211,
58.3661096295059));
#146915=CARTESIAN_POINT('Ctrl Pts',(-6.42843889529885,-2.80522464146048,
58.3574377352158));
#146916=CARTESIAN_POINT('Ctrl Pts',(-6.50250368714336,-2.62898416091372,
58.3487658409256));
#146917=CARTESIAN_POINT('Ctrl Pts',(-6.56925079960199,-2.45001438657584,
58.3400939466354));
#146918=CARTESIAN_POINT('Ctrl Pts',(-6.63599770006635,-2.2710451806606,
58.3314220798879));
#146919=CARTESIAN_POINT('Ctrl Pts',(-6.69542686840867,-2.08934696440751,
58.3227502131403));
#146920=CARTESIAN_POINT('Ctrl Pts',(-6.7473400140094,-1.90552598981166,
58.3140783463928));
#146921=CARTESIAN_POINT('Ctrl Pts',(-6.79925299896442,-1.7217055840515,
58.3054065064804));
#146922=CARTESIAN_POINT('Ctrl Pts',(-6.84364993053273,-1.53576270641015,
58.2967346665681));
#146923=CARTESIAN_POINT('Ctrl Pts',(-6.88038267538378,-1.34831776773087,
58.2880628266557));
#146924=CARTESIAN_POINT('Ctrl Pts',(-6.91711530956105,-1.1608733938131,
58.2793910128711));
#146925=CARTESIAN_POINT('Ctrl Pts',(-6.94618374861435,-0.971927246615138,
58.2707191990866));
#146926=CARTESIAN_POINT('Ctrl Pts',(-6.96749100433714,-0.782109753794825,
58.262047385302));
#146927=CARTESIAN_POINT('Ctrl Pts',(-6.9887981976002,-0.592292817402312,
58.2533755969378));
#146928=CARTESIAN_POINT('Ctrl Pts',(-7.00234422137977,-0.401604822724534,
58.2447038085736));
#146929=CARTESIAN_POINT('Ctrl Pts',(-7.00808387899861,-0.210682005448528,
58.2360320202095));
#146930=CARTESIAN_POINT('Ctrl Pts',(-7.01382352026048,-0.0197597322676766,
58.2273602565583));
#146931=CARTESIAN_POINT('Ctrl Pts',(-7.01175683134594,0.171397078306313,
58.2186884929072));
#146932=CARTESIAN_POINT('Ctrl Pts',(-7.00189070777957,0.362150630000985,
58.210016729256));
#146933=CARTESIAN_POINT('Ctrl Pts',(-6.9915780829724,0.561536923516253,
58.2009525163107));
#146934=CARTESIAN_POINT('Ctrl Pts',(-6.97274368607516,0.760482277946813,
58.1918883033653));
#146935=CARTESIAN_POINT('Ctrl Pts',(-6.94545616842791,0.958261537862561,
58.1828240904199));
#146936=CARTESIAN_POINT('Ctrl Pts',(-6.91902138570714,1.14986019590593,
58.1740431341291));
#146937=CARTESIAN_POINT('Ctrl Pts',(-6.88465388689258,1.34036422799789,
58.1652621778383));
#146938=CARTESIAN_POINT('Ctrl Pts',(-6.84247124235198,1.52912192453256,
58.1564812215475));
#146939=CARTESIAN_POINT('Ctrl Pts',(-6.80080846652261,1.71555332736278,
58.147808483802));
#146940=CARTESIAN_POINT('Ctrl Pts',(-6.75152215882473,1.90028091508853,
58.1391357460565));
#146941=CARTESIAN_POINT('Ctrl Pts',(-6.69477680033874,2.08268820425579,
58.130463008311));
#146942=CARTESIAN_POINT('Ctrl Pts',(-6.63803201373068,2.26509365512815,
58.1217903579691));
#146943=CARTESIAN_POINT('Ctrl Pts',(-6.57382841116582,2.44517858291869,
58.1131177076272));
#146944=CARTESIAN_POINT('Ctrl Pts',(-6.50238025225844,2.62234201002453,
58.1044450572853));
#146945=CARTESIAN_POINT('Ctrl Pts',(-6.43093279007603,2.79950370952556,
58.0957724915145));
#146946=CARTESIAN_POINT('Ctrl Pts',(-6.35224101918865,2.97374370184446,
58.0870999257437));
#146947=CARTESIAN_POINT('Ctrl Pts',(-6.26656754386312,3.14448052636702,
58.078427359973));
#146948=CARTESIAN_POINT('Ctrl Pts',(-6.18089487601068,3.31521574169382,
58.0697548759412));
#146949=CARTESIAN_POINT('Ctrl Pts',(-6.08824076282076,3.48244760135704,
58.0610823919094));
#146950=CARTESIAN_POINT('Ctrl Pts',(-5.98891439681757,3.64561804226544,
58.0524099078776));
#146951=CARTESIAN_POINT('Ctrl Pts',(-5.88958893454135,3.80878699855768,
58.0437375027529));
#146952=CARTESIAN_POINT('Ctrl Pts',(-5.78359148865815,3.96789436736601,
58.0350650976283));
#146953=CARTESIAN_POINT('Ctrl Pts',(-5.67127577279106,4.12240920718131,
58.0263926925036));
#146954=CARTESIAN_POINT('Ctrl Pts',(-5.55896104217282,4.27692269157125,
58.0177203634545));
#146955=CARTESIAN_POINT('Ctrl Pts',(-5.44032831951742,4.42684349779038,
58.0090480344054));
#146956=CARTESIAN_POINT('Ctrl Pts',(-5.31577347544553,4.57167134866995,
58.0003757053562));
#146957=CARTESIAN_POINT('Ctrl Pts',(-5.19121968333082,4.71649797637192,
57.9917034495513));
#146958=CARTESIAN_POINT('Ctrl Pts',(-5.06074405512004,4.8562315194283,57.9830311937463));
#146959=CARTESIAN_POINT('Ctrl Pts',(-4.92478197318643,4.99040570285402,
57.9743589379414));
#146960=CARTESIAN_POINT('Ctrl Pts',(-4.78882099517689,5.12457879687227,
57.9656867525496));
#146961=CARTESIAN_POINT('Ctrl Pts',(-4.64737385477618,5.25319242205562,
57.9570145671577));
#146962=CARTESIAN_POINT('Ctrl Pts',(-4.50091253739251,5.37581741628591,
57.9483423817659));
#146963=CARTESIAN_POINT('Ctrl Pts',(-4.3544523613803,5.49844145490095,57.9396702639563));
#146964=CARTESIAN_POINT('Ctrl Pts',(-4.20297830437536,5.61507677360282,
57.9309981461467));
#146965=CARTESIAN_POINT('Ctrl Pts',(-4.04699580205666,5.72533418593498,
57.9223260283371));
#146966=CARTESIAN_POINT('Ctrl Pts',(-3.89101446440432,5.83559077501392,
57.9136539752791));
#146967=CARTESIAN_POINT('Ctrl Pts',(-3.73052498074915,5.93946938906479,
57.9049819222212));
#146968=CARTESIAN_POINT('Ctrl Pts',(-3.56606286128093,6.03662341312533,
57.8963098691632));
#146969=CARTESIAN_POINT('Ctrl Pts',(-3.40160191612509,6.13377674347491,
57.8876378780265));
#146970=CARTESIAN_POINT('Ctrl Pts',(-3.2331686364694,6.2242054354536,57.8789658868898));
#146971=CARTESIAN_POINT('Ctrl Pts',(-3.06132503079386,6.30760775717189,
57.8702938957531));
#146972=CARTESIAN_POINT('Ctrl Pts',(-2.8894825960632,6.39100951058552,57.8616219637075));
#146973=CARTESIAN_POINT('Ctrl Pts',(-2.7142301373335,6.46738486553392,57.8529500316619));
#146974=CARTESIAN_POINT('Ctrl Pts',(-2.5361524085633,6.53647898512942,57.8442780996162));
#146975=CARTESIAN_POINT('Ctrl Pts',(-2.35807583511184,6.60557265646151,
57.8356062238317));
#146976=CARTESIAN_POINT('Ctrl Pts',(-2.17717429308117,6.66738508423481,
57.8269343480472));
#146977=CARTESIAN_POINT('Ctrl Pts',(-1.99405137754989,6.72171002544675,
57.8182624722626));
#146978=CARTESIAN_POINT('Ctrl Pts',(-1.81092959032083,6.77603463193842,
57.8095906499094));
#146979=CARTESIAN_POINT('Ctrl Pts',(-1.62558672925683,6.82287176341404,
57.8009188275561));
#146980=CARTESIAN_POINT('Ctrl Pts',(-1.43864120070387,6.86206514528515,
57.7922470052029));
#146981=CARTESIAN_POINT('Ctrl Pts',(-1.25169676301303,6.90125829845556,
57.7835752334514));
#146982=CARTESIAN_POINT('Ctrl Pts',(-1.06314995450122,6.93280773300277,
57.7749034616998));
#146983=CARTESIAN_POINT('Ctrl Pts',(-0.873629864321623,6.95660818378219,
57.7662316899483));
#146984=CARTESIAN_POINT('Ctrl Pts',(-0.679495509708901,6.98098810649739,
57.7573487857098));
#146985=CARTESIAN_POINT('Ctrl Pts',(-0.48434018208405,6.99723686027501,
57.7484658814713));
#146986=CARTESIAN_POINT('Ctrl Pts',(-0.288847078968885,7.00529756166511,
57.7395829772329));
#146987=CARTESIAN_POINT('Ctrl Pts',(-0.0979805523943737,7.0131674969803,
57.7309102974765));
#146988=CARTESIAN_POINT('Ctrl Pts',(0.0932076478891657,7.01323255451603,
57.7222376177202));
#146989=CARTESIAN_POINT('Ctrl Pts',(0.284079486226396,7.00549251716147,
57.7135649379638));
#146990=CARTESIAN_POINT('Ctrl Pts',(0.474947621918049,6.99775262995276,
57.7048924264453));
#146991=CARTESIAN_POINT('Ctrl Pts',(0.665499124053657,6.98220796234689,
57.6962199149268));
#146992=CARTESIAN_POINT('Ctrl Pts',(0.855098106421533,6.95891038819256,
57.6875474034082));
#146993=CARTESIAN_POINT('Ctrl Pts',(1.04469365841792,6.93561323555597,57.6788750487995));
#146994=CARTESIAN_POINT('Ctrl Pts',(1.23333644315622,6.90456349171623,57.6702026941907));
#146995=CARTESIAN_POINT('Ctrl Pts',(1.42039696672986,6.86586476850547,57.661530339582));
#146996=CARTESIAN_POINT('Ctrl Pts',(1.60745435009459,6.82716669493512,57.6528581305571));
#146997=CARTESIAN_POINT('Ctrl Pts',(1.79292924726445,6.78081995649295,57.6441859215323));
#146998=CARTESIAN_POINT('Ctrl Pts',(1.97620275621391,6.72697920532185,57.6355137125075));
#146999=CARTESIAN_POINT('Ctrl Pts',(2.15947342778787,6.67313928769417,57.6268416377427));
#147000=CARTESIAN_POINT('Ctrl Pts',(2.3405425068073,6.61180566956694,57.618169562978));
#147001=CARTESIAN_POINT('Ctrl Pts',(2.51880581149286,6.54318300573122,57.6094974882132));
#147002=CARTESIAN_POINT('Ctrl Pts',(2.69706658906144,6.47456131471208,57.6008255363865));
#147003=CARTESIAN_POINT('Ctrl Pts',(2.87252140682272,6.39865088679973,57.5921535845598));
#147004=CARTESIAN_POINT('Ctrl Pts',(3.04458483295129,6.31570500874312,57.5834816327332));
#147005=CARTESIAN_POINT('Ctrl Pts',(3.21664604443053,6.23276019829303,57.5748097925242));
#147006=CARTESIAN_POINT('Ctrl Pts',(3.38531569579111,6.14278024223614,57.5661379523153));
#147007=CARTESIAN_POINT('Ctrl Pts',(3.55003100942567,6.04606536473236,57.5574661121063));
#147008=CARTESIAN_POINT('Ctrl Pts',(3.72225670716351,5.9449406611928,57.5483988693728));
#147009=CARTESIAN_POINT('Ctrl Pts',(3.89015872998899,5.8364526481946,57.5393316266393));
#147010=CARTESIAN_POINT('Ctrl Pts',(4.05312466660087,5.72099702844632,57.5302643839057));
#147011=CARTESIAN_POINT('Ctrl Pts',(4.20899688868252,5.61056705531127,57.5215918275273));
#147012=CARTESIAN_POINT('Ctrl Pts',(4.36035338104125,5.49376336253442,57.5129192711489));
#147013=CARTESIAN_POINT('Ctrl Pts',(4.50668904925292,5.37097573778208,57.5042467147704));
#147014=CARTESIAN_POINT('Ctrl Pts',(4.65301950884331,5.2481924834901,57.49557446708));
#147015=CARTESIAN_POINT('Ctrl Pts',(4.7943292842724,5.11942590603737,57.4869022193895));
#147016=CARTESIAN_POINT('Ctrl Pts',(4.930146841728,4.98510568408529,57.4782299716991));
#147017=CARTESIAN_POINT('Ctrl Pts',(5.06596027420137,4.85078954163911,57.4695579873978));
#147018=CARTESIAN_POINT('Ctrl Pts',(5.19628162053707,4.71092029195257,57.4608860030965));
#147019=CARTESIAN_POINT('Ctrl Pts',(5.32067604038424,4.56596463365422,57.4522140187951));
#147020=CARTESIAN_POINT('Ctrl Pts',(5.44506733164634,4.4210126210669,57.4435422525988));
#147021=CARTESIAN_POINT('Ctrl Pts',(5.56353180975929,4.27097467138257,57.4348704864024));
#147022=CARTESIAN_POINT('Ctrl Pts',(5.67567421678466,4.11635138774934,57.4261987202061));
#147023=CARTESIAN_POINT('Ctrl Pts',(5.78782406006403,3.9617178509207,57.4175263789778));
#147024=CARTESIAN_POINT('Ctrl Pts',(5.89365082654566,3.80249860161938,57.4088540377496));
#147025=CARTESIAN_POINT('Ctrl Pts',(5.99280137736245,3.63922494687849,57.4001816965214));
#147026=CARTESIAN_POINT('Ctrl Pts',(6.09194609291145,3.47596090121682,57.391509865683));
#147027=CARTESIAN_POINT('Ctrl Pts',(6.18441523160766,3.30864317036249,57.3828380348447));
#147028=CARTESIAN_POINT('Ctrl Pts',(6.26990026463242,3.13783001994409,57.3741662040063));
#147029=CARTESIAN_POINT('Ctrl Pts',(6.35538670852655,2.96701405037675,57.3654942300455));
#147030=CARTESIAN_POINT('Ctrl Pts',(6.43388868897279,2.79270279979035,57.3568222560848));
#147031=CARTESIAN_POINT('Ctrl Pts',(6.50514427077518,2.6154778872896,57.3481502821241));
#147032=CARTESIAN_POINT('Ctrl Pts',(6.52787183386361,2.55895052090203,57.3453842835832));
#147033=CARTESIAN_POINT('Ctrl Pts',(6.5498625512979,2.50212689663814,57.3426182850423));
#147034=CARTESIAN_POINT('Ctrl Pts',(6.57110895151816,2.4450263208763,57.3398522865015));
#147035=CARTESIAN_POINT('Origin',(0.,0.,50.));
#147036=CARTESIAN_POINT('',(6.57110895151813,2.44502632087638,55.3399173263397));
#147037=CARTESIAN_POINT('',(6.57110895151812,2.44502632087641,55.886985753209));
#147038=CARTESIAN_POINT('',(6.57110895151814,2.44502632087636,50.));
#147039=CARTESIAN_POINT('',(7.01124831048998,-0.00486735569172974,57.7735343569399));
#147040=CARTESIAN_POINT('Ctrl Pts',(6.57110895151812,2.44502632087642,55.886985753209));
#147041=CARTESIAN_POINT('Ctrl Pts',(6.50692229192473,2.61753061247478,55.8953627491612));
#147042=CARTESIAN_POINT('Ctrl Pts',(6.43589784857362,2.78761567826404,55.9037397451133));
#147043=CARTESIAN_POINT('Ctrl Pts',(6.35824132120199,2.954723991147,55.9121167410655));
#147044=CARTESIAN_POINT('Ctrl Pts',(6.28063626007775,3.1217215543214,55.92048818523));
#147045=CARTESIAN_POINT('Ctrl Pts',(6.19640801680893,3.28574600083383,55.9288596293946));
#147046=CARTESIAN_POINT('Ctrl Pts',(6.10581046081725,3.44625959252559,55.9372310735591));
#147047=CARTESIAN_POINT('Ctrl Pts',(6.01525966353638,3.6066903408279,55.9455981971001));
#147048=CARTESIAN_POINT('Ctrl Pts',(5.91834626998841,3.76361356190755,55.9539653206411));
#147049=CARTESIAN_POINT('Ctrl Pts',(5.8153703705518,3.91651554520192,55.962332444182));
#147050=CARTESIAN_POINT('Ctrl Pts',(5.7124277728145,4.06936808104401,55.9706968618527));
#147051=CARTESIAN_POINT('Ctrl Pts',(5.60342676106945,4.21820169925229,55.9790612795233));
#147052=CARTESIAN_POINT('Ctrl Pts',(5.48871137006098,4.36253069429469,55.9874256971939));
#147053=CARTESIAN_POINT('Ctrl Pts',(5.37401714775546,4.50683305596561,55.9957885713587));
#147054=CARTESIAN_POINT('Ctrl Pts',(5.25361085293471,4.64663219454363,56.0041514455235));
#147055=CARTESIAN_POINT('Ctrl Pts',(5.12787778651435,4.78147424640902,56.0125143196883));
#147056=CARTESIAN_POINT('Ctrl Pts',(5.00215116167431,4.91630939002082,56.0208767654048));
#147057=CARTESIAN_POINT('Ctrl Pts',(4.87109853372871,5.04618771315425,56.0292392111212));
#147058=CARTESIAN_POINT('Ctrl Pts',(4.73514344505988,5.17069077756604,56.0376016568377));
#147059=CARTESIAN_POINT('Ctrl Pts',(4.59917720012601,5.2952040585074,56.0459647887636));
#147060=CARTESIAN_POINT('Ctrl Pts',(4.45830793515744,5.41434097976978,56.0543279206894));
#147061=CARTESIAN_POINT('Ctrl Pts',(4.3129940934042,5.52772181940811,56.0626910526153));
#147062=CARTESIAN_POINT('Ctrl Pts',(4.16759669615451,5.64116785305844,56.0710589933442));
#147063=CARTESIAN_POINT('Ctrl Pts',(4.01774987339592,5.74885098721903,56.079426934073));
#147064=CARTESIAN_POINT('Ctrl Pts',(3.86394387481114,5.85043282969812,56.0877948748019));
#147065=CARTESIAN_POINT('Ctrl Pts',(3.71009612548348,5.9520422466374,56.096165087014));
#147066=CARTESIAN_POINT('Ctrl Pts',(3.55228733458885,6.04754689257731,56.1045352992261));
#147067=CARTESIAN_POINT('Ctrl Pts',(3.39103505703203,6.13665281765881,56.1129055114382));
#147068=CARTESIAN_POINT('Ctrl Pts',(3.22963973294287,6.22583778840581,56.1212831488466));
#147069=CARTESIAN_POINT('Ctrl Pts',(3.06479510755026,6.30861253885692,56.1296607862551));
#147070=CARTESIAN_POINT('Ctrl Pts',(2.89704270074082,6.38472945022609,56.1380384236636));
#147071=CARTESIAN_POINT('Ctrl Pts',(2.75189695517394,6.4505886892144,56.1452870733305));
#147072=CARTESIAN_POINT('Ctrl Pts',(2.60457481242047,6.51146432822324,56.1525357229974));
#147073=CARTESIAN_POINT('Ctrl Pts',(2.45543802521295,6.56722549230939,56.1597843726644));
#147074=CARTESIAN_POINT('Ctrl Pts',(2.29366480687932,6.62771132642955,56.1676472038755));
#147075=CARTESIAN_POINT('Ctrl Pts',(2.12941952631151,6.68230366807814,56.1755100350867));
#147076=CARTESIAN_POINT('Ctrl Pts',(1.96318930483182,6.7307885359662,56.1833728662979));
#147077=CARTESIAN_POINT('Ctrl Pts',(1.79708680933532,6.77923614963317,56.1912296559611));
#147078=CARTESIAN_POINT('Ctrl Pts',(1.62900276959128,6.82158551575422,56.1990864456244));
#147079=CARTESIAN_POINT('Ctrl Pts',(1.45944377323308,6.85767091914385,56.2069432352877));
#147080=CARTESIAN_POINT('Ctrl Pts',(1.28998040012236,6.89373597207415,56.2147955940935));
#147081=CARTESIAN_POINT('Ctrl Pts',(1.11904409680735,6.92354401026403,56.2226479528993));
#147082=CARTESIAN_POINT('Ctrl Pts',(0.947155836532505,6.94697937119598,
56.2305003117051));
#147083=CARTESIAN_POINT('Ctrl Pts',(0.775308161083144,6.97040919876553,
56.2383508164773));
#147084=CARTESIAN_POINT('Ctrl Pts',(0.602509352318679,6.9874692839556,56.2462013212495));
#147085=CARTESIAN_POINT('Ctrl Pts',(0.429289721358449,6.99809523353577,
56.2540518260217));
#147086=CARTESIAN_POINT('Ctrl Pts',(0.256097955977921,7.00871947373551,
56.2619010678951));
#147087=CARTESIAN_POINT('Ctrl Pts',(0.0824858841641347,7.01291161844657,
56.2697503097685));
#147088=CARTESIAN_POINT('Ctrl Pts',(-0.0910123971688293,7.01065926329768,
56.2775995516419));
#147089=CARTESIAN_POINT('Ctrl Pts',(-0.264569133466189,7.00840614928629,
56.2854514380784));
#147090=CARTESIAN_POINT('Ctrl Pts',(-0.438011620873844,6.99970420337629,
56.2933033245149));
#147091=CARTESIAN_POINT('Ctrl Pts',(-0.610806899742382,6.98459315162502,
56.3011552109514));
#147092=CARTESIAN_POINT('Ctrl Pts',(-0.737688319046612,6.97349729468995,
56.3069207532845));
#147093=CARTESIAN_POINT('Ctrl Pts',(-0.864220788215814,6.95894687722375,
56.3126862956176));
#147094=CARTESIAN_POINT('Ctrl Pts',(-0.990195679420402,6.94097536942447,
56.3184518379507));
#147095=CARTESIAN_POINT('Ctrl Pts',(-1.20116038014341,6.91087926274668,
56.328107142283));
#147096=CARTESIAN_POINT('Ctrl Pts',(-1.41045364027579,6.87120349826754,
56.3377624466153));
#147097=CARTESIAN_POINT('Ctrl Pts',(-1.61730105857216,6.822167093266,56.3474177509476));
#147098=CARTESIAN_POINT('Ctrl Pts',(-1.8252943727057,6.77285903579315,56.357126543852));
#147099=CARTESIAN_POINT('Ctrl Pts',(-2.03081463764949,6.714086402269,56.3668353367563));
#147100=CARTESIAN_POINT('Ctrl Pts',(-2.23309720570835,6.64611942657951,
56.3765441296607));
#147101=CARTESIAN_POINT('Ctrl Pts',(-2.43635317461807,6.5778253880462,56.3862996420989));
#147102=CARTESIAN_POINT('Ctrl Pts',(-2.63634017815743,6.50024834306042,
56.396055154537));
#147103=CARTESIAN_POINT('Ctrl Pts',(-2.83230581991641,6.41370955882535,
56.4058106669752));
#147104=CARTESIAN_POINT('Ctrl Pts',(-3.02846549780603,6.32708508788166,
56.4155758388714));
#147105=CARTESIAN_POINT('Ctrl Pts',(-3.22059581891455,6.23148115437375,
56.4253410107675));
#147106=CARTESIAN_POINT('Ctrl Pts',(-3.40796591218387,6.12726651157698,
56.4351061826637));
#147107=CARTESIAN_POINT('Ctrl Pts',(-3.59508053060769,6.023193963067,56.4448580399709));
#147108=CARTESIAN_POINT('Ctrl Pts',(-3.77744786015144,5.91053418880033,
56.454609897278));
#147109=CARTESIAN_POINT('Ctrl Pts',(-3.95436413596618,5.78970041044305,
56.4643617545852));
#147110=CARTESIAN_POINT('Ctrl Pts',(-4.03151244816047,5.73700812979566,
56.4686142708025));
#147111=CARTESIAN_POINT('Ctrl Pts',(-4.10762450529992,5.68276207628728,
56.4728667870198));
#147112=CARTESIAN_POINT('Ctrl Pts',(-4.18264341832615,5.62699925338834,
56.4771193032371));
#147113=CARTESIAN_POINT('Ctrl Pts',(-4.3243548941933,5.52166272406854,56.4851523488385));
#147114=CARTESIAN_POINT('Ctrl Pts',(-4.4622325460807,5.41085938963786,56.4931853944399));
#147115=CARTESIAN_POINT('Ctrl Pts',(-4.59582437413559,5.29490555955451,
56.5012184400412));
#147116=CARTESIAN_POINT('Ctrl Pts',(-4.72933032421962,5.17902626905778,
56.5092463216916));
#147117=CARTESIAN_POINT('Ctrl Pts',(-4.85855565887089,5.05800331269003,
56.5172742033419));
#147118=CARTESIAN_POINT('Ctrl Pts',(-4.98307962490636,4.93219464481513,
56.5253020849923));
#147119=CARTESIAN_POINT('Ctrl Pts',(-5.10754736714371,4.80644278079391,
56.5333263419749));
#147120=CARTESIAN_POINT('Ctrl Pts',(-5.22731770999815,4.67590976764803,
56.5413505989576));
#147121=CARTESIAN_POINT('Ctrl Pts',(-5.34200514475477,4.54099191762258,
56.5493748559402));
#147122=CARTESIAN_POINT('Ctrl Pts',(-5.45667871263212,4.40609038053971,
56.5573981427085));
#147123=CARTESIAN_POINT('Ctrl Pts',(-5.56627035338833,4.26680533672825,
56.5654214294767));
#147124=CARTESIAN_POINT('Ctrl Pts',(-5.67043330268262,4.12356796019272,
56.573444716245));
#147125=CARTESIAN_POINT('Ctrl Pts',(-5.77458771675235,3.9803423206825,56.5814673455764));
#147126=CARTESIAN_POINT('Ctrl Pts',(-5.87331411303707,3.83316529243472,
56.5894899749079));
#147127=CARTESIAN_POINT('Ctrl Pts',(-5.96630789651182,3.68249869606504,
56.5975126042393));
#147128=CARTESIAN_POINT('Ctrl Pts',(-6.05933663902847,3.53177545978182,
56.6055382495082));
#147129=CARTESIAN_POINT('Ctrl Pts',(-6.14662827354817,3.37756034850298,
56.6135638947772));
#147130=CARTESIAN_POINT('Ctrl Pts',(-6.22792298894739,3.2203418772299,56.6215895400461));
#147131=CARTESIAN_POINT('Ctrl Pts',(-6.2758593068327,3.12763628647436,56.6263219495386));
#147132=CARTESIAN_POINT('Ctrl Pts',(-6.32171136420164,3.0338868994117,56.631054359031));
#147133=CARTESIAN_POINT('Ctrl Pts',(-6.36543360472109,2.93919743916387,
56.6357867685235));
#147134=CARTESIAN_POINT('Ctrl Pts',(-6.44608962056194,2.76452032941438,
56.6445168173604));
#147135=CARTESIAN_POINT('Ctrl Pts',(-6.51953573015837,2.58655576663999,
56.6532468661973));
#147136=CARTESIAN_POINT('Ctrl Pts',(-6.58553315998018,2.40590514387029,
56.6619769150341));
#147137=CARTESIAN_POINT('Ctrl Pts',(-6.65154967304157,2.22520228574651,
56.6707094881756));
#147138=CARTESIAN_POINT('Ctrl Pts',(-6.71011311323383,2.04181207464561,
56.679442061317));
#147139=CARTESIAN_POINT('Ctrl Pts',(-6.76103393689184,1.85635305550881,
56.6881746344584));
#147140=CARTESIAN_POINT('Ctrl Pts',(-6.81267817211495,1.66825929502929,
56.6970312677377));
#147141=CARTESIAN_POINT('Ctrl Pts',(-6.85646090792406,1.47803777657233,
56.705887901017));
#147142=CARTESIAN_POINT('Ctrl Pts',(-6.89223750002692,1.28634707825015,
56.7147445342963));
#147143=CARTESIAN_POINT('Ctrl Pts',(-6.92753540368285,1.09722118885126,
56.7234826664054));
#147144=CARTESIAN_POINT('Ctrl Pts',(-6.95504004827874,0.906665467779782,
56.7322207985145));
#147145=CARTESIAN_POINT('Ctrl Pts',(-6.97466431412637,0.715321094161304,
56.7409589306236));
#147146=CARTESIAN_POINT('Ctrl Pts',(-6.99468777829888,0.520084378581257,
56.749874814488));
#147147=CARTESIAN_POINT('Ctrl Pts',(-7.00650678903345,0.324026875386856,
56.7587906983524));
#147148=CARTESIAN_POINT('Ctrl Pts',(-7.01008451422468,0.127834525568464,
56.7677065822168));
#147149=CARTESIAN_POINT('Ctrl Pts',(-7.01366223941591,-0.0683578242499944,
56.7766224660812));
#147150=CARTESIAN_POINT('Ctrl Pts',(-7.00899867963198,-0.2646847182196,
56.7855383499456));
#147151=CARTESIAN_POINT('Ctrl Pts',(-6.99611344218485,-0.460459842527483,
56.79445423381));
#147152=CARTESIAN_POINT('Ctrl Pts',(-6.98348140291007,-0.652387936164065,
56.8031949183031));
#147153=CARTESIAN_POINT('Ctrl Pts',(-6.96294646113462,-0.843806128364029,
56.8119356027962));
#147154=CARTESIAN_POINT('Ctrl Pts',(-6.93457453531067,-1.0340708760626,
56.8206762872894));
#147155=CARTESIAN_POINT('Ctrl Pts',(-6.90620771406765,-1.22430139197131,
56.8294153991881));
#147156=CARTESIAN_POINT('Ctrl Pts',(-6.87000676502785,-1.41337860711619,
56.8381545110868));
#147157=CARTESIAN_POINT('Ctrl Pts',(-6.82608918743713,-1.60066641360838,
56.8468936229856));
#147158=CARTESIAN_POINT('Ctrl Pts',(-6.78160259439649,-1.79038080328941,
56.8557459626615));
#147159=CARTESIAN_POINT('Ctrl Pts',(-6.72919806200088,-1.9782588097309,
56.8645983023374));
#147160=CARTESIAN_POINT('Ctrl Pts',(-6.66905099348429,-2.16365094430831,
56.8734506420133));
#147161=CARTESIAN_POINT('Ctrl Pts',(-6.60970368333869,-2.34657797268516,
56.8821852746598));
#147162=CARTESIAN_POINT('Ctrl Pts',(-6.54281855888771,-2.5270845635597,
56.8909199073064));
#147163=CARTESIAN_POINT('Ctrl Pts',(-6.46861428828942,-2.70456202588107,
56.899654539953));
#147164=CARTESIAN_POINT('Ctrl Pts',(-6.39291006378181,-2.88562699079874,
56.9085657331435));
#147165=CARTESIAN_POINT('Ctrl Pts',(-6.30958773748115,-3.06353878594618,
56.9174769263341));
#147166=CARTESIAN_POINT('Ctrl Pts',(-6.21893156124203,-3.23767150882972,
56.9263881195247));
#147167=CARTESIAN_POINT('Ctrl Pts',(-6.12827538500291,-3.41180423171327,
56.9352993127153));
#147168=CARTESIAN_POINT('Ctrl Pts',(-6.03028548685395,-3.58215760723677,
56.9442105059059));
#147169=CARTESIAN_POINT('Ctrl Pts',(-5.92529694580897,-3.74813055622226,
56.9531216990964));
#147170=CARTESIAN_POINT('Ctrl Pts',(-5.83074138788335,-3.89761034359408,
56.9611473639502));
#147171=CARTESIAN_POINT('Ctrl Pts',(-5.73046512865698,-4.04360545461279,
56.9691730288041));
#147172=CARTESIAN_POINT('Ctrl Pts',(-5.62476393444491,-4.18564896333506,
56.9771986936579));
#147173=CARTESIAN_POINT('Ctrl Pts',(-5.51909628719897,-4.32764739093205,
56.9852218113625));
#147174=CARTESIAN_POINT('Ctrl Pts',(-5.40800735137135,-4.46569641937993,
56.9932449290672));
#147175=CARTESIAN_POINT('Ctrl Pts',(-5.29183575164625,-4.59935875314142,
57.0012680467719));
#147176=CARTESIAN_POINT('Ctrl Pts',(-5.17567880217664,-4.73300423091277,
57.0092901526912));
#147177=CARTESIAN_POINT('Ctrl Pts',(-5.05444070639232,-4.86226383970237,
57.0173122586105));
#147178=CARTESIAN_POINT('Ctrl Pts',(-4.92849980263377,-4.98673402719044,
57.0253343645298));
#147179=CARTESIAN_POINT('Ctrl Pts',(-4.80251209880957,-5.11125046822101,
57.0333594514908));
#147180=CARTESIAN_POINT('Ctrl Pts',(-4.67181835475729,-5.23097367248907,
57.0413845384518));
#147181=CARTESIAN_POINT('Ctrl Pts',(-4.53683346077818,-5.34553727062711,
57.0494096254128));
#147182=CARTESIAN_POINT('Ctrl Pts',(-4.40182198219965,-5.46012343149254,
57.0574362928745));
#147183=CARTESIAN_POINT('Ctrl Pts',(-4.26251795525101,-5.56954773139381,
57.0654629603362));
#147184=CARTESIAN_POINT('Ctrl Pts',(-4.11936847988045,-5.67348481001469,
57.0734896277979));
#147185=CARTESIAN_POINT('Ctrl Pts',(-3.97610408461541,-5.77750532895611,
57.08152273904));
#147186=CARTESIAN_POINT('Ctrl Pts',(-3.82898837722223,-5.87602962067472,
57.089555850282));
#147187=CARTESIAN_POINT('Ctrl Pts',(-3.67849700825313,-5.96877594844813,
57.0975889615241));
#147188=CARTESIAN_POINT('Ctrl Pts',(-3.58982202693959,-6.02342545385527,
57.102322362477));
#147189=CARTESIAN_POINT('Ctrl Pts',(-3.49997551423724,-6.07606970813474,
57.1070557634299));
#147190=CARTESIAN_POINT('Ctrl Pts',(-3.40905855337498,-6.12665866049031,
57.1117891643827));
#147191=CARTESIAN_POINT('Ctrl Pts',(-3.22176678416488,-6.23087347694808,
57.1215401176751));
#147192=CARTESIAN_POINT('Ctrl Pts',(-3.02982105839677,-6.32642565514109,
57.1312910709674));
#147193=CARTESIAN_POINT('Ctrl Pts',(-2.83396501958068,-6.41297659673674,
57.1410420242597));
#147194=CARTESIAN_POINT('Ctrl Pts',(-2.6378268134008,-6.49965223119951,
57.1508070256294));
#147195=CARTESIAN_POINT('Ctrl Pts',(-2.43776706077307,-6.57730067369326,
57.160572026999));
#147196=CARTESIAN_POINT('Ctrl Pts',(-2.23455086245205,-6.64563082074342,
57.1703370283687));
#147197=CARTESIAN_POINT('Ctrl Pts',(-2.03167338342854,-6.71384707559601,
57.1800857535044));
#147198=CARTESIAN_POINT('Ctrl Pts',(-1.82565000952821,-6.77277606441918,
57.18983447864));
#147199=CARTESIAN_POINT('Ctrl Pts',(-1.61725958615924,-6.82217692481484,
57.1995832037756));
#147200=CARTESIAN_POINT('Ctrl Pts',(-1.40944111369837,-6.87144219900405,
57.2093051724409));
#147201=CARTESIAN_POINT('Ctrl Pts',(-1.19926860009142,-6.91123154178717,
57.2190271411061));
#147202=CARTESIAN_POINT('Ctrl Pts',(-0.987531454857761,-6.94135492452061,
57.2287491097713));
#147203=CARTESIAN_POINT('Ctrl Pts',(-0.777195319008167,-6.97127898869877,
57.2384067507093));
#147204=CARTESIAN_POINT('Ctrl Pts',(-0.565315230750769,-6.99166454913837,
57.2480643916473));
#147205=CARTESIAN_POINT('Ctrl Pts',(-0.352681222158356,-7.00237406299013,
57.2577220325852));
#147206=CARTESIAN_POINT('Ctrl Pts',(-0.259221254615671,-7.00708126304533,
57.2619668982799));
#147207=CARTESIAN_POINT('Ctrl Pts',(-0.165615844256471,-7.00991978170583,
57.2662117639746));
#147208=CARTESIAN_POINT('Ctrl Pts',(-0.0719330421756044,-7.01088098600621,
57.2704566296693));
#147209=CARTESIAN_POINT('Ctrl Pts',(0.101354661770682,-7.01265895253301,
57.2783084766835));
#147210=CARTESIAN_POINT('Ctrl Pts',(0.274836025498248,-7.00800916941368,
57.2861603236976));
#147211=CARTESIAN_POINT('Ctrl Pts',(0.44797733170565,-6.99692381499026,
57.2940121707118));
#147212=CARTESIAN_POINT('Ctrl Pts',(0.621069536438241,-6.98584160428375,
57.3018617910056));
#147213=CARTESIAN_POINT('Ctrl Pts',(0.793821495172513,-6.96832747701064,
57.3097114112994));
#147214=CARTESIAN_POINT('Ctrl Pts',(0.965700916892863,-6.94442569991301,
57.3175610315932));
#147215=CARTESIAN_POINT('Ctrl Pts',(1.13756661623999,-6.92052583106654,
57.3254100251952));
#147216=CARTESIAN_POINT('Ctrl Pts',(1.30855953952385,-6.89023938089365,
57.3332590187973));
#147217=CARTESIAN_POINT('Ctrl Pts',(1.47815419782025,-6.85366228595825,
57.3411080123993));
#147218=CARTESIAN_POINT('Ctrl Pts',(1.64783471692615,-6.81706667311071,
57.348960979717));
#147219=CARTESIAN_POINT('Ctrl Pts',(1.81611518324735,-6.77417413269953,
57.3568139470346));
#147220=CARTESIAN_POINT('Ctrl Pts',(1.98248162466146,-6.72513146119685,
57.3646669143523));
#147221=CARTESIAN_POINT('Ctrl Pts',(2.14889031756157,-6.67607633450351,
57.3725218760598));
#147222=CARTESIAN_POINT('Ctrl Pts',(2.31338365545163,-6.62086808638544,
57.3803768377673));
#147223=CARTESIAN_POINT('Ctrl Pts',(2.47546507066133,-6.55970267972838,
57.3882317994748));
#147224=CARTESIAN_POINT('Ctrl Pts',(2.63770736522403,-6.49847656129239,
57.3960945578884));
#147225=CARTESIAN_POINT('Ctrl Pts',(2.79753260411244,-6.43128162237353,
57.403957316302));
#147226=CARTESIAN_POINT('Ctrl Pts',(2.95446583461559,-6.35836128216927,
57.4118200747156));
#147227=CARTESIAN_POINT('Ctrl Pts',(3.06958980062205,-6.30486796695527,
57.4175880814622));
#147228=CARTESIAN_POINT('Ctrl Pts',(3.18315789980236,-6.24829452918601,
57.4233560882089));
#147229=CARTESIAN_POINT('Ctrl Pts',(3.29499208989736,-6.18875219167918,
57.4291240949556));
#147230=CARTESIAN_POINT('Ctrl Pts',(3.45743196144031,-6.10226656820607,
57.4375021613966));
#147231=CARTESIAN_POINT('Ctrl Pts',(3.61657259156186,-6.00932420993033,
57.4458802278377));
#147232=CARTESIAN_POINT('Ctrl Pts',(3.77188826441528,-5.91020181408946,
57.4542582942787));
#147233=CARTESIAN_POINT('Ctrl Pts',(3.92709773425678,-5.81114719696528,
57.4626306318974));
#147234=CARTESIAN_POINT('Ctrl Pts',(4.07848718506613,-5.70592114362543,
57.4710029695161));
#147235=CARTESIAN_POINT('Ctrl Pts',(4.22555676910864,-5.59484553437717,
57.4793753071348));
#147236=CARTESIAN_POINT('Ctrl Pts',(4.37254735656861,-5.48382958799933,
57.4877431476573));
#147237=CARTESIAN_POINT('Ctrl Pts',(4.51522244211506,-5.36697054826797,
57.4961109881799));
#147238=CARTESIAN_POINT('Ctrl Pts',(4.65311199744705,-5.24463299971641,
57.5044788287024));
#147239=CARTESIAN_POINT('Ctrl Pts',(4.79094768695342,-5.12234324168127,
57.5128434003724));
#147240=CARTESIAN_POINT('Ctrl Pts',(4.92400132865464,-4.99457946042438,
57.5212079720423));
#147241=CARTESIAN_POINT('Ctrl Pts',(5.05183642380995,-4.86174611734993,
57.5295725437122));
#147242=CARTESIAN_POINT('Ctrl Pts',(5.17964029283286,-4.72894522132418,
57.5379350721777));
#147243=CARTESIAN_POINT('Ctrl Pts',(5.30222793002041,-4.5910774699408,57.5462976006433));
#147244=CARTESIAN_POINT('Ctrl Pts',(5.41919980444543,-4.44858404911031,
57.5546601291088));
#147245=CARTESIAN_POINT('Ctrl Pts',(5.53618101359193,-4.3060792568591,57.5630233249303));
#147246=CARTESIAN_POINT('Ctrl Pts',(5.64754535141674,-4.15894830787069,
57.5713865207518));
#147247=CARTESIAN_POINT('Ctrl Pts',(5.75293320475518,-4.00766591722979,
57.5797497165733));
#147248=CARTESIAN_POINT('Ctrl Pts',(5.8583282453339,-3.85637320943319,57.588113482748));
#147249=CARTESIAN_POINT('Ctrl Pts',(5.95774580056145,-3.70092876512131,
57.5964772489227));
#147250=CARTESIAN_POINT('Ctrl Pts',(6.05086918737543,-3.54183690191554,
57.6048410150973));
#147251=CARTESIAN_POINT('Ctrl Pts',(6.14401134055583,-3.38271297827572,
57.6132064667509));
#147252=CARTESIAN_POINT('Ctrl Pts',(6.23085663000172,-3.21994045382377,
57.6215719184044));
#147253=CARTESIAN_POINT('Ctrl Pts',(6.31113378383685,-3.05404926695905,
57.629937370058));
#147254=CARTESIAN_POINT('Ctrl Pts',(6.39143782233269,-2.88810252346259,
57.6383056232848));
#147255=CARTESIAN_POINT('Ctrl Pts',(6.46516919588372,-2.71903533075755,
57.6466738765116));
#147256=CARTESIAN_POINT('Ctrl Pts',(6.53210414895704,-2.5473990558368,57.6550421297385));
#147257=CARTESIAN_POINT('Ctrl Pts',(6.59910116028132,-2.37560364960222,
57.6634181415299));
#147258=CARTESIAN_POINT('Ctrl Pts',(6.65928903976748,-2.20123470802503,
57.6717941533214));
#147259=CARTESIAN_POINT('Ctrl Pts',(6.71249303090066,-2.02486144528707,
57.6801701651128));
#147260=CARTESIAN_POINT('Ctrl Pts',(6.76572311392852,-1.8484016869217,57.6885502846039));
#147261=CARTESIAN_POINT('Ctrl Pts',(6.81196238989097,-1.66993596367686,
57.6969304040951));
#147262=CARTESIAN_POINT('Ctrl Pts',(6.85108676488036,-1.49004587264327,
57.7053105235862));
#147263=CARTESIAN_POINT('Ctrl Pts',(6.8902558444242,-1.30995023439335,57.7137002184254));
#147264=CARTESIAN_POINT('Ctrl Pts',(6.92229371470968,-1.12842729894076,
57.7220899132646));
#147265=CARTESIAN_POINT('Ctrl Pts',(6.94712769003129,-0.946067344801934,
57.7304796081038));
#147266=CARTESIAN_POINT('Ctrl Pts',(6.96289435241049,-0.83029015685037,
57.7358060805787));
#147267=CARTESIAN_POINT('Ctrl Pts',(6.97575834093414,-0.714175705115564,
57.7411325530537));
#147268=CARTESIAN_POINT('Ctrl Pts',(6.98571194797933,-0.597875524134276,
57.7464590255286));
#147269=CARTESIAN_POINT('Ctrl Pts',(7.00257721922354,-0.400817905816182,
57.7554841359893));
#147270=CARTESIAN_POINT('Ctrl Pts',(7.01111079365633,-0.202955311594732,
57.7645092464499));
#147271=CARTESIAN_POINT('Ctrl Pts',(7.01124831048953,-0.00486735633776691,
57.7735343569105));
#147272=CARTESIAN_POINT('Ctrl Pts',(7.01124831048998,-0.00486735569163166,
57.7735343569399));
#147273=CARTESIAN_POINT('Ctrl Pts',(7.01137216007327,0.173533450955664,
57.7816624987251));
#147274=CARTESIAN_POINT('Ctrl Pts',(7.00468277305869,0.352181946036952,
57.7897906405102));
#147275=CARTESIAN_POINT('Ctrl Pts',(6.9911500422492,0.530516398671202,57.7979187822954));
#147276=CARTESIAN_POINT('Ctrl Pts',(6.97763572442698,0.708608204787677,
57.8060358647183));
#147277=CARTESIAN_POINT('Ctrl Pts',(6.9572966460282,0.886386467559613,57.8141529471413));
#147278=CARTESIAN_POINT('Ctrl Pts',(6.93015469145915,1.06328853795513,57.8222700295642));
#147279=CARTESIAN_POINT('Ctrl Pts',(6.90303402361234,1.24005186870217,57.8303807459726));
#147280=CARTESIAN_POINT('Ctrl Pts',(6.86912115405176,1.41594002501076,57.838491462381));
#147281=CARTESIAN_POINT('Ctrl Pts',(6.82848988511768,1.59039380385664,57.8466021787894));
#147282=CARTESIAN_POINT('Ctrl Pts',(6.78788803830109,1.76472125636045,57.8547070220252));
#147283=CARTESIAN_POINT('Ctrl Pts',(6.74057756546112,1.93761605511888,57.8628118652611));
#147284=CARTESIAN_POINT('Ctrl Pts',(6.68668361174142,2.10852764719099,57.870916708497));
#147285=CARTESIAN_POINT('Ctrl Pts',(6.65102377983819,2.22161414804974,57.8762794129832));
#147286=CARTESIAN_POINT('Ctrl Pts',(6.61248274091082,2.33383255763744,57.8816421174695));
#147287=CARTESIAN_POINT('Ctrl Pts',(6.57110895151813,2.44502632087639,57.8870048219557));
#147288=CARTESIAN_POINT('',(7.01124998181045,-0.000505037546988676,57.2264656430896));
#147289=CARTESIAN_POINT('Ctrl Pts',(6.57110895151816,2.4450263208763,57.3398522865015));
#147290=CARTESIAN_POINT('Ctrl Pts',(6.63771924680899,2.266008408508,57.3311805125693));
#147291=CARTESIAN_POINT('Ctrl Pts',(6.69700989700473,2.08426710051955,57.3225087386372));
#147292=CARTESIAN_POINT('Ctrl Pts',(6.74878307789422,1.90040877971785,57.3138369647051));
#147293=CARTESIAN_POINT('Ctrl Pts',(6.80055978789531,1.71653792623954,57.3051645996628));
#147294=CARTESIAN_POINT('Ctrl Pts',(6.84481792613573,1.53055004459453,57.2964922346204));
#147295=CARTESIAN_POINT('Ctrl Pts',(6.88140980451098,1.3430657708691,57.2878198695781));
#147296=CARTESIAN_POINT('Ctrl Pts',(6.91799949925383,1.15559268532943,57.2791480220619));
#147297=CARTESIAN_POINT('Ctrl Pts',(6.94692379517689,0.966623665170781,
57.2704761745458));
#147298=CARTESIAN_POINT('Ctrl Pts',(6.96808618426389,0.776789219267855,
57.2618043270297));
#147299=CARTESIAN_POINT('Ctrl Pts',(6.98924897510677,0.586951169466182,
57.2531323148835));
#147300=CARTESIAN_POINT('Ctrl Pts',(7.00264953276857,0.396247943319445,
57.2444603027373));
#147301=CARTESIAN_POINT('Ctrl Pts',(7.00824314361839,0.205315860142146,
57.2357882905911));
#147302=CARTESIAN_POINT('Ctrl Pts',(7.01024757124657,0.136896809746564,
57.2326807414239));
#147303=CARTESIAN_POINT('Ctrl Pts',(7.01125,0.0684484052929644,57.2295731922568));
#147304=CARTESIAN_POINT('Ctrl Pts',(7.01125,8.58630487052188E-16,57.2264656430896));
#147305=CARTESIAN_POINT('Ctrl Pts',(7.01124998181045,-0.000505037546988675,
57.2264656430896));
#147306=CARTESIAN_POINT('Ctrl Pts',(7.01123724491756,-0.177326623645792,
57.2184554091803));
#147307=CARTESIAN_POINT('Ctrl Pts',(7.00453108466972,-0.354163812240794,
57.2104451752711));
#147308=CARTESIAN_POINT('Ctrl Pts',(6.99115392040837,-0.530465289777442,
57.2024349413618));
#147309=CARTESIAN_POINT('Ctrl Pts',(6.97777149517461,-0.706836103175747,
57.194421557187));
#147310=CARTESIAN_POINT('Ctrl Pts',(6.957712851468,-0.882670417579134,57.1864081730122));
#147311=CARTESIAN_POINT('Ctrl Pts',(6.93105236669831,-1.05742122760315,
57.1783947888374));
#147312=CARTESIAN_POINT('Ctrl Pts',(6.90438587943545,-1.23221138201846,
57.1703796004837));
#147313=CARTESIAN_POINT('Ctrl Pts',(6.8711146549574,-1.40591718416178,57.16236441213));
#147314=CARTESIAN_POINT('Ctrl Pts',(6.83136423261756,-1.57800167421124,
57.1543492237764));
#147315=CARTESIAN_POINT('Ctrl Pts',(6.79158278043253,-1.75022049629471,
57.1463277786324));
#147316=CARTESIAN_POINT('Ctrl Pts',(6.74531212406688,-1.92081512357284,
57.1383063334885));
#147317=CARTESIAN_POINT('Ctrl Pts',(6.69272786200115,-2.08926310638309,
57.1302848883446));
#147318=CARTESIAN_POINT('Ctrl Pts',(6.6708820426386,-2.15924382038188,57.1269524266012));
#147319=CARTESIAN_POINT('Ctrl Pts',(6.64794711619884,-2.22885425457659,
57.1236199648578));
#147320=CARTESIAN_POINT('Ctrl Pts',(6.62393811561288,-2.29805796337492,
57.1202875031143));
#147321=CARTESIAN_POINT('Ctrl Pts',(6.55368655366752,-2.50055154981511,
57.1105365498516));
#147322=CARTESIAN_POINT('Ctrl Pts',(6.47419318465181,-2.69968513413424,
57.1007855965888));
#147323=CARTESIAN_POINT('Ctrl Pts',(6.3857870322112,-2.89471078723649,57.0910346433261));
#147324=CARTESIAN_POINT('Ctrl Pts',(6.29725351413347,-3.09001741135576,
57.0812696419871));
#147325=CARTESIAN_POINT('Ctrl Pts',(6.19978154373158,-3.28120423083926,
57.071504640648));
#147326=CARTESIAN_POINT('Ctrl Pts',(6.09374778772134,-3.467544442706,57.061739639309));
#147327=CARTESIAN_POINT('Ctrl Pts',(5.98789076800703,-3.65357406405831,
57.0519909142034));
#147328=CARTESIAN_POINT('Ctrl Pts',(5.87350050281105,-3.83477319006731,
57.0422421890978));
#147329=CARTESIAN_POINT('Ctrl Pts',(5.75099737952567,-4.01044333000591,
57.0324934639922));
#147330=CARTESIAN_POINT('Ctrl Pts',(5.62883047979592,-4.18563132355114,
57.0227714953556));
#147331=CARTESIAN_POINT('Ctrl Pts',(5.49859519654304,-4.35532059252179,
57.013049526719));
#147332=CARTESIAN_POINT('Ctrl Pts',(5.36075366068567,-4.51884351930283,
57.0033275580824));
#147333=CARTESIAN_POINT('Ctrl Pts',(5.22382418622545,-4.68128445763867,
56.9936699171699));
#147334=CARTESIAN_POINT('Ctrl Pts',(5.07938879163111,-4.83764033191866,
56.9840122762575));
#147335=CARTESIAN_POINT('Ctrl Pts',(4.92794503770073,-4.98728225268039,
56.974354635345));
#147336=CARTESIAN_POINT('Ctrl Pts',(4.86138029135914,-5.0530550312801,56.970109769506));
#147337=CARTESIAN_POINT('Ctrl Pts',(4.79346217679016,-5.11753107602661,
56.9658649036669));
#147338=CARTESIAN_POINT('Ctrl Pts',(4.72423569398403,-5.18065861355361,
56.9616200378279));
#147339=CARTESIAN_POINT('Ctrl Pts',(4.59618553305735,-5.29742738486149,
56.9537681907924));
#147340=CARTESIAN_POINT('Ctrl Pts',(4.46370883211363,-5.40953147895155,
56.9459163437568));
#147341=CARTESIAN_POINT('Ctrl Pts',(4.32719841650096,-5.51660950464428,
56.9380644967213));
#147342=CARTESIAN_POINT('Ctrl Pts',(4.19072671413717,-5.62365716387566,
56.930214876406));
#147343=CARTESIAN_POINT('Ctrl Pts',(4.05022387242283,-5.7256813547798,56.9223652560908));
#147344=CARTESIAN_POINT('Ctrl Pts',(3.90611635385955,-5.82236048288072,
56.9145156357755));
#147345=CARTESIAN_POINT('Ctrl Pts',(3.76202034043703,-5.91903189239077,
56.9066666421519));
#147346=CARTESIAN_POINT('Ctrl Pts',(3.61432054026825,-6.01035887671013,
56.8988176485283));
#147347=CARTESIAN_POINT('Ctrl Pts',(3.46347276498308,-6.09606290721483,
56.8909686549048));
#147348=CARTESIAN_POINT('Ctrl Pts',(3.31254861988543,-6.18181032716113,
56.8831156875655));
#147349=CARTESIAN_POINT('Ctrl Pts',(3.15847364742723,-6.26192891668545,
56.8752627202263));
#147350=CARTESIAN_POINT('Ctrl Pts',(3.00172895266888,-6.33618574989791,
56.867409752887));
#147351=CARTESIAN_POINT('Ctrl Pts',(2.8449444500238,-6.41046144185141,56.8595547911578));
#147352=CARTESIAN_POINT('Ctrl Pts',(2.68548922490902,-6.47887226125682,
56.8516998294287));
#147353=CARTESIAN_POINT('Ctrl Pts',(2.52386415672786,-6.54123354428539,
56.8438448676995));
#147354=CARTESIAN_POINT('Ctrl Pts',(2.36207866215702,-6.60365672609986,
56.8359821092643));
#147355=CARTESIAN_POINT('Ctrl Pts',(2.1981193835196,-6.66001825472769,56.8281193508291));
#147356=CARTESIAN_POINT('Ctrl Pts',(2.03250269519127,-6.71018325804447,
56.8202565923939));
#147357=CARTESIAN_POINT('Ctrl Pts',(1.91100867218322,-6.74698358371626,
56.8144885857764));
#147358=CARTESIAN_POINT('Ctrl Pts',(1.78862303317405,-6.7804503082767,56.808720579159));
#147359=CARTESIAN_POINT('Ctrl Pts',(1.66555265432867,-6.81054776931773,
56.8029525725415));
#147360=CARTESIAN_POINT('Ctrl Pts',(1.48679214367329,-6.85426452354895,
56.7945745061208));
#147361=CARTESIAN_POINT('Ctrl Pts',(1.30619072169333,-6.8909680429163,56.7861964397));
#147362=CARTESIAN_POINT('Ctrl Pts',(1.12432479047456,-6.92051445544508,
56.7778183732792));
#147363=CARTESIAN_POINT('Ctrl Pts',(0.942583217022785,-6.95004066448738,
56.7694460356809));
#147364=CARTESIAN_POINT('Ctrl Pts',(0.759579181637139,-6.97241947122276,
56.7610736980826));
#147365=CARTESIAN_POINT('Ctrl Pts',(0.575899895042257,-6.98755793345503,
56.7527013604843));
#147366=CARTESIAN_POINT('Ctrl Pts',(0.392319269475441,-7.00268826425194,
56.7443335199822));
#147367=CARTESIAN_POINT('Ctrl Pts',(0.208064442775255,-7.01058597802294,
56.7359656794802));
#147368=CARTESIAN_POINT('Ctrl Pts',(0.0237288361009822,-7.01120984601355,
56.7275978389782));
#147369=CARTESIAN_POINT('Ctrl Pts',(-0.160534760840535,-7.01183347029341,
56.7192332673289));
#147370=CARTESIAN_POINT('Ctrl Pts',(-0.344878746602167,-7.00518891401741,
56.7108686956796));
#147371=CARTESIAN_POINT('Ctrl Pts',(-0.528708140090684,-6.99128702494053,
56.7025041240303));
#147372=CARTESIAN_POINT('Ctrl Pts',(-0.712492629783648,-6.97738853166219,
56.6941415955854));
#147373=CARTESIAN_POINT('Ctrl Pts',(-0.89576245044932,-6.9562362660491,
56.6857790671405));
#147374=CARTESIAN_POINT('Ctrl Pts',(-1.07792572532216,-6.92789309192836,
56.6774165386956));
#147375=CARTESIAN_POINT('Ctrl Pts',(-1.26010353739538,-6.89954765593348,
56.6690533428946));
#147376=CARTESIAN_POINT('Ctrl Pts',(-1.44117430156223,-6.86401020950662,
56.6606901470937));
#147377=CARTESIAN_POINT('Ctrl Pts',(-1.62055357410303,-6.82139521476083,
56.6523269512928));
#147378=CARTESIAN_POINT('Ctrl Pts',(-1.79994507995217,-6.77877731375746,
56.6439631851387));
#147379=CARTESIAN_POINT('Ctrl Pts',(-1.97764454418465,-6.72908097776443,
56.6355994189845));
#147380=CARTESIAN_POINT('Ctrl Pts',(-2.15307981856414,-6.67247134556544,
56.6272356528303));
#147381=CARTESIAN_POINT('Ctrl Pts',(-2.32855044692903,-6.6158503053066,
56.6188702011972));
#147382=CARTESIAN_POINT('Ctrl Pts',(-2.50175566270643,-6.55231329178988,
56.610504749564));
#147383=CARTESIAN_POINT('Ctrl Pts',(-2.67214011610176,-6.48207480382784,
56.6021392979309));
#147384=CARTESIAN_POINT('Ctrl Pts',(-2.84258163091896,-6.41181279313286,
56.5937710447243));
#147385=CARTESIAN_POINT('Ctrl Pts',(-3.01020019581222,-6.33484495803051,
56.5854027915176));
#147386=CARTESIAN_POINT('Ctrl Pts',(-3.17446162221211,-6.25143343334971,
56.577034538311));
#147387=CARTESIAN_POINT('Ctrl Pts',(-3.33887534239639,-6.16794457428167,
56.5686585265394));
#147388=CARTESIAN_POINT('Ctrl Pts',(-3.49992541083501,-6.07800023637808,
56.5602825147678));
#147389=CARTESIAN_POINT('Ctrl Pts',(-3.65710229183514,-5.98190850728713,
56.5519065029962));
#147390=CARTESIAN_POINT('Ctrl Pts',(-3.81435625432398,-5.88576965362237,
56.5435263835248));
#147391=CARTESIAN_POINT('Ctrl Pts',(-3.96773296456334,-5.78347757372875,
56.5351462640533));
#147392=CARTESIAN_POINT('Ctrl Pts',(-4.11675242066685,-5.67538334118795,
56.5267661445818));
#147393=CARTESIAN_POINT('Ctrl Pts',(-4.26594215038535,-5.56716559728684,
56.5183764497617));
#147394=CARTESIAN_POINT('Ctrl Pts',(-4.41076441511358,-5.45313265159622,
56.5099867549417));
#147395=CARTESIAN_POINT('Ctrl Pts',(-4.55077176871854,-5.33367629984557,
56.5015970601216));
#147396=CARTESIAN_POINT('Ctrl Pts',(-4.63966002571034,-5.25783551991287,
56.496270587404));
#147397=CARTESIAN_POINT('Ctrl Pts',(-4.72660820663073,-5.17980947826596,
56.4909441146863));
#147398=CARTESIAN_POINT('Ctrl Pts',(-4.81150961224631,-5.09970605170155,
56.4856176419687));
#147399=CARTESIAN_POINT('Ctrl Pts',(-4.94510349810382,-4.97366187201275,
56.4772363415284));
#147400=CARTESIAN_POINT('Ctrl Pts',(-5.0738972911768,-4.84221812688308,
56.4688550410881));
#147401=CARTESIAN_POINT('Ctrl Pts',(-5.19744339804855,-4.70576334791514,
56.4604737406478));
#147402=CARTESIAN_POINT('Ctrl Pts',(-5.32083292830701,-4.5694815054136,
56.4521030622795));
#147403=CARTESIAN_POINT('Ctrl Pts',(-5.43898780833956,-4.42820152638251,
56.4437323839112));
#147404=CARTESIAN_POINT('Ctrl Pts',(-5.55149553377463,-4.28235027770737,
56.4353617055429));
#147405=CARTESIAN_POINT('Ctrl Pts',(-5.66387558224888,-4.13666454516981,
56.4270005264581));
#147406=CARTESIAN_POINT('Ctrl Pts',(-5.77062105016662,-3.98641814031486,
56.4186393473732));
#147407=CARTESIAN_POINT('Ctrl Pts',(-5.87135786437864,-3.83207298872284,
56.4102781682883));
#147408=CARTESIAN_POINT('Ctrl Pts',(-5.97196396067764,-3.67792811819247,
56.4019278388208));
#147409=CARTESIAN_POINT('Ctrl Pts',(-6.06657677685428,-3.51969538253832,
56.3935775093532));
#147410=CARTESIAN_POINT('Ctrl Pts',(-6.15486398766265,-3.35786775437531,
56.3852271798856));
#147411=CARTESIAN_POINT('Ctrl Pts',(-6.24308326673597,-3.1961646429057,
56.3768832754977));
#147412=CARTESIAN_POINT('Ctrl Pts',(-6.32498648358142,-3.03087243757995,
56.3685393711099));
#147413=CARTESIAN_POINT('Ctrl Pts',(-6.40028532324032,-2.86251189405645,
56.360195466722));
#147414=CARTESIAN_POINT('Ctrl Pts',(-6.47552368239123,-2.69428657879464,
56.3518582642114));
#147415=CARTESIAN_POINT('Ctrl Pts',(-6.54416811039554,-2.52299813867956,
56.3435210617007));
#147416=CARTESIAN_POINT('Ctrl Pts',(-6.60597677508422,-2.34919079888117,
56.3351838591901));
#147417=CARTESIAN_POINT('Ctrl Pts',(-6.62632384476534,-2.29197438639628,
56.3324392983541));
#147418=CARTESIAN_POINT('Ctrl Pts',(-6.64593050863622,-2.2344851838378,
56.3296947375181));
#147419=CARTESIAN_POINT('Ctrl Pts',(-6.66478926863333,-2.17674311006374,
56.3269501766821));
#147420=CARTESIAN_POINT('Ctrl Pts',(-6.72208447980906,-2.00131565295013,
56.3186118663845));
#147421=CARTESIAN_POINT('Ctrl Pts',(-6.77242574454439,-1.82369680889926,
56.3102735560869));
#147422=CARTESIAN_POINT('Ctrl Pts',(-6.81567017129344,-1.64446546897187,
56.3019352457894));
#147423=CARTESIAN_POINT('Ctrl Pts',(-6.85894180596994,-1.46512136276081,
56.2935916893096));
#147424=CARTESIAN_POINT('Ctrl Pts',(-6.89510761963376,-1.28416305558202,
56.2852481328298));
#147425=CARTESIAN_POINT('Ctrl Pts',(-6.92407593220963,-1.10217922657585,
56.2769045763501));
#147426=CARTESIAN_POINT('Ctrl Pts',(-6.95306628375251,-0.920056945059139,
56.2685546721286));
#147427=CARTESIAN_POINT('Ctrl Pts',(-6.97484816026935,-0.736907908656635,
56.2602047679072));
#147428=CARTESIAN_POINT('Ctrl Pts',(-6.98938172955969,-0.55332594462682,
56.2518548636857));
#147429=CARTESIAN_POINT('Ctrl Pts',(-7.0039370981293,-0.369468621225876,
56.2434924352253));
#147430=CARTESIAN_POINT('Ctrl Pts',(-7.01122240806667,-0.185177399485568,
56.235130006765));
#147431=CARTESIAN_POINT('Ctrl Pts',(-7.01124992172658,-0.00104765881511994,
56.2267675783046));
#147432=CARTESIAN_POINT('Ctrl Pts',(-7.01127745891443,0.183239537890237,
56.2183979988277));
#147433=CARTESIAN_POINT('Ctrl Pts',(-7.00403482928812,0.367364651384708,
56.2100284193507));
#147434=CARTESIAN_POINT('Ctrl Pts',(-6.98958621935857,0.550736819772151,
56.2016588398738));
#147435=CARTESIAN_POINT('Ctrl Pts',(-6.97511532420791,0.734391817396487,
56.1932763513398));
#147436=CARTESIAN_POINT('Ctrl Pts',(-6.95341627750075,0.917291224500392,
56.1848938628059));
#147437=CARTESIAN_POINT('Ctrl Pts',(-6.92460468464367,1.09885236674949,
56.1765113742719));
#147438=CARTESIAN_POINT('Ctrl Pts',(-6.91517705927983,1.15826214802212,
56.1737684866465));
#147439=CARTESIAN_POINT('Ctrl Pts',(-6.90498829125462,1.21752874795626,
56.1710255990212));
#147440=CARTESIAN_POINT('Ctrl Pts',(-6.89404359273626,1.27663209420416,
56.1682827113958));
#147441=CARTESIAN_POINT('Ctrl Pts',(-6.86056630663616,1.45741547791228,
56.1598928563787));
#147442=CARTESIAN_POINT('Ctrl Pts',(-6.81994515962662,1.63703541942779,
56.1515030013616));
#147443=CARTESIAN_POINT('Ctrl Pts',(-6.77227735248947,1.81490661563019,
56.1431131463445));
#147444=CARTESIAN_POINT('Ctrl Pts',(-6.72465353254082,1.99261367477013,
56.1347310333688));
#147445=CARTESIAN_POINT('Ctrl Pts',(-6.66999609999171,2.16857488955242,
56.126348920393));
#147446=CARTESIAN_POINT('Ctrl Pts',(-6.6084532761143,2.34221516089241,56.1179668074173));
#147447=CARTESIAN_POINT('Ctrl Pts',(-6.54695819642816,2.51572072417377,
56.1095911971852));
#147448=CARTESIAN_POINT('Ctrl Pts',(-6.47858848436843,2.68690862505205,
56.1012155869531));
#147449=CARTESIAN_POINT('Ctrl Pts',(-6.40354228977823,2.85521850398911,
56.0928399767209));
#147450=CARTESIAN_POINT('Ctrl Pts',(-6.32854330036063,3.02342251350895,
56.0844696348722));
#147451=CARTESIAN_POINT('Ctrl Pts',(-6.2468763355756,3.18875181124019,56.0760992930235));
#147452=CARTESIAN_POINT('Ctrl Pts',(-6.15878797446274,3.35066519487,56.0677289511748));
#147453=CARTESIAN_POINT('Ctrl Pts',(-6.07074210947161,3.5125004672627,56.0593626473972));
#147454=CARTESIAN_POINT('Ctrl Pts',(-5.97628118258174,3.67092282354423,
56.0509963436196));
#147455=CARTESIAN_POINT('Ctrl Pts',(-5.87569830779665,3.82541448189024,
56.042630039842));
#147456=CARTESIAN_POINT('Ctrl Pts',(-5.77514356321215,3.97986293326541,
56.0342660758843));
#147457=CARTESIAN_POINT('Ctrl Pts',(-5.66847046265733,4.13038260273449,
56.0259021119265));
#147458=CARTESIAN_POINT('Ctrl Pts',(-5.55601644007937,4.27648312051711,
56.0175381479687));
#147459=CARTESIAN_POINT('Ctrl Pts',(-5.4435797222972,4.42256115587032,56.0091754710853));
#147460=CARTESIAN_POINT('Ctrl Pts',(-5.32536405655652,4.56422113502112,
56.0008127942018));
#147461=CARTESIAN_POINT('Ctrl Pts',(-5.20174855583322,4.7010039911052,55.9924501173184));
#147462=CARTESIAN_POINT('Ctrl Pts',(-5.07813560011289,4.83778403109605,
55.9840876126062));
#147463=CARTESIAN_POINT('Ctrl Pts',(-4.9491232517426,4.96968690467919,55.9757251078941));
#147464=CARTESIAN_POINT('Ctrl Pts',(-4.8151293233923,5.09628846922028,55.9673626031819));
#147465=CARTESIAN_POINT('Ctrl Pts',(-4.68112029327568,5.22290430237241,
55.9589991559749));
#147466=CARTESIAN_POINT('Ctrl Pts',(-4.54212880305775,5.34421740996469,
55.9506357087678));
#147467=CARTESIAN_POINT('Ctrl Pts',(-4.39860806628166,5.45984190629564,
55.9422722615608));
#147468=CARTESIAN_POINT('Ctrl Pts',(-4.25500282041639,5.57553448561647,
55.9339038897183));
#147469=CARTESIAN_POINT('Ctrl Pts',(-4.10686325439232,5.68553155319408,
55.9255355178758));
#147470=CARTESIAN_POINT('Ctrl Pts',(-3.95467489630229,5.78948814896934,
55.9171671460333));
#147471=CARTESIAN_POINT('Ctrl Pts',(-3.80244093857533,5.89347589287633,
55.9087962668064));
#147472=CARTESIAN_POINT('Ctrl Pts',(-3.64615604426595,5.99141937507047,
55.9004253875795));
#147473=CARTESIAN_POINT('Ctrl Pts',(-3.48633361420345,6.08301771269615,
55.8920545083526));
#147474=CARTESIAN_POINT('Ctrl Pts',(-3.32637576825999,6.17469366063961,
55.8836765365669));
#147475=CARTESIAN_POINT('Ctrl Pts',(-3.16287468543343,6.26001356257396,
55.8752985647811));
#147476=CARTESIAN_POINT('Ctrl Pts',(-2.99636821242039,6.3387225919815,55.8669205929954));
#147477=CARTESIAN_POINT('Ctrl Pts',(-2.8905519644874,6.3887428345561,55.8615963222712));
#147478=CARTESIAN_POINT('Ctrl Pts',(-2.78352237841438,6.43609408750066,
55.856272051547));
#147479=CARTESIAN_POINT('Ctrl Pts',(-2.6754215039807,6.48072112797161,55.8509477808228));
#147480=CARTESIAN_POINT('Ctrl Pts',(-2.51577917410116,6.54662591138558,
55.8430849491133));
#147481=CARTESIAN_POINT('Ctrl Pts',(-2.35346751901651,6.60672388344153,
55.8352221174038));
#147482=CARTESIAN_POINT('Ctrl Pts',(-2.18896617001708,6.66078476375125,
55.8273592856943));
#147483=CARTESIAN_POINT('Ctrl Pts',(-2.02459121863661,6.71480410539522,
55.8195024955353));
#147484=CARTESIAN_POINT('Ctrl Pts',(-1.85803027908938,6.76279546176815,
55.8116457053763));
#147485=CARTESIAN_POINT('Ctrl Pts',(-1.68978406494728,6.80457613495141,
55.8037889152173));
#147486=CARTESIAN_POINT('Ctrl Pts',(-1.52163273375822,6.84633324579972,
55.7959365559185));
#147487=CARTESIAN_POINT('Ctrl Pts',(-1.35179838744811,6.88188654919576,
55.7880841966197));
#147488=CARTESIAN_POINT('Ctrl Pts',(-1.18079780428295,6.9111028865081,55.7802318373209));
#147489=CARTESIAN_POINT('Ctrl Pts',(-1.00983759645948,6.94031232548372,
55.7723813320607));
#147490=CARTESIAN_POINT('Ctrl Pts',(-0.837712073892817,6.96318770382964,
55.7645308268005));
#147491=CARTESIAN_POINT('Ctrl Pts',(-0.66494907568763,6.9796467882868,55.7566803215403));
#147492=CARTESIAN_POINT('Ctrl Pts',(-0.49221386965655,6.99610322499099,
55.7488310791814));
#147493=CARTESIAN_POINT('Ctrl Pts',(-0.318841772228494,7.00614538938612,
55.7409818368225));
#147494=CARTESIAN_POINT('Ctrl Pts',(-0.14536615867979,7.00974287990727,
55.7331325944636));
#147495=CARTESIAN_POINT('Ctrl Pts',(0.028167902071642,7.01334158249077,
55.7252807075471));
#147496=CARTESIAN_POINT('Ctrl Pts',(0.201805166826835,7.01049126617955,
55.7174288206305));
#147497=CARTESIAN_POINT('Ctrl Pts',(0.375011639626966,7.00121366854664,
55.709576933714));
#147498=CARTESIAN_POINT('Ctrl Pts',(0.502194920866248,6.99440124814517,
55.7038113943215));
#147499=CARTESIAN_POINT('Ctrl Pts',(0.629145902603533,6.98412447108672,
55.698045854929));
#147500=CARTESIAN_POINT('Ctrl Pts',(0.755654947645477,6.9704097557173,55.6922803155365));
#147501=CARTESIAN_POINT('Ctrl Pts',(0.967514223858894,6.94744230962937,
55.6826250137968));
#147502=CARTESIAN_POINT('Ctrl Pts',(1.17802593747764,6.91484431154008,55.6729697120572));
#147503=CARTESIAN_POINT('Ctrl Pts',(1.38640874482444,6.87280854925949,55.6633144103175));
#147504=CARTESIAN_POINT('Ctrl Pts',(1.59594594977885,6.83053991755926,55.6536056202053));
#147505=CARTESIAN_POINT('Ctrl Pts',(1.80333056029977,6.77872872847641,55.6438968300932));
#147506=CARTESIAN_POINT('Ctrl Pts',(2.00778925425767,6.71761928610035,55.634188039981));
#147507=CARTESIAN_POINT('Ctrl Pts',(2.21323181874091,6.65621578051764,55.6244325304447));
#147508=CARTESIAN_POINT('Ctrl Pts',(2.41572020486721,6.58542435393008,55.6146770209085));
#147509=CARTESIAN_POINT('Ctrl Pts',(2.61449161453801,6.50554072771898,55.6049215113722));
#147510=CARTESIAN_POINT('Ctrl Pts',(2.81345983918247,6.42557800414768,55.5951563423464));
#147511=CARTESIAN_POINT('Ctrl Pts',(3.00870369433969,6.3365050981482,55.5853911733206));
#147512=CARTESIAN_POINT('Ctrl Pts',(3.19948029428995,6.23866591579885,55.5756260042948));
#147513=CARTESIAN_POINT('Ctrl Pts',(3.38999677842398,6.14096013303196,55.5658741496635));
#147514=CARTESIAN_POINT('Ctrl Pts',(3.57605814715117,6.03451197991433,55.5561222950322));
#147515=CARTESIAN_POINT('Ctrl Pts',(3.75694710651464,5.91971071939764,55.5463704404009));
#147516=CARTESIAN_POINT('Ctrl Pts',(3.83582807475557,5.86964887694633,55.5421179103506));
#147517=CARTESIAN_POINT('Ctrl Pts',(3.91372574775415,5.81799920250456,55.5378653803003));
#147518=CARTESIAN_POINT('Ctrl Pts',(3.99058202083765,5.76479676115883,55.53361285025));
#147519=CARTESIAN_POINT('Ctrl Pts',(4.13576384025537,5.66429712824473,55.5255798033032));
#147520=CARTESIAN_POINT('Ctrl Pts',(4.27729829741059,5.55820455855653,55.5175467563565));
#147521=CARTESIAN_POINT('Ctrl Pts',(4.4147229865368,5.44681994512794,55.5095137094097));
#147522=CARTESIAN_POINT('Ctrl Pts',(4.55205933369662,5.33550693408638,55.5014858264198));
#147523=CARTESIAN_POINT('Ctrl Pts',(4.68529088804447,5.21890888078641,55.4934579434299));
#147524=CARTESIAN_POINT('Ctrl Pts',(4.81398506889093,5.09736935281281,55.48543006044));
#147525=CARTESIAN_POINT('Ctrl Pts',(4.9426211429497,4.97588470122523,55.4774058021244));
#147526=CARTESIAN_POINT('Ctrl Pts',(5.06672365669603,4.84946326856371,55.4693815438088));
#147527=CARTESIAN_POINT('Ctrl Pts',(5.18589396084689,4.7184881465732,55.4613572854932));
#147528=CARTESIAN_POINT('Ctrl Pts',(5.3050498559007,4.58752886102161,55.4533339974052));
#147529=CARTESIAN_POINT('Ctrl Pts',(5.41927447695573,4.45201724861941,55.4453107093172));
#147530=CARTESIAN_POINT('Ctrl Pts',(5.52820672190483,4.31237254911798,55.4372874212292));
#147531=CARTESIAN_POINT('Ctrl Pts',(5.63713004073727,4.17273929237051,55.4292647905847));
#147532=CARTESIAN_POINT('Ctrl Pts',(5.74076162494552,4.02897391469021,55.4212421599403));
#147533=CARTESIAN_POINT('Ctrl Pts',(5.83878148468279,3.88152770653842,55.4132195292959));
#147534=CARTESIAN_POINT('Ctrl Pts',(5.93683819271826,3.73402606939643,55.4051938827291));
#147535=CARTESIAN_POINT('Ctrl Pts',(6.02927876143492,3.58284114470238,55.3971682361623));
#147536=CARTESIAN_POINT('Ctrl Pts',(6.11582705957431,3.42845241178563,55.3891425895955));
#147537=CARTESIAN_POINT('Ctrl Pts',(6.16686111599986,3.3374155748226,55.3844101880516));
#147538=CARTESIAN_POINT('Ctrl Pts',(6.21584728934764,3.24526527880537,55.3796777865076));
#147539=CARTESIAN_POINT('Ctrl Pts',(6.26273655294488,3.15210365167582,55.3749453849637));
#147540=CARTESIAN_POINT('Ctrl Pts',(6.34919419481366,2.98032585061109,55.3662194582488));
#147541=CARTESIAN_POINT('Ctrl Pts',(6.42856377990602,2.80502227980312,55.3574935315339));
#147542=CARTESIAN_POINT('Ctrl Pts',(6.50058655335303,2.62678530239259,55.348767604819));
#147543=CARTESIAN_POINT('Ctrl Pts',(6.52493627278427,2.5665263011836,55.3458175119926));
#147544=CARTESIAN_POINT('Ctrl Pts',(6.54844665376745,2.50593217957409,55.3428674191661));
#147545=CARTESIAN_POINT('Ctrl Pts',(6.57110895151813,2.44502632087638,55.3399173263397));
#147546=CARTESIAN_POINT('Origin',(0.,0.,50.));
#147547=CARTESIAN_POINT('',(6.57110895151814,2.44502632087635,53.3398059204455));
#147548=CARTESIAN_POINT('',(6.57110895151814,2.44502632087637,53.8869540129975));
#147549=CARTESIAN_POINT('',(6.57110895151814,2.44502632087636,50.));
#147550=CARTESIAN_POINT('',(7.01124705281182,0.00642860308702523,55.773534356869));
#147551=CARTESIAN_POINT('Ctrl Pts',(6.57110895151814,2.44502632087636,53.8869540129975));
#147552=CARTESIAN_POINT('Ctrl Pts',(6.50353113000907,2.62664449980998,53.8957638417488));
#147553=CARTESIAN_POINT('Ctrl Pts',(6.42844709549375,2.80538575922644,53.9045736705001));
#147554=CARTESIAN_POINT('Ctrl Pts',(6.34612790280083,2.98065214404377,53.9133834992514));
#147555=CARTESIAN_POINT('Ctrl Pts',(6.26808555048096,3.1468126772838,53.9217356190523));
#147556=CARTESIAN_POINT('Ctrl Pts',(6.18354076655633,3.30985002457295,53.9300877388533));
#147557=CARTESIAN_POINT('Ctrl Pts',(6.09276264047734,3.46927513600516,53.9384398586542));
#147558=CARTESIAN_POINT('Ctrl Pts',(6.00730213029333,3.61936141722321,53.9463027266175));
#147559=CARTESIAN_POINT('Ctrl Pts',(5.91616768828528,3.76650633753764,53.9541655945807));
#147560=CARTESIAN_POINT('Ctrl Pts',(5.81959624471386,3.91023351105946,53.9620284625439));
#147561=CARTESIAN_POINT('Ctrl Pts',(5.72309900317295,4.05385024978065,53.9698852889616));
#147562=CARTESIAN_POINT('Ctrl Pts',(5.62117327908481,4.19405414961448,53.9777421153793));
#147563=CARTESIAN_POINT('Ctrl Pts',(5.51410187190258,4.33039341270288,53.9855989417971));
#147564=CARTESIAN_POINT('Ctrl Pts',(5.40709084775426,4.46665578711892,53.9934513373492));
#147565=CARTESIAN_POINT('Ctrl Pts',(5.29494014783479,4.59905756132789,54.0013037329013));
#147566=CARTESIAN_POINT('Ctrl Pts',(5.17797568436643,4.7271761522721,54.0091561284534));
#147567=CARTESIAN_POINT('Ctrl Pts',(5.06103883857755,4.85526449182134,54.0170066698958));
#147568=CARTESIAN_POINT('Ctrl Pts',(4.93929074204122,4.97907137395758,54.0248572113383));
#147569=CARTESIAN_POINT('Ctrl Pts',(4.81309732348821,5.09820759847328,54.0327077527807));
#147570=CARTESIAN_POINT('Ctrl Pts',(4.68692420563802,5.21732465757514,54.0405570313086));
#147571=CARTESIAN_POINT('Ctrl Pts',(4.55630746885099,5.33177229508453,54.0484063098365));
#147572=CARTESIAN_POINT('Ctrl Pts',(4.42164925644293,5.44119880315889,54.0562555883643));
#147573=CARTESIAN_POINT('Ctrl Pts',(4.28694567770733,5.55066217700413,54.0641075113127));
#147574=CARTESIAN_POINT('Ctrl Pts',(4.14819820004141,5.6551008016911,54.0719594342611));
#147575=CARTESIAN_POINT('Ctrl Pts',(4.0058414920635,5.75420372449243,54.0798113572095));
#147576=CARTESIAN_POINT('Ctrl Pts',(3.90131521226575,5.82697064910488,54.0855766794532));
#147577=CARTESIAN_POINT('Ctrl Pts',(3.79484377077415,5.89686176940799,54.091342001697));
#147578=CARTESIAN_POINT('Ctrl Pts',(3.68660877623829,5.96376913482261,54.0971073239407));
#147579=CARTESIAN_POINT('Ctrl Pts',(3.50534659890811,6.07581953761967,54.1067625640726));
#147580=CARTESIAN_POINT('Ctrl Pts',(3.31923040315571,6.17944381964446,54.1164178042044));
#147581=CARTESIAN_POINT('Ctrl Pts',(3.12899509086528,6.27431400902449,54.1260730443363));
#147582=CARTESIAN_POINT('Ctrl Pts',(2.93770603920344,6.36970969733803,54.1357817661617));
#147583=CARTESIAN_POINT('Ctrl Pts',(2.74225217857912,6.45625407208534,54.145490487987));
#147584=CARTESIAN_POINT('Ctrl Pts',(2.54339373412106,6.53366473548603,54.1551992098124));
#147585=CARTESIAN_POINT('Ctrl Pts',(2.34357847294275,6.61144786391968,54.1649546456076));
#147586=CARTESIAN_POINT('Ctrl Pts',(2.14032583552511,6.68000918165012,54.1747100814028));
#147587=CARTESIAN_POINT('Ctrl Pts',(1.93441933500118,6.73911332438279,54.184465517198));
#147588=CARTESIAN_POINT('Ctrl Pts',(1.72830896972415,6.79827598518766,54.1942306116951));
#147589=CARTESIAN_POINT('Ctrl Pts',(1.51953952560415,6.84796274221861,54.2039957061922));
#147590=CARTESIAN_POINT('Ctrl Pts',(1.30890841130126,6.88798848237458,54.2137608006893));
#147591=CARTESIAN_POINT('Ctrl Pts',(1.098564428644,6.92795965957256,54.2235125834416));
#147592=CARTESIAN_POINT('Ctrl Pts',(0.886363885309897,6.95829613468245,
54.2332643661938));
#147593=CARTESIAN_POINT('Ctrl Pts',(0.673111867682699,6.97886430417476,
54.2430161489461));
#147594=CARTESIAN_POINT('Ctrl Pts',(0.580109871664257,6.98783435209513,
54.2472690290397));
#147595=CARTESIAN_POINT('Ctrl Pts',(0.486908028073329,6.99494717353388,
54.2515219091334));
#147596=CARTESIAN_POINT('Ctrl Pts',(0.393573741917043,7.00019473101809,
54.255774789227));
#147597=CARTESIAN_POINT('Ctrl Pts',(0.217279127273066,7.01010658830655,
54.2638078485465));
#147598=CARTESIAN_POINT('Ctrl Pts',(0.040425745098178,7.01336470575221,
54.2718409078661));
#147599=CARTESIAN_POINT('Ctrl Pts',(-0.136436700210057,7.00992236685513,
54.2798739671856));
#147600=CARTESIAN_POINT('Ctrl Pts',(-0.313185452402696,7.00648224080902,
54.2879018625849));
#147601=CARTESIAN_POINT('Ctrl Pts',(-0.489942891161812,6.99635023926621,
54.2959297579843));
#147602=CARTESIAN_POINT('Ctrl Pts',(-0.666156623046019,6.97953164016555,
54.3039576533837));
#147603=CARTESIAN_POINT('Ctrl Pts',(-0.842290793328995,6.96272063476749,
54.3119819241381));
#147604=CARTESIAN_POINT('Ctrl Pts',(-1.0178813813776,6.93922907782464,54.3200061948925));
#147605=CARTESIAN_POINT('Ctrl Pts',(-1.19237848016099,6.90911427916408,
54.328030465647));
#147606=CARTESIAN_POINT('Ctrl Pts',(-1.3668544805284,6.87900312167895,54.3360537661881));
#147607=CARTESIAN_POINT('Ctrl Pts',(-1.54023689264898,6.84227037227052,
54.3440770667293));
#147608=CARTESIAN_POINT('Ctrl Pts',(-1.71198322303292,6.79902493057305,
54.3521003672704));
#147609=CARTESIAN_POINT('Ctrl Pts',(-1.88371548052415,6.75578303240666,
54.3601230103824));
#147610=CARTESIAN_POINT('Ctrl Pts',(-2.05381156874999,6.70602959835288,
54.3681456534944));
#147611=CARTESIAN_POINT('Ctrl Pts',(-2.22174173798897,6.64992407567017,
54.3761682966063));
#147612=CARTESIAN_POINT('Ctrl Pts',(-2.38973503612754,6.59379746160213,
54.3841939556185));
#147613=CARTESIAN_POINT('Ctrl Pts',(-2.55556044177969,6.53131410776282,
54.3922196146307));
#147614=CARTESIAN_POINT('Ctrl Pts',(-2.71870548857921,6.46268264955578,
54.4002452736429));
#147615=CARTESIAN_POINT('Ctrl Pts',(-2.81490390688788,6.42221413484906,
54.4049776005998));
#147616=CARTESIAN_POINT('Ctrl Pts',(-2.91017076440804,6.37960892477289,
54.4097099275567));
#147617=CARTESIAN_POINT('Ctrl Pts',(-3.00440463526238,6.33491746987393,
54.4144422545136));
#147618=CARTESIAN_POINT('Ctrl Pts',(-3.17824421839563,6.25247212597776,
54.4231722975224));
#147619=CARTESIAN_POINT('Ctrl Pts',(-3.34865412282789,6.16288344747847,
54.4319023405312));
#147620=CARTESIAN_POINT('Ctrl Pts',(-3.51506571933231,6.06646021591462,
54.4406323835399));
#147621=CARTESIAN_POINT('Ctrl Pts',(-3.68152543207951,5.9700091045412,54.449364950753));
#147622=CARTESIAN_POINT('Ctrl Pts',(-3.84398429229108,5.86671963295671,
54.4580975179661));
#147623=CARTESIAN_POINT('Ctrl Pts',(-4.00190048133327,5.75694529242762,
54.4668300851791));
#147624=CARTESIAN_POINT('Ctrl Pts',(-4.16206028373926,5.64561131967269,
54.4756867213975));
#147625=CARTESIAN_POINT('Ctrl Pts',(-4.31754711202974,5.52760696979519,
54.4845433576159));
#147626=CARTESIAN_POINT('Ctrl Pts',(-4.46782797217122,5.40334523916291,
54.4933999938343));
#147627=CARTESIAN_POINT('Ctrl Pts',(-4.6160979330381,5.28074624737677,54.5021381199289));
#147628=CARTESIAN_POINT('Ctrl Pts',(-4.7593001826618,5.15205648890996,54.5108762460234));
#147629=CARTESIAN_POINT('Ctrl Pts',(-4.89695704387536,5.0177124541906,54.519614372118));
#147630=CARTESIAN_POINT('Ctrl Pts',(-5.03741434505067,4.88063537441898,
54.5285302633983));
#147631=CARTESIAN_POINT('Ctrl Pts',(-5.17209799958015,4.73767170116489,
54.5374461546786));
#147632=CARTESIAN_POINT('Ctrl Pts',(-5.30054026203266,4.58932451381145,
54.546362045959));
#147633=CARTESIAN_POINT('Ctrl Pts',(-5.42898252448522,4.44097732645797,
54.5552779372393));
#147634=CARTESIAN_POINT('Ctrl Pts',(-5.55118320150893,4.28724685761481,
54.5641938285196));
#147635=CARTESIAN_POINT('Ctrl Pts',(-5.66671764406679,4.12867263232654,
54.5731097197999));
#147636=CARTESIAN_POINT('Ctrl Pts',(-5.7799817066632,3.97321456647546,54.581850403926));
#147637=CARTESIAN_POINT('Ctrl Pts',(-5.88685113118549,3.81308483500101,
54.590591088052));
#147638=CARTESIAN_POINT('Ctrl Pts',(-5.98696423013525,3.64881979132719,
54.599331772178));
#147639=CARTESIAN_POINT('Ctrl Pts',(-6.0870593168541,3.48458430202668,54.6080708836905));
#147640=CARTESIAN_POINT('Ctrl Pts',(-6.18040036318854,3.31621522010431,
54.6168099952029));
#147641=CARTESIAN_POINT('Ctrl Pts',(-6.26667004960582,3.14427623657232,
54.6255491067154));
#147642=CARTESIAN_POINT('Ctrl Pts',(-6.35405748974329,2.97010952454761,
54.6344014465796));
#147643=CARTESIAN_POINT('Ctrl Pts',(-6.43418890444417,2.7922800038065,54.6432537864439));
#147644=CARTESIAN_POINT('Ctrl Pts',(-6.50678286093266,2.61139873691724,
54.6521061263081));
#147645=CARTESIAN_POINT('Ctrl Pts',(-6.57841155134463,2.43292260895761,
54.6608407585314));
#147646=CARTESIAN_POINT('Ctrl Pts',(-6.6427018948626,2.25147565357265,54.6695753907547));
#147647=CARTESIAN_POINT('Ctrl Pts',(-6.69943181608028,2.06766532693067,
54.6783100229779));
#147648=CARTESIAN_POINT('Ctrl Pts',(-6.75730847336472,1.88013946664295,
54.6872212166627));
#147649=CARTESIAN_POINT('Ctrl Pts',(-6.807315694583,1.69015394239007,54.6961324103474));
#147650=CARTESIAN_POINT('Ctrl Pts',(-6.84927073344378,1.49837144343133,
54.7050436040322));
#147651=CARTESIAN_POINT('Ctrl Pts',(-6.89122577230458,1.30658894447253,
54.7139547977169));
#147652=CARTESIAN_POINT('Ctrl Pts',(-6.92512855086331,1.1130097640552,54.7228659914017));
#147653=CARTESIAN_POINT('Ctrl Pts',(-6.95085125227764,0.918310095343839,
54.7317771850864));
#147654=CARTESIAN_POINT('Ctrl Pts',(-6.97401782472743,0.742958218085718,
54.7398028512397));
#147655=CARTESIAN_POINT('Ctrl Pts',(-6.99055942297077,0.566616825996988,
54.747828517393));
#147656=CARTESIAN_POINT('Ctrl Pts',(-7.00040399381127,0.389833920960158,
54.7558541835463));
#147657=CARTESIAN_POINT('Ctrl Pts',(-7.01024544024081,0.213107122223639,
54.7638773025617));
#147658=CARTESIAN_POINT('Ctrl Pts',(-7.01339407050618,0.0359394550822815,
54.7719004215771));
#147659=CARTESIAN_POINT('Ctrl Pts',(-7.00982972206353,-0.141116371037569,
54.7799235405925));
#147660=CARTESIAN_POINT('Ctrl Pts',(-7.00626582311167,-0.318149869103393,
54.787945647833));
#147661=CARTESIAN_POINT('Ctrl Pts',(-6.99599063966237,-0.495071187861098,
54.7959677550735));
#147662=CARTESIAN_POINT('Ctrl Pts',(-6.97903612023533,-0.671328082945003,
54.8039898623141));
#147663=CARTESIAN_POINT('Ctrl Pts',(-6.9620753004268,-0.847650475944406,
54.8120149506085));
#147664=CARTESIAN_POINT('Ctrl Pts',(-6.93843021838755,-1.0233075865209,
54.8200400389029));
#147665=CARTESIAN_POINT('Ctrl Pts',(-6.90818470985104,-1.19775230205596,
54.8280651271973));
#147666=CARTESIAN_POINT('Ctrl Pts',(-6.87793324458435,-1.3722313737699,
54.8360917960003));
#147667=CARTESIAN_POINT('Ctrl Pts',(-6.8410788344518,-1.5454972150915,54.8441184648033));
#147668=CARTESIAN_POINT('Ctrl Pts',(-6.79775631958861,-1.71701356488324,
54.8521451336063));
#147669=CARTESIAN_POINT('Ctrl Pts',(-6.75439902553422,-1.88866760751076,
54.8601782461961));
#147670=CARTESIAN_POINT('Ctrl Pts',(-6.70456335463898,-2.05856900043394,
54.8682113587859));
#147671=CARTESIAN_POINT('Ctrl Pts',(-6.64843401704203,-2.2261966857262,
54.8762444713757));
#147672=CARTESIAN_POINT('Ctrl Pts',(-6.61536063351217,-2.32496882456212,
54.8809778643747));
#147673=CARTESIAN_POINT('Ctrl Pts',(-6.58010302925627,-2.42295187452145,
54.8857112573737));
#147674=CARTESIAN_POINT('Ctrl Pts',(-6.54270675095957,-2.52004264516458,
54.8904446503727));
#147675=CARTESIAN_POINT('Ctrl Pts',(-6.46566914564606,-2.72005293520058,
54.9001956009555));
#147676=CARTESIAN_POINT('Ctrl Pts',(-6.37950825511883,-2.91639359711574,
54.9099465515383));
#147677=CARTESIAN_POINT('Ctrl Pts',(-6.28457812809835,-3.10832821856507,
54.9196975021211));
#147678=CARTESIAN_POINT('Ctrl Pts',(-6.1895112379634,-3.30053935472502,
54.9294625006191));
#147679=CARTESIAN_POINT('Ctrl Pts',(-6.08564985756998,-3.48833171860857,
54.939227499117));
#147680=CARTESIAN_POINT('Ctrl Pts',(-5.9733949394707,-3.67099161802446,
54.948992497615));
#147681=CARTESIAN_POINT('Ctrl Pts',(-5.86132712748513,-3.85334706054448,
54.9587412198468));
#147682=CARTESIAN_POINT('Ctrl Pts',(-5.74089375861056,-4.03058710381781,
54.9684899420787));
#147683=CARTESIAN_POINT('Ctrl Pts',(-5.61253852683564,-4.2020278256201,
54.9782386643105));
#147684=CARTESIAN_POINT('Ctrl Pts',(-5.48453557941323,-4.37299801043815,
54.987960630155));
#147685=CARTESIAN_POINT('Ctrl Pts',(-5.34865419813391,-4.53820061719486,
54.9976825959995));
#147686=CARTESIAN_POINT('Ctrl Pts',(-5.20537875608043,-4.69698398637323,
55.007404561844));
#147687=CARTESIAN_POINT('Ctrl Pts',(-5.06305132705065,-4.85471673096605,
55.0170622001939));
#147688=CARTESIAN_POINT('Ctrl Pts',(-4.91342737247014,-5.00611485176101,
55.0267198385437));
#147689=CARTESIAN_POINT('Ctrl Pts',(-4.75702536968583,-5.15056658967394,
55.0363774768935));
#147690=CARTESIAN_POINT('Ctrl Pts',(-4.68828106127532,-5.21405832663855,
55.0406223564821));
#147691=CARTESIAN_POINT('Ctrl Pts',(-4.61822785765543,-5.27620843656793,
55.0448672360707));
#147692=CARTESIAN_POINT('Ctrl Pts',(-4.54691247897004,-5.33696669195963,
55.0491121156593));
#147693=CARTESIAN_POINT('Ctrl Pts',(-4.41499884814111,-5.44935257869675,
55.0569639631751));
#147694=CARTESIAN_POINT('Ctrl Pts',(-4.27881843737147,-5.55692722135325,
55.0648158106908));
#147695=CARTESIAN_POINT('Ctrl Pts',(-4.13877603120052,-5.65934267614712,
55.0726676582066));
#147696=CARTESIAN_POINT('Ctrl Pts',(-3.99877333985031,-5.76172908679973,
55.080517279006));
#147697=CARTESIAN_POINT('Ctrl Pts',(-3.85491113930223,-5.85895899499041,
55.0883668998054));
#147698=CARTESIAN_POINT('Ctrl Pts',(-3.70762649059494,-5.95072536492306,
55.0962165206048));
#147699=CARTESIAN_POINT('Ctrl Pts',(-3.5603536006087,-6.0424844085311,55.1040655147163));
#147700=CARTESIAN_POINT('Ctrl Pts',(-3.40965913056299,-6.12878058113111,
55.1119145088278));
#147701=CARTESIAN_POINT('Ctrl Pts',(-3.25600802220571,-6.20935087765477,
55.1197635029393));
#147702=CARTESIAN_POINT('Ctrl Pts',(-3.10227912470417,-6.28996196460608,
55.1276164707712));
#147703=CARTESIAN_POINT('Ctrl Pts',(-2.94559093636288,-6.36484120605821,
55.1354694386031));
#147704=CARTESIAN_POINT('Ctrl Pts',(-2.78643214072944,-6.433772026394,55.143322406435));
#147705=CARTESIAN_POINT('Ctrl Pts',(-2.62723292404789,-6.50272035286883,
55.1511773686599));
#147706=CARTESIAN_POINT('Ctrl Pts',(-2.46556220551837,-6.56571711004186,
55.1590323308847));
#147707=CARTESIAN_POINT('Ctrl Pts',(-2.30192680489228,-6.62259462351565,
55.1668872931096));
#147708=CARTESIAN_POINT('Ctrl Pts',(-2.13812898240354,-6.67952859269308,
55.1747500520435));
#147709=CARTESIAN_POINT('Ctrl Pts',(-1.97236294751005,-6.73033107539278,
55.1826128109774));
#147710=CARTESIAN_POINT('Ctrl Pts',(-1.80514932766534,-6.77488468295434,
55.1904755699112));
#147711=CARTESIAN_POINT('Ctrl Pts',(-1.68248388892909,-6.80756855059561,
55.1962435735893));
#147712=CARTESIAN_POINT('Ctrl Pts',(-1.55903971638853,-6.83689065907245,
55.2020115772675));
#147713=CARTESIAN_POINT('Ctrl Pts',(-1.43502477046539,-6.86282234001805,
55.2077795809456));
#147714=CARTESIAN_POINT('Ctrl Pts',(-1.25489218013704,-6.90048829088814,
55.2161576472814));
#147715=CARTESIAN_POINT('Ctrl Pts',(-1.07315613852357,-6.93108293641786,
55.2245357136171));
#147716=CARTESIAN_POINT('Ctrl Pts',(-0.890397569983565,-6.95448191671151,
55.2329137799528));
#147717=CARTESIAN_POINT('Ctrl Pts',(-0.707763969636188,-6.97786489705342,
55.2412861174638));
#147718=CARTESIAN_POINT('Ctrl Pts',(-0.524109561367762,-6.99406198019323,
55.2496584549748));
#147719=CARTESIAN_POINT('Ctrl Pts',(-0.340024355208382,-7.00300007142404,
55.2580307924858));
#147720=CARTESIAN_POINT('Ctrl Pts',(-0.156038028158063,-7.01193336166885,
55.2663986328985));
#147721=CARTESIAN_POINT('Ctrl Pts',(0.0283783077945347,-7.01361541849126,
55.2747664733111));
#147722=CARTESIAN_POINT('Ctrl Pts',(0.212630178955949,-7.0080250405872,
55.2831343137238));
#147723=CARTESIAN_POINT('Ctrl Pts',(0.396810073053705,-7.00243684653605,
55.2914988852818));
#147724=CARTESIAN_POINT('Ctrl Pts',(0.580825302401443,-6.98958189295206,
55.2998634568399));
#147725=CARTESIAN_POINT('Ctrl Pts',(0.764081589738954,-6.96949107802873,
55.3082280283979));
#147726=CARTESIAN_POINT('Ctrl Pts',(0.947293113236532,-6.94940517066975,
55.31659055675));
#147727=CARTESIAN_POINT('Ctrl Pts',(1.12974573803573,-6.92208696300415,
55.324953085102));
#147728=CARTESIAN_POINT('Ctrl Pts',(1.31085004288317,-6.88761923508938,
55.3333156134541));
#147729=CARTESIAN_POINT('Ctrl Pts',(1.49196880038271,-6.85314875654932,
55.3416788091603));
#147730=CARTESIAN_POINT('Ctrl Pts',(1.67173869895743,-6.8115276733912,55.3500420048665));
#147731=CARTESIAN_POINT('Ctrl Pts',(1.84957948553568,-6.76289008406802,
55.3584052005727));
#147732=CARTESIAN_POINT('Ctrl Pts',(2.02743240047959,-6.71424917776409,
55.3667689666312));
#147733=CARTESIAN_POINT('Ctrl Pts',(2.20335562386006,-6.65859089766998,
55.3751327326897));
#147734=CARTESIAN_POINT('Ctrl Pts',(2.37678289939389,-6.59609957563171,
55.3834964987482));
#147735=CARTESIAN_POINT('Ctrl Pts',(2.55024512424107,-6.53359566025258,
55.3918619502848));
#147736=CARTESIAN_POINT('Ctrl Pts',(2.72121008895998,-6.46425606861821,
55.4002274018214));
#147737=CARTESIAN_POINT('Ctrl Pts',(2.88912999007159,-6.3883138982809,55.408592853358));
#147738=CARTESIAN_POINT('Ctrl Pts',(3.05710612721923,-6.312346295064,55.4169611064675));
#147739=CARTESIAN_POINT('Ctrl Pts',(3.22203486782568,-6.22977183939668,
55.425329359577));
#147740=CARTESIAN_POINT('Ctrl Pts',(3.38339116340422,-6.14087052443693,
55.4336976126864));
#147741=CARTESIAN_POINT('Ctrl Pts',(3.5448970592932,-6.05188678527259,55.4420736243606));
#147742=CARTESIAN_POINT('Ctrl Pts',(3.70282360319209,-5.95656462381894,
55.4504496360348));
#147743=CARTESIAN_POINT('Ctrl Pts',(3.85667193453369,-5.85522912889668,
55.458825647709));
#147744=CARTESIAN_POINT('Ctrl Pts',(4.01059571499958,-5.75384393779452,
55.4672057670829));
#147745=CARTESIAN_POINT('Ctrl Pts',(4.16043702371027,-5.64643971852223,
55.4755858864567));
#147746=CARTESIAN_POINT('Ctrl Pts',(4.30572796616131,-5.53338352582905,
55.4839660058306));
#147747=CARTESIAN_POINT('Ctrl Pts',(4.4511849219402,-5.42019815209771,55.4923557005537));
#147748=CARTESIAN_POINT('Ctrl Pts',(4.59208086652548,-5.30134810742315,
55.5007453952768));
#147749=CARTESIAN_POINT('Ctrl Pts',(4.72798181539348,-5.17724004811527,
55.5091350899998));
#147750=CARTESIAN_POINT('Ctrl Pts',(4.81426300592747,-5.09844596167848,
55.5144615638394));
#147751=CARTESIAN_POINT('Ctrl Pts',(4.8985315577186,-5.01753325389086,55.519788037679));
#147752=CARTESIAN_POINT('Ctrl Pts',(4.98068446859895,-4.9346133371073,55.5251145115186));
#147753=CARTESIAN_POINT('Ctrl Pts',(5.10995352083697,-4.80413738757123,
55.533495811921));
#147754=CARTESIAN_POINT('Ctrl Pts',(5.23424319083462,-4.66842675091216,
55.5418771123234));
#147755=CARTESIAN_POINT('Ctrl Pts',(5.35311923683061,-4.52788482613837,
55.5502584127257));
#147756=CARTESIAN_POINT('Ctrl Pts',(5.47184462483593,-4.38752101768579,
55.5586290910564));
#147757=CARTESIAN_POINT('Ctrl Pts',(5.58516985216965,-4.24233837165848,
55.5669997693871));
#147758=CARTESIAN_POINT('Ctrl Pts',(5.69269703844291,-4.09277741772055,
55.5753704477178));
#147759=CARTESIAN_POINT('Ctrl Pts',(5.80010219981773,-3.9433861897919,55.5837316267655));
#147760=CARTESIAN_POINT('Ctrl Pts',(5.90172224425848,-3.78962682138928,
55.5920928058132));
#147761=CARTESIAN_POINT('Ctrl Pts',(5.99719888257382,-3.63197358544295,
55.6004539848609));
#147762=CARTESIAN_POINT('Ctrl Pts',(6.09255162868244,-3.47452492317708,
55.608804314292));
#147763=CARTESIAN_POINT('Ctrl Pts',(6.18177670032624,-3.31319275055744,
55.6171546437231));
#147764=CARTESIAN_POINT('Ctrl Pts',(6.26455857907563,-3.14848096259607,
55.6255049731542));
#147765=CARTESIAN_POINT('Ctrl Pts',(6.34727676211866,-2.98389591050782,
55.633848877506));
#147766=CARTESIAN_POINT('Ctrl Pts',(6.42356148545388,-2.81593671673851,
55.6421927818578));
#147767=CARTESIAN_POINT('Ctrl Pts',(6.49314215248363,-2.64513355998147,
55.6505366862096));
#147768=CARTESIAN_POINT('Ctrl Pts',(6.56266693188494,-2.47446759339189,
55.6588738886851));
#147769=CARTESIAN_POINT('Ctrl Pts',(6.6254982708226,-2.30096252206304,55.6672110911606));
#147770=CARTESIAN_POINT('Ctrl Pts',(6.68141282022042,-2.12517041394196,
55.675548293636));
#147771=CARTESIAN_POINT('Ctrl Pts',(6.69981958138623,-2.06730062184191,
55.6782928546923));
#147772=CARTESIAN_POINT('Ctrl Pts',(6.71747716175574,-2.00918315349665,
55.6810374157486));
#147773=CARTESIAN_POINT('Ctrl Pts',(6.73437873898325,-1.95083816920585,
55.6837819768049));
#147774=CARTESIAN_POINT('Ctrl Pts',(6.78297200599455,-1.78309208478724,
55.6916727899783));
#147775=CARTESIAN_POINT('Ctrl Pts',(6.82529219203744,-1.61353383431378,
55.6995636031516));
#147776=CARTESIAN_POINT('Ctrl Pts',(6.86121524485502,-1.44268913015557,
55.7074544163249));
#147777=CARTESIAN_POINT('Ctrl Pts',(6.89714304061904,-1.27182186924851,
55.715346271328));
#147778=CARTESIAN_POINT('Ctrl Pts',(6.92667195235105,-1.09966818756756,
55.723238126331));
#147779=CARTESIAN_POINT('Ctrl Pts',(6.94972928813047,-0.926762852191188,
55.7311299813341));
#147780=CARTESIAN_POINT('Ctrl Pts',(6.97280535063941,-0.753717086390481,
55.7390282459517));
#147781=CARTESIAN_POINT('Ctrl Pts',(6.98939929757199,-0.579918822786608,
55.7469265105693));
#147782=CARTESIAN_POINT('Ctrl Pts',(6.99949039413753,-0.405907359968376,
55.7548247751868));
#147783=CARTESIAN_POINT('Ctrl Pts',(7.00745839743096,-0.268506642432263,
55.7610613024142));
#147784=CARTESIAN_POINT('Ctrl Pts',(7.0113730362753,-0.13097312713087,55.7672978296416));
#147785=CARTESIAN_POINT('Ctrl Pts',(7.01124705281182,0.00642860308711848,
55.773534356869));
#147786=CARTESIAN_POINT('Ctrl Pts',(7.01124705281098,0.00642860400140193,
55.7735343569105));
#147787=CARTESIAN_POINT('Ctrl Pts',(7.01105339139811,0.217642113168657,
55.7831211270235));
#147788=CARTESIAN_POINT('Ctrl Pts',(7.00131167594713,0.428520891988302,
55.7927078971364));
#147789=CARTESIAN_POINT('Ctrl Pts',(6.98213567539767,0.638285181434724,
55.8022946672493));
#147790=CARTESIAN_POINT('Ctrl Pts',(6.9628194060205,0.84958385709994,55.8119515627777));
#147791=CARTESIAN_POINT('Ctrl Pts',(6.93393038498918,1.0597516130558,55.8216084583061));
#147792=CARTESIAN_POINT('Ctrl Pts',(6.89563491151376,1.2680085684303,55.8312653538345));
#147793=CARTESIAN_POINT('Ctrl Pts',(6.88085100385837,1.34840584041663,55.8349933832535));
#147794=CARTESIAN_POINT('Ctrl Pts',(6.86466574189174,1.42851852440994,55.8387214126724));
#147795=CARTESIAN_POINT('Ctrl Pts',(6.84709064213326,1.50830245670791,55.8424494420914));
#147796=CARTESIAN_POINT('Ctrl Pts',(6.80754063442373,1.68784369293669,55.8508387880574));
#147797=CARTESIAN_POINT('Ctrl Pts',(6.76089090729276,1.86598150139765,55.8592281340235));
#147798=CARTESIAN_POINT('Ctrl Pts',(6.70725831382453,2.04213429385331,55.8676174799895));
#147799=CARTESIAN_POINT('Ctrl Pts',(6.6659849047502,2.1776941426776,55.8740735710627));
#147800=CARTESIAN_POINT('Ctrl Pts',(6.62057715257561,2.31207849286783,55.8805296621359));
#147801=CARTESIAN_POINT('Ctrl Pts',(6.57110895151812,2.44502632087642,55.886985753209));
#147802=CARTESIAN_POINT('',(7.01124999682065,-0.000211145429389691,55.2264656430482));
#147803=CARTESIAN_POINT('Ctrl Pts',(6.57110895151813,2.44502632087638,55.3399173263397));
#147804=CARTESIAN_POINT('Ctrl Pts',(6.63816763466189,2.26480334768358,55.331187878767));
#147805=CARTESIAN_POINT('Ctrl Pts',(6.69779687952727,2.08184970904798,55.3224584311943));
#147806=CARTESIAN_POINT('Ctrl Pts',(6.74980327540723,1.89678209233477,55.3137289836216));
#147807=CARTESIAN_POINT('Ctrl Pts',(6.80183255142163,1.71163305540624,55.3049956955417));
#147808=CARTESIAN_POINT('Ctrl Pts',(6.84623220132626,1.52436844594368,55.2962624074619));
#147809=CARTESIAN_POINT('Ctrl Pts',(6.88285906775861,1.33561881383617,55.287529119382));
#147810=CARTESIAN_POINT('Ctrl Pts',(6.91949072354235,1.14684450071162,55.2787946893321));
#147811=CARTESIAN_POINT('Ctrl Pts',(6.94834751786577,0.956585047407869,
55.2700602592821));
#147812=CARTESIAN_POINT('Ctrl Pts',(6.96933759544937,0.765480269605941,
55.2613258292322));
#147813=CARTESIAN_POINT('Ctrl Pts',(6.99033260036295,0.574330630783553,
55.2525893488126));
#147814=CARTESIAN_POINT('Ctrl Pts',(7.00345716960281,0.382335543913326,
55.243852868393));
#147815=CARTESIAN_POINT('Ctrl Pts',(7.00867129074538,0.190140213477998,
55.2351163879733));
#147816=CARTESIAN_POINT('Ctrl Pts',(7.01039227485,0.126703806916737,55.2322328063454));
#147817=CARTESIAN_POINT('Ctrl Pts',(7.01125190782734,0.0632456077901646,
55.2293492247175));
#147818=CARTESIAN_POINT('Ctrl Pts',(7.01124999682068,-0.000211144518860344,
55.2264656430896));
#147819=CARTESIAN_POINT('Ctrl Pts',(7.01124999682065,-0.000211145429297141,
55.2264656430482));
#147820=CARTESIAN_POINT('Ctrl Pts',(7.0112477462756,-0.0749422636437259,
55.2230697352579));
#147821=CARTESIAN_POINT('Ctrl Pts',(7.01005060799595,-0.149671035804848,
55.2196738274676));
#147822=CARTESIAN_POINT('Ctrl Pts',(7.00765927269795,-0.224361494625235,
55.2162779196773));
#147823=CARTESIAN_POINT('Ctrl Pts',(7.00150424893689,-0.41660619955968,
55.2075372411295));
#147824=CARTESIAN_POINT('Ctrl Pts',(6.98743363633494,-0.608607698602225,
55.1987965625817));
#147825=CARTESIAN_POINT('Ctrl Pts',(6.96549162193804,-0.79972059321427,
55.1900558840339));
#147826=CARTESIAN_POINT('Ctrl Pts',(6.94355355540339,-0.990799102315082,
55.1813167781309));
#147827=CARTESIAN_POINT('Ctrl Pts',(6.91374694663639,-1.18098905436653,
55.1725776722279));
#147828=CARTESIAN_POINT('Ctrl Pts',(6.87616778480095,-1.36965074298726,
55.1638385663249));
#147829=CARTESIAN_POINT('Ctrl Pts',(6.83810169186425,-1.56075701097914,
55.1549862236637));
#147830=CARTESIAN_POINT('Ctrl Pts',(6.7920602499044,-1.75029485064277,55.1461338810025));
#147831=CARTESIAN_POINT('Ctrl Pts',(6.73819686859386,-1.93760922855254,
55.1372815383414));
#147832=CARTESIAN_POINT('Ctrl Pts',(6.6850497474794,-2.12243275219755,55.1285469116597));
#147833=CARTESIAN_POINT('Ctrl Pts',(6.62428751394606,-2.30509131460187,
55.119812284978));
#147834=CARTESIAN_POINT('Ctrl Pts',(6.55610819284299,-2.48496920025924,
55.1110776582963));
#147835=CARTESIAN_POINT('Ctrl Pts',(6.48655059951523,-2.66848338926529,
55.1021664576454));
#147836=CARTESIAN_POINT('Ctrl Pts',(6.40927292840654,-2.84910299986734,
55.0932552569945));
#147837=CARTESIAN_POINT('Ctrl Pts',(6.32453817181363,-3.02619290128245,
55.0843440563435));
#147838=CARTESIAN_POINT('Ctrl Pts',(6.23980341522072,-3.20328280269756,
55.0754328556926));
#147839=CARTESIAN_POINT('Ctrl Pts',(6.14761169182779,-3.37684271566718,
55.0665216550417));
#147840=CARTESIAN_POINT('Ctrl Pts',(6.04827762928387,-3.54626060542712,
55.0576104543908));
#147841=CARTESIAN_POINT('Ctrl Pts',(5.95881457135179,-3.69884313450292,
55.0495847757901));
#147842=CARTESIAN_POINT('Ctrl Pts',(5.86351657780664,-3.84813579674568,
55.0415590971894));
#147843=CARTESIAN_POINT('Ctrl Pts',(5.76266350826657,-3.99366196028068,
55.0335334185887));
#147844=CARTESIAN_POINT('Ctrl Pts',(5.66184244664213,-4.1391419379218,55.0255102871117));
#147845=CARTESIAN_POINT('Ctrl Pts',(5.55547002759096,-4.28085749581419,
55.0174871556348));
#147846=CARTESIAN_POINT('Ctrl Pts',(5.44386994354426,-4.41836017095432,
55.0094640241578));
#147847=CARTESIAN_POINT('Ctrl Pts',(5.33228393297764,-4.55584550613296,
55.0014419044487));
#147848=CARTESIAN_POINT('Ctrl Pts',(5.21547180194833,-4.6891187326226,54.9934197847396));
#147849=CARTESIAN_POINT('Ctrl Pts',(5.09379807142342,-4.81776377275423,
54.9853976650305));
#147850=CARTESIAN_POINT('Ctrl Pts',(4.9720791267729,-4.94645661755971,54.9773725642907));
#147851=CARTESIAN_POINT('Ctrl Pts',(4.84549522359992,-5.07051757167975,
54.9693474635509));
#147852=CARTESIAN_POINT('Ctrl Pts',(4.7144486674688,-5.18956648712604,54.9613223628111));
#147853=CARTESIAN_POINT('Ctrl Pts',(4.58337630236738,-5.3086388486667,54.9532956815675));
#147854=CARTESIAN_POINT('Ctrl Pts',(4.44783981064288,-5.42269696511521,
54.9452690003238));
#147855=CARTESIAN_POINT('Ctrl Pts',(4.30827507160288,-5.53140058845002,
54.9372423190802));
#147856=CARTESIAN_POINT('Ctrl Pts',(4.16859829159107,-5.6401914778069,54.9292091941089));
#147857=CARTESIAN_POINT('Ctrl Pts',(4.02488710034641,-5.74361907094462,
54.9211760691376));
#147858=CARTESIAN_POINT('Ctrl Pts',(3.87760738209954,-5.84138575620436,
54.9131429441663));
#147859=CARTESIAN_POINT('Ctrl Pts',(3.79082648474781,-5.89899233488972,
54.9084096258123));
#147860=CARTESIAN_POINT('Ctrl Pts',(3.70280716923416,-5.95463436232717,
54.9036763074583));
#147861=CARTESIAN_POINT('Ctrl Pts',(3.61364876866986,-6.00825841148588,
54.8989429891043));
#147862=CARTESIAN_POINT('Ctrl Pts',(3.42997789160466,-6.11872670250984,
54.889192110578));
#147863=CARTESIAN_POINT('Ctrl Pts',(3.24136375540439,-6.2206942963535,54.8794412320516));
#147864=CARTESIAN_POINT('Ctrl Pts',(3.04853815308218,-6.31379772337555,
54.8696903535253));
#147865=CARTESIAN_POINT('Ctrl Pts',(2.85543479600782,-6.40703526080092,
54.8599254293908));
#147866=CARTESIAN_POINT('Ctrl Pts',(2.65810787306583,-6.49138307414728,
54.8501605052563));
#147867=CARTESIAN_POINT('Ctrl Pts',(2.45731222308588,-6.56652443845089,
54.8403955811218));
#147868=CARTESIAN_POINT('Ctrl Pts',(2.25685122170069,-6.64154057119707,
54.8306469313346));
#147869=CARTESIAN_POINT('Ctrl Pts',(2.05293308272549,-6.70738090720442,
54.8208982815474));
#147870=CARTESIAN_POINT('Ctrl Pts',(1.84632807593882,-6.76377847053702,
54.8111496317601));
#147871=CARTESIAN_POINT('Ctrl Pts',(1.64029004573899,-6.82002126463889,
54.8014277347427));
#147872=CARTESIAN_POINT('Ctrl Pts',(1.43157990615793,-6.86687300734899,
54.7917058377253));
#147873=CARTESIAN_POINT('Ctrl Pts',(1.22098019931334,-6.904117171325,54.7819839407078));
#147874=CARTESIAN_POINT('Ctrl Pts',(1.01177380921548,-6.94111492984223,
54.7723263632573));
#147875=CARTESIAN_POINT('Ctrl Pts',(0.800702812731656,-6.96863177940732,
54.7626687858067));
#147876=CARTESIAN_POINT('Ctrl Pts',(0.588552144967729,-6.98650362736282,
54.7530112083561));
#147877=CARTESIAN_POINT('Ctrl Pts',(0.49529604656456,-6.99435964228444,
54.7487659801767));
#147878=CARTESIAN_POINT('Ctrl Pts',(0.401831556430714,-7.00035262339382,
54.7445207519973));
#147879=CARTESIAN_POINT('Ctrl Pts',(0.308226413662711,-7.0044716460573,
54.7402755238179));
#147880=CARTESIAN_POINT('Ctrl Pts',(0.135096336517516,-7.0120901025908,
54.7324236402519));
#147881=CARTESIAN_POINT('Ctrl Pts',(-0.0384439618467919,-7.01329093163461,
54.7245717566859));
#147882=CARTESIAN_POINT('Ctrl Pts',(-0.211861327003002,-7.00804832607628,
54.7167198731199));
#147883=CARTESIAN_POINT('Ctrl Pts',(-0.385229514743517,-7.00280720720754,
54.7088702161783));
#147884=CARTESIAN_POINT('Ctrl Pts',(-0.558474457710154,-6.99112629990335,
54.7010205592367));
#147885=CARTESIAN_POINT('Ctrl Pts',(-0.731062671239445,-6.97303190392961,
54.6931709022951));
#147886=CARTESIAN_POINT('Ctrl Pts',(-0.903637107778184,-6.95493895235534,
54.6853218719585));
#147887=CARTESIAN_POINT('Ctrl Pts',(-1.07555453993769,-6.93043357180747,
54.677472841622));
#147888=CARTESIAN_POINT('Ctrl Pts',(-1.24628653963422,-6.89959393179241,
54.6696238112855));
#147889=CARTESIAN_POINT('Ctrl Pts',(-1.41710497670054,-6.86873867843378,
54.6617708071799));
#147890=CARTESIAN_POINT('Ctrl Pts',(-1.58673640628852,-6.83154282599992,
54.6539178030743));
#147891=CARTESIAN_POINT('Ctrl Pts',(-1.75466219618514,-6.7881357632106,
54.6460647989688));
#147892=CARTESIAN_POINT('Ctrl Pts',(-1.922630634798,-6.74471767617357,54.6382098004075));
#147893=CARTESIAN_POINT('Ctrl Pts',(-2.08889220514317,-6.69508534519298,
54.6303548018463));
#147894=CARTESIAN_POINT('Ctrl Pts',(-2.25294401222274,-6.63941788414389,
54.622499803285));
#147895=CARTESIAN_POINT('Ctrl Pts',(-2.4171586526295,-6.58369516909875,
54.6146370080675));
#147896=CARTESIAN_POINT('Ctrl Pts',(-2.57915879281569,-6.52192549566605,
54.60677421285));
#147897=CARTESIAN_POINT('Ctrl Pts',(-2.73846154073518,-6.4543361356854,
54.5989114176325));
#147898=CARTESIAN_POINT('Ctrl Pts',(-2.85531873874926,-6.40475567755736,
54.5931436312654));
#147899=CARTESIAN_POINT('Ctrl Pts',(-2.97072489308552,-6.35204464108381,
54.5873758448984));
#147900=CARTESIAN_POINT('Ctrl Pts',(-3.08449833512118,-6.29630817091529,
54.5816080585314));
#147901=CARTESIAN_POINT('Ctrl Pts',(-3.24976105988727,-6.21534761664107,
54.5732300040942));
#147902=CARTESIAN_POINT('Ctrl Pts',(-3.41194408556617,-6.12782279722444,
54.564851949657));
#147903=CARTESIAN_POINT('Ctrl Pts',(-3.57051266870268,-6.03399252942309,
54.5564738952198));
#147904=CARTESIAN_POINT('Ctrl Pts',(-3.72897282251262,-5.94022642283544,
54.5481015697031));
#147905=CARTESIAN_POINT('Ctrl Pts',(-3.88382317933206,-5.84016363092992,
54.5397292441864));
#147906=CARTESIAN_POINT('Ctrl Pts',(-4.03455332592352,-5.73410899990395,
54.5313569186696));
#147907=CARTESIAN_POINT('Ctrl Pts',(-4.18520250831488,-5.62811133577254,
54.5229890903199));
#147908=CARTESIAN_POINT('Ctrl Pts',(-4.33173562505888,-5.51612843863671,
54.5146212619701));
#147909=CARTESIAN_POINT('Ctrl Pts',(-4.47367062579133,-5.39850883989568,
54.5062534336204));
#147910=CARTESIAN_POINT('Ctrl Pts',(-4.61555017954625,-5.28093518930849,
54.4978888741669));
#147911=CARTESIAN_POINT('Ctrl Pts',(-4.75283494655109,-5.15772943761216,
54.4895243147134));
#147912=CARTESIAN_POINT('Ctrl Pts',(-4.88507504265928,-5.02928110072279,
54.4811597552599));
#147913=CARTESIAN_POINT('Ctrl Pts',(-5.017282836326,-4.90086414005748,54.472797239027));
#147914=CARTESIAN_POINT('Ctrl Pts',(-5.14444818127107,-4.76720737716857,
54.4644347227941));
#147915=CARTESIAN_POINT('Ctrl Pts',(-5.26615690214589,-4.62873827781192,
54.4560722065612));
#147916=CARTESIAN_POINT('Ctrl Pts',(-5.38787533644869,-4.49025812740145,
54.4477090229259));
#147917=CARTESIAN_POINT('Ctrl Pts',(-5.50413605511812,-4.34696511608873,
54.4393458392906));
#147918=CARTESIAN_POINT('Ctrl Pts',(-5.61456364759881,-4.19932156539149,
54.4309826556552));
#147919=CARTESIAN_POINT('Ctrl Pts',(-5.724998771629,-4.05166794488572,54.4226189016214));
#147920=CARTESIAN_POINT('Ctrl Pts',(-5.82959977905141,-3.8996634565157,
54.4142551475876));
#147921=CARTESIAN_POINT('Ctrl Pts',(-5.92803316711366,-3.74380145468485,
54.4058913935538));
#147922=CARTESIAN_POINT('Ctrl Pts',(-6.02648639246817,-3.58790804196648,
54.3975259539716));
#147923=CARTESIAN_POINT('Ctrl Pts',(-6.11876934441629,-3.42815584362014,
54.3891605143895));
#147924=CARTESIAN_POINT('Ctrl Pts',(-6.2045930419162,-3.26506535106191,
54.3807950748073));
#147925=CARTESIAN_POINT('Ctrl Pts',(-6.2904454826061,-3.10192023791346,
54.3724268335582));
#147926=CARTESIAN_POINT('Ctrl Pts',(-6.36983420218175,-2.93543489201752,
54.364058592309));
#147927=CARTESIAN_POINT('Ctrl Pts',(-6.44251698659686,-2.76615282294941,
54.3556903510599));
#147928=CARTESIAN_POINT('Ctrl Pts',(-6.51526716039136,-2.59671380043394,
54.3473143510191));
#147929=CARTESIAN_POINT('Ctrl Pts',(-6.58129884465704,-2.42447317550418,
54.3389383509783));
#147930=CARTESIAN_POINT('Ctrl Pts',(-6.64041819490054,-2.24999394651049,
54.3305623509374));
#147931=CARTESIAN_POINT('Ctrl Pts',(-6.69956653892374,-2.07542914803224,
54.3221822430723));
#147932=CARTESIAN_POINT('Ctrl Pts',(-6.75179568935851,-1.89862386941246,
54.3138021352073));
#147933=CARTESIAN_POINT('Ctrl Pts',(-6.79696201811788,-1.72015519263901,
54.3054220273422));
#147934=CARTESIAN_POINT('Ctrl Pts',(-6.84217995684615,-1.54148258601093,
54.2970323438238));
#147935=CARTESIAN_POINT('Ctrl Pts',(-6.880318873142,-1.36114310361073,54.2886426603054));
#147936=CARTESIAN_POINT('Ctrl Pts',(-6.91128622526463,-1.17972423683137,
54.280252976787));
#147937=CARTESIAN_POINT('Ctrl Pts',(-6.93094742005016,-1.06454126402203,
54.2749263605109));
#147938=CARTESIAN_POINT('Ctrl Pts',(-6.9477188042965,-0.948923346076843,
54.2695997442348));
#147939=CARTESIAN_POINT('Ctrl Pts',(-6.96158756580647,-0.833021684056731,
54.2642731279587));
#147940=CARTESIAN_POINT('Ctrl Pts',(-6.98340956402631,-0.650654580803841,
54.2558918885228));
#147941=CARTESIAN_POINT('Ctrl Pts',(-6.99808673708094,-0.467216904398952,
54.2475106490869));
#147942=CARTESIAN_POINT('Ctrl Pts',(-7.00552433630664,-0.283293727278623,
54.2391294096509));
#147943=CARTESIAN_POINT('Ctrl Pts',(-7.01295250963259,-0.0996036416945087,
54.2307587920192));
#147944=CARTESIAN_POINT('Ctrl Pts',(-7.01315938068839,0.0845703936586706,
54.2223881743875));
#147945=CARTESIAN_POINT('Ctrl Pts',(-7.00610170299844,0.268636352235332,
54.2140175567558));
#147946=CARTESIAN_POINT('Ctrl Pts',(-6.99905203428671,0.452493434703441,
54.2056564380126));
#147947=CARTESIAN_POINT('Ctrl Pts',(-6.98475425997115,0.636242359411314,
54.1972953192695));
#147948=CARTESIAN_POINT('Ctrl Pts',(-6.96321710275037,0.819288802843555,
54.1889342005264));
#147949=CARTESIAN_POINT('Ctrl Pts',(-6.94170789054723,1.00209773878867,
54.1805839305508));
#147950=CARTESIAN_POINT('Ctrl Pts',(-6.91297806944858,1.18420568763883,
54.1722336605751));
#147951=CARTESIAN_POINT('Ctrl Pts',(-6.87708830778799,1.36502123404209,
54.1638833905995));
#147952=CARTESIAN_POINT('Ctrl Pts',(-6.84122615889285,1.54569766508087,
54.1555395451314));
#147953=CARTESIAN_POINT('Ctrl Pts',(-6.7982151107814,1.72508335519677,54.1471956996634));
#147954=CARTESIAN_POINT('Ctrl Pts',(-6.74816742335769,1.90259375296833,
54.1388518541954));
#147955=CARTESIAN_POINT('Ctrl Pts',(-6.6981599286592,2.07996159417015,54.1305147095741));
#147956=CARTESIAN_POINT('Ctrl Pts',(-6.64112715350645,2.25545683213024,
54.1221775649529));
#147957=CARTESIAN_POINT('Ctrl Pts',(-6.57723208423473,2.42850667543109,
54.1138404203317));
#147958=CARTESIAN_POINT('Ctrl Pts',(-6.55619528906484,2.48548155861368,
54.1110955011119));
#147959=CARTESIAN_POINT('Ctrl Pts',(-6.53441503618932,2.54219146814402,
54.108350581892));
#147960=CARTESIAN_POINT('Ctrl Pts',(-6.51189833282458,2.59861629823575,
54.1056056626722));
#147961=CARTESIAN_POINT('Ctrl Pts',(-6.44349740817105,2.77002285314629,
54.0972671856893));
#147962=CARTESIAN_POINT('Ctrl Pts',(-6.36835293155707,2.93865662908672,
54.0889287087064));
#147963=CARTESIAN_POINT('Ctrl Pts',(-6.28672608723384,3.10398158283737,
54.0805902317235));
#147964=CARTESIAN_POINT('Ctrl Pts',(-6.20504785834692,3.26941060958855,
54.0722465056218));
#147965=CARTESIAN_POINT('Ctrl Pts',(-6.1168792673513,3.43152636572703,54.0639027795201));
#147966=CARTESIAN_POINT('Ctrl Pts',(-6.02252708990521,3.58981810317152,
54.0555590534185));
#147967=CARTESIAN_POINT('Ctrl Pts',(-5.9281031021205,3.74823031460582,54.0472089770044));
#147968=CARTESIAN_POINT('Ctrl Pts',(-5.82748630799288,3.90281242090337,
54.0388589005904));
#147969=CARTESIAN_POINT('Ctrl Pts',(-5.72102659059777,4.05308293921717,
54.0305088241764));
#147970=CARTESIAN_POINT('Ctrl Pts',(-5.61440715990367,4.20357889679388,
54.0221462207871));
#147971=CARTESIAN_POINT('Ctrl Pts',(-5.50192747889674,4.34975007302886,
54.0137836173978));
#147972=CARTESIAN_POINT('Ctrl Pts',(-5.38397842384047,4.49114716905607,
54.0054210140085));
#147973=CARTESIAN_POINT('Ctrl Pts',(-5.26592848664575,4.63266520239312,
53.9970512580624));
#147974=CARTESIAN_POINT('Ctrl Pts',(-5.14240006074251,4.76940076577675,
53.9886815021163));
#147975=CARTESIAN_POINT('Ctrl Pts',(-5.01382099609593,4.90094129546637,
53.9803117461702));
#147976=CARTESIAN_POINT('Ctrl Pts',(-4.88504360187024,5.03268472271138,
53.9719290801117));
#147977=CARTESIAN_POINT('Ctrl Pts',(-4.75120023883623,5.15921687887051,
53.9635464140532));
#147978=CARTESIAN_POINT('Ctrl Pts',(-4.61275299158931,5.2801644293605,53.9551637479947));
#147979=CARTESIAN_POINT('Ctrl Pts',(-4.56746887668824,5.31972464368259,
53.9524218977917));
#147980=CARTESIAN_POINT('Ctrl Pts',(-4.52169245438644,5.35868772824994,
53.9496800475887));
#147981=CARTESIAN_POINT('Ctrl Pts',(-4.47544056682393,5.39704162438337,
53.9469381973857));
#147982=CARTESIAN_POINT('Ctrl Pts',(-4.33391683922757,5.51439870178506,
53.9385485535963));
#147983=CARTESIAN_POINT('Ctrl Pts',(-4.18765352090479,5.62628592099622,
53.9301589098068));
#147984=CARTESIAN_POINT('Ctrl Pts',(-4.0371002004268,5.73231615790807,53.9217692660174));
#147985=CARTESIAN_POINT('Ctrl Pts',(-3.88668583235713,5.83824853476125,
53.9133873654062));
#147986=CARTESIAN_POINT('Ctrl Pts',(-3.73198962274071,5.93833451712331,
53.9050054647951));
#147987=CARTESIAN_POINT('Ctrl Pts',(-3.57349379823855,6.03222750204687,
53.896623564184));
#147988=CARTESIAN_POINT('Ctrl Pts',(-3.41512094837784,6.12604763674746,
53.8882481669696));
#147989=CARTESIAN_POINT('Ctrl Pts',(-3.25295464300533,6.21368418686658,
53.8798727697552));
#147990=CARTESIAN_POINT('Ctrl Pts',(-3.08750600255809,6.29483385377786,
53.8714973725407));
#147991=CARTESIAN_POINT('Ctrl Pts',(-2.92216143775945,6.37593247340223,
53.8631272438791));
#147992=CARTESIAN_POINT('Ctrl Pts',(-2.75353894922176,6.4505522017272,53.8547571152175));
#147993=CARTESIAN_POINT('Ctrl Pts',(-2.58217456944514,6.51843547604875,
53.8463869865559));
#147994=CARTESIAN_POINT('Ctrl Pts',(-2.41089285598169,6.58628600342474,
53.838020895651));
#147995=CARTESIAN_POINT('Ctrl Pts',(-2.23687219403378,6.64740643630317,
53.8296548047461));
#147996=CARTESIAN_POINT('Ctrl Pts',(-2.06066934216875,6.70158700792177,
53.8212887138412));
#147997=CARTESIAN_POINT('Ctrl Pts',(-1.88451573485769,6.75575243734457,
53.812924961062));
#147998=CARTESIAN_POINT('Ctrl Pts',(-1.70618146716293,6.80298177499312,
53.8045612082828));
#147999=CARTESIAN_POINT('Ctrl Pts',(-1.52623976564818,6.84311469582779,
53.7961974555036));
#148000=CARTESIAN_POINT('Ctrl Pts',(-1.34632572539831,6.88324144729013,
53.7878349884296));
#148001=CARTESIAN_POINT('Ctrl Pts',(-1.16480506470539,6.91627388541577,
53.7794725213556));
#148002=CARTESIAN_POINT('Ctrl Pts',(-0.982262957190229,6.94210242256854,
53.7711100542816));
#148003=CARTESIAN_POINT('Ctrl Pts',(-0.799724568665301,6.96793043350804,
53.7627477575789));
#148004=CARTESIAN_POINT('Ctrl Pts',(-0.616165100303348,6.98655479047963,
53.7543854608762));
#148005=CARTESIAN_POINT('Ctrl Pts',(-0.432177064832101,6.99791751502782,
53.7460231641734));
#148006=CARTESIAN_POINT('Ctrl Pts',(-0.248168243395415,7.00928152327469,
53.737659922744));
#148007=CARTESIAN_POINT('Ctrl Pts',(-0.0637310863896442,7.01338224377359,
53.7292966813146));
#148008=CARTESIAN_POINT('Ctrl Pts',(0.120539222708804,7.01021375268178,
53.7209334398852));
#148009=CARTESIAN_POINT('Ctrl Pts',(0.304918144002506,7.00704339402501,
53.7125652690126));
#148010=CARTESIAN_POINT('Ctrl Pts',(0.489129691880897,6.99659526681974,
53.7041970981401));
#148011=CARTESIAN_POINT('Ctrl Pts',(0.672580091473121,6.97891557357259,
53.6958289272675));
#148012=CARTESIAN_POINT('Ctrl Pts',(0.856085518248708,6.96123057718233,
53.6874582463057));
#148013=CARTESIAN_POINT('Ctrl Pts',(1.0388290147668,6.93630972631325,53.6790875653439));
#148014=CARTESIAN_POINT('Ctrl Pts',(1.22022364519409,6.90425092375771,53.6707168843821));
#148015=CARTESIAN_POINT('Ctrl Pts',(1.40177210295799,6.87216493450872,53.6623391048665));
#148016=CARTESIAN_POINT('Ctrl Pts',(1.58196908598455,6.83292896081518,53.6539613253508));
#148017=CARTESIAN_POINT('Ctrl Pts',(1.76023839636499,6.78669192983315,53.6455835458351));
#148018=CARTESIAN_POINT('Ctrl Pts',(1.87358558721402,6.75729350133288,53.6402567861611));
#148019=CARTESIAN_POINT('Ctrl Pts',(1.98615374499486,6.72506579399611,53.634930026487));
#148020=CARTESIAN_POINT('Ctrl Pts',(2.09779821810326,6.6900574884393,53.629603266813));
#148021=CARTESIAN_POINT('Ctrl Pts',(2.26260797048975,6.63837817096261,53.6217398955375));
#148022=CARTESIAN_POINT('Ctrl Pts',(2.42574672627303,6.58052935195627,53.6138765242621));
#148023=CARTESIAN_POINT('Ctrl Pts',(2.58669862915145,6.51664152493031,53.6060131529867));
#148024=CARTESIAN_POINT('Ctrl Pts',(2.74752679726607,6.45280281285761,53.5981558268239));
#148025=CARTESIAN_POINT('Ctrl Pts',(2.90617110371796,6.38293446500579,53.5902985006611));
#148026=CARTESIAN_POINT('Ctrl Pts',(3.06212998960766,6.30721701618435,53.5824411744984));
#148027=CARTESIAN_POINT('Ctrl Pts',(3.21800085446169,6.23154230124258,53.5745882829017));
#148028=CARTESIAN_POINT('Ctrl Pts',(3.37118897178812,6.15002521807402,53.566735391305));
#148029=CARTESIAN_POINT('Ctrl Pts',(3.52121218575977,6.06289463089677,53.5588824997083));
#148030=CARTESIAN_POINT('Ctrl Pts',(3.67119985365704,5.97578468819348,53.5510314687535));
#148031=CARTESIAN_POINT('Ctrl Pts',(3.81802377709204,5.88306407266356,53.5431804377986));
#148032=CARTESIAN_POINT('Ctrl Pts',(3.96122593330704,5.78500783645068,53.5353294068438));
#148033=CARTESIAN_POINT('Ctrl Pts',(4.10440499417583,5.68696741454384,53.5274796420869));
#148034=CARTESIAN_POINT('Ctrl Pts',(4.24396313754947,5.58359330299941,53.51962987733));
#148035=CARTESIAN_POINT('Ctrl Pts',(4.37947129523831,5.4752038990967,53.5117801125732));
#148036=CARTESIAN_POINT('Ctrl Pts',(4.51502498564773,5.36677807477085,53.5039277101807));
#148037=CARTESIAN_POINT('Ctrl Pts',(4.64652567396897,5.25333383046175,53.4960753077881));
#148038=CARTESIAN_POINT('Ctrl Pts',(4.77357721788263,5.13522999557098,53.4882229053956));
#148039=CARTESIAN_POINT('Ctrl Pts',(4.86681209160202,5.0485612641835,53.4824605374392));
#148040=CARTESIAN_POINT('Ctrl Pts',(4.9576517174774,4.95938413182107,53.4766981694828));
#148041=CARTESIAN_POINT('Ctrl Pts',(5.04595229654346,4.86785291309298,53.4709358015264));
#148042=CARTESIAN_POINT('Ctrl Pts',(5.19375898840963,4.71463844059719,53.4612901507962));
#148043=CARTESIAN_POINT('Ctrl Pts',(5.33437537846057,4.55490577118934,53.4516445000659));
#148044=CARTESIAN_POINT('Ctrl Pts',(5.46732638077762,4.38930163107449,53.4419988493356));
#148045=CARTESIAN_POINT('Ctrl Pts',(5.60132159491213,4.22239681780098,53.432277440602));
#148046=CARTESIAN_POINT('Ctrl Pts',(5.72753053363526,4.04952800389971,53.4225560318684));
#148047=CARTESIAN_POINT('Ctrl Pts',(5.84551417401756,3.87138096857695,53.4128346231348));
#148048=CARTESIAN_POINT('Ctrl Pts',(5.96383325771917,3.69272743733103,53.4030855751318));
#148049=CARTESIAN_POINT('Ctrl Pts',(6.07388021664457,3.50876568583934,53.3933365271289));
#148050=CARTESIAN_POINT('Ctrl Pts',(6.17525959117132,3.32021016565919,53.3835874791259));
#148051=CARTESIAN_POINT('Ctrl Pts',(6.27678527771802,3.13138251972213,53.3738243611712));
#148052=CARTESIAN_POINT('Ctrl Pts',(6.36961833797077,2.93794787726775,53.3640612432166));
#148053=CARTESIAN_POINT('Ctrl Pts',(6.45340892105336,2.74064588375968,53.3542981252619));
#148054=CARTESIAN_POINT('Ctrl Pts',(6.49486802245064,2.64302198553866,53.3494673903231));
#148055=CARTESIAN_POINT('Ctrl Pts',(6.53411406089336,2.5444516133034,53.3446366553843));
#148056=CARTESIAN_POINT('Ctrl Pts',(6.57110895151815,2.44502632087634,53.3398059204455));
#148057=CARTESIAN_POINT('Origin',(0.,0.,50.));
#148058=CARTESIAN_POINT('',(6.57110895151816,2.4450263208763,51.3398522865015));
#148059=CARTESIAN_POINT('',(6.57110895151813,2.44502632087638,51.8867297377812));
#148060=CARTESIAN_POINT('',(6.57110895151814,2.44502632087636,50.));
#148061=CARTESIAN_POINT('',(7.01124961176728,-0.00233323662125234,53.7735343569105));
#148062=CARTESIAN_POINT('Ctrl Pts',(6.57110895151814,2.44502632087637,51.8867297377812));
#148063=CARTESIAN_POINT('Ctrl Pts',(6.49738188562511,2.64317084738811,51.8963190332494));
#148064=CARTESIAN_POINT('Ctrl Pts',(6.41477564156754,2.83774523706095,51.9059083287176));
#148065=CARTESIAN_POINT('Ctrl Pts',(6.32365121254535,3.02804588878268,51.9154976241858));
#148066=CARTESIAN_POINT('Ctrl Pts',(6.22946919857259,3.22473187992474,51.9254086784384));
#148067=CARTESIAN_POINT('Ctrl Pts',(6.1261876257228,3.41685231034913,51.935319732691));
#148068=CARTESIAN_POINT('Ctrl Pts',(6.01425257633941,3.60366376213081,51.9452307869436));
#148069=CARTESIAN_POINT('Ctrl Pts',(5.90515769409783,3.78573518163498,51.9548903645517));
#148070=CARTESIAN_POINT('Ctrl Pts',(5.78784316266017,3.96276371850206,51.9645499421597));
#148071=CARTESIAN_POINT('Ctrl Pts',(5.6627647591983,4.13409262650002,51.9742095197677));
#148072=CARTESIAN_POINT('Ctrl Pts',(5.53280193451934,4.31211207843014,51.9842463123426));
#148073=CARTESIAN_POINT('Ctrl Pts',(5.39445678623906,4.48397777650178,51.9942831049175));
#148074=CARTESIAN_POINT('Ctrl Pts',(5.24828784053023,4.64898927783691,52.0043198974924));
#148075=CARTESIAN_POINT('Ctrl Pts',(5.1021188948214,4.81400077917204,52.0143566900673));
#148076=CARTESIAN_POINT('Ctrl Pts',(4.94812618434371,4.97215800313843,52.0243934826422));
#148077=CARTESIAN_POINT('Ctrl Pts',(4.7869157045588,5.12279851252695,52.0344302752171));
#148078=CARTESIAN_POINT('Ctrl Pts',(4.65746671048288,5.24376001846283,52.0424896315585));
#148079=CARTESIAN_POINT('Ctrl Pts',(4.52330104608478,5.35993212343665,52.0505489879));
#148080=CARTESIAN_POINT('Ctrl Pts',(4.38481438060566,5.47092582751163,52.0586083442415));
#148081=CARTESIAN_POINT('Ctrl Pts',(4.24641501525139,5.58184956265357,52.0666626200735));
#148082=CARTESIAN_POINT('Ctrl Pts',(4.10370035448013,5.68760116891075,52.0747168959055));
#148083=CARTESIAN_POINT('Ctrl Pts',(3.95710130850763,5.78782997303024,52.0827711717375));
#148084=CARTESIAN_POINT('Ctrl Pts',(3.81056701941027,5.88801450329985,52.0908218897719));
#148085=CARTESIAN_POINT('Ctrl Pts',(3.66015206190331,5.98268088453343,52.0988726078063));
#148086=CARTESIAN_POINT('Ctrl Pts',(3.50631865348546,6.07152007842516,52.1069233258408));
#148087=CARTESIAN_POINT('Ctrl Pts',(3.35250310584948,6.16034895766886,52.1149731091489));
#148088=CARTESIAN_POINT('Ctrl Pts',(3.19527020929626,6.2433518090098,52.1230228924571));
#148089=CARTESIAN_POINT('Ctrl Pts',(3.03510944213073,6.32026401638325,52.1310726757653));
#148090=CARTESIAN_POINT('Ctrl Pts',(2.87496110514854,6.39717025454928,52.1391218343245));
#148091=CARTESIAN_POINT('Ctrl Pts',(2.71188568012388,6.46798663639252,52.1471709928837));
#148092=CARTESIAN_POINT('Ctrl Pts',(2.54639517432985,6.53249555519555,52.1552201514429));
#148093=CARTESIAN_POINT('Ctrl Pts',(2.38084358045904,6.59702828639657,52.1632722812155));
#148094=CARTESIAN_POINT('Ctrl Pts',(2.21287546535397,6.65524877389044,52.1713244109881));
#148095=CARTESIAN_POINT('Ctrl Pts',(2.04302102858217,6.70698826890812,52.1793765407607));
#148096=CARTESIAN_POINT('Ctrl Pts',(1.94654110256793,6.73637709587191,52.1839502740084));
#148097=CARTESIAN_POINT('Ctrl Pts',(1.84945286413414,6.7636757918757,52.188524007256));
#148098=CARTESIAN_POINT('Ctrl Pts',(1.751855358782,6.78886068235362,52.1930977405036));
#148099=CARTESIAN_POINT('Ctrl Pts',(1.56596748980799,6.83682876928772,52.2018090443796));
#148100=CARTESIAN_POINT('Ctrl Pts',(1.37813987116082,6.87714975211457,52.2105203482555));
#148101=CARTESIAN_POINT('Ctrl Pts',(1.18900391786138,6.90969581427506,52.2192316521315));
#148102=CARTESIAN_POINT('Ctrl Pts',(0.999821277320133,6.94224991026438,
52.2279451063482));
#148103=CARTESIAN_POINT('Ctrl Pts',(0.80932993070789,6.96702520816864,52.2366585605649));
#148104=CARTESIAN_POINT('Ctrl Pts',(0.618169440027649,6.98394538251237,
52.2453720147816));
#148105=CARTESIAN_POINT('Ctrl Pts',(0.423660139694004,7.00116196979676,
52.2542381140323));
#148106=CARTESIAN_POINT('Ctrl Pts',(0.22845832857096,7.01024563163166,52.263104213283));
#148107=CARTESIAN_POINT('Ctrl Pts',(0.0332415144088999,7.01117119775433,
52.2719703125337));
#148108=CARTESIAN_POINT('Ctrl Pts',(-0.158727631150627,7.01208136596135,
52.2806889134642));
#148109=CARTESIAN_POINT('Ctrl Pts',(-0.350711002208583,7.00510277572953,
52.2894075143947));
#148110=CARTESIAN_POINT('Ctrl Pts',(-0.542065010767642,6.99026409276513,
52.2981261153252));
#148111=CARTESIAN_POINT('Ctrl Pts',(-0.738274912213163,6.97504885612623,
52.307065963736));
#148112=CARTESIAN_POINT('Ctrl Pts',(-0.933822781115421,6.95156933986731,
52.3160058121468));
#148113=CARTESIAN_POINT('Ctrl Pts',(-1.12802008593984,6.91991309542369,
52.3249456605575));
#148114=CARTESIAN_POINT('Ctrl Pts',(-1.32221739076425,6.88825685098008,
52.3338855089683));
#148115=CARTESIAN_POINT('Ctrl Pts',(-1.51506382311917,6.848423935652,52.3428253573791));
#148116=CARTESIAN_POINT('Ctrl Pts',(-1.70588084663852,6.80055858732001,
52.3517652057899));
#148117=CARTESIAN_POINT('Ctrl Pts',(-1.89259041650315,6.75372357001568,
52.3605126184717));
#148118=CARTESIAN_POINT('Ctrl Pts',(-2.07737841994065,6.69919308793782,
52.3692600311535));
#148119=CARTESIAN_POINT('Ctrl Pts',(-2.25962264990725,6.63714788463585,
52.3780074438353));
#148120=CARTESIAN_POINT('Ctrl Pts',(-2.44183590375321,6.57511322718054,
52.386753369716));
#148121=CARTESIAN_POINT('Ctrl Pts',(-2.6215059896338,6.5055664873029,52.3954992955967));
#148122=CARTESIAN_POINT('Ctrl Pts',(-2.79802728278639,6.42873781447673,
52.4042452214775));
#148123=CARTESIAN_POINT('Ctrl Pts',(-2.97662802191316,6.35100408894243,
52.4130941756107));
#148124=CARTESIAN_POINT('Ctrl Pts',(-3.15200504087013,6.26581586515213,
52.421943129744));
#148125=CARTESIAN_POINT('Ctrl Pts',(-3.32355202203126,6.17346163180366,
52.4307920838772));
#148126=CARTESIAN_POINT('Ctrl Pts',(-3.49301548090057,6.08222908595224,
52.4395335631189));
#148127=CARTESIAN_POINT('Ctrl Pts',(-3.65874117300866,5.98400376189612,
52.4482750423606));
#148128=CARTESIAN_POINT('Ctrl Pts',(-3.82016857284352,5.87911036106303,
52.4570165216023));
#148129=CARTESIAN_POINT('Ctrl Pts',(-3.98457305329781,5.77228249240697,
52.4659192131813));
#148130=CARTESIAN_POINT('Ctrl Pts',(-4.1445189012361,5.65853833707336,52.4748219047603));
#148131=CARTESIAN_POINT('Ctrl Pts',(-4.29944325999532,5.53826816040726,
52.4837245963393));
#148132=CARTESIAN_POINT('Ctrl Pts',(-4.45436761875454,5.41799798374116,
52.4926272879184));
#148133=CARTESIAN_POINT('Ctrl Pts',(-4.60427024354619,5.29120195842042,
52.5015299794974));
#148134=CARTESIAN_POINT('Ctrl Pts',(-4.74862154391487,5.15831561608706,
52.5104326710764));
#148135=CARTESIAN_POINT('Ctrl Pts',(-4.87874294222263,5.03852898003835,
52.5184577506843));
#148136=CARTESIAN_POINT('Ctrl Pts',(-5.00441227347482,4.91373879624791,
52.5264828302922));
#148137=CARTESIAN_POINT('Ctrl Pts',(-5.12522316360501,4.78431960530928,
52.5345079099001));
#148138=CARTESIAN_POINT('Ctrl Pts',(-5.24599570916076,4.6549414911626,52.5425304424011));
#148139=CARTESIAN_POINT('Ctrl Pts',(-5.36191263375501,4.52093756261607,
52.550552974902));
#148140=CARTESIAN_POINT('Ctrl Pts',(-5.47260438858179,4.38271922082345,
52.5585755074029));
#148141=CARTESIAN_POINT('Ctrl Pts',(-5.58328218852011,4.24451830419088,
52.5665970285047));
#148142=CARTESIAN_POINT('Ctrl Pts',(-5.68873590216296,4.1021043190771,52.5746185496065));
#148143=CARTESIAN_POINT('Ctrl Pts',(-5.78863628977454,3.95592169629345,
52.5826400707083));
#148144=CARTESIAN_POINT('Ctrl Pts',(-5.88857383065286,3.80968470773498,
52.5906645750389));
#148145=CARTESIAN_POINT('Ctrl Pts',(-5.98295371015508,3.65967658290397,
52.5986890793694));
#148146=CARTESIAN_POINT('Ctrl Pts',(-6.0714898159291,3.50637105531763,52.6067135837));
#148147=CARTESIAN_POINT('Ctrl Pts',(-6.16004336901296,3.35303531667765,
52.6147396693743));
#148148=CARTESIAN_POINT('Ctrl Pts',(-6.24275067848505,3.1964012026647,52.6227657550486));
#148149=CARTESIAN_POINT('Ctrl Pts',(-6.31937174657498,3.03696679123923,
52.6307918407229));
#148150=CARTESIAN_POINT('Ctrl Pts',(-6.3960543660021,2.8774043027527,52.6388243739229));
#148151=CARTESIAN_POINT('Ctrl Pts',(-6.46664082868963,2.7150373583768,52.6468569071229));
#148152=CARTESIAN_POINT('Ctrl Pts',(-6.53093916853663,2.55038431209378,
52.6548894403228));
#148153=CARTESIAN_POINT('Ctrl Pts',(-6.5688568109,2.45328607693165,52.6596263390029));
#148154=CARTESIAN_POINT('Ctrl Pts',(-6.60458860855919,2.35539315621848,
52.6643632376829));
#148155=CARTESIAN_POINT('Ctrl Pts',(-6.63810335611066,2.25681421390695,
52.6691001363629));
#148156=CARTESIAN_POINT('Ctrl Pts',(-6.7070829409835,2.05392041297912,52.6788495550041));
#148157=CARTESIAN_POINT('Ctrl Pts',(-6.76670966664594,1.84799973121889,
52.6885989736453));
#148158=CARTESIAN_POINT('Ctrl Pts',(-6.81678354254027,1.63984410742365,
52.6983483922864));
#148159=CARTESIAN_POINT('Ctrl Pts',(-6.86692900026164,1.43139092008672,
52.7081117479594));
#148160=CARTESIAN_POINT('Ctrl Pts',(-6.90749428319051,1.22069643805856,
52.7178751036323));
#148161=CARTESIAN_POINT('Ctrl Pts',(-6.93832997257971,1.00856519576182,
52.7276384593053));
#148162=CARTESIAN_POINT('Ctrl Pts',(-6.9691141134063,0.796788576982175,
52.7373854934053));
#148163=CARTESIAN_POINT('Ctrl Pts',(-6.99020116242303,0.583580036267177,
52.7471325275054));
#148164=CARTESIAN_POINT('Ctrl Pts',(-7.00149359135956,0.369748634413932,
52.7568795616055));
#148165=CARTESIAN_POINT('Ctrl Pts',(-7.01275505981469,0.156503494664312,
52.7665998722372));
#148166=CARTESIAN_POINT('Ctrl Pts',(-7.01427551555764,-0.0573610567043534,
52.7763201828688));
#148167=CARTESIAN_POINT('Ctrl Pts',(-7.00600933329113,-0.271034655233487,
52.7860404935005));
#148168=CARTESIAN_POINT('Ctrl Pts',(-6.99779775869817,-0.483296693052025,
52.7956965902626));
#148169=CARTESIAN_POINT('Ctrl Pts',(-6.97992839641362,-0.695370244413059,
52.8053526870247));
#148170=CARTESIAN_POINT('Ctrl Pts',(-6.9524073705954,-0.90645370305976,
52.8150087837868));
#148171=CARTESIAN_POINT('Ctrl Pts',(-6.94028598709886,-0.999423477112943,
52.8192617230742));
#148172=CARTESIAN_POINT('Ctrl Pts',(-6.9262929634038,-1.09220109507887,
52.8235146623617));
#148173=CARTESIAN_POINT('Ctrl Pts',(-6.91043201460631,-1.18471766003728,
52.8277676016491));
#148174=CARTESIAN_POINT('Ctrl Pts',(-6.88114734309575,-1.35553450388971,
52.8356199648071));
#148175=CARTESIAN_POINT('Ctrl Pts',(-6.84550330118022,-1.52539042967983,
52.843472327965));
#148176=CARTESIAN_POINT('Ctrl Pts',(-6.80358783046252,-1.69375889538101,
52.8513246911229));
#148177=CARTESIAN_POINT('Ctrl Pts',(-6.76168421922834,-1.86207972322893,
52.8591748325482));
#148178=CARTESIAN_POINT('Ctrl Pts',(-6.71351280089283,-2.02891355839185,
52.8670249739734));
#148179=CARTESIAN_POINT('Ctrl Pts',(-6.65921250695034,-2.19374459538394,
52.8748751153986));
#148180=CARTESIAN_POINT('Ctrl Pts',(-6.60491651439462,-2.35856257531884,
52.8827246349765));
#148181=CARTESIAN_POINT('Ctrl Pts',(-6.54449273278661,-2.52137771088187,
52.8905741545544));
#148182=CARTESIAN_POINT('Ctrl Pts',(-6.47812970861941,-2.68169014630748,
52.8984236741323));
#148183=CARTESIAN_POINT('Ctrl Pts',(-6.41173303607269,-2.84208386575736,
52.9062771736917));
#148184=CARTESIAN_POINT('Ctrl Pts',(-6.33939125012485,-2.99997199676093,
52.9141306732512));
#148185=CARTESIAN_POINT('Ctrl Pts',(-6.26134087109187,-3.15487512565783,
52.9219841728107));
#148186=CARTESIAN_POINT('Ctrl Pts',(-6.18327063117989,-3.30981767156125,
52.9298396707897));
#148187=CARTESIAN_POINT('Ctrl Pts',(-6.09948908840324,-3.46177336806262,
52.9376951687687));
#148188=CARTESIAN_POINT('Ctrl Pts',(-6.01027801610609,-3.61028873244396,
52.9455506667477));
#148189=CARTESIAN_POINT('Ctrl Pts',(-5.92097835337921,-3.75895157896641,
52.9534139655739));
#148190=CARTESIAN_POINT('Ctrl Pts',(-5.82623860074293,-3.904166950647,52.9612772644001));
#148191=CARTESIAN_POINT('Ctrl Pts',(-5.72638334820141,-4.04551113111083,
52.9691405632263));
#148192=CARTESIAN_POINT('Ctrl Pts',(-5.65317628529437,-4.14913504720336,
52.9749053977961));
#148193=CARTESIAN_POINT('Ctrl Pts',(-5.57722062337591,-4.25067889836404,
52.9806702323659));
#148194=CARTESIAN_POINT('Ctrl Pts',(-5.49865742519521,-4.34998771065454,
52.9864350669357));
#148195=CARTESIAN_POINT('Ctrl Pts',(-5.38448370215646,-4.49431046090313,
52.9948129415739));
#148196=CARTESIAN_POINT('Ctrl Pts',(-5.26454865711783,-4.63423138252872,
53.0031908162122));
#148197=CARTESIAN_POINT('Ctrl Pts',(-5.13921861863479,-4.76928281320972,
53.0115686908504));
#148198=CARTESIAN_POINT('Ctrl Pts',(-5.01397434899191,-4.90424182227565,
53.0199408321417));
#148199=CARTESIAN_POINT('Ctrl Pts',(-4.88334266962664,-5.03433774401859,
53.028312973433));
#148200=CARTESIAN_POINT('Ctrl Pts',(-4.74772973120227,-5.15913645506281,
53.0366851147243));
#148201=CARTESIAN_POINT('Ctrl Pts',(-4.61218970251025,-5.28386807043957,
53.0450527548921));
#148202=CARTESIAN_POINT('Ctrl Pts',(-4.47167399595628,-5.40330793152722,
53.0534203950599));
#148203=CARTESIAN_POINT('Ctrl Pts',(-4.32662543794832,-5.51705889783664,
53.0617880352277));
#148204=CARTESIAN_POINT('Ctrl Pts',(-4.18163360499046,-5.63076537884163,
53.07015240301));
#148205=CARTESIAN_POINT('Ctrl Pts',(-4.03211271387152,-5.7387871990518,
53.0785167707922));
#148206=CARTESIAN_POINT('Ctrl Pts',(-3.87853882063992,-5.84076734507454,
53.0868811385745));
#148207=CARTESIAN_POINT('Ctrl Pts',(-3.72500249747157,-5.94272254284302,
53.0952434601116));
#148208=CARTESIAN_POINT('Ctrl Pts',(-3.56741542335055,-6.0386388326411,
53.1036057816488));
#148209=CARTESIAN_POINT('Ctrl Pts',(-3.40628316674059,-6.12820214667236,
53.1119681031859));
#148210=CARTESIAN_POINT('Ctrl Pts',(-3.24513811494998,-6.21777257274193,
53.1203310887578));
#148211=CARTESIAN_POINT('Ctrl Pts',(-3.08044760260133,-6.30098885019583,
53.1286940743297));
#148212=CARTESIAN_POINT('Ctrl Pts',(-2.91274303831639,-6.3775821872587,
53.1370570599016));
#148213=CARTESIAN_POINT('Ctrl Pts',(-2.74502707181406,-6.45418073189527,
53.145420614072));
#148214=CARTESIAN_POINT('Ctrl Pts',(-2.57429694378769,-6.5241553014348,
53.1537841682425));
#148215=CARTESIAN_POINT('Ctrl Pts',(-2.40110550043158,-6.58728464075276,
53.162147722413));
#148216=CARTESIAN_POINT('Ctrl Pts',(-2.22787918181044,-6.65042669231791,
53.1705129607381));
#148217=CARTESIAN_POINT('Ctrl Pts',(-2.05219086849353,-6.7067206524817,
53.1788781990632));
#148218=CARTESIAN_POINT('Ctrl Pts',(-1.87461048231744,-6.75599453093959,
53.1872434373883));
#148219=CARTESIAN_POINT('Ctrl Pts',(-1.69697064230528,-6.80528490627056,
53.1956114763915));
#148220=CARTESIAN_POINT('Ctrl Pts',(-1.51743778300031,-6.84755042541538,
53.2039795153948));
#148221=CARTESIAN_POINT('Ctrl Pts',(-1.3365944002167,-6.8826696834738,53.212347554398));
#148222=CARTESIAN_POINT('Ctrl Pts',(-1.15558334281819,-6.91782150345393,
53.2207233520911));
#148223=CARTESIAN_POINT('Ctrl Pts',(-0.973259656936354,-6.94581375911681,
53.2290991497842));
#148224=CARTESIAN_POINT('Ctrl Pts',(-0.790214623164005,-6.96657644843131,
53.2374749474773));
#148225=CARTESIAN_POINT('Ctrl Pts',(-0.607079819284237,-6.9873493203157,
53.2458548528822));
#148226=CARTESIAN_POINT('Ctrl Pts',(-0.423223289275351,-7.00088552477128,
53.2542347582872));
#148227=CARTESIAN_POINT('Ctrl Pts',(-0.239239424257183,-7.00716712091135,
53.2626146636922));
#148228=CARTESIAN_POINT('Ctrl Pts',(-0.0550452854087596,-7.01345589624228,
53.2710041464305));
#148229=CARTESIAN_POINT('Ctrl Pts',(0.129276150356669,-7.01247349094504,
53.2793936291688));
#148230=CARTESIAN_POINT('Ctrl Pts',(0.313131156556268,-7.00425409599721,
53.2877831119071));
#148231=CARTESIAN_POINT('Ctrl Pts',(0.429915033188503,-6.99903317313294,
53.2931120737743));
#148232=CARTESIAN_POINT('Ctrl Pts',(0.546510788298153,-6.99089336650238,
53.2984410356414));
#148233=CARTESIAN_POINT('Ctrl Pts',(0.662767741419831,-6.97985425946941,
53.3037699975085));
#148234=CARTESIAN_POINT('Ctrl Pts',(0.845618554035697,-6.96249177372269,
53.3121514747591));
#148235=CARTESIAN_POINT('Ctrl Pts',(1.02799978744619,-6.93791956892268,
53.3205329520096));
#148236=CARTESIAN_POINT('Ctrl Pts',(1.20931955548607,-6.90616918234842,
53.3289144292601));
#148237=CARTESIAN_POINT('Ctrl Pts',(1.39040950741343,-6.87445903821706,
53.3372852832977));
#148238=CARTESIAN_POINT('Ctrl Pts',(1.57044035504783,-6.83558889990403,
53.3456561373352));
#148239=CARTESIAN_POINT('Ctrl Pts',(1.74882434320985,-6.78964210979464,
53.3540269913727));
#148240=CARTESIAN_POINT('Ctrl Pts',(1.92700586840388,-6.74374746855574,
53.362388344625));
#148241=CARTESIAN_POINT('Ctrl Pts',(2.10354394422297,-6.69079226518622,
53.3707496978774));
#148242=CARTESIAN_POINT('Ctrl Pts',(2.27785959632453,-6.63091111552042,
53.3791110511297));
#148243=CARTESIAN_POINT('Ctrl Pts',(2.45194899597982,-6.57110768840239,
53.3874615517902));
#148244=CARTESIAN_POINT('Ctrl Pts',(2.62382141714329,-6.50439635146568,
53.3958120524506));
#148245=CARTESIAN_POINT('Ctrl Pts',(2.7929117479289,-6.43096186668688,53.4041625531111));
#148246=CARTESIAN_POINT('Ctrl Pts',(2.96187193696155,-6.35758390135854,
53.4125066267406));
#148247=CARTESIAN_POINT('Ctrl Pts',(3.12805400352092,-6.27749323003578,
53.4208507003701));
#148248=CARTESIAN_POINT('Ctrl Pts',(3.29091048807659,-6.19092357584614,
53.4291947739996));
#148249=CARTESIAN_POINT('Ctrl Pts',(3.45363610160427,-6.10442348879511,
53.4375321423542));
#148250=CARTESIAN_POINT('Ctrl Pts',(3.61304117445129,-6.01145495582541,
53.4458695107088));
#148251=CARTESIAN_POINT('Ctrl Pts',(3.76860050051226,-5.9122987771288,53.4542068790634));
#148252=CARTESIAN_POINT('Ctrl Pts',(3.81978947701362,-5.87967004679298,
53.4569504069739));
#148253=CARTESIAN_POINT('Ctrl Pts',(3.87056221194856,-5.8463716738514,53.4596939348844));
#148254=CARTESIAN_POINT('Ctrl Pts',(3.92090057162729,-5.81241475377599,
53.4624374627949));
#148255=CARTESIAN_POINT('Ctrl Pts',(4.07389115569456,-5.70921137034,53.470775714977));
#148256=CARTESIAN_POINT('Ctrl Pts',(4.2227417677762,-5.60000642957328,53.4791139671591));
#148257=CARTESIAN_POINT('Ctrl Pts',(4.36698398876145,-5.48516885833072,
53.4874522193411));
#148258=CARTESIAN_POINT('Ctrl Pts',(4.51131694716161,-5.37025904704446,
53.4957957168074));
#148259=CARTESIAN_POINT('Ctrl Pts',(4.65103547577643,-5.24970974185834,
53.5041392142737));
#148260=CARTESIAN_POINT('Ctrl Pts',(4.7857055458016,-5.12392905799679,53.51248271174));
#148261=CARTESIAN_POINT('Ctrl Pts',(4.92047806053816,-4.99805269165838,
53.5208325561785));
#148262=CARTESIAN_POINT('Ctrl Pts',(5.05019421714145,-4.86693723213022,
53.529182400617));
#148263=CARTESIAN_POINT('Ctrl Pts',(5.17445773021242,-4.73102671317178,
53.5375322450555));
#148264=CARTESIAN_POINT('Ctrl Pts',(5.29890761930794,-4.59491234948376,
53.5458946129675));
#148265=CARTESIAN_POINT('Ctrl Pts',(5.41788830112758,-4.45398879682521,
53.5542569808795));
#148266=CARTESIAN_POINT('Ctrl Pts',(5.53104363784399,-4.30873332184362,
53.5626193487914));
#148267=CARTESIAN_POINT('Ctrl Pts',(5.64429573273144,-4.16335364013435,
53.5709888672935));
#148268=CARTESIAN_POINT('Ctrl Pts',(5.7517123531769,-4.01363491088012,53.5793583857955));
#148269=CARTESIAN_POINT('Ctrl Pts',(5.85298110386718,-3.86008274008133,
53.5877279042975));
#148270=CARTESIAN_POINT('Ctrl Pts',(5.95440604789685,-3.70629373584512,
53.5961103316489));
#148271=CARTESIAN_POINT('Ctrl Pts',(6.04966400466087,-3.54865975488553,
53.6044927590003));
#148272=CARTESIAN_POINT('Ctrl Pts',(6.13848817773367,-3.38771153646883,
53.6128751863516));
#148273=CARTESIAN_POINT('Ctrl Pts',(6.16755692568737,-3.33503935238987,
53.6156184335949));
#148274=CARTESIAN_POINT('Ctrl Pts',(6.19593699709623,-3.28201237487052,
53.6183616808381));
#148275=CARTESIAN_POINT('Ctrl Pts',(6.22362016802609,-3.22864965064946,
53.6211049280814));
#148276=CARTESIAN_POINT('Ctrl Pts',(6.31279000626182,-3.05676379629179,
53.6299411597957));
#148277=CARTESIAN_POINT('Ctrl Pts',(6.39488485271589,-2.88108616740664,
53.63877739151));
#148278=CARTESIAN_POINT('Ctrl Pts',(6.46960175896294,-2.70219903836183,
53.6476136232243));
#148279=CARTESIAN_POINT('Ctrl Pts',(6.54422323585766,-2.52354038616014,
53.6564385691946));
#148280=CARTESIAN_POINT('Ctrl Pts',(6.61148547670641,-2.34168065360165,
53.665263515165));
#148281=CARTESIAN_POINT('Ctrl Pts',(6.67113258381076,-2.15722428405542,
53.6740884611354));
#148282=CARTESIAN_POINT('Ctrl Pts',(6.73065862261849,-1.97314231352942,
53.6828954947337));
#148283=CARTESIAN_POINT('Ctrl Pts',(6.78260030170666,-1.78647447390649,
53.691702528332));
#148284=CARTESIAN_POINT('Ctrl Pts',(6.82675078815544,-1.59784236985976,
53.7005095619303));
#148285=CARTESIAN_POINT('Ctrl Pts',(6.87084338698309,-1.40945758956077,
53.7093050482441));
#148286=CARTESIAN_POINT('Ctrl Pts',(6.90716511315425,-1.2191139350955,53.718100534558));
#148287=CARTESIAN_POINT('Ctrl Pts',(6.93555892679197,-1.02744777750318,
53.7268960208719));
#148288=CARTESIAN_POINT('Ctrl Pts',(6.96389349720157,-0.836181528216391,
53.7356731555473));
#148289=CARTESIAN_POINT('Ctrl Pts',(6.98433312971832,-0.643598539623538,
53.7444502902227));
#148290=CARTESIAN_POINT('Ctrl Pts',(6.99677184506829,-0.450344657523186,
53.7532274248982));
#148291=CARTESIAN_POINT('Ctrl Pts',(7.00636465472937,-0.301306139067398,
53.7599964022356));
#148292=CARTESIAN_POINT('Ctrl Pts',(7.01119984858409,-0.151868905524662,
53.7667653795731));
#148293=CARTESIAN_POINT('Ctrl Pts',(7.01124961176728,-0.00233323662125234,
53.7735343569105));
#148294=CARTESIAN_POINT('Ctrl Pts',(7.01124961574396,-0.00232125615213359,
53.7735348992261));
#148295=CARTESIAN_POINT('Ctrl Pts',(7.01131371635395,0.191291748034507,
53.7822991096566));
#148296=CARTESIAN_POINT('Ctrl Pts',(7.00335363842858,0.384791190643915,
53.7910633200871));
#148297=CARTESIAN_POINT('Ctrl Pts',(6.98742384762321,0.577524489668229,
53.7998275305177));
#148298=CARTESIAN_POINT('Ctrl Pts',(6.97146745755452,0.770579611108935,
53.8086063752609));
#148299=CARTESIAN_POINT('Ctrl Pts',(6.94751476422251,0.962865767552298,
53.8173852200042));
#148300=CARTESIAN_POINT('Ctrl Pts',(6.9156720775946,1.15373579197248,53.8261640647475));
#148301=CARTESIAN_POINT('Ctrl Pts',(6.88380340884426,1.34476155728231,53.8349500726118));
#148302=CARTESIAN_POINT('Ctrl Pts',(6.84403193840754,1.53436862407777,53.8437360804762));
#148303=CARTESIAN_POINT('Ctrl Pts',(6.79651493802973,1.72192080527496,53.8525220883405));
#148304=CARTESIAN_POINT('Ctrl Pts',(6.74894331126548,1.90968859978627,53.8613181967553));
#148305=CARTESIAN_POINT('Ctrl Pts',(6.69360842302094,2.09539653188144,53.8701143051701));
#148306=CARTESIAN_POINT('Ctrl Pts',(6.63071768709321,2.27842259393846,53.8789104135849));
#148307=CARTESIAN_POINT('Ctrl Pts',(6.611547547197,2.33421197471973,53.8815916133891));
#148308=CARTESIAN_POINT('Ctrl Pts',(6.59167571245204,2.38975230369193,53.8842728131933));
#148309=CARTESIAN_POINT('Ctrl Pts',(6.57110895151814,2.44502632087636,53.8869540129975));
#148310=CARTESIAN_POINT('',(7.01125,-2.00130710614754E-13,53.2264656430896));
#148311=CARTESIAN_POINT('Ctrl Pts',(6.57110895151815,2.44502632087634,53.3398059204455));
#148312=CARTESIAN_POINT('Ctrl Pts',(6.64140535766679,2.25610183374145,53.3306267257104));
#148313=CARTESIAN_POINT('Ctrl Pts',(6.70357143908928,2.06408955382915,53.3214475309752));
#148314=CARTESIAN_POINT('Ctrl Pts',(6.75737442391738,1.86963029968155,53.31226833624));
#148315=CARTESIAN_POINT('Ctrl Pts',(6.80474661620868,1.69841375454496,53.3041862831817));
#148316=CARTESIAN_POINT('Ctrl Pts',(6.84565607039973,1.52521926086687,53.2961042301234));
#148317=CARTESIAN_POINT('Ctrl Pts',(6.87993901121358,1.35057978826928,53.2880221770651));
#148318=CARTESIAN_POINT('Ctrl Pts',(6.91419962127447,1.17605406994208,53.2799453883839));
#148319=CARTESIAN_POINT('Ctrl Pts',(6.94184224021634,1.00008559936461,53.2718685997028));
#148320=CARTESIAN_POINT('Ctrl Pts',(6.96275330735328,0.823221078107828,
53.2637918110216));
#148321=CARTESIAN_POINT('Ctrl Pts',(6.98365362487211,0.646447476460647,
53.2557191743234));
#148322=CARTESIAN_POINT('Ctrl Pts',(6.99782924055202,0.468779099787468,
53.2476465376252));
#148323=CARTESIAN_POINT('Ctrl Pts',(7.0052179552401,0.290771322660413,53.2395739009269));
#148324=CARTESIAN_POINT('Ctrl Pts',(7.0092171928638,0.1944223053211,53.2352044816478));
#148325=CARTESIAN_POINT('Ctrl Pts',(7.01122899283649,0.097973988105694,
53.2308350623687));
#148326=CARTESIAN_POINT('Ctrl Pts',(7.01124983631059,0.00151503620485756,
53.2264656430896));
#148327=CARTESIAN_POINT('Ctrl Pts',(7.01125,-8.58630487052188E-16,53.2264656430896));
#148328=CARTESIAN_POINT('Ctrl Pts',(7.01125,-0.191009525814462,53.2177938341508));
#148329=CARTESIAN_POINT('Ctrl Pts',(7.00344006572041,-0.382018909628726,
53.209122025212));
#148330=CARTESIAN_POINT('Ctrl Pts',(6.98784625534317,-0.572390840411034,
53.2004502162733));
#148331=CARTESIAN_POINT('Ctrl Pts',(6.97225246786074,-0.762762491689531,
53.1917784200664));
#148332=CARTESIAN_POINT('Ctrl Pts',(6.94887485033525,-0.952496408757991,
53.1831066238596));
#148333=CARTESIAN_POINT('Ctrl Pts',(6.91779140296513,-1.14095953809139,
53.1744348276527));
#148334=CARTESIAN_POINT('Ctrl Pts',(6.88670800059787,-1.32942239456645,
53.165763044001));
#148335=CARTESIAN_POINT('Ctrl Pts',(6.84791883692705,-1.51661418677696,
53.1570912603492));
#148336=CARTESIAN_POINT('Ctrl Pts',(6.80155333291305,-1.70191034488875,
53.1484194766975));
#148337=CARTESIAN_POINT('Ctrl Pts',(6.75518789508205,-1.88720623850532,
53.139747705424));
#148338=CARTESIAN_POINT('Ctrl Pts',(6.70124620748597,-2.07060622793696,
53.1310759341505));
#148339=CARTESIAN_POINT('Ctrl Pts',(6.63990824732571,-2.25149839653418,
53.122404162877));
#148340=CARTESIAN_POINT('Ctrl Pts',(6.57857037346951,-2.43239031061157,
53.113732403805));
#148341=CARTESIAN_POINT('Ctrl Pts',(6.50983633907179,-2.61077414196406,
53.1050606447329));
#148342=CARTESIAN_POINT('Ctrl Pts',(6.43393547556233,-2.78605471209748,
53.0963888856608));
#148343=CARTESIAN_POINT('Ctrl Pts',(6.35803471730007,-2.96133503917979,
53.0877171386133));
#148344=CARTESIAN_POINT('Ctrl Pts',(6.27496726266193,-3.1335118530473,53.0790453915659));
#148345=CARTESIAN_POINT('Ctrl Pts',(6.18501026583403,-3.30201068654051,
53.0703736445184));
#148346=CARTESIAN_POINT('Ctrl Pts',(6.09151188668825,-3.47714289832064,
53.0613605124454));
#148347=CARTESIAN_POINT('Ctrl Pts',(5.99057066119165,-3.64830137931007,
53.0523473803724));
#148348=CARTESIAN_POINT('Ctrl Pts',(5.88255038916588,-3.81486926138032,
53.0433342482994));
#148349=CARTESIAN_POINT('Ctrl Pts',(5.77621793389049,-3.97883452029324,
53.034461946415));
#148350=CARTESIAN_POINT('Ctrl Pts',(5.66302622906376,-4.13835132493741,
53.0255896445306));
#148351=CARTESIAN_POINT('Ctrl Pts',(5.54337059052903,-4.29286257158994,
53.0167173426463));
#148352=CARTESIAN_POINT('Ctrl Pts',(5.42558457134642,-4.44495958001353,
53.0079836704789));
#148353=CARTESIAN_POINT('Ctrl Pts',(5.30153533574937,-4.59220608124103,
52.9992499983114));
#148354=CARTESIAN_POINT('Ctrl Pts',(5.17164269972312,-4.73410375349976,
52.990516326144));
#148355=CARTESIAN_POINT('Ctrl Pts',(5.04265587431577,-4.87501189762002,
52.98184355853));
#148356=CARTESIAN_POINT('Ctrl Pts',(4.9079071016412,-5.01064538261968,52.973170790916));
#148357=CARTESIAN_POINT('Ctrl Pts',(4.7678460760923,-5.14055156157307,52.964498023302));
#148358=CARTESIAN_POINT('Ctrl Pts',(4.62778576967364,-5.27045707353532,
52.9558253002176));
#148359=CARTESIAN_POINT('Ctrl Pts',(4.48241347329788,-5.39463514506495,
52.9471525771331));
#148360=CARTESIAN_POINT('Ctrl Pts',(4.3322143300549,-5.51267136341058,52.9384798540486));
#148361=CARTESIAN_POINT('Ctrl Pts',(4.18201594573482,-5.63070698534541,
52.9298071747855));
#148362=CARTESIAN_POINT('Ctrl Pts',(4.02699098676462,-5.74260064062568,
52.9211344955224));
#148363=CARTESIAN_POINT('Ctrl Pts',(3.86765680431923,-5.84797891638668,
52.9124618162592));
#148364=CARTESIAN_POINT('Ctrl Pts',(3.70832341394854,-5.9533566682961,52.9037891801093));
#148365=CARTESIAN_POINT('Ctrl Pts',(3.54468107996522,-6.0522189487593,52.8951165439594));
#148366=CARTESIAN_POINT('Ctrl Pts',(3.37727590612859,-6.14423583665075,
52.8864439078095));
#148367=CARTESIAN_POINT('Ctrl Pts',(3.20987155082483,-6.23625227462273,
52.8777713140647));
#148368=CARTESIAN_POINT('Ctrl Pts',(3.0387046414804,-6.32142325013736,52.8690987203199));
#148369=CARTESIAN_POINT('Ctrl Pts',(2.86434638712907,-6.3994645351811,52.8604261265751));
#148370=CARTESIAN_POINT('Ctrl Pts',(2.68998897107704,-6.47750544500914,
52.8517535745274));
#148371=CARTESIAN_POINT('Ctrl Pts',(2.51244050005463,-6.5484166168872,52.8430810224797));
#148372=CARTESIAN_POINT('Ctrl Pts',(2.33229347360944,-6.61196141212718,
52.834408470432));
#148373=CARTESIAN_POINT('Ctrl Pts',(2.15214729859256,-6.6755059070356,52.8257359593734));
#148374=CARTESIAN_POINT('Ctrl Pts',(1.96940286066657,-6.73168400046413,
52.8170634483147));
#148375=CARTESIAN_POINT('Ctrl Pts',(1.78466999315593,-6.78030822146227,
52.808390937256));
#148376=CARTESIAN_POINT('Ctrl Pts',(1.59993798367095,-6.8289322166163,52.7997184664785));
#148377=CARTESIAN_POINT('Ctrl Pts',(1.41321783783529,-6.87000233723084,
52.7910459957009));
#148378=CARTESIAN_POINT('Ctrl Pts',(1.22513265045758,-6.9033815301838,52.7823735249233));
#148379=CARTESIAN_POINT('Ctrl Pts',(1.03704832132629,-6.93676057082506,
52.7737010937188));
#148380=CARTESIAN_POINT('Ctrl Pts',(0.847599242850681,-6.96244870438827,
52.7650286625143));
#148381=CARTESIAN_POINT('Ctrl Pts',(0.657417610665334,-6.98036020902124,
52.7563562313099));
#148382=CARTESIAN_POINT('Ctrl Pts',(0.467236830772413,-6.99827163338443,
52.7476838389706));
#148383=CARTESIAN_POINT('Ctrl Pts',(0.276323786585382,-7.0084064719186,
52.7390114466313));
#148384=CARTESIAN_POINT('Ctrl Pts',(0.085315553319391,-7.01073090475321,
52.7303390542921));
#148385=CARTESIAN_POINT('Ctrl Pts',(-0.10569183953708,-7.01305532736065,
52.7216667001101));
#148386=CARTESIAN_POINT('Ctrl Pts',(-0.296794136563897,-7.00756940957902,
52.7129943459281));
#148387=CARTESIAN_POINT('Ctrl Pts',(-0.487353636616802,-6.99429145770867,
52.7043219917462));
#148388=CARTESIAN_POINT('Ctrl Pts',(-0.677912313784566,-6.98101356317594,
52.6956496750137));
#148389=CARTESIAN_POINT('Ctrl Pts',(-0.867927915270643,-6.95994372163462,
52.6869773582812));
#148390=CARTESIAN_POINT('Ctrl Pts',(-1.05676637166343,-6.93115224174317,
52.6783050415487));
#148391=CARTESIAN_POINT('Ctrl Pts',(-1.24560402801217,-6.90236088383138,
52.6696327615579));
#148392=CARTESIAN_POINT('Ctrl Pts',(-1.43326426841352,-6.86584799585126,
52.660960481567));
#148393=CARTESIAN_POINT('Ctrl Pts',(-1.61912088843974,-6.82173541784773,
52.6522882015762));
#148394=CARTESIAN_POINT('Ctrl Pts',(-1.80497673622023,-6.77762302313468,
52.6436159576192));
#148395=CARTESIAN_POINT('Ctrl Pts',(-1.98902870222734,-6.72591106718914,
52.6349437136622));
#148396=CARTESIAN_POINT('Ctrl Pts',(-2.17066262760151,-6.66677210647208,
52.6262714697052));
#148397=CARTESIAN_POINT('Ctrl Pts',(-2.35229581309592,-6.6076333866556,
52.6175992610743));
#148398=CARTESIAN_POINT('Ctrl Pts',(-2.53151070755718,-6.54106781055492,
52.6089270524434));
#148399=CARTESIAN_POINT('Ctrl Pts',(-2.70770929770798,-6.46729749753371,
52.6002548438125));
#148400=CARTESIAN_POINT('Ctrl Pts',(-2.8839071844959,-6.39352747899442,
52.5915826698));
#148401=CARTESIAN_POINT('Ctrl Pts',(-3.05708852904455,-6.31255289079054,
52.5829104957875));
#148402=CARTESIAN_POINT('Ctrl Pts',(-3.22667545573855,-6.22464393084732,
52.574238321775));
#148403=CARTESIAN_POINT('Ctrl Pts',(-3.39626171929933,-6.1367353146532,
52.5655661816732));
#148404=CARTESIAN_POINT('Ctrl Pts',(-3.56225334094397,-6.04189251170717,
52.5568940415713));
#148405=CARTESIAN_POINT('Ctrl Pts',(-3.72409644022225,-5.94043199324965,
52.5482219014695));
#148406=CARTESIAN_POINT('Ctrl Pts',(-3.88593891985202,-5.83897186325391,
52.5395497945707));
#148407=CARTESIAN_POINT('Ctrl Pts',(-4.04363266823177,-5.73089421932567,
52.5308776876718));
#148408=CARTESIAN_POINT('Ctrl Pts',(-4.19665149726035,-5.61655969193264,
52.522205580773));
#148409=CARTESIAN_POINT('Ctrl Pts',(-4.34966975290987,-5.50222559296417,
52.5135335063696));
#148410=CARTESIAN_POINT('Ctrl Pts',(-4.49801289671993,-5.38163482746555,
52.5048614319661));
#148411=CARTESIAN_POINT('Ctrl Pts',(-4.64118594513171,-5.255189776327,52.4961893575627));
#148412=CARTESIAN_POINT('Ctrl Pts',(-4.78435846873845,-5.12874518867653,
52.487517314947));
#148413=CARTESIAN_POINT('Ctrl Pts',(-4.92236072197161,-4.99644654635204,
52.4788452723313));
#148414=CARTESIAN_POINT('Ctrl Pts',(-5.05473222958171,-4.85873529323506,
52.4701732297156));
#148415=CARTESIAN_POINT('Ctrl Pts',(-5.18710326277897,-4.7210245336683,
52.46150121818));
#148416=CARTESIAN_POINT('Ctrl Pts',(-5.3138433939023,-4.57790140690153,
52.4528292066445));
#148417=CARTESIAN_POINT('Ctrl Pts',(-5.43452972930885,-4.42984347169945,
52.444157195109));
#148418=CARTESIAN_POINT('Ctrl Pts',(-5.55521564202676,-4.28178605505159,
52.4354852139461));
#148419=CARTESIAN_POINT('Ctrl Pts',(-5.66984762200097,-4.1287940847108,
52.4268132327831));
#148420=CARTESIAN_POINT('Ctrl Pts',(-5.77804317951857,-3.971378045228,52.4181412516202));
#148421=CARTESIAN_POINT('Ctrl Pts',(-5.88623836692132,-3.81396254423323,
52.4094693001224));
#148422=CARTESIAN_POINT('Ctrl Pts',(-5.98799701504699,-3.65212323844896,
52.4007973486246));
#148423=CARTESIAN_POINT('Ctrl Pts',(-6.08297959063358,-3.48640012942223,
52.3921253971267));
#148424=CARTESIAN_POINT('Ctrl Pts',(-6.17796184905218,-3.3206775737819,
52.3834534745865));
#148425=CARTESIAN_POINT('Ctrl Pts',(-6.26616793897898,-3.15107148726813,
52.3747815520462));
#148426=CARTESIAN_POINT('Ctrl Pts',(-6.34730354929467,-2.97814778270175,
52.3661096295059));
#148427=CARTESIAN_POINT('Ctrl Pts',(-6.42843889529886,-2.80522464146042,
52.3574377352158));
#148428=CARTESIAN_POINT('Ctrl Pts',(-6.50250368714325,-2.62898416091396,
52.3487658409256));
#148429=CARTESIAN_POINT('Ctrl Pts',(-6.56925079960179,-2.4500143865764,
52.3400939466354));
#148430=CARTESIAN_POINT('Ctrl Pts',(-6.63599770006617,-2.2710451806611,
52.3314220798879));
#148431=CARTESIAN_POINT('Ctrl Pts',(-6.69542686840853,-2.08934696440795,
52.3227502131404));
#148432=CARTESIAN_POINT('Ctrl Pts',(-6.74734001400929,-1.90552598981205,
52.3140783463928));
#148433=CARTESIAN_POINT('Ctrl Pts',(-6.79925299896423,-1.7217055840522,
52.3054065064805));
#148434=CARTESIAN_POINT('Ctrl Pts',(-6.84364993053248,-1.53576270641118,
52.2967346665681));
#148435=CARTESIAN_POINT('Ctrl Pts',(-6.88038267538351,-1.34831776773224,
52.2880628266558));
#148436=CARTESIAN_POINT('Ctrl Pts',(-6.91711530956076,-1.1608733938148,
52.2793910128712));
#148437=CARTESIAN_POINT('Ctrl Pts',(-6.94618374861406,-0.971927246617174,
52.2707191990867));
#148438=CARTESIAN_POINT('Ctrl Pts',(-6.96749100433688,-0.782109753797198,
52.2620473853021));
#148439=CARTESIAN_POINT('Ctrl Pts',(-6.98879819760004,-0.592292817404362,
52.2533755969379));
#148440=CARTESIAN_POINT('Ctrl Pts',(-7.00234422137968,-0.401604822726262,
52.2447038085737));
#148441=CARTESIAN_POINT('Ctrl Pts',(-7.00808387899857,-0.210682005449926,
52.2360320202095));
#148442=CARTESIAN_POINT('Ctrl Pts',(-7.01382352026046,-0.0197597322696063,
52.2273602565584));
#148443=CARTESIAN_POINT('Ctrl Pts',(-7.01175683134598,0.171397078303853,
52.2186884929073));
#148444=CARTESIAN_POINT('Ctrl Pts',(-7.00189070777973,0.362150629997999,
52.2100167292562));
#148445=CARTESIAN_POINT('Ctrl Pts',(-6.99157808297264,0.561536923513271,
52.2009525163108));
#148446=CARTESIAN_POINT('Ctrl Pts',(-6.97274368607548,0.760482277943844,
52.1918883033654));
#148447=CARTESIAN_POINT('Ctrl Pts',(-6.94545616842832,0.958261537859603,
52.1828240904201));
#148448=CARTESIAN_POINT('Ctrl Pts',(-6.91902138570762,1.14986019590305,
52.1740431341293));
#148449=CARTESIAN_POINT('Ctrl Pts',(-6.88465388689313,1.34036422799509,
52.1652621778384));
#148450=CARTESIAN_POINT('Ctrl Pts',(-6.84247124235259,1.52912192452984,
52.1564812215476));
#148451=CARTESIAN_POINT('Ctrl Pts',(-6.80080846652329,1.71555332736007,
52.1478084838021));
#148452=CARTESIAN_POINT('Ctrl Pts',(-6.75152215882549,1.90028091508584,
52.1391357460566));
#148453=CARTESIAN_POINT('Ctrl Pts',(-6.69477680033957,2.08268820425313,
52.1304630083111));
#148454=CARTESIAN_POINT('Ctrl Pts',(-6.6380320137316,2.26509365512544,52.1217903579692));
#148455=CARTESIAN_POINT('Ctrl Pts',(-6.57382841116684,2.44517858291594,
52.1131177076273));
#148456=CARTESIAN_POINT('Ctrl Pts',(-6.50238025225956,2.62234201002176,
52.1044450572854));
#148457=CARTESIAN_POINT('Ctrl Pts',(-6.43093279007722,2.79950370952282,
52.0957724915146));
#148458=CARTESIAN_POINT('Ctrl Pts',(-6.35224101918992,2.97374370184175,
52.0870999257439));
#148459=CARTESIAN_POINT('Ctrl Pts',(-6.26656754386446,3.14448052636435,
52.0784273599731));
#148460=CARTESIAN_POINT('Ctrl Pts',(-6.18089487601213,3.31521574169113,
52.0697548759413));
#148461=CARTESIAN_POINT('Ctrl Pts',(-6.08824076282231,3.48244760135432,
52.0610823919095));
#148462=CARTESIAN_POINT('Ctrl Pts',(-5.98891439681922,3.64561804226272,
52.0524099078778));
#148463=CARTESIAN_POINT('Ctrl Pts',(-5.88958893454311,3.80878699855495,
52.0437375027531));
#148464=CARTESIAN_POINT('Ctrl Pts',(-5.78359148866003,3.96789436736326,
52.0350650976284));
#148465=CARTESIAN_POINT('Ctrl Pts',(-5.67127577279305,4.12240920717856,
52.0263926925038));
#148466=CARTESIAN_POINT('Ctrl Pts',(-5.55896104217497,4.27692269156845,
52.0177203634547));
#148467=CARTESIAN_POINT('Ctrl Pts',(-5.44032831951973,4.42684349778754,
52.0090480344055));
#148468=CARTESIAN_POINT('Ctrl Pts',(-5.315773475448,4.57167134866708,52.0003757053564));
#148469=CARTESIAN_POINT('Ctrl Pts',(-5.19121968333332,4.71649797636917,
51.9917034495515));
#148470=CARTESIAN_POINT('Ctrl Pts',(-5.06074405512257,4.85623151942566,
51.9830311937465));
#148471=CARTESIAN_POINT('Ctrl Pts',(-4.92478197318899,4.9904057028515,51.9743589379416));
#148472=CARTESIAN_POINT('Ctrl Pts',(-4.78882099517946,5.12457879686986,
51.9656867525497));
#148473=CARTESIAN_POINT('Ctrl Pts',(-4.64737385477877,5.25319242205333,
51.9570145671579));
#148474=CARTESIAN_POINT('Ctrl Pts',(-4.5009125373951,5.37581741628374,51.948342381766));
#148475=CARTESIAN_POINT('Ctrl Pts',(-4.35445236138306,5.49844145489876,
51.9396702639564));
#148476=CARTESIAN_POINT('Ctrl Pts',(-4.20297830437828,5.61507677360063,
51.9309981461468));
#148477=CARTESIAN_POINT('Ctrl Pts',(-4.04699580205975,5.7253341859328,51.9223260283373));
#148478=CARTESIAN_POINT('Ctrl Pts',(-3.89101446440741,5.83559077501185,
51.9136539752793));
#148479=CARTESIAN_POINT('Ctrl Pts',(-3.73052498075225,5.93946938906285,
51.9049819222214));
#148480=CARTESIAN_POINT('Ctrl Pts',(-3.56606286128402,6.0366234131235,51.8963098691634));
#148481=CARTESIAN_POINT('Ctrl Pts',(-3.40160191612828,6.13377674347314,
51.8876378780267));
#148482=CARTESIAN_POINT('Ctrl Pts',(-3.2331686364727,6.22420543545189,51.87896588689));
#148483=CARTESIAN_POINT('Ctrl Pts',(-3.06132503079727,6.30760775717023,
51.8702938957533));
#148484=CARTESIAN_POINT('Ctrl Pts',(-2.88948259606659,6.39100951058399,
51.8616219637077));
#148485=CARTESIAN_POINT('Ctrl Pts',(-2.71423013733688,6.46738486553251,
51.852950031662));
#148486=CARTESIAN_POINT('Ctrl Pts',(-2.53615240856665,6.53647898512812,
51.8442780996164));
#148487=CARTESIAN_POINT('Ctrl Pts',(-2.35807583511529,6.60557265646028,
51.8356062238319));
#148488=CARTESIAN_POINT('Ctrl Pts',(-2.17717429308471,6.66738508423366,
51.8269343480473));
#148489=CARTESIAN_POINT('Ctrl Pts',(-1.99405137755352,6.72171002544568,
51.8182624722628));
#148490=CARTESIAN_POINT('Ctrl Pts',(-1.81092959032436,6.77603463193748,
51.8095906499095));
#148491=CARTESIAN_POINT('Ctrl Pts',(-1.62558672926026,6.82287176341322,
51.8009188275563));
#148492=CARTESIAN_POINT('Ctrl Pts',(-1.43864120070719,6.86206514528446,
51.7922470052031));
#148493=CARTESIAN_POINT('Ctrl Pts',(-1.25169676301637,6.90125829845495,
51.7835752334515));
#148494=CARTESIAN_POINT('Ctrl Pts',(-1.06314995450457,6.93280773300226,
51.7749034617));
#148495=CARTESIAN_POINT('Ctrl Pts',(-0.873629864324986,6.95660818378177,
51.7662316899485));
#148496=CARTESIAN_POINT('Ctrl Pts',(-0.67949550971221,6.98098810649707,
51.75734878571));
#148497=CARTESIAN_POINT('Ctrl Pts',(-0.484340182087299,6.99723686027479,
51.7484658814715));
#148498=CARTESIAN_POINT('Ctrl Pts',(-0.288847078972072,7.00529756166498,
51.739582977233));
#148499=CARTESIAN_POINT('Ctrl Pts',(-0.0979805523976308,7.01316749698026,
51.7309102974767));
#148500=CARTESIAN_POINT('Ctrl Pts',(0.093207647885845,7.01323255451608,
51.7222376177203));
#148501=CARTESIAN_POINT('Ctrl Pts',(0.284079486223013,7.00549251716161,
51.713564937964));
#148502=CARTESIAN_POINT('Ctrl Pts',(0.474947621914736,6.99775262995299,
51.7048924264455));
#148503=CARTESIAN_POINT('Ctrl Pts',(0.665499124050418,6.9822079623472,51.6962199149269));
#148504=CARTESIAN_POINT('Ctrl Pts',(0.85509810641837,6.95891038819295,51.6875474034084));
#148505=CARTESIAN_POINT('Ctrl Pts',(1.04469365841483,6.93561323555644,51.6788750487996));
#148506=CARTESIAN_POINT('Ctrl Pts',(1.23333644315321,6.90456349171677,51.6702026941909));
#148507=CARTESIAN_POINT('Ctrl Pts',(1.42039696672693,6.86586476850607,51.6615303395821));
#148508=CARTESIAN_POINT('Ctrl Pts',(1.60745435009168,6.8271666949358,51.6528581305573));
#148509=CARTESIAN_POINT('Ctrl Pts',(1.79292924726155,6.78081995649372,51.6441859215325));
#148510=CARTESIAN_POINT('Ctrl Pts',(1.97620275621103,6.72697920532269,51.6355137125076));
#148511=CARTESIAN_POINT('Ctrl Pts',(2.15947342778489,6.67313928769513,51.6268416377429));
#148512=CARTESIAN_POINT('Ctrl Pts',(2.34054250680423,6.61180566956803,51.6181695629781));
#148513=CARTESIAN_POINT('Ctrl Pts',(2.51880581148969,6.54318300573244,51.6094974882134));
#148514=CARTESIAN_POINT('Ctrl Pts',(2.69706658905806,6.47456131471348,51.6008255363867));
#148515=CARTESIAN_POINT('Ctrl Pts',(2.87252140681914,6.39865088680132,51.59215358456));
#148516=CARTESIAN_POINT('Ctrl Pts',(3.04458483294752,6.31570500874494,51.5834816327333));
#148517=CARTESIAN_POINT('Ctrl Pts',(3.21664604442681,6.23276019829495,51.5748097925244));
#148518=CARTESIAN_POINT('Ctrl Pts',(3.38531569578744,6.14278024223816,51.5661379523155));
#148519=CARTESIAN_POINT('Ctrl Pts',(3.55003100942206,6.04606536473447,51.5574661121065));
#148520=CARTESIAN_POINT('Ctrl Pts',(3.72225670716014,5.94494066119492,51.548398869373));
#148521=CARTESIAN_POINT('Ctrl Pts',(3.89015872998584,5.8364526481967,51.5393316266394));
#148522=CARTESIAN_POINT('Ctrl Pts',(4.05312466659795,5.72099702844839,51.5302643839059));
#148523=CARTESIAN_POINT('Ctrl Pts',(4.20899688867971,5.61056705531338,51.5215918275275));
#148524=CARTESIAN_POINT('Ctrl Pts',(4.36035338103854,5.49376336253657,51.512919271149));
#148525=CARTESIAN_POINT('Ctrl Pts',(4.50668904925033,5.37097573778426,51.5042467147706));
#148526=CARTESIAN_POINT('Ctrl Pts',(4.65301950884067,5.24819248349244,51.4955744670802));
#148527=CARTESIAN_POINT('Ctrl Pts',(4.79432928426973,5.11942590603987,51.4869022193897));
#148528=CARTESIAN_POINT('Ctrl Pts',(4.93014684172531,4.98510568408795,51.4782299716993));
#148529=CARTESIAN_POINT('Ctrl Pts',(5.06596027419871,4.85078954164189,51.469557987398));
#148530=CARTESIAN_POINT('Ctrl Pts',(5.19628162053444,4.71092029195547,51.4608860030966));
#148531=CARTESIAN_POINT('Ctrl Pts',(5.32067604038165,4.56596463365724,51.4522140187953));
#148532=CARTESIAN_POINT('Ctrl Pts',(5.44506733164383,4.42101262106999,51.443542252599));
#148533=CARTESIAN_POINT('Ctrl Pts',(5.56353180975687,4.27097467138573,51.4348704864026));
#148534=CARTESIAN_POINT('Ctrl Pts',(5.67567421678232,4.11635138775256,51.4261987202062));
#148535=CARTESIAN_POINT('Ctrl Pts',(5.78782406006177,3.96171785092399,51.417526378978));
#148536=CARTESIAN_POINT('Ctrl Pts',(5.8936508265435,3.80249860162274,51.4088540377498));
#148537=CARTESIAN_POINT('Ctrl Pts',(5.99280137736038,3.6392249468819,51.4001816965216));
#148538=CARTESIAN_POINT('Ctrl Pts',(6.09194609290926,3.47596090122063,51.3915098656832));
#148539=CARTESIAN_POINT('Ctrl Pts',(6.18441523160539,3.3086431703667,51.3828380348449));
#148540=CARTESIAN_POINT('Ctrl Pts',(6.2699002646301,3.13783001994872,51.3741662040065));
#148541=CARTESIAN_POINT('Ctrl Pts',(6.35538670852435,2.96701405038144,51.3654942300458));
#148542=CARTESIAN_POINT('Ctrl Pts',(6.43388868897073,2.79270279979511,51.356822256085));
#148543=CARTESIAN_POINT('Ctrl Pts',(6.50514427077325,2.61547788729441,51.3481502821243));
#148544=CARTESIAN_POINT('Ctrl Pts',(6.52787183386237,2.55895052090526,51.3453842835833));
#148545=CARTESIAN_POINT('Ctrl Pts',(6.5498625512973,2.50212689663976,51.3426182850424));
#148546=CARTESIAN_POINT('Ctrl Pts',(6.57110895151816,2.4450263208763,51.3398522865015));
#148547=CARTESIAN_POINT('Origin',(0.,0.,50.));
#148548=CARTESIAN_POINT('',(6.57110895151812,2.44502632087642,49.3398351631816));
#148549=CARTESIAN_POINT('',(6.57110895151815,2.44502632087633,49.8869210003222));
#148550=CARTESIAN_POINT('',(6.57110895151814,2.44502632087636,50.));
#148551=CARTESIAN_POINT('',(7.01125,3.46460097481842E-12,51.7735343569105));
#148552=CARTESIAN_POINT('Ctrl Pts',(6.57110895151815,2.44502632087633,49.8869210003222));
#148553=CARTESIAN_POINT('Ctrl Pts',(6.50449838733148,2.62404495591329,49.895592809261));
#148554=CARTESIAN_POINT('Ctrl Pts',(6.43056821795871,2.80033990715968,49.9042646181997));
#148555=CARTESIAN_POINT('Ctrl Pts',(6.34956511459254,2.97332295892145,49.9129364271385));
#148556=CARTESIAN_POINT('Ctrl Pts',(6.26856213015516,3.14630575670943,49.9216082233453));
#148557=CARTESIAN_POINT('Ctrl Pts',(6.18048635294282,3.31597640754664,49.9302800195521));
#148558=CARTESIAN_POINT('Ctrl Pts',(6.08563165071566,3.48176879966316,49.938951815759));
#148559=CARTESIAN_POINT('Ctrl Pts',(5.99077708581972,3.64756095174443,49.9476235994107));
#148560=CARTESIAN_POINT('Ctrl Pts',(5.88914375658112,3.80947460983729,49.9562953830624));
#148561=CARTESIAN_POINT('Ctrl Pts',(5.78107076500233,3.96696954519888,49.9649671667142));
#148562=CARTESIAN_POINT('Ctrl Pts',(5.67299792768882,4.12446425574944,49.9736389379876));
#148563=CARTESIAN_POINT('Ctrl Pts',(5.55848560711395,4.27754002202474,49.9823107092611));
#148564=CARTESIAN_POINT('Ctrl Pts',(5.43791587524921,4.42568610457323,49.9909824805346));
#148565=CARTESIAN_POINT('Ctrl Pts',(5.31734631302949,4.573831978676,49.9996542396066));
#148566=CARTESIAN_POINT('Ctrl Pts',(5.19071953583903,4.71704796266761,50.0083259986787));
#148567=CARTESIAN_POINT('Ctrl Pts',(5.05845803451681,4.85485621574237,50.0169977577508));
#148568=CARTESIAN_POINT('Ctrl Pts',(4.9261967165929,4.99266427772752,50.0256695047983));
#148569=CARTESIAN_POINT('Ctrl Pts',(4.78830088681858,5.12506441890826,50.0343412518457));
#148570=CARTESIAN_POINT('Ctrl Pts',(4.64523063400523,5.25161488681333,50.0430129988932));
#148571=CARTESIAN_POINT('Ctrl Pts',(4.49652806262455,5.38314733060835,50.0520261309662));
#148572=CARTESIAN_POINT('Ctrl Pts',(4.34223563524025,5.50835996364214,50.0610392630393));
#148573=CARTESIAN_POINT('Ctrl Pts',(4.18290943344624,5.62680151010203,50.0700523951123));
#148574=CARTESIAN_POINT('Ctrl Pts',(4.0260727035553,5.74339240739846,50.0789246969966));
#148575=CARTESIAN_POINT('Ctrl Pts',(3.8643586282048,5.85342208902574,50.087796998881));
#148576=CARTESIAN_POINT('Ctrl Pts',(3.69833198496549,5.95650628233373,50.0966693007654));
#148577=CARTESIAN_POINT('Ctrl Pts',(3.5348995080268,6.05797978512129,50.1054029729328));
#148578=CARTESIAN_POINT('Ctrl Pts',(3.36728850947182,6.15272311279854,50.1141366451002));
#148579=CARTESIAN_POINT('Ctrl Pts',(3.19606623001071,6.24041562845658,50.1228703172676));
#148580=CARTESIAN_POINT('Ctrl Pts',(3.02603797481211,6.32749661743909,50.1315430848816));
#148581=CARTESIAN_POINT('Ctrl Pts',(2.85244891335465,6.40762471321549,50.1402158524956));
#148582=CARTESIAN_POINT('Ctrl Pts',(2.67587836095273,6.48053250588908,50.1488886201096));
#148583=CARTESIAN_POINT('Ctrl Pts',(2.49930871513574,6.55343992422444,50.1575613431941));
#148584=CARTESIAN_POINT('Ctrl Pts',(2.31975787165094,6.6191270051938,50.1662340662785));
#148585=CARTESIAN_POINT('Ctrl Pts',(2.137825035802,6.6773745348601,50.174906789363));
#148586=CARTESIAN_POINT('Ctrl Pts',(1.95589311921941,6.73562177021454,50.1835794686261));
#148587=CARTESIAN_POINT('Ctrl Pts',(1.77157950497145,6.78642944284865,50.1922521478893));
#148588=CARTESIAN_POINT('Ctrl Pts',(1.58549928668899,6.82962799678055,50.2009248271524));
#148589=CARTESIAN_POINT('Ctrl Pts',(1.39941999343982,6.87282633596582,50.2095974633023));
#148590=CARTESIAN_POINT('Ctrl Pts',(1.21157439050756,6.90841556788897,50.2182700994522));
#148591=CARTESIAN_POINT('Ctrl Pts',(1.02258935229219,6.93627692491286,50.2269427356021));
#148592=CARTESIAN_POINT('Ctrl Pts',(0.833605238125191,6.96413814570776,
50.2356153293469));
#148593=CARTESIAN_POINT('Ctrl Pts',(0.643481980916576,6.98427152577614,
50.2442879230917));
#148594=CARTESIAN_POINT('Ctrl Pts',(0.452854049808002,6.99660987708137,
50.2529605168364));
#148595=CARTESIAN_POINT('Ctrl Pts',(0.262227035221766,7.00894816906488,
50.2616330688842));
#148596=CARTESIAN_POINT('Ctrl Pts',(0.0710956351219621,7.01349148893087,
50.2703056209319));
#148597=CARTESIAN_POINT('Ctrl Pts',(-0.119902323156486,7.01022467510148,
50.2789781729796));
#148598=CARTESIAN_POINT('Ctrl Pts',(-0.310899378721912,7.00695787671203,
50.2876506840382));
#148599=CARTESIAN_POINT('Ctrl Pts',(-0.501762709652217,6.99588102335287,
50.2963231950969));
#148600=CARTESIAN_POINT('Ctrl Pts',(-0.691855389204572,6.97703107940108,
50.3049957061555));
#148601=CARTESIAN_POINT('Ctrl Pts',(-0.881947185836504,6.95818122300132,
50.3136681769331));
#148602=CARTESIAN_POINT('Ctrl Pts',(-1.07126805552919,6.93155837629142,
50.3223406477107));
#148603=CARTESIAN_POINT('Ctrl Pts',(-1.25918622472362,6.89725138109133,
50.3310131184883));
#148604=CARTESIAN_POINT('Ctrl Pts',(-1.44710353643389,6.86294454243654,
50.3396855496928));
#148605=CARTESIAN_POINT('Ctrl Pts',(-1.63361788096937,6.82095367648074,
50.3483579808972));
#148606=CARTESIAN_POINT('Ctrl Pts',(-1.81810685596554,6.77141890764344,
50.3570304121017));
#148607=CARTESIAN_POINT('Ctrl Pts',(-2.00259500418079,6.72188436079449,
50.365702804441));
#148608=CARTESIAN_POINT('Ctrl Pts',(-2.18505752664021,6.66480605238715,
50.3743751967802));
#148609=CARTESIAN_POINT('Ctrl Pts',(-2.36488554744824,6.60037445225424,
50.3830475891195));
#148610=CARTESIAN_POINT('Ctrl Pts',(-2.54471277703807,6.53594313561138,
50.3917199433015));
#148611=CARTESIAN_POINT('Ctrl Pts',(-2.7219052607291,6.46415868780939,50.4003922974834));
#148612=CARTESIAN_POINT('Ctrl Pts',(-2.89587171389858,6.38526065083815,
50.4090646516654));
#148613=CARTESIAN_POINT('Ctrl Pts',(-3.06983741583593,6.30636295456905,
50.4177369683979));
#148614=CARTESIAN_POINT('Ctrl Pts',(-3.24057685640759,6.22035184793775,
50.4264092851304));
#148615=CARTESIAN_POINT('Ctrl Pts',(-3.40752028946761,6.12751434428077,
50.4350816018628));
#148616=CARTESIAN_POINT('Ctrl Pts',(-3.57446301524526,6.03467723394461,
50.4437538818537));
#148617=CARTESIAN_POINT('Ctrl Pts',(-3.73760951742141,5.93501392252171,
50.4524261618445));
#148618=CARTESIAN_POINT('Ctrl Pts',(-3.89641539158832,5.82885697703192,
50.4610984418354));
#148619=CARTESIAN_POINT('Ctrl Pts',(-4.05522060590707,5.72270047263075,
50.4697706857923));
#148620=CARTESIAN_POINT('Ctrl Pts',(-4.20968499214109,5.61005054602573,
50.4784429297493));
#148621=CARTESIAN_POINT('Ctrl Pts',(-4.35929312155931,5.49128309621947,
50.4871151737063));
#148622=CARTESIAN_POINT('Ctrl Pts',(-4.50890064155372,5.37251613020852,
50.4957873823372));
#148623=CARTESIAN_POINT('Ctrl Pts',(-4.65365172183319,5.24763186748397,
50.5044595909681));
#148624=CARTESIAN_POINT('Ctrl Pts',(-4.79306334970965,5.11704702813743,
50.513131799599));
#148625=CARTESIAN_POINT('Ctrl Pts',(-4.93247442107221,4.98646271006935,
50.5218039736115));
#148626=CARTESIAN_POINT('Ctrl Pts',(-5.06654587536628,4.85017805510816,
50.530476147624));
#148627=CARTESIAN_POINT('Ctrl Pts',(-5.19483033978528,4.70864782112088,
50.5391483216365));
#148628=CARTESIAN_POINT('Ctrl Pts',(-5.3231143025755,4.56711814055711,50.5478204617383));
#148629=CARTESIAN_POINT('Ctrl Pts',(-5.44561113000544,4.42034313247858,
50.5564926018401));
#148630=CARTESIAN_POINT('Ctrl Pts',(-5.56191207495125,4.26881255538487,
50.565164741942));
#148631=CARTESIAN_POINT('Ctrl Pts',(-5.67821257461588,4.11728255845596,
50.5738368488408));
#148632=CARTESIAN_POINT('Ctrl Pts',(-5.78831706632212,3.96099725428024,
50.5825089557396));
#148633=CARTESIAN_POINT('Ctrl Pts',(-5.89185815647313,3.80047813130152,
50.5911810626385));
#148634=CARTESIAN_POINT('Ctrl Pts',(-5.99539885864389,3.63995960980621,
50.5998531370419));
#148635=CARTESIAN_POINT('Ctrl Pts',(-6.09237605450623,3.47520753995041,
50.6085252114454));
#148636=CARTESIAN_POINT('Ctrl Pts',(-6.18246615568055,3.30677165772973,
50.6171972858489));
#148637=CARTESIAN_POINT('Ctrl Pts',(-6.27255592662674,3.13833639291612,
50.6258693284645));
#148638=CARTESIAN_POINT('Ctrl Pts',(-6.35575851943845,2.96621759322332,
50.6345413710802));
#148639=CARTESIAN_POINT('Ctrl Pts',(-6.43179631013648,2.79098957135543,
50.6432134136959));
#148640=CARTESIAN_POINT('Ctrl Pts',(-6.50783382831893,2.61576217749586,
50.6518854252315));
#148641=CARTESIAN_POINT('Ctrl Pts',(-6.57670648270601,2.43742584432079,
50.660557436767));
#148642=CARTESIAN_POINT('Ctrl Pts',(-6.63818446599478,2.25657562645829,
50.6692294483026));
#148643=CARTESIAN_POINT('Ctrl Pts',(-6.69966223396472,2.07572604200071,
50.6779014294655));
#148644=CARTESIAN_POINT('Ctrl Pts',(-6.75374529124755,1.89236285939156,
50.6865734106284));
#148645=CARTESIAN_POINT('Ctrl Pts',(-6.80025318023398,1.70709790205998,
50.6952453917913));
#148646=CARTESIAN_POINT('Ctrl Pts',(-6.84676091012637,1.52183357848221,
50.7039173432891));
#148647=CARTESIAN_POINT('Ctrl Pts',(-6.88569345442289,1.33466776867811,
50.712589294787));
#148648=CARTESIAN_POINT('Ctrl Pts',(-6.9169209087468,1.14622497994126,50.7212612462848));
#148649=CARTESIAN_POINT('Ctrl Pts',(-6.94814825879533,0.957782820456561,
50.7299331688251));
#148650=CARTESIAN_POINT('Ctrl Pts',(-6.97167052392505,0.768063970771273,
50.7386050913653));
#148651=CARTESIAN_POINT('Ctrl Pts',(-6.98740921903153,0.57770145256284,
50.7472770139056));
#148652=CARTESIAN_POINT('Ctrl Pts',(-7.00314786286684,0.387339554488891,
50.7559489081958));
#148653=CARTESIAN_POINT('Ctrl Pts',(-7.01110296401745,0.19633427513781,
50.764620802486));
#148654=CARTESIAN_POINT('Ctrl Pts',(-7.01124797942393,0.00532292437921427,
50.7732926967761));
#148655=CARTESIAN_POINT('Ctrl Pts',(-7.01139299436982,-0.185687819711979,
50.7819645635237));
#148656=CARTESIAN_POINT('Ctrl Pts',(-7.00372797299438,-0.376704351160972,
50.7906364302712));
#148657=CARTESIAN_POINT('Ctrl Pts',(-6.98827849031203,-0.567089326598777,
50.7993082970188));
#148658=CARTESIAN_POINT('Ctrl Pts',(-6.97282905543826,-0.757473712888272,
50.8079801369311));
#148659=CARTESIAN_POINT('Ctrl Pts',(-6.94959523043372,-0.947226264001188,
50.8166519768435));
#148660=CARTESIAN_POINT('Ctrl Pts',(-6.91865453650893,-1.13571385786402,
50.8253238167558));
#148661=CARTESIAN_POINT('Ctrl Pts',(-6.88771393580689,-1.32420088382328,
50.8339956305404));
#148662=CARTESIAN_POINT('Ctrl Pts',(-6.84906655865514,-1.51142267990746,
50.8426674443249));
#148663=CARTESIAN_POINT('Ctrl Pts',(-6.80284135383523,-1.69675457183686,
50.8513392581095));
#148664=CARTESIAN_POINT('Ctrl Pts',(-6.75661628451883,-1.88208592048857,
50.8600110464737));
#148665=CARTESIAN_POINT('Ctrl Pts',(-6.70281350071472,-2.06552710051522,
50.8686828348379));
#148666=CARTESIAN_POINT('Ctrl Pts',(-6.64161251687621,-2.24646605542423,
50.877354623202));
#148667=CARTESIAN_POINT('Ctrl Pts',(-6.58041170744959,-2.42740449468945,
50.8860263868532));
#148668=CARTESIAN_POINT('Ctrl Pts',(-6.51181283117328,-2.60584045408488,
50.8946981505043));
#148669=CARTESIAN_POINT('Ctrl Pts',(-6.4360447687628,-2.78117858056274,
50.9033699141555));
#148670=CARTESIAN_POINT('Ctrl Pts',(-6.35684774728306,-2.96445180845203,
50.9124341271008));
#148671=CARTESIAN_POINT('Ctrl Pts',(-6.26981768815725,-3.14433998862126,
50.9214983400462));
#148672=CARTESIAN_POINT('Ctrl Pts',(-6.17527181578168,-3.32018742900344,
50.9305625529916));
#148673=CARTESIAN_POINT('Ctrl Pts',(-6.08368050191785,-3.49053963687367,
50.9393435092824));
#148674=CARTESIAN_POINT('Ctrl Pts',(-5.98503618716671,-3.65709956718525,
50.9481244655732));
#148675=CARTESIAN_POINT('Ctrl Pts',(-5.87967633130162,-3.81929742251524,
50.956905421864));
#148676=CARTESIAN_POINT('Ctrl Pts',(-5.77561495477753,-3.97949631379415,
50.9655781596095));
#148677=CARTESIAN_POINT('Ctrl Pts',(-5.66500279405277,-4.13543980257547,
50.974250897355));
#148678=CARTESIAN_POINT('Ctrl Pts',(-5.54820899034624,-4.28660746534379,
50.9829236351005));
#148679=CARTESIAN_POINT('Ctrl Pts',(-5.43141636368402,-4.43777360464914,
50.9915962854424));
#148680=CARTESIAN_POINT('Ctrl Pts',(-5.3084423924273,-4.58416378940542,
51.0002689357843));
#148681=CARTESIAN_POINT('Ctrl Pts',(-5.1796974640714,-4.72528948776605,
51.0089415861262));
#148682=CARTESIAN_POINT('Ctrl Pts',(-5.05095379116855,-4.86641380994285,
51.017614151897));
#148683=CARTESIAN_POINT('Ctrl Pts',(-4.91643946526993,-5.00227353854812,
51.0262867176678));
#148684=CARTESIAN_POINT('Ctrl Pts',(-4.7766033774798,-5.13241529270076,
51.0349592834386));
#148685=CARTESIAN_POINT('Ctrl Pts',(-4.63676860764581,-5.26255582026642,
51.0436317674703));
#148686=CARTESIAN_POINT('Ctrl Pts',(-4.49161238427032,-5.38697828766175,
51.0523042515021));
#148687=CARTESIAN_POINT('Ctrl Pts',(-4.34161910267662,-5.50526748939354,
51.0609767355339));
#148688=CARTESIAN_POINT('Ctrl Pts',(-4.19162718580574,-5.62355561486398,
51.0696491406585));
#148689=CARTESIAN_POINT('Ctrl Pts',(-4.03679852186387,-5.73571041041401,
51.0783215457832));
#148690=CARTESIAN_POINT('Ctrl Pts',(-3.87764977431607,-5.84135761533623,
51.0869939509079));
#148691=CARTESIAN_POINT('Ctrl Pts',(-3.7185024228429,-5.94700389350669,
51.095666279957));
#148692=CARTESIAN_POINT('Ctrl Pts',(-3.55503530028467,-6.04614253816448,
51.1043386090061));
#148693=CARTESIAN_POINT('Ctrl Pts',(-3.38779388709415,-6.13844272931397,
51.1130109380553));
#148694=CARTESIAN_POINT('Ctrl Pts',(-3.2205538863803,-6.23074214092049,
51.1216831938602));
#148695=CARTESIAN_POINT('Ctrl Pts',(-3.04953990753596,-6.31620307732955,
51.1303554496652));
#148696=CARTESIAN_POINT('Ctrl Pts',(-2.8753226048127,-6.39454036508904,
51.1390277054701));
#148697=CARTESIAN_POINT('Ctrl Pts',(-2.70110671662106,-6.47287701680052,
51.147699890862));
#148698=CARTESIAN_POINT('Ctrl Pts',(-2.52368781567611,-6.54409001910944,
51.1563720762538));
#148699=CARTESIAN_POINT('Ctrl Pts',(-2.34365791912394,-6.60794174615876,
51.1650442616456));
#148700=CARTESIAN_POINT('Ctrl Pts',(-2.16362942554312,-6.67179297561215,
51.1737163794552));
#148701=CARTESIAN_POINT('Ctrl Pts',(-1.9809902447871,-6.72828294965083,
51.1823884972648));
#148702=CARTESIAN_POINT('Ctrl Pts',(-1.79634980371192,-6.77722317363123,
51.1910606150744));
#148703=CARTESIAN_POINT('Ctrl Pts',(-1.61171074128151,-6.82616303219231,
51.1997326681323));
#148704=CARTESIAN_POINT('Ctrl Pts',(-1.42507072299637,-6.86755318072527,
51.2084047211903));
#148705=CARTESIAN_POINT('Ctrl Pts',(-1.23705251633842,-6.90125551145013,
51.2170767742482));
#148706=CARTESIAN_POINT('Ctrl Pts',(-1.04903565219108,-6.93495760152948,
51.2257487653849));
#148707=CARTESIAN_POINT('Ctrl Pts',(-0.859640898940478,-6.96097193353402,
51.2344207565216));
#148708=CARTESIAN_POINT('Ctrl Pts',(-0.669500206861603,-6.97921170588142,
51.2430927476583));
#148709=CARTESIAN_POINT('Ctrl Pts',(-0.479360810404349,-6.99745135394274,
51.251764679704));
#148710=CARTESIAN_POINT('Ctrl Pts',(-0.288475768015695,-7.00791652123613,
51.2604366117496));
#148711=CARTESIAN_POINT('Ctrl Pts',(-0.0974819939219479,-7.01057228929001,
51.2691085437952));
#148712=CARTESIAN_POINT('Ctrl Pts',(0.0935105410576831,-7.01322804011402,
51.2777804195797));
#148713=CARTESIAN_POINT('Ctrl Pts',(0.284611522344142,-7.00807448913604,
51.2864522953643));
#148714=CARTESIAN_POINT('Ctrl Pts',(0.475183323466561,-6.9951288316656,
51.2951241711488));
#148715=CARTESIAN_POINT('Ctrl Pts',(0.665753950390968,-6.98218325395913,
51.3037959935021));
#148716=CARTESIAN_POINT('Ctrl Pts',(0.855795120323774,-6.96144568508285,
51.3124678158553));
#148717=CARTESIAN_POINT('Ctrl Pts',(1.04467275076075,-6.93298531704186,
51.3211396382086));
#148718=CARTESIAN_POINT('Ctrl Pts',(1.23354927906118,-6.90452511507248,
51.3298114099601));
#148719=CARTESIAN_POINT('Ctrl Pts',(1.42126200062561,-6.86834224643157,
51.3384831817116));
#148720=CARTESIAN_POINT('Ctrl Pts',(1.60718460924404,-6.82455743578359,
51.3471549534632));
#148721=CARTESIAN_POINT('Ctrl Pts',(1.79763389405547,-6.77970659200791,
51.3560378577016));
#148722=CARTESIAN_POINT('Ctrl Pts',(1.98620448431563,-6.72687898190959,
51.3649207619401));
#148723=CARTESIAN_POINT('Ctrl Pts',(2.1722362342754,-6.66625954377723,51.3738036661786));
#148724=CARTESIAN_POINT('Ctrl Pts',(2.3538653218573,-6.60707473666721,51.382476345935));
#148725=CARTESIAN_POINT('Ctrl Pts',(2.53307410227384,-6.54046283696636,
51.3911490256913));
#148726=CARTESIAN_POINT('Ctrl Pts',(2.70926451773964,-6.46664614274022,
51.3998217054477));
#148727=CARTESIAN_POINT('Ctrl Pts',(2.8854515153589,-6.39283088045425,51.4084942169662));
#148728=CARTESIAN_POINT('Ctrl Pts',(3.05862000314123,-6.31181121311156,
51.4171667284847));
#148729=CARTESIAN_POINT('Ctrl Pts',(3.22819210343966,-6.22385751008085,
51.4258392400033));
#148730=CARTESIAN_POINT('Ctrl Pts',(3.39776113570845,-6.13590539837659,
51.434511594612));
#148731=CARTESIAN_POINT('Ctrl Pts',(3.5637336585096,-6.04101963284044,51.4431839492208));
#148732=CARTESIAN_POINT('Ctrl Pts',(3.72555582775144,-5.93951684371779,
51.4518563038295));
#148733=CARTESIAN_POINT('Ctrl Pts',(3.88737528046379,-5.83801575853546,
51.4605285128544));
#148734=CARTESIAN_POINT('Ctrl Pts',(4.04504427838822,-5.72989802299727,
51.4692007218792));
#148735=CARTESIAN_POINT('Ctrl Pts',(4.1980367036313,-5.61552440983604,51.477872930904));
#148736=CARTESIAN_POINT('Ctrl Pts',(4.35102676029984,-5.50115256736659,
51.4865450056688));
#148737=CARTESIAN_POINT('Ctrl Pts',(4.49934016166372,-5.38052521116008,
51.4952170804335));
#148738=CARTESIAN_POINT('Ctrl Pts',(4.64248202336599,-5.25404484423417,
51.5038891551983));
#148739=CARTESIAN_POINT('Ctrl Pts',(4.78562185584416,-5.12756627033376,
51.512561107025));
#148740=CARTESIAN_POINT('Ctrl Pts',(4.92359008252347,-4.99523503982289,
51.5212330588517));
#148741=CARTESIAN_POINT('Ctrl Pts',(5.05592635132112,-4.85749269608475,
51.5299050106784));
#148742=CARTESIAN_POINT('Ctrl Pts',(5.18826091680221,-4.71975212524545,
51.5385768508873));
#148743=CARTESIAN_POINT('Ctrl Pts',(5.3149634726937,-4.57660078535456,51.5472486910962));
#148744=CARTESIAN_POINT('Ctrl Pts',(5.43561126741774,-4.42851631046125,
51.5559205313051));
#148745=CARTESIAN_POINT('Ctrl Pts',(5.56176013705507,-4.27367975367746,
51.5649877740387));
#148746=CARTESIAN_POINT('Ctrl Pts',(5.68128895686456,-4.11344992041185,
51.5740550167723));
#148747=CARTESIAN_POINT('Ctrl Pts',(5.79376175353962,-3.94841123817182,
51.5831222595058));
#148748=CARTESIAN_POINT('Ctrl Pts',(5.90133874236269,-3.79055649462878,
51.5917948158842));
#148749=CARTESIAN_POINT('Ctrl Pts',(6.00246078174151,-3.62830291661796,
51.6004673722627));
#148750=CARTESIAN_POINT('Ctrl Pts',(6.09679041553231,-3.46219196342049,
51.6091399286411));
#148751=CARTESIAN_POINT('Ctrl Pts',(6.19111669178666,-3.29608692271898,
51.6178121763316));
#148752=CARTESIAN_POINT('Ctrl Pts',(6.2786509059623,-3.12612502860927,51.626484424022));
#148753=CARTESIAN_POINT('Ctrl Pts',(6.35910096686043,-2.9528734235952,51.6351566717125));
#148754=CARTESIAN_POINT('Ctrl Pts',(6.43954858436979,-2.77962708049169,
51.6438286560138));
#148755=CARTESIAN_POINT('Ctrl Pts',(6.5129123595191,-2.60309148404068,51.6525006403151));
#148756=CARTESIAN_POINT('Ctrl Pts',(6.57894750102417,-2.42385567665813,
51.6611726246164));
#148757=CARTESIAN_POINT('Ctrl Pts',(6.6449809817109,-2.24462437714989,51.6698443908127));
#148758=CARTESIAN_POINT('Ctrl Pts',(6.70368609940859,-2.06269326910016,
51.6785161570091));
#148759=CARTESIAN_POINT('Ctrl Pts',(6.75486698389381,-1.87866936750494,
51.6871879232055));
#148760=CARTESIAN_POINT('Ctrl Pts',(6.80605126222495,-1.69463326313567,
51.6958602644337));
#148761=CARTESIAN_POINT('Ctrl Pts',(6.84971023276614,-1.50850436117982,
51.7045326056619));
#148762=CARTESIAN_POINT('Ctrl Pts',(6.88569820761715,-1.3209037648966,51.7132049468901));
#148763=CARTESIAN_POINT('Ctrl Pts',(6.92168406448219,-1.13331420939665,
51.7218767777285));
#148764=CARTESIAN_POINT('Ctrl Pts',(6.9499997755378,-0.944253411829444,
51.7305486085668));
#148765=CARTESIAN_POINT('Ctrl Pts',(6.9705508637184,-0.754352184867711,
51.7392204394052));
#148766=CARTESIAN_POINT('Ctrl Pts',(6.99110229108004,-0.564447823721784,
51.7478924133659));
#148767=CARTESIAN_POINT('Ctrl Pts',(7.0038888085648,-0.373703287796009,
51.7565643873266));
#148768=CARTESIAN_POINT('Ctrl Pts',(7.00886775178455,-0.182755028643803,
51.7652363612874));
#148769=CARTESIAN_POINT('Ctrl Pts',(7.01045582731892,-0.121850486192426,
51.7680023598284));
#148770=CARTESIAN_POINT('Ctrl Pts',(7.01125000000003,-0.0609252433289545,
51.7707683583695));
#148771=CARTESIAN_POINT('Ctrl Pts',(7.01125,3.46460095547362E-12,51.7735343569105));
#148772=CARTESIAN_POINT('Ctrl Pts',(7.01124999999651,-6.99800587777282E-6,
51.7736935453439));
#148773=CARTESIAN_POINT('Ctrl Pts',(7.01125016734379,0.167656998790483,
51.7812920136671));
#148774=CARTESIAN_POINT('Ctrl Pts',(7.00523183104702,0.335486844567159,
51.7888904819904));
#148775=CARTESIAN_POINT('Ctrl Pts',(6.99318534782853,0.502976394492236,
51.7964889503137));
#148776=CARTESIAN_POINT('Ctrl Pts',(6.98114140614357,0.670430607937701,
51.8040858155332));
#148777=CARTESIAN_POINT('Ctrl Pts',(6.96307186471559,0.837544268886115,
51.8116826807527));
#148778=CARTESIAN_POINT('Ctrl Pts',(6.9390191791175,1.00381242985907,51.8192795459723));
#148779=CARTESIAN_POINT('Ctrl Pts',(6.91496982024836,1.17005759426877,51.8268753604687));
#148780=CARTESIAN_POINT('Ctrl Pts',(6.88493902506947,1.33545709566369,51.8344711749652));
#148781=CARTESIAN_POINT('Ctrl Pts',(6.8490208902499,1.49951305676892,51.8420669894617));
#148782=CARTESIAN_POINT('Ctrl Pts',(6.81309084638302,1.66362341240805,51.8496653224329));
#148783=CARTESIAN_POINT('Ctrl Pts',(6.77126965611079,1.82638894818059,51.8572636554041));
#148784=CARTESIAN_POINT('Ctrl Pts',(6.72370207982196,1.98732405618659,51.8648619883752));
#148785=CARTESIAN_POINT('Ctrl Pts',(6.7009547367353,2.06428501157083,51.8684955955604));
#148786=CARTESIAN_POINT('Ctrl Pts',(6.67689401063677,2.14082759811051,51.8721292027455));
#148787=CARTESIAN_POINT('Ctrl Pts',(6.65153969883759,2.21690013245694,51.8757628099306));
#148788=CARTESIAN_POINT('Ctrl Pts',(6.62603162985497,2.29343399656497,51.8794184525475));
#148789=CARTESIAN_POINT('Ctrl Pts',(6.59921527121467,2.36948942895206,51.8830740951643));
#148790=CARTESIAN_POINT('Ctrl Pts',(6.57110895151814,2.44502632087637,51.8867297377812));
#148791=CARTESIAN_POINT('',(7.01124899179693,-0.00375999023141351,51.2264656430896));
#148792=CARTESIAN_POINT('Ctrl Pts',(6.57110895151816,2.4450263208763,51.3398522865015));
#148793=CARTESIAN_POINT('Ctrl Pts',(6.63771924680899,2.266008408508,51.3311805125694));
#148794=CARTESIAN_POINT('Ctrl Pts',(6.69700989700473,2.08426710051955,51.3225087386372));
#148795=CARTESIAN_POINT('Ctrl Pts',(6.74878307789422,1.90040877971785,51.3138369647051));
#148796=CARTESIAN_POINT('Ctrl Pts',(6.80055978789531,1.71653792623954,51.3051645996628));
#148797=CARTESIAN_POINT('Ctrl Pts',(6.84481792613573,1.53055004459453,51.2964922346204));
#148798=CARTESIAN_POINT('Ctrl Pts',(6.88140980451098,1.3430657708691,51.2878198695781));
#148799=CARTESIAN_POINT('Ctrl Pts',(6.91799949925383,1.15559268532943,51.2791480220619));
#148800=CARTESIAN_POINT('Ctrl Pts',(6.94692379517689,0.966623665170781,
51.2704761745458));
#148801=CARTESIAN_POINT('Ctrl Pts',(6.96808618426389,0.776789219267855,
51.2618043270297));
#148802=CARTESIAN_POINT('Ctrl Pts',(6.98924897510677,0.586951169466182,
51.2531323148835));
#148803=CARTESIAN_POINT('Ctrl Pts',(7.00264953276857,0.396247943319445,
51.2444603027373));
#148804=CARTESIAN_POINT('Ctrl Pts',(7.00824314361839,0.205315860142146,
51.2357882905911));
#148805=CARTESIAN_POINT('Ctrl Pts',(7.01024757124657,0.136896809746564,
51.2326807414239));
#148806=CARTESIAN_POINT('Ctrl Pts',(7.01125,0.0684484052929644,51.2295731922568));
#148807=CARTESIAN_POINT('Ctrl Pts',(7.01125,8.58630487052188E-16,51.2264656430896));
#148808=CARTESIAN_POINT('Ctrl Pts',(7.01124899179693,-0.00375999023141351,
51.2264656430896));
#148809=CARTESIAN_POINT('Ctrl Pts',(7.01114686516534,-0.194195389987069,
51.2178782345103));
#148810=CARTESIAN_POINT('Ctrl Pts',(7.00328188214509,-0.384378067801461,
51.209290825931));
#148811=CARTESIAN_POINT('Ctrl Pts',(6.9877404724221,-0.573680793276399,
51.2007034173516));
#148812=CARTESIAN_POINT('Ctrl Pts',(6.97216474589871,-0.763401515828795,
51.1920970470184));
#148813=CARTESIAN_POINT('Ctrl Pts',(6.94887874818298,-0.952238122132306,
51.1834906766853));
#148814=CARTESIAN_POINT('Ctrl Pts',(6.9180198950668,-1.13957329468532,51.1748843063521));
#148815=CARTESIAN_POINT('Ctrl Pts',(6.88705732364092,-1.32753811110005,
51.1662490095328));
#148816=CARTESIAN_POINT('Ctrl Pts',(6.84847101251243,-1.51399111503323,
51.1576137127136));
#148817=CARTESIAN_POINT('Ctrl Pts',(6.80244897060659,-1.69832698995022,
51.1489784158944));
#148818=CARTESIAN_POINT('Ctrl Pts',(6.75634013910903,-1.88301049036709,
51.1403268344026));
#148819=CARTESIAN_POINT('Ctrl Pts',(6.70276764581104,-2.06556861579921,
51.1316752529107));
#148820=CARTESIAN_POINT('Ctrl Pts',(6.64196799252027,-2.24541482778488,
51.1230236714189));
#148821=CARTESIAN_POINT('Ctrl Pts',(6.58099956891383,-2.42576026468925,
51.1143480744918));
#148822=CARTESIAN_POINT('Ctrl Pts',(6.51276396106416,-2.60337846703591,
51.1056724775646));
#148823=CARTESIAN_POINT('Ctrl Pts',(6.43754508372162,-2.77770406227007,
51.0969968806375));
#148824=CARTESIAN_POINT('Ctrl Pts',(6.41999360611982,-2.81838097594212,
51.094972527835));
#148825=CARTESIAN_POINT('Ctrl Pts',(6.40206209931074,-2.85887873757411,
51.0929481750325));
#148826=CARTESIAN_POINT('Ctrl Pts',(6.38375451036624,-2.89919038938092,
51.09092382223));
#148827=CARTESIAN_POINT('Ctrl Pts',(6.30905780118092,-3.06366577392893,
51.0826642697005));
#148828=CARTESIAN_POINT('Ctrl Pts',(6.22790629528599,-3.22546041629001,
51.074404717171));
#148829=CARTESIAN_POINT('Ctrl Pts',(6.14051288283972,-3.38404020339289,
51.0661451646414));
#148830=CARTESIAN_POINT('Ctrl Pts',(6.05322118716208,-3.54243542025116,
51.057895225365));
#148831=CARTESIAN_POINT('Ctrl Pts',(5.95970222323858,-3.69762293679834,
51.0496452860886));
#148832=CARTESIAN_POINT('Ctrl Pts',(5.86021662995801,-3.84908919258356,
51.0413953468122));
#148833=CARTESIAN_POINT('Ctrl Pts',(5.76082890037866,-4.00040645143455,
51.0331535229781));
#148834=CARTESIAN_POINT('Ctrl Pts',(5.65548642398,-4.1480094566598,51.0249116991439));
#148835=CARTESIAN_POINT('Ctrl Pts',(5.54449549951053,-4.2914095840886,51.0166698753098));
#148836=CARTESIAN_POINT('Ctrl Pts',(5.43359376933599,-4.43469447260648,
51.008434674753));
#148837=CARTESIAN_POINT('Ctrl Pts',(5.31705284651501,-4.57378294220874,
51.0001994741961));
#148838=CARTESIAN_POINT('Ctrl Pts',(5.19522219400986,-4.7082154705756,50.9919642736392));
#148839=CARTESIAN_POINT('Ctrl Pts',(5.07346751947766,-4.84256416198687,
50.9837342088494));
#148840=CARTESIAN_POINT('Ctrl Pts',(4.94642992078197,-4.97226244427602,
50.9755041440595));
#148841=CARTESIAN_POINT('Ctrl Pts',(4.81449914552032,-5.0968838068259,50.9672740792697));
#148842=CARTESIAN_POINT('Ctrl Pts',(4.68262164753145,-5.22145484384474,
50.9590473380062));
#148843=CARTESIAN_POINT('Ctrl Pts',(4.54585516074474,-5.34095281011707,
50.9508205967427));
#148844=CARTESIAN_POINT('Ctrl Pts',(4.40462653196979,-5.45498777967172,
50.9425938554792));
#148845=CARTESIAN_POINT('Ctrl Pts',(4.26342782703677,-5.56899858723859,
50.9343688573162));
#148846=CARTESIAN_POINT('Ctrl Pts',(4.11776913183774,-5.67754848776479,
50.9261438591533));
#148847=CARTESIAN_POINT('Ctrl Pts',(3.96811085296037,-5.78028743412627,
50.9179188609904));
#148848=CARTESIAN_POINT('Ctrl Pts',(3.81845986875505,-5.88302137276667,
50.9096942637318));
#148849=CARTESIAN_POINT('Ctrl Pts',(3.66480997364422,-5.9799447266635,50.9014696664733));
#148850=CARTESIAN_POINT('Ctrl Pts',(3.50765125758459,-6.07075030104725,
50.8932450692148));
#148851=CARTESIAN_POINT('Ctrl Pts',(3.35047456404471,-6.16156626273539,
50.8850195311397));
#148852=CARTESIAN_POINT('Ctrl Pts',(3.18978854848019,-6.24626287833383,
50.8767939930645));
#148853=CARTESIAN_POINT('Ctrl Pts',(3.02610884015156,-6.32457839306753,
50.8685684549893));
#148854=CARTESIAN_POINT('Ctrl Pts',(2.86231442999977,-6.40294878896159,
50.8603371527042));
#148855=CARTESIAN_POINT('Ctrl Pts',(2.69552244617433,-6.47492899902809,
50.852105850419));
#148856=CARTESIAN_POINT('Ctrl Pts',(2.52627036974207,-6.54030462451584,
50.8438745481338));
#148857=CARTESIAN_POINT('Ctrl Pts',(2.35695843339274,-6.60570337160778,
50.835640334658));
#148858=CARTESIAN_POINT('Ctrl Pts',(2.18518499436796,-6.66449276065142,
50.8274061211821));
#148859=CARTESIAN_POINT('Ctrl Pts',(2.01150401975149,-6.71650788289745,
50.8191719077062));
#148860=CARTESIAN_POINT('Ctrl Pts',(1.83763489346561,-6.76857935404472,
50.8109287739614));
#148861=CARTESIAN_POINT('Ctrl Pts',(1.66185443491329,-6.81386180185788,
50.8026856402165));
#148862=CARTESIAN_POINT('Ctrl Pts',(1.48472933798092,-6.85224090027772,
50.7944425064716));
#148863=CARTESIAN_POINT('Ctrl Pts',(1.33536468048928,-6.88460492429011,
50.7874913015335));
#148864=CARTESIAN_POINT('Ctrl Pts',(1.18504413502541,-6.91206079366791,
50.7805400965954));
#148865=CARTESIAN_POINT('Ctrl Pts',(1.03411085615969,-6.93456857343503,
50.7735888916573));
#148866=CARTESIAN_POINT('Ctrl Pts',(0.852786367835311,-6.9616084130268,
50.7652380250484));
#148867=CARTESIAN_POINT('Ctrl Pts',(0.670243323763772,-6.98155555507229,
50.7568871584396));
#148868=CARTESIAN_POINT('Ctrl Pts',(0.487063628053379,-6.99431165910753,
50.7485362918308));
#148869=CARTESIAN_POINT('Ctrl Pts',(0.304043063887654,-7.00705668168239,
50.7401926797722));
#148870=CARTESIAN_POINT('Ctrl Pts',(0.120387279841823,-7.01262309418271,
50.7318490677136));
#148871=CARTESIAN_POINT('Ctrl Pts',(-0.0633147710334978,-7.01096411360585,
50.723505455655));
#148872=CARTESIAN_POINT('Ctrl Pts',(-0.246882989121302,-7.0093063416491,
50.7151679221831));
#148873=CARTESIAN_POINT('Ctrl Pts',(-0.430497076145864,-7.00043367259616,
50.7068303887113));
#148874=CARTESIAN_POINT('Ctrl Pts',(-0.61356573293114,-6.98435134095305,
50.6984928552395));
#148875=CARTESIAN_POINT('Ctrl Pts',(-0.796509835818056,-6.96827995119992,
50.6901609943515));
#148876=CARTESIAN_POINT('Ctrl Pts',(-0.97890891887683,-6.94500871154048,
50.6818291334635));
#148877=CARTESIAN_POINT('Ctrl Pts',(-1.16017422465034,-6.91459487829598,
50.6734972725755));
#148878=CARTESIAN_POINT('Ctrl Pts',(-1.34136576371141,-6.88419342209452,
50.6651688023748));
#148879=CARTESIAN_POINT('Ctrl Pts',(-1.52142411862375,-6.84665522173497,
50.6568403321742));
#148880=CARTESIAN_POINT('Ctrl Pts',(-1.69976754339773,-6.80208915414313,
50.6485118619736));
#148881=CARTESIAN_POINT('Ctrl Pts',(-1.87806378529055,-6.75753487703628,
50.6401855951691));
#148882=CARTESIAN_POINT('Ctrl Pts',(-2.05464568012357,-6.705956520383,50.6318593283647));
#148883=CARTESIAN_POINT('Ctrl Pts',(-2.22894313884969,-6.64751374923549,
50.6235330615602));
#148884=CARTESIAN_POINT('Ctrl Pts',(-2.28903353967636,-6.62736515057351,
50.6206625164971));
#148885=CARTESIAN_POINT('Ctrl Pts',(-2.34885253725066,-6.60640110093273,
50.6177919714339));
#148886=CARTESIAN_POINT('Ctrl Pts',(-2.408377186239,-6.58462951815085,50.6149214263707));
#148887=CARTESIAN_POINT('Ctrl Pts',(-2.58802914240775,-6.51892047992671,
50.6062578047512));
#148888=CARTESIAN_POINT('Ctrl Pts',(-2.76490399357511,-6.44588668882583,
50.5975941831317));
#148889=CARTESIAN_POINT('Ctrl Pts',(-2.9384196596914,-6.36579268167281,
50.5889305615122));
#148890=CARTESIAN_POINT('Ctrl Pts',(-3.11207603129979,-6.28563372553309,
50.5802599144801));
#148891=CARTESIAN_POINT('Ctrl Pts',(-3.28236752256699,-6.19840324020155,
50.571589267448));
#148892=CARTESIAN_POINT('Ctrl Pts',(-3.44873578605048,-6.10441217813106,
50.5629186204159));
#148893=CARTESIAN_POINT('Ctrl Pts',(-3.619288361139,-6.00805715623099,50.554029898805));
#148894=CARTESIAN_POINT('Ctrl Pts',(-3.78571750450639,-5.90459720012164,
50.545141177194));
#148895=CARTESIAN_POINT('Ctrl Pts',(-3.94745299325198,-5.7944146752339,
50.536252455583));
#148896=CARTESIAN_POINT('Ctrl Pts',(-4.1055484615931,-5.68671191926959,
50.5275637836228));
#148897=CARTESIAN_POINT('Ctrl Pts',(-4.25915907189742,-5.57258613754218,
50.5188751116625));
#148898=CARTESIAN_POINT('Ctrl Pts',(-4.40778493321005,-5.45243601934644,
50.5101864397023));
#148899=CARTESIAN_POINT('Ctrl Pts',(-4.56154378005493,-5.32813636208025,
50.501197693266));
#148900=CARTESIAN_POINT('Ctrl Pts',(-4.70996717776444,-5.19738905481171,
50.4922089468296));
#148901=CARTESIAN_POINT('Ctrl Pts',(-4.85254158261168,-5.06067848727071,
50.4832202003933));
#148902=CARTESIAN_POINT('Ctrl Pts',(-4.99511598745892,-4.9239679197297,
50.4742314539569));
#148903=CARTESIAN_POINT('Ctrl Pts',(-5.13184118669585,-4.78129434844169,
50.4652427075206));
#148904=CARTESIAN_POINT('Ctrl Pts',(-5.26224758495059,-4.63318215886033,
50.4562539610843));
#148905=CARTESIAN_POINT('Ctrl Pts',(-5.38755233669695,-4.49086428646692,
50.4476168646243));
#148906=CARTESIAN_POINT('Ctrl Pts',(-5.50714608811164,-4.34338555826818,
50.4389797681644));
#148907=CARTESIAN_POINT('Ctrl Pts',(-5.6206143895385,-4.19121944624864,
50.4303426717045));
#148908=CARTESIAN_POINT('Ctrl Pts',(-5.73398628081987,-4.03918262458434,
50.4217129138908));
#148909=CARTESIAN_POINT('Ctrl Pts',(-5.84124293139716,-3.88246659835011,
50.4130831560772));
#148910=CARTESIAN_POINT('Ctrl Pts',(-5.94201028610278,-3.72157766576875,
50.4044533982635));
#148911=CARTESIAN_POINT('Ctrl Pts',(-6.04599828610969,-3.55554653027593,
50.395547823058));
#148912=CARTESIAN_POINT('Ctrl Pts',(-6.14307510290476,-3.38507156342488,
50.3866422478526));
#148913=CARTESIAN_POINT('Ctrl Pts',(-6.23287680377116,-3.21074342037967,
50.3777366726471));
#148914=CARTESIAN_POINT('Ctrl Pts',(-6.31973521627337,-3.04212895524955,
50.3691229813996));
#148915=CARTESIAN_POINT('Ctrl Pts',(-6.39978767404947,-2.86991016399872,
50.360509290152));
#148916=CARTESIAN_POINT('Ctrl Pts',(-6.47275013472672,-2.69464881865806,
50.3518955989045));
#148917=CARTESIAN_POINT('Ctrl Pts',(-6.54942120960752,-2.51047910168861,
50.3428440817201));
#148918=CARTESIAN_POINT('Ctrl Pts',(-6.61826259867565,-2.32294975584741,
50.3337925645356));
#148919=CARTESIAN_POINT('Ctrl Pts',(-6.67900042040682,-2.13274000916791,
50.3247410473512));
#148920=CARTESIAN_POINT('Ctrl Pts',(-6.73973824213799,-1.9425302624884,
50.3156895301668));
#148921=CARTESIAN_POINT('Ctrl Pts',(-6.79237234741334,-1.74964046124067,
50.3066380129823));
#148922=CARTESIAN_POINT('Ctrl Pts',(-6.8366883706311,-1.55477287260149,
50.2975864957979));
#148923=CARTESIAN_POINT('Ctrl Pts',(-6.87773839777344,-1.37426660823085,
50.2892020560598));
#148924=CARTESIAN_POINT('Ctrl Pts',(-6.91163053864259,-1.19215520593247,
50.2808176163217));
#148925=CARTESIAN_POINT('Ctrl Pts',(-6.93826242264715,-1.00902978993809,
50.2724331765837));
#148926=CARTESIAN_POINT('Ctrl Pts',(-6.96490149311032,-0.825854958617998,
50.2640464743534));
#148927=CARTESIAN_POINT('Ctrl Pts',(-6.98427635294729,-0.641665888901126,
50.2556597721232));
#148928=CARTESIAN_POINT('Ctrl Pts',(-6.99633636889544,-0.457060144588258,
50.2472730698929));
#148929=CARTESIAN_POINT('Ctrl Pts',(-7.00840113260011,-0.272381725153531,
50.238883066007));
#148930=CARTESIAN_POINT('Ctrl Pts',(-7.01314528820371,-0.0872866274934254,
50.2304930621211));
#148931=CARTESIAN_POINT('Ctrl Pts',(-7.01057028857457,0.097625772496311,
50.2221030582351));
#148932=CARTESIAN_POINT('Ctrl Pts',(-7.00799288167434,0.282711040189968,
50.2137052108476));
#148933=CARTESIAN_POINT('Ctrl Pts',(-6.9980826523609,0.467612944374797,
50.2053073634601));
#148934=CARTESIAN_POINT('Ctrl Pts',(-6.98089314537137,0.651734190761063,
50.1969095160725));
#148935=CARTESIAN_POINT('Ctrl Pts',(-6.96369459592466,0.835952293240432,
50.1885072510379));
#148936=CARTESIAN_POINT('Ctrl Pts',(-6.9392091680795,1.01938859684581,50.1801049860033));
#148937=CARTESIAN_POINT('Ctrl Pts',(-6.90754197487244,1.20145346471486,
50.1717027209686));
#148938=CARTESIAN_POINT('Ctrl Pts',(-6.87584176519267,1.3837081548932,50.1632916956643));
#148939=CARTESIAN_POINT('Ctrl Pts',(-6.83694489388335,1.56458823472889,
50.1548806703599));
#148940=CARTESIAN_POINT('Ctrl Pts',(-6.79100728441987,1.74351559369462,
50.1464696450555));
#148941=CARTESIAN_POINT('Ctrl Pts',(-6.77726115282142,1.79705688701902,
50.1439527735408));
#148942=CARTESIAN_POINT('Ctrl Pts',(-6.76288492067004,1.85042343905972,
50.1414359020261));
#148943=CARTESIAN_POINT('Ctrl Pts',(-6.74788362291677,1.90360005622813,
50.1389190305114));
#148944=CARTESIAN_POINT('Ctrl Pts',(-6.69886596229565,2.0773579147955,50.1306949984468));
#148945=CARTESIAN_POINT('Ctrl Pts',(-6.64308337158687,2.24939632808308,
50.1224709663821));
#148946=CARTESIAN_POINT('Ctrl Pts',(-6.58067605921214,2.41915877242735,
50.1142469343175));
#148947=CARTESIAN_POINT('Ctrl Pts',(-6.51832251648744,2.58877495078333,
50.1060299880142));
#148948=CARTESIAN_POINT('Ctrl Pts',(-6.44935574289596,2.75611874316578,
50.097813041711));
#148949=CARTESIAN_POINT('Ctrl Pts',(-6.37396598305644,2.92064790917004,
50.0895960954078));
#148950=CARTESIAN_POINT('Ctrl Pts',(-6.29862732739923,3.08506554638696,
50.081384719096));
#148951=CARTESIAN_POINT('Ctrl Pts',(-6.21687450492783,3.24667204463256,
50.0731733427843));
#148952=CARTESIAN_POINT('Ctrl Pts',(-6.12894626796018,3.40494408279447,
50.0649619664726));
#148953=CARTESIAN_POINT('Ctrl Pts',(-6.04106148598651,3.56313790136841,
50.0567546483033));
#148954=CARTESIAN_POINT('Ctrl Pts',(-5.94700753964128,3.71800024127984,
50.0485473301339));
#148955=CARTESIAN_POINT('Ctrl Pts',(-5.84706972497163,3.869031169921,50.0403400119646));
#148956=CARTESIAN_POINT('Ctrl Pts',(-5.74716295158532,4.02001518745183,
50.0321352430374));
#148957=CARTESIAN_POINT('Ctrl Pts',(-5.64137614378662,4.16716987677307,
50.0239304741103));
#148958=CARTESIAN_POINT('Ctrl Pts',(-5.53003876001613,4.31002295530074,
50.0157257051831));
#148959=CARTESIAN_POINT('Ctrl Pts',(-5.41869192894773,4.45288815532384,
50.0075202400576));
#148960=CARTESIAN_POINT('Ctrl Pts',(-5.30179378764467,4.59145073660134,
49.9993147749322));
#148961=CARTESIAN_POINT('Ctrl Pts',(-5.17971542014312,4.72526980487164,
49.9911093098067));
#148962=CARTESIAN_POINT('Ctrl Pts',(-5.05762626039362,4.85910070331786,
49.9829031192831));
#148963=CARTESIAN_POINT('Ctrl Pts',(-4.93035619510045,4.98818699599834,
49.9746969287596));
#148964=CARTESIAN_POINT('Ctrl Pts',(-4.7983146184668,5.11212317777142,49.966490738236));
#148965=CARTESIAN_POINT('Ctrl Pts',(-4.66623938327661,5.23609095196477,
49.9582824558825));
#148966=CARTESIAN_POINT('Ctrl Pts',(-4.52939046556829,5.35490576114034,
49.950074173529));
#148967=CARTESIAN_POINT('Ctrl Pts',(-4.38821206241735,5.46820093428861,
49.9418658911754));
#148968=CARTESIAN_POINT('Ctrl Pts',(-4.24697416290341,5.58154385305943,
49.9336541496317));
#148969=CARTESIAN_POINT('Ctrl Pts',(-4.10140341208564,5.68936228277764,
49.925442408088));
#148970=CARTESIAN_POINT('Ctrl Pts',(-3.95197498637103,5.79133147640486,
49.9172306665443));
#148971=CARTESIAN_POINT('Ctrl Pts',(-3.80236826487776,5.89342233815975,
49.9090091268725));
#148972=CARTESIAN_POINT('Ctrl Pts',(-3.64889495842309,5.98964982288017,
49.9007875872007));
#148973=CARTESIAN_POINT('Ctrl Pts',(-3.49205803781394,6.07973331841448,
49.8925660475289));
#148974=CARTESIAN_POINT('Ctrl Pts',(-3.33512346264137,6.16987290446876,
49.8843393887126));
#148975=CARTESIAN_POINT('Ctrl Pts',(-3.17482140377513,6.25386071168839,
49.8761127298962));
#148976=CARTESIAN_POINT('Ctrl Pts',(-3.01167720518098,6.33146325696464,
49.8678860710799));
#148977=CARTESIAN_POINT('Ctrl Pts',(-2.84828125709027,6.40918555152939,
49.8596467176214));
#148978=CARTESIAN_POINT('Ctrl Pts',(-2.68203472247581,6.48050275408142,
49.851407364163));
#148979=CARTESIAN_POINT('Ctrl Pts',(-2.51348197790676,6.54522993555138,
49.8431680107045));
#148980=CARTESIAN_POINT('Ctrl Pts',(-2.36630103640591,6.60174997344102,
49.8359733737826));
#148981=CARTESIAN_POINT('Ctrl Pts',(-2.21736203517322,6.65324594581425,
49.8287787368606));
#148982=CARTESIAN_POINT('Ctrl Pts',(-2.0670347233137,6.69962640862276,49.8215840999386));
#148983=CARTESIAN_POINT('Ctrl Pts',(-1.90024344144612,6.7510864976096,49.8136015005032));
#148984=CARTESIAN_POINT('Ctrl Pts',(-1.73121745408192,6.79641013066064,
49.8056189010677));
#148985=CARTESIAN_POINT('Ctrl Pts',(-1.56045933555508,6.83539268985909,
49.7976363016322));
#148986=CARTESIAN_POINT('Ctrl Pts',(-1.38991509841071,6.87432642184084,
49.7896637007222));
#148987=CARTESIAN_POINT('Ctrl Pts',(-1.2176434041049,6.90693480175379,49.7816910998123));
#148988=CARTESIAN_POINT('Ctrl Pts',(-1.0441653504234,6.93306175390608,49.7737184989023));
#148989=CARTESIAN_POINT('Ctrl Pts',(-0.870866908181658,6.95916165537735,
49.7657541524677));
#148990=CARTESIAN_POINT('Ctrl Pts',(-0.696364955962511,6.97879342840225,
49.7577898060332));
#148991=CARTESIAN_POINT('Ctrl Pts',(-0.521194181197202,6.99185119893052,
49.7498254595986));
#148992=CARTESIAN_POINT('Ctrl Pts',(-0.346166793694386,7.00489828092943,
49.7418676324355));
#148993=CARTESIAN_POINT('Ctrl Pts',(-0.170472041520858,7.01138204324479,
49.7339098052724));
#148994=CARTESIAN_POINT('Ctrl Pts',(0.00534687895631584,7.01124796119674,
49.7259519781093));
#148995=CARTESIAN_POINT('Ctrl Pts',(0.181059950969795,7.01111395987026,
49.7179989418059));
#148996=CARTESIAN_POINT('Ctrl Pts',(0.356896672224531,7.00437004559262,
49.7100459055025));
#148997=CARTESIAN_POINT('Ctrl Pts',(0.53231051110847,6.99101366629071,49.7020928691991));
#148998=CARTESIAN_POINT('Ctrl Pts',(0.714130602427552,6.97716950142996,
49.6938493817061));
#148999=CARTESIAN_POINT('Ctrl Pts',(0.895495928886207,6.95622072434907,
49.685605894213));
#149000=CARTESIAN_POINT('Ctrl Pts',(1.0757993490757,6.9282236051551,49.67736240672));
#149001=CARTESIAN_POINT('Ctrl Pts',(1.24968766269844,6.90122260962314,49.6694122184372));
#149002=CARTESIAN_POINT('Ctrl Pts',(1.4225879440712,6.86766627608292,49.6614620301544));
#149003=CARTESIAN_POINT('Ctrl Pts',(1.59396264879154,6.82765769768502,49.6535118418716));
#149004=CARTESIAN_POINT('Ctrl Pts',(1.76535290166246,6.7876454894667,49.6455609322996));
#149005=CARTESIAN_POINT('Ctrl Pts',(1.93521694017008,6.74117995505776,49.6376100227276));
#149006=CARTESIAN_POINT('Ctrl Pts',(2.10302955462439,6.6884148536762,49.6296591131556));
#149007=CARTESIAN_POINT('Ctrl Pts',(2.27089027670589,6.63563462587619,49.6217059242592));
#149008=CARTESIAN_POINT('Ctrl Pts',(2.43669804965809,6.57655134781931,49.6137527353627));
#149009=CARTESIAN_POINT('Ctrl Pts',(2.5999450286778,6.51136793695101,49.6057995464663));
#149010=CARTESIAN_POINT('Ctrl Pts',(2.76327080887429,6.44615306130759,49.5978425184749));
#149011=CARTESIAN_POINT('Ctrl Pts',(2.92403299011285,6.37483232927915,49.5898854904836));
#149012=CARTESIAN_POINT('Ctrl Pts',(3.08174593827678,6.29765579675601,49.5819284624923));
#149013=CARTESIAN_POINT('Ctrl Pts',(3.23965263439011,6.22038445404074,49.5739616594135));
#149014=CARTESIAN_POINT('Ctrl Pts',(3.39450228635389,6.13724311373323,49.5659948563347));
#149015=CARTESIAN_POINT('Ctrl Pts',(3.54583533107336,6.04852695847608,49.558028053256));
#149016=CARTESIAN_POINT('Ctrl Pts',(3.69727876073859,5.95974609211764,49.550055439053));
#149017=CARTESIAN_POINT('Ctrl Pts',(3.84520016447192,5.86538251282993,49.54208282485));
#149018=CARTESIAN_POINT('Ctrl Pts',(3.98917137484191,5.76577300148401,49.534110210647));
#149019=CARTESIAN_POINT('Ctrl Pts',(4.1333501474075,5.66601988386553,49.5261261023869));
#149020=CARTESIAN_POINT('Ctrl Pts',(4.27356706678711,5.5610059623044,49.5181419941268));
#149021=CARTESIAN_POINT('Ctrl Pts',(4.40942872327172,5.45110675889643,49.5101578858667));
#149022=CARTESIAN_POINT('Ctrl Pts',(4.4429439673612,5.42399610293387,49.5081883136997));
#149023=CARTESIAN_POINT('Ctrl Pts',(4.47619435967196,5.39658832312724,49.5062187415327));
#149024=CARTESIAN_POINT('Ctrl Pts',(4.50917436348155,5.36888937511482,49.5042491693657));
#149025=CARTESIAN_POINT('Ctrl Pts',(4.64638763713034,5.25364792895385,49.496054766288));
#149026=CARTESIAN_POINT('Ctrl Pts',(4.77937035689912,5.13298339543888,49.4878603632103));
#149027=CARTESIAN_POINT('Ctrl Pts',(4.90766902805733,5.00723589154205,49.4796659601326));
#149028=CARTESIAN_POINT('Ctrl Pts',(5.03582349476579,4.88162972464771,49.4714807673559));
#149029=CARTESIAN_POINT('Ctrl Pts',(5.15930414786905,4.75095220810401,49.4632955745792));
#149030=CARTESIAN_POINT('Ctrl Pts',(5.27768968001487,4.61558427546985,49.4551103818026));
#149031=CARTESIAN_POINT('Ctrl Pts',(5.39596273489216,4.48034495496451,49.4469329657205));
#149032=CARTESIAN_POINT('Ctrl Pts',(5.50915008003478,4.34042435702449,49.4387555496384));
#149033=CARTESIAN_POINT('Ctrl Pts',(5.61686638443958,4.19624100616882,49.4305781335563));
#149034=CARTESIAN_POINT('Ctrl Pts',(5.72448335994765,4.05219061172347,49.4224082581499));
#149035=CARTESIAN_POINT('Ctrl Pts',(5.82663914104444,3.90388558009215,49.4142383827435));
#149036=CARTESIAN_POINT('Ctrl Pts',(5.92298797670736,3.75177824375056,49.4060685073371));
#149037=CARTESIAN_POINT('Ctrl Pts',(6.0192848778625,3.59975289718694,49.3979030357043));
#149038=CARTESIAN_POINT('Ctrl Pts',(6.10978087998942,3.44392962425402,49.3897375640715));
#149039=CARTESIAN_POINT('Ctrl Pts',(6.19417266954185,3.28479093739628,49.3815720924387));
#149040=CARTESIAN_POINT('Ctrl Pts',(6.27853476099334,3.12570825263085,49.3734094942963));
#149041=CARTESIAN_POINT('Ctrl Pts',(6.35679675379812,2.96331278812909,49.365246896154));
#149042=CARTESIAN_POINT('Ctrl Pts',(6.42870047017853,2.79811308335213,49.3570842980116));
#149043=CARTESIAN_POINT('Ctrl Pts',(6.47934924960681,2.68174686711097,49.3513345864016));
#149044=CARTESIAN_POINT('Ctrl Pts',(6.52684414272043,2.56398981785157,49.3455848747916));
#149045=CARTESIAN_POINT('Ctrl Pts',(6.57110895151812,2.44502632087643,49.3398351631816));
#149046=CARTESIAN_POINT('Origin',(0.,0.,50.));
#149047=CARTESIAN_POINT('',(6.57110895151816,2.44502632087632,47.3397953554189));
#149048=CARTESIAN_POINT('',(6.57110895151812,2.44502632087642,47.8869530982584));
#149049=CARTESIAN_POINT('',(6.57110895151814,2.44502632087636,50.));
#149050=CARTESIAN_POINT('',(7.01124999999811,5.14667476088492E-6,49.7734178143132));
#149051=CARTESIAN_POINT('Ctrl Pts',(6.57110895151812,2.44502632087642,47.8869530982584));
#149052=CARTESIAN_POINT('Ctrl Pts',(6.51463505187432,2.59680225241057,47.8943274580956));
#149053=CARTESIAN_POINT('Ctrl Pts',(6.45289207376814,2.74664578379087,47.9017018179328));
#149054=CARTESIAN_POINT('Ctrl Pts',(6.38600797641393,2.89422333064981,47.90907617777));
#149055=CARTESIAN_POINT('Ctrl Pts',(6.31139718170492,3.0588495794581,47.9173024508257));
#149056=CARTESIAN_POINT('Ctrl Pts',(6.23035139912944,3.22073266371939,47.9255287238814));
#149057=CARTESIAN_POINT('Ctrl Pts',(6.14309824714195,3.37934468328721,47.9337549969371));
#149058=CARTESIAN_POINT('Ctrl Pts',(6.05590682677823,3.53784448481712,47.9419754499029));
#149059=CARTESIAN_POINT('Ctrl Pts',(5.96251695279652,3.69307752994855,47.9501959028687));
#149060=CARTESIAN_POINT('Ctrl Pts',(5.86320334614051,3.84453808464772,47.9584163558345));
#149061=CARTESIAN_POINT('Ctrl Pts',(5.76394352395888,3.99591661406759,47.9666323569154));
#149062=CARTESIAN_POINT('Ctrl Pts',(5.65876655127818,4.14352643512401,47.9748483579963));
#149063=CARTESIAN_POINT('Ctrl Pts',(5.54799198093946,4.2868883286052,47.9830643590772));
#149064=CARTESIAN_POINT('Ctrl Pts',(5.43725477539619,4.43020186543008,47.9912775888615));
#149065=CARTESIAN_POINT('Ctrl Pts',(5.32092394576607,4.56927005576485,47.9994908186457));
#149066=CARTESIAN_POINT('Ctrl Pts',(5.19936123939148,4.70364425364137,48.0077040484299));
#149067=CARTESIAN_POINT('Ctrl Pts',(5.07782294310237,4.83799146885393,48.0159156289778));
#149068=CARTESIAN_POINT('Ctrl Pts',(4.95105509758945,4.96764631462191,48.0241272095256));
#149069=CARTESIAN_POINT('Ctrl Pts',(4.81945855553145,5.09219459506554,48.0323387900734));
#149070=CARTESIAN_POINT('Ctrl Pts',(4.68784883333586,5.21675534972352,48.0405511930574));
#149071=CARTESIAN_POINT('Ctrl Pts',(4.55140969910055,5.33620827810491,48.0487635960415));
#149072=CARTESIAN_POINT('Ctrl Pts',(4.41057787328124,5.45017700503589,48.0569759990255));
#149073=CARTESIAN_POINT('Ctrl Pts',(4.34902759899551,5.49998681444358,48.0605652137025));
#149074=CARTESIAN_POINT('Ctrl Pts',(4.28663870993172,5.54874959094404,48.0641544283794));
#149075=CARTESIAN_POINT('Ctrl Pts',(4.22344961252298,5.59643636012949,48.0677436430564));
#149076=CARTESIAN_POINT('Ctrl Pts',(4.07564924571124,5.70797651921876,48.0761388768478));
#149077=CARTESIAN_POINT('Ctrl Pts',(3.9234191645242,5.813664558907,48.0845341106393));
#149078=CARTESIAN_POINT('Ctrl Pts',(3.76725238731245,5.91315787145825,48.0929293444308));
#149079=CARTESIAN_POINT('Ctrl Pts',(3.61107845045146,6.01265574539721,48.1013249631116));
#149080=CARTESIAN_POINT('Ctrl Pts',(3.45096773100342,6.10595815233807,48.1097205817925));
#149081=CARTESIAN_POINT('Ctrl Pts',(3.28744105561792,6.1927665762838,48.1181162004733));
#149082=CARTESIAN_POINT('Ctrl Pts',(3.12388684239997,6.27958961873644,48.1265132329732));
#149083=CARTESIAN_POINT('Ctrl Pts',(2.95691581233362,6.35991634618527,48.1349102654732));
#149084=CARTESIAN_POINT('Ctrl Pts',(2.78707257109982,6.43349462158189,48.1433072979731));
#149085=CARTESIAN_POINT('Ctrl Pts',(2.61712751558886,6.50711700423217,48.1517093641605));
#149086=CARTESIAN_POINT('Ctrl Pts',(2.44430710591814,6.57398272280881,48.1601114303479));
#149087=CARTESIAN_POINT('Ctrl Pts',(2.26917603244139,6.6338877512582,48.1685134965354));
#149088=CARTESIAN_POINT('Ctrl Pts',(2.09398709362871,6.69381257302311,48.1769183388628));
#149089=CARTESIAN_POINT('Ctrl Pts',(1.91648627641171,6.74677201820913,48.1853231811902));
#149090=CARTESIAN_POINT('Ctrl Pts',(1.73725332938764,6.792611974199,48.1937280235177));
#149091=CARTESIAN_POINT('Ctrl Pts',(1.55788446949918,6.83848669076065,48.2021392392614));
#149092=CARTESIAN_POINT('Ctrl Pts',(1.37678117094426,6.87723105851779,48.2105504550052));
#149093=CARTESIAN_POINT('Ctrl Pts',(1.19453427722378,6.90874188423894,48.218961670749));
#149094=CARTESIAN_POINT('Ctrl Pts',(1.14073163628928,6.91804446058038,48.2214448166137));
#149095=CARTESIAN_POINT('Ctrl Pts',(1.08682937379787,6.92671694796164,48.2239279624783));
#149096=CARTESIAN_POINT('Ctrl Pts',(1.03284279133955,6.9347575538643,48.2264111083429));
#149097=CARTESIAN_POINT('Ctrl Pts',(0.836866110723315,6.96394575550984,
48.2354251755774));
#149098=CARTESIAN_POINT('Ctrl Pts',(0.639662547652286,6.9848205477569,48.2444392428119));
#149099=CARTESIAN_POINT('Ctrl Pts',(0.441915919871735,6.99730926015593,
48.2534533100463));
#149100=CARTESIAN_POINT('Ctrl Pts',(0.244216234661515,7.00979500789121,
48.2624652374542));
#149101=CARTESIAN_POINT('Ctrl Pts',(0.0459739666607946,7.01389863951236,
48.2714771648622));
#149102=CARTESIAN_POINT('Ctrl Pts',(-0.152123700502803,7.00959948515215,
48.2804890922701));
#149103=CARTESIAN_POINT('Ctrl Pts',(-0.350051838192558,7.00530400995378,
48.2894933073847));
#149104=CARTESIAN_POINT('Ctrl Pts',(-0.547835397827325,6.99262012224001,
48.2984975224993));
#149105=CARTESIAN_POINT('Ctrl Pts',(-0.744788474997783,6.97157921062441,
48.3075017376139));
#149106=CARTESIAN_POINT('Ctrl Pts',(-0.941583074783314,6.95055522948127,
48.3164987075284));
#149107=CARTESIAN_POINT('Ctrl Pts',(-1.13754830323584,6.92118767471165,
48.3254956774428));
#149108=CARTESIAN_POINT('Ctrl Pts',(-1.33200279437177,6.88355977080797,
48.3344926473573));
#149109=CARTESIAN_POINT('Ctrl Pts',(-1.52613539751012,6.84599415382073,
48.3434747242414));
#149110=CARTESIAN_POINT('Ctrl Pts',(-1.71876203702228,6.80019553628115,
48.3524568011256));
#149111=CARTESIAN_POINT('Ctrl Pts',(-1.90921095828222,6.74629825009798,
48.3614388780097));
#149112=CARTESIAN_POINT('Ctrl Pts',(-2.07629015342896,6.69901462603489,
48.3693187765495));
#149113=CARTESIAN_POINT('Ctrl Pts',(-2.24169328504685,6.64549871121803,
48.3771986750894));
#149114=CARTESIAN_POINT('Ctrl Pts',(-2.40497280154338,6.58587369954333,
48.3850785736292));
#149115=CARTESIAN_POINT('Ctrl Pts',(-2.57539384840242,6.52364080513861,
48.393303123696));
#149116=CARTESIAN_POINT('Ctrl Pts',(-2.74343544721625,6.45477517583604,
48.4015276737627));
#149117=CARTESIAN_POINT('Ctrl Pts',(-2.90856058795098,6.3794907217362,48.4097522238295));
#149118=CARTESIAN_POINT('Ctrl Pts',(-3.07367624415493,6.3042105918581,48.4179763014909));
#149119=CARTESIAN_POINT('Ctrl Pts',(-3.23587546241489,6.22251251541378,
48.4262003791523));
#149120=CARTESIAN_POINT('Ctrl Pts',(-3.39464265267125,6.13465792226145,
48.4344244568137));
#149121=CARTESIAN_POINT('Ctrl Pts',(-3.55342668942099,6.04679400702047,
48.4426494071168));
#149122=CARTESIAN_POINT('Ctrl Pts',(-3.70877767108523,5.95277244110612,
48.4508743574199));
#149123=CARTESIAN_POINT('Ctrl Pts',(-3.86020578286179,5.85289995442092,
48.459099307723));
#149124=CARTESIAN_POINT('Ctrl Pts',(-4.01172801401266,5.75296539249852,
48.4673293702023));
#149125=CARTESIAN_POINT('Ctrl Pts',(-4.15932221583622,5.64717283459909,
48.4755594326815));
#149126=CARTESIAN_POINT('Ctrl Pts',(-4.30252799035537,5.5358720590986,48.4837894951607));
#149127=CARTESIAN_POINT('Ctrl Pts',(-4.44578393186894,5.42453229337302,
48.4920224407464));
#149128=CARTESIAN_POINT('Ctrl Pts',(-4.5846481140489,5.30768068128211,48.5002553863321));
#149129=CARTESIAN_POINT('Ctrl Pts',(-4.71869403801562,5.18570661897642,
48.5084883319178));
#149130=CARTESIAN_POINT('Ctrl Pts',(-4.85286155771467,5.06362191156499,
48.5167287457728));
#149131=CARTESIAN_POINT('Ctrl Pts',(-4.982201839449,4.93640571065444,48.5249691596277));
#149132=CARTESIAN_POINT('Ctrl Pts',(-5.10632535682955,4.80448414636781,
48.5332095734826));
#149133=CARTESIAN_POINT('Ctrl Pts',(-5.15922816702545,4.74825772269336,
48.536721728627));
#149134=CARTESIAN_POINT('Ctrl Pts',(-5.2111838141935,4.69117696147659,48.5402338837714));
#149135=CARTESIAN_POINT('Ctrl Pts',(-5.26216439543281,4.63327664163702,
48.5437460389157));
#149136=CARTESIAN_POINT('Ctrl Pts',(-5.3819779525632,4.497200451246,48.5520002367065));
#149137=CARTESIAN_POINT('Ctrl Pts',(-5.49661766467963,4.35635166722079,
48.5602544344973));
#149138=CARTESIAN_POINT('Ctrl Pts',(-5.60569258271975,4.21115628189465,
48.5685086322881));
#149139=CARTESIAN_POINT('Ctrl Pts',(-5.71468122007305,4.06607574934855,
48.5767563008248));
#149140=CARTESIAN_POINT('Ctrl Pts',(-5.81811362944432,3.91665573995058,
48.5850039693615));
#149141=CARTESIAN_POINT('Ctrl Pts',(-5.91563833670354,3.76335616595392,
48.5932516378982));
#149142=CARTESIAN_POINT('Ctrl Pts',(-6.01310318906929,3.61015067816299,
48.6014942445041));
#149143=CARTESIAN_POINT('Ctrl Pts',(-6.10466738136032,3.45307065968898,
48.6097368511099));
#149144=CARTESIAN_POINT('Ctrl Pts',(-6.19002191479071,3.29260614968004,
48.6179794577158));
#149145=CARTESIAN_POINT('Ctrl Pts',(-6.27533918726352,3.13221168939264,
48.6262184660663));
#149146=CARTESIAN_POINT('Ctrl Pts',(-6.35445204293472,2.96843598493146,
48.6344574744167));
#149147=CARTESIAN_POINT('Ctrl Pts',(-6.42709658715709,2.80179514273505,
48.6426964827671));
#149148=CARTESIAN_POINT('Ctrl Pts',(-6.49972228675129,2.63519752862607,
48.650933353847));
#149149=CARTESIAN_POINT('Ctrl Pts',(-6.56588288287072,2.46573657282829,
48.6591702249268));
#149150=CARTESIAN_POINT('Ctrl Pts',(-6.62536181871064,2.29395015936946,
48.6674070960066));
#149151=CARTESIAN_POINT('Ctrl Pts',(-6.68484926816119,2.12213915699334,
48.6756451460839));
#149152=CARTESIAN_POINT('Ctrl Pts',(-6.73765302742374,1.94800235401809,
48.6838831961612));
#149153=CARTESIAN_POINT('Ctrl Pts',(-6.7836055886088,1.7720953080169,48.6921212462384));
#149154=CARTESIAN_POINT('Ctrl Pts',(-6.82956375477965,1.59616680605181,
48.7003603011379));
#149155=CARTESIAN_POINT('Ctrl Pts',(-6.86866896967914,1.41846796286247,
48.7085993560374));
#149156=CARTESIAN_POINT('Ctrl Pts',(-6.90080430639761,1.23956705639681,
48.7168384109369));
#149157=CARTESIAN_POINT('Ctrl Pts',(-6.932948728012,1.06061557332974,48.7250797950777));
#149158=CARTESIAN_POINT('Ctrl Pts',(-6.95811928290728,0.880461687592994,
48.7333211792186));
#149159=CARTESIAN_POINT('Ctrl Pts',(-6.97625058249306,0.699681622429293,
48.7415625633594));
#149160=CARTESIAN_POINT('Ctrl Pts',(-6.99438992270689,0.518821387322052,
48.7498076022799));
#149161=CARTESIAN_POINT('Ctrl Pts',(-7.0054837509383,0.337334760735345,
48.7580526412005));
#149162=CARTESIAN_POINT('Ctrl Pts',(-7.00951871315642,0.155801066780609,
48.7662976801209));
#149163=CARTESIAN_POINT('Ctrl Pts',(-7.01355852014873,-0.0259505944580573,
48.7745526188496));
#149164=CARTESIAN_POINT('Ctrl Pts',(-7.01052251805914,-0.207749092278264,
48.7828075575782));
#149165=CARTESIAN_POINT('Ctrl Pts',(-7.00044950268285,-0.389015838864519,
48.7910624963068));
#149166=CARTESIAN_POINT('Ctrl Pts',(-6.99037012363632,-0.57039710148762,
48.7993226501281));
#149167=CARTESIAN_POINT('Ctrl Pts',(-6.97324489693582,-0.751245601443899,
48.8075828039493));
#149168=CARTESIAN_POINT('Ctrl Pts',(-6.94916433108735,-0.930989614358494,
48.8158429577705));
#149169=CARTESIAN_POINT('Ctrl Pts',(-6.92504725073931,-1.11100618161099,
48.8241156368532));
#149170=CARTESIAN_POINT('Ctrl Pts',(-6.89395381022648,-1.28991457612809,
48.8323883159359));
#149171=CARTESIAN_POINT('Ctrl Pts',(-6.85602560790063,-1.46715351150136,
48.8406609950185));
#149172=CARTESIAN_POINT('Ctrl Pts',(-6.82481875155469,-1.61298351809075,
48.8474676531752));
#149173=CARTESIAN_POINT('Ctrl Pts',(-6.7889858638027,-1.7576834940798,48.8542743113319));
#149174=CARTESIAN_POINT('Ctrl Pts',(-6.7486307173724,-1.90094976341766,
48.8610809694886));
#149175=CARTESIAN_POINT('Ctrl Pts',(-6.70130433897402,-2.06896485626637,
48.8690634576727));
#149176=CARTESIAN_POINT('Ctrl Pts',(-6.64761112439817,-2.23552497683376,
48.8770459458569));
#149177=CARTESIAN_POINT('Ctrl Pts',(-6.58765216540073,-2.40009697933044,
48.8850284340411));
#149178=CARTESIAN_POINT('Ctrl Pts',(-6.52776817218238,-2.56446321994284,
48.8930009418411));
#149179=CARTESIAN_POINT('Ctrl Pts',(-6.46163414743741,-2.7268459441573,
48.9009734496411));
#149180=CARTESIAN_POINT('Ctrl Pts',(-6.38940200334982,-2.8867228135187,
48.9089459574412));
#149181=CARTESIAN_POINT('Ctrl Pts',(-6.3172444826564,-3.04643451327602,
48.9169102288029));
#149182=CARTESIAN_POINT('Ctrl Pts',(-6.23900153118579,-3.20364517460469,
48.9248745001647));
#149183=CARTESIAN_POINT('Ctrl Pts',(-6.15487459551915,-3.35784831044122,
48.9328387715265));
#149184=CARTESIAN_POINT('Ctrl Pts',(-6.07081633352349,-3.51192556869374,
48.9407965415728));
#149185=CARTESIAN_POINT('Ctrl Pts',(-5.98088382397672,-3.66299986365458,
48.9487543116191));
#149186=CARTESIAN_POINT('Ctrl Pts',(-5.88532625238966,-3.81058544917092,
48.9567120816654));
#149187=CARTESIAN_POINT('Ctrl Pts',(-5.78982599496341,-3.9580825148155,
48.964665078747));
#149188=CARTESIAN_POINT('Ctrl Pts',(-5.68870759294114,-4.10209472566131,
48.9726180758287));
#149189=CARTESIAN_POINT('Ctrl Pts',(-5.58226568439211,-4.24216175921643,
48.9805710729103));
#149190=CARTESIAN_POINT('Ctrl Pts',(-5.47193526020129,-4.38734569511109,
48.9888146073749));
#149191=CARTESIAN_POINT('Ctrl Pts',(-5.35588521613781,-4.52829039198769,
48.9970581418396));
#149192=CARTESIAN_POINT('Ctrl Pts',(-5.23449250536215,-4.66451656378317,
49.0053016763042));
#149193=CARTESIAN_POINT('Ctrl Pts',(-5.11741946947604,-4.7958952223314,
49.0132518703483));
#149194=CARTESIAN_POINT('Ctrl Pts',(-4.99537773349444,-4.92288510432967,
49.0212020643924));
#149195=CARTESIAN_POINT('Ctrl Pts',(-4.86874576639462,-5.04509080440724,
49.0291522584365));
#149196=CARTESIAN_POINT('Ctrl Pts',(-4.74210204530033,-5.16730784763263,
49.0371031904186));
#149197=CARTESIAN_POINT('Ctrl Pts',(-4.61086751207262,-5.28473956635985,
49.0450541224006));
#149198=CARTESIAN_POINT('Ctrl Pts',(-4.47545648116745,-5.39702842754013,
49.0530050543827));
#149199=CARTESIAN_POINT('Ctrl Pts',(-4.34000634767566,-5.50934971432778,
49.0609582823521));
#149200=CARTESIAN_POINT('Ctrl Pts',(-4.20037760186455,-5.616524950249,49.0689115103214));
#149201=CARTESIAN_POINT('Ctrl Pts',(-4.0570164057572,-5.71823787944476,
49.0768647382908));
#149202=CARTESIAN_POINT('Ctrl Pts',(-3.91358570704467,-5.82000011984712,
49.084821822046));
#149203=CARTESIAN_POINT('Ctrl Pts',(-3.76641925880851,-5.91629456772982,
49.0927789058011));
#149204=CARTESIAN_POINT('Ctrl Pts',(-3.61599074299558,-6.00684921644203,
49.1007359895563));
#149205=CARTESIAN_POINT('Ctrl Pts',(-3.46537696563385,-6.09751538852055,
49.1087028729272));
#149206=CARTESIAN_POINT('Ctrl Pts',(-3.31149341907474,-6.18242745899568,
49.1166697562982));
#149207=CARTESIAN_POINT('Ctrl Pts',(-3.15483752095674,-6.26135981867067,
49.1246366396692));
#149208=CARTESIAN_POINT('Ctrl Pts',(-2.99806707295894,-6.34034989524251,
49.1326093485822));
#149209=CARTESIAN_POINT('Ctrl Pts',(-2.83852057282886,-6.41335140127589,
49.1405820574953));
#149210=CARTESIAN_POINT('Ctrl Pts',(-2.67671331754712,-6.48018768078255,
49.1485547664084));
#149211=CARTESIAN_POINT('Ctrl Pts',(-2.51467237314459,-6.54712048816966,
49.1565389898567));
#149212=CARTESIAN_POINT('Ctrl Pts',(-2.35036450340084,-6.60787017223447,
49.164523213305));
#149213=CARTESIAN_POINT('Ctrl Pts',(-2.18431866091726,-6.66231030124451,
49.1725074367532));
#149214=CARTESIAN_POINT('Ctrl Pts',(-2.14335973009001,-6.67573917995051,
49.1744769245226));
#149215=CARTESIAN_POINT('Ctrl Pts',(-2.10229508780297,-6.68878438460215,
49.176446412292));
#149216=CARTESIAN_POINT('Ctrl Pts',(-2.06113274009001,-6.70144450027224,
49.1784159000614));
#149217=CARTESIAN_POINT('Ctrl Pts',(-1.88891025134105,-6.75441418615501,
49.1866561998511));
#149218=CARTESIAN_POINT('Ctrl Pts',(-1.71441685224321,-6.80081079918157,
49.1948964996408));
#149219=CARTESIAN_POINT('Ctrl Pts',(-1.53819039578885,-6.84043835355622,
49.2031367994305));
#149220=CARTESIAN_POINT('Ctrl Pts',(-1.36217376504217,-6.88001872500609,
49.2113672878288));
#149221=CARTESIAN_POINT('Ctrl Pts',(-1.18442852288641,-6.91284601743312,
49.2195977762271));
#149222=CARTESIAN_POINT('Ctrl Pts',(-1.00550902170901,-6.93877353498165,
49.2278282646254));
#149223=CARTESIAN_POINT('Ctrl Pts',(-0.826769649261018,-6.9646749497814,
49.2360504669096));
#149224=CARTESIAN_POINT('Ctrl Pts',(-0.646858714141219,-6.98369037941077,
49.2442726691937));
#149225=CARTESIAN_POINT('Ctrl Pts',(-0.466342382286715,-6.99572378992933,
49.2524948714779));
#149226=CARTESIAN_POINT('Ctrl Pts',(-0.28597460846228,-7.00774729741173,
49.2607103072043));
#149227=CARTESIAN_POINT('Ctrl Pts',(-0.105002775211771,-7.01280021177242,
49.2689257429307));
#149228=CARTESIAN_POINT('Ctrl Pts',(0.0759999335337276,-7.01083807918874,
49.2771411786572));
#149229=CARTESIAN_POINT('Ctrl Pts',(0.256886936402633,-7.00887720089718,
49.2853513626711));
#149230=CARTESIAN_POINT('Ctrl Pts',(0.43780442954631,-6.99991021597309,
49.293561546685));
#149231=CARTESIAN_POINT('Ctrl Pts',(0.618177072252241,-6.98394470695764,
49.3017717306989));
#149232=CARTESIAN_POINT('Ctrl Pts',(0.798474546826755,-6.96798585137622,
49.3099784932173));
#149233=CARTESIAN_POINT('Ctrl Pts',(0.978227278392545,-6.94503431356391,
49.3181852557357));
#149234=CARTESIAN_POINT('Ctrl Pts',(1.15686258505065,-6.91514971073005,
49.3263920182541));
#149235=CARTESIAN_POINT('Ctrl Pts',(1.33545890920995,-6.8852716294317,49.3345969898605));
#149236=CARTESIAN_POINT('Ctrl Pts',(1.51293795230025,-6.84846355431093,
49.3428019614669));
#149237=CARTESIAN_POINT('Ctrl Pts',(1.68873452703979,-6.80483668133804,
49.3510069330734));
#149238=CARTESIAN_POINT('Ctrl Pts',(1.86452200785808,-6.76121206517446,
49.3592114802382));
#149239=CARTESIAN_POINT('Ctrl Pts',(2.03862685710062,-6.71076943764895,
49.3674160274031));
#149240=CARTESIAN_POINT('Ctrl Pts',(2.21049620691852,-6.65367064722164,
49.375620574568));
#149241=CARTESIAN_POINT('Ctrl Pts',(2.38238528005077,-6.5965653042741,49.3838260632671));
#149242=CARTESIAN_POINT('Ctrl Pts',(2.55203801354117,-6.53280238624694,
49.3920315519661));
#149243=CARTESIAN_POINT('Ctrl Pts',(2.71891857186782,-6.46259300606593,
49.4002370406652));
#149244=CARTESIAN_POINT('Ctrl Pts',(2.88591860377642,-6.39233336139503,
49.4084484038599));
#149245=CARTESIAN_POINT('Ctrl Pts',(3.05014217433,-6.31561816665135,49.4166597670547));
#149246=CARTESIAN_POINT('Ctrl Pts',(3.21107437139439,-6.2327063097722,49.4248711302495));
#149247=CARTESIAN_POINT('Ctrl Pts',(3.37206445358993,-6.14976463062132,
49.4330854469603));
#149248=CARTESIAN_POINT('Ctrl Pts',(3.52976049776058,-6.06062201245151,
49.4412997636712));
#149249=CARTESIAN_POINT('Ctrl Pts',(3.68367371229846,-5.96558249828307,
49.4495140803821));
#149250=CARTESIAN_POINT('Ctrl Pts',(3.8377586158128,-5.87043696828643,49.4577375600984));
#149251=CARTESIAN_POINT('Ctrl Pts',(3.9880519661498,-5.76938158669269,49.4659610398148));
#149252=CARTESIAN_POINT('Ctrl Pts',(4.13409439688657,-5.66276346672992,
49.4741845195311));
#149253=CARTESIAN_POINT('Ctrl Pts',(4.26176121613083,-5.56956044223369,
49.4813732898988));
#149254=CARTESIAN_POINT('Ctrl Pts',(4.38617991706146,-5.47210719630128,
49.4885620602665));
#149255=CARTESIAN_POINT('Ctrl Pts',(4.50706545228633,-5.37065988229631,
49.4957508306342));
#149256=CARTESIAN_POINT('Ctrl Pts',(4.6484910384279,-5.25197532819353,49.5041610681452));
#149257=CARTESIAN_POINT('Ctrl Pts',(4.78533802794167,-5.12760708804512,
49.5125713056563));
#149258=CARTESIAN_POINT('Ctrl Pts',(4.91714286723303,-4.99793283125327,
49.5209815431673));
#149259=CARTESIAN_POINT('Ctrl Pts',(5.04883326038516,-4.86837117061592,
49.5293844780692));
#149260=CARTESIAN_POINT('Ctrl Pts',(5.17549000107735,-4.73351290448966,
49.5377874129712));
#149261=CARTESIAN_POINT('Ctrl Pts',(5.29668369780876,-4.59377495833948,
49.5461903478732));
#149262=CARTESIAN_POINT('Ctrl Pts',(5.41778724163909,-4.45414095968474,
49.5545870320461));
#149263=CARTESIAN_POINT('Ctrl Pts',(5.53343563203491,-4.30963476240791,
49.562983716219));
#149264=CARTESIAN_POINT('Ctrl Pts',(5.64323702120201,-4.16070937281554,
49.5713804003919));
#149265=CARTESIAN_POINT('Ctrl Pts',(5.75295723959736,-4.01189407644602,
49.5797708773088));
#149266=CARTESIAN_POINT('Ctrl Pts',(5.85683888789494,-3.85866636558156,
49.5881613542257));
#149267=CARTESIAN_POINT('Ctrl Pts',(5.95453086573895,-3.70151168192972,
49.5965518311426));
#149268=CARTESIAN_POINT('Ctrl Pts',(6.05217899339721,-3.54442753899393,
49.6049385418959));
#149269=CARTESIAN_POINT('Ctrl Pts',(6.1436428190526,-3.38342021257108,49.6133252526492));
#149270=CARTESIAN_POINT('Ctrl Pts',(6.2286145561511,-3.21900408098571,49.6217119634025));
#149271=CARTESIAN_POINT('Ctrl Pts',(6.31355606045063,-3.05464644837922,
49.6300956901785));
#149272=CARTESIAN_POINT('Ctrl Pts',(6.39200993482019,-2.88688271754616,
49.6384794169544));
#149273=CARTESIAN_POINT('Ctrl Pts',(6.46371414703572,-2.7162521951966,49.6468631437303));
#149274=CARTESIAN_POINT('Ctrl Pts',(6.48525334435847,-2.66499656632052,
49.6493815277938));
#149275=CARTESIAN_POINT('Ctrl Pts',(6.50618381300509,-2.6134824140297,49.6518999118572));
#149276=CARTESIAN_POINT('Ctrl Pts',(6.52649928291784,-2.56172474566901,
49.6544182959207));
#149277=CARTESIAN_POINT('Ctrl Pts',(6.59416463280609,-2.38933391473736,
49.6628063538657));
#149278=CARTESIAN_POINT('Ctrl Pts',(6.65498010262475,-2.21430015321486,
49.6711944118106));
#149279=CARTESIAN_POINT('Ctrl Pts',(6.70876036467014,-2.03719437755236,
49.6795824697556));
#149280=CARTESIAN_POINT('Ctrl Pts',(6.76258461466526,-1.85994374354111,
49.6879773884606));
#149281=CARTESIAN_POINT('Ctrl Pts',(6.80936206295708,-1.68061801858394,
49.6963723071656));
#149282=CARTESIAN_POINT('Ctrl Pts',(6.8489575222117,-1.49980246080603,49.7047672258705));
#149283=CARTESIAN_POINT('Ctrl Pts',(6.88856939771308,-1.31891193703781,
49.7131656251023));
#149284=CARTESIAN_POINT('Ctrl Pts',(6.92099328199438,-1.13653066598544,
49.7215640243341));
#149285=CARTESIAN_POINT('Ctrl Pts',(6.94614538059307,-0.953252807058868,
49.7299624235659));
#149286=CARTESIAN_POINT('Ctrl Pts',(6.97132356719064,-0.769784850572,49.7383695336982));
#149287=CARTESIAN_POINT('Ctrl Pts',(6.98921485666406,-0.585418769512334,
49.7467766438305));
#149288=CARTESIAN_POINT('Ctrl Pts',(6.99978734403713,-0.400753915461443,
49.7551837539629));
#149289=CARTESIAN_POINT('Ctrl Pts',(7.00743084934709,-0.267248266062745,
49.7612617740797));
#149290=CARTESIAN_POINT('Ctrl Pts',(7.01125009806236,-0.133586540720038,
49.7673397941964));
#149291=CARTESIAN_POINT('Ctrl Pts',(7.01124999999811,5.14667476088493E-6,
49.7734178143132));
#149292=CARTESIAN_POINT('Ctrl Pts',(7.01125,3.41650028888675E-12,49.7735343569105));
#149293=CARTESIAN_POINT('Ctrl Pts',(7.01124999999991,0.191008754743501,
49.7822061308426));
#149294=CARTESIAN_POINT('Ctrl Pts',(7.00344012881,0.38201736748625,49.7908779047747));
#149295=CARTESIAN_POINT('Ctrl Pts',(6.98784644419154,0.572388534912878,
49.7995496787068));
#149296=CARTESIAN_POINT('Ctrl Pts',(6.97225169663174,0.762772678963538,
49.8082220437492));
#149297=CARTESIAN_POINT('Ctrl Pts',(6.94887209704289,0.952519007629858,
49.8168944087915));
#149298=CARTESIAN_POINT('Ctrl Pts',(6.9177856624606,1.14099434299849,49.8255667738339));
#149299=CARTESIAN_POINT('Ctrl Pts',(6.88670108297151,1.32945843103956,49.83423862135));
#149300=CARTESIAN_POINT('Ctrl Pts',(6.84791063501112,1.51665139731078,49.8429104688661));
#149301=CARTESIAN_POINT('Ctrl Pts',(6.80154374572929,1.7019486588704,49.8515823163822));
#149302=CARTESIAN_POINT('Ctrl Pts',(6.7551759761985,1.8872494381929,49.8602543285284));
#149303=CARTESIAN_POINT('Ctrl Pts',(6.70123154646077,2.07065416525498,49.8689263406747));
#149304=CARTESIAN_POINT('Ctrl Pts',(6.63989045285515,2.25155087363867,49.8775983528209));
#149305=CARTESIAN_POINT('Ctrl Pts',(6.6179093415363,2.31637382429816,49.880705901988));
#149306=CARTESIAN_POINT('Ctrl Pts',(6.59497889661508,2.38087486019083,49.8838134511551));
#149307=CARTESIAN_POINT('Ctrl Pts',(6.57110895151815,2.44502632087633,49.8869210003222));
#149308=CARTESIAN_POINT('',(7.01124962123882,-0.00230459943256138,49.2264656431155));
#149309=CARTESIAN_POINT('Ctrl Pts',(6.57110895151812,2.44502632087643,49.3398351631816));
#149310=CARTESIAN_POINT('Ctrl Pts',(6.63393545901991,2.27617749405085,49.3316744072807));
#149311=CARTESIAN_POINT('Ctrl Pts',(6.69025281322801,2.10489771849203,49.3235136513798));
#149312=CARTESIAN_POINT('Ctrl Pts',(6.73988482605375,1.93172956027246,49.3153528954789));
#149313=CARTESIAN_POINT('Ctrl Pts',(6.78953780024269,1.75848826698436,49.3071886930007));
#149314=CARTESIAN_POINT('Ctrl Pts',(6.83249969278043,1.58335733548993,49.2990244905225));
#149315=CARTESIAN_POINT('Ctrl Pts',(6.86864450317827,1.40689347551938,49.2908602880443));
#149316=CARTESIAN_POINT('Ctrl Pts',(6.90479730607753,1.23039059507434,49.2826942802612));
#149317=CARTESIAN_POINT('Ctrl Pts',(6.9341299589928,1.05255454485122,49.2745282724782));
#149318=CARTESIAN_POINT('Ctrl Pts',(6.95656788542627,0.873950695380447,
49.2663622646952));
#149319=CARTESIAN_POINT('Ctrl Pts',(6.97902400505887,0.695202029702612,
49.2581896357208));
#149320=CARTESIAN_POINT('Ctrl Pts',(6.9945741935382,0.515684671185068,49.2500170067464));
#149321=CARTESIAN_POINT('Ctrl Pts',(7.00319582682655,0.335968411639008,
49.2418443777719));
#149322=CARTESIAN_POINT('Ctrl Pts',(7.008603707655,0.223242193525074,49.2367181328865));
#149323=CARTESIAN_POINT('Ctrl Pts',(7.01128667968011,0.11043776212266,49.231591888001));
#149324=CARTESIAN_POINT('Ctrl Pts',(7.01124962123882,-0.00230459943246711,
49.2264656431155));
#149325=CARTESIAN_POINT('Ctrl Pts',(7.01124962123863,-0.00230460000231739,
49.2264656430896));
#149326=CARTESIAN_POINT('Ctrl Pts',(7.0111543134133,-0.292258150983308,
49.2132818416574));
#149327=CARTESIAN_POINT('Ctrl Pts',(6.99306880246358,-0.581786799269796,
49.2000980402251));
#149328=CARTESIAN_POINT('Ctrl Pts',(6.95717055138536,-0.869140081595806,
49.1869142387928));
#149329=CARTESIAN_POINT('Ctrl Pts',(6.93473364888314,-1.04873984998543,
49.1786741808942));
#149330=CARTESIAN_POINT('Ctrl Pts',(6.90531789339566,-1.22763027984424,
49.1704341229955));
#149331=CARTESIAN_POINT('Ctrl Pts',(6.86898335526019,-1.40523813912747,
49.1621940650969));
#149332=CARTESIAN_POINT('Ctrl Pts',(6.83267575384516,-1.58271432828368,
49.1539601159903));
#149333=CARTESIAN_POINT('Ctrl Pts',(6.78945965786096,-1.75890950466602,
49.1457261668836));
#149334=CARTESIAN_POINT('Ctrl Pts',(6.73944670513276,-1.93325752841551,
49.137492217777));
#149335=CARTESIAN_POINT('Ctrl Pts',(6.6894626438119,-2.10750483506075,49.1292630252457));
#149336=CARTESIAN_POINT('Ctrl Pts',(6.63268964487006,-2.27990678465444,
49.1210338327145));
#149337=CARTESIAN_POINT('Ctrl Pts',(6.56929005055234,-2.44990913999153,
49.1128046401832));
#149338=CARTESIAN_POINT('Ctrl Pts',(6.50591565050843,-2.6198439383366,49.1045787178389));
#149339=CARTESIAN_POINT('Ctrl Pts',(6.43592002366576,-2.78738072007506,
49.0963527954947));
#149340=CARTESIAN_POINT('Ctrl Pts',(6.35951490614674,-2.95198182938131,
49.0881268731504));
#149341=CARTESIAN_POINT('Ctrl Pts',(6.28312779743214,-3.11654414195143,
49.0799028896688));
#149342=CARTESIAN_POINT('Ctrl Pts',(6.20033435550908,-3.27817184906863,
49.0716789061871));
#149343=CARTESIAN_POINT('Ctrl Pts',(6.11139394687428,-3.43634843818382,
49.0634549227055));
#149344=CARTESIAN_POINT('Ctrl Pts',(6.02244980194379,-3.5945316721359,49.0552305937427));
#149345=CARTESIAN_POINT('Ctrl Pts',(5.92735834133822,-3.74926319654111,
49.0470062647799));
#149346=CARTESIAN_POINT('Ctrl Pts',(5.82642447659114,-3.90005184338359,
49.0387819358171));
#149347=CARTESIAN_POINT('Ctrl Pts',(5.78332654716101,-3.96443735439881,
49.0352702150469));
#149348=CARTESIAN_POINT('Ctrl Pts',(5.73916396958308,-4.02810433437554,
49.0317584942767));
#149349=CARTESIAN_POINT('Ctrl Pts',(5.69396288521739,-4.09101616035269,
49.0282467735065));
#149350=CARTESIAN_POINT('Ctrl Pts',(5.57839100933724,-4.25187154347584,
49.0192678703967));
#149351=CARTESIAN_POINT('Ctrl Pts',(5.45607575093163,-4.40772067452792,
49.0102889672868));
#149352=CARTESIAN_POINT('Ctrl Pts',(5.32746421809379,-4.55804251487744,
49.001310064177));
#149353=CARTESIAN_POINT('Ctrl Pts',(5.1986842859189,-4.7085611812635,48.9923194044128));
#149354=CARTESIAN_POINT('Ctrl Pts',(5.06359174978242,-4.85353792162908,
48.9833287446486));
#149355=CARTESIAN_POINT('Ctrl Pts',(4.92267206018854,-4.99248699050275,
48.9743380848845));
#149356=CARTESIAN_POINT('Ctrl Pts',(4.78153217249342,-5.13165317822774,
48.9653333765071));
#149357=CARTESIAN_POINT('Ctrl Pts',(4.63454708033781,-5.26477269728677,
48.9563286681298));
#149358=CARTESIAN_POINT('Ctrl Pts',(4.48223860910744,-5.39139718565852,
48.9473239597524));
#149359=CARTESIAN_POINT('Ctrl Pts',(4.32984940165237,-5.51808879559654,
48.9383144781267));
#149360=CARTESIAN_POINT('Ctrl Pts',(4.17213135487001,-5.63827835741899,
48.929304996501));
#149361=CARTESIAN_POINT('Ctrl Pts',(4.00963852602667,-5.75155852383532,
48.9202955148753));
#149362=CARTESIAN_POINT('Ctrl Pts',(3.84706374338567,-5.86489582347964,
48.9112814892876));
#149363=CARTESIAN_POINT('Ctrl Pts',(3.67970955101394,-5.97131663517501,
48.9022674637));
#149364=CARTESIAN_POINT('Ctrl Pts',(3.50815945691212,-6.0704566374679,48.8932534381123));
#149365=CARTESIAN_POINT('Ctrl Pts',(3.35797501485197,-6.15724927962969,
48.8853620614815));
#149366=CARTESIAN_POINT('Ctrl Pts',(3.20457525062338,-6.23846235574786,
48.8774706848508));
#149367=CARTESIAN_POINT('Ctrl Pts',(3.04836791990124,-6.31387991550497,
48.86957930822));
#149368=CARTESIAN_POINT('Ctrl Pts',(2.88188031053688,-6.39426083725818,
48.8611685862406));
#149369=CARTESIAN_POINT('Ctrl Pts',(2.71211133539213,-6.46810118178353,
48.8527578642613));
#149370=CARTESIAN_POINT('Ctrl Pts',(2.53960042779602,-6.53514010788126,
48.8443471422819));
#149371=CARTESIAN_POINT('Ctrl Pts',(2.36719949029477,-6.60213629884319,
48.8359417818643));
#149372=CARTESIAN_POINT('Ctrl Pts',(2.19206040635686,-6.66233959912067,
48.8275364214467));
#149373=CARTESIAN_POINT('Ctrl Pts',(2.01474359368856,-6.7155368224879,48.8191310610291));
#149374=CARTESIAN_POINT('Ctrl Pts',(1.8375180199141,-6.76870667306548,48.8107300256148));
#149375=CARTESIAN_POINT('Ctrl Pts',(1.6581172615034,-6.81487754270127,48.8023289902005));
#149376=CARTESIAN_POINT('Ctrl Pts',(1.4771184101876,-6.8538855961261,48.7939279547861));
#149377=CARTESIAN_POINT('Ctrl Pts',(1.29619290096818,-6.89287784319419,
48.7855303235345));
#149378=CARTESIAN_POINT('Ctrl Pts',(1.11367090665178,-6.92471299539992,
48.7771326922829));
#149379=CARTESIAN_POINT('Ctrl Pts',(0.930141722771828,-6.94927787169711,
48.7687350610314));
#149380=CARTESIAN_POINT('Ctrl Pts',(0.746659319491453,-6.97383648653975,
48.7603395702907));
#149381=CARTESIAN_POINT('Ctrl Pts',(0.562170559411362,-6.99112847922829,
48.7519440795501));
#149382=CARTESIAN_POINT('Ctrl Pts',(0.377272445272298,-7.00109220511616,
48.7435485888094));
#149383=CARTESIAN_POINT('Ctrl Pts',(0.192389203732857,-7.01105512955451,
48.7351537733746));
#149384=CARTESIAN_POINT('Ctrl Pts',(0.00709699690991861,-7.0136909444913,
48.7267589579397));
#149385=CARTESIAN_POINT('Ctrl Pts',(-0.178003978355003,-7.00899002326225,
48.7183641425049));
#149386=CARTESIAN_POINT('Ctrl Pts',(-0.232776987931474,-7.00759897924896,
48.7158800426478));
#149387=CARTESIAN_POINT('Ctrl Pts',(-0.287533248423897,-7.00556586290797,
48.7133959427907));
#149388=CARTESIAN_POINT('Ctrl Pts',(-0.342257216702542,-7.00289130003565,
48.7109118429336));
#149389=CARTESIAN_POINT('Ctrl Pts',(-0.523177875600953,-6.99404903781773,
48.7026992626501));
#149390=CARTESIAN_POINT('Ctrl Pts',(-0.703804957775542,-6.97818886163649,
48.6944866823667));
#149391=CARTESIAN_POINT('Ctrl Pts',(-0.883563655581548,-6.95535346542758,
48.6862741020833));
#149392=CARTESIAN_POINT('Ctrl Pts',(-1.06330372176843,-6.93252043606049,
48.6780623730169));
#149393=CARTESIAN_POINT('Ctrl Pts',(-1.24217523938604,-6.90271367141434,
48.6698506439505));
#149394=CARTESIAN_POINT('Ctrl Pts',(-1.41960952695709,-6.86602762545219,
48.6616389148841));
#149395=CARTESIAN_POINT('Ctrl Pts',(-1.59705484946293,-6.82933929792356,
48.6534266751165));
#149396=CARTESIAN_POINT('Ctrl Pts',(-1.7730624247913,-6.78577090772626,
48.645214435349));
#149397=CARTESIAN_POINT('Ctrl Pts',(-1.94707453745135,-6.73546786111467,
48.6370021955814));
#149398=CARTESIAN_POINT('Ctrl Pts',(-2.12118466334839,-6.68513648104771,
48.6287853302267));
#149399=CARTESIAN_POINT('Ctrl Pts',(-2.29329674790264,-6.62806296212458,
48.6205684648719));
#149400=CARTESIAN_POINT('Ctrl Pts',(-2.46286823844427,-6.5644425964862,
48.6123515995171));
#149401=CARTESIAN_POINT('Ctrl Pts',(-2.63249341959451,-6.50080208703625,
48.6041321324957));
#149402=CARTESIAN_POINT('Ctrl Pts',(-2.79957608169925,-6.4306107277192,
48.5959126654742));
#149403=CARTESIAN_POINT('Ctrl Pts',(-2.96359411896677,-6.3541117758917,
48.5876931984527));
#149404=CARTESIAN_POINT('Ctrl Pts',(-3.12775415315384,-6.27754659588778,
48.5794666155127));
#149405=CARTESIAN_POINT('Ctrl Pts',(-3.28884395258761,-6.19466306970273,
48.5712400325727));
#149406=CARTESIAN_POINT('Ctrl Pts',(-3.44636568945316,-6.10575057606025,
48.5630134496326));
#149407=CARTESIAN_POINT('Ctrl Pts',(-3.51510070519197,-6.06695338037475,
48.5594237589708));
#149408=CARTESIAN_POINT('Ctrl Pts',(-3.58315670515217,-6.02700881618113,
48.555834068309));
#149409=CARTESIAN_POINT('Ctrl Pts',(-3.65049407409528,-5.98594349935708,
48.5522443776472));
#149410=CARTESIAN_POINT('Ctrl Pts',(-3.82915323051799,-5.87698921472776,
48.5427202290871));
#149411=CARTESIAN_POINT('Ctrl Pts',(-4.00285577337634,-5.76007938028789,
48.533196080527));
#149412=CARTESIAN_POINT('Ctrl Pts',(-4.17096818931078,-5.63565887241745,
48.5236719319669));
#149413=CARTESIAN_POINT('Ctrl Pts',(-4.33914537389983,-5.5111904290697,
48.5141441140391));
#149414=CARTESIAN_POINT('Ctrl Pts',(-4.50172804277483,-5.37920559321943,
48.5046162961112));
#149415=CARTESIAN_POINT('Ctrl Pts',(-4.65811393997038,-5.24019093972287,
48.4950884781833));
#149416=CARTESIAN_POINT('Ctrl Pts',(-4.81421893533291,-5.1014259856665,
48.4855777742124));
#149417=CARTESIAN_POINT('Ctrl Pts',(-4.96414932030537,-4.95565651457983,
48.4760670702415));
#149418=CARTESIAN_POINT('Ctrl Pts',(-5.10733913016107,-4.80340645500936,
48.4665563662707));
#149419=CARTESIAN_POINT('Ctrl Pts',(-5.2502234378214,-4.65148122810325,
48.4570659538341));
#149420=CARTESIAN_POINT('Ctrl Pts',(-5.38639581029265,-4.49310309591276,
48.4475755413976));
#149421=CARTESIAN_POINT('Ctrl Pts',(-5.51532812086316,-4.32883151459099,
48.438085128961));
#149422=CARTESIAN_POINT('Ctrl Pts',(-5.64362606150262,-4.16536817870633,
48.4286414110439));
#149423=CARTESIAN_POINT('Ctrl Pts',(-5.76475491902691,-3.9960693127224,
48.4191976931268));
#149424=CARTESIAN_POINT('Ctrl Pts',(-5.87822958593923,-3.82152371410787,
48.4097539752097));
#149425=CARTESIAN_POINT('Ctrl Pts',(-5.94302351683683,-3.72185833713127,
48.4043616209267));
#149426=CARTESIAN_POINT('Ctrl Pts',(-6.00532252882905,-3.62048299862126,
48.3989692666437));
#149427=CARTESIAN_POINT('Ctrl Pts',(-6.06504169686301,-3.51751272603427,
48.3935769123607));
#149428=CARTESIAN_POINT('Ctrl Pts',(-6.15236834452326,-3.36694048918445,
48.3856917351549));
#149429=CARTESIAN_POINT('Ctrl Pts',(-6.23414206732846,-3.21301399738746,
48.3778065579491));
#149430=CARTESIAN_POINT('Ctrl Pts',(-6.31009330272946,-3.05619846759808,
48.3699213807432));
#149431=CARTESIAN_POINT('Ctrl Pts',(-6.38602530597681,-2.89942264618669,
48.3620382001994));
#149432=CARTESIAN_POINT('Ctrl Pts',(-6.45613759027239,-2.739759582739,48.3541550196555));
#149433=CARTESIAN_POINT('Ctrl Pts',(-6.52020675079018,-2.5776986808877,
48.3462718391116));
#149434=CARTESIAN_POINT('Ctrl Pts',(-6.5842726076758,-2.4156461354688,48.3383890650523));
#149435=CARTESIAN_POINT('Ctrl Pts',(-6.64229582294004,-2.25119635027543,
48.330506290993));
#149436=CARTESIAN_POINT('Ctrl Pts',(-6.69410139158002,-2.08485805793737,
48.3226235169338));
#149437=CARTESIAN_POINT('Ctrl Pts',(-6.74593478824017,-1.91843041486979,
48.3147365085421));
#149438=CARTESIAN_POINT('Ctrl Pts',(-6.79154375300138,-1.75011259990219,
48.3068495001505));
#149439=CARTESIAN_POINT('Ctrl Pts',(-6.83080326259212,-1.58042821737047,
48.2989624917589));
#149440=CARTESIAN_POINT('Ctrl Pts',(-6.87007359128198,-1.41069707337455,
48.2910733098728));
#149441=CARTESIAN_POINT('Ctrl Pts',(-6.90299090701275,-1.23959898324818,
48.2831841279868));
#149442=CARTESIAN_POINT('Ctrl Pts',(-6.92948157068107,-1.0676664854211,
48.2752949461007));
#149443=CARTESIAN_POINT('Ctrl Pts',(-6.95599887859821,-0.895561058281625,
48.2673978292936));
#149444=CARTESIAN_POINT('Ctrl Pts',(-6.97607658060606,-0.722619923094152,
48.2595007124864));
#149445=CARTESIAN_POINT('Ctrl Pts',(-6.98969298956055,-0.549380081717617,
48.2516035956793));
#149446=CARTESIAN_POINT('Ctrl Pts',(-6.99928781427546,-0.427306345742015,
48.2460388794777));
#149447=CARTESIAN_POINT('Ctrl Pts',(-7.00567548191634,-0.305084359689145,
48.240474163276));
#149448=CARTESIAN_POINT('Ctrl Pts',(-7.00886393579073,-0.182901317852169,
48.2349094470743));
#149449=CARTESIAN_POINT('Ctrl Pts',(-7.0136627053592,0.0009897735821425,
48.2265342935304));
#149450=CARTESIAN_POINT('Ctrl Pts',(-7.01122326831066,0.185193758841107,
48.2181591399865));
#149451=CARTESIAN_POINT('Ctrl Pts',(-7.00152690421748,0.369117287618403,
48.2097839864426));
#149452=CARTESIAN_POINT('Ctrl Pts',(-6.99183724965269,0.552913548058271,
48.2014146281979));
#149453=CARTESIAN_POINT('Ctrl Pts',(-6.97490069659784,0.736429411317662,
48.1930452699531));
#149454=CARTESIAN_POINT('Ctrl Pts',(-6.95075058721552,0.919071725613981,
48.1846759117083));
#149455=CARTESIAN_POINT('Ctrl Pts',(-6.92661362404325,1.10161461782533,
48.1763111093577));
#149456=CARTESIAN_POINT('Ctrl Pts',(-6.89527097699532,1.28328458365763,
48.1679463070071));
#149457=CARTESIAN_POINT('Ctrl Pts',(-6.85680784497028,1.4634933343388,48.1595815046564));
#149458=CARTESIAN_POINT('Ctrl Pts',(-6.81835997906454,1.64363055968799,
48.1512200223181));
#149459=CARTESIAN_POINT('Ctrl Pts',(-6.77279733241736,1.8223074050096,48.1428585399797));
#149460=CARTESIAN_POINT('Ctrl Pts',(-6.72025633178953,1.99894507116699,
48.1344970576413));
#149461=CARTESIAN_POINT('Ctrl Pts',(-6.66772844373725,2.17553865413762,
48.1261376620651));
#149462=CARTESIAN_POINT('Ctrl Pts',(-6.60822576893657,2.35009375780528,
48.1177782664888));
#149463=CARTESIAN_POINT('Ctrl Pts',(-6.54193491543914,2.52204562303267,
48.1094188709126));
#149464=CARTESIAN_POINT('Ctrl Pts',(-6.4756391357662,2.69401026626827,48.1010588541367));
#149465=CARTESIAN_POINT('Ctrl Pts',(-6.40255428225458,2.86337097533321,
48.0926988373609));
#149466=CARTESIAN_POINT('Ctrl Pts',(-6.32291581769584,3.02958117977251,
48.0843388205851));
#149467=CARTESIAN_POINT('Ctrl Pts',(-6.24327214762705,3.19580224842039,
48.0759782573629));
#149468=CARTESIAN_POINT('Ctrl Pts',(-6.15707415439254,3.3588721048185,48.0676176941406));
#149469=CARTESIAN_POINT('Ctrl Pts',(-6.06460422482876,3.51826692544628,
48.0592571309184));
#149470=CARTESIAN_POINT('Ctrl Pts',(-5.9721158442247,3.67769355101074,48.0508948994664));
#149471=CARTESIAN_POINT('Ctrl Pts',(-5.87335319704827,3.83344339386688,
48.0425326680145));
#149472=CARTESIAN_POINT('Ctrl Pts',(-5.76864335165365,3.98501950358115,
48.0341704365625));
#149473=CARTESIAN_POINT('Ctrl Pts',(-5.66389855846263,4.13664620310389,
48.025805414145));
#149474=CARTESIAN_POINT('Ctrl Pts',(-5.55320279612925,4.28409612106476,
48.0174403917276));
#149475=CARTESIAN_POINT('Ctrl Pts',(-5.43692520276366,4.42690308252319,
48.0090753693102));
#149476=CARTESIAN_POINT('Ctrl Pts',(-5.32053966812708,4.56984261264322,
48.0007025815862));
#149477=CARTESIAN_POINT('Ctrl Pts',(-5.19856215605856,4.70813031790278,
47.9923297938623));
#149478=CARTESIAN_POINT('Ctrl Pts',(-5.07140148787643,4.841333856621,47.9839570061383));
#149479=CARTESIAN_POINT('Ctrl Pts',(-4.94417838928989,4.97460279253247,
47.9755801077367));
#149480=CARTESIAN_POINT('Ctrl Pts',(-4.81176729192242,5.10278235082226,
47.967203209335));
#149481=CARTESIAN_POINT('Ctrl Pts',(-4.67461276146979,5.22547816881899,
47.9588263109334));
#149482=CARTESIAN_POINT('Ctrl Pts',(-4.53730088598192,5.34831474467287,
47.9504398024709));
#149483=CARTESIAN_POINT('Ctrl Pts',(-4.39523495349272,5.46565479488748,
47.9420532940085));
#149484=CARTESIAN_POINT('Ctrl Pts',(-4.24889242112825,5.57714440876143,
47.9336667855461));
#149485=CARTESIAN_POINT('Ctrl Pts',(-4.15529036118381,5.64845421427322,
47.9283026958646));
#149486=CARTESIAN_POINT('Ctrl Pts',(-4.05993936491755,5.71737145869807,
47.922938606183));
#149487=CARTESIAN_POINT('Ctrl Pts',(-3.96297029502821,5.78381301592851,
47.9175745165015));
#149488=CARTESIAN_POINT('Ctrl Pts',(-3.81161611212275,5.88751832749905,
47.9092019765596));
#149489=CARTESIAN_POINT('Ctrl Pts',(-3.65601025415236,5.98540131201746,
47.9008294366177));
#149490=CARTESIAN_POINT('Ctrl Pts',(-3.49662611191066,6.07710723913973,
47.8924568966757));
#149491=CARTESIAN_POINT('Ctrl Pts',(-3.3374438431573,6.16869701295372,47.8840949612634));
#149492=CARTESIAN_POINT('Ctrl Pts',(-3.17449310946873,6.25412515821576,
47.875733025851));
#149493=CARTESIAN_POINT('Ctrl Pts',(-3.00827736862891,6.33307933282816,
47.8673710904386));
#149494=CARTESIAN_POINT('Ctrl Pts',(-2.8422497503453,6.41194414730489,47.8590186190436));
#149495=CARTESIAN_POINT('Ctrl Pts',(-2.67296478500967,6.48434945447317,
47.8506661476487));
#149496=CARTESIAN_POINT('Ctrl Pts',(-2.5009520785021,6.55002788265333,47.8423136762537));
#149497=CARTESIAN_POINT('Ctrl Pts',(-2.32916097188154,6.61562169887336,
47.8339719651494));
#149498=CARTESIAN_POINT('Ctrl Pts',(-2.15464943880652,6.67450580441283,
47.825630254045));
#149499=CARTESIAN_POINT('Ctrl Pts',(-1.97796860756911,6.72646019463218,
47.8172885429407));
#149500=CARTESIAN_POINT('Ctrl Pts',(-1.80142253261501,6.77837495870488,
47.8089531941451));
#149501=CARTESIAN_POINT('Ctrl Pts',(-1.62271077067838,6.82337044759098,
47.8006178453494));
#149502=CARTESIAN_POINT('Ctrl Pts',(-1.44240228279849,6.86127555321004,
47.7922824965538));
#149503=CARTESIAN_POINT('Ctrl Pts',(-1.26223618799388,6.89915072443931,
47.7839537303431));
#149504=CARTESIAN_POINT('Ctrl Pts',(-1.08047620279392,6.92994661192153,
47.7756249641325));
#149505=CARTESIAN_POINT('Ctrl Pts',(-0.897704377648231,6.95354250816454,
47.7672961979218));
#149506=CARTESIAN_POINT('Ctrl Pts',(-0.836338759730766,6.96146482743949,
47.7644998156862));
#149507=CARTESIAN_POINT('Ctrl Pts',(-0.774859178520908,6.96857592923775,
47.7617034334506));
#149508=CARTESIAN_POINT('Ctrl Pts',(-0.713287932486978,6.97487253560009,
47.758907051215));
#149509=CARTESIAN_POINT('Ctrl Pts',(-0.529553038553202,6.99366225282443,
47.750562360689));
#149510=CARTESIAN_POINT('Ctrl Pts',(-0.34515329223523,7.00517965295675,
47.7422176701629));
#149511=CARTESIAN_POINT('Ctrl Pts',(-0.160685625171539,7.00940844097155,
47.7338729796368));
#149512=CARTESIAN_POINT('Ctrl Pts',(0.0239015034585188,7.01363996755647,
47.7255228850754));
#149513=CARTESIAN_POINT('Ctrl Pts',(0.208556313908372,7.01057345934576,
47.7171727905139));
#149514=CARTESIAN_POINT('Ctrl Pts',(0.392683226795378,7.00024474185679,
47.7088226959525));
#149515=CARTESIAN_POINT('Ctrl Pts',(0.576953270014772,6.98990799537985,
47.7004661104779));
#149516=CARTESIAN_POINT('Ctrl Pts',(0.760694271244567,6.9722977970693,47.6921095250032));
#149517=CARTESIAN_POINT('Ctrl Pts',(0.943316662251313,6.94750172631998,
47.6837529395286));
#149518=CARTESIAN_POINT('Ctrl Pts',(1.12621645255707,6.92266799089764,47.6753836605888));
#149519=CARTESIAN_POINT('Ctrl Pts',(1.30799391308432,6.89062661468306,47.667014381649));
#149520=CARTESIAN_POINT('Ctrl Pts',(1.48806903357164,6.85151640980485,47.6586451027092));
#149521=CARTESIAN_POINT('Ctrl Pts',(1.66830008658007,6.81237233821129,47.6502685765564));
#149522=CARTESIAN_POINT('Ctrl Pts',(1.84682554268267,6.76614730615661,47.6418920504035));
#149523=CARTESIAN_POINT('Ctrl Pts',(2.02308084742507,6.71302990066944,47.6335155242507));
#149524=CARTESIAN_POINT('Ctrl Pts',(2.19960972899756,6.65983004835073,47.6251259963702));
#149525=CARTESIAN_POINT('Ctrl Pts',(2.37386110953577,6.59971655072576,47.6167364684897));
#149526=CARTESIAN_POINT('Ctrl Pts',(2.54528935663812,6.53292649992978,47.6083469406092));
#149527=CARTESIAN_POINT('Ctrl Pts',(2.60051016768242,6.51141195470758,47.605644489049));
#149528=CARTESIAN_POINT('Ctrl Pts',(2.65543822837897,6.48920499253787,47.6029420374888));
#149529=CARTESIAN_POINT('Ctrl Pts',(2.71005585341318,6.46631454801582,47.6002395859286));
#149530=CARTESIAN_POINT('Ctrl Pts',(2.87960170853735,6.39525726589795,47.59185054557));
#149531=CARTESIAN_POINT('Ctrl Pts',(3.04649674636681,6.31746679995528,47.5834615052114));
#149532=CARTESIAN_POINT('Ctrl Pts',(3.21018958197694,6.23316207155459,47.5750724648528));
#149533=CARTESIAN_POINT('Ctrl Pts',(3.37372780399423,6.14893697191042,47.5666913482355));
#149534=CARTESIAN_POINT('Ctrl Pts',(3.53406956243541,6.05821002621535,47.5583102316181));
#149535=CARTESIAN_POINT('Ctrl Pts',(3.69068428208039,5.9612478637031,47.5499291150007));
#149536=CARTESIAN_POINT('Ctrl Pts',(3.85429633078517,5.85995356587825,47.5411735416848));
#149537=CARTESIAN_POINT('Ctrl Pts',(4.01384031646739,5.75185422115874,47.5324179683689));
#149538=CARTESIAN_POINT('Ctrl Pts',(4.16873914753686,5.63730791089982,47.523662395053));
#149539=CARTESIAN_POINT('Ctrl Pts',(4.31677978741585,5.5278331721337,47.5152944773144));
#149540=CARTESIAN_POINT('Ctrl Pts',(4.46057741905618,5.41247023983569,47.5069265595758));
#149541=CARTESIAN_POINT('Ctrl Pts',(4.59965704948135,5.29157647489447,47.4985586418372));
#149542=CARTESIAN_POINT('Ctrl Pts',(4.73867542173533,5.17073595808833,47.490194409781));
#149543=CARTESIAN_POINT('Ctrl Pts',(4.87297968789883,5.04436968066918,47.4818301777247));
#149544=CARTESIAN_POINT('Ctrl Pts',(5.00212771071479,4.91287542363932,47.4734659456684));
#149545=CARTESIAN_POINT('Ctrl Pts',(5.1312361384931,4.78142148097079,47.4651042779726));
#149546=CARTESIAN_POINT('Ctrl Pts',(5.25519124492781,4.64484292801901,47.4567426102768));
#149547=CARTESIAN_POINT('Ctrl Pts',(5.3735872615183,4.50357485841506,47.448380942581));
#149548=CARTESIAN_POINT('Ctrl Pts',(5.49196282015109,4.36233119889074,47.4400207197197));
#149549=CARTESIAN_POINT('Ctrl Pts',(5.60478099394573,4.21639989101749,47.4316604968583));
#149550=CARTESIAN_POINT('Ctrl Pts',(5.7116755962774,4.06624992411795,47.423300273997));
#149551=CARTESIAN_POINT('Ctrl Pts',(5.81858358501917,3.91608115393938,47.414939004185));
#149552=CARTESIAN_POINT('Ctrl Pts',(5.91956632664644,3.76169293515637,47.406577734373));
#149553=CARTESIAN_POINT('Ctrl Pts',(6.01429994629887,3.6035847039371,47.398216464561));
#149554=CARTESIAN_POINT('Ctrl Pts',(6.10903907307722,3.4454672814514,47.3898547086854));
#149555=CARTESIAN_POINT('Ctrl Pts',(6.19752818793235,3.28362969949976,47.3814929528098));
#149556=CARTESIAN_POINT('Ctrl Pts',(6.27948847744328,3.11859760536,47.3731311969342));
#149557=CARTESIAN_POINT('Ctrl Pts',(6.36148111448179,2.95350037747987,47.3647661408979));
#149558=CARTESIAN_POINT('Ctrl Pts',(6.43693963536268,2.78520641485026,47.3564010848616));
#149559=CARTESIAN_POINT('Ctrl Pts',(6.50563230234053,2.61426374133205,47.3480360288252));
#149560=CARTESIAN_POINT('Ctrl Pts',(6.52818938709538,2.55813011682139,47.3452891376898));
#149561=CARTESIAN_POINT('Ctrl Pts',(6.5500172888635,2.50171103305673,47.3425422465544));
#149562=CARTESIAN_POINT('Ctrl Pts',(6.57110895151816,2.44502632087632,47.3397953554189));
#149563=CARTESIAN_POINT('Origin',(0.,0.,50.));
#149564=CARTESIAN_POINT('',(6.57110895151812,2.4450263208764,45.3397873838214));
#149565=CARTESIAN_POINT('',(6.57110895151812,2.4450263208764,45.8869210003222));
#149566=CARTESIAN_POINT('',(6.57110895151814,2.44502632087636,50.));
#149567=CARTESIAN_POINT('',(7.01125,3.56735040812906E-12,47.7735343569105));
#149568=CARTESIAN_POINT('Ctrl Pts',(6.57110895151812,2.4450263208764,45.8869210003222));
#149569=CARTESIAN_POINT('Ctrl Pts',(6.50449838733133,2.62404495591367,45.895592809261));
#149570=CARTESIAN_POINT('Ctrl Pts',(6.43056821795842,2.80033990716037,45.9042646181998));
#149571=CARTESIAN_POINT('Ctrl Pts',(6.34956511459209,2.97332295892242,45.9129364271385));
#149572=CARTESIAN_POINT('Ctrl Pts',(6.26856213015448,3.14630575671081,45.9216082233454));
#149573=CARTESIAN_POINT('Ctrl Pts',(6.18048635294189,3.3159764075484,45.9302800195522));
#149574=CARTESIAN_POINT('Ctrl Pts',(6.08563165071444,3.48176879966529,45.9389518157591));
#149575=CARTESIAN_POINT('Ctrl Pts',(5.99077708581834,3.6475609517467,45.9476235994108));
#149576=CARTESIAN_POINT('Ctrl Pts',(5.88914375657957,3.8094746098397,45.9562953830625));
#149577=CARTESIAN_POINT('Ctrl Pts',(5.7810707650006,3.9669695452014,45.9649671667143));
#149578=CARTESIAN_POINT('Ctrl Pts',(5.67299792768672,4.12446425575235,45.9736389379878));
#149579=CARTESIAN_POINT('Ctrl Pts',(5.55848560711145,4.27754002202802,45.9823107092613));
#149580=CARTESIAN_POINT('Ctrl Pts',(5.43791587524628,4.42568610457684,45.9909824805348));
#149581=CARTESIAN_POINT('Ctrl Pts',(5.31734631302621,4.57383197867983,45.9996542396069));
#149582=CARTESIAN_POINT('Ctrl Pts',(5.19071953583538,4.71704796267164,46.0083259986789));
#149583=CARTESIAN_POINT('Ctrl Pts',(5.05845803451277,4.85485621574658,46.016997757751));
#149584=CARTESIAN_POINT('Ctrl Pts',(4.92619671658875,4.99266427773161,46.0256695047985));
#149585=CARTESIAN_POINT('Ctrl Pts',(4.78830088681432,5.12506441891224,46.034341251846));
#149586=CARTESIAN_POINT('Ctrl Pts',(4.64523063400086,5.25161488681719,46.0430129988935));
#149587=CARTESIAN_POINT('Ctrl Pts',(4.49652806262013,5.38314733061205,46.0520261309665));
#149588=CARTESIAN_POINT('Ctrl Pts',(4.34223563523578,5.50835996364566,46.0610392630395));
#149589=CARTESIAN_POINT('Ctrl Pts',(4.18290943344173,5.62680151010538,46.0700523951125));
#149590=CARTESIAN_POINT('Ctrl Pts',(4.02607270355069,5.74339240740169,46.0789246969969));
#149591=CARTESIAN_POINT('Ctrl Pts',(3.8643586282001,5.85342208902884,46.0877969988812));
#149592=CARTESIAN_POINT('Ctrl Pts',(3.69833198496072,5.9565062823367,46.0966693007656));
#149593=CARTESIAN_POINT('Ctrl Pts',(3.53489950802194,6.05797978512413,46.105402972933));
#149594=CARTESIAN_POINT('Ctrl Pts',(3.36728850946689,6.15272311280124,46.1141366451004));
#149595=CARTESIAN_POINT('Ctrl Pts',(3.19606623000572,6.24041562845914,46.1228703172679));
#149596=CARTESIAN_POINT('Ctrl Pts',(3.02603797480699,6.32749661744154,46.1315430848818));
#149597=CARTESIAN_POINT('Ctrl Pts',(2.8524489133494,6.40762471321783,46.1402158524958));
#149598=CARTESIAN_POINT('Ctrl Pts',(2.67587836094736,6.48053250589129,46.1488886201098));
#149599=CARTESIAN_POINT('Ctrl Pts',(2.49930871513026,6.55343992422653,46.1575613431943));
#149600=CARTESIAN_POINT('Ctrl Pts',(2.31975787164533,6.61912700519576,46.1662340662788));
#149601=CARTESIAN_POINT('Ctrl Pts',(2.13782503579629,6.67737453486193,46.1749067893633));
#149602=CARTESIAN_POINT('Ctrl Pts',(1.95589311921358,6.73562177021623,46.1835794686264));
#149603=CARTESIAN_POINT('Ctrl Pts',(1.77157950496551,6.7864294428502,46.1922521478895));
#149604=CARTESIAN_POINT('Ctrl Pts',(1.58549928668296,6.82962799678195,46.2009248271527));
#149605=CARTESIAN_POINT('Ctrl Pts',(1.39941999343375,6.87282633596706,46.2095974633026));
#149606=CARTESIAN_POINT('Ctrl Pts',(1.21157439050145,6.90841556789004,46.2182700994525));
#149607=CARTESIAN_POINT('Ctrl Pts',(1.02258935228606,6.93627692491377,46.2269427356024));
#149608=CARTESIAN_POINT('Ctrl Pts',(0.833605238118976,6.96413814570851,
46.2356153293472));
#149609=CARTESIAN_POINT('Ctrl Pts',(0.643481980910279,6.98427152577672,
46.2442879230919));
#149610=CARTESIAN_POINT('Ctrl Pts',(0.452854049801629,6.99660987708178,
46.2529605168367));
#149611=CARTESIAN_POINT('Ctrl Pts',(0.262227035215384,7.00894816906512,
46.2616330688844));
#149612=CARTESIAN_POINT('Ctrl Pts',(0.0710956351155785,7.01349148893093,
46.2703056209321));
#149613=CARTESIAN_POINT('Ctrl Pts',(-0.119902323162865,7.01022467510137,
46.2789781729798));
#149614=CARTESIAN_POINT('Ctrl Pts',(-0.310899378728219,7.00695787671175,
46.2876506840385));
#149615=CARTESIAN_POINT('Ctrl Pts',(-0.501762709658449,6.99588102335243,
46.2963231950972));
#149616=CARTESIAN_POINT('Ctrl Pts',(-0.691855389210719,6.97703107940047,
46.3049957061558));
#149617=CARTESIAN_POINT('Ctrl Pts',(-0.881947185842832,6.95818122300052,
46.3136681769334));
#149618=CARTESIAN_POINT('Ctrl Pts',(-1.07126805553568,6.93155837629042,
46.322340647711));
#149619=CARTESIAN_POINT('Ctrl Pts',(-1.25918622473028,6.89725138109012,
46.3310131184886));
#149620=CARTESIAN_POINT('Ctrl Pts',(-1.44710353644051,6.86294454243514,
46.339685549693));
#149621=CARTESIAN_POINT('Ctrl Pts',(-1.63361788097595,6.82095367647916,
46.3483579808975));
#149622=CARTESIAN_POINT('Ctrl Pts',(-1.81810685597207,6.77141890764169,
46.357030412102));
#149623=CARTESIAN_POINT('Ctrl Pts',(-2.00259500418734,6.72188436079254,
46.3657028044413));
#149624=CARTESIAN_POINT('Ctrl Pts',(-2.18505752664676,6.66480605238501,
46.3743751967805));
#149625=CARTESIAN_POINT('Ctrl Pts',(-2.36488554745479,6.60037445225189,
46.3830475891198));
#149626=CARTESIAN_POINT('Ctrl Pts',(-2.54471277704449,6.53594313560888,
46.3917199433018));
#149627=CARTESIAN_POINT('Ctrl Pts',(-2.72190526073538,6.46415868780674,
46.4003922974837));
#149628=CARTESIAN_POINT('Ctrl Pts',(-2.89587171390473,6.38526065083537,
46.4090646516657));
#149629=CARTESIAN_POINT('Ctrl Pts',(-3.06983741584206,6.30636295456607,
46.4177369683982));
#149630=CARTESIAN_POINT('Ctrl Pts',(-3.2405768564137,6.22035184793457,46.4264092851306));
#149631=CARTESIAN_POINT('Ctrl Pts',(-3.40752028947368,6.12751434427739,
46.4350816018631));
#149632=CARTESIAN_POINT('Ctrl Pts',(-3.57446301525142,6.03467723394097,
46.443753881854));
#149633=CARTESIAN_POINT('Ctrl Pts',(-3.73760951742763,5.9350139225178,46.4524261618448));
#149634=CARTESIAN_POINT('Ctrl Pts',(-3.89641539159459,5.82885697702773,
46.4610984418357));
#149635=CARTESIAN_POINT('Ctrl Pts',(-4.05522060591328,5.72270047262635,
46.4697706857927));
#149636=CARTESIAN_POINT('Ctrl Pts',(-4.20968499214723,5.61005054602113,
46.4784429297497));
#149637=CARTESIAN_POINT('Ctrl Pts',(-4.35929312156537,5.49128309621466,
46.4871151737067));
#149638=CARTESIAN_POINT('Ctrl Pts',(-4.50890064155975,5.37251613020347,
46.4957873823375));
#149639=CARTESIAN_POINT('Ctrl Pts',(-4.65365172183918,5.24763186747866,
46.5044595909684));
#149640=CARTESIAN_POINT('Ctrl Pts',(-4.79306334971558,5.11704702813187,
46.5131317995993));
#149641=CARTESIAN_POINT('Ctrl Pts',(-4.93247442107824,4.9864627100634,46.5218039736118));
#149642=CARTESIAN_POINT('Ctrl Pts',(-5.06654587537236,4.85017805510181,
46.5304761476244));
#149643=CARTESIAN_POINT('Ctrl Pts',(-5.1948303397914,4.70864782111412,46.5391483216369));
#149644=CARTESIAN_POINT('Ctrl Pts',(-5.32311430258135,4.56711814055029,
46.5478204617387));
#149645=CARTESIAN_POINT('Ctrl Pts',(-5.44561113001101,4.42034313247171,
46.5564926018405));
#149646=CARTESIAN_POINT('Ctrl Pts',(-5.56191207495656,4.26881255537795,
46.5651647419424));
#149647=CARTESIAN_POINT('Ctrl Pts',(-5.67821257462083,4.11728255844911,
46.5738368488412));
#149648=CARTESIAN_POINT('Ctrl Pts',(-5.78831706632673,3.96099725427349,
46.58250895574));
#149649=CARTESIAN_POINT('Ctrl Pts',(-5.89185815647741,3.80047813129488,
46.5911810626388));
#149650=CARTESIAN_POINT('Ctrl Pts',(-5.99539885864796,3.6399596097995,46.5998531370423));
#149651=CARTESIAN_POINT('Ctrl Pts',(-6.09237605451008,3.47520753994365,
46.6085252114457));
#149652=CARTESIAN_POINT('Ctrl Pts',(-6.18246615568418,3.30677165772293,
46.6171972858492));
#149653=CARTESIAN_POINT('Ctrl Pts',(-6.27255592663025,3.13833639290911,
46.6258693284649));
#149654=CARTESIAN_POINT('Ctrl Pts',(-6.35575851944183,2.9662175932161,46.6345413710806));
#149655=CARTESIAN_POINT('Ctrl Pts',(-6.4317963101397,2.79098957134801,46.6432134136963));
#149656=CARTESIAN_POINT('Ctrl Pts',(-6.50783382832182,2.61576217748865,
46.6518854252318));
#149657=CARTESIAN_POINT('Ctrl Pts',(-6.57670648270859,2.43742584431381,
46.6605574367673));
#149658=CARTESIAN_POINT('Ctrl Pts',(-6.63818446599706,2.25657562645157,
46.6692294483029));
#149659=CARTESIAN_POINT('Ctrl Pts',(-6.69966223396684,2.07572604199386,
46.6779014294658));
#149660=CARTESIAN_POINT('Ctrl Pts',(-6.7537452912495,1.8923628593846,46.6865734106287));
#149661=CARTESIAN_POINT('Ctrl Pts',(-6.80025318023576,1.70709790205291,
46.6952453917916));
#149662=CARTESIAN_POINT('Ctrl Pts',(-6.846760910128,1.52183357847489,46.7039173432895));
#149663=CARTESIAN_POINT('Ctrl Pts',(-6.88569345442436,1.33466776867056,
46.7125892947873));
#149664=CARTESIAN_POINT('Ctrl Pts',(-6.91692090874809,1.14622497993348,
46.7212612462851));
#149665=CARTESIAN_POINT('Ctrl Pts',(-6.94814825879637,0.957782820449011,
46.7299331688254));
#149666=CARTESIAN_POINT('Ctrl Pts',(-6.97167052392585,0.768063970763964,
46.7386050913656));
#149667=CARTESIAN_POINT('Ctrl Pts',(-6.98740921903211,0.577701452555783,
46.7472770139059));
#149668=CARTESIAN_POINT('Ctrl Pts',(-7.00314786286725,0.387339554481687,
46.7559489081961));
#149669=CARTESIAN_POINT('Ctrl Pts',(-7.01110296401766,0.196334275130466,
46.7646208024863));
#149670=CARTESIAN_POINT('Ctrl Pts',(-7.01124797942393,0.00532292437173847,
46.7732926967765));
#149671=CARTESIAN_POINT('Ctrl Pts',(-7.01139299436962,-0.185687819719586,
46.781964563524));
#149672=CARTESIAN_POINT('Ctrl Pts',(-7.00372797299397,-0.376704351168703,
46.7906364302716));
#149673=CARTESIAN_POINT('Ctrl Pts',(-6.98827849031139,-0.567089326606621,
46.7993082970191));
#149674=CARTESIAN_POINT('Ctrl Pts',(-6.97282905543744,-0.757473712895766,
46.8079801369314));
#149675=CARTESIAN_POINT('Ctrl Pts',(-6.94959523043274,-0.947226264008327,
46.8166519768438));
#149676=CARTESIAN_POINT('Ctrl Pts',(-6.91865453650782,-1.1357138578708,
46.8253238167561));
#149677=CARTESIAN_POINT('Ctrl Pts',(-6.88771393580554,-1.32420088383036,
46.8339956305407));
#149678=CARTESIAN_POINT('Ctrl Pts',(-6.84906655865352,-1.51142267991482,
46.8426674443253));
#149679=CARTESIAN_POINT('Ctrl Pts',(-6.80284135383333,-1.69675457184448,
46.8513392581098));
#149680=CARTESIAN_POINT('Ctrl Pts',(-6.75661628451684,-1.88208592049568,
46.860011046474));
#149681=CARTESIAN_POINT('Ctrl Pts',(-6.70281350071267,-2.06552710052184,
46.8686828348382));
#149682=CARTESIAN_POINT('Ctrl Pts',(-6.64161251687414,-2.24646605543035,
46.8773546232023));
#149683=CARTESIAN_POINT('Ctrl Pts',(-6.58041170744734,-2.42740449469558,
46.8860263868535));
#149684=CARTESIAN_POINT('Ctrl Pts',(-6.51181283117083,-2.60584045409099,
46.8946981505046));
#149685=CARTESIAN_POINT('Ctrl Pts',(-6.43604476876016,-2.78117858056885,
46.9033699141557));
#149686=CARTESIAN_POINT('Ctrl Pts',(-6.35684774728027,-2.964451808458,46.9124341271011));
#149687=CARTESIAN_POINT('Ctrl Pts',(-6.26981768815432,-3.14433998862709,
46.9214983400465));
#149688=CARTESIAN_POINT('Ctrl Pts',(-6.17527181577862,-3.32018742900912,
46.9305625529918));
#149689=CARTESIAN_POINT('Ctrl Pts',(-6.08368050191467,-3.49053963687921,
46.9393435092827));
#149690=CARTESIAN_POINT('Ctrl Pts',(-5.98503618716342,-3.65709956719063,
46.9481244655735));
#149691=CARTESIAN_POINT('Ctrl Pts',(-5.87967633129822,-3.81929742252048,
46.9569054218643));
#149692=CARTESIAN_POINT('Ctrl Pts',(-5.77561495477403,-3.97949631379923,
46.9655781596098));
#149693=CARTESIAN_POINT('Ctrl Pts',(-5.66500279404917,-4.1354398025804,
46.9742508973553));
#149694=CARTESIAN_POINT('Ctrl Pts',(-5.54820899034255,-4.28660746534857,
46.9829236351008));
#149695=CARTESIAN_POINT('Ctrl Pts',(-5.43141636368016,-4.43777360465386,
46.9915962854427));
#149696=CARTESIAN_POINT('Ctrl Pts',(-5.30844239242327,-4.58416378941009,
47.0002689357846));
#149697=CARTESIAN_POINT('Ctrl Pts',(-5.1796974640672,-4.72528948777066,
47.0089415861265));
#149698=CARTESIAN_POINT('Ctrl Pts',(-5.05095379116422,-4.86641380994734,
47.0176141518973));
#149699=CARTESIAN_POINT('Ctrl Pts',(-4.91643946526549,-5.00227353855249,
47.0262867176681));
#149700=CARTESIAN_POINT('Ctrl Pts',(-4.77660337747524,-5.132415292705,47.0349592834388));
#149701=CARTESIAN_POINT('Ctrl Pts',(-4.63676860764104,-5.26255582027063,
47.0436317674706));
#149702=CARTESIAN_POINT('Ctrl Pts',(-4.49161238426534,-5.38697828766591,
47.0523042515024));
#149703=CARTESIAN_POINT('Ctrl Pts',(-4.34161910267142,-5.50526748939764,
47.0609767355342));
#149704=CARTESIAN_POINT('Ctrl Pts',(-4.19162718580059,-5.62355561486781,
47.0696491406588));
#149705=CARTESIAN_POINT('Ctrl Pts',(-4.03679852185878,-5.73571041041759,
47.0783215457835));
#149706=CARTESIAN_POINT('Ctrl Pts',(-3.87764977431105,-5.84135761533956,
47.0869939509081));
#149707=CARTESIAN_POINT('Ctrl Pts',(-3.71850242283774,-5.94700389350991,
47.0956662799573));
#149708=CARTESIAN_POINT('Ctrl Pts',(-3.55503530027938,-6.0461425381676,
47.1043386090064));
#149709=CARTESIAN_POINT('Ctrl Pts',(-3.38779388708872,-6.13844272931697,
47.1130109380556));
#149710=CARTESIAN_POINT('Ctrl Pts',(-3.22055388637478,-6.23074214092334,
47.1216831938605));
#149711=CARTESIAN_POINT('Ctrl Pts',(-3.04953990753037,-6.31620307733225,
47.1303554496654));
#149712=CARTESIAN_POINT('Ctrl Pts',(-2.87532260480704,-6.39454036509159,
47.1390277054704));
#149713=CARTESIAN_POINT('Ctrl Pts',(-2.70110671661545,-6.47287701680285,
47.1476998908622));
#149714=CARTESIAN_POINT('Ctrl Pts',(-2.52368781567056,-6.54409001911157,
47.1563720762541));
#149715=CARTESIAN_POINT('Ctrl Pts',(-2.34365791911847,-6.6079417461607,
47.1650442616459));
#149716=CARTESIAN_POINT('Ctrl Pts',(-2.16362942553754,-6.67179297561396,
47.1737163794555));
#149717=CARTESIAN_POINT('Ctrl Pts',(-1.98099024478141,-6.72828294965251,
47.1823884972651));
#149718=CARTESIAN_POINT('Ctrl Pts',(-1.79634980370613,-6.77722317363277,
47.1910606150747));
#149719=CARTESIAN_POINT('Ctrl Pts',(-1.61171074127587,-6.82616303219364,
47.1997326681326));
#149720=CARTESIAN_POINT('Ctrl Pts',(-1.42507072299089,-6.8675531807264,
47.2084047211905));
#149721=CARTESIAN_POINT('Ctrl Pts',(-1.23705251633311,-6.90125551145108,
47.2170767742485));
#149722=CARTESIAN_POINT('Ctrl Pts',(-1.04903565218561,-6.93495760153032,
47.2257487653852));
#149723=CARTESIAN_POINT('Ctrl Pts',(-0.85964089893486,-6.96097193353472,
47.2344207565219));
#149724=CARTESIAN_POINT('Ctrl Pts',(-0.66950020685584,-6.97921170588198,
47.2430927476586));
#149725=CARTESIAN_POINT('Ctrl Pts',(-0.479360810398374,-6.99745135394315,
47.2517646797042));
#149726=CARTESIAN_POINT('Ctrl Pts',(-0.288475768009516,-7.00791652123639,
47.2604366117498));
#149727=CARTESIAN_POINT('Ctrl Pts',(-0.0974819939155687,-7.0105722892901,
47.2691085437955));
#149728=CARTESIAN_POINT('Ctrl Pts',(0.0935105410641958,-7.01322804011393,
47.27778041958));
#149729=CARTESIAN_POINT('Ctrl Pts',(0.284611522350782,-7.00807448913577,
47.2864522953646));
#149730=CARTESIAN_POINT('Ctrl Pts',(0.475183323473319,-6.99512883166514,
47.2951241711491));
#149731=CARTESIAN_POINT('Ctrl Pts',(0.665753950397314,-6.98218325395852,
47.3037959935024));
#149732=CARTESIAN_POINT('Ctrl Pts',(0.855795120329706,-6.9614456850821,
47.3124678158556));
#149733=CARTESIAN_POINT('Ctrl Pts',(1.04467275076626,-6.93298531704103,
47.3211396382088));
#149734=CARTESIAN_POINT('Ctrl Pts',(1.23354927906719,-6.90452511507142,
47.3298114099604));
#149735=CARTESIAN_POINT('Ctrl Pts',(1.42126200063211,-6.86834224643024,
47.3384831817119));
#149736=CARTESIAN_POINT('Ctrl Pts',(1.60718460925101,-6.82455743578195,
47.3471549534635));
#149737=CARTESIAN_POINT('Ctrl Pts',(1.79763389406226,-6.77970659200611,
47.356037857702));
#149738=CARTESIAN_POINT('Ctrl Pts',(1.98620448432225,-6.72687898190764,
47.3649207619404));
#149739=CARTESIAN_POINT('Ctrl Pts',(2.17223623428182,-6.66625954377514,
47.3738036661789));
#149740=CARTESIAN_POINT('Ctrl Pts',(2.3538653218636,-6.60707473666497,47.3824763459353));
#149741=CARTESIAN_POINT('Ctrl Pts',(2.53307410228002,-6.54046283696397,
47.3911490256916));
#149742=CARTESIAN_POINT('Ctrl Pts',(2.70926451774568,-6.46664614273769,
47.3998217054479));
#149743=CARTESIAN_POINT('Ctrl Pts',(2.88545151536487,-6.39283088045156,
47.4084942169665));
#149744=CARTESIAN_POINT('Ctrl Pts',(3.05862000314713,-6.3118112131087,47.417166728485));
#149745=CARTESIAN_POINT('Ctrl Pts',(3.22819210344548,-6.22385751007784,
47.4258392400036));
#149746=CARTESIAN_POINT('Ctrl Pts',(3.39776113571412,-6.13590539837345,
47.4345115946123));
#149747=CARTESIAN_POINT('Ctrl Pts',(3.56373365851512,-6.04101963283718,
47.4431839492211));
#149748=CARTESIAN_POINT('Ctrl Pts',(3.72555582775681,-5.93951684371442,
47.4518563038298));
#149749=CARTESIAN_POINT('Ctrl Pts',(3.88737528046907,-5.83801575853195,
47.4605285128546));
#149750=CARTESIAN_POINT('Ctrl Pts',(4.0450442783934,-5.72989802299362,47.4692007218795));
#149751=CARTESIAN_POINT('Ctrl Pts',(4.19803670363638,-5.61552440983225,
47.4778729309043));
#149752=CARTESIAN_POINT('Ctrl Pts',(4.35102676030492,-5.50115256736257,
47.4865450056691));
#149753=CARTESIAN_POINT('Ctrl Pts',(4.49934016166879,-5.38052521115584,
47.4952170804338));
#149754=CARTESIAN_POINT('Ctrl Pts',(4.64248202337103,-5.25404484422971,
47.5038891551986));
#149755=CARTESIAN_POINT('Ctrl Pts',(4.78562185584888,-5.12756627032935,
47.5125611070253));
#149756=CARTESIAN_POINT('Ctrl Pts',(4.92359008252787,-4.99523503981853,
47.5212330588519));
#149757=CARTESIAN_POINT('Ctrl Pts',(5.05592635132523,-4.85749269608048,
47.5299050106786));
#149758=CARTESIAN_POINT('Ctrl Pts',(5.18826091680615,-4.71975212524111,
47.5385768508876));
#149759=CARTESIAN_POINT('Ctrl Pts',(5.31496347269748,-4.57660078535016,
47.5472486910965));
#149760=CARTESIAN_POINT('Ctrl Pts',(5.43561126742136,-4.42851631045681,
47.5559205313054));
#149761=CARTESIAN_POINT('Ctrl Pts',(5.56176013705839,-4.27367975367312,
47.5649877740389));
#149762=CARTESIAN_POINT('Ctrl Pts',(5.6812889568676,-4.11344992040764,47.5740550167725));
#149763=CARTESIAN_POINT('Ctrl Pts',(5.79376175354239,-3.94841123816776,
47.583122259506));
#149764=CARTESIAN_POINT('Ctrl Pts',(5.90133874236535,-3.79055649462464,
47.5917948158845));
#149765=CARTESIAN_POINT('Ctrl Pts',(6.00246078174406,-3.62830291661375,
47.6004673722629));
#149766=CARTESIAN_POINT('Ctrl Pts',(6.09679041553473,-3.46219196341621,
47.6091399286413));
#149767=CARTESIAN_POINT('Ctrl Pts',(6.19111669178891,-3.29608692271475,
47.6178121763318));
#149768=CARTESIAN_POINT('Ctrl Pts',(6.27865090596437,-3.1261250286051,47.6264844240222));
#149769=CARTESIAN_POINT('Ctrl Pts',(6.35910096686233,-2.9528734235911,47.6351566717127));
#149770=CARTESIAN_POINT('Ctrl Pts',(6.43954858437163,-2.77962708048742,
47.643828656014));
#149771=CARTESIAN_POINT('Ctrl Pts',(6.51291235952087,-2.60309148403624,
47.6525006403153));
#149772=CARTESIAN_POINT('Ctrl Pts',(6.57894750102587,-2.42385567665353,
47.6611726246166));
#149773=CARTESIAN_POINT('Ctrl Pts',(6.64498098171233,-2.24462437714561,
47.6698443908129));
#149774=CARTESIAN_POINT('Ctrl Pts',(6.70368609940979,-2.06269326909623,
47.6785161570093));
#149775=CARTESIAN_POINT('Ctrl Pts',(6.7548669838948,-1.87866936750137,47.6871879232056));
#149776=CARTESIAN_POINT('Ctrl Pts',(6.80605126222585,-1.69463326313208,
47.6958602644338));
#149777=CARTESIAN_POINT('Ctrl Pts',(6.84971023276694,-1.5085043611762,47.704532605662));
#149778=CARTESIAN_POINT('Ctrl Pts',(6.88569820761785,-1.32090376489296,
47.7132049468903));
#149779=CARTESIAN_POINT('Ctrl Pts',(6.92168406448285,-1.13331420939267,
47.7218767777286));
#149780=CARTESIAN_POINT('Ctrl Pts',(6.9499997755384,-0.944253411825118,
47.730548608567));
#149781=CARTESIAN_POINT('Ctrl Pts',(6.9705508637189,-0.754352184863043,
47.7392204394054));
#149782=CARTESIAN_POINT('Ctrl Pts',(6.99110229108043,-0.564447823716972,
47.7478924133661));
#149783=CARTESIAN_POINT('Ctrl Pts',(7.00388880856507,-0.373703287791058,
47.7565643873269));
#149784=CARTESIAN_POINT('Ctrl Pts',(7.00886775178468,-0.182755028638717,
47.7652363612876));
#149785=CARTESIAN_POINT('Ctrl Pts',(7.01045582731897,-0.121850486188999,
47.7680023598286));
#149786=CARTESIAN_POINT('Ctrl Pts',(7.01125000000003,-0.0609252433271906,
47.7707683583695));
#149787=CARTESIAN_POINT('Ctrl Pts',(7.01125,3.56735043106814E-12,47.7735343569105));
#149788=CARTESIAN_POINT('Ctrl Pts',(7.01124848872571,0.00460345972294059,
47.7735343569105));
#149789=CARTESIAN_POINT('Ctrl Pts',(7.01111020263014,0.215218570302498,
47.7830916938172));
#149790=CARTESIAN_POINT('Ctrl Pts',(7.00147759625489,0.425596535594836,
47.7926490307239));
#149791=CARTESIAN_POINT('Ctrl Pts',(6.9824391034497,0.634957265582918,47.8022063676305));
#149792=CARTESIAN_POINT('Ctrl Pts',(6.96334835668509,0.844892617060276,
47.8117899360619));
#149793=CARTESIAN_POINT('Ctrl Pts',(6.93480007718454,1.05380505887218,47.8213735044934));
#149794=CARTESIAN_POINT('Ctrl Pts',(6.8969345210992,1.26092060581554,47.8309570729248));
#149795=CARTESIAN_POINT('Ctrl Pts',(6.85898843994858,1.46847660563112,47.8405610218168));
#149796=CARTESIAN_POINT('Ctrl Pts',(6.81168544968352,1.67422797938378,47.8501649707087));
#149797=CARTESIAN_POINT('Ctrl Pts',(6.75521722589369,1.87740959662223,47.8597689196007));
#149798=CARTESIAN_POINT('Ctrl Pts',(6.70193906218384,2.06911287219101,47.8688303124866));
#149799=CARTESIAN_POINT('Ctrl Pts',(6.6405023909177,2.25852859407412,47.8778917053725));
#149800=CARTESIAN_POINT('Ctrl Pts',(6.57110895151812,2.44502632087642,47.8869530982584));
#149801=CARTESIAN_POINT('',(7.01124900031637,0.0037440703390971,47.2264656430477));
#149802=CARTESIAN_POINT('Ctrl Pts',(6.57110895151816,2.44502632087632,47.3397953554189));
#149803=CARTESIAN_POINT('Ctrl Pts',(6.63537926896215,2.27229719535844,47.3314250544072));
#149804=CARTESIAN_POINT('Ctrl Pts',(6.69280958576941,2.09710061241682,47.3230547533954));
#149805=CARTESIAN_POINT('Ctrl Pts',(6.74323350051052,1.92000742709311,47.3146844523836));
#149806=CARTESIAN_POINT('Ctrl Pts',(6.79369723377461,1.74277439564464,47.3063075415514));
#149807=CARTESIAN_POINT('Ctrl Pts',(6.83714342931925,1.56364208808661,47.2979306307192));
#149808=CARTESIAN_POINT('Ctrl Pts',(6.87345634102338,1.38319358390121,47.2895537198869));
#149809=CARTESIAN_POINT('Ctrl Pts',(6.88306397555093,1.3354506958238,47.2873373650432));
#149810=CARTESIAN_POINT('Ctrl Pts',(6.89217254502337,1.28761571539511,47.2851210101995));
#149811=CARTESIAN_POINT('Ctrl Pts',(6.90078051029069,1.23969952459951,47.2829046553557));
#149812=CARTESIAN_POINT('Ctrl Pts',(6.93731384930597,1.03633689611582,47.2734981533114));
#149813=CARTESIAN_POINT('Ctrl Pts',(6.96489074497273,0.831146044054557,
47.264091651267));
#149814=CARTESIAN_POINT('Ctrl Pts',(6.98334685255806,0.624894630611765,
47.2546851492227));
#149815=CARTESIAN_POINT('Ctrl Pts',(7.00180296014339,0.418643217168973,
47.2452786471783));
#149816=CARTESIAN_POINT('Ctrl Pts',(7.01113814671998,0.211331509871976,
47.235872145134));
#149817=CARTESIAN_POINT('Ctrl Pts',(7.01124900031588,0.00374407126288481,
47.2264656430896));
#149818=CARTESIAN_POINT('Ctrl Pts',(7.01124900031637,0.00374407033909243,
47.2264656430477));
#149819=CARTESIAN_POINT('Ctrl Pts',(7.01133805377372,-0.163019880989669,
47.2189089938612));
#149820=CARTESIAN_POINT('Ctrl Pts',(7.00547309213724,-0.329959880594732,
47.2113523446747));
#149821=CARTESIAN_POINT('Ctrl Pts',(6.99364288946165,-0.496573959428494,
47.2037956954882));
#149822=CARTESIAN_POINT('Ctrl Pts',(6.98181519998804,-0.66315264285587,
47.1962406516323));
#149823=CARTESIAN_POINT('Ctrl Pts',(6.96402480635603,-0.829405141217421,
47.1886856077763));
#149824=CARTESIAN_POINT('Ctrl Pts',(6.94031258484574,-0.994830531865516,
47.1811305639204));
#149825=CARTESIAN_POINT('Ctrl Pts',(6.91660374076276,-1.16023236030828,
47.1735765961598));
#149826=CARTESIAN_POINT('Ctrl Pts',(6.88697480798972,-1.32480691708793,
47.1660226283992));
#149827=CARTESIAN_POINT('Ctrl Pts',(6.85151831906088,-1.4880602427567,47.1584686606386));
#149828=CARTESIAN_POINT('Ctrl Pts',(6.81604972350294,-1.65136931132397,
47.1509121135734));
#149829=CARTESIAN_POINT('Ctrl Pts',(6.77474968933664,-1.81335585520407,
47.1433555665082));
#149830=CARTESIAN_POINT('Ctrl Pts',(6.72776143470871,-1.97353810202544,
47.135799019443));
#149831=CARTESIAN_POINT('Ctrl Pts',(6.70379677739981,-2.05523325504701,
47.1319450763184));
#149832=CARTESIAN_POINT('Ctrl Pts',(6.67835333670491,-2.13645932533242,
47.1280911331939));
#149833=CARTESIAN_POINT('Ctrl Pts',(6.65145502672404,-2.21715416468216,
47.1242371900694));
#149834=CARTESIAN_POINT('Ctrl Pts',(6.58406734638552,-2.41931697873763,
47.1145820003009));
#149835=CARTESIAN_POINT('Ctrl Pts',(6.50755438751975,-2.61811991118926,
47.1049268105323));
#149836=CARTESIAN_POINT('Ctrl Pts',(6.42227030571619,-2.81284032302157,
47.0952716207638));
#149837=CARTESIAN_POINT('Ctrl Pts',(6.33651370934528,-3.00863957898522,
47.0855629366301));
#149838=CARTESIAN_POINT('Ctrl Pts',(6.2418885974367,-3.2003109294957,47.0758542524964));
#149839=CARTESIAN_POINT('Ctrl Pts',(6.13879776728405,-3.38715050372556,
47.0661455683627));
#149840=CARTESIAN_POINT('Ctrl Pts',(6.03521067167438,-3.57488949865616,
47.0563901479231));
#149841=CARTESIAN_POINT('Ctrl Pts',(5.92307619790506,-3.757750059978,47.0466347274835));
#149842=CARTESIAN_POINT('Ctrl Pts',(5.8028451586132,-3.93504950765036,47.036879307044));
#149843=CARTESIAN_POINT('Ctrl Pts',(5.68249490884342,-4.11252474979324,
47.0271142139912));
#149844=CARTESIAN_POINT('Ctrl Pts',(5.55403206681813,-4.2844278237235,47.0173491209385));
#149845=CARTESIAN_POINT('Ctrl Pts',(5.41795030919277,-4.45010573016169,
47.0075840278858));
#149846=CARTESIAN_POINT('Ctrl Pts',(5.2820537653651,-4.61555814102444,46.997832225593));
#149847=CARTESIAN_POINT('Ctrl Pts',(5.13855905542658,-4.77480228909225,
46.9880804233002));
#149848=CARTESIAN_POINT('Ctrl Pts',(4.98799875327024,-4.92721980429883,
46.9783286210073));
#149849=CARTESIAN_POINT('Ctrl Pts',(4.92233624928531,-4.99369227782795,
46.9740756555992));
#149850=CARTESIAN_POINT('Ctrl Pts',(4.85533038262588,-5.0588667289273,46.969822690191));
#149851=CARTESIAN_POINT('Ctrl Pts',(4.7870277619448,-5.12269380003039,46.9655697247829));
#149852=CARTESIAN_POINT('Ctrl Pts',(4.65802278161931,-5.24324569056962,
46.9575370356513));
#149853=CARTESIAN_POINT('Ctrl Pts',(4.5243262391785,-5.35904729458481,46.9495043465197));
#149854=CARTESIAN_POINT('Ctrl Pts',(4.38633022244782,-5.46971057206329,
46.9414716573881));
#149855=CARTESIAN_POINT('Ctrl Pts',(4.24842295027931,-5.58030268253027,
46.9334441340395));
#149856=CARTESIAN_POINT('Ctrl Pts',(4.10622199235734,-5.68576281560668,
46.9254166106909));
#149857=CARTESIAN_POINT('Ctrl Pts',(3.96015481489761,-5.78574112837269,
46.9173890873423));
#149858=CARTESIAN_POINT('Ctrl Pts',(3.81415362062243,-5.88567427775856,
46.9093651902811));
#149859=CARTESIAN_POINT('Ctrl Pts',(3.66428998616904,-5.9801303308086,46.9013412932198));
#149860=CARTESIAN_POINT('Ctrl Pts',(3.51102280616601,-6.06880098677508,
46.8933173961586));
#149861=CARTESIAN_POINT('Ctrl Pts',(3.35777418886415,-6.15746090354163,
46.8852944708983));
#149862=CARTESIAN_POINT('Ctrl Pts',(3.20112316035059,-6.24033662872264,
46.8772715456381));
#149863=CARTESIAN_POINT('Ctrl Pts',(3.04155597700651,-6.31716422148704,
46.8692486203779));
#149864=CARTESIAN_POINT('Ctrl Pts',(2.88200189084887,-6.39398550828499,
46.8612263536349));
#149865=CARTESIAN_POINT('Ctrl Pts',(2.71953245875733,-6.46475949605074,
46.853204086892));
#149866=CARTESIAN_POINT('Ctrl Pts',(2.55465653826101,-6.5292692189877,46.8451818201491));
#149867=CARTESIAN_POINT('Ctrl Pts',(2.38971864118606,-6.59380319102001,
46.8371565378497));
#149868=CARTESIAN_POINT('Ctrl Pts',(2.22237279135252,-6.65206806339079,
46.8291312555503));
#149869=CARTESIAN_POINT('Ctrl Pts',(2.05314609058131,-6.70389571019946,
46.8211059732509));
#149870=CARTESIAN_POINT('Ctrl Pts',(1.95330961847189,-6.73447179181974,
46.8163714019994));
#149871=CARTESIAN_POINT('Ctrl Pts',(1.85281882675055,-6.76280834132154,
46.811636830748));
#149872=CARTESIAN_POINT('Ctrl Pts',(1.75178407774357,-6.78887907591998,
46.8069022594965));
#149873=CARTESIAN_POINT('Ctrl Pts',(1.56547532649853,-6.83695368445631,
46.798171678521));
#149874=CARTESIAN_POINT('Ctrl Pts',(1.37722330343465,-6.87734522639827,
46.7894410975456));
#149875=CARTESIAN_POINT('Ctrl Pts',(1.18766252571079,-6.90992650377139,
46.7807105165701));
#149876=CARTESIAN_POINT('Ctrl Pts',(0.99804667740148,-6.94251724655207,
46.7719773992144));
#149877=CARTESIAN_POINT('Ctrl Pts',(0.807121585391957,-6.96729314928906,
46.7632442818587));
#149878=CARTESIAN_POINT('Ctrl Pts',(0.615529822806346,-6.98417852003627,
46.7545111645031));
#149879=CARTESIAN_POINT('Ctrl Pts',(0.421234205747432,-7.00130218696391,
46.745654800312));
#149880=CARTESIAN_POINT('Ctrl Pts',(0.22625324723321,-7.01031089814164,
46.7367984361209));
#149881=CARTESIAN_POINT('Ctrl Pts',(0.0312606778596215,-7.01118030951421,
46.7279420719298));
#149882=CARTESIAN_POINT('Ctrl Pts',(-0.161141059103698,-7.01203816916884,
46.7192033807119));
#149883=CARTESIAN_POINT('Ctrl Pts',(-0.353553822554361,-7.00497170861606,
46.710464689494));
#149884=CARTESIAN_POINT('Ctrl Pts',(-0.545331116062804,-6.99001005266471,
46.7017259982761));
#149885=CARTESIAN_POINT('Ctrl Pts',(-0.740982045293665,-6.97474619198464,
46.6928107975984));
#149886=CARTESIAN_POINT('Ctrl Pts',(-0.935971264890385,-6.95126481781544,
46.6838955969208));
#149887=CARTESIAN_POINT('Ctrl Pts',(-1.12961752830356,-6.91965250588853,
46.6749803962431));
#149888=CARTESIAN_POINT('Ctrl Pts',(-1.32326379171673,-6.88804019396161,
46.6660651955655));
#149889=CARTESIAN_POINT('Ctrl Pts',(-1.51556680177303,-6.84829699893491,
46.6571499948878));
#149890=CARTESIAN_POINT('Ctrl Pts',(-1.70585504549666,-6.80056505933541,
46.6482347942101));
#149891=CARTESIAN_POINT('Ctrl Pts',(-1.8924107996392,-6.75376937813924,
46.6394944645229));
#149892=CARTESIAN_POINT('Ctrl Pts',(-2.07704992960731,-6.69929046862994,
46.6307541348356));
#149893=CARTESIAN_POINT('Ctrl Pts',(-2.25915114490896,-6.63730839022541,
46.6220138051484));
#149894=CARTESIAN_POINT('Ctrl Pts',(-2.44121948182397,-6.57533750268928,
46.6132750535282));
#149895=CARTESIAN_POINT('Ctrl Pts',(-2.62075056001516,-6.50586623989363,
46.604536301908));
#149896=CARTESIAN_POINT('Ctrl Pts',(-2.79713963903848,-6.42912407737008,
46.5957975502879));
#149897=CARTESIAN_POINT('Ctrl Pts',(-2.97582506732171,-6.35138283480659,
46.5869450318409));
#149898=CARTESIAN_POINT('Ctrl Pts',(-3.15128584389833,-6.26618014521787,
46.5780925133938));
#149899=CARTESIAN_POINT('Ctrl Pts',(-3.32291432147881,-6.17380490253871,
46.5692399949468));
#149900=CARTESIAN_POINT('Ctrl Pts',(-3.49225022036918,-6.08266358977518,
46.560505726661));
#149901=CARTESIAN_POINT('Ctrl Pts',(-3.65785532263737,-5.98454029265149,
46.5517714583752));
#149902=CARTESIAN_POINT('Ctrl Pts',(-3.81916997763898,-5.87975911448769,
46.5430371900894));
#149903=CARTESIAN_POINT('Ctrl Pts',(-3.98376060551057,-5.77285004349887,
46.5341255465618));
#149904=CARTESIAN_POINT('Ctrl Pts',(-4.14388440592885,-5.65900992260237,
46.5252139030341));
#149905=CARTESIAN_POINT('Ctrl Pts',(-4.2989763871825,-5.53863056945915,
46.5163022595065));
#149906=CARTESIAN_POINT('Ctrl Pts',(-4.4540683684362,-5.41825121631588,
46.5073906159788));
#149907=CARTESIAN_POINT('Ctrl Pts',(-4.60412828264362,-5.29133280628025,
46.4984789724512));
#149908=CARTESIAN_POINT('Ctrl Pts',(-4.7486246754473,-5.15831273327171,
46.4895673289236));
#149909=CARTESIAN_POINT('Ctrl Pts',(-4.87875740055003,-5.03851552409512,
46.4815415475536));
#149910=CARTESIAN_POINT('Ctrl Pts',(-5.00443717117772,-4.9137139901756,
46.4735157661836));
#149911=CARTESIAN_POINT('Ctrl Pts',(-5.12525756911808,-4.78428274798823,
46.4654899848136));
#149912=CARTESIAN_POINT('Ctrl Pts',(-5.24603963359131,-4.65489257128611,
46.457466749835));
#149913=CARTESIAN_POINT('Ctrl Pts',(-5.36196514505517,-4.52087587839287,
46.4494435148564));
#149914=CARTESIAN_POINT('Ctrl Pts',(-5.47266451228036,-4.38264414463771,
46.4414202798778));
#149915=CARTESIAN_POINT('Ctrl Pts',(-5.58334992904249,-4.24442983100647,
46.4333980559967));
#149916=CARTESIAN_POINT('Ctrl Pts',(-5.68881028482749,-4.10200182098042,
46.4253758321155));
#149917=CARTESIAN_POINT('Ctrl Pts',(-5.78871629840333,-3.95580461841832,
46.4173536082344));
#149918=CARTESIAN_POINT('Ctrl Pts',(-5.88865944579762,-3.80955307618052,
46.4093284025927));
#149919=CARTESIAN_POINT('Ctrl Pts',(-5.98304391732017,-3.65952984396228,
46.401303196951));
#149920=CARTESIAN_POINT('Ctrl Pts',(-6.07158355952368,-3.50620872770315,
46.3932779913094));
#149921=CARTESIAN_POINT('Ctrl Pts',(-6.16014064428648,-3.35285740675159,
46.3852512046796));
#149922=CARTESIAN_POINT('Ctrl Pts',(-6.24285043017741,-3.19620722929424,
46.3772244180497));
#149923=CARTESIAN_POINT('Ctrl Pts',(-6.31947287807022,-3.03675634614221,
46.3691976314199));
#149924=CARTESIAN_POINT('Ctrl Pts',(-6.39615683968545,-2.87717745327973,
46.3611644007579));
#149925=CARTESIAN_POINT('Ctrl Pts',(-6.46674355235671,-2.71479369835474,
46.3531311700958));
#149926=CARTESIAN_POINT('Ctrl Pts',(-6.53104100822,-2.5501235090577,46.3450979394338));
#149927=CARTESIAN_POINT('Ctrl Pts',(-6.56892116670468,-2.45310982811927,
46.3403652475016));
#149928=CARTESIAN_POINT('Ctrl Pts',(-6.60461934743842,-2.35530289510654,
46.3356325555694));
#149929=CARTESIAN_POINT('Ctrl Pts',(-6.63810442454595,-2.25681107125154,
46.3308998636373));
#149930=CARTESIAN_POINT('Ctrl Pts',(-6.70709429909258,-2.05388668944988,
46.3211490178614));
#149931=CARTESIAN_POINT('Ctrl Pts',(-6.76672836725575,-1.84793490421423,
46.3113981720856));
#149932=CARTESIAN_POINT('Ctrl Pts',(-6.8168066730418,-1.63974795162941,
46.3016473263097));
#149933=CARTESIAN_POINT('Ctrl Pts',(-6.86695709865057,-1.43126118047285,
46.2918824379408));
#149934=CARTESIAN_POINT('Ctrl Pts',(-6.90752422550909,-1.22053284070518,
46.282117549572));
#149935=CARTESIAN_POINT('Ctrl Pts',(-6.93835866734817,-1.00836777305433,
46.2723526612031));
#149936=CARTESIAN_POINT('Ctrl Pts',(-6.96914171415797,-0.79655634338794,
46.2626040490076));
#149937=CARTESIAN_POINT('Ctrl Pts',(-6.99022449267146,-0.583313009512905,
46.2528554368122));
#149938=CARTESIAN_POINT('Ctrl Pts',(-7.00150950686121,-0.369447138075453,
46.2431068246167));
#149939=CARTESIAN_POINT('Ctrl Pts',(-7.01276355231825,-0.15616816488158,
46.2333849649056));
#149940=CARTESIAN_POINT('Ctrl Pts',(-7.01427350758934,0.0577298954421971,
46.2236631051945));
#149941=CARTESIAN_POINT('Ctrl Pts',(-7.00599378042487,0.271436385085205,
46.2139412454834));
#149942=CARTESIAN_POINT('Ctrl Pts',(-6.99776883006673,0.483729040822207,
46.2042837034021));
#149943=CARTESIAN_POINT('Ctrl Pts',(-6.97988327480615,0.695832604492826,
46.1946261613208));
#149944=CARTESIAN_POINT('Ctrl Pts',(-6.95234327129287,0.90694520264944,
46.1849686192395));
#149945=CARTESIAN_POINT('Ctrl Pts',(-6.94023682415646,0.999749239808647,
46.1807232122766));
#149946=CARTESIAN_POINT('Ctrl Pts',(-6.92626538129789,1.09236168942198,
46.1764778053136));
#149947=CARTESIAN_POINT('Ctrl Pts',(-6.91043263731572,1.18471402778128,
46.1722323983507));
#149948=CARTESIAN_POINT('Ctrl Pts',(-6.88115006925828,1.35551914130519,
46.1643805428249));
#149949=CARTESIAN_POINT('Ctrl Pts',(-6.84550896167075,1.52536372061138,
46.1565286872992));
#149950=CARTESIAN_POINT('Ctrl Pts',(-6.80359719615246,1.69372127429703,
46.1486768317735));
#149951=CARTESIAN_POINT('Ctrl Pts',(-6.76169731632826,1.86203108371913,
46.1408272029435));
#149952=CARTESIAN_POINT('Ctrl Pts',(-6.7135304079491,2.02885433656054,46.1329775741136));
#149953=CARTESIAN_POINT('Ctrl Pts',(-6.65923534359031,2.19367527249993,
46.1251279452837));
#149954=CARTESIAN_POINT('Ctrl Pts',(-6.60494461383931,2.35848305007732,
46.1172789431233));
#149955=CARTESIAN_POINT('Ctrl Pts',(-6.54452682210903,2.52128846690054,
46.1094299409629));
#149956=CARTESIAN_POINT('Ctrl Pts',(-6.47817045745705,2.68159170766743,
46.1015809388025));
#149957=CARTESIAN_POINT('Ctrl Pts',(-6.41178049842918,2.8419761054922,46.0937279629113));
#149958=CARTESIAN_POINT('Ctrl Pts',(-6.33944610536298,2.99985544324744,
46.0858749870201));
#149959=CARTESIAN_POINT('Ctrl Pts',(-6.26140374268369,3.1547503441012,46.078022011129));
#149960=CARTESIAN_POINT('Ctrl Pts',(-6.18334155971995,3.30968458334621,
46.070167040831));
#149961=CARTESIAN_POINT('Ctrl Pts',(-6.0995687033109,3.4616325415747,46.0623120705331));
#149962=CARTESIAN_POINT('Ctrl Pts',(-6.01036689279294,3.61014076962637,
46.0544571002351));
#149963=CARTESIAN_POINT('Ctrl Pts',(-5.92107654222664,3.75879640416695,
46.0465943332406));
#149964=CARTESIAN_POINT('Ctrl Pts',(-5.82634668332283,3.9040051701298,46.0387315662461));
#149965=CARTESIAN_POINT('Ctrl Pts',(-5.72650185387007,4.04534338222637,
46.0308687992516));
#149966=CARTESIAN_POINT('Ctrl Pts',(-5.65325785170397,4.14902603028829,
46.0251008438558));
#149967=CARTESIAN_POINT('Ctrl Pts',(-5.57726218538689,4.25062642081654,
46.0193328884601));
#149968=CARTESIAN_POINT('Ctrl Pts',(-5.49865615895209,4.34998931126483,
46.0135649330644));
#149969=CARTESIAN_POINT('Ctrl Pts',(-5.38447935815423,4.49431586565217,
46.0051868643068));
#149970=CARTESIAN_POINT('Ctrl Pts',(-5.26454100877773,4.63424025674379,
45.9968087955492));
#149971=CARTESIAN_POINT('Ctrl Pts',(-5.13920747913321,4.76929481673353,
45.9884307267917));
#149972=CARTESIAN_POINT('Ctrl Pts',(-5.01395965020853,4.90425702894497,
45.9800583868006));
#149973=CARTESIAN_POINT('Ctrl Pts',(-4.88332421893273,5.03435580870373,
45.9716860468095));
#149974=CARTESIAN_POINT('Ctrl Pts',(-4.74770737391496,5.15915702941609,
45.9633137068184));
#149975=CARTESIAN_POINT('Ctrl Pts',(-4.61216337295632,5.28389121548023,
45.9549458638737));
#149976=CARTESIAN_POINT('Ctrl Pts',(-4.47164353464269,5.40333329402616,
45.9465780209289));
#149977=CARTESIAN_POINT('Ctrl Pts',(-4.32659072151918,5.51708612321433,
45.9382101779841));
#149978=CARTESIAN_POINT('Ctrl Pts',(-4.18159457173026,5.63079451607285,
45.9298456038479));
#149979=CARTESIAN_POINT('Ctrl Pts',(-4.03206923655545,5.73881788889823,
45.9214810297117));
#149980=CARTESIAN_POINT('Ctrl Pts',(-3.87849080642846,5.8407992284404,45.9131164555755));
#149981=CARTESIAN_POINT('Ctrl Pts',(-3.72494989001698,5.94275565759017,
45.9047539246055));
#149982=CARTESIAN_POINT('Ctrl Pts',(-3.56735812681624,6.03867281536022,
45.8963913936355));
#149983=CARTESIAN_POINT('Ctrl Pts',(-3.4062211180323,6.12823663524596,45.8880288626655));
#149984=CARTESIAN_POINT('Ctrl Pts',(-3.2450712491949,6.21780760305832,45.879665664297));
#149985=CARTESIAN_POINT('Ctrl Pts',(-3.0803758538419,6.30102405501996,45.8713024659285));
#149986=CARTESIAN_POINT('Ctrl Pts',(-2.91266637200884,6.37761720142161,
45.8629392675601));
#149987=CARTESIAN_POINT('Ctrl Pts',(-2.74494545227208,6.45421557152931,
45.8545754988156));
#149988=CARTESIAN_POINT('Ctrl Pts',(-2.57421033517372,6.52418959855192,
45.8462117300712));
#149989=CARTESIAN_POINT('Ctrl Pts',(-2.40101389697498,6.58731803005085,
45.8378479613267));
#149990=CARTESIAN_POINT('Ctrl Pts',(-2.22778255561159,6.65045918341671,
45.8294825070857));
#149991=CARTESIAN_POINT('Ctrl Pts',(-2.05208921299349,6.70675187782401,
45.8211170528447));
#149992=CARTESIAN_POINT('Ctrl Pts',(-1.87450381991222,6.75602412604,45.8127515986037));
#149993=CARTESIAN_POINT('Ctrl Pts',(-1.69685895358428,6.80531287550376,
45.8043833427769));
#149994=CARTESIAN_POINT('Ctrl Pts',(-1.51732108997272,6.84757640266265,
45.7960150869501));
#149995=CARTESIAN_POINT('Ctrl Pts',(-1.33647275299985,6.88269330589334,
45.7876468311232));
#149996=CARTESIAN_POINT('Ctrl Pts',(-1.15545674383999,6.91784276749899,
45.7792708167304));
#149997=CARTESIAN_POINT('Ctrl Pts',(-0.973128156483563,6.94583230183678,
45.7708948023376));
#149998=CARTESIAN_POINT('Ctrl Pts',(-0.790078298962019,6.96659191025348,
45.7625187879448));
#149999=CARTESIAN_POINT('Ctrl Pts',(-0.60693867152268,6.98736169943933,
45.7541386658507));
#150000=CARTESIAN_POINT('Ctrl Pts',(-0.423077395749594,7.00089446147565,
45.7457585437567));
#150001=CARTESIAN_POINT('Ctrl Pts',(-0.239088889927075,7.00717225885117,
45.7373784216626));
#150002=CARTESIAN_POINT('Ctrl Pts',(-0.0548901544622398,7.01345722938727,
45.7289887242418));
#150003=CARTESIAN_POINT('Ctrl Pts',(0.129435772677918,7.01247066604149,
45.7205990268209));
#150004=CARTESIAN_POINT('Ctrl Pts',(0.313295138123823,7.00424676313792,
45.7122093294001));
#150005=CARTESIAN_POINT('Ctrl Pts',(0.430023579301856,6.99902558028435,
45.7068828870972));
#150006=CARTESIAN_POINT('Ctrl Pts',(0.546564033290414,6.99088828203294,
45.7015564447944));
#150007=CARTESIAN_POINT('Ctrl Pts',(0.662766037441756,6.97985442126938,
45.6962300024915));
#150008=CARTESIAN_POINT('Ctrl Pts',(0.845612827108903,6.96249236255977,
45.687848710942));
#150009=CARTESIAN_POINT('Ctrl Pts',(1.02799010320501,6.9379208979741,45.6794674193925));
#150010=CARTESIAN_POINT('Ctrl Pts',(1.20930600317479,6.90617155544122,45.671086127843));
#150011=CARTESIAN_POINT('Ctrl Pts',(1.39039211228032,6.87446245046535,45.6627154583307));
#150012=CARTESIAN_POINT('Ctrl Pts',(1.57041920585015,6.83559365275416,45.6543447888184));
#150013=CARTESIAN_POINT('Ctrl Pts',(1.74879955144228,6.7896484954212,45.6459741193061));
#150014=CARTESIAN_POINT('Ctrl Pts',(1.92697746686699,6.743755477722,45.6376129490243));
#150015=CARTESIAN_POINT('Ctrl Pts',(2.10351204360695,6.69080218713475,45.6292517787426));
#150016=CARTESIAN_POINT('Ctrl Pts',(2.27782432946017,6.63092323033674,45.6208906084608));
#150017=CARTESIAN_POINT('Ctrl Pts',(2.45191042672466,6.57112197280511,45.61254028768));
#150018=CARTESIAN_POINT('Ctrl Pts',(2.6237796764463,6.504413080099,45.6041899668992));
#150019=CARTESIAN_POINT('Ctrl Pts',(2.79286698831164,6.43098130522077,45.5958396461183));
#150020=CARTESIAN_POINT('Ctrl Pts',(2.96182419905083,6.35760603107286,45.5874957503384));
#150021=CARTESIAN_POINT('Ctrl Pts',(3.12800343832374,6.27751831316035,45.5791518545585));
#150022=CARTESIAN_POINT('Ctrl Pts',(3.29085726817442,6.19095186566683,45.5708079587786));
#150023=CARTESIAN_POINT('Ctrl Pts',(3.45358029544781,6.10445494748343,45.5624707647329));
#150024=CARTESIAN_POINT('Ctrl Pts',(3.6129829516199,6.01148983100343,45.5541335706871));
#150025=CARTESIAN_POINT('Ctrl Pts',(3.7685400521827,5.9123373074948,45.5457963766414));
#150026=CARTESIAN_POINT('Ctrl Pts',(3.81974961510443,5.87969619131885,45.5430517634959));
#150027=CARTESIAN_POINT('Ctrl Pts',(3.87054261038123,5.84638490046712,45.5403071503504));
#150028=CARTESIAN_POINT('Ctrl Pts',(3.92090088251406,5.81241454406002,45.537562537205));
#150029=CARTESIAN_POINT('Ctrl Pts',(4.07389262539419,5.70921036701297,45.5292242219516));
#150030=CARTESIAN_POINT('Ctrl Pts',(4.22274432084454,5.60000454975874,45.5208859066983));
#150031=CARTESIAN_POINT('Ctrl Pts',(4.36698754506551,5.48516602699888,45.5125475914449));
#150032=CARTESIAN_POINT('Ctrl Pts',(4.5113215240873,5.3702552502575,45.5042040298991));
#150033=CARTESIAN_POINT('Ctrl Pts',(4.65104099202757,5.24970490318,45.4958604683533));
#150034=CARTESIAN_POINT('Ctrl Pts',(4.78571191560507,5.12392310864787,45.4875169068074));
#150035=CARTESIAN_POINT('Ctrl Pts',(4.92048529777488,4.99804561843575,45.4791669974209));
#150036=CARTESIAN_POINT('Ctrl Pts',(5.0502022349229,4.86692896511709,45.4708170880344));
#150037=CARTESIAN_POINT('Ctrl Pts',(5.17446643729791,4.7310171899685,45.4624671786479));
#150038=CARTESIAN_POINT('Ctrl Pts',(5.29891702836845,4.59490155547835,45.4541047449085));
#150039=CARTESIAN_POINT('Ctrl Pts',(5.41789831963236,4.45397666852577,45.4457423111691));
#150040=CARTESIAN_POINT('Ctrl Pts',(5.53105416893855,4.30871980323246,45.4373798774297));
#150041=CARTESIAN_POINT('Ctrl Pts',(5.64430678273894,4.1633387224683,45.4290102926091));
#150042=CARTESIAN_POINT('Ctrl Pts',(5.75172382447618,4.01361853758819,45.4206407077884));
#150043=CARTESIAN_POINT('Ctrl Pts',(5.85299289451728,3.86006486204963,45.4122711229678));
#150044=CARTESIAN_POINT('Ctrl Pts',(5.95441816036588,3.7062743477573,45.4038886290323));
#150045=CARTESIAN_POINT('Ctrl Pts',(6.04967633645704,3.54863880731891,45.3955061350968));
#150046=CARTESIAN_POINT('Ctrl Pts',(6.13850062200587,3.38768898751547,45.3871236411613));
#150047=CARTESIAN_POINT('Ctrl Pts',(6.16756503448613,3.3350242019505,45.3843807847471));
#150048=CARTESIAN_POINT('Ctrl Pts',(6.19594096614935,3.28200472518559,45.3816379283329));
#150049=CARTESIAN_POINT('Ctrl Pts',(6.22362019657571,3.22864959561655,45.3788950719187));
#150050=CARTESIAN_POINT('Ctrl Pts',(6.31278769891644,3.0567682402662,45.370059072797));
#150051=CARTESIAN_POINT('Ctrl Pts',(6.39488058095618,2.88109530724048,45.3612230736754));
#150052=CARTESIAN_POINT('Ctrl Pts',(6.46959591630812,2.7022130267966,45.3523870745538));
#150053=CARTESIAN_POINT('Ctrl Pts',(6.50510935421322,2.61718731247782,45.348187177643));
#150054=CARTESIAN_POINT('Ctrl Pts',(6.53895666757272,2.53143690837865,45.3439872807322));
#150055=CARTESIAN_POINT('Ctrl Pts',(6.57110895151812,2.4450263208764,45.3397873838214));
#150056=CARTESIAN_POINT('Origin',(0.,0.,50.));
#150057=CARTESIAN_POINT('',(6.57110895151813,2.44502632087639,43.3397490455966));
#150058=CARTESIAN_POINT('',(6.57110895151816,2.4450263208763,43.8869849718596));
#150059=CARTESIAN_POINT('',(6.57110895151814,2.44502632087636,50.));
#150060=CARTESIAN_POINT('',(7.01124983644072,-0.00151443390808588,45.7735343569105));
#150061=CARTESIAN_POINT('Ctrl Pts',(6.57110895151816,2.4450263208763,43.8869849718596));
#150062=CARTESIAN_POINT('Ctrl Pts',(6.50404500432959,2.62526344140636,43.8957172526382));
#150063=CARTESIAN_POINT('Ctrl Pts',(6.42955170457269,2.80276609009301,43.9044495334167));
#150064=CARTESIAN_POINT('Ctrl Pts',(6.3478724394879,2.97693501012198,43.9131818141953));
#150065=CARTESIAN_POINT('Ctrl Pts',(6.26622358124146,3.1510390920774,43.9219108441972));
#150066=CARTESIAN_POINT('Ctrl Pts',(6.17739421514608,3.32181167559486,43.9306398741991));
#150067=CARTESIAN_POINT('Ctrl Pts',(6.08167515762305,3.48867508370307,43.9393689042009));
#150068=CARTESIAN_POINT('Ctrl Pts',(6.07063410843983,3.50792252662069,43.9403757846704));
#150069=CARTESIAN_POINT('Ctrl Pts',(6.05950144112564,3.52711798220248,43.9413826651398));
#150070=CARTESIAN_POINT('Ctrl Pts',(6.04827764177913,3.546260584116,43.9423895456092));
#150071=CARTESIAN_POINT('Ctrl Pts',(5.95881474222489,3.69884284430472,43.9504152099604));
#150072=CARTESIAN_POINT('Ctrl Pts',(5.86351692601779,3.84813525201835,43.9584408743116));
#150073=CARTESIAN_POINT('Ctrl Pts',(5.76266405141671,3.99366117654085,43.9664665386628));
#150074=CARTESIAN_POINT('Ctrl Pts',(5.66184318505012,4.13914091469596,43.9744896558645));
#150075=CARTESIAN_POINT('Ctrl Pts',(5.55547097888886,4.28085624863615,43.9825127730662));
#150076=CARTESIAN_POINT('Ctrl Pts',(5.44387112403516,4.41835871646883,43.9905358902679));
#150077=CARTESIAN_POINT('Ctrl Pts',(5.33228534290148,4.55584384403494,43.9985579956842));
#150078=CARTESIAN_POINT('Ctrl Pts',(5.21547345762989,4.68911687957163,44.0065801011005));
#150079=CARTESIAN_POINT('Ctrl Pts',(5.09379998788155,4.81776174649162,44.0146022065168));
#150080=CARTESIAN_POINT('Ctrl Pts',(4.97208130383797,4.94645441830289,44.0226272929761));
#150081=CARTESIAN_POINT('Ctrl Pts',(4.84549767628146,5.07051521716184,44.0306523794354));
#150082=CARTESIAN_POINT('Ctrl Pts',(4.71445140948555,5.18956399614647,44.0386774658947));
#150083=CARTESIAN_POINT('Ctrl Pts',(4.58337933377496,5.30863622119984,44.0467041328551));
#150084=CARTESIAN_POINT('Ctrl Pts',(4.44784314516642,5.4226942199669,44.0547307998155));
#150085=CARTESIAN_POINT('Ctrl Pts',(4.30827872167567,5.53139774549405,44.0627574667759));
#150086=CARTESIAN_POINT('Ctrl Pts',(4.16860225630352,5.64018853787052,44.0707905775193));
#150087=CARTESIAN_POINT('Ctrl Pts',(4.02489139208581,5.74361605384356,44.0788236882628));
#150088=CARTESIAN_POINT('Ctrl Pts',(3.87761201195225,5.84138268282978,44.0868567990063));
#150089=CARTESIAN_POINT('Ctrl Pts',(3.79082959056224,5.89899037228956,44.0915902029694));
#150090=CARTESIAN_POINT('Ctrl Pts',(3.70280870566545,5.95463343971279,44.0963236069325));
#150091=CARTESIAN_POINT('Ctrl Pts',(3.61364869604596,6.0082584551653,44.1010570108956));
#150092=CARTESIAN_POINT('Ctrl Pts',(3.42997638890585,6.11872760328026,44.1108079657267));
#150093=CARTESIAN_POINT('Ctrl Pts',(3.24136075414954,6.22069591698319,44.1205589205577));
#150094=CARTESIAN_POINT('Ctrl Pts',(3.04853359889174,6.31379992230734,44.1303098753887));
#150095=CARTESIAN_POINT('Ctrl Pts',(2.85542863918095,6.40703806178514,44.140074878338));
#150096=CARTESIAN_POINT('Ctrl Pts',(2.65810005696907,6.49138633085964,44.1498398812872));
#150097=CARTESIAN_POINT('Ctrl Pts',(2.4573027054613,6.5665280001103,44.1596048842364));
#150098=CARTESIAN_POINT('Ctrl Pts',(2.25684004256104,6.64154442338308,44.1693536108991));
#150099=CARTESIAN_POINT('Ctrl Pts',(2.05292020121408,6.7073849030508,44.1791023375617));
#150100=CARTESIAN_POINT('Ctrl Pts',(1.84631346506595,6.76378245889208,44.1888510642244));
#150101=CARTESIAN_POINT('Ctrl Pts',(1.64027378596704,6.8200252248548,44.1985730343336));
#150102=CARTESIAN_POINT('Ctrl Pts',(1.43156197258665,6.86687679600982,44.2082950044428));
#150103=CARTESIAN_POINT('Ctrl Pts',(1.22096058025326,6.90412064089031,44.218016974552));
#150104=CARTESIAN_POINT('Ctrl Pts',(1.01175268593837,6.94111805233811,44.2276746167576));
#150105=CARTESIAN_POINT('Ctrl Pts',(0.800680176714006,6.96863442466148,
44.2373322589631));
#150106=CARTESIAN_POINT('Ctrl Pts',(0.588527999355292,6.98650566137857,
44.2469899011686));
#150107=CARTESIAN_POINT('Ctrl Pts',(0.495279987078003,6.99436067055903,
44.2512347595065));
#150108=CARTESIAN_POINT('Ctrl Pts',(0.401823622799947,7.00035296964335,
44.2554796178443));
#150109=CARTESIAN_POINT('Ctrl Pts',(0.308226627566987,7.0044716366446,44.2597244761821));
#150110=CARTESIAN_POINT('Ctrl Pts',(0.135097350216412,7.01209006328105,
44.2675763228644));
#150111=CARTESIAN_POINT('Ctrl Pts',(-0.0384421541657765,7.01329092209141,
44.2754281695466));
#150112=CARTESIAN_POINT('Ctrl Pts',(-0.211858735308332,7.0080484044257,
44.2832800162288));
#150113=CARTESIAN_POINT('Ctrl Pts',(-0.385226136917442,7.0028073734954,
44.2911296361911));
#150114=CARTESIAN_POINT('Ctrl Pts',(-0.55847030371583,6.99112661239508,
44.2989792561534));
#150115=CARTESIAN_POINT('Ctrl Pts',(-0.731057755024403,6.9730324193509,
44.3068288761157));
#150116=CARTESIAN_POINT('Ctrl Pts',(-0.903631427442471,6.95493967089556,
44.3146778693867));
#150117=CARTESIAN_POINT('Ctrl Pts',(-1.07554810943842,6.93043455032811,
44.3225268626577));
#150118=CARTESIAN_POINT('Ctrl Pts',(-1.24627937678613,6.89959522562719,
44.3303758559287));
#150119=CARTESIAN_POINT('Ctrl Pts',(-1.41709708041024,6.86874028787288,
44.3382288229168));
#150120=CARTESIAN_POINT('Ctrl Pts',(-1.5867277943957,6.83154480648655,44.3460817899048));
#150121=CARTESIAN_POINT('Ctrl Pts',(-1.75465289030244,6.78813816867728,
44.3539347568929));
#150122=CARTESIAN_POINT('Ctrl Pts',(-1.92262063355348,6.74472050703731,
44.3617897182713));
#150123=CARTESIAN_POINT('Ctrl Pts',(-2.08888153018173,6.69508865550268,
44.3696446796497));
#150124=CARTESIAN_POINT('Ctrl Pts',(-2.25293268892498,6.63942172645128,
44.3774996410281));
#150125=CARTESIAN_POINT('Ctrl Pts',(-2.41714668220807,6.58369954330203,
44.3853623991147));
#150126=CARTESIAN_POINT('Ctrl Pts',(-2.57914620064869,6.52193045428565,
44.3932251572014));
#150127=CARTESIAN_POINT('Ctrl Pts',(-2.73844835592382,6.45434172975356,
44.401087915288));
#150128=CARTESIAN_POINT('Ctrl Pts',(-2.85531017612821,6.40475959220826,
44.4068559240149));
#150129=CARTESIAN_POINT('Ctrl Pts',(-2.97072084266621,6.35204663273512,
44.4126239327417));
#150130=CARTESIAN_POINT('Ctrl Pts',(-3.0844986649886,6.29630800931653,44.4183919414685));
#150131=CARTESIAN_POINT('Ctrl Pts',(-3.24976160263635,6.21534734001759,
44.426770007133));
#150132=CARTESIAN_POINT('Ctrl Pts',(-3.41194482915532,6.12782239026753,
44.4351480727975));
#150133=CARTESIAN_POINT('Ctrl Pts',(-3.57051360017444,6.03399197824039,
44.4435261384619));
#150134=CARTESIAN_POINT('Ctrl Pts',(-3.7289739436089,5.94022572641882,44.451898475297));
#150135=CARTESIAN_POINT('Ctrl Pts',(-3.88382447702945,5.84016277525746,
44.4602708121322));
#150136=CARTESIAN_POINT('Ctrl Pts',(-4.03455478636337,5.73410797232948,
44.4686431489673));
#150137=CARTESIAN_POINT('Ctrl Pts',(-4.18520413270094,5.62811013547991,
44.4770109887011));
#150138=CARTESIAN_POINT('Ctrl Pts',(-4.33173739947828,5.51612705289056,
44.4853788284348));
#150139=CARTESIAN_POINT('Ctrl Pts',(-4.4736725355593,5.39850725729645,44.4937466681686));
#150140=CARTESIAN_POINT('Ctrl Pts',(-4.61555222536714,5.28093340930558,
44.5021112390464));
#150141=CARTESIAN_POINT('Ctrl Pts',(-4.75283711370391,5.15772744875434,
44.5104758099241));
#150142=CARTESIAN_POINT('Ctrl Pts',(-4.88507731569834,5.02927889285825,
44.5188403808018));
#150143=CARTESIAN_POINT('Ctrl Pts',(-5.01728521550296,4.90086171297014,
44.5272029084737));
#150144=CARTESIAN_POINT('Ctrl Pts',(-5.14445065112782,4.76720472068888,
44.5355654361456));
#150145=CARTESIAN_POINT('Ctrl Pts',(-5.26615944653201,4.62873538303948,
44.5439279638174));
#150146=CARTESIAN_POINT('Ctrl Pts',(-5.38787795471531,4.49025499506224,
44.5522911588477));
#150147=CARTESIAN_POINT('Ctrl Pts',(-5.50413873117204,4.34696173733183,
44.5606543538779));
#150148=CARTESIAN_POINT('Ctrl Pts',(-5.61456636467825,4.19931793260807,
44.5690175489081));
#150149=CARTESIAN_POINT('Ctrl Pts',(-5.72500152916311,4.05166405882544,
44.5773813142942));
#150150=CARTESIAN_POINT('Ctrl Pts',(-5.82960256033757,3.89965930961281,
44.5857450796803));
#150151=CARTESIAN_POINT('Ctrl Pts',(-5.92803595478912,3.74379704060296,
44.5941088450663));
#150152=CARTESIAN_POINT('Ctrl Pts',(-6.02648918573965,3.58790336190987,
44.6024742959355));
#150153=CARTESIAN_POINT('Ctrl Pts',(-6.11877212601422,3.42815089131091,
44.6108397468047));
#150154=CARTESIAN_POINT('Ctrl Pts',(-6.20459579391003,3.26506012145167,
44.6192051976738));
#150155=CARTESIAN_POINT('Ctrl Pts',(-6.29044820404645,3.1019147326946,44.6275734501222));
#150156=CARTESIAN_POINT('Ctrl Pts',(-6.36983687526782,2.93542910621001,
44.6359417025705));
#150157=CARTESIAN_POINT('Ctrl Pts',(-6.44251959285939,2.76614675281753,
44.6443099550189));
#150158=CARTESIAN_POINT('Ctrl Pts',(-6.51526969783219,2.59670745022359,
44.6526859660464));
#150159=CARTESIAN_POINT('Ctrl Pts',(-6.58130129513043,2.42446654162041,
44.6610619770739));
#150160=CARTESIAN_POINT('Ctrl Pts',(-6.64042053958726,2.24998702661318,
44.6694379881014));
#150161=CARTESIAN_POINT('Ctrl Pts',(-6.6995687769112,2.07542194452135,44.6778181068366));
#150162=CARTESIAN_POINT('Ctrl Pts',(-6.75179780201015,1.89861638000929,
44.6861982255718));
#150163=CARTESIAN_POINT('Ctrl Pts',(-6.7969639861086,1.7201474163695,44.694578344307));
#150164=CARTESIAN_POINT('Ctrl Pts',(-6.84218177840511,1.54147452889142,
44.7029680384101));
#150165=CARTESIAN_POINT('Ctrl Pts',(-6.88032052940223,1.36113476478182,
44.7113577325132));
#150166=CARTESIAN_POINT('Ctrl Pts',(-6.9112876966623,1.17971561677563,44.7197474266162));
#150167=CARTESIAN_POINT('Ctrl Pts',(-6.93094825294038,1.06453551846891,
44.7250739084246));
#150168=CARTESIAN_POINT('Ctrl Pts',(-6.94771914402347,0.948920498281068,
44.7304003902331));
#150169=CARTESIAN_POINT('Ctrl Pts',(-6.96158755844055,0.833021745613987,
44.7357268720415));
#150170=CARTESIAN_POINT('Ctrl Pts',(-6.98340973414702,0.650653172769248,
44.744108177822));
#150171=CARTESIAN_POINT('Ctrl Pts',(-6.99808696749465,0.467214027019617,
44.7524894836025));
#150172=CARTESIAN_POINT('Ctrl Pts',(-7.00552451169838,0.283289390011714,
44.7608707893831));
#150173=CARTESIAN_POINT('Ctrl Pts',(-7.0129526298601,0.0995978516326951,
44.7692414730364));
#150174=CARTESIAN_POINT('Ctrl Pts',(-7.01315933114402,-0.0845776270624559,
44.7776121566898));
#150175=CARTESIAN_POINT('Ctrl Pts',(-7.00610137100075,-0.268645010676497,
44.7859828403431));
#150176=CARTESIAN_POINT('Ctrl Pts',(-6.99905142048172,-0.452503508076084,
44.7943440246469));
#150177=CARTESIAN_POINT('Ctrl Pts',(-6.98475325260364,-0.636253829470594,
44.8027052089507));
#150178=CARTESIAN_POINT('Ctrl Pts',(-6.96321559200029,-0.819301642756818,
44.8110663932545));
#150179=CARTESIAN_POINT('Ctrl Pts',(-6.94170587934826,-1.00211192739643,
44.8194167278204));
#150180=CARTESIAN_POINT('Ctrl Pts',(-6.91297544979655,-1.18422119833501,
44.8277670623864));
#150181=CARTESIAN_POINT('Ctrl Pts',(-6.87708497359292,-1.36503803188133,
44.8361173969523));
#150182=CARTESIAN_POINT('Ctrl Pts',(-6.84122211328002,-1.54571573609741,
44.8444613063617));
#150183=CARTESIAN_POINT('Ctrl Pts',(-6.79821024884859,-1.72510266469258,
44.8528052157711));
#150184=CARTESIAN_POINT('Ctrl Pts',(-6.74816164210157,-1.90261425795381,
44.8611491251805));
#150185=CARTESIAN_POINT('Ctrl Pts',(-6.69815323546132,-2.07998327012302,
44.8694863325842));
#150186=CARTESIAN_POINT('Ctrl Pts',(-6.64111944739184,-2.25547963663527,
44.8778235399879));
#150187=CARTESIAN_POINT('Ctrl Pts',(-6.57722326611108,-2.4285305578121,
44.8861607473916));
#150188=CARTESIAN_POINT('Ctrl Pts',(-6.55618924637733,-2.48549728756052,
44.8889052773703));
#150189=CARTESIAN_POINT('Ctrl Pts',(-6.5344119802445,-2.54219911730051,
44.8916498073491));
#150190=CARTESIAN_POINT('Ctrl Pts',(-6.51189847181606,-2.59861594993559,
44.8943943373278));
#150191=CARTESIAN_POINT('Ctrl Pts',(-6.44349898993794,-2.77001891601304,
44.9027326391586));
#150192=CARTESIAN_POINT('Ctrl Pts',(-6.36835622157593,-2.93864926190625,
44.9110709409894));
#150193=CARTESIAN_POINT('Ctrl Pts',(-6.28673133156438,-3.10397096107982,
44.9194092428202));
#150194=CARTESIAN_POINT('Ctrl Pts',(-6.20505508710549,-3.26939667269976,
44.9277527907086));
#150195=CARTESIAN_POINT('Ctrl Pts',(-6.11688873149893,-3.4315092917151,
44.9360963385971));
#150196=CARTESIAN_POINT('Ctrl Pts',(-6.02253902143441,-3.58979808593741,
44.9444398864856));
#150197=CARTESIAN_POINT('Ctrl Pts',(-5.92811753164527,-3.74820730369947,
44.9527897820095));
#150198=CARTESIAN_POINT('Ctrl Pts',(-5.82750347163371,-3.90278661282742,
44.9611396775335));
#150199=CARTESIAN_POINT('Ctrl Pts',(-5.72104670588304,-4.05305454584623,
44.9694895730575));
#150200=CARTESIAN_POINT('Ctrl Pts',(-5.61443026401084,-4.20354786802249,
44.9778519927167));
#150201=CARTESIAN_POINT('Ctrl Pts',(-5.50195379361739,-4.34971662400249,
44.9862144123759));
#150202=CARTESIAN_POINT('Ctrl Pts',(-5.3840081525361,-4.49111153011421,
44.9945768320351));
#150203=CARTESIAN_POINT('Ctrl Pts',(-5.26596165255812,-4.63262734730071,
45.0029464026532));
#150204=CARTESIAN_POINT('Ctrl Pts',(-5.14243686948065,-4.76936092689429,
45.0113159732712));
#150205=CARTESIAN_POINT('Ctrl Pts',(-5.01386163497974,-4.90089972023284,
45.0196855438892));
#150206=CARTESIAN_POINT('Ctrl Pts',(-4.88508808900859,-5.03264139596629,
45.0280680235395));
#150207=CARTESIAN_POINT('Ctrl Pts',(-4.75124876310388,-5.15917204978774,
45.0364505031899));
#150208=CARTESIAN_POINT('Ctrl Pts',(-4.61280572352955,-5.28011836225979,
45.0448329828402));
#150209=CARTESIAN_POINT('Ctrl Pts',(-4.56750398032389,-5.31969477437937,
45.0475759227649));
#150210=CARTESIAN_POINT('Ctrl Pts',(-4.52170953464011,-5.35867358369052,
45.0503188626896));
#150211=CARTESIAN_POINT('Ctrl Pts',(-4.47543924925462,-5.39704271696373,
45.0530618026143));
#150212=CARTESIAN_POINT('Ctrl Pts',(-4.33391186585346,-5.51440276759424,
45.0614516603196));
#150213=CARTESIAN_POINT('Ctrl Pts',(-4.18764471001657,-5.62629262909133,
45.069841518025));
#150214=CARTESIAN_POINT('Ctrl Pts',(-4.03708740208148,-5.7323251713816,
45.0782313757303));
#150215=CARTESIAN_POINT('Ctrl Pts',(-3.88666902607069,-5.83825986850352,
45.0866134914064));
#150216=CARTESIAN_POINT('Ctrl Pts',(-3.7319686574599,-5.938347832997,45.0949956070826));
#150217=CARTESIAN_POINT('Ctrl Pts',(-3.57346855336625,-6.03224245704718,
45.1033777227587));
#150218=CARTESIAN_POINT('Ctrl Pts',(-3.41509141161372,-6.12606423885628,
45.1117533356974));
#150219=CARTESIAN_POINT('Ctrl Pts',(-3.25292069317565,-6.21370209241489,
45.120128948636));
#150220=CARTESIAN_POINT('Ctrl Pts',(-3.08746754778098,-6.29485271502831,
45.1285045615747));
#150221=CARTESIAN_POINT('Ctrl Pts',(-2.92211847483946,-6.37595229271086,
45.13687490613));
#150222=CARTESIAN_POINT('Ctrl Pts',(-2.75349138613453,-6.45057263134097,
45.1452452506854));
#150223=CARTESIAN_POINT('Ctrl Pts',(-2.58212234248166,-6.51845616468785,
45.1536155952408));
#150224=CARTESIAN_POINT('Ctrl Pts',(-2.41083597181675,-6.5863069492114,
45.1619819017192));
#150225=CARTESIAN_POINT('Ctrl Pts',(-2.23681058913936,-6.64742728865912,
45.1703482081975));
#150226=CARTESIAN_POINT('Ctrl Pts',(-2.06060298057893,-6.70160741307108,
45.1787145146759));
#150227=CARTESIAN_POINT('Ctrl Pts',(-1.88444465281964,-6.75577238467574,
45.1870784813104));
#150228=CARTESIAN_POINT('Ctrl Pts',(-1.70610562957134,-6.80300091368879,
45.195442447945));
#150229=CARTESIAN_POINT('Ctrl Pts',(-1.52615916427333,-6.84313267208846,
45.2038064145795));
#150230=CARTESIAN_POINT('Ctrl Pts',(-1.3462403901275,-6.88325825479234,
45.2121690941209));
#150231=CARTESIAN_POINT('Ctrl Pts',(-1.16471498780618,-6.91628917277313,
45.2205317736622));
#150232=CARTESIAN_POINT('Ctrl Pts',(-0.982168157556564,-6.94211583544829,
45.2288944532035));
#150233=CARTESIAN_POINT('Ctrl Pts',(-0.799625086118805,-6.96794196632805,
45.2372569605494));
#150234=CARTESIAN_POINT('Ctrl Pts',(-0.616060954154885,-6.9865640920567,
45.2456194678953));
#150235=CARTESIAN_POINT('Ctrl Pts',(-0.432068301071265,-6.99792423120667,
45.2539819752411));
#150236=CARTESIAN_POINT('Ctrl Pts',(-0.248054911779567,-7.00928565065889,
45.2623454250523));
#150237=CARTESIAN_POINT('Ctrl Pts',(-0.0636132331261454,-7.01338343209129,
45.2707088748634));
#150238=CARTESIAN_POINT('Ctrl Pts',(0.120661524372453,-7.01021164866198,
45.2790723246746));
#150239=CARTESIAN_POINT('Ctrl Pts',(0.305044786671953,-7.00703799762078,
45.2874406990586));
#150240=CARTESIAN_POINT('Ctrl Pts',(0.48926060244824,-6.99658623301968,
45.2958090734425));
#150241=CARTESIAN_POINT('Ctrl Pts',(0.672715169568648,-6.97890255435138,
45.3041774478265));
#150242=CARTESIAN_POINT('Ctrl Pts',(0.856224703716667,-6.96121357726359,
45.3125483295597));
#150243=CARTESIAN_POINT('Ctrl Pts',(1.03897220771171,-6.93628840228828,
45.3209192112928));
#150244=CARTESIAN_POINT('Ctrl Pts',(1.22037071740043,-6.90422492931767,
45.329290093026));
#150245=CARTESIAN_POINT('Ctrl Pts',(1.40192292243896,-6.87213428960405,
45.3376680672408));
#150246=CARTESIAN_POINT('Ctrl Pts',(1.58212352634415,-6.83289332918547,
45.3460460414556));
#150247=CARTESIAN_POINT('Ctrl Pts',(1.76039630212137,-6.78665097245891,
45.3544240156704));
#150248=CARTESIAN_POINT('Ctrl Pts',(1.87368942905185,-6.75726375297266,
45.3597482548427));
#150249=CARTESIAN_POINT('Ctrl Pts',(1.98620423357189,-6.72504992663875,
45.3650724940149));
#150250=CARTESIAN_POINT('Ctrl Pts',(2.09779627068701,-6.6900580990894,45.3703967331871));
#150251=CARTESIAN_POINT('Ctrl Pts',(2.26259546139358,-6.63838214612219,
45.3782595729506));
#150252=CARTESIAN_POINT('Ctrl Pts',(2.42572392454344,-6.58053746583258,
45.3861224127141));
#150253=CARTESIAN_POINT('Ctrl Pts',(2.58666585737656,-6.51665453317747,
45.3939852524775));
#150254=CARTESIAN_POINT('Ctrl Pts',(2.74748412769345,-6.45282068607797,
45.4018420506921));
#150255=CARTESIAN_POINT('Ctrl Pts',(2.90611885664721,-6.38295795286989,
45.4096988489067));
#150256=CARTESIAN_POINT('Ctrl Pts',(3.06206853905006,-6.30724684982757,
45.4175556471213));
#150257=CARTESIAN_POINT('Ctrl Pts',(3.21793027323985,-6.231578444251,45.425408014475));
#150258=CARTESIAN_POINT('Ctrl Pts',(3.37110963112841,-6.15006839571762,
45.4332603818286));
#150259=CARTESIAN_POINT('Ctrl Pts',(3.52112451134335,-6.06294554965794,
45.4411127491822));
#150260=CARTESIAN_POINT('Ctrl Pts',(3.67110397093754,-5.97584327452619,
45.4489632624816));
#150261=CARTESIAN_POINT('Ctrl Pts',(3.81792010630897,-5.88313102351259,
45.4568137757809));
#150262=CARTESIAN_POINT('Ctrl Pts',(3.96111494994963,-5.78508382962473,
45.4646642890803));
#150263=CARTESIAN_POINT('Ctrl Pts',(4.10428675798224,-5.68705240848869,
45.4725135394756));
#150264=CARTESIAN_POINT('Ctrl Pts',(4.24383812087141,-5.583687970988,45.480362789871));
#150265=CARTESIAN_POINT('Ctrl Pts',(4.3793400275334,-5.4753088940939,45.4882120402663));
#150266=CARTESIAN_POINT('Ctrl Pts',(4.51488758676616,-5.36689330270639,
45.4960639351887));
#150267=CARTESIAN_POINT('Ctrl Pts',(4.64638266641554,-5.25345993575891,
45.503915830111));
#150268=CARTESIAN_POINT('Ctrl Pts',(4.77342918296909,-5.13536760102713,
45.5117677250334));
#150269=CARTESIAN_POINT('Ctrl Pts',(4.86671692734786,-5.04865473526423,
45.5175332161801));
#150270=CARTESIAN_POINT('Ctrl Pts',(4.9576068291167,-4.95943075883898,45.5232987073268));
#150271=CARTESIAN_POINT('Ctrl Pts',(5.04595485518052,-4.86785026084207,
45.5290641984735));
#150272=CARTESIAN_POINT('Ctrl Pts',(5.19390725399777,-4.71448458910952,
45.5387194028229));
#150273=CARTESIAN_POINT('Ctrl Pts',(5.33465509669178,-4.55458791352578,
45.5483746071723));
#150274=CARTESIAN_POINT('Ctrl Pts',(5.46772197842277,-4.38880882805035,
45.5580298115217));
#150275=CARTESIAN_POINT('Ctrl Pts',(5.60152591377924,-4.22211149699502,
45.5677384957699));
#150276=CARTESIAN_POINT('Ctrl Pts',(5.72756357639558,-4.04946648164349,
45.5774471800181));
#150277=CARTESIAN_POINT('Ctrl Pts',(5.84539772643407,-3.87155679053007,
45.5871558642664));
#150278=CARTESIAN_POINT('Ctrl Pts',(5.96379884216781,-3.69279107684864,
45.5969112623994));
#150279=CARTESIAN_POINT('Ctrl Pts',(6.07391730816847,-3.50870995229964,
45.6066666605325));
#150280=CARTESIAN_POINT('Ctrl Pts',(6.17535690736826,-3.32002916088386,
45.6164220586655));
#150281=CARTESIAN_POINT('Ctrl Pts',(6.27689695335583,-3.13116153533657,
45.6261871167185));
#150282=CARTESIAN_POINT('Ctrl Pts',(6.36974093440355,-2.93768517167746,
45.6359521747715));
#150283=CARTESIAN_POINT('Ctrl Pts',(6.45353879309377,-2.74034005344844,
45.6457172328245));
#150284=CARTESIAN_POINT('Ctrl Pts',(6.53722245020253,-2.54326388152601,
45.6554689828396));
#150285=CARTESIAN_POINT('Ctrl Pts',(6.61188460991109,-2.34232952769541,
45.6652207328548));
#150286=CARTESIAN_POINT('Ctrl Pts',(6.67722392304667,-2.13829540615726,
45.67497248287));
#150287=CARTESIAN_POINT('Ctrl Pts',(6.70572055576135,-2.04930938619912,
45.6792255431666));
#150288=CARTESIAN_POINT('Ctrl Pts',(6.73244447982265,-1.95973402571245,
45.6834786034633));
#150289=CARTESIAN_POINT('Ctrl Pts',(6.75737353878295,-1.86963349880557,
45.6877316637599));
#150290=CARTESIAN_POINT('Ctrl Pts',(6.80473961416133,-1.69843937728265,
45.6958126256174));
#150291=CARTESIAN_POINT('Ctrl Pts',(6.84564464248862,-1.52526782050514,
45.7038935874748));
#150292=CARTESIAN_POINT('Ctrl Pts',(6.87992489828093,-1.3506516784553,45.7119745493323));
#150293=CARTESIAN_POINT('Ctrl Pts',(6.91418286331631,-1.1761490806568,45.7200502565394));
#150294=CARTESIAN_POINT('Ctrl Pts',(6.94182456104688,-1.0002041206424,45.7281259637466));
#150295=CARTESIAN_POINT('Ctrl Pts',(6.9627364815039,-0.823363377637502,
45.7362016709537));
#150296=CARTESIAN_POINT('Ctrl Pts',(6.98363769465593,-0.646613180490235,
45.7442732432436));
#150297=CARTESIAN_POINT('Ctrl Pts',(6.99781595120447,-0.46896847219117,
45.7523448155335));
#150298=CARTESIAN_POINT('Ctrl Pts',(7.0052091033809,-0.290984502008834,
45.7604163878234));
#150299=CARTESIAN_POINT('Ctrl Pts',(7.00921423555851,-0.19456428650892,
45.7647890441858));
#150300=CARTESIAN_POINT('Ctrl Pts',(7.01122898586229,-0.0980446382295471,
45.7691617005482));
#150301=CARTESIAN_POINT('Ctrl Pts',(7.01124983644072,-0.00151443390808588,
45.7735343569105));
#150302=CARTESIAN_POINT('Ctrl Pts',(7.01125,3.72163509519775E-12,45.7735343569105));
#150303=CARTESIAN_POINT('Ctrl Pts',(7.0112499999999,0.191008754744202,45.7822061308426));
#150304=CARTESIAN_POINT('Ctrl Pts',(7.00344012880995,0.382017367487347,
45.7908779047747));
#150305=CARTESIAN_POINT('Ctrl Pts',(6.98784644419141,0.572388534914368,
45.7995496787069));
#150306=CARTESIAN_POINT('Ctrl Pts',(6.97225169663157,0.762772678965089,
45.8082220437492));
#150307=CARTESIAN_POINT('Ctrl Pts',(6.94887209704267,0.952519007631466,
45.8168944087916));
#150308=CARTESIAN_POINT('Ctrl Pts',(6.91778566246033,1.14099434300015,45.8255667738339));
#150309=CARTESIAN_POINT('Ctrl Pts',(6.88670108297123,1.32945843104102,45.83423862135));
#150310=CARTESIAN_POINT('Ctrl Pts',(6.84791063501084,1.51665139731204,45.8429104688662));
#150311=CARTESIAN_POINT('Ctrl Pts',(6.80154374572903,1.70194865887145,45.8515823163823));
#150312=CARTESIAN_POINT('Ctrl Pts',(6.75517597619824,1.88724943819381,45.8602543285285));
#150313=CARTESIAN_POINT('Ctrl Pts',(6.70123154646052,2.07065416525576,45.8689263406747));
#150314=CARTESIAN_POINT('Ctrl Pts',(6.63989045285493,2.25155087363932,45.8775983528209));
#150315=CARTESIAN_POINT('Ctrl Pts',(6.61790934153613,2.31637382429861,45.880705901988));
#150316=CARTESIAN_POINT('Ctrl Pts',(6.59497889661499,2.38087486019109,45.8838134511551));
#150317=CARTESIAN_POINT('Ctrl Pts',(6.57110895151812,2.4450263208764,45.8869210003222));
#150318=CARTESIAN_POINT('',(7.01124961585759,0.00232091291924789,45.2264650997577));
#150319=CARTESIAN_POINT('Ctrl Pts',(6.57110895151812,2.4450263208764,45.3397873838214));
#150320=CARTESIAN_POINT('Ctrl Pts',(6.63862499196149,2.26357418110171,45.3309680909161));
#150321=CARTESIAN_POINT('Ctrl Pts',(6.69866370151301,2.07920961773414,45.3221487980108));
#150322=CARTESIAN_POINT('Ctrl Pts',(6.75099215188743,1.89254630792865,45.3133295051056));
#150323=CARTESIAN_POINT('Ctrl Pts',(6.80321535316924,1.70625843717859,45.3045279505925));
#150324=CARTESIAN_POINT('Ctrl Pts',(6.84775917915664,1.51768129892919,45.2957263960794));
#150325=CARTESIAN_POINT('Ctrl Pts',(6.88444035403814,1.32744400039749,45.2869248415663));
#150326=CARTESIAN_POINT('Ctrl Pts',(6.92107263670544,1.13746026851895,45.2781350186155));
#150327=CARTESIAN_POINT('Ctrl Pts',(6.94986312529546,0.945821045319097,
45.2693451956647));
#150328=CARTESIAN_POINT('Ctrl Pts',(6.97067887401658,0.753168372835053,
45.260555372714));
#150329=CARTESIAN_POINT('Ctrl Pts',(6.99145429853821,0.560888906470144,
45.2517825773791));
#150330=CARTESIAN_POINT('Ctrl Pts',(7.00428578375525,0.367600166895988,
45.2430097820442));
#150331=CARTESIAN_POINT('Ctrl Pts',(7.00909175428748,0.173952126975464,
45.2342369867093));
#150332=CARTESIAN_POINT('Ctrl Pts',(7.0105108705063,0.116771361435778,45.2316465388361));
#150333=CARTESIAN_POINT('Ctrl Pts',(7.01123057041653,0.0595593314933894,
45.2290560909628));
#150334=CARTESIAN_POINT('Ctrl Pts',(7.01124961187403,0.00233291583925055,
45.2264656430896));
#150335=CARTESIAN_POINT('Ctrl Pts',(7.01124961585759,0.00232091291924789,
45.2264650997577));
#150336=CARTESIAN_POINT('Ctrl Pts',(7.01131373062021,-0.191363477836033,
45.2176976568821));
#150337=CARTESIAN_POINT('Ctrl Pts',(7.00334774553214,-0.384934212827022,
45.2089302140066));
#150338=CARTESIAN_POINT('Ctrl Pts',(6.98740619787143,-0.577737992906812,
45.200162771131));
#150339=CARTESIAN_POINT('Ctrl Pts',(6.97144758934037,-0.770748114325792,
45.1913859452138));
#150340=CARTESIAN_POINT('Ctrl Pts',(6.94749639030405,-0.962989378600591,
45.1826091192966));
#150341=CARTESIAN_POINT('Ctrl Pts',(6.9156588509455,-1.15381507176808,45.1738322933794));
#150342=CARTESIAN_POINT('Ctrl Pts',(6.88378958982525,-1.34483089668847,
45.1650467225533));
#150343=CARTESIAN_POINT('Ctrl Pts',(6.84401833625513,-1.53442807346663,
45.1562611517272));
#150344=CARTESIAN_POINT('Ctrl Pts',(6.79650234356762,-1.72197051553732,
45.1474755809011));
#150345=CARTESIAN_POINT('Ctrl Pts',(6.74891995344015,-1.90977502385842,
45.1386777333787));
#150346=CARTESIAN_POINT('Ctrl Pts',(6.69357125003739,-2.0955188007609,45.1298798858563));
#150347=CARTESIAN_POINT('Ctrl Pts',(6.63066377754691,-2.27857947669757,
45.1210820383339));
#150348=CARTESIAN_POINT('Ctrl Pts',(6.56771463172738,-2.46176142197604,
45.1122783626391));
#150349=CARTESIAN_POINT('Ctrl Pts',(6.49719680749287,-2.64225646939765,
45.1034746869443));
#150350=CARTESIAN_POINT('Ctrl Pts',(6.41936645607332,-2.81946109480885,
45.0946710112495));
#150351=CARTESIAN_POINT('Ctrl Pts',(6.34146504499815,-2.99682750928338,
45.0858592977372));
#150352=CARTESIAN_POINT('Ctrl Pts',(6.25623787113032,-3.17089725727878,
45.0770475842249));
#150353=CARTESIAN_POINT('Ctrl Pts',(6.16398831554795,-3.34108883573729,
45.0682358707126));
#150354=CARTESIAN_POINT('Ctrl Pts',(6.14069231428679,-3.38406772275066,
45.0660106275903));
#150355=CARTESIAN_POINT('Ctrl Pts',(6.11694870338084,-3.42679941624926,
45.0637853844679));
#150356=CARTESIAN_POINT('Ctrl Pts',(6.0927628222351,-3.46927481680103,45.0615601413456));
#150357=CARTESIAN_POINT('Ctrl Pts',(6.0073027253985,-3.61936039038229,45.0536973104828));
#150358=CARTESIAN_POINT('Ctrl Pts',(5.91616874435837,-3.7665046418464,45.04583447962));
#150359=CARTESIAN_POINT('Ctrl Pts',(5.81959780561077,-3.91023118797729,
45.0379716487571));
#150360=CARTESIAN_POINT('Ctrl Pts',(5.72310106890137,-4.05384729920091,
45.0301148594434));
#150361=CARTESIAN_POINT('Ctrl Pts',(5.62117589347774,-4.19405061295756,
45.0222580701298));
#150362=CARTESIAN_POINT('Ctrl Pts',(5.51410507512597,-4.33038933387866,
45.0144012808161));
#150363=CARTESIAN_POINT('Ctrl Pts',(5.40709463966623,-4.46665116619097,
45.0065489223611));
#150364=CARTESIAN_POINT('Ctrl Pts',(5.29494456857491,-4.59905244216715,
44.9986965639061));
#150365=CARTESIAN_POINT('Ctrl Pts',(5.1779807704992,-4.72717058110245,44.990844205451));
#150366=CARTESIAN_POINT('Ctrl Pts',(5.06104458896047,-4.8552584698289,44.9829937010308));
#150367=CARTESIAN_POINT('Ctrl Pts',(4.93929719314165,-4.97906494726934,
44.9751431966105));
#150368=CARTESIAN_POINT('Ctrl Pts',(4.81310450828359,-5.09820081546816,
44.9672926921903));
#150369=CARTESIAN_POINT('Ctrl Pts',(4.68693212386762,-5.2173175184452,44.9594434506698));
#150370=CARTESIAN_POINT('Ctrl Pts',(4.55631615347341,-5.33176484818011,
44.9515942091492));
#150371=CARTESIAN_POINT('Ctrl Pts',(4.42165873698109,-5.44119109903143,
44.9437449676287));
#150372=CARTESIAN_POINT('Ctrl Pts',(4.28695595177435,-5.55065421772452,
44.9358930815454));
#150373=CARTESIAN_POINT('Ctrl Pts',(4.1482092970229,-5.6550926376447,44.9280411954621));
#150374=CARTESIAN_POINT('Ctrl Pts',(4.00585343795195,-5.75419540823464,
44.9201893093787));
#150375=CARTESIAN_POINT('Ctrl Pts',(3.90132326226839,-5.82696536718189,
44.914423764939));
#150376=CARTESIAN_POINT('Ctrl Pts',(3.7948477706504,-5.89685930138269,44.9086582204992));
#150377=CARTESIAN_POINT('Ctrl Pts',(3.6866085941152,-5.9637692474052,44.9028926760594));
#150378=CARTESIAN_POINT('Ctrl Pts',(3.50534516918806,-6.07582041377551,
44.8932373704189));
#150379=CARTESIAN_POINT('Ctrl Pts',(3.31922767169188,-6.17944533608273,
44.8835820647784));
#150380=CARTESIAN_POINT('Ctrl Pts',(3.12899101640001,-6.27431604095523,
44.8739267591378));
#150381=CARTESIAN_POINT('Ctrl Pts',(2.93770048295348,-6.36971231311773,
44.8642179647747));
#150382=CARTESIAN_POINT('Ctrl Pts',(2.74224509309065,-6.45625713339368,
44.8545091704115));
#150383=CARTESIAN_POINT('Ctrl Pts',(2.54338508578354,-6.53366810206287,
44.8448003760484));
#150384=CARTESIAN_POINT('Ctrl Pts',(2.34356814478508,-6.61145157984037,
44.8350448620227));
#150385=CARTESIAN_POINT('Ctrl Pts',(2.14031378982544,-6.68001309520664,
44.825289347997));
#150386=CARTESIAN_POINT('Ctrl Pts',(1.93440554885227,-6.73911728159331,
44.8155338339714));
#150387=CARTESIAN_POINT('Ctrl Pts',(1.72829342657662,-6.79827999035113,
44.8057686604639));
#150388=CARTESIAN_POINT('Ctrl Pts',(1.51952220209997,-6.84796663969157,
44.7960034869565));
#150389=CARTESIAN_POINT('Ctrl Pts',(1.30888929894411,-6.88799211422383,
44.786238313449));
#150390=CARTESIAN_POINT('Ctrl Pts',(1.09854358991336,-6.92796301475094,
44.7764864545777));
#150391=CARTESIAN_POINT('Ctrl Pts',(0.886341312769191,-6.9582990611913,
44.7667345957063));
#150392=CARTESIAN_POINT('Ctrl Pts',(0.673087568189201,-6.97886664781963,
44.756982736835));
#150393=CARTESIAN_POINT('Ctrl Pts',(0.580093666882398,-6.98783558820002,
44.7527302281476));
#150394=CARTESIAN_POINT('Ctrl Pts',(0.486899957340695,-6.99494762616512,
44.7484777194602));
#150395=CARTESIAN_POINT('Ctrl Pts',(0.393573826530796,-7.00019472626083,
44.7442252107729));
#150396=CARTESIAN_POINT('Ctrl Pts',(0.217279532242484,-7.01010656767551,
44.7361921656708));
#150397=CARTESIAN_POINT('Ctrl Pts',(0.0404264676274792,-7.01336469367874,
44.7281591205688));
#150398=CARTESIAN_POINT('Ctrl Pts',(-0.136435664693323,-7.0099223870097,
44.7201260754668));
#150399=CARTESIAN_POINT('Ctrl Pts',(-0.313184103180249,-7.00648229318881,
44.7120981943175));
#150400=CARTESIAN_POINT('Ctrl Pts',(-0.489941232798838,-6.99635034758006,
44.7040703131682));
#150401=CARTESIAN_POINT('Ctrl Pts',(-0.666154661791966,-6.97953182735582,
44.6960424320189));
#150402=CARTESIAN_POINT('Ctrl Pts',(-0.842288528648519,-6.96272090086272,
44.6880181755388));
#150403=CARTESIAN_POINT('Ctrl Pts',(-1.01787881951728,-6.93922944579692,
44.6799939190586));
#150404=CARTESIAN_POINT('Ctrl Pts',(-1.19237562897843,-6.90911477122202,
44.6719696625785));
#150405=CARTESIAN_POINT('Ctrl Pts',(-1.36685133997652,-6.87900373782171,
44.6639463763136));
#150406=CARTESIAN_POINT('Ctrl Pts',(-1.54023347058308,-6.84227113470735,
44.6559230900488));
#150407=CARTESIAN_POINT('Ctrl Pts',(-1.71197952886332,-6.79902586075777,
44.647899803784));
#150408=CARTESIAN_POINT('Ctrl Pts',(-1.88371151406891,-6.75578413037696,
44.6398771749567));
#150409=CARTESIAN_POINT('Ctrl Pts',(-2.05380733942037,-6.70603088557465,
44.6318545461294));
#150410=CARTESIAN_POINT('Ctrl Pts',(-2.22173725671783,-6.6499255728626,
44.6238319173021));
#150411=CARTESIAN_POINT('Ctrl Pts',(-2.38973030372378,-6.59379916854226,
44.6158062725369));
#150412=CARTESIAN_POINT('Ctrl Pts',(-2.55555546915972,-6.53131604511736,
44.6077806277716));
#150413=CARTESIAN_POINT('Ctrl Pts',(-2.71870028816019,-6.46268483725284,
44.5997549830063));
#150414=CARTESIAN_POINT('Ctrl Pts',(-2.81490048196455,-6.42221566674503,
44.5950225704997));
#150415=CARTESIAN_POINT('Ctrl Pts',(-2.91016908229907,-6.37960972293838,
44.5902901579931));
#150416=CARTESIAN_POINT('Ctrl Pts',(-3.00440465758325,-6.33491745928801,
44.5855577454865));
#150417=CARTESIAN_POINT('Ctrl Pts',(-3.1782443670222,-6.25247205473968,
44.5768276962178));
#150418=CARTESIAN_POINT('Ctrl Pts',(-3.3486543913784,-6.16288330584912,
44.5680976469492));
#150419=CARTESIAN_POINT('Ctrl Pts',(-3.51506610075752,-6.06645999490686,
44.5593675976805));
#150420=CARTESIAN_POINT('Ctrl Pts',(-3.68152592846285,-5.97000880294381,
44.5506350240981));
#150421=CARTESIAN_POINT('Ctrl Pts',(-3.84398489648174,-5.8667192416086,
44.5419024505158));
#150422=CARTESIAN_POINT('Ctrl Pts',(-4.00190118553436,-5.75694480290706,
44.5331698769334));
#150423=CARTESIAN_POINT('Ctrl Pts',(-4.16206091546047,-5.64561085147809,
44.5243132438723));
#150424=CARTESIAN_POINT('Ctrl Pts',(-4.31754767340672,-5.52760652875741,
44.5154566108112));
#150425=CARTESIAN_POINT('Ctrl Pts',(-4.46782846641096,-5.40334483049415,
44.5065999777501));
#150426=CARTESIAN_POINT('Ctrl Pts',(-4.61609852361058,-5.28074573621938,
44.4978618451896));
#150427=CARTESIAN_POINT('Ctrl Pts',(-4.75930086157089,-5.15205586697208,
44.4891237126291));
#150428=CARTESIAN_POINT('Ctrl Pts',(-4.89695780246188,-5.01771171385999,
44.4803855800686));
#150429=CARTESIAN_POINT('Ctrl Pts',(-5.03741495546275,-4.8806347372375,
44.4714696967572));
#150430=CARTESIAN_POINT('Ctrl Pts',(-5.17209847168035,-4.73767117845135,
44.4625538134458));
#150431=CARTESIAN_POINT('Ctrl Pts',(-5.30054060723454,-4.589324115113,44.4536379301343));
#150432=CARTESIAN_POINT('Ctrl Pts',(-5.42898274278872,-4.44097705177465,
44.4447220468229));
#150433=CARTESIAN_POINT('Ctrl Pts',(-5.55118330432975,-4.28724671649079,
44.4358061635115));
#150434=CARTESIAN_POINT('Ctrl Pts',(-5.66671764407193,-4.12867263231949,
44.4268902802001));
#150435=CARTESIAN_POINT('Ctrl Pts',(-5.7799817093088,-3.9732145628439,44.4181495959041));
#150436=CARTESIAN_POINT('Ctrl Pts',(-5.88685113604801,-3.81308482769952,
44.4094089116081));
#150437=CARTESIAN_POINT('Ctrl Pts',(-5.98696423681725,-3.64881978036341,
44.4006682273121));
#150438=CARTESIAN_POINT('Ctrl Pts',(-6.08705932554435,-3.48458428709097,
44.3919291156133));
#150439=CARTESIAN_POINT('Ctrl Pts',(-6.18040037346429,-3.31621520118869,
44.3831900039144));
#150440=CARTESIAN_POINT('Ctrl Pts',(-6.26667006107284,-3.14427621371808,
44.3744508922155));
#150441=CARTESIAN_POINT('Ctrl Pts',(-6.35405749967336,-2.97010950317195,
44.3655985524404));
#150442=CARTESIAN_POINT('Ctrl Pts',(-6.43418891288873,-2.79227998418195,
44.3567462126652));
#150443=CARTESIAN_POINT('Ctrl Pts',(-6.50678286800209,-2.61139871930246,
44.3478938728901));
#150444=CARTESIAN_POINT('Ctrl Pts',(-6.57841155959771,-2.43292258699575,
44.3391592404449));
#150445=CARTESIAN_POINT('Ctrl Pts',(-6.64270190388603,-2.25147562730464,
44.3304246079998));
#150446=CARTESIAN_POINT('Ctrl Pts',(-6.69943182549076,-2.06766529643982,
44.3216899755546));
#150447=CARTESIAN_POINT('Ctrl Pts',(-6.75730848011134,-1.88013944175451,
44.3127787821145));
#150448=CARTESIAN_POINT('Ctrl Pts',(-6.80731569909913,-1.69015392345087,
44.3038675886743));
#150449=CARTESIAN_POINT('Ctrl Pts',(-6.84927073622432,-1.49837143072108,
44.2949563952341));
#150450=CARTESIAN_POINT('Ctrl Pts',(-6.8912257733495,-1.30658893799135,
44.286045201794));
#150451=CARTESIAN_POINT('Ctrl Pts',(-6.9251285506676,-1.11300976408271,
44.2771340083538));
#150452=CARTESIAN_POINT('Ctrl Pts',(-6.95085125138724,-0.918310102083431,
44.2682228149136));
#150453=CARTESIAN_POINT('Ctrl Pts',(-6.97401782021059,-0.742958253583889,
44.2601971500202));
#150454=CARTESIAN_POINT('Ctrl Pts',(-6.99055941706707,-0.566616890051982,
44.2521714851268));
#150455=CARTESIAN_POINT('Ctrl Pts',(-7.00040398867454,-0.389834013202616,
44.2441458202334));
#150456=CARTESIAN_POINT('Ctrl Pts',(-7.01024543585677,-0.213107242896276,
44.2361227024889));
#150457=CARTESIAN_POINT('Ctrl Pts',(-7.01339406904623,-0.0359396038173357,
44.2280995847444));
#150458=CARTESIAN_POINT('Ctrl Pts',(-7.00982972561212,0.14111619476412,
44.2200764669999));
#150459=CARTESIAN_POINT('Ctrl Pts',(-7.00626583167286,0.318149665062288,
44.2120543610406));
#150460=CARTESIAN_POINT('Ctrl Pts',(-6.99599065533762,0.495070956576405,
44.2040322550814));
#150461=CARTESIAN_POINT('Ctrl Pts',(-6.9790361450392,0.671327825087306,
44.1960101491221));
#150462=CARTESIAN_POINT('Ctrl Pts',(-6.96207533438705,0.847650191250387,
44.187985062121));
#150463=CARTESIAN_POINT('Ctrl Pts',(-6.93843026353939,1.02330727566344,
44.1799599751198));
#150464=CARTESIAN_POINT('Ctrl Pts',(-6.90818476814346,1.19775196584715,
44.1719348881187));
#150465=CARTESIAN_POINT('Ctrl Pts',(-6.87793331604822,1.37223101204163,
44.1639082206168));
#150466=CARTESIAN_POINT('Ctrl Pts',(-6.8410789210492,1.5454968286583,44.1558815531148));
#150467=CARTESIAN_POINT('Ctrl Pts',(-6.79775642319675,1.71701315469256,
44.1478548856129));
#150468=CARTESIAN_POINT('Ctrl Pts',(-6.75439914619576,1.88866717342872,
44.1398217743306));
#150469=CARTESIAN_POINT('Ctrl Pts',(-6.7045634942428,2.05856854341172,44.1317886630483));
#150470=CARTESIAN_POINT('Ctrl Pts',(-6.64843417739367,2.22619620684338,
44.123755551766));
#150471=CARTESIAN_POINT('Ctrl Pts',(-6.61536074680689,2.32496850984203,
44.119022151053));
#150472=CARTESIAN_POINT('Ctrl Pts',(-6.5801030882891,2.42295172150919,44.11428875034));
#150473=CARTESIAN_POINT('Ctrl Pts',(-6.54270674875877,2.52004265087844,
44.1095553496271));
#150474=CARTESIAN_POINT('Ctrl Pts',(-6.46566912147763,2.72005299742754,
44.0998043963392));
#150475=CARTESIAN_POINT('Ctrl Pts',(-6.379508204051,2.91639371319058,44.0900534430514));
#150476=CARTESIAN_POINT('Ctrl Pts',(-6.28457804557364,3.10832838541777,
44.0803024897635));
#150477=CARTESIAN_POINT('Ctrl Pts',(-6.18951112239274,3.30053957555,44.070537488398));
#150478=CARTESIAN_POINT('Ctrl Pts',(-6.08564970409685,3.48833199018424,
44.0607724870325));
#150479=CARTESIAN_POINT('Ctrl Pts',(-5.97339474361976,3.67099193671082,
44.051007485667));
#150480=CARTESIAN_POINT('Ctrl Pts',(-5.86132688889493,3.85334742696608,
44.0412587605348));
#150481=CARTESIAN_POINT('Ctrl Pts',(-5.74089347275576,4.03058751430809,
44.0315100354026));
#150482=CARTESIAN_POINT('Ctrl Pts',(-5.61253818956788,4.20202827609978,
44.0217613102704));
#150483=CARTESIAN_POINT('Ctrl Pts',(-5.48453519185473,4.37299849948701,
44.0120393416081));
#150484=CARTESIAN_POINT('Ctrl Pts',(-5.34865375627933,4.53820114084512,
44.0023173729457));
#150485=CARTESIAN_POINT('Ctrl Pts',(-5.20537825628705,4.69698454026346,
43.9925954042833));
#150486=CARTESIAN_POINT('Ctrl Pts',(-5.06305077284174,4.85471731141641,
43.9829377633473));
#150487=CARTESIAN_POINT('Ctrl Pts',(-4.91342676057244,5.00611545474773,
43.9732801224114));
#150488=CARTESIAN_POINT('Ctrl Pts',(-4.75702469715459,5.15056721081875,
43.9636224814754));
#150489=CARTESIAN_POINT('Ctrl Pts',(-4.68828060523655,5.2140587311994,43.9593776157638));
#150490=CARTESIAN_POINT('Ctrl Pts',(-4.61822762680022,5.27620863318986,
43.9551327500523));
#150491=CARTESIAN_POINT('Ctrl Pts',(-4.54691248151948,5.33696668978759,
43.9508878843408));
#150492=CARTESIAN_POINT('Ctrl Pts',(-4.41499885970426,5.44935256895409,
43.9430360373324));
#150493=CARTESIAN_POINT('Ctrl Pts',(-4.27881845835598,5.55692720483943,
43.935184190324));
#150494=CARTESIAN_POINT('Ctrl Pts',(-4.13877606194018,5.65934265366668,
43.9273323433156));
#150495=CARTESIAN_POINT('Ctrl Pts',(-3.9987733804172,5.76172905829961,43.9194827230276));
#150496=CARTESIAN_POINT('Ctrl Pts',(-3.8549111900341,5.85895896128015,43.9116331027396));
#150497=CARTESIAN_POINT('Ctrl Pts',(-3.70762655175944,5.95072532681424,
43.9037834824516));
#150498=CARTESIAN_POINT('Ctrl Pts',(-3.56035367227979,6.04248436597748,
43.8959344888554));
#150499=CARTESIAN_POINT('Ctrl Pts',(-3.40965921301176,6.12878053494963,
43.8880854952592));
#150500=CARTESIAN_POINT('Ctrl Pts',(-3.25600811563665,6.20935082866223,
43.880236501663));
#150501=CARTESIAN_POINT('Ctrl Pts',(-3.10227922921283,6.28996191275386,
43.8723835343513));
#150502=CARTESIAN_POINT('Ctrl Pts',(-2.94559105215743,6.36484115217058,
43.8645305670397));
#150503=CARTESIAN_POINT('Ctrl Pts',(-2.78643226795437,6.43377197129356,
43.856677599728));
#150504=CARTESIAN_POINT('Ctrl Pts',(-2.62723306276852,6.50272029652825,
43.8488226380265));
#150505=CARTESIAN_POINT('Ctrl Pts',(-2.46556235588125,6.56571705328878,
43.840967676325));
#150506=CARTESIAN_POINT('Ctrl Pts',(-2.301926966983,6.62259456717505,43.8331127146235));
#150507=CARTESIAN_POINT('Ctrl Pts',(-2.1381291562848,6.67952853674761,43.8252499562161));
#150508=CARTESIAN_POINT('Ctrl Pts',(-1.97236313326889,6.73033102067285,
43.8173871978086));
#150509=CARTESIAN_POINT('Ctrl Pts',(-1.80514952533018,6.77488463028709,
43.8095244394011));
#150510=CARTESIAN_POINT('Ctrl Pts',(-1.68248402110205,6.80756851921147,
43.8037564326188));
#150511=CARTESIAN_POINT('Ctrl Pts',(-1.55903978214239,6.83689064534657,
43.7979884258366));
#150512=CARTESIAN_POINT('Ctrl Pts',(-1.43502476922851,6.86282234027668,
43.7922204190543));
#150513=CARTESIAN_POINT('Ctrl Pts',(-1.25489217619602,6.90048829167832,
43.7838423526097));
#150514=CARTESIAN_POINT('Ctrl Pts',(-1.07315613190083,6.93108293751319,
43.7754642861651));
#150515=CARTESIAN_POINT('Ctrl Pts',(-0.890397560720694,6.95448191789745,
43.7670862197205));
#150516=CARTESIAN_POINT('Ctrl Pts',(-0.707763957678036,6.97786489833721,
43.7587138820982));
#150517=CARTESIAN_POINT('Ctrl Pts',(-0.524109546755221,6.99406198135615,
43.7503415444758));
#150518=CARTESIAN_POINT('Ctrl Pts',(-0.340024337999865,7.00300007225959,
43.7419692068534));
#150519=CARTESIAN_POINT('Ctrl Pts',(-0.156038008303853,7.01193336217968,
43.7336013663271));
#150520=CARTESIAN_POINT('Ctrl Pts',(0.0283783302363337,7.01361541846707,
43.7252335258007));
#150521=CARTESIAN_POINT('Ctrl Pts',(0.212630203911086,7.00802503983003,
43.7168656852744));
#150522=CARTESIAN_POINT('Ctrl Pts',(0.396810100565737,7.00243684504485,
43.7085011136007));
#150523=CARTESIAN_POINT('Ctrl Pts',(0.580825332396124,6.98958189052553,
43.7001365419271));
#150524=CARTESIAN_POINT('Ctrl Pts',(0.76408162212722,6.96949107447792,43.6917719702534));
#150525=CARTESIAN_POINT('Ctrl Pts',(0.947293148055745,6.94940516599079,
43.683409441784));
#150526=CARTESIAN_POINT('Ctrl Pts',(1.12974577519655,6.92208695700521,43.6750469133146));
#150527=CARTESIAN_POINT('Ctrl Pts',(1.31085008228257,6.8876192275909,43.6666843848452));
#150528=CARTESIAN_POINT('Ctrl Pts',(1.49196884206102,6.85314874754353,43.6583211890198));
#150529=CARTESIAN_POINT('Ctrl Pts',(1.67173874281103,6.81152766269534,43.6499579931944));
#150530=CARTESIAN_POINT('Ctrl Pts',(1.84957953144805,6.76289007151147,43.6415947973689));
#150531=CARTESIAN_POINT('Ctrl Pts',(2.02743244847089,6.71424916334124,43.6332310311903));
#150532=CARTESIAN_POINT('Ctrl Pts',(2.20335567381335,6.6585908812086,43.6248672650117));
#150533=CARTESIAN_POINT('Ctrl Pts',(2.37678295118015,6.59609955697148,43.616503498833));
#150534=CARTESIAN_POINT('Ctrl Pts',(2.5502451778748,6.53359563938797,43.6081380471755));
#150535=CARTESIAN_POINT('Ctrl Pts',(2.72121014431174,6.46425604538771,43.599772595518));
#150536=CARTESIAN_POINT('Ctrl Pts',(2.88913004700044,6.3883138725347,43.5914071438606));
#150537=CARTESIAN_POINT('Ctrl Pts',(3.05710618573493,6.31234626679707,43.5830388906297));
#150538=CARTESIAN_POINT('Ctrl Pts',(3.22203492778689,6.22977180845838,43.5746706373989));
#150539=CARTESIAN_POINT('Ctrl Pts',(3.38339122465858,6.14087049068806,43.5663023841681));
#150540=CARTESIAN_POINT('Ctrl Pts',(3.5448971218377,6.05188674871287,43.5579263723726));
#150541=CARTESIAN_POINT('Ctrl Pts',(3.70282366687429,5.95656458430923,43.5495503605772));
#150542=CARTESIAN_POINT('Ctrl Pts',(3.85667199919042,5.85522908630914,43.5411743487818));
#150543=CARTESIAN_POINT('Ctrl Pts',(4.01059578063015,5.75384389212841,43.5327942292866));
#150544=CARTESIAN_POINT('Ctrl Pts',(4.16043709015145,5.64643966964964,43.5244141097915));
#150545=CARTESIAN_POINT('Ctrl Pts',(4.30572803323922,5.53338347363329,43.5160339902963));
#150546=CARTESIAN_POINT('Ctrl Pts',(4.45118498963338,5.42019809659221,43.5076442954532));
#150547=CARTESIAN_POINT('Ctrl Pts',(4.59208093466106,5.30134804849269,43.49925460061));
#150548=CARTESIAN_POINT('Ctrl Pts',(4.72798188378807,5.17723998565566,43.4908649057668));
#150549=CARTESIAN_POINT('Ctrl Pts',(4.81426305039246,5.09844591898154,43.4855384333384));
#150550=CARTESIAN_POINT('Ctrl Pts',(4.89853157930441,5.01753323209812,43.4802119609099));
#150551=CARTESIAN_POINT('Ctrl Pts',(4.98068446843869,4.93461333726906,43.4748854884815));
#150552=CARTESIAN_POINT('Ctrl Pts',(5.10997061793832,4.80412013085434,43.4665030795614));
#150553=CARTESIAN_POINT('Ctrl Pts',(5.23427606721581,4.66839085165557,43.4581206706413));
#150554=CARTESIAN_POINT('Ctrl Pts',(5.35316640439172,4.52782906141474,43.4497382617213));
#150555=CARTESIAN_POINT('Ctrl Pts',(5.47190490539542,4.38744678419992,43.4413665580689));
#150556=CARTESIAN_POINT('Ctrl Pts',(5.58524186683985,4.24224454396566,43.4329948544165));
#150557=CARTESIAN_POINT('Ctrl Pts',(5.69277926922287,4.09266303944099,43.4246231507641));
#150558=CARTESIAN_POINT('Ctrl Pts',(5.80015425178126,3.94330745632778,43.4162640913695));
#150559=CARTESIAN_POINT('Ctrl Pts',(5.90174695544359,3.78958606530125,43.4079050319749));
#150560=CARTESIAN_POINT('Ctrl Pts',(5.99719936852696,3.63197278302576,43.3995459725804));
#150561=CARTESIAN_POINT('Ctrl Pts',(6.09256670581634,3.47449997991365,43.3911943635329));
#150562=CARTESIAN_POINT('Ctrl Pts',(6.18180448879049,3.31314247621896,43.3828427544855));
#150563=CARTESIAN_POINT('Ctrl Pts',(6.26459705733132,3.14840440092688,43.3744911454381));
#150564=CARTESIAN_POINT('Ctrl Pts',(6.34730824439963,2.98382825595517,43.366147745657));
#150565=CARTESIAN_POINT('Ctrl Pts',(6.423586704806,2.8158784578497,43.3578043458758));
#150566=CARTESIAN_POINT('Ctrl Pts',(6.49316189671506,2.64508509230757,43.3494609460947));
#150567=CARTESIAN_POINT('Ctrl Pts',(6.52015758027675,2.57881601673478,43.3462236459287));
#150568=CARTESIAN_POINT('Ctrl Pts',(6.54614457413794,2.51211911340437,43.3429863457626));
#150569=CARTESIAN_POINT('Ctrl Pts',(6.57110895151813,2.44502632087639,43.3397490455966));
#150570=CARTESIAN_POINT('Origin',(0.,0.,50.));
#150571=CARTESIAN_POINT('',(6.57110895151812,2.44502632087641,41.3399811574536));
#150572=CARTESIAN_POINT('',(6.57110895151814,2.44502632087636,41.8868188187145));
#150573=CARTESIAN_POINT('',(6.57110895151814,2.44502632087636,50.));
#150574=CARTESIAN_POINT('',(7.01124999682068,0.000211144444567105,43.773534356952));
#150575=CARTESIAN_POINT('Ctrl Pts',(6.57110895151814,2.44502632087636,41.8868188187145));
#150576=CARTESIAN_POINT('Ctrl Pts',(6.49634775445724,2.64595011749914,41.8965749404131));
#150577=CARTESIAN_POINT('Ctrl Pts',(6.41241070130866,2.84332624237747,41.9063310621117));
#150578=CARTESIAN_POINT('Ctrl Pts',(6.31963860203007,3.03641145140632,41.9160871838103));
#150579=CARTESIAN_POINT('Ctrl Pts',(6.22273057746059,3.23810470105867,41.9262782486737));
#150580=CARTESIAN_POINT('Ctrl Pts',(6.11618184448681,3.43511568285639,41.9364693135372));
#150581=CARTESIAN_POINT('Ctrl Pts',(6.00043438823921,3.62662566512404,41.9466603784007));
#150582=CARTESIAN_POINT('Ctrl Pts',(5.88978216895778,3.80970532181327,41.9564028296004));
#150583=CARTESIAN_POINT('Ctrl Pts',(5.77072362067052,3.98775777918142,41.9661452808002));
#150584=CARTESIAN_POINT('Ctrl Pts',(5.64369136065054,4.16009307446581,41.9758877319999));
#150585=CARTESIAN_POINT('Ctrl Pts',(5.51705865913114,4.33188631821016,41.9855995399662));
#150586=CARTESIAN_POINT('Ctrl Pts',(5.38250232509575,4.49799825636314,41.9953113479326));
#150587=CARTESIAN_POINT('Ctrl Pts',(5.24049601625629,4.65777071849849,42.0050231558989));
#150588=CARTESIAN_POINT('Ctrl Pts',(5.09942435511159,4.81649160085094,42.0146710433324));
#150589=CARTESIAN_POINT('Ctrl Pts',(4.95100046635482,4.96895612026904,42.0243189307659));
#150590=CARTESIAN_POINT('Ctrl Pts',(4.79573326718458,5.11454484705327,42.0339668181994));
#150591=CARTESIAN_POINT('Ctrl Pts',(4.77205912059392,5.13674328225566,42.0354378661903));
#150592=CARTESIAN_POINT('Ctrl Pts',(4.7482259642621,5.15878191801865,42.0369089141811));
#150593=CARTESIAN_POINT('Ctrl Pts',(4.72423569406022,5.18065861348414,42.038379962172));
#150594=CARTESIAN_POINT('Ctrl Pts',(4.59618553349387,5.29742738446687,42.0462318091854));
#150595=CARTESIAN_POINT('Ctrl Pts',(4.46370883293055,5.40953147826222,42.0540836561987));
#150596=CARTESIAN_POINT('Ctrl Pts',(4.32719841771571,5.51660950369144,42.0619355032121));
#150597=CARTESIAN_POINT('Ctrl Pts',(4.19072671575122,5.62365716265816,42.0697851235051));
#150598=CARTESIAN_POINT('Ctrl Pts',(4.0502238744537,5.72568135332894,42.0776347437981));
#150599=CARTESIAN_POINT('Ctrl Pts',(3.90611635632225,5.82236048122854,42.0854843640911));
#150600=CARTESIAN_POINT('Ctrl Pts',(3.76202034333272,5.91903189053648,42.0933333576923));
#150601=CARTESIAN_POINT('Ctrl Pts',(3.614320543612,6.01035887468585,42.1011823512936));
#150602=CARTESIAN_POINT('Ctrl Pts',(3.46347276878749,6.09606290505335,42.1090313448948));
#150603=CARTESIAN_POINT('Ctrl Pts',(3.31254862415192,6.18181032486172,42.1168843122116));
#150604=CARTESIAN_POINT('Ctrl Pts',(3.15847365216846,6.26192891428101,42.1247372795285));
#150605=CARTESIAN_POINT('Ctrl Pts',(3.00172895789514,6.33618574742201,42.1325902468453));
#150606=CARTESIAN_POINT('Ctrl Pts',(2.84494445573594,6.41046143930366,42.140445208552));
#150607=CARTESIAN_POINT('Ctrl Pts',(2.68548923111737,6.47887225867085,42.1483001702587));
#150608=CARTESIAN_POINT('Ctrl Pts',(2.52386416344037,6.54123354169544,42.1561551319654));
#150609=CARTESIAN_POINT('Ctrl Pts',(2.36207866937374,6.6036567235061,42.1640178903782));
#150610=CARTESIAN_POINT('Ctrl Pts',(2.19811939124847,6.66001825216441,42.1718806487909));
#150611=CARTESIAN_POINT('Ctrl Pts',(2.03250270343796,6.71018325554656,42.1797434072037));
#150612=CARTESIAN_POINT('Ctrl Pts',(1.911008677637,6.74698358222734,42.1855114139553));
#150613=CARTESIAN_POINT('Ctrl Pts',(1.78862303579138,6.78045030764135,42.1912794207069));
#150614=CARTESIAN_POINT('Ctrl Pts',(1.66555265408132,6.81054776937822,42.1970474274585));
#150615=CARTESIAN_POINT('Ctrl Pts',(1.48679214299145,6.85426452370882,42.2054254938995));
#150616=CARTESIAN_POINT('Ctrl Pts',(1.30619072057563,6.89096804313974,42.2138035603405));
#150617=CARTESIAN_POINT('Ctrl Pts',(1.12432478892261,6.92051445569722,42.2221816267815));
#150618=CARTESIAN_POINT('Ctrl Pts',(0.942583215032855,6.95004066476883,
42.2305539644002));
#150619=CARTESIAN_POINT('Ctrl Pts',(0.759579179210775,6.97241947149838,
42.2389263020189));
#150620=CARTESIAN_POINT('Ctrl Pts',(0.575899892183811,6.98755793369062,
42.2472986396376));
#150621=CARTESIAN_POINT('Ctrl Pts',(0.392319266182059,7.00268826444776,
42.2556664801601));
#150622=CARTESIAN_POINT('Ctrl Pts',(0.208064439051259,7.01058597814459,
42.2640343206827));
#150623=CARTESIAN_POINT('Ctrl Pts',(0.0237288319533614,7.01120984602758,
42.2724021612053));
#150624=CARTESIAN_POINT('Ctrl Pts',(-0.160534765413851,7.01183347019988,
42.2807667328752));
#150625=CARTESIAN_POINT('Ctrl Pts',(-0.344878751594196,7.00518891378272,
42.289131304545));
#150626=CARTESIAN_POINT('Ctrl Pts',(-0.52870814549189,6.99128702453207,
42.2974958762149));
#150627=CARTESIAN_POINT('Ctrl Pts',(-0.712492635593976,6.97738853108,42.3058584046805));
#150628=CARTESIAN_POINT('Ctrl Pts',(-0.89576245665924,6.95623626526056,
42.314220933146));
#150629=CARTESIAN_POINT('Ctrl Pts',(-1.07792573191966,6.92789309090184,
42.3225834616116));
#150630=CARTESIAN_POINT('Ctrl Pts',(-1.26010354437941,6.89954765466913,
42.330946657433));
#150631=CARTESIAN_POINT('Ctrl Pts',(-1.4411743089208,6.86401020797288,42.3393098532545));
#150632=CARTESIAN_POINT('Ctrl Pts',(-1.62055358182172,6.8213952129271,42.347673049076));
#150633=CARTESIAN_POINT('Ctrl Pts',(-1.7999450880295,6.77877731162408,42.3560368152507));
#150634=CARTESIAN_POINT('Ctrl Pts',(-1.97764455260624,6.72908097530092,
42.3644005814254));
#150635=CARTESIAN_POINT('Ctrl Pts',(-2.15307982731324,6.67247134274227,
42.3727643476));
#150636=CARTESIAN_POINT('Ctrl Pts',(-2.32855045600308,6.61585030212454,
42.3811297992536));
#150637=CARTESIAN_POINT('Ctrl Pts',(-2.50175567208873,6.55231328821959,
42.3894952509071));
#150638=CARTESIAN_POINT('Ctrl Pts',(-2.67214012577323,6.48207479984092,
42.3978607025606));
#150639=CARTESIAN_POINT('Ctrl Pts',(-2.84258164087623,6.4118127887306,42.4062289557875));
#150640=CARTESIAN_POINT('Ctrl Pts',(-3.01020020603632,6.33484495318477,
42.4145972090143));
#150641=CARTESIAN_POINT('Ctrl Pts',(-3.17446163268164,6.2514334280333,42.4229654622412));
#150642=CARTESIAN_POINT('Ctrl Pts',(-3.33887535310399,6.16794456849803,
42.4313414740326));
#150643=CARTESIAN_POINT('Ctrl Pts',(-3.49992542175955,6.07800023010056,
42.439717485824));
#150644=CARTESIAN_POINT('Ctrl Pts',(-3.65710230295307,5.98190850049007,
42.4480934976155));
#150645=CARTESIAN_POINT('Ctrl Pts',(-3.81435626563119,5.88576964630808,
42.4564736171066));
#150646=CARTESIAN_POINT('Ctrl Pts',(-3.96773297603646,5.78347756587186,
42.4648537365977));
#150647=CARTESIAN_POINT('Ctrl Pts',(-4.11675243227998,5.67538333276413,
42.4732338560889));
#150648=CARTESIAN_POINT('Ctrl Pts',(-4.26594216212908,5.56716558830239,
42.481623550928));
#150649=CARTESIAN_POINT('Ctrl Pts',(-4.41076442696253,5.45313264202748,
42.4900132457672));
#150650=CARTESIAN_POINT('Ctrl Pts',(-4.55077178064475,5.33367628966995,
42.4984029406064));
#150651=CARTESIAN_POINT('Ctrl Pts',(-4.63966003343352,5.25783551297988,
42.5037294130814));
#150652=CARTESIAN_POINT('Ctrl Pts',(-4.72660821032529,5.17980947477562,
42.5090558855564));
#150653=CARTESIAN_POINT('Ctrl Pts',(-4.81150961210109,5.09970605183856,
42.5143823580314));
#150654=CARTESIAN_POINT('Ctrl Pts',(-4.94510349747565,4.9736618726126,42.5227636584386));
#150655=CARTESIAN_POINT('Ctrl Pts',(-5.0738972901008,4.84221812798493,42.5311449588458));
#150656=CARTESIAN_POINT('Ctrl Pts',(-5.19744339656311,4.70576334955579,
42.539526259253));
#150657=CARTESIAN_POINT('Ctrl Pts',(-5.32083292642105,4.56948150758307,
42.5478969375889));
#150658=CARTESIAN_POINT('Ctrl Pts',(-5.43898780609068,4.42820152911682,
42.5562676159247));
#150659=CARTESIAN_POINT('Ctrl Pts',(-5.55149553120376,4.28235028104015,
42.5646382942606));
#150660=CARTESIAN_POINT('Ctrl Pts',(-5.66387557936526,4.13666454908889,
42.5729994733137));
#150661=CARTESIAN_POINT('Ctrl Pts',(-5.77062104701019,3.98641814485308,
42.5813606523668));
#150662=CARTESIAN_POINT('Ctrl Pts',(-5.87135786099275,3.83207299391057,
42.5897218314199));
#150663=CARTESIAN_POINT('Ctrl Pts',(-5.97196395707572,3.67792812400876,
42.5980721608568));
#150664=CARTESIAN_POINT('Ctrl Pts',(-6.06657677307801,3.51969538901241,
42.6064224902938));
#150665=CARTESIAN_POINT('Ctrl Pts',(-6.15486398375714,3.35786776153398,
42.6147728197307));
#150666=CARTESIAN_POINT('Ctrl Pts',(-6.24308326270857,3.19616465073514,
42.6231167240886));
#150667=CARTESIAN_POINT('Ctrl Pts',(-6.32498647947614,3.0308724461063,42.6314606284466));
#150668=CARTESIAN_POINT('Ctrl Pts',(-6.40028531910473,2.86251190330321,
42.6398045328045));
#150669=CARTESIAN_POINT('Ctrl Pts',(-6.47552367823529,2.69428658873902,
42.6481417352864));
#150670=CARTESIAN_POINT('Ctrl Pts',(-6.544168106265,2.52299814934422,42.6564789377682));
#150671=CARTESIAN_POINT('Ctrl Pts',(-6.60597677102849,2.34919081028596,
42.6648161402501));
#150672=CARTESIAN_POINT('Ctrl Pts',(-6.62632384218751,2.29197439395809,
42.6675607012726));
#150673=CARTESIAN_POINT('Ctrl Pts',(-6.64593050743587,2.23448518751981,
42.6703052622952));
#150674=CARTESIAN_POINT('Ctrl Pts',(-6.6647892687086,2.17674310983329,42.6730498233177));
#150675=CARTESIAN_POINT('Ctrl Pts',(-6.72208447986242,2.00131565276619,
42.6813881336148));
#150676=CARTESIAN_POINT('Ctrl Pts',(-6.77242574458169,1.82369680875694,
42.689726443912));
#150677=CARTESIAN_POINT('Ctrl Pts',(-6.81567017131908,1.64446546886562,
42.6980647542091));
#150678=CARTESIAN_POINT('Ctrl Pts',(-6.85894180598198,1.46512136269862,
42.706408310688));
#150679=CARTESIAN_POINT('Ctrl Pts',(-6.89510761963726,1.28416305555848,
42.714751867167));
#150680=CARTESIAN_POINT('Ctrl Pts',(-6.92407593220817,1.10217922658505,
42.7230954236459));
#150681=CARTESIAN_POINT('Ctrl Pts',(-6.95306628374478,0.920056945109259,
42.7314453278662));
#150682=CARTESIAN_POINT('Ctrl Pts',(-6.97484816025958,0.73690790874185,
42.7397952320865));
#150683=CARTESIAN_POINT('Ctrl Pts',(-6.98938172955066,0.553325944740973,
42.7481451363067));
#150684=CARTESIAN_POINT('Ctrl Pts',(-7.00393709812007,0.369468621380576,
42.7565075647654));
#150685=CARTESIAN_POINT('Ctrl Pts',(-7.01122240806093,0.185177399674693,
42.764869993224));
#150686=CARTESIAN_POINT('Ctrl Pts',(-7.01124992172655,0.0010476590323406,
42.7732324216827));
#150687=CARTESIAN_POINT('Ctrl Pts',(-7.0112774589201,-0.183239537638157,
42.7816020011576));
#150688=CARTESIAN_POINT('Ctrl Pts',(-7.00403482930223,-0.367364651104122,
42.7899715806325));
#150689=CARTESIAN_POINT('Ctrl Pts',(-6.98958621938242,-0.55073681946946,
42.7983411601074));
#150690=CARTESIAN_POINT('Ctrl Pts',(-6.97511532424224,-0.734391817062343,
42.8067236486389));
#150691=CARTESIAN_POINT('Ctrl Pts',(-6.95341627754758,-0.91729122414129,
42.8151061371704));
#150692=CARTESIAN_POINT('Ctrl Pts',(-6.9246046847036,-1.09885236637184,
42.8234886257019));
#150693=CARTESIAN_POINT('Ctrl Pts',(-6.91517705931131,-1.15826214784472,
42.826231513336));
#150694=CARTESIAN_POINT('Ctrl Pts',(-6.90498829125242,-1.2175287479788,
42.8289744009701));
#150695=CARTESIAN_POINT('Ctrl Pts',(-6.89404359269516,-1.27663209442611,
42.8317172886042));
#150696=CARTESIAN_POINT('Ctrl Pts',(-6.86056630610528,-1.45741548074663,
42.8401071437409));
#150697=CARTESIAN_POINT('Ctrl Pts',(-6.81994515840763,-1.63703542479715,
42.8484969988776));
#150698=CARTESIAN_POINT('Ctrl Pts',(-6.77227735039567,-1.81490662344314,
42.8568868540143));
#150699=CARTESIAN_POINT('Ctrl Pts',(-6.72465352956857,-1.99261368504108,
42.8652689671104));
#150700=CARTESIAN_POINT('Ctrl Pts',(-6.66999609595334,-2.1685749021898,
42.8736510802064));
#150701=CARTESIAN_POINT('Ctrl Pts',(-6.60845327083364,-2.34221517579155,
42.8820331933024));
#150702=CARTESIAN_POINT('Ctrl Pts',(-6.54695818990252,-2.51572074134322,
42.8904088036553));
#150703=CARTESIAN_POINT('Ctrl Pts',(-6.47858847642109,-2.68690864438706,
42.8987844140081));
#150704=CARTESIAN_POINT('Ctrl Pts',(-6.40354228024374,-2.85521852537259,
42.9071600243609));
#150705=CARTESIAN_POINT('Ctrl Pts',(-6.32854328923818,-3.02342253694367,
42.9155303663304));
#150706=CARTESIAN_POINT('Ctrl Pts',(-6.24687632269961,-3.18875183660909,
42.9239007083));
#150707=CARTESIAN_POINT('Ctrl Pts',(-6.15878795967867,-3.35066522204429,
42.9322710502695));
#150708=CARTESIAN_POINT('Ctrl Pts',(-6.07074209278142,-3.5125004962396,
42.9406373541678));
#150709=CARTESIAN_POINT('Ctrl Pts',(-5.97628116383119,-3.67092285419517,
42.949003658066));
#150710=CARTESIAN_POINT('Ctrl Pts',(-5.87569828684232,-3.82541451407534,
42.9573699619643));
#150711=CARTESIAN_POINT('Ctrl Pts',(-5.7751435400653,-3.97986296696787,
42.9657339260418));
#150712=CARTESIAN_POINT('Ctrl Pts',(-5.66847043717592,-4.13038263781536,
42.9740978901194));
#150713=CARTESIAN_POINT('Ctrl Pts',(-5.55601641213195,-4.27648315682646,
42.9824618541969));
#150714=CARTESIAN_POINT('Ctrl Pts',(-5.443579691894,-4.42256119339517,42.9908245311993));
#150715=CARTESIAN_POINT('Ctrl Pts',(-5.32536402356713,-4.56422117361238,
42.9991872082018));
#150716=CARTESIAN_POINT('Ctrl Pts',(-5.20174852013774,-4.70100403060291,
43.0075498852042));
#150717=CARTESIAN_POINT('Ctrl Pts',(-5.07813556172623,-4.83778407148377,
43.0159123900343));
#150718=CARTESIAN_POINT('Ctrl Pts',(-4.94912321054614,-4.96968694579816,
43.0242748948645));
#150719=CARTESIAN_POINT('Ctrl Pts',(-4.81512927927796,-5.09628851090087,
43.0326373996947));
#150720=CARTESIAN_POINT('Ctrl Pts',(-4.68112024626328,-5.22290434459561,
43.0410008470185));
#150721=CARTESIAN_POINT('Ctrl Pts',(-4.54212875304066,-5.34421745256245,
43.0493642943423));
#150722=CARTESIAN_POINT('Ctrl Pts',(-4.39860801316389,-5.45984194908886,
43.057727741666));
#150723=CARTESIAN_POINT('Ctrl Pts',(-4.25500276424368,-5.57553452856696,
43.0660961136226));
#150724=CARTESIAN_POINT('Ctrl Pts',(-4.10686319507153,-5.68553159612633,
43.0744644855791));
#150725=CARTESIAN_POINT('Ctrl Pts',(-3.95467483375107,-5.78948819169674,
43.0828328575356));
#150726=CARTESIAN_POINT('Ctrl Pts',(-3.80244087282097,-5.8934759353795,
43.0912037368751));
#150727=CARTESIAN_POINT('Ctrl Pts',(-3.64615597522751,-5.99141941716492,
43.0995746162145));
#150728=CARTESIAN_POINT('Ctrl Pts',(-3.48633354181123,-6.08301775418599,
43.1079454955539));
#150729=CARTESIAN_POINT('Ctrl Pts',(-3.32637569257764,-6.17469370148621,
43.1163234674488));
#150730=CARTESIAN_POINT('Ctrl Pts',(-3.16287460639404,-6.26001360258637,
43.1247014393436));
#150731=CARTESIAN_POINT('Ctrl Pts',(-2.99636812996869,-6.33872263095712,
43.1330794112385));
#150732=CARTESIAN_POINT('Ctrl Pts',(-2.89055190929516,-6.38874285896196,
43.1384036805513));
#150733=CARTESIAN_POINT('Ctrl Pts',(-2.7835223511343,-6.4360940987398,43.1437279498642));
#150734=CARTESIAN_POINT('Ctrl Pts',(-2.67542150514982,-6.48072112748897,
43.149052219177));
#150735=CARTESIAN_POINT('Ctrl Pts',(-2.51577918564716,-6.54662590665278,
43.1569150503604));
#150736=CARTESIAN_POINT('Ctrl Pts',(-2.35346754120656,-6.60672387524485,
43.1647778815438));
#150737=CARTESIAN_POINT('Ctrl Pts',(-2.18896620306236,-6.66078475289142,
43.1726407127272));
#150738=CARTESIAN_POINT('Ctrl Pts',(-2.02459126248158,-6.7148040918898,
43.1804975023628));
#150739=CARTESIAN_POINT('Ctrl Pts',(-1.85803033394368,-6.76279544641317,
43.1883542919984));
#150740=CARTESIAN_POINT('Ctrl Pts',(-1.68978413096512,-6.80457611855716,
43.196211081634));
#150741=CARTESIAN_POINT('Ctrl Pts',(-1.52163281087943,-6.84633322838018,
43.2040634404122));
#150742=CARTESIAN_POINT('Ctrl Pts',(-1.3517984758257,-6.88188653155631,
43.2119157991904));
#150743=CARTESIAN_POINT('Ctrl Pts',(-1.18079790401445,-6.91110286946845,
43.2197681579686));
#150744=CARTESIAN_POINT('Ctrl Pts',(-1.00983770743147,-6.94031230906266,
43.2276186627133));
#150745=CARTESIAN_POINT('Ctrl Pts',(-0.837712196201336,-6.96318768883827,
43.2354691674581));
#150746=CARTESIAN_POINT('Ctrl Pts',(-0.664949209373088,-6.97964677555062,
43.2433196722029));
#150747=CARTESIAN_POINT('Ctrl Pts',(-0.49221401466333,-6.99610321451476,
43.2511689140489));
#150748=CARTESIAN_POINT('Ctrl Pts',(-0.318841928596641,-7.0061453819911,
43.2590181558949));
#150749=CARTESIAN_POINT('Ctrl Pts',(-0.145366326392328,-7.00974287642929,
43.266867397741));
#150750=CARTESIAN_POINT('Ctrl Pts',(0.0281677231400067,-7.01334158293382,
43.2747192841503));
#150751=CARTESIAN_POINT('Ctrl Pts',(0.201804976693194,-7.01049127137047,
43.2825711705596));
#150752=CARTESIAN_POINT('Ctrl Pts',(0.375011438366876,-7.00121367932689,
43.290423056969));
#150753=CARTESIAN_POINT('Ctrl Pts',(0.502194788160678,-6.99440125891994,
43.2961885994672));
#150754=CARTESIAN_POINT('Ctrl Pts',(0.629145838212761,-6.9841244781284,
43.3019541419654));
#150755=CARTESIAN_POINT('Ctrl Pts',(0.755654950975328,-6.97040975535632,
43.3077196844635));
#150756=CARTESIAN_POINT('Ctrl Pts',(0.967514283888188,-6.94744230301925,
43.3173749888197));
#150757=CARTESIAN_POINT('Ctrl Pts',(1.17802605320893,-6.91484429355787,
43.3270302931758));
#150758=CARTESIAN_POINT('Ctrl Pts',(1.3864089148058,-6.87280851497021,43.336685597532));
#150759=CARTESIAN_POINT('Ctrl Pts',(1.59594617834613,-6.83053986605855,
43.3463943904621));
#150760=CARTESIAN_POINT('Ctrl Pts',(1.80333084590281,-6.77872865440678,
43.3561031833923));
#150761=CARTESIAN_POINT('Ctrl Pts',(2.0077895948559,-6.71761918430097,43.3658119763224));
#150762=CARTESIAN_POINT('Ctrl Pts',(2.21323221664931,-6.65621565024225,
43.3755674887875));
#150763=CARTESIAN_POINT('Ctrl Pts',(2.41572065796738,-6.58542418978038,
43.3853230012527));
#150764=CARTESIAN_POINT('Ctrl Pts',(2.61449212019618,-6.50554052450156,
43.3950785137178));
#150765=CARTESIAN_POINT('Ctrl Pts',(2.8134603967454,-6.4255777621073,43.4048436856408));
#150766=CARTESIAN_POINT('Ctrl Pts',(3.0087043011956,-6.33650481214536,43.4146088575637));
#150767=CARTESIAN_POINT('Ctrl Pts',(3.19948094731155,-6.23866558089872,
43.4243740294867));
#150768=CARTESIAN_POINT('Ctrl Pts',(3.38999747379362,-6.14095975122681,
43.434125886819));
#150769=CARTESIAN_POINT('Ctrl Pts',(3.57605888192642,-6.0345115466269,43.4438777441513));
#150770=CARTESIAN_POINT('Ctrl Pts',(3.75694787726415,-5.91971023024104,
43.4536296014836));
#150771=CARTESIAN_POINT('Ctrl Pts',(3.83582858036914,-5.86964854165137,
43.4578821175724));
#150772=CARTESIAN_POINT('Ctrl Pts',(3.91372599458072,-5.8179990315438,43.4621346336612));
#150773=CARTESIAN_POINT('Ctrl Pts',(3.99058201580301,-5.76479676464397,
43.4663871497499));
#150774=CARTESIAN_POINT('Ctrl Pts',(4.13576381249401,-5.66429714764961,
43.4744201953904));
#150775=CARTESIAN_POINT('Ctrl Pts',(4.27729824822765,-5.55820459552755,
43.4824532410308));
#150776=CARTESIAN_POINT('Ctrl Pts',(4.41472291734786,-5.44682000120654,
43.4904862866713));
#150777=CARTESIAN_POINT('Ctrl Pts',(4.55205924459962,-5.3355070091913,43.4985141683607));
#150778=CARTESIAN_POINT('Ctrl Pts',(4.68529078044798,-5.21890897645063,
43.5065420500502));
#150779=CARTESIAN_POINT('Ctrl Pts',(4.81398494431232,-5.09736947046556,
43.5145699317396));
#150780=CARTESIAN_POINT('Ctrl Pts',(4.94262100149232,-4.97588484076622,
43.5225941887613));
#150781=CARTESIAN_POINT('Ctrl Pts',(5.06672349986906,-4.84946343141362,
43.5306184457829));
#150782=CARTESIAN_POINT('Ctrl Pts',(5.18589379026815,-4.71848833404919,
43.5386427028046));
#150783=CARTESIAN_POINT('Ctrl Pts',(5.30504967176225,-4.58752907291143,
43.5466659896117));
#150784=CARTESIAN_POINT('Ctrl Pts',(5.41927428085916,-4.45201748622546,
43.5546892764187));
#150785=CARTESIAN_POINT('Ctrl Pts',(5.5282065155607,-4.31237281363895,43.5627125632258));
#150786=CARTESIAN_POINT('Ctrl Pts',(5.63712982423646,-4.17273958368876,
43.570735192596));
#150787=CARTESIAN_POINT('Ctrl Pts',(5.74076139998949,-4.02897423399752,
43.5787578219662));
#150788=CARTESIAN_POINT('Ctrl Pts',(5.83878125308421,-3.88152805492018,
43.5867804513364));
#150789=CARTESIAN_POINT('Ctrl Pts',(5.93683795466156,-3.73402644658235,
43.5948060966438));
#150790=CARTESIAN_POINT('Ctrl Pts',(6.02927851871268,-3.58284155176477,
43.6028317419511));
#150791=CARTESIAN_POINT('Ctrl Pts',(6.1158268140924,-3.42845284968723,43.6108573872585));
#150792=CARTESIAN_POINT('Ctrl Pts',(6.16686096010099,-3.33741586820384,
43.6155897965178));
#150793=CARTESIAN_POINT('Ctrl Pts',(6.2158472163727,-3.24526542402008,43.6203222057771));
#150794=CARTESIAN_POINT('Ctrl Pts',(6.26273655600089,-3.15210364560401,
43.6250546150364));
#150795=CARTESIAN_POINT('Ctrl Pts',(6.34919623652668,-2.98032179363219,
43.6337807475842));
#150796=CARTESIAN_POINT('Ctrl Pts',(6.42856752581141,-2.8050140054996,43.642506880132));
#150797=CARTESIAN_POINT('Ctrl Pts',(6.50059165124866,-2.6267726864379,43.6512330126798));
#150798=CARTESIAN_POINT('Ctrl Pts',(6.57263660920447,-2.44847981221239,
43.6599616692058));
#150799=CARTESIAN_POINT('Ctrl Pts',(6.63733005850005,-2.26725196788813,
43.6686903257318));
#150800=CARTESIAN_POINT('Ctrl Pts',(6.6944618396993,-2.0837003717689,43.6774189822577));
#150801=CARTESIAN_POINT('Ctrl Pts',(6.75162131715772,-1.9000597937823,43.6861518702487));
#150802=CARTESIAN_POINT('Ctrl Pts',(6.80121171769005,-1.71409347458198,
43.6948847582397));
#150803=CARTESIAN_POINT('Ctrl Pts',(6.84307272926248,-1.52642791658307,
43.7036176462306));
#150804=CARTESIAN_POINT('Ctrl Pts',(6.88493932166326,-1.33873733937833,
43.7123516984732));
#150805=CARTESIAN_POINT('Ctrl Pts',(6.9190744118959,-1.14934733992793,43.7210857507157));
#150806=CARTESIAN_POINT('Ctrl Pts',(6.94536873237034,-0.958895058863315,
43.7298198029583));
#150807=CARTESIAN_POINT('Ctrl Pts',(6.97167056821407,-0.768388343259293,
43.7385563515433));
#150808=CARTESIAN_POINT('Ctrl Pts',(6.99012711894441,-0.576819011385682,
43.7472929001283));
#150809=CARTESIAN_POINT('Ctrl Pts',(7.00068079599258,-0.384831073486362,
43.7560294487132));
#150810=CARTESIAN_POINT('Ctrl Pts',(7.00772938984235,-0.256606096340531,
43.7618644181124));
#150811=CARTESIAN_POINT('Ctrl Pts',(7.01125386375248,-0.128194519087721,
43.7676993875115));
#150812=CARTESIAN_POINT('Ctrl Pts',(7.01124999682071,0.000211143533935008,
43.7735343569106));
#150813=CARTESIAN_POINT('Ctrl Pts',(7.01124999682068,0.000211144444558622,
43.773534356952));
#150814=CARTESIAN_POINT('Ctrl Pts',(7.01124774628611,0.0749422630139,43.7769302647423));
#150815=CARTESIAN_POINT('Ctrl Pts',(7.01005060800529,0.149671035510726,
43.7803261725325));
#150816=CARTESIAN_POINT('Ctrl Pts',(7.00765927269819,0.224361494617859,
43.7837220803227));
#150817=CARTESIAN_POINT('Ctrl Pts',(7.00150410130018,0.416610810819736,
43.7924629684945));
#150818=CARTESIAN_POINT('Ctrl Pts',(6.9874329611689,0.608616908168221,43.8012038566662));
#150819=CARTESIAN_POINT('Ctrl Pts',(6.96549004337687,0.799734342214806,
43.809944744838));
#150820=CARTESIAN_POINT('Ctrl Pts',(6.94355157327669,0.990813037955818,
43.8186838612865));
#150821=CARTESIAN_POINT('Ctrl Pts',(6.91374454384324,1.18100315827288,43.8274229777351));
#150822=CARTESIAN_POINT('Ctrl Pts',(6.87616494592498,1.36966499514754,43.8361620941836));
#150823=CARTESIAN_POINT('Ctrl Pts',(6.83859395994941,1.55828359726144,43.8448992079292));
#150824=CARTESIAN_POINT('Ctrl Pts',(6.79325401590017,1.74537434692778,43.8536363216748));
#150825=CARTESIAN_POINT('Ctrl Pts',(6.74029227680452,1.93030738115706,43.8623734354205));
#150826=CARTESIAN_POINT('Ctrl Pts',(6.69056304853439,2.10395305878985,43.8705772809002));
#150827=CARTESIAN_POINT('Ctrl Pts',(6.63411451374727,2.27569627709552,43.8787811263799));
#150828=CARTESIAN_POINT('Ctrl Pts',(6.57110895151816,2.4450263208763,43.8869849718596));
#150829=CARTESIAN_POINT('',(7.01124705281206,-0.0064286028199779,43.2264656431312));
#150830=CARTESIAN_POINT('Ctrl Pts',(6.57110895151813,2.44502632087639,43.3397490455966));
#150831=CARTESIAN_POINT('Ctrl Pts',(6.63159529232099,2.28246678844903,43.3319053714627));
#150832=CARTESIAN_POINT('Ctrl Pts',(6.68607576390869,2.11758215313251,43.3240616973289));
#150833=CARTESIAN_POINT('Ctrl Pts',(6.7343787389157,1.95083816943902,43.316218023195));
#150834=CARTESIAN_POINT('Ctrl Pts',(6.78297200597525,1.78309208487557,43.308327210013));
#150835=CARTESIAN_POINT('Ctrl Pts',(6.82529219205804,1.61353383424519,43.300436396831));
#150836=CARTESIAN_POINT('Ctrl Pts',(6.86121524490491,1.4426891299183,43.292545583649));
#150837=CARTESIAN_POINT('Ctrl Pts',(6.8971430406971,1.2718218688479,43.2846537286376));
#150838=CARTESIAN_POINT('Ctrl Pts',(6.9266719524471,1.09966818699195,43.2767618736261));
#150839=CARTESIAN_POINT('Ctrl Pts',(6.94972928823205,0.926762851429489,
43.2688700186146));
#150840=CARTESIAN_POINT('Ctrl Pts',(6.97280535074523,0.7537170854522,43.2609717539891));
#150841=CARTESIAN_POINT('Ctrl Pts',(6.9893992976703,0.579918821660726,43.2530734893635));
#150842=CARTESIAN_POINT('Ctrl Pts',(6.99949039421429,0.405907358644683,
43.245175224738));
#150843=CARTESIAN_POINT('Ctrl Pts',(7.00745839745054,0.268506641644989,
43.2389386975357));
#150844=CARTESIAN_POINT('Ctrl Pts',(7.01137303626983,0.130973126874985,
43.2327021703335));
#150845=CARTESIAN_POINT('Ctrl Pts',(7.01124705281206,-0.00642860282006959,
43.2264656431312));
#150846=CARTESIAN_POINT('Ctrl Pts',(7.01124705281122,-0.00642860373435615,
43.2264656430897));
#150847=CARTESIAN_POINT('Ctrl Pts',(7.01105339140945,-0.217642109582684,
43.2168788731295));
#150848=CARTESIAN_POINT('Ctrl Pts',(7.00131167626943,-0.428520885109439,
43.2072921031694));
#150849=CARTESIAN_POINT('Ctrl Pts',(6.98213567632272,-0.638285171315712,
43.1977053332092));
#150850=CARTESIAN_POINT('Ctrl Pts',(6.96281940757936,-0.849583843425604,
43.1880484378481));
#150851=CARTESIAN_POINT('Ctrl Pts',(6.93393038750432,-1.05975159588273,
43.1783915424869));
#150852=CARTESIAN_POINT('Ctrl Pts',(6.89563491529918,-1.26800854784458,
43.1687346471258));
#150853=CARTESIAN_POINT('Ctrl Pts',(6.88085100660889,-1.34840582680821,
43.1650066173867));
#150854=CARTESIAN_POINT('Ctrl Pts',(6.86466574336499,-1.4285185177329,43.1612785876477));
#150855=CARTESIAN_POINT('Ctrl Pts',(6.84709064208999,-1.50830245690437,
43.1575505579087));
#150856=CARTESIAN_POINT('Ctrl Pts',(6.8075382339915,-1.68785458991562,43.1491607027759));
#150857=CARTESIAN_POINT('Ctrl Pts',(6.76088524413027,-1.8660031247024,43.1407708476431));
#150858=CARTESIAN_POINT('Ctrl Pts',(6.70724854843079,-2.04216636738369,
43.1323809925103));
#150859=CARTESIAN_POINT('Ctrl Pts',(6.65366134792218,-2.21816704909422,
43.1239988794182));
#150860=CARTESIAN_POINT('Ctrl Pts',(6.59310338389595,-2.39218577783364,
43.1156167663261));
#150861=CARTESIAN_POINT('Ctrl Pts',(6.52574217979552,-2.56365277784212,
43.1072346532341));
#150862=CARTESIAN_POINT('Ctrl Pts',(6.4584332337127,-2.73498675579992,43.0988590428852));
#150863=CARTESIAN_POINT('Ctrl Pts',(6.38433168979245,-2.90377264688196,
43.0904834325363));
#150864=CARTESIAN_POINT('Ctrl Pts',(6.30365447480766,-3.06945708957421,
43.0821078221875));
#150865=CARTESIAN_POINT('Ctrl Pts',(6.22302800698904,-3.23503731429183,
43.0737374802219));
#150866=CARTESIAN_POINT('Ctrl Pts',(6.13583425884974,-3.39751968566467,
43.0653671382563));
#150867=CARTESIAN_POINT('Ctrl Pts',(6.04233791305133,-3.55637162104898,
43.0569967962907));
#150868=CARTESIAN_POINT('Ctrl Pts',(5.9488866723286,-3.71514692211667,43.0486304923964));
#150869=CARTESIAN_POINT('Ctrl Pts',(5.84913906371482,-3.87029499701398,
43.0402641885021));
#150870=CARTESIAN_POINT('Ctrl Pts',(5.74340548889108,-4.02130823895356,
43.0318978846077));
#150871=CARTESIAN_POINT('Ctrl Pts',(5.63770148478455,-4.17227924672222,
43.0235339205341));
#150872=CARTESIAN_POINT('Ctrl Pts',(5.52601503976411,-4.31911745755718,
43.0151699564605));
#150873=CARTESIAN_POINT('Ctrl Pts',(5.40869992621494,-4.46134415514681,
43.0068059923869));
#150874=CARTESIAN_POINT('Ctrl Pts',(5.29140286551229,-4.60354896641108,
42.9984433153883));
#150875=CARTESIAN_POINT('Ctrl Pts',(5.16847907229621,-4.74114342583738,
42.9900806383898));
#150876=CARTESIAN_POINT('Ctrl Pts',(5.04032291908206,-4.87368150722594,
42.9817179613912));
#150877=CARTESIAN_POINT('Ctrl Pts',(4.91216940436875,-5.00621685989779,
42.9733554565649));
#150878=CARTESIAN_POINT('Ctrl Pts',(4.77878397320084,-5.13369580612759,
42.9649929517386));
#150879=CARTESIAN_POINT('Ctrl Pts',(4.64059849850934,-5.25570852865081,
42.9566304469123));
#150880=CARTESIAN_POINT('Ctrl Pts',(4.50239744966423,-5.37773500258233,
42.9482669995923));
#150881=CARTESIAN_POINT('Ctrl Pts',(4.35939552542613,-5.49429380742749,
42.9399035522723));
#150882=CARTESIAN_POINT('Ctrl Pts',(4.21205868985145,-5.60501455446343,
42.9315401049523));
#150883=CARTESIAN_POINT('Ctrl Pts',(4.06463509820729,-5.71580049698688,
42.9231717329995));
#150884=CARTESIAN_POINT('Ctrl Pts',(3.91287175712499,-5.82074131411516,
42.9148033610467));
#150885=CARTESIAN_POINT('Ctrl Pts',(3.75726554725558,-5.91950860882103,
42.9064349890939));
#150886=CARTESIAN_POINT('Ctrl Pts',(3.60161271369882,-6.01830549678974,
42.8980641097582));
#150887=CARTESIAN_POINT('Ctrl Pts',(3.44211499581521,-6.11092500229065,
42.8896932304224));
#150888=CARTESIAN_POINT('Ctrl Pts',(3.27929564532388,-6.19708372002992,
42.8813223510867));
#150889=CARTESIAN_POINT('Ctrl Pts',(3.11633833975749,-6.28331543911907,
42.8729443791954));
#150890=CARTESIAN_POINT('Ctrl Pts',(2.95005407118001,-6.36307528302324,
42.8645664073041));
#150891=CARTESIAN_POINT('Ctrl Pts',(2.78098897074107,-6.43612670067305,
42.8561884354128));
#150892=CARTESIAN_POINT('Ctrl Pts',(2.67354672270923,-6.48255147144969,
42.8508641660538));
#150893=CARTESIAN_POINT('Ctrl Pts',(2.56498179745355,-6.52626786962235,
42.8455398966948));
#150894=CARTESIAN_POINT('Ctrl Pts',(2.45543802545239,-6.56722549221987,
42.8402156273357));
#150895=CARTESIAN_POINT('Ctrl Pts',(2.2936648075827,-6.62771132617328,42.8323527961471));
#150896=CARTESIAN_POINT('Ctrl Pts',(2.12941952748639,-6.68230366769121,
42.8244899649584));
#150897=CARTESIAN_POINT('Ctrl Pts',(1.96318930648301,-6.73078853548459,
42.8166271337697));
#150898=CARTESIAN_POINT('Ctrl Pts',(1.79708681146244,-6.77923614905696,
42.808770344129));
#150899=CARTESIAN_POINT('Ctrl Pts',(1.62900277219913,-6.82158551511934,
42.8009135544882));
#150900=CARTESIAN_POINT('Ctrl Pts',(1.45944377632387,-6.85767091848607,
42.7930567648474));
#150901=CARTESIAN_POINT('Ctrl Pts',(1.28998040369568,-6.89373597139351,
42.7852044060641));
#150902=CARTESIAN_POINT('Ctrl Pts',(1.11904410086539,-6.92354400959627,
42.7773520472808));
#150903=CARTESIAN_POINT('Ctrl Pts',(0.94715584107491,-6.94697937057666,
42.7694996884974));
#150904=CARTESIAN_POINT('Ctrl Pts',(0.775308166108197,-6.97040919819487,
42.7616491837476));
#150905=CARTESIAN_POINT('Ctrl Pts',(0.602509357826003,-6.98746928346902,
42.7537986789978));
#150906=CARTESIAN_POINT('Ctrl Pts',(0.429289727345191,-6.99809523316852,
42.745948174248));
#150907=CARTESIAN_POINT('Ctrl Pts',(0.256097962443485,-7.00871947348761,
42.738098932397));
#150908=CARTESIAN_POINT('Ctrl Pts',(0.0824858911056665,-7.01291161835322,
42.730249690546));
#150909=CARTESIAN_POINT('Ctrl Pts',(-0.0910123897566303,-7.01065926339391,
42.7224004486949));
#150910=CARTESIAN_POINT('Ctrl Pts',(-0.26456912558573,-7.00840614957212,
42.7145485622807));
#150911=CARTESIAN_POINT('Ctrl Pts',(-0.438011612530421,-6.99970420388659,
42.7066966758665));
#150912=CARTESIAN_POINT('Ctrl Pts',(-0.610806890943731,-6.98459315239447,
42.6988447894522));
#150913=CARTESIAN_POINT('Ctrl Pts',(-0.737688313234154,-6.97349729535931,
42.6930792469846));
#150914=CARTESIAN_POINT('Ctrl Pts',(-0.864220785375445,-6.95894687763085,
42.6873137045169));
#150915=CARTESIAN_POINT('Ctrl Pts',(-0.990195679522643,-6.94097536940989,
42.6815481620493));
#150916=CARTESIAN_POINT('Ctrl Pts',(-1.20116038087808,-6.9108792626387,
42.6718928576882));
#150917=CARTESIAN_POINT('Ctrl Pts',(-1.41045364162706,-6.87120349800956,
42.6622375533272));
#150918=CARTESIAN_POINT('Ctrl Pts',(-1.61730106051943,-6.82216709280436,
42.6525822489661));
#150919=CARTESIAN_POINT('Ctrl Pts',(-1.82529437531023,-6.772859035113,42.6428734560302));
#150920=CARTESIAN_POINT('Ctrl Pts',(-2.03081464088909,-6.71408640131081,
42.6331646630942));
#150921=CARTESIAN_POINT('Ctrl Pts',(-2.23309720955559,-6.64611942528684,
42.6234558701582));
#150922=CARTESIAN_POINT('Ctrl Pts',(-2.43635317912132,-6.57782538640216,
42.6137003576861));
#150923=CARTESIAN_POINT('Ctrl Pts',(-2.63634018328757,-6.50024834100388,
42.603944845214));
#150924=CARTESIAN_POINT('Ctrl Pts',(-2.83230582563868,-6.41370955629839,
42.5941893327419));
#150925=CARTESIAN_POINT('Ctrl Pts',(-3.02846550412476,-6.32708508488216,
42.5844241608115));
#150926=CARTESIAN_POINT('Ctrl Pts',(-3.22059582579476,-6.23148115084333,
42.5746589888812));
#150927=CARTESIAN_POINT('Ctrl Pts',(-3.40796591958496,-6.12726650746052,
42.5648938169509));
#150928=CARTESIAN_POINT('Ctrl Pts',(-3.59508053850253,-6.02319395837999,
42.5551419596109));
#150929=CARTESIAN_POINT('Ctrl Pts',(-3.77744786850087,-5.9105341834902,
42.545390102271));
#150930=CARTESIAN_POINT('Ctrl Pts',(-3.95436414472565,-5.78970040446034,
42.5356382449311));
#150931=CARTESIAN_POINT('Ctrl Pts',(-4.03151245391501,-5.73700812569414,
42.531385728875));
#150932=CARTESIAN_POINT('Ctrl Pts',(-4.1076245081266,-5.6827620741858,42.527133212819));
#150933=CARTESIAN_POINT('Ctrl Pts',(-4.18264341830858,-5.6269992534014,
42.5228806967629));
#150934=CARTESIAN_POINT('Ctrl Pts',(-4.32435489412508,-5.52166272411994,
42.5148476511644));
#150935=CARTESIAN_POINT('Ctrl Pts',(-4.46223254596517,-5.41085938973109,
42.5068146055659));
#150936=CARTESIAN_POINT('Ctrl Pts',(-4.5958243739763,-5.29490555969277,
42.4987815599674));
#150937=CARTESIAN_POINT('Ctrl Pts',(-4.72933032401663,-5.17902626924102,
42.4907536783199));
#150938=CARTESIAN_POINT('Ctrl Pts',(-4.85855565862773,-5.05800331292143,
42.4827257966724));
#150939=CARTESIAN_POINT('Ctrl Pts',(-4.98307962462678,-4.9321946450976,
42.4746979150249));
#150940=CARTESIAN_POINT('Ctrl Pts',(-5.10754736682769,-4.80644278112744,
42.4666736580451));
#150941=CARTESIAN_POINT('Ctrl Pts',(-5.22731770964945,-4.67590976803552,
42.4586494010653));
#150942=CARTESIAN_POINT('Ctrl Pts',(-5.3420051443773,-4.54099191806663,
42.4506251440856));
#150943=CARTESIAN_POINT('Ctrl Pts',(-5.45667871222614,-4.40609038104002,
42.4426018573202));
#150944=CARTESIAN_POINT('Ctrl Pts',(-5.56627035295775,-4.26680533728741,
42.4345785705548));
#150945=CARTESIAN_POINT('Ctrl Pts',(-5.67043330223153,-4.12356796081303,
42.4265552837894));
#150946=CARTESIAN_POINT('Ctrl Pts',(-5.77458771628075,-3.98034232136396,
42.4185326544608));
#150947=CARTESIAN_POINT('Ctrl Pts',(-5.87331411254904,-3.83316529317963,
42.4105100251322));
#150948=CARTESIAN_POINT('Ctrl Pts',(-5.96630789601164,-3.68249869687543,
42.4024873958036));
#150949=CARTESIAN_POINT('Ctrl Pts',(-6.05933663851642,-3.53177546065724,
42.3944617505376));
#150950=CARTESIAN_POINT('Ctrl Pts',(-6.1466282730285,-3.37756034944542,
42.3864361052715));
#150951=CARTESIAN_POINT('Ctrl Pts',(-6.22792298842453,-3.22034187824109,
42.3784104600054));
#150952=CARTESIAN_POINT('Ctrl Pts',(-6.27585930649862,-3.12763628715733,
42.3736780504957));
#150953=CARTESIAN_POINT('Ctrl Pts',(-6.32171136404131,-3.03388689975875,
42.3689456409861));
#150954=CARTESIAN_POINT('Ctrl Pts',(-6.36543360471897,-2.93919743916847,
42.3642132314764));
#150955=CARTESIAN_POINT('Ctrl Pts',(-6.4460896205419,-2.76452032945811,
42.3554831826414));
#150956=CARTESIAN_POINT('Ctrl Pts',(-6.51953573012396,-2.58655576672363,
42.3467531338065));
#150957=CARTESIAN_POINT('Ctrl Pts',(-6.58553315993489,-2.40590514399426,
42.3380230849715));
#150958=CARTESIAN_POINT('Ctrl Pts',(-6.6515496729849,-2.22520228591219,
42.329290511832));
#150959=CARTESIAN_POINT('Ctrl Pts',(-6.71011311316938,-2.04181207485348,
42.3205579386925));
#150960=CARTESIAN_POINT('Ctrl Pts',(-6.76103393682314,-1.85635305575902,
42.311825365553));
#150961=CARTESIAN_POINT('Ctrl Pts',(-6.8126781720589,-1.6682592952607,42.3029687322727));
#150962=CARTESIAN_POINT('Ctrl Pts',(-6.85646090787913,-1.4780377767837,
42.2941120989925));
#150963=CARTESIAN_POINT('Ctrl Pts',(-6.89223749999138,-1.28634707844057,
42.2852554657122));
#150964=CARTESIAN_POINT('Ctrl Pts',(-6.92753540364462,-1.09722118908503,
42.2765173336052));
#150965=CARTESIAN_POINT('Ctrl Pts',(-6.95504004824143,-0.90666546805699,
42.2677792014981));
#150966=CARTESIAN_POINT('Ctrl Pts',(-6.97466431409351,-0.715321094481741,
42.259041069391));
#150967=CARTESIAN_POINT('Ctrl Pts',(-6.99468777828065,-0.520084378847368,
42.2501251855241));
#150968=CARTESIAN_POINT('Ctrl Pts',(-7.00650678902527,-0.324026875597594,
42.2412093016573));
#150969=CARTESIAN_POINT('Ctrl Pts',(-7.01008451422186,-0.127834525723511,
42.2322934177905));
#150970=CARTESIAN_POINT('Ctrl Pts',(-7.01366223941844,0.0683578241506386,
42.2233775339236));
#150971=CARTESIAN_POINT('Ctrl Pts',(-7.00899867963518,0.264684718176251,
42.2144616500568));
#150972=CARTESIAN_POINT('Ctrl Pts',(-6.99611344218405,0.460459842539722,
42.20554576619));
#150973=CARTESIAN_POINT('Ctrl Pts',(-6.98348140290468,0.652387936240791,
42.196805081694));
#150974=CARTESIAN_POINT('Ctrl Pts',(-6.9629464611194,0.843806128503964,
42.188064397198));
#150975=CARTESIAN_POINT('Ctrl Pts',(-6.93457453528062,1.03407087626406,
42.179323712702));
#150976=CARTESIAN_POINT('Ctrl Pts',(-6.90620771402259,1.22430139223555,
42.1705846008004));
#150977=CARTESIAN_POINT('Ctrl Pts',(-6.87000676496269,1.41337860744149,
42.1618454888987));
#150978=CARTESIAN_POINT('Ctrl Pts',(-6.82608918734702,1.60066641399265,
42.1531063769971));
#150979=CARTESIAN_POINT('Ctrl Pts',(-6.78160259430321,1.79038080363917,
42.1442540373226));
#150980=CARTESIAN_POINT('Ctrl Pts',(-6.72919806190732,1.97825881004582,
42.1354016976482));
#150981=CARTESIAN_POINT('Ctrl Pts',(-6.66905099339334,2.16365094458865,
42.1265493579737));
#150982=CARTESIAN_POINT('Ctrl Pts',(-6.60970368322049,2.3465779730233,42.1178147253242));
#150983=CARTESIAN_POINT('Ctrl Pts',(-6.54281855873748,2.52708456395344,
42.1090800926747));
#150984=CARTESIAN_POINT('Ctrl Pts',(-6.46861428810261,2.70456202632788,
42.1003454600252));
#150985=CARTESIAN_POINT('Ctrl Pts',(-6.39291006361437,2.88562699116408,
42.0914342668383));
#150986=CARTESIAN_POINT('Ctrl Pts',(-6.30958773733975,3.06353878623212,
42.0825230736513));
#150987=CARTESIAN_POINT('Ctrl Pts',(-6.21893156113291,3.23767150903932,
42.0736118804644));
#150988=CARTESIAN_POINT('Ctrl Pts',(-6.12827538492605,3.41180423184659,
42.0647006872775));
#150989=CARTESIAN_POINT('Ctrl Pts',(-6.03028548681558,3.58215760729687,
42.0557894940906));
#150990=CARTESIAN_POINT('Ctrl Pts',(-5.92529694581475,3.74813055621311,
42.0468783009037));
#150991=CARTESIAN_POINT('Ctrl Pts',(-5.83074138790573,3.89761034355921,
42.0388526360512));
#150992=CARTESIAN_POINT('Ctrl Pts',(-5.73046512869765,4.04360545455386,
42.0308269711987));
#150993=CARTESIAN_POINT('Ctrl Pts',(-5.62476393450537,4.1856489632538,42.0228013063462));
#150994=CARTESIAN_POINT('Ctrl Pts',(-5.51909628727948,4.32764739082815,
42.0147781886429));
#150995=CARTESIAN_POINT('Ctrl Pts',(-5.40800735147344,4.46569641925513,
42.0067550709396));
#150996=CARTESIAN_POINT('Ctrl Pts',(-5.29183575177128,4.59935875299757,
41.9987319532363));
#150997=CARTESIAN_POINT('Ctrl Pts',(-5.17567880232444,4.73300423075006,
41.9907098473183));
#150998=CARTESIAN_POINT('Ctrl Pts',(-5.05444070656423,4.86226383952261,
41.9826877414003));
#150999=CARTESIAN_POINT('Ctrl Pts',(-4.92849980283099,4.98673402699551,
41.9746656354824));
#151000=CARTESIAN_POINT('Ctrl Pts',(-4.80251209903253,5.1112504680105,41.9666405485228));
#151001=CARTESIAN_POINT('Ctrl Pts',(-4.6718183550072,5.23097367226489,41.9586154615631));
#151002=CARTESIAN_POINT('Ctrl Pts',(-4.53683346105611,5.34553727039123,
41.9505903746035));
#151003=CARTESIAN_POINT('Ctrl Pts',(-4.40182198250564,5.46012343124491,
41.9425637071432));
#151004=CARTESIAN_POINT('Ctrl Pts',(-4.26251795558613,5.56954773113641,
41.9345370396829));
#151005=CARTESIAN_POINT('Ctrl Pts',(-4.11936848024561,5.67348480974956,
41.9265103722225));
#151006=CARTESIAN_POINT('Ctrl Pts',(-3.97610408501076,5.77750532868313,
41.9184772609818));
#151007=CARTESIAN_POINT('Ctrl Pts',(-3.82898837764871,5.87602962039594,
41.9104441497411));
#151008=CARTESIAN_POINT('Ctrl Pts',(-3.67849700871148,5.96877594816565,
41.9024110385005));
#151009=CARTESIAN_POINT('Ctrl Pts',(-3.58982202724712,6.02342545367514,
41.8976776375393));
#151010=CARTESIAN_POINT('Ctrl Pts',(-3.49997551438973,6.07606970805002,
41.8929442365782));
#151011=CARTESIAN_POINT('Ctrl Pts',(-3.40905855336876,6.12665866049377,
41.8882108356171));
#151012=CARTESIAN_POINT('Ctrl Pts',(-3.22176678412568,6.23087347696965,
41.8784598823231));
#151013=CARTESIAN_POINT('Ctrl Pts',(-3.0298210583233,6.32642565517752,41.8687089290291));
#151014=CARTESIAN_POINT('Ctrl Pts',(-2.83396501947201,6.41297659678476,
41.8589579757351));
#151015=CARTESIAN_POINT('Ctrl Pts',(-2.63782681325505,6.49965223125995,
41.8491929743637));
#151016=CARTESIAN_POINT('Ctrl Pts',(-2.43776706058922,6.57730067376265,
41.8394279729922));
#151017=CARTESIAN_POINT('Ctrl Pts',(-2.23455086222943,6.64563082081827,
41.8296629716208));
#151018=CARTESIAN_POINT('Ctrl Pts',(-2.03167338316677,6.71384707567646,
41.8199142464834));
#151019=CARTESIAN_POINT('Ctrl Pts',(-1.82565000922661,6.77277606450171,
41.8101655213459));
#151020=CARTESIAN_POINT('Ctrl Pts',(-1.61725958581747,6.82217692489586,
41.8004167962085));
#151021=CARTESIAN_POINT('Ctrl Pts',(-1.40944111331638,6.87144219908361,
41.7906948275415));
#151022=CARTESIAN_POINT('Ctrl Pts',(-1.19926859966887,6.91123154186169,
41.7809728588745));
#151023=CARTESIAN_POINT('Ctrl Pts',(-0.987531454394643,6.9413549245865,
41.7712508902075));
#151024=CARTESIAN_POINT('Ctrl Pts',(-0.777195318508695,6.97127898875551,
41.7615932492679));
#151025=CARTESIAN_POINT('Ctrl Pts',(-0.565315230214999,6.99166454918276,
41.7519356083283));
#151026=CARTESIAN_POINT('Ctrl Pts',(-0.35268122158664,7.00237406301893,
41.7422779673888));
#151027=CARTESIAN_POINT('Ctrl Pts',(-0.259221254235411,7.00708126305683,
41.7380331017028));
#151028=CARTESIAN_POINT('Ctrl Pts',(-0.16561584406838,7.0099197817077,41.7337882360168));
#151029=CARTESIAN_POINT('Ctrl Pts',(-0.0719330421799695,7.01088098600616,
41.7295433703308));
#151030=CARTESIAN_POINT('Ctrl Pts',(0.101354661761592,7.01265895253302,
41.7216915233168));
#151031=CARTESIAN_POINT('Ctrl Pts',(0.274836025484513,7.00800916941411,
41.7138396763029));
#151032=CARTESIAN_POINT('Ctrl Pts',(0.447977331687376,6.99692381499143,
41.705987829289));
#151033=CARTESIAN_POINT('Ctrl Pts',(0.621069536415629,6.98584160428565,
41.6981382089953));
#151034=CARTESIAN_POINT('Ctrl Pts',(0.793821495145662,6.96832747701359,
41.6902885887017));
#151035=CARTESIAN_POINT('Ctrl Pts',(0.965700916861905,6.94442569991732,
41.6824389684081));
#151036=CARTESIAN_POINT('Ctrl Pts',(1.13756661620472,6.92052583107223,41.6745899748063));
#151037=CARTESIAN_POINT('Ctrl Pts',(1.30855953948441,6.89023938090103,41.6667409812045));
#151038=CARTESIAN_POINT('Ctrl Pts',(1.47815419777677,6.85366228596762,41.6588919876026));
#151039=CARTESIAN_POINT('Ctrl Pts',(1.64783471687858,6.81706667312209,41.6510390202852));
#151040=CARTESIAN_POINT('Ctrl Pts',(1.81611518319584,6.77417413271322,41.6431860529677));
#151041=CARTESIAN_POINT('Ctrl Pts',(1.98248162460617,6.72513146121315,41.6353330856503));
#151042=CARTESIAN_POINT('Ctrl Pts',(2.14889031750256,6.67607633452239,41.627478123943));
#151043=CARTESIAN_POINT('Ctrl Pts',(2.31338365538907,6.62086808640719,41.6196231622357));
#151044=CARTESIAN_POINT('Ctrl Pts',(2.4754650705954,6.55970267975326,41.6117682005284));
#151045=CARTESIAN_POINT('Ctrl Pts',(2.63770736515455,6.49847656132048,41.603905442115));
#151046=CARTESIAN_POINT('Ctrl Pts',(2.79753260403959,6.4312816224051,41.5960426837016));
#151047=CARTESIAN_POINT('Ctrl Pts',(2.95446583453959,6.35836128220458,41.5881799252883));
#151048=CARTESIAN_POINT('Ctrl Pts',(3.06958980057272,6.30486796697987,41.5824119185403));
#151049=CARTESIAN_POINT('Ctrl Pts',(3.18315789977903,6.24829452919848,41.5766439117923));
#151050=CARTESIAN_POINT('Ctrl Pts',(3.29499208989923,6.18875219167818,41.5708759050443));
#151051=CARTESIAN_POINT('Ctrl Pts',(3.45744846422137,6.10225778185758,41.5624969874491));
#151052=CARTESIAN_POINT('Ctrl Pts',(3.61660492633648,6.00930532445614,41.5541180698539));
#151053=CARTESIAN_POINT('Ctrl Pts',(3.7719356013268,5.91017160342604,41.5457391522587));
#151054=CARTESIAN_POINT('Ctrl Pts',(3.93086885978249,5.8087386745655,41.5371659024751));
#151055=CARTESIAN_POINT('Ctrl Pts',(4.0857963892189,5.70083440572801,41.5285926526916));
#151056=CARTESIAN_POINT('Ctrl Pts',(4.23618184298822,5.58680498636179,41.520019402908));
#151057=CARTESIAN_POINT('Ctrl Pts',(4.38295992378626,5.47551084913252,41.5116518040619));
#151058=CARTESIAN_POINT('Ctrl Pts',(4.52541105514494,5.35838225339701,41.5032842052158));
#151059=CARTESIAN_POINT('Ctrl Pts',(4.66306599911358,5.23578475974814,41.4949166063697));
#151060=CARTESIAN_POINT('Ctrl Pts',(4.80067075234893,5.11323196669577,41.486552058456));
#151061=CARTESIAN_POINT('Ctrl Pts',(4.93348255967734,4.98521446964347,41.4781875105422));
#151062=CARTESIAN_POINT('Ctrl Pts',(5.06106576744254,4.85213765881815,41.4698229626285));
#151063=CARTESIAN_POINT('Ctrl Pts',(5.18861947139895,4.71909162220559,41.461460349029));
#151064=CARTESIAN_POINT('Ctrl Pts',(5.31094675979103,4.58098884209341,41.4530977354296));
#151065=CARTESIAN_POINT('Ctrl Pts',(5.42764901555431,4.43827136692343,41.4447351218301));
#151066=CARTESIAN_POINT('Ctrl Pts',(5.54947121660713,4.28929261034159,41.4360056247987));
#151067=CARTESIAN_POINT('Ctrl Pts',(5.66516342534486,4.13528538849491,41.4272761277673));
#151068=CARTESIAN_POINT('Ctrl Pts',(5.77431886242675,3.97679119863272,41.418546630736));
#151069=CARTESIAN_POINT('Ctrl Pts',(5.87889964190271,3.82493943236876,41.4101829831855));
#151070=CARTESIAN_POINT('Ctrl Pts',(5.97748020051843,3.66896942009114,41.4018193356349));
#151071=CARTESIAN_POINT('Ctrl Pts',(6.06974688604635,3.50938731145917,41.3934556880844));
#151072=CARTESIAN_POINT('Ctrl Pts',(6.16202538967972,3.34978476253312,41.3850909692646));
#151073=CARTESIAN_POINT('Ctrl Pts',(6.2479882470465,3.18656948144339,41.3767262504448));
#151074=CARTESIAN_POINT('Ctrl Pts',(6.32736743218011,3.02027282553852,41.368361531625));
#151075=CARTESIAN_POINT('Ctrl Pts',(6.40678194226691,2.85390216507471,41.3599930903772));
#151076=CARTESIAN_POINT('Ctrl Pts',(6.4796067910886,2.68444768954274,41.3516246491294));
#151077=CARTESIAN_POINT('Ctrl Pts',(6.54562151305036,2.51246205352286,41.3432562078816));
#151078=CARTESIAN_POINT('Ctrl Pts',(6.55423329378749,2.49002610979205,41.3421645244056));
#151079=CARTESIAN_POINT('Ctrl Pts',(6.56272924917659,2.46754711609132,41.3410728409296));
#151080=CARTESIAN_POINT('Ctrl Pts',(6.57110895151812,2.44502632087641,41.3399811574536));
#151081=CARTESIAN_POINT('Origin',(0.,0.,50.));
#151082=CARTESIAN_POINT('',(6.57110895151813,2.44502632087639,39.3399667765699));
#151083=CARTESIAN_POINT('',(6.57110895151814,2.44502632087636,39.8869210003223));
#151084=CARTESIAN_POINT('',(6.57110895151814,2.44502632087636,50.));
#151085=CARTESIAN_POINT('',(7.01125,4.02193903181747E-12,41.7735343569105));
#151086=CARTESIAN_POINT('Ctrl Pts',(6.57110895151814,2.44502632087636,39.8869210003223));
#151087=CARTESIAN_POINT('Ctrl Pts',(6.50449838733148,2.62404495591329,39.895592809261));
#151088=CARTESIAN_POINT('Ctrl Pts',(6.43056821795872,2.80033990715965,39.9042646181998));
#151089=CARTESIAN_POINT('Ctrl Pts',(6.34956511459257,2.97332295892139,39.9129364271386));
#151090=CARTESIAN_POINT('Ctrl Pts',(6.26856213015487,3.14630575671006,39.9216082233454));
#151091=CARTESIAN_POINT('Ctrl Pts',(6.18048635294215,3.31597640754793,39.9302800195523));
#151092=CARTESIAN_POINT('Ctrl Pts',(6.08563165071456,3.48176879966508,39.9389518157591));
#151093=CARTESIAN_POINT('Ctrl Pts',(5.99077708581872,3.64756095174606,39.9476235994108));
#151094=CARTESIAN_POINT('Ctrl Pts',(5.88914375658023,3.80947460983865,39.9562953830625));
#151095=CARTESIAN_POINT('Ctrl Pts',(5.78107076500159,3.96696954519996,39.9649671667143));
#151096=CARTESIAN_POINT('Ctrl Pts',(5.67299792768795,4.12446425575064,39.9736389379878));
#151097=CARTESIAN_POINT('Ctrl Pts',(5.55848560711295,4.27754002202605,39.9823107092612));
#151098=CARTESIAN_POINT('Ctrl Pts',(5.43791587524807,4.42568610457464,39.9909824805347));
#151099=CARTESIAN_POINT('Ctrl Pts',(5.31734631302823,4.57383197867747,39.9996542396068));
#151100=CARTESIAN_POINT('Ctrl Pts',(5.19071953583763,4.71704796266914,40.0083259986788));
#151101=CARTESIAN_POINT('Ctrl Pts',(5.05845803451528,4.85485621574396,40.0169977577509));
#151102=CARTESIAN_POINT('Ctrl Pts',(4.9261967165914,4.99266427772899,40.0256695047984));
#151103=CARTESIAN_POINT('Ctrl Pts',(4.78830088681711,5.12506441890963,40.0343412518459));
#151104=CARTESIAN_POINT('Ctrl Pts',(4.6452306340038,5.25161488681459,40.0430129988934));
#151105=CARTESIAN_POINT('Ctrl Pts',(4.49652806262312,5.38314733060955,40.0520261309664));
#151106=CARTESIAN_POINT('Ctrl Pts',(4.34223563523881,5.50835996364327,40.0610392630394));
#151107=CARTESIAN_POINT('Ctrl Pts',(4.1829094334448,5.6268015101031,40.0700523951124));
#151108=CARTESIAN_POINT('Ctrl Pts',(4.0260727035538,5.7433924073995,40.0789246969968));
#151109=CARTESIAN_POINT('Ctrl Pts',(3.86435862820325,5.85342208902676,40.0877969988811));
#151110=CARTESIAN_POINT('Ctrl Pts',(3.69833198496388,5.95650628233473,40.0966693007655));
#151111=CARTESIAN_POINT('Ctrl Pts',(3.53489950802516,6.05797978512224,40.1054029729329));
#151112=CARTESIAN_POINT('Ctrl Pts',(3.36728850947017,6.15272311279945,40.1141366451003));
#151113=CARTESIAN_POINT('Ctrl Pts',(3.19606623000903,6.24041562845744,40.1228703172678));
#151114=CARTESIAN_POINT('Ctrl Pts',(3.02603797481029,6.32749661743996,40.1315430848817));
#151115=CARTESIAN_POINT('Ctrl Pts',(2.85244891335269,6.40762471321637,40.1402158524957));
#151116=CARTESIAN_POINT('Ctrl Pts',(2.67587836095063,6.48053250588994,40.1488886201097));
#151117=CARTESIAN_POINT('Ctrl Pts',(2.49930871513362,6.55343992422525,40.1575613431942));
#151118=CARTESIAN_POINT('Ctrl Pts',(2.31975787164879,6.61912700519455,40.1662340662787));
#151119=CARTESIAN_POINT('Ctrl Pts',(2.13782503579984,6.6773745348608,40.1749067893631));
#151120=CARTESIAN_POINT('Ctrl Pts',(1.95589311921716,6.73562177021519,40.1835794686263));
#151121=CARTESIAN_POINT('Ctrl Pts',(1.77157950496912,6.78642944284926,40.1922521478894));
#151122=CARTESIAN_POINT('Ctrl Pts',(1.58549928668659,6.82962799678111,40.2009248271525));
#151123=CARTESIAN_POINT('Ctrl Pts',(1.39941999343734,6.87282633596633,40.2095974633024));
#151124=CARTESIAN_POINT('Ctrl Pts',(1.211574390505,6.90841556788942,40.2182700994524));
#151125=CARTESIAN_POINT('Ctrl Pts',(1.02258935228956,6.93627692491325,40.2269427356023));
#151126=CARTESIAN_POINT('Ctrl Pts',(0.833605238122552,6.96413814570808,
40.235615329347));
#151127=CARTESIAN_POINT('Ctrl Pts',(0.643481980913932,6.98427152577638,
40.2442879230918));
#151128=CARTESIAN_POINT('Ctrl Pts',(0.452854049805355,6.99660987708154,
40.2529605168366));
#151129=CARTESIAN_POINT('Ctrl Pts',(0.262227035219116,7.00894816906498,
40.2616330688843));
#151130=CARTESIAN_POINT('Ctrl Pts',(0.0710956351193099,7.0134914889309,
40.270305620932));
#151131=CARTESIAN_POINT('Ctrl Pts',(-0.119902323159135,7.01022467510144,
40.2789781729797));
#151132=CARTESIAN_POINT('Ctrl Pts',(-0.310899378724558,7.00695787671191,
40.2876506840384));
#151133=CARTESIAN_POINT('Ctrl Pts',(-0.50176270965486,6.99588102335268,
40.296323195097));
#151134=CARTESIAN_POINT('Ctrl Pts',(-0.691855389207205,6.97703107940082,
40.3049957061557));
#151135=CARTESIAN_POINT('Ctrl Pts',(-0.881947185839328,6.95818122300097,
40.3136681769333));
#151136=CARTESIAN_POINT('Ctrl Pts',(-1.07126805553219,6.93155837629096,
40.3223406477109));
#151137=CARTESIAN_POINT('Ctrl Pts',(-1.25918622472681,6.89725138109075,
40.3310131184885));
#151138=CARTESIAN_POINT('Ctrl Pts',(-1.44710353643705,6.86294454243587,
40.3396855496929));
#151139=CARTESIAN_POINT('Ctrl Pts',(-1.63361788097252,6.82095367647998,
40.3483579808974));
#151140=CARTESIAN_POINT('Ctrl Pts',(-1.81810685596866,6.77141890764261,
40.3570304121019));
#151141=CARTESIAN_POINT('Ctrl Pts',(-2.00259500418376,6.7218843607936,40.3657028044411));
#151142=CARTESIAN_POINT('Ctrl Pts',(-2.18505752664302,6.66480605238623,
40.3743751967804));
#151143=CARTESIAN_POINT('Ctrl Pts',(-2.3648855474509,6.60037445225329,40.3830475891197));
#151144=CARTESIAN_POINT('Ctrl Pts',(-2.54471277704058,6.5359431356104,40.3917199433016));
#151145=CARTESIAN_POINT('Ctrl Pts',(-2.72190526073146,6.46415868780839,
40.4003922974836));
#151146=CARTESIAN_POINT('Ctrl Pts',(-2.89587171390079,6.38526065083715,
40.4090646516655));
#151147=CARTESIAN_POINT('Ctrl Pts',(-3.06983741583811,6.30636295456799,
40.417736968398));
#151148=CARTESIAN_POINT('Ctrl Pts',(-3.24057685640974,6.22035184793663,
40.4264092851305));
#151149=CARTESIAN_POINT('Ctrl Pts',(-3.40752028946972,6.12751434427959,
40.435081601863));
#151150=CARTESIAN_POINT('Ctrl Pts',(-3.5744630152474,6.03467723394335,40.4437538818538));
#151151=CARTESIAN_POINT('Ctrl Pts',(-3.73760951742357,5.93501392252036,
40.4524261618447));
#151152=CARTESIAN_POINT('Ctrl Pts',(-3.89641539159049,5.82885697703047,
40.4610984418355));
#151153=CARTESIAN_POINT('Ctrl Pts',(-4.0552206059092,5.72270047262924,40.4697706857925));
#151154=CARTESIAN_POINT('Ctrl Pts',(-4.20968499214318,5.61005054602416,
40.4784429297495));
#151155=CARTESIAN_POINT('Ctrl Pts',(-4.35929312156135,5.49128309621785,
40.4871151737065));
#151156=CARTESIAN_POINT('Ctrl Pts',(-4.50890064155582,5.37251613020677,
40.4957873823374));
#151157=CARTESIAN_POINT('Ctrl Pts',(-4.65365172183535,5.24763186748207,
40.5044595909682));
#151158=CARTESIAN_POINT('Ctrl Pts',(-4.79306334971184,5.11704702813538,
40.5131317995991));
#151159=CARTESIAN_POINT('Ctrl Pts',(-4.93247442107444,4.98646271006714,
40.5218039736116));
#151160=CARTESIAN_POINT('Ctrl Pts',(-5.06654587536853,4.8501780551058,40.5304761476241));
#151161=CARTESIAN_POINT('Ctrl Pts',(-5.19483033978756,4.70864782111836,
40.5391483216367));
#151162=CARTESIAN_POINT('Ctrl Pts',(-5.32311430257757,4.56711814055468,
40.5478204617385));
#151163=CARTESIAN_POINT('Ctrl Pts',(-5.44561113000732,4.42034313247626,
40.5564926018403));
#151164=CARTESIAN_POINT('Ctrl Pts',(-5.56191207495295,4.26881255538265,
40.5651647419421));
#151165=CARTESIAN_POINT('Ctrl Pts',(-5.67821257461744,4.11728255845381,
40.573836848841));
#151166=CARTESIAN_POINT('Ctrl Pts',(-5.78831706632354,3.96099725427816,
40.5825089557398));
#151167=CARTESIAN_POINT('Ctrl Pts',(-5.89185815647442,3.80047813129952,
40.5911810626386));
#151168=CARTESIAN_POINT('Ctrl Pts',(-5.99539885864498,3.6399596098044,40.5998531370421));
#151169=CARTESIAN_POINT('Ctrl Pts',(-6.09237605450714,3.4752075399488,40.6085252114455));
#151170=CARTESIAN_POINT('Ctrl Pts',(-6.18246615568129,3.30677165772833,
40.6171972858489));
#151171=CARTESIAN_POINT('Ctrl Pts',(-6.27255592662742,3.13833639291476,
40.6258693284646));
#151172=CARTESIAN_POINT('Ctrl Pts',(-6.35575851943906,2.96621759322201,
40.6345413710803));
#151173=CARTESIAN_POINT('Ctrl Pts',(-6.43179631013703,2.79098957135417,
40.643213413696));
#151174=CARTESIAN_POINT('Ctrl Pts',(-6.50783382831937,2.61576217749477,
40.6518854252315));
#151175=CARTESIAN_POINT('Ctrl Pts',(-6.57670648270635,2.43742584431986,
40.6605574367671));
#151176=CARTESIAN_POINT('Ctrl Pts',(-6.63818446599503,2.25657562645756,
40.6692294483026));
#151177=CARTESIAN_POINT('Ctrl Pts',(-6.69966223396491,2.07572604200009,
40.6779014294655));
#151178=CARTESIAN_POINT('Ctrl Pts',(-6.75374529124769,1.89236285939106,
40.6865734106284));
#151179=CARTESIAN_POINT('Ctrl Pts',(-6.80025318023408,1.70709790205962,
40.6952453917913));
#151180=CARTESIAN_POINT('Ctrl Pts',(-6.8467609101265,1.52183357848165,40.7039173432892));
#151181=CARTESIAN_POINT('Ctrl Pts',(-6.88569345442305,1.33466776867736,
40.712589294787));
#151182=CARTESIAN_POINT('Ctrl Pts',(-6.91692090874696,1.14622497994031,
40.7212612462849));
#151183=CARTESIAN_POINT('Ctrl Pts',(-6.94814825879545,0.957782820455669,
40.7299331688251));
#151184=CARTESIAN_POINT('Ctrl Pts',(-6.97167052392514,0.76806397077045,
40.7386050913654));
#151185=CARTESIAN_POINT('Ctrl Pts',(-6.98740921903159,0.577701452562083,
40.7472770139056));
#151186=CARTESIAN_POINT('Ctrl Pts',(-7.00314786286689,0.387339554488134,
40.7559489081958));
#151187=CARTESIAN_POINT('Ctrl Pts',(-7.01110296401747,0.196334275137052,
40.764620802486));
#151188=CARTESIAN_POINT('Ctrl Pts',(-7.01124797942393,0.00532292437845766,
40.7732926967762));
#151189=CARTESIAN_POINT('Ctrl Pts',(-7.0113929943698,-0.185687819713,40.7819645635237));
#151190=CARTESIAN_POINT('Ctrl Pts',(-7.00372797299432,-0.376704351162253,
40.7906364302713));
#151191=CARTESIAN_POINT('Ctrl Pts',(-6.9882784903119,-0.567089326600318,
40.7993082970188));
#151192=CARTESIAN_POINT('Ctrl Pts',(-6.97282905543812,-0.757473712889477,
40.8079801369312));
#151193=CARTESIAN_POINT('Ctrl Pts',(-6.94959523043359,-0.947226264002061,
40.8166519768435));
#151194=CARTESIAN_POINT('Ctrl Pts',(-6.91865453650885,-1.13571385786456,
40.8253238167559));
#151195=CARTESIAN_POINT('Ctrl Pts',(-6.88771393580673,-1.32420088382415,
40.8339956305404));
#151196=CARTESIAN_POINT('Ctrl Pts',(-6.84906655865489,-1.51142267990864,
40.842667444325));
#151197=CARTESIAN_POINT('Ctrl Pts',(-6.80284135383486,-1.69675457183835,
40.8513392581096));
#151198=CARTESIAN_POINT('Ctrl Pts',(-6.75661628451863,-1.88208592048921,
40.8600110464737));
#151199=CARTESIAN_POINT('Ctrl Pts',(-6.70281350071476,-2.06552710051504,
40.8686828348379));
#151200=CARTESIAN_POINT('Ctrl Pts',(-6.64161251687655,-2.24646605542323,
40.877354623202));
#151201=CARTESIAN_POINT('Ctrl Pts',(-6.58041170744998,-2.4274044946884,
40.8860263868531));
#151202=CARTESIAN_POINT('Ctrl Pts',(-6.51181283117372,-2.60584045408377,
40.8946981505043));
#151203=CARTESIAN_POINT('Ctrl Pts',(-6.4360447687633,-2.78117858056159,
40.9033699141554));
#151204=CARTESIAN_POINT('Ctrl Pts',(-6.35684774728359,-2.96445180845089,
40.9124341271008));
#151205=CARTESIAN_POINT('Ctrl Pts',(-6.26981768815781,-3.14433998862013,
40.9214983400461));
#151206=CARTESIAN_POINT('Ctrl Pts',(-6.17527181578228,-3.32018742900233,
40.9305625529915));
#151207=CARTESIAN_POINT('Ctrl Pts',(-6.08368050191848,-3.49053963687257,
40.9393435092823));
#151208=CARTESIAN_POINT('Ctrl Pts',(-5.98503618716738,-3.65709956718416,
40.9481244655732));
#151209=CARTESIAN_POINT('Ctrl Pts',(-5.87967633130231,-3.81929742251417,
40.956905421864));
#151210=CARTESIAN_POINT('Ctrl Pts',(-5.77561495477829,-3.97949631379304,
40.9655781596095));
#151211=CARTESIAN_POINT('Ctrl Pts',(-5.6650027940536,-4.13543980257433,
40.9742508973549));
#151212=CARTESIAN_POINT('Ctrl Pts',(-5.54820899034715,-4.28660746534262,
40.9829236351004));
#151213=CARTESIAN_POINT('Ctrl Pts',(-5.431416363685,-4.43777360464794,40.9915962854423));
#151214=CARTESIAN_POINT('Ctrl Pts',(-5.30844239242835,-4.5841637894042,
41.0002689357843));
#151215=CARTESIAN_POINT('Ctrl Pts',(-5.17969746407253,-4.72528948776481,
41.0089415861262));
#151216=CARTESIAN_POINT('Ctrl Pts',(-5.05095379116967,-4.86641380994168,
41.0176141518969));
#151217=CARTESIAN_POINT('Ctrl Pts',(-4.91643946527104,-5.00227353854703,
41.0262867176677));
#151218=CARTESIAN_POINT('Ctrl Pts',(-4.77660337748089,-5.13241529269974,
41.0349592834385));
#151219=CARTESIAN_POINT('Ctrl Pts',(-4.63676860764683,-5.26255582026552,
41.0436317674703));
#151220=CARTESIAN_POINT('Ctrl Pts',(-4.49161238427127,-5.38697828766097,
41.0523042515021));
#151221=CARTESIAN_POINT('Ctrl Pts',(-4.34161910267748,-5.50526748939286,
41.0609767355338));
#151222=CARTESIAN_POINT('Ctrl Pts',(-4.19162718580667,-5.62355561486328,
41.0696491406585));
#151223=CARTESIAN_POINT('Ctrl Pts',(-4.03679852186487,-5.7357104104133,
41.0783215457832));
#151224=CARTESIAN_POINT('Ctrl Pts',(-3.87764977431715,-5.84135761533551,
41.0869939509078));
#151225=CARTESIAN_POINT('Ctrl Pts',(-3.71850242284401,-5.947003893506,41.095666279957));
#151226=CARTESIAN_POINT('Ctrl Pts',(-3.5550353002858,-6.04614253816382,
41.1043386090061));
#151227=CARTESIAN_POINT('Ctrl Pts',(-3.3877938870953,-6.13844272931334,
41.1130109380552));
#151228=CARTESIAN_POINT('Ctrl Pts',(-3.22055388638152,-6.23074214091986,
41.1216831938602));
#151229=CARTESIAN_POINT('Ctrl Pts',(-3.04953990753726,-6.31620307732892,
41.1303554496651));
#151230=CARTESIAN_POINT('Ctrl Pts',(-2.87532260481408,-6.39454036508843,
41.13902770547));
#151231=CARTESIAN_POINT('Ctrl Pts',(-2.70110671662252,-6.47287701679991,
41.1476998908619));
#151232=CARTESIAN_POINT('Ctrl Pts',(-2.52368781567764,-6.54409001910884,
41.1563720762537));
#151233=CARTESIAN_POINT('Ctrl Pts',(-2.34365791912555,-6.60794174615819,
41.1650442616456));
#151234=CARTESIAN_POINT('Ctrl Pts',(-2.16362942554456,-6.67179297561169,
41.1737163794552));
#151235=CARTESIAN_POINT('Ctrl Pts',(-1.98099024478836,-6.72828294965046,
41.1823884972648));
#151236=CARTESIAN_POINT('Ctrl Pts',(-1.79634980371301,-6.77722317363094,
41.1910606150743));
#151237=CARTESIAN_POINT('Ctrl Pts',(-1.61171074128267,-6.82616303219204,
41.1997326681323));
#151238=CARTESIAN_POINT('Ctrl Pts',(-1.4250707229976,-6.86755318072501,
41.2084047211902));
#151239=CARTESIAN_POINT('Ctrl Pts',(-1.23705251633973,-6.9012555114499,
41.2170767742482));
#151240=CARTESIAN_POINT('Ctrl Pts',(-1.04903565219232,-6.9349576015293,
41.2257487653849));
#151241=CARTESIAN_POINT('Ctrl Pts',(-0.859640898941661,-6.96097193353387,
41.2344207565216));
#151242=CARTESIAN_POINT('Ctrl Pts',(-0.669500206862725,-6.97921170588132,
41.2430927476583));
#151243=CARTESIAN_POINT('Ctrl Pts',(-0.479360810405145,-6.99745135394269,
41.2517646797039));
#151244=CARTESIAN_POINT('Ctrl Pts',(-0.288475768016168,-7.00791652123612,
41.2604366117495));
#151245=CARTESIAN_POINT('Ctrl Pts',(-0.0974819939220911,-7.01057228929001,
41.2691085437952));
#151246=CARTESIAN_POINT('Ctrl Pts',(0.0935105410571396,-7.01322804011401,
41.2777804195797));
#151247=CARTESIAN_POINT('Ctrl Pts',(0.284611522343203,-7.00807448913607,
41.2864522953642));
#151248=CARTESIAN_POINT('Ctrl Pts',(0.475183323465225,-6.99512883166569,
41.2951241711488));
#151249=CARTESIAN_POINT('Ctrl Pts',(0.665753950389368,-6.98218325395928,
41.303795993502));
#151250=CARTESIAN_POINT('Ctrl Pts',(0.855795120321911,-6.96144568508307,
41.3124678158552));
#151251=CARTESIAN_POINT('Ctrl Pts',(1.04467275075863,-6.93298531704218,
41.3211396382085));
#151252=CARTESIAN_POINT('Ctrl Pts',(1.23354927905906,-6.90452511507286,
41.32981140996));
#151253=CARTESIAN_POINT('Ctrl Pts',(1.42126200062351,-6.868342246432,41.3384831817115));
#151254=CARTESIAN_POINT('Ctrl Pts',(1.60718460924195,-6.82455743578408,
41.3471549534631));
#151255=CARTESIAN_POINT('Ctrl Pts',(1.79763389405345,-6.77970659200845,
41.3560378577016));
#151256=CARTESIAN_POINT('Ctrl Pts',(1.9862044843137,-6.72687898191017,41.36492076194));
#151257=CARTESIAN_POINT('Ctrl Pts',(2.17223623427354,-6.66625954377784,
41.3738036661785));
#151258=CARTESIAN_POINT('Ctrl Pts',(2.35386532185533,-6.60707473666791,
41.3824763459349));
#151259=CARTESIAN_POINT('Ctrl Pts',(2.53307410227177,-6.54046283696716,
41.3911490256912));
#151260=CARTESIAN_POINT('Ctrl Pts',(2.70926451773746,-6.46664614274114,
41.3998217054475));
#151261=CARTESIAN_POINT('Ctrl Pts',(2.88545151535656,-6.3928308804553,41.4084942169661));
#151262=CARTESIAN_POINT('Ctrl Pts',(3.05862000313874,-6.31181121311276,
41.4171667284846));
#151263=CARTESIAN_POINT('Ctrl Pts',(3.22819210343704,-6.22385751008221,
41.4258392400031));
#151264=CARTESIAN_POINT('Ctrl Pts',(3.39776113570586,-6.13590539837803,
41.4345115946119));
#151265=CARTESIAN_POINT('Ctrl Pts',(3.56373365850705,-6.04101963284194,
41.4431839492206));
#151266=CARTESIAN_POINT('Ctrl Pts',(3.72555582774893,-5.93951684371936,
41.4518563038294));
#151267=CARTESIAN_POINT('Ctrl Pts',(3.88737528046132,-5.83801575853711,
41.4605285128542));
#151268=CARTESIAN_POINT('Ctrl Pts',(4.04504427838579,-5.72989802299899,
41.469200721879));
#151269=CARTESIAN_POINT('Ctrl Pts',(4.19803670362892,-5.61552440983782,
41.4778729309039));
#151270=CARTESIAN_POINT('Ctrl Pts',(4.35102676029745,-5.50115256736847,
41.4865450056686));
#151271=CARTESIAN_POINT('Ctrl Pts',(4.49934016166134,-5.38052521116207,
41.4952170804334));
#151272=CARTESIAN_POINT('Ctrl Pts',(4.64248202336361,-5.25404484423627,
41.5038891551981));
#151273=CARTESIAN_POINT('Ctrl Pts',(4.78562185584173,-5.12756627033602,
41.5125611070248));
#151274=CARTESIAN_POINT('Ctrl Pts',(4.92359008252101,-4.9952350398253,41.5212330588515));
#151275=CARTESIAN_POINT('Ctrl Pts',(5.05592635131864,-4.85749269608733,
41.5299050106782));
#151276=CARTESIAN_POINT('Ctrl Pts',(5.18826091679979,-4.7197521252481,41.5385768508871));
#151277=CARTESIAN_POINT('Ctrl Pts',(5.31496347269136,-4.57660078535727,
41.547248691096));
#151278=CARTESIAN_POINT('Ctrl Pts',(5.43561126741548,-4.42851631046402,
41.555920531305));
#151279=CARTESIAN_POINT('Ctrl Pts',(5.56176013705297,-4.27367975368019,
41.5649877740385));
#151280=CARTESIAN_POINT('Ctrl Pts',(5.68128895686261,-4.11344992041455,
41.5740550167721));
#151281=CARTESIAN_POINT('Ctrl Pts',(5.79376175353782,-3.94841123817446,
41.5831222595057));
#151282=CARTESIAN_POINT('Ctrl Pts',(5.901338742361,-3.79055649463141,41.5917948158841));
#151283=CARTESIAN_POINT('Ctrl Pts',(6.00246078173993,-3.62830291662058,
41.6004673722625));
#151284=CARTESIAN_POINT('Ctrl Pts',(6.09679041553083,-3.4621919634231,41.6091399286409));
#151285=CARTESIAN_POINT('Ctrl Pts',(6.19111669178522,-3.29608692272168,
41.6178121763314));
#151286=CARTESIAN_POINT('Ctrl Pts',(6.2786509059609,-3.12612502861207,41.6264844240218));
#151287=CARTESIAN_POINT('Ctrl Pts',(6.35910096685908,-2.9528734235981,41.6351566717123));
#151288=CARTESIAN_POINT('Ctrl Pts',(6.43954858436857,-2.77962708049451,
41.6438286560136));
#151289=CARTESIAN_POINT('Ctrl Pts',(6.51291235951801,-2.60309148404341,
41.6525006403149));
#151290=CARTESIAN_POINT('Ctrl Pts',(6.5789475010232,-2.42385567666076,41.6611726246162));
#151291=CARTESIAN_POINT('Ctrl Pts',(6.64498098171,-2.24462437715255,41.6698443908126));
#151292=CARTESIAN_POINT('Ctrl Pts',(6.70368609940776,-2.06269326910285,
41.6785161570089));
#151293=CARTESIAN_POINT('Ctrl Pts',(6.75486698389305,-1.87866936750765,
41.6871879232053));
#151294=CARTESIAN_POINT('Ctrl Pts',(6.80605126222429,-1.69463326313834,
41.6958602644335));
#151295=CARTESIAN_POINT('Ctrl Pts',(6.84971023276557,-1.50850436118244,
41.7045326056617));
#151296=CARTESIAN_POINT('Ctrl Pts',(6.88569820761666,-1.32090376489917,
41.7132049468899));
#151297=CARTESIAN_POINT('Ctrl Pts',(6.92168406448176,-1.13331420939924,
41.7218767777283));
#151298=CARTESIAN_POINT('Ctrl Pts',(6.94999977553745,-0.944253411832044,
41.7305486085667));
#151299=CARTESIAN_POINT('Ctrl Pts',(6.97055086371812,-0.754352184870321,
41.739220439405));
#151300=CARTESIAN_POINT('Ctrl Pts',(6.99110229107982,-0.564447823724469,
41.7478924133658));
#151301=CARTESIAN_POINT('Ctrl Pts',(7.00388880856466,-0.373703287798768,
41.7565643873265));
#151302=CARTESIAN_POINT('Ctrl Pts',(7.00886775178448,-0.182755028646632,
41.7652363612872));
#151303=CARTESIAN_POINT('Ctrl Pts',(7.0104558273189,-0.121850486194127,
41.7680023598283));
#151304=CARTESIAN_POINT('Ctrl Pts',(7.01125000000004,-0.0609252433295258,
41.7707683583694));
#151305=CARTESIAN_POINT('Ctrl Pts',(7.01125,4.02193902006209E-12,41.7735343569105));
#151306=CARTESIAN_POINT('Ctrl Pts',(7.01124998181045,0.000505037549962183,
41.7735343569106));
#151307=CARTESIAN_POINT('Ctrl Pts',(7.01123724491749,0.17732662351218,41.7815445908137));
#151308=CARTESIAN_POINT('Ctrl Pts',(7.00453108467992,0.3541638119717,41.7895548247167));
#151309=CARTESIAN_POINT('Ctrl Pts',(6.99115392043893,0.530465289374704,
41.7975650586198));
#151310=CARTESIAN_POINT('Ctrl Pts',(6.97777149522567,0.70683610263744,41.8055784427883));
#151311=CARTESIAN_POINT('Ctrl Pts',(6.9577128515498,0.882670416907103,41.8135918269568));
#151312=CARTESIAN_POINT('Ctrl Pts',(6.93105236682085,1.05742122679996,41.8216052111253));
#151313=CARTESIAN_POINT('Ctrl Pts',(6.90438587959873,1.23221138108406,41.8296203994727));
#151314=CARTESIAN_POINT('Ctrl Pts',(6.87111465517143,1.40591718309873,41.8376355878201));
#151315=CARTESIAN_POINT('Ctrl Pts',(6.83136423289208,1.5780016730228,41.8456507761675));
#151316=CARTESIAN_POINT('Ctrl Pts',(6.79158278076775,1.75022049498012,41.8536722213051));
#151317=CARTESIAN_POINT('Ctrl Pts',(6.74531212447262,1.92081512213539,41.8616936664427));
#151318=CARTESIAN_POINT('Ctrl Pts',(6.69272786248699,2.08926310482675,41.8697151115803));
#151319=CARTESIAN_POINT('Ctrl Pts',(6.67088204297652,2.15924381935659,41.8730475733488));
#151320=CARTESIAN_POINT('Ctrl Pts',(6.64794711637243,2.2288542540769,41.8763800351172));
#151321=CARTESIAN_POINT('Ctrl Pts',(6.62393811560608,2.29805796339452,41.8797124968857));
#151322=CARTESIAN_POINT('Ctrl Pts',(6.60687208473663,2.3472492084192,41.8820812708286));
#151323=CARTESIAN_POINT('Ctrl Pts',(6.58926087510141,2.39624227854239,41.8844500447716));
#151324=CARTESIAN_POINT('Ctrl Pts',(6.57110895151814,2.44502632087636,41.8868188187145));
#151325=CARTESIAN_POINT('',(7.01124831048998,0.00486735569483713,41.2264656430603));
#151326=CARTESIAN_POINT('Ctrl Pts',(6.57110895151812,2.44502632087641,41.3399811574536));
#151327=CARTESIAN_POINT('Ctrl Pts',(6.63540837522956,2.27221897106586,41.3316044138032));
#151328=CARTESIAN_POINT('Ctrl Pts',(6.69285885618379,2.09694930863153,41.3232276701529));
#151329=CARTESIAN_POINT('Ctrl Pts',(6.74329558569568,1.91978936512241,41.3148509265025));
#151330=CARTESIAN_POINT('Ctrl Pts',(6.79375827707833,1.74253823006299,41.3064698709957));
#151331=CARTESIAN_POINT('Ctrl Pts',(6.83719993386948,1.56339519127442,41.2980888154889));
#151332=CARTESIAN_POINT('Ctrl Pts',(6.87350661199057,1.38294375063556,41.2897077599821));
#151333=CARTESIAN_POINT('Ctrl Pts',(6.90985313126439,1.20229429151141,41.2813175075196));
#151334=CARTESIAN_POINT('Ctrl Pts',(6.93904897149081,1.02033388554537,41.272927255057));
#151335=CARTESIAN_POINT('Ctrl Pts',(6.96103174076659,0.837653667418768,
41.2645370025945));
#151336=CARTESIAN_POINT('Ctrl Pts',(6.97063507313572,0.757848487737961,
41.2608716598869));
#151337=CARTESIAN_POINT('Ctrl Pts',(6.97886250284089,0.677905979988461,
41.2572063171792));
#151338=CARTESIAN_POINT('Ctrl Pts',(6.98571194797921,0.597875524135656,
41.2535409744716));
#151339=CARTESIAN_POINT('Ctrl Pts',(7.00257721922344,0.400817905817786,
41.2445158640109));
#151340=CARTESIAN_POINT('Ctrl Pts',(7.01111079365624,0.202955311596569,
41.2354907535503));
#151341=CARTESIAN_POINT('Ctrl Pts',(7.01124831048953,0.00486735634087431,
41.2264656430897));
#151342=CARTESIAN_POINT('Ctrl Pts',(7.01124831048998,0.00486735569473905,
41.2264656430603));
#151343=CARTESIAN_POINT('Ctrl Pts',(7.01137214962453,-0.173518399805182,
41.2183381870224));
#151344=CARTESIAN_POINT('Ctrl Pts',(7.00468390246701,-0.3521518018721,41.2102107309844));
#151345=CARTESIAN_POINT('Ctrl Pts',(6.99115346725259,-0.530471262013475,
41.2020832749465));
#151346=CARTESIAN_POINT('Ctrl Pts',(6.97763733581708,-0.708602210691984,
41.1939644108964));
#151347=CARTESIAN_POINT('Ctrl Pts',(6.9572934459719,-0.886419525895315,
41.1858455468463));
#151348=CARTESIAN_POINT('Ctrl Pts',(6.93014369785625,-1.0633601880658,41.1777266827962));
#151349=CARTESIAN_POINT('Ctrl Pts',(6.90302301034407,-1.24011145612475,
41.1696165090326));
#151350=CARTESIAN_POINT('Ctrl Pts',(6.86911103699095,-1.41598759104888,
41.161506335269));
#151351=CARTESIAN_POINT('Ctrl Pts',(6.8284815706003,-1.5904295025156,41.1533961615053));
#151352=CARTESIAN_POINT('Ctrl Pts',(6.78787723653177,-1.76476350879184,
41.1452910044825));
#151353=CARTESIAN_POINT('Ctrl Pts',(6.74056376343523,-1.93766471239729,
41.1371858474596));
#151354=CARTESIAN_POINT('Ctrl Pts',(6.6866663154689,-2.10858249733642,41.1290806904367));
#151355=CARTESIAN_POINT('Ctrl Pts',(6.63279534084035,-2.27941633091193,
41.1209795145032));
#151356=CARTESIAN_POINT('Ctrl Pts',(6.57234694147109,-2.44826834774683,
41.1128783385697));
#151357=CARTESIAN_POINT('Ctrl Pts',(6.50549659757984,-2.61460141921807,
41.1047771626363));
#151358=CARTESIAN_POINT('Ctrl Pts',(6.47825517631646,-2.68238191227508,
41.1014759448192));
#151359=CARTESIAN_POINT('Ctrl Pts',(6.44995125512438,-2.74974429710525,
41.0981747270021));
#151360=CARTESIAN_POINT('Ctrl Pts',(6.42059905730838,-2.81665303290817,
41.094873509185));
#151361=CARTESIAN_POINT('Ctrl Pts',(6.34646043726233,-2.9856530298607,41.0865351988832));
#151362=CARTESIAN_POINT('Ctrl Pts',(6.26567581471887,-3.15165466081349,
41.0781968885814));
#151363=CARTESIAN_POINT('Ctrl Pts',(6.17852427623076,-3.31413100684436,
41.0698585782795));
#151364=CARTESIAN_POINT('Ctrl Pts',(6.0913179049518,-3.47670957747911,41.0615150217958));
#151365=CARTESIAN_POINT('Ctrl Pts',(5.99773678244351,-3.63575815040036,
41.053171465312));
#151366=CARTESIAN_POINT('Ctrl Pts',(5.89810470852122,-3.79077662357199,
41.0448279088283));
#151367=CARTESIAN_POINT('Ctrl Pts',(5.79839683495163,-3.94591303412189,
41.0364780046032));
#151368=CARTESIAN_POINT('Ctrl Pts',(5.69262900436411,-4.09701295376923,
41.0281281003781));
#151369=CARTESIAN_POINT('Ctrl Pts',(5.58116711335151,-4.24360698172482,
41.0197781961529));
#151370=CARTESIAN_POINT('Ctrl Pts',(5.46953803775052,-4.39042088987445,
41.0114157676894));
#151371=CARTESIAN_POINT('Ctrl Pts',(5.35219803326611,-4.53271513966923,
41.0030533392258));
#151372=CARTESIAN_POINT('Ctrl Pts',(5.22955288163524,-4.6700538777064,40.9946909107622));
#151373=CARTESIAN_POINT('Ctrl Pts',(5.10680285168081,-4.80751005908653,
40.9863213312823));
#151374=CARTESIAN_POINT('Ctrl Pts',(4.97873885001386,-4.94000203849765,
40.9779517518025));
#151375=CARTESIAN_POINT('Ctrl Pts',(4.84580237287659,-5.06713192304321,
40.9695821723226));
#151376=CARTESIAN_POINT('Ctrl Pts',(4.71266085741989,-5.19445788994659,
40.9611996837861));
#151377=CARTESIAN_POINT('Ctrl Pts',(4.57463209395228,-5.31640501878586,
40.9528171952496));
#151378=CARTESIAN_POINT('Ctrl Pts',(4.4321904714524,-5.43261577762192,40.9444347067131));
#151379=CARTESIAN_POINT('Ctrl Pts',(4.38558123851817,-5.4706418421457,40.9416918191083));
#151380=CARTESIAN_POINT('Ctrl Pts',(4.33849974626909,-5.50805405801666,
40.9389489315035));
#151381=CARTESIAN_POINT('Ctrl Pts',(4.29096325386699,-5.54484092796748,
40.9362060438987));
#151382=CARTESIAN_POINT('Ctrl Pts',(4.14556018154508,-5.65736340578749,
40.9278161887659));
#151383=CARTESIAN_POINT('Ctrl Pts',(3.99560443078829,-5.7642590311646,40.9194263336331));
#151384=CARTESIAN_POINT('Ctrl Pts',(3.84155841605414,-5.86515605065574,
40.9110364785003));
#151385=CARTESIAN_POINT('Ctrl Pts',(3.68765455282264,-5.96595996379188,
40.9026543654082));
#151386=CARTESIAN_POINT('Ctrl Pts',(3.52966822361529,-6.0607761266698,40.894272252316));
#151387=CARTESIAN_POINT('Ctrl Pts',(3.36809309514428,-6.14927438523778,
40.8858901392239));
#151388=CARTESIAN_POINT('Ctrl Pts',(3.20664331472822,-6.23770398791371,
40.8775145288751));
#151389=CARTESIAN_POINT('Ctrl Pts',(3.04161057306857,-6.31982530073939,
40.8691389185262));
#151390=CARTESIAN_POINT('Ctrl Pts',(2.87351595328109,-6.39535242412325,
40.8607633081773));
#151391=CARTESIAN_POINT('Ctrl Pts',(2.70552706750532,-6.47083203982508,
40.8523929662117));
#151392=CARTESIAN_POINT('Ctrl Pts',(2.53448044288411,-6.5397256021328,40.8440226242461));
#151393=CARTESIAN_POINT('Ctrl Pts',(2.36092051771228,-6.60179376166396,
40.8356522822805));
#151394=CARTESIAN_POINT('Ctrl Pts',(2.18744432237532,-6.66383197789604,
40.8272859783861));
#151395=CARTESIAN_POINT('Ctrl Pts',(2.01145755334718,-6.71905124713815,
40.8189196744918));
#151396=CARTESIAN_POINT('Ctrl Pts',(1.83352375126998,-6.7672606877546,40.8105533705975));
#151397=CARTESIAN_POINT('Ctrl Pts',(1.65563971228979,-6.8154566455418,40.8021894065239));
#151398=CARTESIAN_POINT('Ctrl Pts',(1.47581004260668,-6.85664659655255,
40.7938254424502));
#151399=CARTESIAN_POINT('Ctrl Pts',(1.29461307415031,-6.89068962809522,
40.7854614783766));
#151400=CARTESIAN_POINT('Ctrl Pts',(1.11344398889634,-6.92472742098106,
40.7770988013781));
#151401=CARTESIAN_POINT('Ctrl Pts',(0.930908347286462,-6.95162042649606,
40.7687361243795));
#151402=CARTESIAN_POINT('Ctrl Pts',(0.74759471092878,-6.97127884327484,
40.760373447381));
#151403=CARTESIAN_POINT('Ctrl Pts',(0.564284848663807,-6.99093685532274,
40.7520109425547));
#151404=CARTESIAN_POINT('Ctrl Pts',(0.380197350407759,-7.00336054099146,
40.7436484377284));
#151405=CARTESIAN_POINT('Ctrl Pts',(0.195926373028393,-7.00851192614038,
40.735285932902));
#151406=CARTESIAN_POINT('Ctrl Pts',(0.0116346274421183,-7.01366389187466,
40.7269224855821));
#151407=CARTESIAN_POINT('Ctrl Pts',(-0.172840309972789,-7.01154191435022,
40.7185590382621));
#151408=CARTESIAN_POINT('Ctrl Pts',(-0.356903367504056,-7.00216013447024,
40.7101955909421));
#151409=CARTESIAN_POINT('Ctrl Pts',(-0.541074806536332,-6.99277283033461,
40.7018272189893));
#151410=CARTESIAN_POINT('Ctrl Pts',(-0.724833552436218,-6.97611719761188,
40.6934588470365));
#151411=CARTESIAN_POINT('Ctrl Pts',(-0.907587698239172,-6.95225942643864,
40.6850904750837));
#151412=CARTESIAN_POINT('Ctrl Pts',(-1.09039660196088,-6.92839450685358,
40.6767195957479));
#151413=CARTESIAN_POINT('Ctrl Pts',(-1.27219998011878,-6.89732319371964,
40.6683487164122));
#151414=CARTESIAN_POINT('Ctrl Pts',(-1.45241450265757,-6.85916311768207,
40.6599778370764));
#151415=CARTESIAN_POINT('Ctrl Pts',(-1.63278171901212,-6.82097070902481,
40.6515998651851));
#151416=CARTESIAN_POINT('Ctrl Pts',(-1.81155706909424,-6.77567760934077,
40.6432218932938));
#151417=CARTESIAN_POINT('Ctrl Pts',(-1.98816967393339,-6.72345208283302,
40.6348439214025));
#151418=CARTESIAN_POINT('Ctrl Pts',(-2.10040842246875,-6.6902623354638,
40.6295196520436));
#151419=CARTESIAN_POINT('Ctrl Pts',(-2.21177399737371,-6.65427379297501,
40.6241953826847));
#151420=CARTESIAN_POINT('Ctrl Pts',(-2.32212367178371,-6.61553990354844,
40.6188711133258));
#151421=CARTESIAN_POINT('Ctrl Pts',(-2.48508703881005,-6.55833805793604,
40.6110082821365));
#151422=CARTESIAN_POINT('Ctrl Pts',(-2.64617268895314,-6.49502732338543,
40.6031454509472));
#151423=CARTESIAN_POINT('Ctrl Pts',(-2.8048695116593,-6.42575548749438,
40.5952826197578));
#151424=CARTESIAN_POINT('Ctrl Pts',(-2.96344439680532,-6.35653687786528,
40.5874258301164));
#151425=CARTESIAN_POINT('Ctrl Pts',(-3.11963375749355,-6.28136642706268,
40.5795690404749));
#151426=CARTESIAN_POINT('Ctrl Pts',(-3.27294245944832,-6.20044145360961,
40.5717122508334));
#151427=CARTESIAN_POINT('Ctrl Pts',(-3.42616470255202,-6.119562118011,40.5638598920495));
#151428=CARTESIAN_POINT('Ctrl Pts',(-3.57650918240588,-6.03293489279218,
40.5560075332654));
#151429=CARTESIAN_POINT('Ctrl Pts',(-3.72350178664801,-5.94080474408384,
40.5481551744814));
#151430=CARTESIAN_POINT('Ctrl Pts',(-3.87045968422133,-5.84869634837849,
40.540304669731));
#151431=CARTESIAN_POINT('Ctrl Pts',(-4.01406695407394,-5.75108781031097,
40.5324541649805));
#151432=CARTESIAN_POINT('Ctrl Pts',(-4.15387516093496,-5.6482694438091,
40.52460366023));
#151433=CARTESIAN_POINT('Ctrl Pts',(-4.29366087706154,-5.54546761754209,
40.5167544183783));
#151434=CARTESIAN_POINT('Ctrl Pts',(-4.42964844123719,-5.43745785970932,
40.5089051765267));
#151435=CARTESIAN_POINT('Ctrl Pts',(-4.5614198192569,-5.3245728274661,40.501055934675));
#151436=CARTESIAN_POINT('Ctrl Pts',(-4.69323559363341,-5.21164976204569,
40.4932040482601));
#151437=CARTESIAN_POINT('Ctrl Pts',(-4.82083205446145,-5.09384838970508,
40.4853521618452));
#151438=CARTESIAN_POINT('Ctrl Pts',(-4.94382543929532,-4.97154066545537,
40.4775002754303));
#151439=CARTESIAN_POINT('Ctrl Pts',(-5.03413795090556,-4.8817316258778,
40.4717347329666));
#151440=CARTESIAN_POINT('Ctrl Pts',(-5.12196929038965,-4.78949368930015,
40.4659691905029));
#151441=CARTESIAN_POINT('Ctrl Pts',(-5.2071807138275,-4.69498621681076,
40.4602036480393));
#151442=CARTESIAN_POINT('Ctrl Pts',(-5.34988059565206,-4.5367186440878,
40.4505483436795));
#151443=CARTESIAN_POINT('Ctrl Pts',(-5.48515969510513,-4.3721665230661,
40.4408930393198));
#151444=CARTESIAN_POINT('Ctrl Pts',(-5.6125637345342,-4.20199415614675,
40.4312377349601));
#151445=CARTESIAN_POINT('Ctrl Pts',(-5.74067356843957,-4.03087906624053,
40.4215289420256));
#151446=CARTESIAN_POINT('Ctrl Pts',(-5.86082086345623,-3.85408135829778,
40.4118201490911));
#151447=CARTESIAN_POINT('Ctrl Pts',(-5.97259164393436,-3.67229841071031,
40.4021113561567));
#151448=CARTESIAN_POINT('Ctrl Pts',(-6.08490027489926,-3.4896407081428,
40.3923558436861));
#151449=CARTESIAN_POINT('Ctrl Pts',(-6.18875157813822,-3.30194972112196,
40.3826003312156));
#151450=CARTESIAN_POINT('Ctrl Pts',(-6.28377368037099,-3.10995416306685,
40.3728448187451));
#151451=CARTESIAN_POINT('Ctrl Pts',(-6.3788898691041,-2.9177684998708,40.3630796468164));
#151452=CARTESIAN_POINT('Ctrl Pts',(-6.46515936331029,-2.7212697796119,
40.3533144748877));
#151453=CARTESIAN_POINT('Ctrl Pts',(-6.54225724021333,-2.52120938546885,
40.3435493029589));
#151454=CARTESIAN_POINT('Ctrl Pts',(-6.61924999591036,-2.3214217691344,
40.3337974456206));
#151455=CARTESIAN_POINT('Ctrl Pts',(-6.68709611428237,-2.11808222026033,
40.3240455882822));
#151456=CARTESIAN_POINT('Ctrl Pts',(-6.74551997477061,-1.91195889926293,
40.3142937309439));
#151457=CARTESIAN_POINT('Ctrl Pts',(-6.77099700920683,-1.82207420312553,
40.3100412148802));
#151458=CARTESIAN_POINT('Ctrl Pts',(-6.79468293255453,-1.73166039905347,
40.3057886988166));
#151459=CARTESIAN_POINT('Ctrl Pts',(-6.81655777172292,-1.6407823460971,
40.301536182753));
#151460=CARTESIAN_POINT('Ctrl Pts',(-6.85787956284112,-1.46911279037676,
40.293503137154));
#151461=CARTESIAN_POINT('Ctrl Pts',(-6.89275525666553,-1.29570197245542,
40.2854700915551));
#151462=CARTESIAN_POINT('Ctrl Pts',(-6.92104045229321,-1.12108234319386,
40.2774370459562));
#151463=CARTESIAN_POINT('Ctrl Pts',(-6.94930746510802,-0.946574966153722,
40.2694091643083));
#151464=CARTESIAN_POINT('Ctrl Pts',(-6.97099235446394,-0.770860684894565,
40.2613812826604));
#151465=CARTESIAN_POINT('Ctrl Pts',(-6.98600139184853,-0.594483906923033,
40.2533534010125));
#151466=CARTESIAN_POINT('Ctrl Pts',(-7.00100365250474,-0.418186764805898,
40.2453291440324));
#151467=CARTESIAN_POINT('Ctrl Pts',(-7.00933603181675,-0.241228086057471,
40.2373048870522));
#151468=CARTESIAN_POINT('Ctrl Pts',(-7.01095643732055,-0.0641591497259766,
40.229280630072));
#151469=CARTESIAN_POINT('Ctrl Pts',(-7.01257664690082,0.112888377167703,
40.2212573433063));
#151470=CARTESIAN_POINT('Ctrl Pts',(-7.00748648807207,0.290045768821117,
40.2132340565405));
#151471=CARTESIAN_POINT('Ctrl Pts',(-6.995695951825,0.466759801310355,40.2052107697747));
#151472=CARTESIAN_POINT('Ctrl Pts',(-6.98390638170722,0.643459353660757,
40.1971881404457));
#151473=CARTESIAN_POINT('Ctrl Pts',(-6.96541755621622,0.819715253647495,
40.1891655111167));
#151474=CARTESIAN_POINT('Ctrl Pts',(-6.94029147898427,0.994977763187888,
40.1811428817878));
#151475=CARTESIAN_POINT('Ctrl Pts',(-6.91515595613599,1.17030615895504,
40.1731172365213));
#151476=CARTESIAN_POINT('Ctrl Pts',(-6.88337825212799,1.3446400555813,40.1650915912548));
#151477=CARTESIAN_POINT('Ctrl Pts',(-6.84507185866578,1.51743791049314,
40.1570659459883));
#151478=CARTESIAN_POINT('Ctrl Pts',(-6.8224840748064,1.61933005552018,40.152333536481));
#151479=CARTESIAN_POINT('Ctrl Pts',(-6.79762723464555,1.72068831273158,
40.1476011269737));
#151480=CARTESIAN_POINT('Ctrl Pts',(-6.7705328119863,1.82140385535907,40.1428687174664));
#151481=CARTESIAN_POINT('Ctrl Pts',(-6.7205507399375,2.00719749899378,40.1341386686318));
#151482=CARTESIAN_POINT('Ctrl Pts',(-6.66292661929775,2.1908961035576,40.1254086197973));
#151483=CARTESIAN_POINT('Ctrl Pts',(-6.59786241262099,2.37188493536746,
40.1166785709627));
#151484=CARTESIAN_POINT('Ctrl Pts',(-6.53277939254755,2.55292610032427,
40.1079459978237));
#151485=CARTESIAN_POINT('Ctrl Pts',(-6.46025208497953,2.73125567076011,
40.0992134246846));
#151486=CARTESIAN_POINT('Ctrl Pts',(-6.38053124061272,2.9062772837541,40.0904808515455));
#151487=CARTESIAN_POINT('Ctrl Pts',(-6.29967783439212,3.08378535815026,
40.081624218265));
#151488=CARTESIAN_POINT('Ctrl Pts',(-6.21142506240932,3.25789050536534,
40.0727675849846));
#151489=CARTESIAN_POINT('Ctrl Pts',(-6.11608379789225,3.42799439026086,
40.0639109517041));
#151490=CARTESIAN_POINT('Ctrl Pts',(-6.02201819325634,3.59582229630618,
40.0551728195975));
#151491=CARTESIAN_POINT('Ctrl Pts',(-5.92105276121328,3.75975511736256,
40.0464346874909));
#151492=CARTESIAN_POINT('Ctrl Pts',(-5.81353139612541,3.9192447319304,40.0376965553842));
#151493=CARTESIAN_POINT('Ctrl Pts',(-5.70382282309353,4.0819786966019,40.0287806715169));
#151494=CARTESIAN_POINT('Ctrl Pts',(-5.58728889987423,4.24008650266873,
40.0198647876495));
#151495=CARTESIAN_POINT('Ctrl Pts',(-5.46434081005095,4.39301787773641,
40.0109489037822));
#151496=CARTESIAN_POINT('Ctrl Pts',(-5.34139272022769,4.54594925280407,
40.0020330199148));
#151497=CARTESIAN_POINT('Ctrl Pts',(-5.21203065802288,4.69370396499372,
39.9931171360474));
#151498=CARTESIAN_POINT('Ctrl Pts',(-5.07670938084948,4.8357676148565,39.9842012521801));
#151499=CARTESIAN_POINT('Ctrl Pts',(-4.94404720096804,4.97503967810018,
39.9754605676838));
#151500=CARTESIAN_POINT('Ctrl Pts',(-4.80564374229953,5.10885705662395,
39.9667198831874));
#151501=CARTESIAN_POINT('Ctrl Pts',(-4.66196191853821,5.23676786124796,
39.9579791986911));
#151502=CARTESIAN_POINT('Ctrl Pts',(-4.5183059455227,5.36465565259437,39.9492400867891));
#151503=CARTESIAN_POINT('Ctrl Pts',(-4.36937370839542,5.48663881032757,
39.940500974887));
#151504=CARTESIAN_POINT('Ctrl Pts',(-4.2156629617881,5.602304200515,39.9317618629849));
#151505=CARTESIAN_POINT('Ctrl Pts',(-4.05996067123436,5.71946820230066,
39.9229095233107));
#151506=CARTESIAN_POINT('Ctrl Pts',(-3.89935539730565,5.83014939443262,
39.9140571836364));
#151507=CARTESIAN_POINT('Ctrl Pts',(-3.73439792679716,5.93396146657805,
39.9052048439621));
#151508=CARTESIAN_POINT('Ctrl Pts',(-3.57163384851286,6.03639317934285,
39.8964702113122));
#151509=CARTESIAN_POINT('Ctrl Pts',(-3.40463283988954,6.13213717324393,
39.8877355786624));
#151510=CARTESIAN_POINT('Ctrl Pts',(-3.23395276923682,6.22086618155748,
39.8790009460125));
#151511=CARTESIAN_POINT('Ctrl Pts',(-3.05982259758143,6.31138874455716,
39.870089752826));
#151512=CARTESIAN_POINT('Ctrl Pts',(-2.88186329143038,6.39460954863071,
39.8611785596395));
#151513=CARTESIAN_POINT('Ctrl Pts',(-2.70069410207354,6.47023012956457,
39.852267366453));
#151514=CARTESIAN_POINT('Ctrl Pts',(-2.5195249127167,6.54585071049844,39.8433561732665));
#151515=CARTESIAN_POINT('Ctrl Pts',(-2.33514611470285,6.61387093909444,
39.8344449800801));
#151516=CARTESIAN_POINT('Ctrl Pts',(-2.14820008149872,6.67404397440929,
39.8255337868936));
#151517=CARTESIAN_POINT('Ctrl Pts',(-1.97983135953655,6.72823745944292,
39.8175081220413));
#151518=CARTESIAN_POINT('Ctrl Pts',(-1.80930274092191,6.77609026319815,
39.8094824571889));
#151519=CARTESIAN_POINT('Ctrl Pts',(-1.6371404659451,6.81743336287675,39.8014567923366));
#151520=CARTESIAN_POINT('Ctrl Pts',(-1.46503283105088,6.85876334126976,
39.7934336746334));
#151521=CARTESIAN_POINT('Ctrl Pts',(-1.29129292805766,6.89358764334553,
39.7854105569303));
#151522=CARTESIAN_POINT('Ctrl Pts',(-1.11646092111208,6.92178745513972,
39.7773874392271));
#151523=CARTESIAN_POINT('Ctrl Pts',(-0.941650962013093,6.94998371069078,
39.7693653333093));
#151524=CARTESIAN_POINT('Ctrl Pts',(-0.765749535176425,6.97155708222192,
39.7613432273915));
#151525=CARTESIAN_POINT('Ctrl Pts',(-0.589305679083936,6.98644010774439,
39.7533211214737));
#151526=CARTESIAN_POINT('Ctrl Pts',(-0.412796255858879,7.00132866384939,
39.7452960345142));
#151527=CARTESIAN_POINT('Ctrl Pts',(-0.235744366070753,7.00952187356422,
39.7372709475548));
#151528=CARTESIAN_POINT('Ctrl Pts',(-0.058703291197909,7.01100424233951,
39.7292458605953));
#151529=CARTESIAN_POINT('Ctrl Pts',(0.118372651028557,7.0124869030599,39.7212191931352));
#151530=CARTESIAN_POINT('Ctrl Pts',(0.295437407472944,7.00725609560299,
39.713192525675));
#151531=CARTESIAN_POINT('Ctrl Pts',(0.471939239027446,6.99534844858826,
39.7051658582148));
#151532=CARTESIAN_POINT('Ctrl Pts',(0.648582765630539,6.98343124215647,
39.6971327469743));
#151533=CARTESIAN_POINT('Ctrl Pts',(0.824662099716163,6.9648265245611,39.6890996357338));
#151534=CARTESIAN_POINT('Ctrl Pts',(0.999631529077732,6.93962271082324,
39.6810665244933));
#151535=CARTESIAN_POINT('Ctrl Pts',(1.10272987297771,6.92477170818914,39.6763331235313));
#151536=CARTESIAN_POINT('Ctrl Pts',(1.20544302501413,6.90763047736772,39.6715997225693));
#151537=CARTESIAN_POINT('Ctrl Pts',(1.30766130588529,6.88822534994249,39.6668663216073));
#151538=CARTESIAN_POINT('Ctrl Pts',(1.51823414570626,6.84825018352223,39.6571153683131));
#151539=CARTESIAN_POINT('Ctrl Pts',(1.72683044092951,6.79864205883999,39.647364415019));
#151540=CARTESIAN_POINT('Ctrl Pts',(1.93266228092448,6.73961742759868,39.6376134617249));
#151541=CARTESIAN_POINT('Ctrl Pts',(2.13879066030014,6.68050776030271,39.6278484603532));
#151542=CARTESIAN_POINT('Ctrl Pts',(2.34214658070593,6.61195446061618,39.6180834589815));
#151543=CARTESIAN_POINT('Ctrl Pts',(2.54195608500686,6.53422419453118,39.6083184576098));
#151544=CARTESIAN_POINT('Ctrl Pts',(2.74143254826272,6.45662348869478,39.5985697324722));
#151545=CARTESIAN_POINT('Ctrl Pts',(2.9373743740537,6.36987640089905,39.5888210073346));
#151546=CARTESIAN_POINT('Ctrl Pts',(3.12902924000294,6.27429697876237,39.579072282197));
#151547=CARTESIAN_POINT('Ctrl Pts',(3.32015808765932,6.17897988507854,39.5693503135299));
#151548=CARTESIAN_POINT('Ctrl Pts',(3.50702342871833,6.07487886873456,39.5596283448627));
#151549=CARTESIAN_POINT('Ctrl Pts',(3.68889739733891,5.96235377635429,39.5499063761955));
#151550=CARTESIAN_POINT('Ctrl Pts',(3.86956795341381,5.85057323311923,39.5402487352557));
#151551=CARTESIAN_POINT('Ctrl Pts',(4.04531291705903,5.73047972519665,39.5305910943159));
#151552=CARTESIAN_POINT('Ctrl Pts',(4.21543757065316,5.6024737973886,39.520933453376));
#151553=CARTESIAN_POINT('Ctrl Pts',(4.29021321293793,5.54621078514499,39.5166885876909));
#151554=CARTESIAN_POINT('Ctrl Pts',(4.36390331476689,5.48841979199353,39.5124437220058));
#151555=CARTESIAN_POINT('Ctrl Pts',(4.43645009465356,5.42913778791333,39.5081988563207));
#151556=CARTESIAN_POINT('Ctrl Pts',(4.57064190642958,5.3194822036729,39.5003470093067));
#151557=CARTESIAN_POINT('Ctrl Pts',(4.70086432803269,5.20476723100338,39.4924951622927));
#151558=CARTESIAN_POINT('Ctrl Pts',(4.82670255274817,5.08532880252539,39.4846433152787));
#151559=CARTESIAN_POINT('Ctrl Pts',(4.95250509075984,4.9659242458207,39.476793694985));
#151560=CARTESIAN_POINT('Ctrl Pts',(5.07392562865895,4.84179916021885,39.4689440746914));
#151561=CARTESIAN_POINT('Ctrl Pts',(5.19058382647801,4.71332855875812,39.4610944543978));
#151562=CARTESIAN_POINT('Ctrl Pts',(5.30723271063323,4.58486821403047,39.4532454607958));
#151563=CARTESIAN_POINT('Ctrl Pts',(5.41911975572065,4.45206332700402,39.4453964671939));
#151564=CARTESIAN_POINT('Ctrl Pts',(5.52590294796685,4.31532422561171,39.437547473592));
#151565=CARTESIAN_POINT('Ctrl Pts',(5.63274020141575,4.17851589721728,39.4296945062745));
#151566=CARTESIAN_POINT('Ctrl Pts',(5.73446820410757,4.03776967582786,39.4218415389569));
#151567=CARTESIAN_POINT('Ctrl Pts',(5.83078636959375,3.893527561821,39.4139885716394));
#151568=CARTESIAN_POINT('Ctrl Pts',(5.92712899665755,3.74924881516388,39.4061336099321));
#151569=CARTESIAN_POINT('Ctrl Pts',(6.0180588494187,3.60147273203062,39.3982786482248));
#151570=CARTESIAN_POINT('Ctrl Pts',(6.10332020439736,3.45066791289671,39.3904236865174));
#151571=CARTESIAN_POINT('Ctrl Pts',(6.18866618839779,3.29971340737413,39.382560928104));
#151572=CARTESIAN_POINT('Ctrl Pts',(6.26833226194025,3.14572450021766,39.3746981696906));
#151573=CARTESIAN_POINT('Ctrl Pts',(6.34210970178402,2.98919238140289,39.3668354112771));
#151574=CARTESIAN_POINT('Ctrl Pts',(6.39623177300444,2.87436266515472,39.3610674045295));
#151575=CARTESIAN_POINT('Ctrl Pts',(6.44718587698939,2.75816478950835,39.3552993977819));
#151576=CARTESIAN_POINT('Ctrl Pts',(6.49490656785073,2.64079821974142,39.3495313910343));
#151577=CARTESIAN_POINT('Ctrl Pts',(6.5212836758092,2.57592508765594,39.3463431862128));
#151578=CARTESIAN_POINT('Ctrl Pts',(6.54668794650828,2.5106587777768,39.3431549813914));
#151579=CARTESIAN_POINT('Ctrl Pts',(6.57110895151813,2.44502632087639,39.3399667765699));
#151580=CARTESIAN_POINT('Origin',(0.,0.,50.));
#151581=CARTESIAN_POINT('',(6.57110895151815,2.44502632087632,37.3396717263878));
#151582=CARTESIAN_POINT('',(6.57110895151815,2.44502632087634,37.8869079341164));
#151583=CARTESIAN_POINT('',(6.57110895151814,2.44502632087636,50.));
#151584=CARTESIAN_POINT('',(7.01124859079596,-0.00444528532742304,39.7735343569106));
#151585=CARTESIAN_POINT('Ctrl Pts',(6.57110895151815,2.44502632087634,37.8869079341164));
#151586=CARTESIAN_POINT('Ctrl Pts',(6.50741728312095,2.61620030324556,37.8951906864515));
#151587=CARTESIAN_POINT('Ctrl Pts',(6.43702403551672,2.78490829906528,37.9034734387866));
#151588=CARTESIAN_POINT('Ctrl Pts',(6.36015189142897,2.9506091710785,37.9117561911217));
#151589=CARTESIAN_POINT('Ctrl Pts',(6.28327867586599,3.11631235269791,37.9200390589052));
#151590=CARTESIAN_POINT('Ctrl Pts',(6.1999265260549,3.27900801963681,37.9283219266887));
#151591=CARTESIAN_POINT('Ctrl Pts',(6.11036541085665,3.4381770036324,37.9366047944722));
#151592=CARTESIAN_POINT('Ctrl Pts',(6.02078937949257,3.59737249679946,37.9448890417453));
#151593=CARTESIAN_POINT('Ctrl Pts',(5.92500248757278,3.75303984112838,37.9531732890184));
#151594=CARTESIAN_POINT('Ctrl Pts',(5.8233197606272,3.90468609852173,37.9614575362915));
#151595=CARTESIAN_POINT('Ctrl Pts',(5.72160457869351,4.05638075821139,37.9697444277222));
#151596=CARTESIAN_POINT('Ctrl Pts',(5.6139899992133,4.204051491555,37.9780313191528));
#151597=CARTESIAN_POINT('Ctrl Pts',(5.50083348302282,4.34723562215749,37.9863182105834));
#151598=CARTESIAN_POINT('Ctrl Pts',(5.38757363012207,4.49055051126615,37.9946126697629));
#151599=CARTESIAN_POINT('Ctrl Pts',(5.26876193959305,4.62937034612297,38.0029071289424));
#151600=CARTESIAN_POINT('Ctrl Pts',(5.14479585166997,4.76326591816366,38.0112015881219));
#151601=CARTESIAN_POINT('Ctrl Pts',(5.02076609707923,4.89723025646961,38.0195003071808));
#151602=CARTESIAN_POINT('Ctrl Pts',(4.89157690281415,5.02626504698509,38.0277990262396));
#151603=CARTESIAN_POINT('Ctrl Pts',(4.75766173974975,5.14997877011366,38.0360977452985));
#151604=CARTESIAN_POINT('Ctrl Pts',(4.62359552391064,5.27383203906154,38.0444058250937));
#151605=CARTESIAN_POINT('Ctrl Pts',(4.48479294459382,5.39235202756019,38.0527139048889));
#151606=CARTESIAN_POINT('Ctrl Pts',(4.34172048039621,5.50518753836852,38.0610219846842));
#151607=CARTESIAN_POINT('Ctrl Pts',(4.28046381981624,5.55349820824982,38.0645790997932));
#151608=CARTESIAN_POINT('Ctrl Pts',(4.21842480052611,5.60076737341295,38.0681362149023));
#151609=CARTESIAN_POINT('Ctrl Pts',(4.15564160387849,5.64696993285906,38.0716933300113));
#151610=CARTESIAN_POINT('Ctrl Pts',(4.00771138083173,5.75583273834117,38.0800746304163));
#151611=CARTESIAN_POINT('Ctrl Pts',(3.85532845952342,5.85900610843247,38.0884559308212));
#151612=CARTESIAN_POINT('Ctrl Pts',(3.69895524447288,5.95611926189247,38.0968372312262));
#151613=CARTESIAN_POINT('Ctrl Pts',(3.54278020958101,6.05310933864683,38.1052079095598));
#151614=CARTESIAN_POINT('Ctrl Pts',(3.38262523533465,6.14405433362492,38.1135785878934));
#151615=CARTESIAN_POINT('Ctrl Pts',(3.21898415822728,6.22862485237165,38.121949266227));
#151616=CARTESIAN_POINT('Ctrl Pts',(3.05552878564632,6.31309939809982,38.1303104452779));
#151617=CARTESIAN_POINT('Ctrl Pts',(2.88859548451051,6.39121373611139,38.1386716243288));
#151618=CARTESIAN_POINT('Ctrl Pts',(2.71870570115949,6.46268256012802,38.1470328033797));
#151619=CARTESIAN_POINT('Ctrl Pts',(2.54903636984284,6.53405864491492,38.1553831328144));
#151620=CARTESIAN_POINT('Ctrl Pts',(2.37641850897576,6.59880628941818,38.1637334622492));
#151621=CARTESIAN_POINT('Ctrl Pts',(2.20139663399204,6.65668682020933,38.172083791684));
#151622=CARTESIAN_POINT('Ctrl Pts',(2.02650942787135,6.71452281539443,38.1804276960398));
#151623=CARTESIAN_POINT('Ctrl Pts',(1.84922220359946,6.76550212414569,38.1887716003956));
#151624=CARTESIAN_POINT('Ctrl Pts',(1.67009892933501,6.80943434719317,38.1971155047514));
#151625=CARTESIAN_POINT('Ctrl Pts',(1.49111952800193,6.85333128360502,38.2054527072312));
#151626=CARTESIAN_POINT('Ctrl Pts',(1.31030733510672,6.89019234507996,38.2137899097109));
#151627=CARTESIAN_POINT('Ctrl Pts',(1.12824108496155,6.91987706658903,38.2221271121907));
#151628=CARTESIAN_POINT('Ctrl Pts',(1.06830588040342,6.92964911305277,38.2248716732264));
#151629=CARTESIAN_POINT('Ctrl Pts',(1.00823488466737,6.93864387184466,38.2276162342621));
#151630=CARTESIAN_POINT('Ctrl Pts',(0.948049037357854,6.94685753310552,
38.2303607952978));
#151631=CARTESIAN_POINT('Ctrl Pts',(0.765197111634277,6.97181163520638,
38.2386991055997));
#151632=CARTESIAN_POINT('Ctrl Pts',(0.58143451101858,6.98953177441645,38.2470374159015));
#151633=CARTESIAN_POINT('Ctrl Pts',(0.397356357405064,6.99998103481215,
38.2553757262034));
#151634=CARTESIAN_POINT('Ctrl Pts',(0.213162388063885,7.0104368695279,38.2637192826871));
#151635=CARTESIAN_POINT('Ctrl Pts',(0.0286527968454356,7.01361268227092,
38.2720628391709));
#151636=CARTESIAN_POINT('Ctrl Pts',(-0.155576835271572,7.00952369357768,
38.2804063956546));
#151637=CARTESIAN_POINT('Ctrl Pts',(-0.339946628489893,7.00543159399967,
38.2887562998798));
#151638=CARTESIAN_POINT('Ctrl Pts',(-0.524035710558252,6.99406367562809,
38.297106204105));
#151639=CARTESIAN_POINT('Ctrl Pts',(-0.707252720335791,6.97548709066812,
38.3054561083301));
#151640=CARTESIAN_POINT('Ctrl Pts',(-0.890744542069787,6.9568826422054,
38.3138185367937));
#151641=CARTESIAN_POINT('Ctrl Pts',(-1.07336135136743,6.93104795352586,
38.3221809652573));
#151642=CARTESIAN_POINT('Ctrl Pts',(-1.25451958893951,6.89810170724287,
38.3305433937209));
#151643=CARTESIAN_POINT('Ctrl Pts',(-1.43583274150005,6.86512728742811,
38.3389129732008));
#151644=CARTESIAN_POINT('Ctrl Pts',(-1.61568451465483,6.82502924727088,
38.3472825526807));
#151645=CARTESIAN_POINT('Ctrl Pts',(-1.79350509200037,6.77797654521383,
38.3556521321606));
#151646=CARTESIAN_POINT('Ctrl Pts',(-1.9715999359211,6.73085127009667,38.3640346206971));
#151647=CARTESIAN_POINT('Ctrl Pts',(-2.147657011031,6.67674999395358,38.3724171092336));
#151648=CARTESIAN_POINT('Ctrl Pts',(-2.32112376405493,6.61589079674381,
38.3807995977701));
#151649=CARTESIAN_POINT('Ctrl Pts',(-2.37788492807296,6.59597667017714,
38.3835424853748));
#151650=CARTESIAN_POINT('Ctrl Pts',(-2.43436892247531,6.57533934513625,
38.3862853729796));
#151651=CARTESIAN_POINT('Ctrl Pts',(-2.49055693275816,6.5539875440216,38.3890282605843));
#151652=CARTESIAN_POINT('Ctrl Pts',(-2.66242298576839,6.48867735126408,
38.3974181157171));
#151653=CARTESIAN_POINT('Ctrl Pts',(-2.83186510552309,6.41654712207573,
38.4058079708499));
#151654=CARTESIAN_POINT('Ctrl Pts',(-2.99832485660819,6.33779730006771,
38.4141978259827));
#151655=CARTESIAN_POINT('Ctrl Pts',(-3.16463100096848,6.25912014729149,
38.4225799390747));
#151656=CARTESIAN_POINT('Ctrl Pts',(-3.32795996722671,6.17383571881745,
38.4309620521668));
#151657=CARTESIAN_POINT('Ctrl Pts',(-3.48777249563118,6.08219282670475,
38.4393441652589));
#151658=CARTESIAN_POINT('Ctrl Pts',(-3.64746104338508,5.99062103005306,
38.4477197756078));
#151659=CARTESIAN_POINT('Ctrl Pts',(-3.80363830796303,5.89270076724283,
38.4560953859567));
#151660=CARTESIAN_POINT('Ctrl Pts',(-3.95578847193318,5.78872733230894,
38.4644709963055));
#151661=CARTESIAN_POINT('Ctrl Pts',(-4.10784293119061,5.68481929820973,
38.4728413382711));
#151662=CARTESIAN_POINT('Ctrl Pts',(-4.255875069918,5.57486586886209,38.4812116802367));
#151663=CARTESIAN_POINT('Ctrl Pts',(-4.39939659076811,5.45920655403676,
38.4895820222023));
#151664=CARTESIAN_POINT('Ctrl Pts',(-4.54284887309337,5.34360303628143,
38.4979483260966));
#151665=CARTESIAN_POINT('Ctrl Pts',(-4.68179462141739,5.22229932821294,
38.5063146299909));
#151666=CARTESIAN_POINT('Ctrl Pts',(-4.81577691361292,5.095676528275,38.5146809338852));
#151667=CARTESIAN_POINT('Ctrl Pts',(-4.94972173471686,4.96908914118497,
38.5230448979588));
#151668=CARTESIAN_POINT('Ctrl Pts',(-5.07870562797996,4.83718585297268,
38.5314088620324));
#151669=CARTESIAN_POINT('Ctrl Pts',(-5.20230657686934,4.70038645674609,
38.539772826106));
#151670=CARTESIAN_POINT('Ctrl Pts',(-5.32588850562665,4.56360811167329,
38.5481355031046));
#151671=CARTESIAN_POINT('Ctrl Pts',(-5.44408892129556,4.42193540456572,
38.5564981801031));
#151672=CARTESIAN_POINT('Ctrl Pts',(-5.55652406798816,4.27582352820698,
38.5648608571016));
#151673=CARTESIAN_POINT('Ctrl Pts',(-5.66895689984657,4.12971466002473,
38.5732233619279));
#151674=CARTESIAN_POINT('Ctrl Pts',(-5.77562449930101,3.9791670655361,38.5815858667542));
#151675=CARTESIAN_POINT('Ctrl Pts',(-5.87618440035542,3.82466775753394,
38.5899483715805));
#151676=CARTESIAN_POINT('Ctrl Pts',(-5.97675563498432,3.67015103673206,
38.5983118189005));
#151677=CARTESIAN_POINT('Ctrl Pts',(-6.07121761998585,3.51168199018858,
38.6066752662205));
#151678=CARTESIAN_POINT('Ctrl Pts',(-6.15927186734454,3.34977560840097,
38.6150387135404));
#151679=CARTESIAN_POINT('Ctrl Pts',(-6.24737796351867,3.18777389158571,
38.6234070854932));
#151680=CARTESIAN_POINT('Ctrl Pts',(-6.32906862455444,3.02233108365615,
38.631775457446));
#151681=CARTESIAN_POINT('Ctrl Pts',(-6.40409141329911,2.85398663847758,
38.6401438293988));
#151682=CARTESIAN_POINT('Ctrl Pts',(-6.47913668083207,2.68559175290345,
38.6485147087346));
#151683=CARTESIAN_POINT('Ctrl Pts',(-6.54750996339649,2.51429379891466,
38.6568855880703));
#151684=CARTESIAN_POINT('Ctrl Pts',(-6.60900717989436,2.34065175936209,
38.6652564674061));
#151685=CARTESIAN_POINT('Ctrl Pts',(-6.67055650231875,2.16686259478713,
38.6736344392974));
#151686=CARTESIAN_POINT('Ctrl Pts',(-6.72521801252274,1.99072568787033,
38.6820124111886));
#151687=CARTESIAN_POINT('Ctrl Pts',(-6.77283731893325,1.8128158245572,38.6903903830799));
#151688=CARTESIAN_POINT('Ctrl Pts',(-6.80309977592282,1.69975265769545,
38.695714652439));
#151689=CARTESIAN_POINT('Ctrl Pts',(-6.8305191081714,1.5859737199079,38.701038921798));
#151690=CARTESIAN_POINT('Ctrl Pts',(-6.85506642330607,1.47162865375803,
38.706363191157));
#151691=CARTESIAN_POINT('Ctrl Pts',(-6.8913176686956,1.3027649295854,38.7142260223463));
#151692=CARTESIAN_POINT('Ctrl Pts',(-6.92137795629598,1.13231489320976,
38.7220888535356));
#151693=CARTESIAN_POINT('Ctrl Pts',(-6.94510661887911,0.960791660507956,
38.7299516847249));
#151694=CARTESIAN_POINT('Ctrl Pts',(-6.96881704911719,0.789400220769712,
38.7378084743663));
#151695=CARTESIAN_POINT('Ctrl Pts',(-6.98620547721606,0.616937599793814,
38.7456652640077));
#151696=CARTESIAN_POINT('Ctrl Pts',(-6.99718182459533,0.443929134043713,
38.7535220536491));
#151697=CARTESIAN_POINT('Ctrl Pts',(-7.00815198183427,0.27101823687844,
38.7613744124331));
#151698=CARTESIAN_POINT('Ctrl Pts',(-7.01271722755952,0.09756248660523,
38.7692267712171));
#151699=CARTESIAN_POINT('Ctrl Pts',(-7.01083909849228,-0.0759058466254896,
38.777079130001));
#151700=CARTESIAN_POINT('Ctrl Pts',(-7.00896141287323,-0.2493332219587,
38.7849296347515));
#151701=CARTESIAN_POINT('Ctrl Pts',(-7.00064337606947,-0.422772793341922,
38.7927801395019));
#151702=CARTESIAN_POINT('Ctrl Pts',(-6.98589860771008,-0.595690528122043,
38.8006306442524));
#151703=CARTESIAN_POINT('Ctrl Pts',(-6.97115621131921,-0.768580445888531,
38.808479886104));
#151704=CARTESIAN_POINT('Ctrl Pts',(-6.94998917689365,-0.940948314271634,
38.8163291279557));
#151705=CARTESIAN_POINT('Ctrl Pts',(-6.92246310930327,-1.11226393577931,
38.8241783698073));
#151706=CARTESIAN_POINT('Ctrl Pts',(-6.89492776764194,-1.28363727687313,
38.8320302562222));
#151707=CARTESIAN_POINT('Ctrl Pts',(-6.86102917391573,-1.45395728592724,
38.839882142637));
#151708=CARTESIAN_POINT('Ctrl Pts',(-6.82088434046041,-1.6227024916977,
38.8477340290519));
#151709=CARTESIAN_POINT('Ctrl Pts',(-6.79140648892726,-1.74660999596395,
38.8534995715158));
#151710=CARTESIAN_POINT('Ctrl Pts',(-6.75856187735805,-1.86966856995148,
38.8592651139797));
#151711=CARTESIAN_POINT('Ctrl Pts',(-6.72241403827056,-1.99167669579251,
38.8650306564436));
#151712=CARTESIAN_POINT('Ctrl Pts',(-6.66187881707776,-2.19599842211283,
38.8746859608036));
#151713=CARTESIAN_POINT('Ctrl Pts',(-6.59211003230734,-2.39726976124543,
38.8843412651637));
#151714=CARTESIAN_POINT('Ctrl Pts',(-6.51343727596498,-2.59475652317707,
38.8939965695238));
#151715=CARTESIAN_POINT('Ctrl Pts',(-6.43432868731119,-2.79333732472205,
38.9037053624587));
#151716=CARTESIAN_POINT('Ctrl Pts',(-6.34621726945475,-2.98809147764601,
38.9134141553936));
#151717=CARTESIAN_POINT('Ctrl Pts',(-6.24948186147165,-3.17830190913904,
38.9231229483285));
#151718=CARTESIAN_POINT('Ctrl Pts',(-6.15228095449145,-3.36942764937933,
38.9328784607994));
#151719=CARTESIAN_POINT('Ctrl Pts',(-6.04637289994086,-3.55596580573971,
38.9426339732703));
#151720=CARTESIAN_POINT('Ctrl Pts',(-5.93218523844047,-3.73721886692886,
38.9523894857412));
#151721=CARTESIAN_POINT('Ctrl Pts',(-5.8178845135879,-3.9186513965336,38.9621546576703));
#151722=CARTESIAN_POINT('Ctrl Pts',(-5.69528781363722,-4.09478833717525,
38.9719198295994));
#151723=CARTESIAN_POINT('Ctrl Pts',(-5.56486651916761,-4.2649603968088,
38.9816850015284));
#151724=CARTESIAN_POINT('Ctrl Pts',(-5.43462305117419,-4.43490043069964,
38.9914368588671));
#151725=CARTESIAN_POINT('Ctrl Pts',(-5.29657633458902,-4.59889180839344,
39.0011887162059));
#151726=CARTESIAN_POINT('Ctrl Pts',(-5.15123779077445,-4.75629853829606,
39.0109405735446));
#151727=CARTESIAN_POINT('Ctrl Pts',(-5.08785965976759,-4.82493927245572,
39.0151930896064));
#151728=CARTESIAN_POINT('Ctrl Pts',(-5.02309545812617,-4.89232827088929,
39.0194456056682));
#151729=CARTESIAN_POINT('Ctrl Pts',(-4.95699008883871,-4.95841464801552,
39.02369812173));
#151730=CARTESIAN_POINT('Ctrl Pts',(-4.83211638158264,-5.08325247888805,
39.0317311673287));
#151731=CARTESIAN_POINT('Ctrl Pts',(-4.70239330496352,-5.20350034449388,
39.0397642129274));
#151732=CARTESIAN_POINT('Ctrl Pts',(-4.568199694016,-5.31875719676055,39.0477972585261));
#151733=CARTESIAN_POINT('Ctrl Pts',(-4.4340923478886,-5.43393995748473,
39.0558251401738));
#151734=CARTESIAN_POINT('Ctrl Pts',(-4.29552046478516,-5.54413785345578,
39.0638530218215));
#151735=CARTESIAN_POINT('Ctrl Pts',(-4.15289952349382,-5.6489868215694,
39.0718809034692));
#151736=CARTESIAN_POINT('Ctrl Pts',(-4.01034297696333,-5.75378844934041,
39.0799051604492));
#151737=CARTESIAN_POINT('Ctrl Pts',(-3.86374130711362,-5.85324574130714,
39.0879294174292));
#151738=CARTESIAN_POINT('Ctrl Pts',(-3.71354280167257,-5.94703509512478,
39.0959536744092));
#151739=CARTESIAN_POINT('Ctrl Pts',(-3.56336245676058,-6.04081310885432,
39.1039769611748));
#151740=CARTESIAN_POINT('Ctrl Pts',(-3.40958644915615,-6.12892434887665,
39.1120002479404));
#151741=CARTESIAN_POINT('Ctrl Pts',(-3.25269190644824,-6.21108862633807,
39.120023534706));
#151742=CARTESIAN_POINT('Ctrl Pts',(-3.09581021984847,-6.29324617116993,
39.1280461640348));
#151743=CARTESIAN_POINT('Ctrl Pts',(-2.93581083381414,-6.3694575575606,
39.1360687933636));
#151744=CARTESIAN_POINT('Ctrl Pts',(-2.77319504630513,-6.43948878387475,
39.1440914226925));
#151745=CARTESIAN_POINT('Ctrl Pts',(-2.61051812683718,-6.50954633694424,
39.1521170679588));
#151746=CARTESIAN_POINT('Ctrl Pts',(-2.4452231791185,-6.57341894642677,
39.1601427132251));
#151747=CARTESIAN_POINT('Ctrl Pts',(-2.27783138026074,-6.63092080827388,
39.1681683584914));
#151748=CARTESIAN_POINT('Ctrl Pts',(-2.1791269752883,-6.66482741001396,
39.1729007679997));
#151749=CARTESIAN_POINT('Ctrl Pts',(-2.07969383548703,-6.69651983058423,
39.177633177508));
#151750=CARTESIAN_POINT('Ctrl Pts',(-1.9796412180197,-6.72596812439797,
39.1823655870163));
#151751=CARTESIAN_POINT('Ctrl Pts',(-1.79507049669824,-6.78029246861277,
39.1910956358511));
#151752=CARTESIAN_POINT('Ctrl Pts',(-1.608298733072,-6.8270046181273,39.1998256846859));
#151753=CARTESIAN_POINT('Ctrl Pts',(-1.41995570841795,-6.86595604039461,
39.2085557335207));
#151754=CARTESIAN_POINT('Ctrl Pts',(-1.23155822414363,-6.90491872551421,
39.21728830666));
#151755=CARTESIAN_POINT('Ctrl Pts',(-1.04158884023543,-6.93611614871323,
39.2260208797993));
#151756=CARTESIAN_POINT('Ctrl Pts',(-0.850687128366196,-6.95945098209134,
39.2347534529386));
#151757=CARTESIAN_POINT('Ctrl Pts',(-0.657073352947585,-6.98311732402648,
39.2436100862189));
#151758=CARTESIAN_POINT('Ctrl Pts',(-0.462500844959412,-6.99869593705051,
39.2524667194993));
#151759=CARTESIAN_POINT('Ctrl Pts',(-0.267642234618632,-7.00613975001558,
39.2613233527796));
#151760=CARTESIAN_POINT('Ctrl Pts',(-0.0753908197272747,-7.01348396525051,
39.2700614848865));
#151761=CARTESIAN_POINT('Ctrl Pts',(0.117138810563617,-7.01290972725781,
39.2787996169934));
#151762=CARTESIAN_POINT('Ctrl Pts',(0.30929962673723,-7.00442433775969,
39.2875377491003));
#151763=CARTESIAN_POINT('Ctrl Pts',(0.505369393118843,-6.99576633781109,
39.2964536329674));
#151764=CARTESIAN_POINT('Ctrl Pts',(0.701054883679541,-6.97887188955622,
39.3053695168345));
#151765=CARTESIAN_POINT('Ctrl Pts',(0.895672117856525,-6.95380457158485,
39.3142854007016));
#151766=CARTESIAN_POINT('Ctrl Pts',(1.09028935203351,-6.92873725361349,
39.3232012845686));
#151767=CARTESIAN_POINT('Ctrl Pts',(1.28383803066942,-6.89549711059129,
39.3321171684357));
#151768=CARTESIAN_POINT('Ctrl Pts',(1.47564203379495,-6.8542036116968,39.3410330523028));
#151769=CARTESIAN_POINT('Ctrl Pts',(1.66367703979096,-6.8137215404903,39.3497737367989));
#151770=CARTESIAN_POINT('Ctrl Pts',(1.85005527164544,-6.76549537689399,
39.358514421295));
#151771=CARTESIAN_POINT('Ctrl Pts',(2.03414967565739,-6.70968416987886,
39.3672551057911));
#151772=CARTESIAN_POINT('Ctrl Pts',(2.21821095802815,-6.65388300422693,
39.3759942176929));
#151773=CARTESIAN_POINT('Ctrl Pts',(2.39998897122777,-6.59049959992355,
39.3847333295946));
#151774=CARTESIAN_POINT('Ctrl Pts',(2.57887153826412,-6.51974295134641,
39.3934724414964));
#151775=CARTESIAN_POINT('Ctrl Pts',(2.76007178641663,-6.44806954854909,
39.4023247811708));
#151776=CARTESIAN_POINT('Ctrl Pts',(2.93830076272921,-6.36883059153292,
39.4111771208452));
#151777=CARTESIAN_POINT('Ctrl Pts',(3.11294149546067,-6.28229431086599,
39.4200294605196));
#151778=CARTESIAN_POINT('Ctrl Pts',(3.28526008039774,-6.19690867833332,
39.4287640931692));
#151779=CARTESIAN_POINT('Ctrl Pts',(3.45408500727737,-6.10441871503209,
39.4374987258189));
#151780=CARTESIAN_POINT('Ctrl Pts',(3.61884597437017,-6.00512950537162,
39.4462333584685));
#151781=CARTESIAN_POINT('Ctrl Pts',(3.78693739461582,-5.9038332787144,39.4551445516553));
#151782=CARTESIAN_POINT('Ctrl Pts',(3.95079854881783,-5.79546013156801,
39.4640557448421));
#151783=CARTESIAN_POINT('Ctrl Pts',(4.10985167050952,-5.68038254071943,
39.4729669380288));
#151784=CARTESIAN_POINT('Ctrl Pts',(4.26890479220121,-5.56530494987085,
39.4818781312156));
#151785=CARTESIAN_POINT('Ctrl Pts',(4.42314962789435,-5.44352308209216,
39.4907893244024));
#151786=CARTESIAN_POINT('Ctrl Pts',(4.57204038024953,-5.31545607863217,
39.4997005175891));
#151787=CARTESIAN_POINT('Ctrl Pts',(4.70613547312795,-5.20011542481734,
39.5077261824416));
#151788=CARTESIAN_POINT('Ctrl Pts',(4.83594899628487,-5.07962330971981,
39.5157518472941));
#151789=CARTESIAN_POINT('Ctrl Pts',(4.96106213968239,-4.95434042115699,
39.5237775121466));
#151790=CARTESIAN_POINT('Ctrl Pts',(5.08613557523666,-4.82909729431037,
39.5318006298499));
#151791=CARTESIAN_POINT('Ctrl Pts',(5.20651134231518,-4.69906668019109,
39.5398237475532));
#151792=CARTESIAN_POINT('Ctrl Pts',(5.32180619379329,-4.5646473465322,39.5478468652565));
#151793=CARTESIAN_POINT('Ctrl Pts',(5.43708650558191,-4.43024496432731,
39.5558689711744));
#151794=CARTESIAN_POINT('Ctrl Pts',(5.54728693992884,-4.29145524355056,
39.5638910770924));
#151795=CARTESIAN_POINT('Ctrl Pts',(5.65206342294826,-4.14871132105746,
39.5719131830103));
#151796=CARTESIAN_POINT('Ctrl Pts',(5.75687884126272,-4.00591435444058,
39.57993826997));
#151797=CARTESIAN_POINT('Ctrl Pts',(5.85626606227109,-3.85916054473022,
39.5879633569296));
#151798=CARTESIAN_POINT('Ctrl Pts',(5.94992312729261,-3.70891376845143,
39.5959884438892));
#151799=CARTESIAN_POINT('Ctrl Pts',(6.04359863760414,-3.55863740182233,
39.6040151113495));
#151800=CARTESIAN_POINT('Ctrl Pts',(6.13154155728599,-3.4048670139046,39.6120417788098));
#151801=CARTESIAN_POINT('Ctrl Pts',(6.21349519491764,-3.2480923671034,39.6200684462701));
#151802=CARTESIAN_POINT('Ctrl Pts',(6.29551462464098,-3.09119186216786,
39.6281015575108));
#151803=CARTESIAN_POINT('Ctrl Pts',(6.37153500763469,-2.93128261046679,
39.6361346687515));
#151804=CARTESIAN_POINT('Ctrl Pts',(6.44134697281337,-2.76887625912174,
39.6441677799922));
#151805=CARTESIAN_POINT('Ctrl Pts',(6.48248271875035,-2.67318053718666,
39.6489011809534));
#151806=CARTESIAN_POINT('Ctrl Pts',(6.52146382345709,-2.57661819013828,
39.6536345819146));
#151807=CARTESIAN_POINT('Ctrl Pts',(6.55825550999511,-2.47929651879699,
39.6583679828758));
#151808=CARTESIAN_POINT('Ctrl Pts',(6.63609765095225,-2.27338784834488,
39.6683826927056));
#151809=CARTESIAN_POINT('Ctrl Pts',(6.70417624722286,-2.06397613249315,
39.6783974025354));
#151810=CARTESIAN_POINT('Ctrl Pts',(6.76225540238797,-1.85189860288697,
39.6884121123653));
#151811=CARTESIAN_POINT('Ctrl Pts',(6.82040337169505,-1.63956979667062,
39.6984386879611));
#151812=CARTESIAN_POINT('Ctrl Pts',(6.86852822639077,-1.42456881701543,
39.7084652635569));
#151813=CARTESIAN_POINT('Ctrl Pts',(6.90644452585608,-1.20774607172724,
39.7184918391527));
#151814=CARTESIAN_POINT('Ctrl Pts',(6.94423360637603,-0.991650822565392,
39.7284847730064));
#151815=CARTESIAN_POINT('Ctrl Pts',(6.97188254054378,-0.773745968779786,
39.73847770686));
#151816=CARTESIAN_POINT('Ctrl Pts',(6.98925819898149,-0.554884123461851,
39.7484706407136));
#151817=CARTESIAN_POINT('Ctrl Pts',(7.00378508295101,-0.371905121907101,
39.7568252127792));
#151818=CARTESIAN_POINT('Ctrl Pts',(7.01113204989888,-0.188257378415018,
39.7651797848449));
#151819=CARTESIAN_POINT('Ctrl Pts',(7.01124859079596,-0.00444528532742304,
39.7735343569106));
#151820=CARTESIAN_POINT('Ctrl Pts',(7.01125,4.27274591884109E-12,39.7735343569106));
#151821=CARTESIAN_POINT('Ctrl Pts',(7.01124999999988,0.191008754744388,
39.7822061308427));
#151822=CARTESIAN_POINT('Ctrl Pts',(7.00344012880995,0.382017367487167,
39.7908779047748));
#151823=CARTESIAN_POINT('Ctrl Pts',(6.98784644419146,0.572388534913825,
39.7995496787069));
#151824=CARTESIAN_POINT('Ctrl Pts',(6.97225169663163,0.762772678964547,
39.8082220437493));
#151825=CARTESIAN_POINT('Ctrl Pts',(6.94887209704274,0.95251900763093,39.8168944087916));
#151826=CARTESIAN_POINT('Ctrl Pts',(6.91778566246042,1.14099434299962,39.825566773834));
#151827=CARTESIAN_POINT('Ctrl Pts',(6.88670108297129,1.32945843104071,39.8342386213501));
#151828=CARTESIAN_POINT('Ctrl Pts',(6.84791063501086,1.51665139731196,39.8429104688662));
#151829=CARTESIAN_POINT('Ctrl Pts',(6.80154374572899,1.7019486588716,39.8515823163824));
#151830=CARTESIAN_POINT('Ctrl Pts',(6.75517597619819,1.88724943819403,39.8602543285286));
#151831=CARTESIAN_POINT('Ctrl Pts',(6.70123154646044,2.07065416525604,39.8689263406748));
#151832=CARTESIAN_POINT('Ctrl Pts',(6.63989045285482,2.25155087363966,39.877598352821));
#151833=CARTESIAN_POINT('Ctrl Pts',(6.61790934153606,2.31637382429882,39.8807059019881));
#151834=CARTESIAN_POINT('Ctrl Pts',(6.59497889661496,2.38087486019118,39.8838134511552));
#151835=CARTESIAN_POINT('Ctrl Pts',(6.57110895151814,2.44502632087636,39.8869210003223));
#151836=CARTESIAN_POINT('',(7.01124999602994,0.000235945347496286,39.2264656431317));
#151837=CARTESIAN_POINT('Ctrl Pts',(6.57110895151813,2.44502632087639,39.3399667765699));
#151838=CARTESIAN_POINT('Ctrl Pts',(6.64421271995929,2.24855693194103,39.3304229520256));
#151839=CARTESIAN_POINT('Ctrl Pts',(6.70850190625911,2.04880522801078,39.3208791274812));
#151840=CARTESIAN_POINT('Ctrl Pts',(6.76372928243494,1.84650826059135,39.3113353029369));
#151841=CARTESIAN_POINT('Ctrl Pts',(6.81886334836796,1.6445530870513,39.3018076033046));
#151842=CARTESIAN_POINT('Ctrl Pts',(6.86496615835579,1.4400613342989,39.2922799036724));
#151843=CARTESIAN_POINT('Ctrl Pts',(6.90184075352121,1.23378311527345,39.2827522040401));
#151844=CARTESIAN_POINT('Ctrl Pts',(6.93853377568314,1.02852062416622,39.273271419446));
#151845=CARTESIAN_POINT('Ctrl Pts',(6.96608920614919,0.821489313606136,
39.2637906348519));
#151846=CARTESIAN_POINT('Ctrl Pts',(6.98436207776607,0.61344350119897,39.2543098502577));
#151847=CARTESIAN_POINT('Ctrl Pts',(7.0022506683511,0.409772921165857,39.2450284478824));
#151848=CARTESIAN_POINT('Ctrl Pts',(7.01124310084812,0.205130188839553,
39.235747045507));
#151849=CARTESIAN_POINT('Ctrl Pts',(7.01124999602994,0.000235945347480019,
39.2264656431317));
#151850=CARTESIAN_POINT('Ctrl Pts',(7.01124999602997,0.000235944418096841,
39.2264656430896));
#151851=CARTESIAN_POINT('Ctrl Pts',(7.01125624170091,-0.185358445530651,
39.2180584951759));
#151852=CARTESIAN_POINT('Ctrl Pts',(7.00388885553632,-0.370934254546438,
39.2096513472621));
#151853=CARTESIAN_POINT('Ctrl Pts',(6.98917832624288,-0.555889275374905,
39.2012441993484));
#151854=CARTESIAN_POINT('Ctrl Pts',(6.97446405541024,-0.740891338457691,
39.1928349131245));
#151855=CARTESIAN_POINT('Ctrl Pts',(6.95240294147731,-0.925271977684133,
39.1844256269007));
#151856=CARTESIAN_POINT('Ctrl Pts',(6.92307738877438,-1.10843404474104,
39.1760163406768));
#151857=CARTESIAN_POINT('Ctrl Pts',(6.89374093683712,-1.29166418643262,
39.1676039290291));
#151858=CARTESIAN_POINT('Ctrl Pts',(6.85713471151255,-1.47367453500346,
39.1591915173815));
#151859=CARTESIAN_POINT('Ctrl Pts',(6.81339236826982,-1.65387756454419,
39.1507791057338));
#151860=CARTESIAN_POINT('Ctrl Pts',(6.76962863059373,-1.83416873160611,
39.1423625795653));
#151861=CARTESIAN_POINT('Ctrl Pts',(6.71872188872574,-2.0126505040424,39.1339460533969));
#151862=CARTESIAN_POINT('Ctrl Pts',(6.66085597739889,-2.1887494627868,39.1255295272284));
#151863=CARTESIAN_POINT('Ctrl Pts',(6.60292446423264,-2.36504806265572,
39.1171034593525));
#151864=CARTESIAN_POINT('Ctrl Pts',(6.53801811449966,-2.53895814410867,
39.1086773914766));
#151865=CARTESIAN_POINT('Ctrl Pts',(6.46636985185425,-2.70992389220259,
39.1002513236007));
#151866=CARTESIAN_POINT('Ctrl Pts',(6.39467912786007,-2.88099096077507,
39.0918202621325));
#151867=CARTESIAN_POINT('Ctrl Pts',(6.31623865159298,-3.04910992165933,
39.0833892006644));
#151868=CARTESIAN_POINT('Ctrl Pts',(6.2313281825243,-3.21374791235692,39.0749581391963));
#151869=CARTESIAN_POINT('Ctrl Pts',(6.14630796696497,-3.37859869709397,
39.06651618061));
#151870=CARTESIAN_POINT('Ctrl Pts',(6.05480119927518,-3.5399592370319,39.0580742220238));
#151871=CARTESIAN_POINT('Ctrl Pts',(5.95713277845971,-3.69732276414988,
39.0496322634376));
#151872=CARTESIAN_POINT('Ctrl Pts',(5.8898921681621,-3.80566095077819,39.0438203291122));
#151873=CARTESIAN_POINT('Ctrl Pts',(5.81973201113902,-3.91210524289392,
39.0380083947868));
#151874=CARTESIAN_POINT('Ctrl Pts',(5.74676973213542,-4.01649899891836,
39.0321964604614));
#151875=CARTESIAN_POINT('Ctrl Pts',(5.64155196051087,-4.16704361636195,
39.0238151600566));
#151876=CARTESIAN_POINT('Ctrl Pts',(5.53029242921354,-4.31362675214747,
39.0154338596518));
#151877=CARTESIAN_POINT('Ctrl Pts',(5.41331025385954,-4.45574894467352,
39.007052559247));
#151878=CARTESIAN_POINT('Ctrl Pts',(5.29647633628785,-4.59769101812572,
38.9986818809135));
#151879=CARTESIAN_POINT('Ctrl Pts',(5.17393443490431,-4.73518316441594,
38.9903112025801));
#151880=CARTESIAN_POINT('Ctrl Pts',(5.04604670723755,-4.86775504631007,
38.9819405242466));
#151881=CARTESIAN_POINT('Ctrl Pts',(4.9183041101841,-5.00017648188007,38.9735793451959));
#151882=CARTESIAN_POINT('Ctrl Pts',(4.78522800433629,-5.12768854751416,
38.9652181661451));
#151883=CARTESIAN_POINT('Ctrl Pts',(4.64722083488818,-5.24985381456296,
38.9568569870944));
#151884=CARTESIAN_POINT('Ctrl Pts',(4.50939274602224,-5.37186055776671,
38.9485066576597));
#151885=CARTESIAN_POINT('Ctrl Pts',(4.36664660049408,-5.4885341250155,38.9401563282251));
#151886=CARTESIAN_POINT('Ctrl Pts',(4.21942164598243,-5.59947386241912,
38.9318059987905));
#151887=CARTESIAN_POINT('Ctrl Pts',(4.07230997226684,-5.71032823833081,
38.9234620944349));
#151888=CARTESIAN_POINT('Ctrl Pts',(3.92072661773254,-5.8154573800439,38.9151181900793));
#151889=CARTESIAN_POINT('Ctrl Pts',(3.76514473331342,-5.91450012255492,
38.9067742857237));
#151890=CARTESIAN_POINT('Ctrl Pts',(3.60968781323395,-6.01346331331762,
38.8984370832441));
#151891=CARTESIAN_POINT('Ctrl Pts',(3.45023904403302,-6.10634967911778,
38.8900998807645));
#151892=CARTESIAN_POINT('Ctrl Pts',(3.28730157298377,-6.19284061887261,
38.8817626782849));
#151893=CARTESIAN_POINT('Ctrl Pts',(3.23366345689626,-6.2213129588274,38.8790181172483));
#151894=CARTESIAN_POINT('Ctrl Pts',(3.17964750752207,-6.24909258139602,
38.8762735562117));
#151895=CARTESIAN_POINT('Ctrl Pts',(3.12527233755018,-6.27616916427877,
38.8735289951751));
#151896=CARTESIAN_POINT('Ctrl Pts',(2.9600739564974,-6.35843111691236,38.8651906848731));
#151897=CARTESIAN_POINT('Ctrl Pts',(2.79169365376994,-6.43413296875984,
38.8568523745711));
#151898=CARTESIAN_POINT('Ctrl Pts',(2.62068329857847,-6.50304894730556,
38.8485140642691));
#151899=CARTESIAN_POINT('Ctrl Pts',(2.44956534947534,-6.57200828544607,
38.8401705077853));
#151900=CARTESIAN_POINT('Ctrl Pts',(2.2758143512251,-6.63417311188344,38.8318269513015));
#151901=CARTESIAN_POINT('Ctrl Pts',(2.09999932365371,-6.68936689105583,
38.8234833948177));
#151902=CARTESIAN_POINT('Ctrl Pts',(1.92405053677385,-6.74460266141542,
38.8151334905923));
#151903=CARTESIAN_POINT('Ctrl Pts',(1.74603490058279,-6.7928567076473,38.806783586367));
#151904=CARTESIAN_POINT('Ctrl Pts',(1.56653408794348,-6.83400303729894,
38.7984336821417));
#151905=CARTESIAN_POINT('Ctrl Pts',(1.38676403736921,-6.87521108340002,
38.790071253678));
#151906=CARTESIAN_POINT('Ctrl Pts',(1.2055046784367,-6.90929003552121,38.7817088252142));
#151907=CARTESIAN_POINT('Ctrl Pts',(1.02334681547847,-6.93616521269138,
38.7733463967505));
#151908=CARTESIAN_POINT('Ctrl Pts',(0.841033182715451,-6.96306337180169,
38.7649768172705));
#151909=CARTESIAN_POINT('Ctrl Pts',(0.657819837884503,-6.98274542983526,
38.7566072377904));
#151910=CARTESIAN_POINT('Ctrl Pts',(0.474300687146857,-6.99518873374207,
38.7482376583104));
#151911=CARTESIAN_POINT('Ctrl Pts',(0.290498480479108,-7.00765122992908,
38.7398551697738));
#151912=CARTESIAN_POINT('Ctrl Pts',(0.106389852255073,-7.01285265196182,
38.7314726812371));
#151913=CARTESIAN_POINT('Ctrl Pts',(-0.0774318940327818,-7.01082240998062,
38.7230901927005));
#151914=CARTESIAN_POINT('Ctrl Pts',(-0.137581381506239,-7.010158081537,
38.7203473050965));
#151915=CARTESIAN_POINT('Ctrl Pts',(-0.197700200088622,-7.00871986779992,
38.7176044174926));
#151916=CARTESIAN_POINT('Ctrl Pts',(-0.257767731967355,-7.00650999848401,
38.7148615298886));
#151917=CARTESIAN_POINT('Ctrl Pts',(-0.441500339136088,-6.9997505223042,
38.7064716747558));
#151918=CARTESIAN_POINT('Ctrl Pts',(-0.625123584587192,-6.9857538927227,
38.6980818196231));
#151919=CARTESIAN_POINT('Ctrl Pts',(-0.808044247700737,-6.96453092865972,
38.6896919644903));
#151920=CARTESIAN_POINT('Ctrl Pts',(-0.990796114190347,-6.94332754885049,
38.6813098513982));
#151921=CARTESIAN_POINT('Ctrl Pts',(-1.17284636583428,-6.91491116563033,
38.6729277383062));
#151922=CARTESIAN_POINT('Ctrl Pts',(-1.35360443769717,-6.87934456098446,
38.6645456252141));
#151923=CARTESIAN_POINT('Ctrl Pts',(-1.53422227960679,-6.8438055484857,
38.6561700148653));
#151924=CARTESIAN_POINT('Ctrl Pts',(-1.71354961894566,-6.8011274369386,
38.6477944045164));
#151925=CARTESIAN_POINT('Ctrl Pts',(-1.89100319271344,-6.75142455246651,
38.6394187941676));
#151926=CARTESIAN_POINT('Ctrl Pts',(-2.06834514554848,-6.70175293184674,
38.631048452202));
#151927=CARTESIAN_POINT('Ctrl Pts',(-2.24381536715877,-6.64506543719887,
38.6226781102364));
#151928=CARTESIAN_POINT('Ctrl Pts',(-2.41684248556805,-6.581527099576,38.6143077682709));
#151929=CARTESIAN_POINT('Ctrl Pts',(-2.5897861311839,-6.51801941450389,
38.6059414643765));
#151930=CARTESIAN_POINT('Ctrl Pts',(-2.76028871592533,-6.44766759032456,
38.5975751604822));
#151931=CARTESIAN_POINT('Ctrl Pts',(-2.92779525273806,-6.37068611065908,
38.5892088565878));
#151932=CARTESIAN_POINT('Ctrl Pts',(-3.09525494266641,-6.29372616055623,
38.5808448925142));
#151933=CARTESIAN_POINT('Ctrl Pts',(-3.2597199564803,-6.21014038788161,
38.5724809284406));
#151934=CARTESIAN_POINT('Ctrl Pts',(-3.42065596391555,-6.12019111948548,
38.564116964367));
#151935=CARTESIAN_POINT('Ctrl Pts',(-3.58156720597369,-6.03025569278699,
38.5557542873685));
#151936=CARTESIAN_POINT('Ctrl Pts',(-3.73895023759169,-5.93395888306768,
38.54739161037));
#151937=CARTESIAN_POINT('Ctrl Pts',(-3.89229561965599,-5.83160881504468,
38.5390289333714));
#151938=CARTESIAN_POINT('Ctrl Pts',(-4.04563784461916,-5.7292608542225,
38.5306664285452));
#151939=CARTESIAN_POINT('Ctrl Pts',(-4.19494231265526,-5.62086006638377,
38.5223039237189));
#151940=CARTESIAN_POINT('Ctrl Pts',(-4.33972849282946,-5.50675795464302,
38.5139414188926));
#151941=CARTESIAN_POINT('Ctrl Pts',(-4.48453099108833,-5.39264298305669,
38.5055779715726));
#151942=CARTESIAN_POINT('Ctrl Pts',(-4.62481392843816,-5.27282561031236,
38.4972145242526));
#151943=CARTESIAN_POINT('Ctrl Pts',(-4.76012946020875,-5.14769794029844,
38.4888510769326));
#151944=CARTESIAN_POINT('Ctrl Pts',(-4.89552466956728,-5.02249659159589,
38.4804827049798));
#151945=CARTESIAN_POINT('Ctrl Pts',(-5.02594638639755,-4.89197892009062,
38.472114333027));
#151946=CARTESIAN_POINT('Ctrl Pts',(-5.15098254249893,-4.75657496623056,
38.4637459610742));
#151947=CARTESIAN_POINT('Ctrl Pts',(-5.27605616270038,-4.62113044180728,
38.4553750817385));
#151948=CARTESIAN_POINT('Ctrl Pts',(-5.39574078546048,-4.48079696082687,
38.4470042024027));
#151949=CARTESIAN_POINT('Ctrl Pts',(-5.50966388458783,-4.33603856548446,
38.438633323067));
#151950=CARTESIAN_POINT('Ctrl Pts',(-5.62368350952496,-4.1911575179193,
38.4302553511757));
#151951=CARTESIAN_POINT('Ctrl Pts',(-5.73193165718274,-4.04184432625667,
38.4218773792844));
#151952=CARTESIAN_POINT('Ctrl Pts',(-5.83407780103354,-3.88859393277155,
38.4134994073932));
#151953=CARTESIAN_POINT('Ctrl Pts',(-5.89899250723136,-3.7912020597869,
38.4081751380341));
#151954=CARTESIAN_POINT('Ctrl Pts',(-5.96144366641284,-3.69222065152121,
38.402850868675));
#151955=CARTESIAN_POINT('Ctrl Pts',(-6.02135593370038,-3.59178218746506,
38.3975265993159));
#151956=CARTESIAN_POINT('Ctrl Pts',(-6.10983380964514,-3.44345560319153,
38.3896637681265));
#151957=CARTESIAN_POINT('Ctrl Pts',(-6.19295614892028,-3.29164153103512,
38.3818009369372));
#151958=CARTESIAN_POINT('Ctrl Pts',(-6.27042519721691,-3.13678089904399,
38.3739381057479));
#151959=CARTESIAN_POINT('Ctrl Pts',(-6.34783472077548,-2.98203925700769,
38.3660813161065));
#151960=CARTESIAN_POINT('Ctrl Pts',(-6.41959942216686,-2.82425604909293,
38.3582245264651));
#151961=CARTESIAN_POINT('Ctrl Pts',(-6.48546554701166,-2.66389999831539,
38.3503677368237));
#151962=CARTESIAN_POINT('Ctrl Pts',(-6.55129452648003,-2.50363438075955,
38.3425153780397));
#151963=CARTESIAN_POINT('Ctrl Pts',(-6.61123140219707,-2.34079915821629,
38.3346630192557));
#151964=CARTESIAN_POINT('Ctrl Pts',(-6.66506908723199,-2.17588617002924,
38.3268106604717));
#151965=CARTESIAN_POINT('Ctrl Pts',(-6.71889406056143,-2.0110121197225,
38.3189601557213));
#151966=CARTESIAN_POINT('Ctrl Pts',(-6.76662258314972,-1.84406163967041,
38.3111096509708));
#151967=CARTESIAN_POINT('Ctrl Pts',(-6.80809633639841,-1.67554493727223,
38.3032591462203));
#151968=CARTESIAN_POINT('Ctrl Pts',(-6.84956341782725,-1.50705534390062,
38.2954099043687));
#151969=CARTESIAN_POINT('Ctrl Pts',(-6.88477764469847,-1.33700040094602,
38.287560662517));
#151970=CARTESIAN_POINT('Ctrl Pts',(-6.91363116893351,-1.16590335039021,
38.2797114206653));
#151971=CARTESIAN_POINT('Ctrl Pts',(-6.94249441448566,-0.99474865388884,
38.2718595342505));
#151972=CARTESIAN_POINT('Ctrl Pts',(-6.96499261329928,-0.822551525018547,
38.2640076478356));
#151973=CARTESIAN_POINT('Ctrl Pts',(-6.98106940870108,-0.649843422216428,
38.2561557614207));
#151974=CARTESIAN_POINT('Ctrl Pts',(-6.99287439946038,-0.523026011987538,
38.2503902189569));
#151975=CARTESIAN_POINT('Ctrl Pts',(-7.00121818321528,-0.395933280436445,
38.2446246764931));
#151976=CARTESIAN_POINT('Ctrl Pts',(-7.006096328775,-0.26877647669662,38.2388591340293));
#151977=CARTESIAN_POINT('Ctrl Pts',(-7.01426554795703,-0.0558324824022358,
38.2292038296696));
#151978=CARTESIAN_POINT('Ctrl Pts',(-7.01271064726137,0.157182581771933,
38.2195485253098));
#151979=CARTESIAN_POINT('Ctrl Pts',(-7.00150842649841,0.369467611803443,
38.2098932209501));
#151980=CARTESIAN_POINT('Ctrl Pts',(-6.99024414753392,0.582928661077378,
38.2001844280156));
#151981=CARTESIAN_POINT('Ctrl Pts',(-6.9692254208714,0.795651521071237,
38.190475635081));
#151982=CARTESIAN_POINT('Ctrl Pts',(-6.93858118165131,1.00683551195533,
38.1807668421465));
#151983=CARTESIAN_POINT('Ctrl Pts',(-6.90778947975004,1.21903573813549,
38.1710113296759));
#151984=CARTESIAN_POINT('Ctrl Pts',(-6.86727943479273,1.42968220986307,
38.1612558172054));
#151985=CARTESIAN_POINT('Ctrl Pts',(-6.81723238420865,1.63797716168356,
38.1515003047348));
#151986=CARTESIAN_POINT('Ctrl Pts',(-6.76713577934516,1.84647835755082,
38.1417351328061));
#151987=CARTESIAN_POINT('Ctrl Pts',(-6.7074833003174,2.05262334157793,38.1319699608774));
#151988=CARTESIAN_POINT('Ctrl Pts',(-6.63850685770685,2.25562702206706,
38.1222047889487));
#151989=CARTESIAN_POINT('Ctrl Pts',(-6.56962446291061,2.45835391164434,
38.1124529316103));
#151990=CARTESIAN_POINT('Ctrl Pts',(-6.49144352552242,2.65794802213785,
38.102701074272));
#151991=CARTESIAN_POINT('Ctrl Pts',(-6.40424455977526,2.85364296664614,
38.0929492169336));
#151992=CARTESIAN_POINT('Ctrl Pts',(-6.36621949545174,2.93898013537233,
38.0886967008701));
#151993=CARTESIAN_POINT('Ctrl Pts',(-6.32648020594196,3.02357604425985,
38.0844441848065));
#151994=CARTESIAN_POINT('Ctrl Pts',(-6.28505290906249,3.10736809740737,
38.080191668743));
#151995=CARTESIAN_POINT('Ctrl Pts',(-6.20679632874674,3.26565212824915,
38.0721586231441));
#151996=CARTESIAN_POINT('Ctrl Pts',(-6.12247476552803,3.42114328480809,
38.0641255775452));
#151997=CARTESIAN_POINT('Ctrl Pts',(-6.03231847320291,3.57334023014251,
38.0560925319463));
#151998=CARTESIAN_POINT('Ctrl Pts',(-5.94222013681373,3.72543933742053,
38.0480646502984));
#151999=CARTESIAN_POINT('Ctrl Pts',(-5.8462947233995,3.87424813462715,38.0400367686505));
#152000=CARTESIAN_POINT('Ctrl Pts',(-5.74481905402391,4.01928856876734,
38.0320088870026));
#152001=CARTESIAN_POINT('Ctrl Pts',(-5.64338920191287,4.16426351572245,
38.0239846300224));
#152002=CARTESIAN_POINT('Ctrl Pts',(-5.53641429326912,4.3054731876663,38.0159603730422));
#152003=CARTESIAN_POINT('Ctrl Pts',(-5.42421519844507,4.44246733735405,
38.007936116062));
#152004=CARTESIAN_POINT('Ctrl Pts',(-5.312029669635,4.57944492305299,37.9999128292962));
#152005=CARTESIAN_POINT('Ctrl Pts',(-5.19462143896387,4.71220771341635,
37.9918895425304));
#152006=CARTESIAN_POINT('Ctrl Pts',(-5.07235261321641,4.84033733635339,
37.9838662557646));
#152007=CARTESIAN_POINT('Ctrl Pts',(-4.9500938063094,4.96845646020989,37.9758436264357));
#152008=CARTESIAN_POINT('Ctrl Pts',(-4.82297545369296,5.0919429103813,37.9678209971067));
#152009=CARTESIAN_POINT('Ctrl Pts',(-4.69139736489977,5.2104143143431,37.9597983677778));
#152010=CARTESIAN_POINT('Ctrl Pts',(-4.55976981211172,5.32893025511929,
37.9517727225113));
#152011=CARTESIAN_POINT('Ctrl Pts',(-4.4236794485809,5.44242714026978,37.9437470772448));
#152012=CARTESIAN_POINT('Ctrl Pts',(-4.28356036646062,5.5505618769083,37.9357214319784));
#152013=CARTESIAN_POINT('Ctrl Pts',(-4.20093761721511,5.61432470702978,
37.930989022471));
#152014=CARTESIAN_POINT('Ctrl Pts',(-4.11691470232539,5.67622388780985,
37.9262566129637));
#152015=CARTESIAN_POINT('Ctrl Pts',(-4.03158551017522,5.73619602494939,
37.9215242034564));
#152016=CARTESIAN_POINT('Ctrl Pts',(-3.87417562978967,5.84682881890563,
37.9127941546218));
#152017=CARTESIAN_POINT('Ctrl Pts',(-3.71224031257984,5.95095695937954,
37.9040641057872));
#152018=CARTESIAN_POINT('Ctrl Pts',(-3.5463284714095,6.0482378372027,37.8953340569527));
#152019=CARTESIAN_POINT('Ctrl Pts',(-3.38036865662394,6.14554684391267,
37.8866014838136));
#152020=CARTESIAN_POINT('Ctrl Pts',(-3.21043025909689,6.23600449743395,
37.8778689106746));
#152021=CARTESIAN_POINT('Ctrl Pts',(-3.03708788225907,6.3193135511648,37.8691363375355));
#152022=CARTESIAN_POINT('Ctrl Pts',(-2.86128290024866,6.40380614299168,
37.8602797042551));
#152023=CARTESIAN_POINT('Ctrl Pts',(-2.68197674511356,6.48094534690321,
37.8514230709746));
#152024=CARTESIAN_POINT('Ctrl Pts',(-2.49979144674987,6.55047092087708,
37.8425664376942));
#152025=CARTESIAN_POINT('Ctrl Pts',(-2.32004377575778,6.61906624722028,
37.8338283055875));
#152026=CARTESIAN_POINT('Ctrl Pts',(-2.13749379631818,6.68025034069134,
37.8250901734809));
#152027=CARTESIAN_POINT('Ctrl Pts',(-1.95275672189837,6.73382266974567,
37.8163520413742));
#152028=CARTESIAN_POINT('Ctrl Pts',(-1.76426171158982,6.78848477127057,
37.8074361575068));
#152029=CARTESIAN_POINT('Ctrl Pts',(-1.5734899565185,6.83522202693568,37.7985202736395));
#152030=CARTESIAN_POINT('Ctrl Pts',(-1.38110971377457,6.87387536408812,
37.7896043897722));
#152031=CARTESIAN_POINT('Ctrl Pts',(-1.18872947103065,6.91252870124056,
37.7806885059048));
#152032=CARTESIAN_POINT('Ctrl Pts',(-0.994741038299275,6.94309806627354,
37.7717726220374));
#152033=CARTESIAN_POINT('Ctrl Pts',(-0.799823146441631,6.96547984685307,
37.7628567381701));
#152034=CARTESIAN_POINT('Ctrl Pts',(-0.608735440415276,6.98742181978826,
37.7541160536738));
#152035=CARTESIAN_POINT('Ctrl Pts',(-0.416734168982142,7.001497328095,37.7453753691775));
#152036=CARTESIAN_POINT('Ctrl Pts',(-0.224464276876075,7.00765598120417,
37.7366346846812));
#152037=CARTESIAN_POINT('Ctrl Pts',(-0.0322289773166385,7.01381352626936,
37.7278955727793));
#152038=CARTESIAN_POINT('Ctrl Pts',(0.160274572842149,7.01205705195769,
37.7191564608773));
#152039=CARTESIAN_POINT('Ctrl Pts',(0.352399506944261,7.00238824616327,
37.7104173489753));
#152040=CARTESIAN_POINT('Ctrl Pts',(0.547013696080467,6.9925941670741,37.701565009301));
#152041=CARTESIAN_POINT('Ctrl Pts',(0.741239103951189,6.97468128782051,
37.6927126696267));
#152042=CARTESIAN_POINT('Ctrl Pts',(0.934405330218199,6.94870586809946,
37.6838603299524));
#152043=CARTESIAN_POINT('Ctrl Pts',(1.12500308051652,6.9230758360925,37.6751256973025));
#152044=CARTESIAN_POINT('Ctrl Pts',(1.31456936496239,6.88959639388524,37.6663910646527));
#152045=CARTESIAN_POINT('Ctrl Pts',(1.50246617357085,6.84837367261567,37.6576564320028));
#152046=CARTESIAN_POINT('Ctrl Pts',(1.69416109970754,6.80631768152435,37.6487452388163));
#152047=CARTESIAN_POINT('Ctrl Pts',(1.88411804984048,6.75620207544141,37.6398340456297));
#152048=CARTESIAN_POINT('Ctrl Pts',(2.07167033626311,6.69819442688457,37.6309228524432));
#152049=CARTESIAN_POINT('Ctrl Pts',(2.25922262268577,6.64018677832772,37.6220116592566));
#152050=CARTESIAN_POINT('Ctrl Pts',(2.44436995182194,6.57428716399278,37.6131004660701));
#152051=CARTESIAN_POINT('Ctrl Pts',(2.62646095606413,6.5007176072162,37.6041892728836));
#152052=CARTESIAN_POINT('Ctrl Pts',(2.790457105859,6.43445884773664,37.5961636080312));
#152053=CARTESIAN_POINT('Ctrl Pts',(2.95204935192554,6.36194783750325,37.5881379431789));
#152054=CARTESIAN_POINT('Ctrl Pts',(3.1107253513043,6.28339194633382,37.5801122783266));
#152055=CARTESIAN_POINT('Ctrl Pts',(3.26935099081321,6.20486098687726,37.5720891606234));
#152056=CARTESIAN_POINT('Ctrl Pts',(3.42506189818271,6.12028912847709,37.5640660429202));
#152057=CARTESIAN_POINT('Ctrl Pts',(3.57736720696016,6.02993121263138,37.556042925217));
#152058=CARTESIAN_POINT('Ctrl Pts',(3.72965330870442,5.93958469171012,37.5480208192992));
#152059=CARTESIAN_POINT('Ctrl Pts',(3.87853435245044,5.84345375425896,37.5399987133815));
#152060=CARTESIAN_POINT('Ctrl Pts',(4.02354555772512,5.74183835608514,37.5319766074637));
#152061=CARTESIAN_POINT('Ctrl Pts',(4.168610649654,5.64018519728577,37.5239515205042));
#152062=CARTESIAN_POINT('Ctrl Pts',(4.30980272814773,5.53304371449926,37.5159264335448));
#152063=CARTESIAN_POINT('Ctrl Pts',(4.44668704903017,5.42075648323068,37.5079013465853));
#152064=CARTESIAN_POINT('Ctrl Pts',(4.58359832859468,5.30844713755373,37.4998746791251));
#152065=CARTESIAN_POINT('Ctrl Pts',(4.71619988259121,5.19099026376917,37.4918480116649));
#152066=CARTESIAN_POINT('Ctrl Pts',(4.84409154499778,5.06876747012339,37.4838213442047));
#152067=CARTESIAN_POINT('Ctrl Pts',(4.97208587838034,4.94644655644947,37.4757882329642));
#152068=CARTESIAN_POINT('Ctrl Pts',(5.09536250986243,4.81935234124115,37.4677551217237));
#152069=CARTESIAN_POINT('Ctrl Pts',(5.2135590791038,4.68790233379434,37.4597220104831));
#152070=CARTESIAN_POINT('Ctrl Pts',(5.28320479143095,4.6104472142185,37.4549886095211));
#152071=CARTESIAN_POINT('Ctrl Pts',(5.3510874609904,4.53148040746574,37.4502552085592));
#152072=CARTESIAN_POINT('Ctrl Pts',(5.41713974441532,4.45109239984702,37.4455218075972));
#152073=CARTESIAN_POINT('Ctrl Pts',(5.55327203889334,4.28541449503861,37.4357663729592));
#152074=CARTESIAN_POINT('Ctrl Pts',(5.68170806712042,4.1136009511796,37.4260109383213));
#152075=CARTESIAN_POINT('Ctrl Pts',(5.8019809021497,3.93632368760373,37.4162555036833));
#152076=CARTESIAN_POINT('Ctrl Pts',(5.92237218882039,3.75887183112954,37.4064904613293));
#152077=CARTESIAN_POINT('Ctrl Pts',(6.03458419037899,3.5759455307003,37.3967254189754));
#152078=CARTESIAN_POINT('Ctrl Pts',(6.13819351279977,3.38824541052192,37.3869603766214));
#152079=CARTESIAN_POINT('Ctrl Pts',(6.24164532400683,3.20083063989562,37.3772101794921));
#152080=CARTESIAN_POINT('Ctrl Pts',(6.33652057679012,3.00865658784191,37.3674599823628));
#152081=CARTESIAN_POINT('Ctrl Pts',(6.42244268309691,2.81244671857709,37.3577097852336));
#152082=CARTESIAN_POINT('Ctrl Pts',(6.47542855231128,2.69144933014814,37.3516970989516));
#152083=CARTESIAN_POINT('Ctrl Pts',(6.52501054568903,2.56891768540196,37.3456844126697));
#152084=CARTESIAN_POINT('Ctrl Pts',(6.57110895151815,2.44502632087632,37.3396717263878));
#152085=CARTESIAN_POINT('Origin',(0.,0.,50.));
#152086=CARTESIAN_POINT('',(6.57110895151813,2.44502632087638,35.339859805629));
#152087=CARTESIAN_POINT('',(6.57110895151814,2.44502632087637,35.887150555484));
#152088=CARTESIAN_POINT('',(6.57110895151814,2.44502632087636,50.));
#152089=CARTESIAN_POINT('',(7.01124977383073,0.0017808589384362,37.7735343569413));
#152090=CARTESIAN_POINT('Ctrl Pts',(6.57110895151814,2.44502632087637,35.887150555484));
#152091=CARTESIAN_POINT('Ctrl Pts',(6.50697260986517,2.61739538093721,35.8955166861323));
#152092=CARTESIAN_POINT('Ctrl Pts',(6.43598672426158,2.7874094371462,35.9038828167805));
#152093=CARTESIAN_POINT('Ctrl Pts',(6.35834255681135,2.95450613347506,35.9122489474287));
#152094=CARTESIAN_POINT('Ctrl Pts',(6.28080917678768,3.12136440606158,35.9206031407723));
#152095=CARTESIAN_POINT('Ctrl Pts',(6.19663660155576,3.28531332604793,35.9289573341158));
#152096=CARTESIAN_POINT('Ctrl Pts',(6.10606457648596,3.4458093316786,35.9373115274593));
#152097=CARTESIAN_POINT('Ctrl Pts',(6.01556812576292,3.60617141758325,35.9456587499672));
#152098=CARTESIAN_POINT('Ctrl Pts',(5.91868302593814,3.76308604655054,35.9540059724751));
#152099=CARTESIAN_POINT('Ctrl Pts',(5.81569599752269,3.91603200023935,35.9623531949829));
#152100=CARTESIAN_POINT('Ctrl Pts',(5.71280280293965,4.06883860137854,35.9706928121458));
#152101=CARTESIAN_POINT('Ctrl Pts',(5.60381895001064,4.21768346804293,35.9790324293087));
#152102=CARTESIAN_POINT('Ctrl Pts',(5.48907577094334,4.36207218456352,35.9873720464716));
#152103=CARTESIAN_POINT('Ctrl Pts',(5.38980949117741,4.48698532402578,35.9945867914103));
#152104=CARTESIAN_POINT('Ctrl Pts',(5.28623355591924,4.60856365262259,36.0018015363491));
#152105=CARTESIAN_POINT('Ctrl Pts',(5.17858847666944,4.72650483463273,36.0090162812878));
#152106=CARTESIAN_POINT('Ctrl Pts',(5.05417963327136,4.86281321161698,36.0173545915896));
#152107=CARTESIAN_POINT('Ctrl Pts',(4.92443695717153,4.99415069566618,36.0256929018913));
#152108=CARTESIAN_POINT('Ctrl Pts',(4.78979374023273,5.12010766376327,36.0340312121931));
#152109=CARTESIAN_POINT('Ctrl Pts',(4.6550658103508,5.24614387971047,36.0423747686768));
#152110=CARTESIAN_POINT('Ctrl Pts',(4.51543142896972,5.36679260359018,36.0507183251604));
#152111=CARTESIAN_POINT('Ctrl Pts',(4.37135764285955,5.48168394936387,36.0590618816441));
#152112=CARTESIAN_POINT('Ctrl Pts',(4.22717424604053,5.59666270397291,36.0674117858691));
#152113=CARTESIAN_POINT('Ctrl Pts',(4.07854496340376,5.70587513937817,36.0757616900942));
#152114=CARTESIAN_POINT('Ctrl Pts',(3.92596687288046,5.80899394693653,36.0841115943193));
#152115=CARTESIAN_POINT('Ctrl Pts',(3.77315992651249,5.91226742507521,36.0924740227828));
#152116=CARTESIAN_POINT('Ctrl Pts',(3.61639260810419,6.00942882716261,36.1008364512463));
#152117=CARTESIAN_POINT('Ctrl Pts',(3.45618901935108,6.10019540875676,36.1091988797098));
#152118=CARTESIAN_POINT('Ctrl Pts',(3.29584843469025,6.19103960815168,36.1175684591896));
#152119=CARTESIAN_POINT('Ctrl Pts',(3.13206600719092,6.27547792630944,36.1259380386695));
#152120=CARTESIAN_POINT('Ctrl Pts',(2.96538749692936,6.35327502596535,36.1343076181493));
#152121=CARTESIAN_POINT('Ctrl Pts',(2.79845190537391,6.43119211816865,36.1426901066857));
#152122=CARTESIAN_POINT('Ctrl Pts',(2.62861160649927,6.50244739624754,36.1510725952221));
#152123=CARTESIAN_POINT('Ctrl Pts',(2.45643057633427,6.56685429914126,36.1594550837585));
#152124=CARTESIAN_POINT('Ctrl Pts',(2.40009012189321,6.58792929314436,36.1621979713637));
#152125=CARTESIAN_POINT('Ctrl Pts',(2.34349914850339,6.60827143021347,36.1649408589689));
#152126=CARTESIAN_POINT('Ctrl Pts',(2.28667769040872,6.62787535358708,36.1676837465741));
#152127=CARTESIAN_POINT('Ctrl Pts',(2.11287406792392,6.68783919491568,36.176073601707));
#152128=CARTESIAN_POINT('Ctrl Pts',(1.93656216285418,6.74101356882624,36.1844634568398));
#152129=CARTESIAN_POINT('Ctrl Pts',(1.7582991684868,6.78719460429702,36.1928533119726));
#152130=CARTESIAN_POINT('Ctrl Pts',(1.58020067271138,6.83333302455573,36.2012354250648));
#152131=CARTESIAN_POINT('Ctrl Pts',(1.40015499349404,6.87249088908847,36.2096175381569));
#152132=CARTESIAN_POINT('Ctrl Pts',(1.21873558913368,6.90451375016945,36.2179996512491));
#152133=CARTESIAN_POINT('Ctrl Pts',(1.03745692778057,6.93651176829725,36.226375261598));
#152134=CARTESIAN_POINT('Ctrl Pts',(0.85480698856528,6.96138576164031,36.2347508719469));
#152135=CARTESIAN_POINT('Ctrl Pts',(0.671371010187525,6.97903199084084,
36.2431264822958));
#152136=CARTESIAN_POINT('Ctrl Pts',(0.488050415764371,6.99666712030114,
36.2514968242614));
#152137=CARTESIAN_POINT('Ctrl Pts',(0.303945094401395,7.00708351927838,
36.2598671662271));
#152138=CARTESIAN_POINT('Ctrl Pts',(0.119647482316103,7.01022902924544,
36.2682375081927));
#152139=CARTESIAN_POINT('Ctrl Pts',(-0.0645612197947758,7.01337302173646,
36.276603812087));
#152140=CARTESIAN_POINT('Ctrl Pts',(-0.248961699547538,7.00925311447268,
36.2849701159814));
#152141=CARTESIAN_POINT('Ctrl Pts',(-0.432958966321623,6.99786918254276,
36.2933364198758));
#152142=CARTESIAN_POINT('Ctrl Pts',(-0.616904774217498,6.98648843437953,
36.3017003839494));
#152143=CARTESIAN_POINT('Ctrl Pts',(-0.800447266164052,6.9678477312557,
36.3100643480231));
#152144=CARTESIAN_POINT('Ctrl Pts',(-0.982993461921201,6.9419990216306,
36.3184283120968));
#152145=CARTESIAN_POINT('Ctrl Pts',(-1.16551156685233,6.91615428969236,
36.3267909890953));
#152146=CARTESIAN_POINT('Ctrl Pts',(-1.34703335595318,6.88310380882598,
36.3351536660939));
#152147=CARTESIAN_POINT('Ctrl Pts',(-1.5269725464287,6.8429512204131,36.3435163430925));
#152148=CARTESIAN_POINT('Ctrl Pts',(-1.70690803228521,6.8027994586686,36.3518788479189));
#152149=CARTESIAN_POINT('Ctrl Pts',(-1.88526066381444,6.7555459529077,36.3602413527452));
#152150=CARTESIAN_POINT('Ctrl Pts',(-2.06145547495954,6.70134522967287,
36.3686038575716));
#152151=CARTESIAN_POINT('Ctrl Pts',(-2.2376701440898,6.64713839776123,36.3769673048916));
#152152=CARTESIAN_POINT('Ctrl Pts',(-2.41172619401986,6.58598288446914,
36.3853307522116));
#152153=CARTESIAN_POINT('Ctrl Pts',(-2.58306450104343,6.51808287351037,
36.3936941995317));
#152154=CARTESIAN_POINT('Ctrl Pts',(-2.75450369687716,6.45014288111702,
36.4020625714845));
#152155=CARTESIAN_POINT('Ctrl Pts',(-2.92322164584411,6.3754505756709,36.4104309434374));
#152156=CARTESIAN_POINT('Ctrl Pts',(-3.08867890971672,6.29425842773961,
36.4187993153902));
#152157=CARTESIAN_POINT('Ctrl Pts',(-3.25418574890983,6.21304195251884,
36.427170194726));
#152158=CARTESIAN_POINT('Ctrl Pts',(-3.4164296621465,6.12532190106307,36.4355410740618));
#152159=CARTESIAN_POINT('Ctrl Pts',(-3.57489582796128,6.03139671898019,
36.4439119533976));
#152160=CARTESIAN_POINT('Ctrl Pts',(-3.73349626044479,5.93739195510619,
36.4522899252889));
#152161=CARTESIAN_POINT('Ctrl Pts',(-3.88831226944412,5.83717172743768,
36.4606678971803));
#152162=CARTESIAN_POINT('Ctrl Pts',(-4.03885706119026,5.73107845014999,
36.4690458690716));
#152163=CARTESIAN_POINT('Ctrl Pts',(-4.13452950222651,5.66365530851938,
36.4743701384301));
#152164=CARTESIAN_POINT('Ctrl Pts',(-4.22847752743682,5.59386107507974,
36.4796944077886));
#152165=CARTESIAN_POINT('Ctrl Pts',(-4.32058308092259,5.52179213691945,
36.4850186771471));
#152166=CARTESIAN_POINT('Ctrl Pts',(-4.45660370082115,5.41536140312544,
36.4928815083364));
#152167=CARTESIAN_POINT('Ctrl Pts',(-4.58888712415335,5.30374629795429,
36.5007443395257));
#152168=CARTESIAN_POINT('Ctrl Pts',(-4.71699660523404,5.18725067725771,
36.5086071707149));
#152169=CARTESIAN_POINT('Ctrl Pts',(-4.84500765108876,5.0708445680684,36.5164639603563));
#152170=CARTESIAN_POINT('Ctrl Pts',(-4.96885085225944,4.94956565568369,
36.5243207499977));
#152171=CARTESIAN_POINT('Ctrl Pts',(-5.08812047633207,4.82375958986664,
36.532177539639));
#152172=CARTESIAN_POINT('Ctrl Pts',(-5.20732283798267,4.69802447271534,
36.540029898423));
#152173=CARTESIAN_POINT('Ctrl Pts',(-5.32195649181786,4.56776755666268,
36.5478822572069));
#152174=CARTESIAN_POINT('Ctrl Pts',(-5.43165089414721,4.43337288377707,
36.5557346159909));
#152175=CARTESIAN_POINT('Ctrl Pts',(-5.54131939634823,4.29900994304188,
36.5635851207413));
#152176=CARTESIAN_POINT('Ctrl Pts',(-5.64605072073049,4.16051147969021,
36.5714356254917));
#152177=CARTESIAN_POINT('Ctrl Pts',(-5.74551318439922,4.01829625717103,
36.5792861302421));
#152178=CARTESIAN_POINT('Ctrl Pts',(-5.84495964769236,3.87610391259889,
36.5871353720937));
#152179=CARTESIAN_POINT('Ctrl Pts',(-5.93913872138399,3.73019631349701,
36.5949846139453));
#152180=CARTESIAN_POINT('Ctrl Pts',(-6.02776109465621,3.58102258415791,
36.6028338557969));
#152181=CARTESIAN_POINT('Ctrl Pts',(-6.11641332654064,3.43179859526953,
36.6106857422118));
#152182=CARTESIAN_POINT('Ctrl Pts',(-6.19950492344001,3.27930660641339,
36.6185376286266));
#152183=CARTESIAN_POINT('Ctrl Pts',(-6.27679163657645,3.12402197711604,
36.6263895150414));
#152184=CARTESIAN_POINT('Ctrl Pts',(-6.33354230806458,3.00999840661106,
36.6321550575054));
#152185=CARTESIAN_POINT('Ctrl Pts',(-6.3871640476193,2.89446966478179,36.6379205999694));
#152186=CARTESIAN_POINT('Ctrl Pts',(-6.43757652936217,2.77763118341966,
36.6436861424334));
#152187=CARTESIAN_POINT('Ctrl Pts',(-6.52200013005698,2.58196683690696,
36.6533414467934));
#152188=CARTESIAN_POINT('Ctrl Pts',(-6.59737977147376,2.38272892649935,
36.6629967511533));
#152189=CARTESIAN_POINT('Ctrl Pts',(-6.66349814332539,2.18069233419095,
36.6726520555133));
#152190=CARTESIAN_POINT('Ctrl Pts',(-6.72998279855346,1.9775364970626,36.6823608484481));
#152191=CARTESIAN_POINT('Ctrl Pts',(-6.78710332593054,1.77155094565415,
36.6920696413829));
#152192=CARTESIAN_POINT('Ctrl Pts',(-6.83469119428504,1.56352897039438,
36.7017784343178));
#152193=CARTESIAN_POINT('Ctrl Pts',(-6.88250805950276,1.35450597572647,
36.7115339467886));
#152194=CARTESIAN_POINT('Ctrl Pts',(-6.92070031477104,1.14342695868886,
36.7212894592593));
#152195=CARTESIAN_POINT('Ctrl Pts',(-6.94914935517812,0.931101391862117,
36.7310449717301));
#152196=CARTESIAN_POINT('Ctrl Pts',(-6.97762656451199,0.71856559005865,
36.7408101436591));
#152197=CARTESIAN_POINT('Ctrl Pts',(-6.9963412682042,0.504780809117193,
36.7505753155881));
#152198=CARTESIAN_POINT('Ctrl Pts',(-7.00522660158058,0.290562941559598,
36.7603404875171));
#152199=CARTESIAN_POINT('Ctrl Pts',(-7.01409982000649,0.0766371552045,36.7700923448557));
#152200=CARTESIAN_POINT('Ctrl Pts',(-7.01317045261364,-0.13772049964646,
36.7798442021943));
#152201=CARTESIAN_POINT('Ctrl Pts',(-7.00242371329551,-0.351694045978458,
36.789596059533));
#152202=CARTESIAN_POINT('Ctrl Pts',(-6.99773735663737,-0.445002008871643,
36.7938485755953));
#152203=CARTESIAN_POINT('Ctrl Pts',(-6.99118480247846,-0.538236889470219,
36.7981010916576));
#152204=CARTESIAN_POINT('Ctrl Pts',(-6.98276792694817,-0.631330848988084,
36.80235360772));
#152205=CARTESIAN_POINT('Ctrl Pts',(-6.96686836444377,-0.807186274532689,
36.8103866533187));
#152206=CARTESIAN_POINT('Ctrl Pts',(-6.94430472223209,-0.982624320124002,
36.8184196989175));
#152207=CARTESIAN_POINT('Ctrl Pts',(-6.91511093451619,-1.15709434612508,
36.8264527445163));
#152208=CARTESIAN_POINT('Ctrl Pts',(-6.8859359136911,-1.33145221607574,
36.834480626164));
#152209=CARTESIAN_POINT('Ctrl Pts',(-6.85013929144488,-1.50484294506531,
36.8425085078118));
#152210=CARTESIAN_POINT('Ctrl Pts',(-6.80780683283171,-1.67672081437247,
36.8505363894595));
#152211=CARTESIAN_POINT('Ctrl Pts',(-6.7654934877409,-1.84852107912734,
36.8585606464396));
#152212=CARTESIAN_POINT('Ctrl Pts',(-6.71665026953412,-2.01880948907865,
36.8665849034197));
#152213=CARTESIAN_POINT('Ctrl Pts',(-6.66141405653836,-2.18705037204293,
36.8746091603997));
#152214=CARTESIAN_POINT('Ctrl Pts',(-6.60618452216337,-2.35527091297083,
36.8826324471654));
#152215=CARTESIAN_POINT('Ctrl Pts',(-6.54456363959391,-2.52144406954191,
36.890655733931));
#152216=CARTESIAN_POINT('Ctrl Pts',(-6.47673824465091,-2.68504902614017,
36.8986790206967));
#152217=CARTESIAN_POINT('Ctrl Pts',(-6.408918407394,-2.84864057677166,36.9067016500256));
#152218=CARTESIAN_POINT('Ctrl Pts',(-6.33489521457951,-3.00966400945426,
36.9147242793545));
#152219=CARTESIAN_POINT('Ctrl Pts',(-6.25490365127451,-3.16761848646153,
36.9227469086833));
#152220=CARTESIAN_POINT('Ctrl Pts',(-6.17488201683647,-3.32563234310704,
36.9307725539497));
#152221=CARTESIAN_POINT('Ctrl Pts',(-6.08888769818116,-3.48057461346246,
36.9387981992161));
#152222=CARTESIAN_POINT('Ctrl Pts',(-5.99720182275231,-3.63196873054771,
36.9468238444824));
#152223=CARTESIAN_POINT('Ctrl Pts',(-5.94313824353517,-3.72123992748797,
36.9515562539904));
#152224=CARTESIAN_POINT('Ctrl Pts',(-5.88709656573008,-3.80927792587232,
36.9562886634983));
#152225=CARTESIAN_POINT('Ctrl Pts',(-5.8291414931858,-3.89598973496076,
36.9610210730063));
#152226=CARTESIAN_POINT('Ctrl Pts',(-5.72222965204426,-4.05595017934251,
36.9697511218411));
#152227=CARTESIAN_POINT('Ctrl Pts',(-5.60875089323653,-4.21147602253064,
36.9784811706758));
#152228=CARTESIAN_POINT('Ctrl Pts',(-5.48909361083986,-4.36204973538095,
36.9872112195106));
#152229=CARTESIAN_POINT('Ctrl Pts',(-5.36940172939094,-4.51266698680788,
36.9959437926498));
#152230=CARTESIAN_POINT('Ctrl Pts',(-5.24352792878021,-4.65832903524911,
37.0046763657891));
#152231=CARTESIAN_POINT('Ctrl Pts',(-5.11190092571569,-4.79855139476146,
37.0134089389283));
#152232=CARTESIAN_POINT('Ctrl Pts',(-4.97840395095815,-4.94076583672582,
37.0222655722087));
#152233=CARTESIAN_POINT('Ctrl Pts',(-4.83898925941136,-5.07738464154304,
37.031122205489));
#152234=CARTESIAN_POINT('Ctrl Pts',(-4.69414314873293,-5.20794073139314,
37.0399788387694));
#152235=CARTESIAN_POINT('Ctrl Pts',(-4.55123506953378,-5.33674998930722,
37.0487169708763));
#152236=CARTESIAN_POINT('Ctrl Pts',(-4.40304023446243,-5.45965759341299,
37.0574551029831));
#152237=CARTESIAN_POINT('Ctrl Pts',(-4.2500601198248,-5.57625461581291,
37.0661932350899));
#152238=CARTESIAN_POINT('Ctrl Pts',(-4.09396807184302,-5.69522346387589,
37.0751091189571));
#152239=CARTESIAN_POINT('Ctrl Pts',(-3.93289420716951,-5.80762205691641,
37.0840250028242));
#152240=CARTESIAN_POINT('Ctrl Pts',(-3.76740442870148,-5.91306100366811,
37.0929408866914));
#152241=CARTESIAN_POINT('Ctrl Pts',(-3.60191465023345,-6.0184999504198,
37.1018567705585));
#152242=CARTESIAN_POINT('Ctrl Pts',(-3.43200921628418,-6.1169790935156,
37.1107726544257));
#152243=CARTESIAN_POINT('Ctrl Pts',(-3.25828380186181,-6.20815699133204,
37.1196885382928));
#152244=CARTESIAN_POINT('Ctrl Pts',(-3.08797213573322,-6.29754322041576,
37.128429222789));
#152245=CARTESIAN_POINT('Ctrl Pts',(-2.91397113395903,-6.37992197705981,
37.1371699072851));
#152246=CARTESIAN_POINT('Ctrl Pts',(-2.73686415548148,-6.45501364498486,
37.1459105917812));
#152247=CARTESIAN_POINT('Ctrl Pts',(-2.55978904149134,-6.53009180267147,
37.154649703683));
#152248=CARTESIAN_POINT('Ctrl Pts',(-2.37960931878053,-6.59788538310423,
37.1633888155848));
#152249=CARTESIAN_POINT('Ctrl Pts',(-2.19692892241399,-6.6581626498878,
37.1721279274866));
#152250=CARTESIAN_POINT('Ctrl Pts',(-2.01188163858686,-6.71922089541757,
37.180980267161));
#152251=CARTESIAN_POINT('Ctrl Pts',(-1.82426869335081,-6.77256658958483,
37.1898326068354));
#152252=CARTESIAN_POINT('Ctrl Pts',(-1.63473565426649,-6.81801040650203,
37.1986849465098));
#152253=CARTESIAN_POINT('Ctrl Pts',(-1.44772278170734,-6.86284997000397,
37.2074195791594));
#152254=CARTESIAN_POINT('Ctrl Pts',(-1.25884083652015,-6.89999643726298,
37.2161542118091));
#152255=CARTESIAN_POINT('Ctrl Pts',(-1.06872316363582,-6.92931867949572,
37.2248888444588));
#152256=CARTESIAN_POINT('Ctrl Pts',(-0.874762481001771,-6.95923363707719,
37.2338000376455));
#152257=CARTESIAN_POINT('Ctrl Pts',(-0.679515864651398,-6.98100461965341,
37.2427112308323));
#152258=CARTESIAN_POINT('Ctrl Pts',(-0.483665567513508,-6.99454746079415,
37.251622424019));
#152259=CARTESIAN_POINT('Ctrl Pts',(-0.287815270375584,-7.00809030193489,
37.2605336172057));
#152260=CARTESIAN_POINT('Ctrl Pts',(-0.0913615939282992,-7.01340496728706,
37.2694448103925));
#152261=CARTESIAN_POINT('Ctrl Pts',(0.105007858586513,-7.01046360179804,
37.2783560035792));
#152262=CARTESIAN_POINT('Ctrl Pts',(0.2818635702861,-7.00781452741163,37.2863816684316));
#152263=CARTESIAN_POINT('Ctrl Pts',(0.458732234533989,-6.99846700358845,
37.294407333284));
#152264=CARTESIAN_POINT('Ctrl Pts',(0.635061200238224,-6.98242965123545,
37.3024329981364));
#152265=CARTESIAN_POINT('Ctrl Pts',(0.811334203453862,-6.96639738874471,
37.3104561158397));
#152266=CARTESIAN_POINT('Ctrl Pts',(0.987067484512773,-6.94367955795455,
37.3184792335429));
#152267=CARTESIAN_POINT('Ctrl Pts',(1.16171130125491,-6.91433680225636,
37.3265023512461));
#152268=CARTESIAN_POINT('Ctrl Pts',(1.33633309388306,-6.8849977469365,37.334524457164));
#152269=CARTESIAN_POINT('Ctrl Pts',(1.50986533455861,-6.84903549215509,
37.3425465630818));
#152270=CARTESIAN_POINT('Ctrl Pts',(1.68176633951627,-6.80656216762692,
37.3505686689997));
#152271=CARTESIAN_POINT('Ctrl Pts',(1.85373122346835,-6.7640730598678,37.3585937559592));
#152272=CARTESIAN_POINT('Ctrl Pts',(2.02406330383963,-6.71506813399237,
37.3666188429188));
#152273=CARTESIAN_POINT('Ctrl Pts',(2.19223353943437,-6.65971010413209,
37.3746439298783));
#152274=CARTESIAN_POINT('Ctrl Pts',(2.36043689531531,-6.6043411717849,37.3826705973385));
#152275=CARTESIAN_POINT('Ctrl Pts',(2.52647721279758,-6.54261676581433,
37.3906972647988));
#152276=CARTESIAN_POINT('Ctrl Pts',(2.68984362313821,-6.47474847739762,
37.398723932259));
#152277=CARTESIAN_POINT('Ctrl Pts',(2.85334118345751,-6.40682570455806,
37.4067570434996));
#152278=CARTESIAN_POINT('Ctrl Pts',(3.01416021444236,-6.33274934744867,
37.4147901547402));
#152279=CARTESIAN_POINT('Ctrl Pts',(3.17181215961908,-6.25277811749246,
37.4228232659808));
#152280=CARTESIAN_POINT('Ctrl Pts',(3.26470641273613,-6.20565616368906,
37.4275566669424));
#152281=CARTESIAN_POINT('Ctrl Pts',(3.35650152545842,-6.15648838283711,
37.432290067904));
#152282=CARTESIAN_POINT('Ctrl Pts',(3.44710205084209,-6.10533488136239,
37.4370234688657));
#152283=CARTESIAN_POINT('Ctrl Pts',(3.63374195281166,-5.99995707631974,
37.44677442216));
#152284=CARTESIAN_POINT('Ctrl Pts',(3.81542117581783,-5.886088554131,37.4565253754544));
#152285=CARTESIAN_POINT('Ctrl Pts',(3.99146280133737,-5.76418695637469,
37.4662763287487));
#152286=CARTESIAN_POINT('Ctrl Pts',(4.16775804784398,-5.64210973649799,
37.4760413301206));
#152287=CARTESIAN_POINT('Ctrl Pts',(4.33839941867826,-5.51197631333704,
37.4858063314925));
#152288=CARTESIAN_POINT('Ctrl Pts',(4.50273931168685,-5.37428741820624,
37.4955713328643));
#152289=CARTESIAN_POINT('Ctrl Pts',(4.66680528414372,-5.23682802193557,
37.5053200580021));
#152290=CARTESIAN_POINT('Ctrl Pts',(4.82459074146358,-5.09183834714575,
37.5150687831399));
#152291=CARTESIAN_POINT('Ctrl Pts',(4.97548376543074,-4.93985706902894,
37.5248175082777));
#152292=CARTESIAN_POINT('Ctrl Pts',(5.12596264655483,-4.78829292059088,
37.5345394769451));
#152293=CARTESIAN_POINT('Ctrl Pts',(5.26958683100278,-4.62977550534586,
37.5442614456124));
#152294=CARTESIAN_POINT('Ctrl Pts',(5.4057822498977,-4.46487903858447,37.5539834142797));
#152295=CARTESIAN_POINT('Ctrl Pts',(5.54107649927796,-4.3010736486752,37.5636410552196));
#152296=CARTESIAN_POINT('Ctrl Pts',(5.66903991458593,-4.13097336285851,
37.5732986961594));
#152297=CARTESIAN_POINT('Ctrl Pts',(5.78914287372278,-3.95518031828194,
37.5829563370993));
#152298=CARTESIAN_POINT('Ctrl Pts',(5.8419322591425,-3.87791322302506,37.5872012027836));
#152299=CARTESIAN_POINT('Ctrl Pts',(5.89320351584413,-3.79954685122038,
37.5914460684679));
#152300=CARTESIAN_POINT('Ctrl Pts',(5.94291376581705,-3.7201347468287,37.5956909341521));
#152301=CARTESIAN_POINT('Ctrl Pts',(6.03486420826598,-3.57324395190023,
37.6035427811659));
#152302=CARTESIAN_POINT('Ctrl Pts',(6.12143268792315,-3.42283350555081,
37.6113946281797));
#152303=CARTESIAN_POINT('Ctrl Pts',(6.2023340012452,-3.26935459984042,37.6192464751936));
#152304=CARTESIAN_POINT('Ctrl Pts',(6.28321237160885,-3.11591921950686,
37.627096095487));
#152305=CARTESIAN_POINT('Ctrl Pts',(6.35842659485689,-2.95941744788961,
37.6349457157805));
#152306=CARTESIAN_POINT('Ctrl Pts',(6.4277366444663,-2.80032644380706,37.642795336074));
#152307=CARTESIAN_POINT('Ctrl Pts',(6.49704116055462,-2.64124814110666,
37.6506443296757));
#152308=CARTESIAN_POINT('Ctrl Pts',(6.56044228970657,-2.47958136747388,
37.6584933232774));
#152309=CARTESIAN_POINT('Ctrl Pts',(6.61774763083798,-2.31582444434768,
37.666342316879));
#152310=CARTESIAN_POINT('Ctrl Pts',(6.67508198398568,-2.15198461588623,
37.6741952841964));
#152311=CARTESIAN_POINT('Ctrl Pts',(6.72631425673012,-1.98605288415579,
37.6820482515137));
#152312=CARTESIAN_POINT('Ctrl Pts',(6.77130144301954,-1.81854428878197,
37.689901218831));
#152313=CARTESIAN_POINT('Ctrl Pts',(6.81630005454276,-1.65099315185304,
37.6977561805382));
#152314=CARTESIAN_POINT('Ctrl Pts',(6.8550503346414,-1.48186472532357,37.7056111422453));
#152315=CARTESIAN_POINT('Ctrl Pts',(6.88746030029639,-1.31168486091027,
37.7134661039525));
#152316=CARTESIAN_POINT('Ctrl Pts',(6.91990243555138,-1.14133607875651,
37.7213288623657));
#152317=CARTESIAN_POINT('Ctrl Pts',(6.94599162967876,-0.96993415126066,
37.729191620779));
#152318=CARTESIAN_POINT('Ctrl Pts',(6.96568766127409,-0.798011258112235,
37.7370543791922));
#152319=CARTESIAN_POINT('Ctrl Pts',(6.98013638743281,-0.67189109063118,
37.742822385941));
#152320=CARTESIAN_POINT('Ctrl Pts',(6.99114573199519,-0.545490689697603,
37.7485903926897));
#152321=CARTESIAN_POINT('Ctrl Pts',(6.99871765569711,-0.419019973669059,
37.7543583994384));
#152322=CARTESIAN_POINT('Ctrl Pts',(7.00710870499226,-0.278867740978047,
37.7607503852625));
#152323=CARTESIAN_POINT('Ctrl Pts',(7.01128541614013,-0.138543129237301,
37.7671423710865));
#152324=CARTESIAN_POINT('Ctrl Pts',(7.0112497738309,0.00178085826187677,
37.7735343569105));
#152325=CARTESIAN_POINT('Ctrl Pts',(7.01124977383073,0.00178085893843706,
37.7735343569413));
#152326=CARTESIAN_POINT('Ctrl Pts',(7.01120348839179,0.184006843444352,
37.7818350468696));
#152327=CARTESIAN_POINT('Ctrl Pts',(7.00404861198355,0.366382945871945,
37.7901357367978));
#152328=CARTESIAN_POINT('Ctrl Pts',(6.98977578673226,0.548325645680976,
37.7984364267261));
#152329=CARTESIAN_POINT('Ctrl Pts',(6.97551647180639,0.730096122749284,
37.8067292594137));
#152330=CARTESIAN_POINT('Ctrl Pts',(6.95415267047731,0.911433679039336,
37.8150220921014));
#152331=CARTESIAN_POINT('Ctrl Pts',(6.92572706700787,1.09175599646377,37.8233149247891));
#152332=CARTESIAN_POINT('Ctrl Pts',(6.89731729855115,1.27197786197714,37.8316031377995));
#152333=CARTESIAN_POINT('Ctrl Pts',(6.86185361922219,1.45118528206985,37.83989135081));
#152334=CARTESIAN_POINT('Ctrl Pts',(6.81943048606037,1.62880152513757,37.8481795638205));
#152335=CARTESIAN_POINT('Ctrl Pts',(6.7770261656842,1.80633900324712,37.8564641013746));
#152336=CARTESIAN_POINT('Ctrl Pts',(6.72766862248195,1.98228638225756,37.8647486389288));
#152337=CARTESIAN_POINT('Ctrl Pts',(6.67150335974477,2.15607733706709,37.8730331764829));
#152338=CARTESIAN_POINT('Ctrl Pts',(6.64014858575329,2.25309773444892,37.8776580956941));
#152339=CARTESIAN_POINT('Ctrl Pts',(6.60667307426906,2.34944627604572,37.8822830149052));
#152340=CARTESIAN_POINT('Ctrl Pts',(6.57110895151815,2.44502632087634,37.8869079341164));
#152341=CARTESIAN_POINT('',(7.01124996031773,-0.000745952192151278,37.2264656431214));
#152342=CARTESIAN_POINT('Ctrl Pts',(6.57110895151815,2.44502632087632,37.3396717263878));
#152343=CARTESIAN_POINT('Ctrl Pts',(6.64524608758582,2.24577971387883,37.3300019052085));
#152344=CARTESIAN_POINT('Ctrl Pts',(6.71037085531289,2.04301503505559,37.3203320840293));
#152345=CARTESIAN_POINT('Ctrl Pts',(6.7661879905331,1.83747833708746,37.31066226285));
#152346=CARTESIAN_POINT('Ctrl Pts',(6.81199683213143,1.66879540481726,37.3027262893369));
#152347=CARTESIAN_POINT('Ctrl Pts',(6.8515373949267,1.49824586114826,37.2947903158238));
#152348=CARTESIAN_POINT('Ctrl Pts',(6.88466960476146,1.32625449887027,37.2868543423107));
#152349=CARTESIAN_POINT('Ctrl Pts',(6.9159947625869,1.16364365598238,37.2793512018913));
#152350=CARTESIAN_POINT('Ctrl Pts',(6.94158734898268,0.999751854630932,
37.2718480614719));
#152351=CARTESIAN_POINT('Ctrl Pts',(6.96134279331623,0.835064713925977,
37.2643449210525));
#152352=CARTESIAN_POINT('Ctrl Pts',(6.98109422578551,0.67041101729056,37.2568433043437));
#152353=CARTESIAN_POINT('Ctrl Pts',(6.99501081379572,0.504962703640699,
37.2493416876349));
#152354=CARTESIAN_POINT('Ctrl Pts',(7.00303936527711,0.339214107724237,
37.2418400709261));
#152355=CARTESIAN_POINT('Ctrl Pts',(7.00852415564163,0.225981190936938,
37.2367152616579));
#152356=CARTESIAN_POINT('Ctrl Pts',(7.01126202048753,0.112608316228521,
37.2315904523896));
#152357=CARTESIAN_POINT('Ctrl Pts',(7.01124996031773,-0.000745952192208719,
37.2264656431214));
#152358=CARTESIAN_POINT('Ctrl Pts',(7.01124996031765,-0.000745952892359531,
37.2264656430897));
#152359=CARTESIAN_POINT('Ctrl Pts',(7.01123049451372,-0.183706054619841,
37.2181939155392));
#152360=CARTESIAN_POINT('Ctrl Pts',(7.00404513626149,-0.366557650698258,
37.2099221879888));
#152361=CARTESIAN_POINT('Ctrl Pts',(6.98974513960931,-0.548716179648486,
37.2016504604383));
#152362=CARTESIAN_POINT('Ctrl Pts',(6.97543598949301,-0.730991308735181,
37.1933734381341));
#152363=CARTESIAN_POINT('Ctrl Pts',(6.95400315525883,-0.912572151207703,
37.1850964158298));
#152364=CARTESIAN_POINT('Ctrl Pts',(6.92554947323097,-1.09288199561078,
37.1768193935256));
#152365=CARTESIAN_POINT('Ctrl Pts',(6.89705104070912,-1.2734754221036,37.1685293535445));
#152366=CARTESIAN_POINT('Ctrl Pts',(6.8615097511004,-1.45279352333023,37.1602393135635));
#152367=CARTESIAN_POINT('Ctrl Pts',(6.81907938420107,-1.63027081016129,
37.1519492735825));
#152368=CARTESIAN_POINT('Ctrl Pts',(6.77853887990636,-1.79984319981468,
37.1440284747298));
#152369=CARTESIAN_POINT('Ctrl Pts',(6.73170975518064,-1.96773496388468,
37.1361076758771));
#152370=CARTESIAN_POINT('Ctrl Pts',(6.67876767326906,-2.13346875510195,
37.1281868770244));
#152371=CARTESIAN_POINT('Ctrl Pts',(6.6227692458331,-2.30877035538027,37.1198088105833));
#152372=CARTESIAN_POINT('Ctrl Pts',(6.55982763905674,-2.48198229565792,
37.1114307441422));
#152373=CARTESIAN_POINT('Ctrl Pts',(6.49012093403737,-2.65253780822629,
37.1030526777011));
#152374=CARTESIAN_POINT('Ctrl Pts',(6.42046189363462,-2.82297669696172,
37.0946803400822));
#152375=CARTESIAN_POINT('Ctrl Pts',(6.3440471016209,-2.99076247609817,37.0863080024634));
#152376=CARTESIAN_POINT('Ctrl Pts',(6.2611037241574,-3.15534573665745,37.0779356648446));
#152377=CARTESIAN_POINT('Ctrl Pts',(6.17820489868872,-3.31984059338274,
37.0695678243219));
#152378=CARTESIAN_POINT('Ctrl Pts',(6.08878462750169,-3.48113606853503,
37.0611999837992));
#152379=CARTESIAN_POINT('Ctrl Pts',(5.99311743063674,-3.63870444321851,
37.0528321432765));
#152380=CARTESIAN_POINT('Ctrl Pts',(5.89748760565659,-3.79621126464925,
37.0444675716064));
#152381=CARTESIAN_POINT('Ctrl Pts',(5.79561589170577,-3.94999360846245,
37.0361029999364));
#152382=CARTESIAN_POINT('Ctrl Pts',(5.68782204544913,-4.09954960231035,
37.0277384282664));
#152383=CARTESIAN_POINT('Ctrl Pts',(5.58005452987191,-4.24906906428684,
37.0193758998007));
#152384=CARTESIAN_POINT('Ctrl Pts',(5.46636795920961,-4.39436396892815,
37.011013371335));
#152385=CARTESIAN_POINT('Ctrl Pts',(5.34712484105499,-4.53496223762367,
37.0026508428694));
#152386=CARTESIAN_POINT('Ctrl Pts',(5.22787220692641,-4.67557172650098,
36.9942876470477));
#152387=CARTESIAN_POINT('Ctrl Pts',(5.10306234737544,-4.81148357605525,
36.9859244512261));
#152388=CARTESIAN_POINT('Ctrl Pts',(4.97309790550928,-4.94225897588535,
36.9775612554045));
#152389=CARTESIAN_POINT('Ctrl Pts',(4.84312460032866,-5.07304329433561,
36.9691974892297));
#152390=CARTESIAN_POINT('Ctrl Pts',(4.70799624350507,-5.19869023117873,
36.9608337230549));
#152391=CARTESIAN_POINT('Ctrl Pts',(4.56815228993548,-5.31879791103754,
36.9524699568801));
#152392=CARTESIAN_POINT('Ctrl Pts',(4.42828015480015,-5.43892979517825,
36.9441045052264));
#152393=CARTESIAN_POINT('Ctrl Pts',(4.28369077743742,-5.55351998223701,
36.9357390535728));
#152394=CARTESIAN_POINT('Ctrl Pts',(4.1348569514438,-5.66220668587759,36.9273736019191));
#152395=CARTESIAN_POINT('Ctrl Pts',(3.98597328129447,-5.77092978848154,
36.9190053486921));
#152396=CARTESIAN_POINT('Ctrl Pts',(3.83284259350427,-5.87374527152244,
36.9106370954652));
#152397=CARTESIAN_POINT('Ctrl Pts',(3.67596727293508,-5.97033425955451,
36.9022688422382));
#152398=CARTESIAN_POINT('Ctrl Pts',(3.51894650656299,-6.06701279935841,
36.8938928304466));
#152399=CARTESIAN_POINT('Ctrl Pts',(3.35817444996285,-6.1574531357209,36.885516818655));
#152400=CARTESIAN_POINT('Ctrl Pts',(3.19417982126245,-6.24138140413962,
36.8771408068635));
#152401=CARTESIAN_POINT('Ctrl Pts',(3.03010476756985,-6.32535083201817,
36.8687606873722));
#152402=CARTESIAN_POINT('Ctrl Pts',(2.86280428564977,-6.40280167943196,
36.860380567881));
#152403=CARTESIAN_POINT('Ctrl Pts',(2.69282834885489,-6.47350770804388,
36.8520004483897));
#152404=CARTESIAN_POINT('Ctrl Pts',(2.52265819302079,-6.54429452725006,
36.8436107535504));
#152405=CARTESIAN_POINT('Ctrl Pts',(2.3498067798204,-6.60832100757938,36.8352210587111));
#152406=CARTESIAN_POINT('Ctrl Pts',(2.17484182970063,-6.66540993325125,
36.8268313638718));
#152407=CARTESIAN_POINT('Ctrl Pts',(2.06375960221987,-6.70165470698321,
36.8215048913983));
#152408=CARTESIAN_POINT('Ctrl Pts',(1.95182576201224,-6.735104124186,36.8161784189248));
#152409=CARTESIAN_POINT('Ctrl Pts',(1.83918801382648,-6.76572346555023,
36.8108519464514));
#152410=CARTESIAN_POINT('Ctrl Pts',(1.66195048764573,-6.81390355085991,
36.8024706460465));
#152411=CARTESIAN_POINT('Ctrl Pts',(1.48261202794092,-6.8551711637321,36.7940893456417));
#152412=CARTESIAN_POINT('Ctrl Pts',(1.30173764763535,-6.88934725930032,
36.7857080452369));
#152413=CARTESIAN_POINT('Ctrl Pts',(1.12109249912861,-6.92348004167044,
36.7773373669034));
#152414=CARTESIAN_POINT('Ctrl Pts',(0.938915628646759,-6.95053915747116,
36.7689666885699));
#152415=CARTESIAN_POINT('Ctrl Pts',(0.755786438101931,-6.97039549971745,
36.7605960102364));
#152416=CARTESIAN_POINT('Ctrl Pts',(0.572865067746541,-6.99022930842446,
36.7522348311856));
#152417=CARTESIAN_POINT('Ctrl Pts',(0.388993855082819,-7.00287659997662,
36.7438736521349));
#152418=CARTESIAN_POINT('Ctrl Pts',(0.204762051816867,-7.00825934627392,
36.7355124730841));
#152419=CARTESIAN_POINT('Ctrl Pts',(0.020769311047764,-7.01363510782295,
36.7271621436494));
#152420=CARTESIAN_POINT('Ctrl Pts',(-0.163582761064816,-7.01176511695514,
36.7188118142148));
#152421=CARTESIAN_POINT('Ctrl Pts',(-0.347700215944274,-7.00262316009739,
36.7104614847801));
#152422=CARTESIAN_POINT('Ctrl Pts',(-0.531676003455989,-6.99348823742857,
36.7021175804244));
#152423=CARTESIAN_POINT('Ctrl Pts',(-0.715417207627831,-6.97709251544897,
36.6937736760688));
#152424=CARTESIAN_POINT('Ctrl Pts',(-0.898329147949554,-6.95346182159967,
36.6854297717131));
#152425=CARTESIAN_POINT('Ctrl Pts',(-1.08109417226004,-6.92985010807105,
36.6770925692335));
#152426=CARTESIAN_POINT('Ctrl Pts',(-1.26303093709266,-6.89901505409134,
36.6687553667538));
#152427=CARTESIAN_POINT('Ctrl Pts',(-1.44354899987888,-6.86103438611473,
36.6604181642742));
#152428=CARTESIAN_POINT('Ctrl Pts',(-1.50297454971891,-6.84853135986369,
36.6576736032378));
#152429=CARTESIAN_POINT('Ctrl Pts',(-1.56224639998774,-6.83525438800011,
36.6549290422014));
#152430=CARTESIAN_POINT('Ctrl Pts',(-1.62134364638561,-6.82120746956322,
36.6521844811651));
#152431=CARTESIAN_POINT('Ctrl Pts',(-1.80088827007163,-6.77853122255637,
36.6438461708632));
#152432=CARTESIAN_POINT('Ctrl Pts',(-1.97867313897385,-6.72877946772553,
36.6355078605612));
#152433=CARTESIAN_POINT('Ctrl Pts',(-2.15412987388545,-6.67213242141778,
36.6271695502593));
#152434=CARTESIAN_POINT('Ctrl Pts',(-2.32969700022063,-6.61544973471078,
36.6188259937755));
#152435=CARTESIAN_POINT('Ctrl Pts',(-2.50293275907081,-6.55186320394812,
36.6104824372917));
#152436=CARTESIAN_POINT('Ctrl Pts',(-2.67328714752828,-6.48160183823105,
36.6021388808078));
#152437=CARTESIAN_POINT('Ctrl Pts',(-2.84377114086221,-6.41128701797309,
36.5937889765826));
#152438=CARTESIAN_POINT('Ctrl Pts',(-3.01136908865483,-6.3342873582255,
36.5854390723574));
#152439=CARTESIAN_POINT('Ctrl Pts',(-3.17555365441934,-6.25087878225166,
36.5770891681321));
#152440=CARTESIAN_POINT('Ctrl Pts',(-3.33998448488285,-6.16734509958608,
36.5687267396685));
#152441=CARTESIAN_POINT('Ctrl Pts',(-3.50099140993622,-6.0773834396258,
36.5603643112048));
#152442=CARTESIAN_POINT('Ctrl Pts',(-3.65807295569729,-5.98131497359035,
36.5520018827411));
#152443=CARTESIAN_POINT('Ctrl Pts',(-3.81528882759326,-5.88516435592044,
36.5436323032611));
#152444=CARTESIAN_POINT('Ctrl Pts',(-3.96857235073418,-5.7828966940442,
36.5352627237811));
#152445=CARTESIAN_POINT('Ctrl Pts',(-4.1174530024884,-5.67487509420245,
36.5268931443012));
#152446=CARTESIAN_POINT('Ctrl Pts',(-4.26656328450854,-5.56668688420415,
36.5185106557646));
#152447=CARTESIAN_POINT('Ctrl Pts',(-4.4112568680101,-5.4527272041818,36.510128167228));
#152448=CARTESIAN_POINT('Ctrl Pts',(-4.5510970485728,-5.33339874910661,
36.5017456786914));
#152449=CARTESIAN_POINT('Ctrl Pts',(-4.59685504706801,-5.29435252329516,
36.4990027910871));
#152450=CARTESIAN_POINT('Ctrl Pts',(-4.6420936902436,-5.25473174628446,
36.4962599034829));
#152451=CARTESIAN_POINT('Ctrl Pts',(-4.68679857597309,-5.21455133935381,
36.4935170158786));
#152452=CARTESIAN_POINT('Ctrl Pts',(-4.82354042219979,-5.09164882129161,
36.4851271607458));
#152453=CARTESIAN_POINT('Ctrl Pts',(-4.9555616510863,-4.96325958095893,
36.476737305613));
#152454=CARTESIAN_POINT('Ctrl Pts',(-5.08241371095259,-4.82977198563464,
36.4683474504802));
#152455=CARTESIAN_POINT('Ctrl Pts',(-5.20914871351634,-4.69640757079198,
36.4599653373881));
#152456=CARTESIAN_POINT('Ctrl Pts',(-5.33072383076894,-4.55795441689385,
36.4515832242959));
#152457=CARTESIAN_POINT('Ctrl Pts',(-5.44672584142834,-4.41483908776037,
36.4432011112038));
#152458=CARTESIAN_POINT('Ctrl Pts',(-5.56263785911342,-4.27183478578982,
36.4348255008549));
#152459=CARTESIAN_POINT('Ctrl Pts',(-5.67298518379625,-4.12417577395732,
36.426449890506));
#152460=CARTESIAN_POINT('Ctrl Pts',(-5.77739322365365,-3.97232351423961,
36.4180742801572));
#152461=CARTESIAN_POINT('Ctrl Pts',(-5.88173558930339,-3.82056677184845,
36.4097039381916));
#152462=CARTESIAN_POINT('Ctrl Pts',(-5.98014593340909,-3.6646223109188,
36.401333596226));
#152463=CARTESIAN_POINT('Ctrl Pts',(-6.07229127951492,-3.50498290712338,
36.3929632542604));
#152464=CARTESIAN_POINT('Ctrl Pts',(-6.16439217230274,-3.34542051753957,
36.384596950366));
#152465=CARTESIAN_POINT('Ctrl Pts',(-6.25023393020387,-3.18216702394998,
36.3762306464717));
#152466=CARTESIAN_POINT('Ctrl Pts',(-6.32952784025315,-3.01574267502389,
36.3678643425773));
#152467=CARTESIAN_POINT('Ctrl Pts',(-6.40879957401827,-2.84936487032361,
36.3595003785037));
#152468=CARTESIAN_POINT('Ctrl Pts',(-6.48152696887386,-2.67981827436776,
36.35113641443));
#152469=CARTESIAN_POINT('Ctrl Pts',(-6.54746782428572,-2.50764663627937,
36.3427724503564));
#152470=CARTESIAN_POINT('Ctrl Pts',(-6.61339853249572,-2.33550149254498,
36.3344097733578));
#152471=CARTESIAN_POINT('Ctrl Pts',(-6.6725446659447,-2.16073241890292,
36.3260470963593));
#152472=CARTESIAN_POINT('Ctrl Pts',(-6.72471247732225,-1.98390238163234,
36.3176844193607));
#152473=CARTESIAN_POINT('Ctrl Pts',(-6.77687921465991,-1.80707598496905,
36.3093219145344));
#152474=CARTESIAN_POINT('Ctrl Pts',(-6.82206782379734,-1.62818902461673,
36.3009594097081));
#152475=CARTESIAN_POINT('Ctrl Pts',(-6.86013454488979,-1.44781925270725,
36.2925969048817));
#152476=CARTESIAN_POINT('Ctrl Pts',(-6.89820555628098,-1.26742915227499,
36.2842334575617));
#152477=CARTESIAN_POINT('Ctrl Pts',(-6.92915301199516,-1.0855562287602,
36.2758700102417));
#152478=CARTESIAN_POINT('Ctrl Pts',(-6.95288426097215,-0.902788466932194,
36.2675065629217));
#152479=CARTESIAN_POINT('Ctrl Pts',(-6.97662948357546,-0.719913086309687,
36.2591381909689));
#152480=CARTESIAN_POINT('Ctrl Pts',(-6.99314996540156,-0.536142140628691,
36.2507698190161));
#152481=CARTESIAN_POINT('Ctrl Pts',(-7.0024048299875,-0.352069821864623,
36.2424014470632));
#152482=CARTESIAN_POINT('Ctrl Pts',(-7.01166246757275,-0.167942350223029,
36.2340305677275));
#152483=CARTESIAN_POINT('Ctrl Pts',(-7.01365013587314,0.0164863459830646,
36.2256596883917));
#152484=CARTESIAN_POINT('Ctrl Pts',(-7.00837910332929,0.200621301255173,
36.2172888090559));
#152485=CARTESIAN_POINT('Ctrl Pts',(-7.00310360469657,0.384912272083683,
36.2089108371646));
#152486=CARTESIAN_POINT('Ctrl Pts',(-6.99055713077544,0.568908676038571,
36.2005328652733));
#152487=CARTESIAN_POINT('Ctrl Pts',(-6.97080299477737,0.752018730154316,
36.192154893382));
#152488=CARTESIAN_POINT('Ctrl Pts',(-6.95824908049263,0.868386660610357,
36.1868306240232));
#152489=CARTESIAN_POINT('Ctrl Pts',(-6.94278524829619,0.984396730679544,
36.1815063546644));
#152490=CARTESIAN_POINT('Ctrl Pts',(-6.92443852335612,1.09989894934115,
36.1761820853057));
#152491=CARTESIAN_POINT('Ctrl Pts',(-6.89734425156818,1.2704715455265,36.1683192541164));
#152492=CARTESIAN_POINT('Ctrl Pts',(-6.86390358510984,1.44029073648348,
36.1604564229272));
#152493=CARTESIAN_POINT('Ctrl Pts',(-6.82417039470933,1.6088272083952,36.152593591738));
#152494=CARTESIAN_POINT('Ctrl Pts',(-6.78446773402093,1.77723418227481,
36.1447368020967));
#152495=CARTESIAN_POINT('Ctrl Pts',(-6.73848225135412,1.94436002841757,
36.1368800124554));
#152496=CARTESIAN_POINT('Ctrl Pts',(-6.68631940867869,2.10968228120413,
36.129023222814));
#152497=CARTESIAN_POINT('Ctrl Pts',(-6.63418598337725,2.27491130006613,
36.1211708640301));
#152498=CARTESIAN_POINT('Ctrl Pts',(-6.57588224238862,2.4383383864304,36.1133185052463));
#152499=CARTESIAN_POINT('Ctrl Pts',(-6.51156428960506,2.59945322420701,
36.1054661464624));
#152500=CARTESIAN_POINT('Ctrl Pts',(-6.4472615230406,2.76053002089053,36.097615641712));
#152501=CARTESIAN_POINT('Ctrl Pts',(-6.37694750432004,2.91929529867078,
36.0897651369616));
#152502=CARTESIAN_POINT('Ctrl Pts',(-6.30082755025666,3.0752558827562,36.0819146322113));
#152503=CARTESIAN_POINT('Ctrl Pts',(-6.22471984149481,3.23119137769909,
36.0740653903597));
#152504=CARTESIAN_POINT('Ctrl Pts',(-6.14280822674209,3.38432273557631,
36.0662161485082));
#152505=CARTESIAN_POINT('Ctrl Pts',(-6.05534512568461,3.53417910855515,
36.0583669066566));
#152506=CARTESIAN_POINT('Ctrl Pts',(-5.9678525565964,3.6840859710793,36.0505150202418));
#152507=CARTESIAN_POINT('Ctrl Pts',(-5.87480495767119,3.8307153149177,36.042663133827));
#152508=CARTESIAN_POINT('Ctrl Pts',(-5.77649954847457,3.97362297267533,
36.0348112474122));
#152509=CARTESIAN_POINT('Ctrl Pts',(-5.70431511007936,4.07855828703809,
36.0290457049479));
#152510=CARTESIAN_POINT('Ctrl Pts',(-5.62929671775047,4.1814874955054,36.0232801624836));
#152511=CARTESIAN_POINT('Ctrl Pts',(-5.55157631074784,4.28224555910138,
36.0175146200193));
#152512=CARTESIAN_POINT('Ctrl Pts',(-5.42142130985316,4.4509807261346,36.0078593156592));
#152513=CARTESIAN_POINT('Ctrl Pts',(-5.28375446149784,4.61354048175918,
35.9982040112991));
#152514=CARTESIAN_POINT('Ctrl Pts',(-5.13914797926629,4.76935893068483,
35.9885487069391));
#152515=CARTESIAN_POINT('Ctrl Pts',(-4.99374040425093,4.92604058458647,
35.9788399140041));
#152516=CARTESIAN_POINT('Ctrl Pts',(-4.84131616604515,5.07590603639355,
35.9691311210692));
#152517=CARTESIAN_POINT('Ctrl Pts',(-4.68248723669843,5.21842311820882,
35.9594223281343));
#152518=CARTESIAN_POINT('Ctrl Pts',(-4.52289400905709,5.36162600432332,
35.9496668156634));
#152519=CARTESIAN_POINT('Ctrl Pts',(-4.35683435035826,5.49740961728959,
35.9399113031925));
#152520=CARTESIAN_POINT('Ctrl Pts',(-4.18495860069878,5.6252775996334,35.9301557907215));
#152521=CARTESIAN_POINT('Ctrl Pts',(-4.0129126676046,5.75327219095182,35.9203906187924));
#152522=CARTESIAN_POINT('Ctrl Pts',(-3.83503916201762,5.87333546055584,
35.9106254468633));
#152523=CARTESIAN_POINT('Ctrl Pts',(-3.6520191350744,5.98501318290532,35.9008602749341));
#152524=CARTESIAN_POINT('Ctrl Pts',(-3.46924865178581,6.09653863521397,
35.8911084175954));
#152525=CARTESIAN_POINT('Ctrl Pts',(-3.2813457043459,6.19970137200236,35.8813565602566));
#152526=CARTESIAN_POINT('Ctrl Pts',(-3.08901667879727,6.29409266857522,
35.8716047029179));
#152527=CARTESIAN_POINT('Ctrl Pts',(-3.00514729454962,6.33525411001299,
35.8673521868562));
#152528=CARTESIAN_POINT('Ctrl Pts',(-2.92043660936041,6.37474814422477,
35.8630996707945));
#152529=CARTESIAN_POINT('Ctrl Pts',(-2.83494485713112,6.41254350624819,
35.8588471547329));
#152530=CARTESIAN_POINT('Ctrl Pts',(-2.67345007756686,6.48393932513552,
35.8508141091341));
#152531=CARTESIAN_POINT('Ctrl Pts',(-2.50908783830989,6.5493050661394,35.8427810635354));
#152532=CARTESIAN_POINT('Ctrl Pts',(-2.34235612441827,6.60840331312339,
35.8347480179366));
#152533=CARTESIAN_POINT('Ctrl Pts',(-2.17573159209201,6.66746356947876,
35.8267201362889));
#152534=CARTESIAN_POINT('Ctrl Pts',(-2.00674096114295,6.72026422965502,
35.8186922546412));
#152535=CARTESIAN_POINT('Ctrl Pts',(-1.83590305423349,6.76661558963978,
35.8106643729934));
#152536=CARTESIAN_POINT('Ctrl Pts',(-1.6651422823232,6.81294602152856,35.8026401160134));
#152537=CARTESIAN_POINT('Ctrl Pts',(-1.4925362482132,6.85283285541069,35.7946158590334));
#152538=CARTESIAN_POINT('Ctrl Pts',(-1.31861978183444,6.88613595810124,
35.7865916020533));
#152539=CARTESIAN_POINT('Ctrl Pts',(-1.14472434372789,6.91943503410747,
35.7785683152877));
#152540=CARTESIAN_POINT('Ctrl Pts',(-0.9695191473153,6.94615188802487,35.7705450285221));
#152541=CARTESIAN_POINT('Ctrl Pts',(-0.793550262889007,6.96619727992029,
35.7625217417564));
#152542=CARTESIAN_POINT('Ctrl Pts',(-0.617595797543047,6.98624102927465,
35.7544991124276));
#152543=CARTESIAN_POINT('Ctrl Pts',(-0.440878133575294,6.99961436800925,
35.7464764830987));
#152544=CARTESIAN_POINT('Ctrl Pts',(-0.263949226028385,7.00627985228816,
35.7384538537699));
#152545=CARTESIAN_POINT('Ctrl Pts',(-0.0869538058082248,7.01294784231463,
35.7304282085035));
#152546=CARTESIAN_POINT('Ctrl Pts',(0.0902526499616381,7.01290292960881,
35.7224025632372));
#152547=CARTESIAN_POINT('Ctrl Pts',(0.267117028962989,7.00615979373423,
35.7143769179709));
#152548=CARTESIAN_POINT('Ctrl Pts',(0.371407044414812,7.00218362991579,
35.7096445084627));
#152549=CARTESIAN_POINT('Ctrl Pts',(0.475578136999383,6.99587948197923,
35.7049120989546));
#152550=CARTESIAN_POINT('Ctrl Pts',(0.579517602897687,6.98725882663808,
35.7001796894465));
#152551=CARTESIAN_POINT('Ctrl Pts',(0.771258535626464,6.97135598856248,
35.6914496406118));
#152552=CARTESIAN_POINT('Ctrl Pts',(0.962306806831938,6.94755946216054,
35.6827195917771));
#152553=CARTESIAN_POINT('Ctrl Pts',(1.15202145315725,6.91595786091598,35.6739895429424));
#152554=CARTESIAN_POINT('Ctrl Pts',(1.34179095570927,6.88434712202898,35.6652569698032));
#152555=CARTESIAN_POINT('Ctrl Pts',(1.53022579344518,6.84492684852203,35.656524396664));
#152556=CARTESIAN_POINT('Ctrl Pts',(1.71669433999845,6.79783694313988,35.6477918235248));
#152557=CARTESIAN_POINT('Ctrl Pts',(1.90581196991434,6.75007805048239,35.6389351902444));
#152558=CARTESIAN_POINT('Ctrl Pts',(2.092906733217,6.69443001733014,35.630078556964));
#152559=CARTESIAN_POINT('Ctrl Pts',(2.2773342966685,6.6310915439102,35.6212219236836));
#152560=CARTESIAN_POINT('Ctrl Pts',(2.45929423139178,6.56860053511913,35.6124837915768));
#152561=CARTESIAN_POINT('Ctrl Pts',(2.63865764175701,6.4986237153111,35.6037456594701));
#152562=CARTESIAN_POINT('Ctrl Pts',(2.81482368315884,6.42140126415007,35.5950075273633));
#152563=CARTESIAN_POINT('Ctrl Pts',(2.99457330782607,6.34260794790351,35.5860916434961));
#152564=CARTESIAN_POINT('Ctrl Pts',(3.17099381509528,6.25627117582011,35.5771757596289));
#152565=CARTESIAN_POINT('Ctrl Pts',(3.34347019431484,6.16269694388977,35.5682598757617));
#152566=CARTESIAN_POINT('Ctrl Pts',(3.51594657353441,6.06912271195942,35.5593439918945));
#152567=CARTESIAN_POINT('Ctrl Pts',(3.68447856179311,5.9683111697409,35.5504281080273));
#152568=CARTESIAN_POINT('Ctrl Pts',(3.84847863845386,5.86061760669167,35.54151222416));
#152569=CARTESIAN_POINT('Ctrl Pts',(4.0092560721689,5.75504024936822,35.5327715396637));
#152570=CARTESIAN_POINT('Ctrl Pts',(4.16569512362814,5.64283761417073,35.5240308551673));
#152571=CARTESIAN_POINT('Ctrl Pts',(4.31726831139562,5.524384209115,35.5152901706709));
#152572=CARTESIAN_POINT('Ctrl Pts',(4.46881422862865,5.40595211579462,35.5065510587689));
#152573=CARTESIAN_POINT('Ctrl Pts',(4.6154958148557,5.28127166709487,35.4978119468669));
#152574=CARTESIAN_POINT('Ctrl Pts',(4.756817478221,5.15075858892564,35.4890728349649));
#152575=CARTESIAN_POINT('Ctrl Pts',(4.89997016712896,5.01855452599095,35.4802204952906));
#152576=CARTESIAN_POINT('Ctrl Pts',(5.03762284930191,4.88036581662593,35.4713681556163));
#152577=CARTESIAN_POINT('Ctrl Pts',(5.16929682606843,4.73666516512397,35.4625158159421));
#152578=CARTESIAN_POINT('Ctrl Pts',(5.29921997169161,4.59487526001356,35.4537811832922));
#152579=CARTESIAN_POINT('Ctrl Pts',(5.4233222392301,4.44771930042879,35.4450465506423));
#152580=CARTESIAN_POINT('Ctrl Pts',(5.54118175105719,4.29568753103048,35.4363119179924));
#152581=CARTESIAN_POINT('Ctrl Pts',(5.66142365713964,4.14058261455706,35.4274007248059));
#152582=CARTESIAN_POINT('Ctrl Pts',(5.77516754427766,3.98040288732872,35.4184895316194));
#152583=CARTESIAN_POINT('Ctrl Pts',(5.88200887951529,3.81570414259324,35.409578338433));
#152584=CARTESIAN_POINT('Ctrl Pts',(5.98885021475291,3.6510053978578,35.4006671452465));
#152585=CARTESIAN_POINT('Ctrl Pts',(6.0887888218152,3.48178788258962,35.39175595206));
#152586=CARTESIAN_POINT('Ctrl Pts',(6.18146681589465,3.30863938296292,35.3828447588735));
#152587=CARTESIAN_POINT('Ctrl Pts',(6.26488919567311,3.1527829680998,35.3748235133809));
#152588=CARTESIAN_POINT('Ctrl Pts',(6.34246700775347,2.99366895795854,35.3668022678882));
#152589=CARTESIAN_POINT('Ctrl Pts',(6.41393984207482,2.83178428993898,35.3587810223955));
#152590=CARTESIAN_POINT('Ctrl Pts',(6.47013863698517,2.7044950430028,35.35247395014));
#152591=CARTESIAN_POINT('Ctrl Pts',(6.52256380139321,2.57549341148191,35.3461668778845));
#152592=CARTESIAN_POINT('Ctrl Pts',(6.57110895151813,2.44502632087638,35.339859805629));
#152593=CARTESIAN_POINT('Origin',(0.,0.,50.));
#152594=CARTESIAN_POINT('',(6.57110895151813,2.44502632087639,33.3398701610928));
#152595=CARTESIAN_POINT('',(6.57110895151815,2.44502632087634,33.8866662574739));
#152596=CARTESIAN_POINT('',(6.57110895151814,2.44502632087636,50.));
#152597=CARTESIAN_POINT('',(7.01124858877573,0.00444847055755681,35.7735343569399));
#152598=CARTESIAN_POINT('Ctrl Pts',(6.57110895151815,2.44502632087633,33.8866662574739));
#152599=CARTESIAN_POINT('Ctrl Pts',(6.50684008859926,2.61775153729806,33.8950354753427));
#152600=CARTESIAN_POINT('Ctrl Pts',(6.4358134696495,2.78778929210781,33.9034046932115));
#152601=CARTESIAN_POINT('Ctrl Pts',(6.35829518664791,2.95460807586219,33.9117739110803));
#152602=CARTESIAN_POINT('Ctrl Pts',(6.2806561267985,3.1216867705186,33.9201561685536));
#152603=CARTESIAN_POINT('Ctrl Pts',(6.1965053400371,3.28553618062757,33.9285384260269));
#152604=CARTESIAN_POINT('Ctrl Pts',(6.10615428911975,3.44565035370167,33.9369206835002));
#152605=CARTESIAN_POINT('Ctrl Pts',(6.07231393013319,3.50562000586014,33.9400601998549));
#152606=CARTESIAN_POINT('Ctrl Pts',(6.03760421129288,3.56506597215157,33.9431997162095));
#152607=CARTESIAN_POINT('Ctrl Pts',(6.00204300290678,3.62396279696105,33.9463392325642));
#152608=CARTESIAN_POINT('Ctrl Pts',(5.90701136331561,3.78135513772714,33.9547290876969));
#152609=CARTESIAN_POINT('Ctrl Pts',(5.80570400173894,3.93514141929994,33.9631189428297));
#152610=CARTESIAN_POINT('Ctrl Pts',(5.69841812432295,4.0848081280383,33.9715087979625));
#152611=CARTESIAN_POINT('Ctrl Pts',(5.59123124881029,4.23433672643643,33.9798909110546));
#152612=CARTESIAN_POINT('Ctrl Pts',(5.47807704596683,4.37975306437033,33.9882730241467));
#152613=CARTESIAN_POINT('Ctrl Pts',(5.35929687460675,4.52057115554333,33.9966551372388));
#152614=CARTESIAN_POINT('Ctrl Pts',(5.24060885148502,4.66128000172298,34.0050307475877));
#152615=CARTESIAN_POINT('Ctrl Pts',(5.11630377263722,4.797397462809,34.0134063579365));
#152616=CARTESIAN_POINT('Ctrl Pts',(4.98676452950965,4.92846893971387,34.0217819682854));
#152617=CARTESIAN_POINT('Ctrl Pts',(4.85730676849,5.05945797071302,34.030152310251));
#152618=CARTESIAN_POINT('Ctrl Pts',(4.72262163835405,5.18540711299538,34.0385226522165));
#152619=CARTESIAN_POINT('Ctrl Pts',(4.58313060334181,5.30589676070047,34.0468929941821));
#152620=CARTESIAN_POINT('Ctrl Pts',(4.44370686244198,5.42632828105784,34.0552592980765));
#152621=CARTESIAN_POINT('Ctrl Pts',(4.2994820884425,5.54130534456897,34.0636256019708));
#152622=CARTESIAN_POINT('Ctrl Pts',(4.15091304341598,5.65044666097284,34.0719919058652));
#152623=CARTESIAN_POINT('Ctrl Pts',(4.00238554898793,5.75955745360903,34.0803558699388));
#152624=CARTESIAN_POINT('Ctrl Pts',(3.84951646994518,5.86283555794422,34.0887198340124));
#152625=CARTESIAN_POINT('Ctrl Pts',(3.69279438675831,5.95994095437416,34.097083798086));
#152626=CARTESIAN_POINT('Ctrl Pts',(3.5360964204957,6.05703140789724,34.1054464750845));
#152627=CARTESIAN_POINT('Ctrl Pts',(3.37554691153541,6.14795087432785,34.1138091520831));
#152628=CARTESIAN_POINT('Ctrl Pts',(3.21166241620954,6.23240331548008,34.1221718290816));
#152629=CARTESIAN_POINT('Ctrl Pts',(3.0477812949664,6.31685401791064,34.1305343339079));
#152630=CARTESIAN_POINT('Ctrl Pts',(2.88056561659312,6.39483781036505,34.1388968387341));
#152631=CARTESIAN_POINT('Ctrl Pts',(2.71055584901467,6.46610497532111,34.1472593435604));
#152632=CARTESIAN_POINT('Ctrl Pts',(2.54052692053521,6.5373801724221,34.1556227908803));
#152633=CARTESIAN_POINT('Ctrl Pts',(2.36770357830753,6.60193710623713,34.1639862382003));
#152634=CARTESIAN_POINT('Ctrl Pts',(2.19264594028158,6.65957433647727,34.1723496855202));
#152635=CARTESIAN_POINT('Ctrl Pts',(2.01748522339739,6.7172455051388,34.180718057473));
#152636=CARTESIAN_POINT('Ctrl Pts',(1.84008789399861,6.76798872457049,34.1890864294258));
#152637=CARTESIAN_POINT('Ctrl Pts',(1.66102989132753,6.81165224175578,34.1974548013786));
#152638=CARTESIAN_POINT('Ctrl Pts',(1.48191823819943,6.85532884167189,34.2058256807143));
#152639=CARTESIAN_POINT('Ctrl Pts',(1.30114524025199,6.89192143685681,34.2141965600501));
#152640=CARTESIAN_POINT('Ctrl Pts',(1.11929739059536,6.92132934586315,34.2225674393858));
#152641=CARTESIAN_POINT('Ctrl Pts',(0.937295463222451,6.95076217187274,
34.2309454112771));
#152642=CARTESIAN_POINT('Ctrl Pts',(0.754217189934041,6.97299810058162,
34.2393233831684));
#152643=CARTESIAN_POINT('Ctrl Pts',(0.570655713252553,6.98798816680683,
34.2477013550596));
#152644=CARTESIAN_POINT('Ctrl Pts',(0.454000900070819,6.99751447595783,
34.2530256244188));
#152645=CARTESIAN_POINT('Ctrl Pts',(0.337151023210004,7.00411544128752,
34.258349893778));
#152646=CARTESIAN_POINT('Ctrl Pts',(0.220258480229419,7.00778943493503,
34.2636741631371));
#152647=CARTESIAN_POINT('Ctrl Pts',(0.0476326661061512,7.0132151543891,
34.2715369943264));
#152648=CARTESIAN_POINT('Ctrl Pts',(-0.125445162474049,7.01226592069182,
34.2793998255156));
#152649=CARTESIAN_POINT('Ctrl Pts',(-0.298444993877957,7.00489522749122,
34.2872626567048));
#152650=CARTESIAN_POINT('Ctrl Pts',(-0.471311897746947,6.99753019769542,
34.2951194463462));
#152651=CARTESIAN_POINT('Ctrl Pts',(-0.644100545156358,6.983753536577,34.3029762359875));
#152652=CARTESIAN_POINT('Ctrl Pts',(-0.816277960669884,6.96357069709389,
34.3108330256288));
#152653=CARTESIAN_POINT('Ctrl Pts',(-0.988358276271211,6.94339923977687,
34.3186853844127));
#152654=CARTESIAN_POINT('Ctrl Pts',(-1.15982766817703,6.91682883499607,
34.3265377431966));
#152655=CARTESIAN_POINT('Ctrl Pts',(-1.33015558243525,6.88391695831787,
34.3343901019805));
#152656=CARTESIAN_POINT('Ctrl Pts',(-1.50044328028575,6.85101285251773,
34.3422406067309));
#152657=CARTESIAN_POINT('Ctrl Pts',(-1.66958966129264,6.81177031883781,
34.3500911114812));
#152658=CARTESIAN_POINT('Ctrl Pts',(-1.83707176431813,6.76629838946267,
34.3579416162316));
#152659=CARTESIAN_POINT('Ctrl Pts',(-2.00452692475201,6.72083377508777,
34.3657908580832));
#152660=CARTESIAN_POINT('Ctrl Pts',(-2.17031797276425,6.66914186280106,
34.3736400999347));
#152661=CARTESIAN_POINT('Ctrl Pts',(-2.3339350297199,6.61138214290676,34.3814893417863));
#152662=CARTESIAN_POINT('Ctrl Pts',(-2.49760721246457,6.55360296263228,
34.3893412282011));
#152663=CARTESIAN_POINT('Ctrl Pts',(-2.65910358102391,6.48975201837551,
34.3971931146159));
#152664=CARTESIAN_POINT('Ctrl Pts',(-2.81793204782319,6.42003781424619,
34.4050450010307));
#152665=CARTESIAN_POINT('Ctrl Pts',(-2.93455781410189,6.36884754186658,
34.410810543495));
#152666=CARTESIAN_POINT('Ctrl Pts',(-3.0497454652282,6.3144969561212,34.4165760859592));
#152667=CARTESIAN_POINT('Ctrl Pts',(-3.16330811802394,6.25708464965465,
34.4223416284234));
#152668=CARTESIAN_POINT('Ctrl Pts',(-3.35348657625233,6.16093874553613,
34.4319969327836));
#152669=CARTESIAN_POINT('Ctrl Pts',(-3.53901044182278,6.05625478979374,
34.4416522371438));
#152670=CARTESIAN_POINT('Ctrl Pts',(-3.71921641498869,5.9434885228272,34.4513075415041));
#152671=CARTESIAN_POINT('Ctrl Pts',(-3.90042069543694,5.8300975518981,34.461016334439));
#152672=CARTESIAN_POINT('Ctrl Pts',(-4.07624798905754,5.70853454413747,
34.4707251273739));
#152673=CARTESIAN_POINT('Ctrl Pts',(-4.24606065560468,5.57930062565426,
34.4804339203088));
#152674=CARTESIAN_POINT('Ctrl Pts',(-4.41669047512317,5.44944482258119,
34.4901894327797));
#152675=CARTESIAN_POINT('Ctrl Pts',(-4.58124762260269,5.31184415030478,
34.4999449452507));
#152676=CARTESIAN_POINT('Ctrl Pts',(-4.73912242441051,5.16704414621643,
34.5097004577216));
#152677=CARTESIAN_POINT('Ctrl Pts',(-4.8971535465599,5.02210076784771,34.5194656296508));
#152678=CARTESIAN_POINT('Ctrl Pts',(-5.04848906772519,4.86994383329936,
34.5292308015798));
#152679=CARTESIAN_POINT('Ctrl Pts',(-5.19255492806774,4.71115695785011,
34.538995973509));
#152680=CARTESIAN_POINT('Ctrl Pts',(-5.33642435787886,4.55258658470232,
34.5487478308477));
#152681=CARTESIAN_POINT('Ctrl Pts',(-5.47304391196111,4.38740436604411,
34.5584996881865));
#152682=CARTESIAN_POINT('Ctrl Pts',(-5.60187946299434,4.21622734735478,
34.5682515455253));
#152683=CARTESIAN_POINT('Ctrl Pts',(-5.65806109394264,4.14158176999892,
34.5725040615868));
#152684=CARTESIAN_POINT('Ctrl Pts',(-5.71276301056878,4.06579668412801,
34.5767565776484));
#152685=CARTESIAN_POINT('Ctrl Pts',(-5.76594319092083,3.98892537929374,
34.58100909371));
#152686=CARTESIAN_POINT('Ctrl Pts',(-5.86640108632521,3.84371471153147,
34.5890421393087));
#152687=CARTESIAN_POINT('Ctrl Pts',(-5.96147480433599,3.6945550188055,34.5970751849074));
#152688=CARTESIAN_POINT('Ctrl Pts',(-6.05083762022762,3.54189083063527,
34.6051082305062));
#152689=CARTESIAN_POINT('Ctrl Pts',(-6.14014299026016,3.38932478088372,
34.6131361121539));
#152690=CARTESIAN_POINT('Ctrl Pts',(-6.22374458135365,3.23325903502649,
34.6211639938016));
#152691=CARTESIAN_POINT('Ctrl Pts',(-6.30135861793038,3.07416755085577,
34.6291918754493));
#152692=CARTESIAN_POINT('Ctrl Pts',(-6.37893761100423,2.91514789805898,
34.6372161324292));
#152693=CARTESIAN_POINT('Ctrl Pts',(-6.45053427202727,2.75310555588188,
34.6452403894092));
#152694=CARTESIAN_POINT('Ctrl Pts',(-6.51591050745011,2.58853951513228,
34.6532646463892));
#152695=CARTESIAN_POINT('Ctrl Pts',(-6.58127883822066,2.42399337209203,
34.6612879331548));
#152696=CARTESIAN_POINT('Ctrl Pts',(-6.64042809904845,2.25692447589421,
34.6693112199205));
#152697=CARTESIAN_POINT('Ctrl Pts',(-6.69316807264476,2.08785241667817,
34.6773345066861));
#152698=CARTESIAN_POINT('Ctrl Pts',(-6.74590372467046,1.91879421140996,
34.6853571360149));
#152699=CARTESIAN_POINT('Ctrl Pts',(-6.79223103023467,1.74773352128503,
34.6933797653437));
#152700=CARTESIAN_POINT('Ctrl Pts',(-6.83200954100363,1.57520544505643,
34.7014023946725));
#152701=CARTESIAN_POINT('Ctrl Pts',(-6.87180300566088,1.40261251055307,
34.7094280399389));
#152702=CARTESIAN_POINT('Ctrl Pts',(-6.90504267801968,1.22855144608101,
34.7174536852052));
#152703=CARTESIAN_POINT('Ctrl Pts',(-6.93163908811575,1.05356827714478,
34.7254793304715));
#152704=CARTESIAN_POINT('Ctrl Pts',(-6.94732195221547,0.950387537779847,
34.7302117399798));
#152705=CARTESIAN_POINT('Ctrl Pts',(-6.96069592775399,0.846886351359701,
34.7349441494881));
#152706=CARTESIAN_POINT('Ctrl Pts',(-6.97175111860425,0.743177571472889,
34.7396765589963));
#152707=CARTESIAN_POINT('Ctrl Pts',(-6.99214503333859,0.551862193668865,
34.748406607831));
#152708=CARTESIAN_POINT('Ctrl Pts',(-7.00465564836262,0.359744518503252,
34.7571366566657));
#152709=CARTESIAN_POINT('Ctrl Pts',(-7.00924961118236,0.167470745624329,
34.7658667055004));
#152710=CARTESIAN_POINT('Ctrl Pts',(-7.01384490235216,-0.02485862345532,
34.7745992786395));
#152711=CARTESIAN_POINT('Ctrl Pts',(-7.0105189655873,-0.217343906477795,
34.7833318517787));
#152712=CARTESIAN_POINT('Ctrl Pts',(-6.99929057855495,-0.40933844120971,
34.7920644249178));
#152713=CARTESIAN_POINT('Ctrl Pts',(-6.98790267436091,-0.604060564788502,
34.8009210581982));
#152714=CARTESIAN_POINT('Ctrl Pts',(-6.96838609170347,-0.798277600731434,
34.8097776914787));
#152715=CARTESIAN_POINT('Ctrl Pts',(-6.94081497261864,-0.991319362452381,
34.8186343247591));
#152716=CARTESIAN_POINT('Ctrl Pts',(-6.91361275330271,-1.1817782380355,
34.8273724568658));
#152717=CARTESIAN_POINT('Ctrl Pts',(-6.87857025954447,-1.37109282257502,
34.8361105889726));
#152718=CARTESIAN_POINT('Ctrl Pts',(-6.83581054283597,-1.55862785325833,
34.8448487210794));
#152719=CARTESIAN_POINT('Ctrl Pts',(-6.7921810046565,-1.74997773606888,
34.8537646049466));
#152720=CARTESIAN_POINT('Ctrl Pts',(-6.74051697392869,-1.93947460023313,
34.8626804888138));
#152721=CARTESIAN_POINT('Ctrl Pts',(-6.68100348636997,-2.12645690706686,
34.8715963726811));
#152722=CARTESIAN_POINT('Ctrl Pts',(-6.62148999881125,-2.31343921390056,
34.8805122565483));
#152723=CARTESIAN_POINT('Ctrl Pts',(-6.55412715193734,-2.49790667708081,
34.8894281404155));
#152724=CARTESIAN_POINT('Ctrl Pts',(-6.47915356094348,-2.67921550014429,
34.8983440242828));
#152725=CARTESIAN_POINT('Ctrl Pts',(-6.40565321995713,-2.85696155902109,
34.9070847087791));
#152726=CARTESIAN_POINT('Ctrl Pts',(-6.32483065806215,-3.03169084006869,
34.9158253932755));
#152727=CARTESIAN_POINT('Ctrl Pts',(-6.23695464382761,-3.20281490775494,
34.9245660777718));
#152728=CARTESIAN_POINT('Ctrl Pts',(-6.14909443994743,-3.37390818737946,
34.9333051896739));
#152729=CARTESIAN_POINT('Ctrl Pts',(-6.05418344311144,-3.54139730555117,
34.942044301576));
#152730=CARTESIAN_POINT('Ctrl Pts',(-5.9525368958658,-3.70471740701721,
34.950783413478));
#152731=CARTESIAN_POINT('Ctrl Pts',(-5.84957337130876,-3.87015355545144,
34.9596357531523));
#152732=CARTESIAN_POINT('Ctrl Pts',(-5.73969867365878,-4.03131164901688,
34.9684880928265));
#152733=CARTESIAN_POINT('Ctrl Pts',(-5.62328718273507,-4.1876327230295,
34.9773404325008));
#152734=CARTESIAN_POINT('Ctrl Pts',(-5.50842358205335,-4.34187524050822,
34.9860750651507));
#152735=CARTESIAN_POINT('Ctrl Pts',(-5.38719612323055,-4.49140835549209,
34.9948096978006));
#152736=CARTESIAN_POINT('Ctrl Pts',(-5.26000708668644,-4.63572561855299,
35.0035443304505));
#152737=CARTESIAN_POINT('Ctrl Pts',(-5.13024707029253,-4.7829600888307,
35.0124555236369));
#152738=CARTESIAN_POINT('Ctrl Pts',(-4.9942820721572,-4.92476536432569,
35.0213667168234));
#152739=CARTESIAN_POINT('Ctrl Pts',(-4.85258201244914,-5.06063971993216,
35.0302779100099));
#152740=CARTESIAN_POINT('Ctrl Pts',(-4.71088195274109,-5.19651407553862,
35.0391891031963));
#152741=CARTESIAN_POINT('Ctrl Pts',(-4.56344704093036,-5.32645729173091,
35.0481002963828));
#152742=CARTESIAN_POINT('Ctrl Pts',(-4.41078738240292,-5.45000745226419,
35.0570114895692));
#152743=CARTESIAN_POINT('Ctrl Pts',(-4.27329790931377,-5.56128011352687,
35.0650371544215));
#152744=CARTESIAN_POINT('Ctrl Pts',(-4.13150697620872,-5.66741791019989,
35.0730628192738));
#152745=CARTESIAN_POINT('Ctrl Pts',(-3.98584443948815,-5.76807339297113,
35.0810884841261));
#152746=CARTESIAN_POINT('Ctrl Pts',(-3.8402281324836,-5.86869693016123,
35.0891116018292));
#152747=CARTESIAN_POINT('Ctrl Pts',(-3.69074296940803,-5.96384140938561,
35.0971347195323));
#152748=CARTESIAN_POINT('Ctrl Pts',(-3.53784990253808,-6.05320118859528,
35.1051578372354));
#152749=CARTESIAN_POINT('Ctrl Pts',(-3.38497611682184,-6.1425496987548,
35.1131799431532));
#152750=CARTESIAN_POINT('Ctrl Pts',(-3.22869560004598,-6.22611477757557,
35.1212020490709));
#152751=CARTESIAN_POINT('Ctrl Pts',(-3.0694961030301,-6.30363547772101,
35.1292241549887));
#152752=CARTESIAN_POINT('Ctrl Pts',(-2.91023744694386,-6.38118498482025,
35.1372492419481));
#152753=CARTESIAN_POINT('Ctrl Pts',(-2.74805797229307,-6.4526854628926,
35.1452743289075));
#152754=CARTESIAN_POINT('Ctrl Pts',(-2.58346813081979,-6.51792290377376,
35.1532994158669));
#152755=CARTESIAN_POINT('Ctrl Pts',(-2.41884587420058,-6.58317319284255,
35.161326083327));
#152756=CARTESIAN_POINT('Ctrl Pts',(-2.25181264907545,-6.6421578605573,
35.1693527507871));
#152757=CARTESIAN_POINT('Ctrl Pts',(-2.08289626832121,-6.69471206982896,
35.1773794182473));
#152758=CARTESIAN_POINT('Ctrl Pts',(-1.91384428209153,-6.7473084694347,
35.1854125294878));
#152759=CARTESIAN_POINT('Ctrl Pts',(-1.74290647352157,-6.79346400008821,
35.1934456407282));
#152760=CARTESIAN_POINT('Ctrl Pts',(-1.57062371247984,-6.83306429914837,
35.2014787519687));
#152761=CARTESIAN_POINT('Ctrl Pts',(-1.469108451146,-6.85639823391749,35.206212152931));
#152762=CARTESIAN_POINT('Ctrl Pts',(-1.36712641924262,-6.87745716469574,
35.2109455538933));
#152763=CARTESIAN_POINT('Ctrl Pts',(-1.26478941082167,-6.89622609176739,
35.2156789548556));
#152764=CARTESIAN_POINT('Ctrl Pts',(-1.05397198855979,-6.9348906656583,
35.22542990815));
#152765=CARTESIAN_POINT('Ctrl Pts',(-0.8415236726413,-6.96385777599858,
35.2351808614444));
#152766=CARTESIAN_POINT('Ctrl Pts',(-0.62825740909946,-6.98304512303992,
35.2449318147389));
#152767=CARTESIAN_POINT('Ctrl Pts',(-0.414683895494878,-7.00226011305435,
35.2546968161108));
#152768=CARTESIAN_POINT('Ctrl Pts',(-0.200290115584286,-7.01166715299412,
35.2644618174828));
#152769=CARTESIAN_POINT('Ctrl Pts',(0.0141058876919451,-7.01123581021438,
35.2742268188548));
#152770=CARTESIAN_POINT('Ctrl Pts',(0.22814453724969,-7.01080518639368,
35.2839755439926));
#152771=CARTESIAN_POINT('Ctrl Pts',(0.442185364857365,-7.00056895396267,
35.2937242691304));
#152772=CARTESIAN_POINT('Ctrl Pts',(0.655413416586412,-6.98054867584623,
35.3034729942682));
#152773=CARTESIAN_POINT('Ctrl Pts',(0.868056239992785,-6.96058334563034,
35.3131949629356));
#152774=CARTESIAN_POINT('Ctrl Pts',(1.07989070109874,-6.93088758190894,
35.322916931603));
#152775=CARTESIAN_POINT('Ctrl Pts',(1.29010813764909,-6.89153448483512,
35.3326389002704));
#152776=CARTESIAN_POINT('Ctrl Pts',(1.49893462032694,-6.85244177692628,
35.3422965412103));
#152777=CARTESIAN_POINT('Ctrl Pts',(1.70616535539039,-6.80381909355923,
35.3519541821502));
#152778=CARTESIAN_POINT('Ctrl Pts',(1.91100791866417,-6.74578944952352,
35.3616118230901));
#152779=CARTESIAN_POINT('Ctrl Pts',(2.00104327749264,-6.72028342313944,
35.3658566887741));
#152780=CARTESIAN_POINT('Ctrl Pts',(2.09061727257798,-6.69296073299207,
35.3701015544581));
#152781=CARTESIAN_POINT('Ctrl Pts',(2.17966267742205,-6.66383502010317,
35.3743464201421));
#152782=CARTESIAN_POINT('Ctrl Pts',(2.34437245817147,-6.60996037275328,
35.382198267156));
#152783=CARTESIAN_POINT('Ctrl Pts',(2.50720483799878,-6.54993521035217,
35.3900501141698));
#152784=CARTESIAN_POINT('Ctrl Pts',(2.66765176712923,-6.48392324228413,
35.3979019611837));
#152785=CARTESIAN_POINT('Ctrl Pts',(2.82805319480719,-6.41792999467677,
35.4057515814772));
#152786=CARTESIAN_POINT('Ctrl Pts',(2.98607016502616,-6.34595346363315,
35.4136012017706));
#152787=CARTESIAN_POINT('Ctrl Pts',(3.1412126793601,-6.26820623986858,35.4214508220641));
#152788=CARTESIAN_POINT('Ctrl Pts',(3.29634280755006,-6.19046522322467,
35.4292998156659));
#152789=CARTESIAN_POINT('Ctrl Pts',(3.44859859600243,-6.10695460259406,
35.4371488092677));
#152790=CARTESIAN_POINT('Ctrl Pts',(3.59751305545061,-6.0179337299743,35.4449978028695));
#152791=CARTESIAN_POINT('Ctrl Pts',(3.74650290592818,-5.92886778869399,
35.4528507701869));
#152792=CARTESIAN_POINT('Ctrl Pts',(3.89214771961881,-5.83428621749232,
35.4607037375042));
#152793=CARTESIAN_POINT('Ctrl Pts',(4.03400772256224,-5.73449285088125,
35.4685567048216));
#152794=CARTESIAN_POINT('Ctrl Pts',(4.17590375317967,-5.63467414010831,
35.4764116665288));
#152795=CARTESIAN_POINT('Ctrl Pts',(4.3140127544162,-5.5296412279062,35.484266628236));
#152796=CARTESIAN_POINT('Ctrl Pts',(4.4479272014945,-5.41973893953439,35.4921215899432));
#152797=CARTESIAN_POINT('Ctrl Pts',(4.58197456985542,-5.30972756395464,
35.4999843483565));
#152798=CARTESIAN_POINT('Ctrl Pts',(4.71181878303615,-5.194837411621,35.5078471067697));
#152799=CARTESIAN_POINT('Ctrl Pts',(4.8370880053887,-5.0754513287613,35.515709865183));
#152800=CARTESIAN_POINT('Ctrl Pts',(4.92898370940593,-4.98787141145826,
35.5214778719315));
#152801=CARTESIAN_POINT('Ctrl Pts',(5.01841814621858,-4.89787280850003,
35.52724587868));
#152802=CARTESIAN_POINT('Ctrl Pts',(5.10525833230909,-4.80561795432061,
35.5330138854284));
#152803=CARTESIAN_POINT('Ctrl Pts',(5.23025566707761,-4.67282677305959,
35.5413163258416));
#152804=CARTESIAN_POINT('Ctrl Pts',(5.3501682762267,-4.53505011661643,35.5496187662548));
#152805=CARTESIAN_POINT('Ctrl Pts',(5.46458990420554,-4.39270801913295,
35.557921206668));
#152806=CARTESIAN_POINT('Ctrl Pts',(5.57892382502303,-4.25047503057869,
35.5662172830441));
#152807=CARTESIAN_POINT('Ctrl Pts',(5.68777494342812,-4.10368383910192,
35.5745133594202));
#152808=CARTESIAN_POINT('Ctrl Pts',(5.79077567238571,-3.95278935368505,
35.5828094357964));
#152809=CARTESIAN_POINT('Ctrl Pts',(5.89370860513702,-3.80199418866874,
35.5911000516043));
#152810=CARTESIAN_POINT('Ctrl Pts',(5.99079863748047,-3.64710139406454,
35.5993906674122));
#152811=CARTESIAN_POINT('Ctrl Pts',(6.08171995297363,-3.48859699250321,
35.6076812832201));
#152812=CARTESIAN_POINT('Ctrl Pts',(6.1726072499452,-3.33015189590659,35.6159687970657));
#152813=CARTESIAN_POINT('Ctrl Pts',(6.25733026206948,-3.16809817812648,
35.6242563109114));
#152814=CARTESIAN_POINT('Ctrl Pts',(6.33560751908777,-3.00294920479493,
35.632543824757));
#152815=CARTESIAN_POINT('Ctrl Pts',(6.4138673460344,-2.83783700534318,35.640829493214));
#152816=CARTESIAN_POINT('Ctrl Pts',(6.48568413442165,-2.66963122940047,
35.649115161671));
#152817=CARTESIAN_POINT('Ctrl Pts',(6.55082310083938,-2.49886839669661,
35.6574008301279));
#152818=CARTESIAN_POINT('Ctrl Pts',(6.61595742777563,-2.32811772646699,
35.6656859084435));
#152819=CARTESIAN_POINT('Ctrl Pts',(6.67441476136455,-2.1548106784762,35.673970986759));
#152820=CARTESIAN_POINT('Ctrl Pts',(6.72600894094853,-1.97950253568426,
35.6822560650745));
#152821=CARTESIAN_POINT('Ctrl Pts',(6.77762160673699,-1.804131579951,35.6905441119352));
#152822=CARTESIAN_POINT('Ctrl Pts',(6.82236610686468,-1.62675842037421,
35.6988321587958));
#152823=CARTESIAN_POINT('Ctrl Pts',(6.8601063107952,-1.44795302654742,35.7071202056565));
#152824=CARTESIAN_POINT('Ctrl Pts',(6.8978531132488,-1.26911637026325,35.715409701605));
#152825=CARTESIAN_POINT('Ctrl Pts',(6.92859311351629,-1.08884731231442,
35.7236991975534));
#152826=CARTESIAN_POINT('Ctrl Pts',(6.95224146597921,-0.907725267478727,
35.7319886935019));
#152827=CARTESIAN_POINT('Ctrl Pts',(6.97590646120624,-0.726475756195862,
35.7402840232659));
#152828=CARTESIAN_POINT('Ctrl Pts',(6.9924697976193,-0.544372394531557,
35.7485793530299));
#152829=CARTESIAN_POINT('Ctrl Pts',(7.00189850003828,-0.36199994152164,
35.7568746827938));
#152830=CARTESIAN_POINT('Ctrl Pts',(7.00821044961767,-0.239912545301506,
35.7624279074994));
#152831=CARTESIAN_POINT('Ctrl Pts',(7.01132609200597,-0.117704634689895,
35.767981132205));
#152832=CARTESIAN_POINT('Ctrl Pts',(7.01124858877614,0.00444846991387958,
35.7735343569106));
#152833=CARTESIAN_POINT('Ctrl Pts',(7.01124858877573,0.00444847055756476,
35.7735343569399));
#152834=CARTESIAN_POINT('Ctrl Pts',(7.01109817222245,0.241520478409522,
35.7843119309956));
#152835=CARTESIAN_POINT('Ctrl Pts',(6.99891979680166,0.478179014117121,
35.7950895050514));
#152836=CARTESIAN_POINT('Ctrl Pts',(6.97486124732339,0.713398306058046,
35.8058670791071));
#152837=CARTESIAN_POINT('Ctrl Pts',(6.9503880517275,0.95267157333437,35.8168304033156));
#152838=CARTESIAN_POINT('Ctrl Pts',(6.91362159642911,1.19045596317276,35.827793727524));
#152839=CARTESIAN_POINT('Ctrl Pts',(6.86476735121365,1.4256913327264,35.8387570517325));
#152840=CARTESIAN_POINT('Ctrl Pts',(6.84754912788099,1.50859784598541,35.8426209731554));
#152841=CARTESIAN_POINT('Ctrl Pts',(6.82882987788821,1.59118788002895,35.8464848945784));
#152842=CARTESIAN_POINT('Ctrl Pts',(6.80862007451949,1.67341544254565,35.8503488160013));
#152843=CARTESIAN_POINT('Ctrl Pts',(6.76477985634542,1.85178799842287,35.8587306470908));
#152844=CARTESIAN_POINT('Ctrl Pts',(6.71387483226996,2.02864465740253,35.8671124781804));
#152845=CARTESIAN_POINT('Ctrl Pts',(6.65602251740218,2.2034043683208,35.8754943092699));
#152846=CARTESIAN_POINT('Ctrl Pts',(6.62920495534626,2.28441459933983,35.8793797246746));
#152847=CARTESIAN_POINT('Ctrl Pts',(6.60089528170328,2.36497433156186,35.8832651400793));
#152848=CARTESIAN_POINT('Ctrl Pts',(6.57110895151814,2.44502632087637,35.887150555484));
#152849=CARTESIAN_POINT('',(7.01124948002267,-0.00270025589932498,35.2264656431181));
#152850=CARTESIAN_POINT('Ctrl Pts',(6.57110895151813,2.44502632087638,35.339859805629));
#152851=CARTESIAN_POINT('Ctrl Pts',(6.63282047719562,2.27917405363134,35.3318421344416));
#152852=CARTESIAN_POINT('Ctrl Pts',(6.68826026819073,2.11095325019693,35.3238244632542));
#152853=CARTESIAN_POINT('Ctrl Pts',(6.73725316088305,1.94088804640335,35.3158067920668));
#152854=CARTESIAN_POINT('Ctrl Pts',(6.78626203881579,1.77076735429258,35.3077865049));
#152855=CARTESIAN_POINT('Ctrl Pts',(6.82881971018949,1.59880141134544,35.2997662177331));
#152856=CARTESIAN_POINT('Ctrl Pts',(6.86480108493105,1.42552889371963,35.2917459305662));
#152857=CARTESIAN_POINT('Ctrl Pts',(6.90078822874227,1.25222859446423,35.2837243574675));
#152858=CARTESIAN_POINT('Ctrl Pts',(6.93019690879352,1.07762166429827,35.2757027843688));
#152859=CARTESIAN_POINT('Ctrl Pts',(6.95295341791382,0.902255690378585,
35.2676812112701));
#152860=CARTESIAN_POINT('Ctrl Pts',(6.9757280400242,0.726750134323181,35.2596532534191));
#152861=CARTESIAN_POINT('Ctrl Pts',(6.99183987564174,0.550484692843579,
35.2516252955681));
#152862=CARTESIAN_POINT('Ctrl Pts',(7.0012671711373,0.374011444818397,35.2435973377171));
#152863=CARTESIAN_POINT('Ctrl Pts',(7.00797313340574,0.248479902585227,
35.2378867728508));
#152864=CARTESIAN_POINT('Ctrl Pts',(7.01129783084764,0.122843288533582,
35.2321762079845));
#152865=CARTESIAN_POINT('Ctrl Pts',(7.01124948002267,-0.00270025589932412,
35.2264656431181));
#152866=CARTESIAN_POINT('Ctrl Pts',(7.01124948002242,-0.00270025652633111,
35.2264656430896));
#152867=CARTESIAN_POINT('Ctrl Pts',(7.01124302160634,-0.0194696138004879,
35.2257028599221));
#152868=CARTESIAN_POINT('Ctrl Pts',(7.01117640060358,-0.0362375540527687,
35.2249400767546));
#152869=CARTESIAN_POINT('Ctrl Pts',(7.01104964859509,-0.0530036549186942,
35.2241772935871));
#152870=CARTESIAN_POINT('Ctrl Pts',(7.00942932847339,-0.267331229823478,
35.2144263402928));
#152871=CARTESIAN_POINT('Ctrl Pts',(6.99797781269597,-0.481439247429157,
35.2046753869986));
#152872=CARTESIAN_POINT('Ctrl Pts',(6.97676695775352,-0.694513772144772,
35.1949244337043));
#152873=CARTESIAN_POINT('Ctrl Pts',(6.95552554459554,-0.907895270684285,
35.1851594323327));
#152874=CARTESIAN_POINT('Ctrl Pts',(6.92449667164411,-1.12024025957128,
35.175394430961));
#152875=CARTESIAN_POINT('Ctrl Pts',(6.88380409671614,-1.33073953895348,
35.1656294295893));
#152876=CARTESIAN_POINT('Ctrl Pts',(6.84317934787919,-1.54088795965175,
35.1558807044516));
#152877=CARTESIAN_POINT('Ctrl Pts',(6.79292309638973,-1.74919678212994,
35.146131979314));
#152878=CARTESIAN_POINT('Ctrl Pts',(6.73320959005129,-1.95486960663398,
35.1363832541763));
#152879=CARTESIAN_POINT('Ctrl Pts',(6.67365997413402,-2.1599779389838,35.1266612855091));
#152880=CARTESIAN_POINT('Ctrl Pts',(6.60470493240658,-2.36246467808975,
35.1169393168419));
#152881=CARTESIAN_POINT('Ctrl Pts',(6.52656815093536,-2.56154928387025,
35.1072173481747));
#152882=CARTESIAN_POINT('Ctrl Pts',(6.44894838013919,-2.7593165988117,35.0975597072349));
#152883=CARTESIAN_POINT('Ctrl Pts',(6.36226796450537,-2.95372659967752,
35.0879020662952));
#152884=CARTESIAN_POINT('Ctrl Pts',(6.26679656646663,-3.14402407068108,
35.0782444253554));
#152885=CARTESIAN_POINT('Ctrl Pts',(6.22483360015293,-3.22766636072133,
35.0739995596705));
#152886=CARTESIAN_POINT('Ctrl Pts',(6.18117295769982,-3.31051428342778,
35.0697546939856));
#152887=CARTESIAN_POINT('Ctrl Pts',(6.13584066416399,-3.39250437088761,
35.0655098283007));
#152888=CARTESIAN_POINT('Ctrl Pts',(6.05198825043613,-3.54416373332055,
35.0576579812868));
#152889=CARTESIAN_POINT('Ctrl Pts',(5.96244740792944,-3.69282388791708,
35.049806134273));
#152890=CARTESIAN_POINT('Ctrl Pts',(5.8674743568157,-3.83801657560389,35.0419542872591));
#152891=CARTESIAN_POINT('Ctrl Pts',(5.77252823929148,-3.98316808781822,
35.0341046669656));
#152892=CARTESIAN_POINT('Ctrl Pts',(5.67215318614924,-4.12485377024618,
35.0262550466721));
#152893=CARTESIAN_POINT('Ctrl Pts',(5.56665003843469,-4.26263227502621,
35.0184054263786));
#152894=CARTESIAN_POINT('Ctrl Pts',(5.46115531379702,-4.40039977995492,
35.0105564327769));
#152895=CARTESIAN_POINT('Ctrl Pts',(5.3505335421293,-4.53426042580745,35.0027074391751));
#152896=CARTESIAN_POINT('Ctrl Pts',(5.23512717183371,-4.66380424731017,
34.9948584455734));
#152897=CARTESIAN_POINT('Ctrl Pts',(5.1196623746722,-4.79341365305638,34.987005478256));
#152898=CARTESIAN_POINT('Ctrl Pts',(4.99940839307808,-4.91870158254952,
34.9791525109387));
#152899=CARTESIAN_POINT('Ctrl Pts',(4.8747462545793,-5.03929315638266,34.9712995436213));
#152900=CARTESIAN_POINT('Ctrl Pts',(4.7500524560862,-5.15991535642348,34.9634445819141));
#152901=CARTESIAN_POINT('Ctrl Pts',(4.62094855420437,-5.27583856974625,
34.955589620207));
#152902=CARTESIAN_POINT('Ctrl Pts',(4.48784978047786,-5.38672729125625,
34.9477346584998));
#152903=CARTESIAN_POINT('Ctrl Pts',(4.35461889509275,-5.49772607909148,
34.9398719000865));
#152904=CARTESIAN_POINT('Ctrl Pts',(4.21738552007152,-5.60368016150462,
34.9320091416732));
#152905=CARTESIAN_POINT('Ctrl Pts',(4.07659552794209,-5.70429622863877,
34.92414638326));
#152906=CARTESIAN_POINT('Ctrl Pts',(3.9733140099245,-5.77810673173918,34.9183783765114));
#152907=CARTESIAN_POINT('Ctrl Pts',(3.86811914002211,-5.84904548256678,
34.9126103697629));
#152908=CARTESIAN_POINT('Ctrl Pts',(3.76119543936316,-5.91701237360662,
34.9068423630144));
#152909=CARTESIAN_POINT('Ctrl Pts',(3.60588808496919,-6.01573471457243,
34.8984642965733));
#152910=CARTESIAN_POINT('Ctrl Pts',(3.44658844908803,-6.10840427875434,
34.8900862301323));
#152911=CARTESIAN_POINT('Ctrl Pts',(3.28379637756903,-6.19469998572687,
34.8817081636913));
#152912=CARTESIAN_POINT('Ctrl Pts',(3.12111562133438,-6.28093668472027,
34.8733358260725));
#152913=CARTESIAN_POINT('Ctrl Pts',(2.95494748011312,-6.36080806232932,
34.8649634884538));
#152914=CARTESIAN_POINT('Ctrl Pts',(2.78581836668374,-6.43403781387299,
34.8565911508351));
#152915=CARTESIAN_POINT('Ctrl Pts',(2.61678009883622,-6.50722823097416,
34.8482233103125));
#152916=CARTESIAN_POINT('Ctrl Pts',(2.44478433097249,-6.57378400487779,
34.8398554697899));
#152917=CARTESIAN_POINT('Ctrl Pts',(2.2703799385927,-6.63347582319675,34.8314876292673));
#152918=CARTESIAN_POINT('Ctrl Pts',(2.09604367636725,-6.6931443232223,34.8231230575974));
#152919=CARTESIAN_POINT('Ctrl Pts',(1.91930097649018,-6.74595410840673,
34.8147584859275));
#152920=CARTESIAN_POINT('Ctrl Pts',(1.74071888859076,-6.7917246935814,34.8063939142575));
#152921=CARTESIAN_POINT('Ctrl Pts',(1.5621804227333,-6.83748409842768,34.798031385792));
#152922=CARTESIAN_POINT('Ctrl Pts',(1.38180378309701,-6.87620765116248,
34.7896688573264));
#152923=CARTESIAN_POINT('Ctrl Pts',(1.20016975603081,-6.90776513202418,
34.7813063288608));
#152924=CARTESIAN_POINT('Ctrl Pts',(1.01852123400088,-6.93932513127159,
34.7729431330393));
#152925=CARTESIAN_POINT('Ctrl Pts',(0.835615446853467,-6.96371785390745,
34.7645799372178));
#152926=CARTESIAN_POINT('Ctrl Pts',(0.652042683505966,-6.98086433770105,
34.7562167413963));
#152927=CARTESIAN_POINT('Ctrl Pts',(0.468457400863963,-6.99801199085048,
34.7478529752216));
#152928=CARTESIAN_POINT('Ctrl Pts',(0.2842053786976,-7.00791238895933,34.7394892090469));
#152929=CARTESIAN_POINT('Ctrl Pts',(0.0998815072620535,-7.01053851333883,
34.7311254428721));
#152930=CARTESIAN_POINT('Ctrl Pts',(-0.0844795093998785,-7.01316516693891,
34.7227599912186));
#152931=CARTESIAN_POINT('Ctrl Pts',(-0.268912075450206,-7.00851461905335,
34.714394539565));
#152932=CARTESIAN_POINT('Ctrl Pts',(-0.452821386676273,-6.99661199111889,
34.7060290879115));
#152933=CARTESIAN_POINT('Ctrl Pts',(-0.636792288769169,-6.98470537701773,
34.6976608346846));
#152934=CARTESIAN_POINT('Ctrl Pts',(-0.820239258643686,-6.96554186118292,
34.6892925814577));
#152935=CARTESIAN_POINT('Ctrl Pts',(-1.00257226334437,-6.93919847095272,
34.6809243282308));
#152936=CARTESIAN_POINT('Ctrl Pts',(-1.18507431675295,-6.91283065664149,
34.6725483164394));
#152937=CARTESIAN_POINT('Ctrl Pts',(-1.3664600153948,-6.87926971278993,
34.6641723046479));
#152938=CARTESIAN_POINT('Ctrl Pts',(-1.54614794455608,-6.83864409777589,
34.6557962928564));
#152939=CARTESIAN_POINT('Ctrl Pts',(-1.72592399489802,-6.79799855945829,
34.6474161733653));
#152940=CARTESIAN_POINT('Ctrl Pts',(-1.90400029633817,-6.75028151973047,
34.6390360538741));
#152941=CARTESIAN_POINT('Ctrl Pts',(-2.07980962689676,-6.69567162265053,
34.630655934383));
#152942=CARTESIAN_POINT('Ctrl Pts',(-2.25581984188595,-6.64099932684553,
34.6222662395437));
#152943=CARTESIAN_POINT('Ctrl Pts',(-2.42955759793642,-6.57941853965937,
34.6138765447045));
#152944=CARTESIAN_POINT('Ctrl Pts',(-2.60047345402414,-6.51115691543491,
34.6054868498653));
#152945=CARTESIAN_POINT('Ctrl Pts',(-2.70898498160337,-6.46781878818804,
34.6001603773907));
#152946=CARTESIAN_POINT('Ctrl Pts',(-2.81635948020739,-6.42178874201992,
34.5948339049161));
#152947=CARTESIAN_POINT('Ctrl Pts',(-2.9224612963494,-6.37313474938667,
34.5895074324415));
#152948=CARTESIAN_POINT('Ctrl Pts',(-3.08941441566749,-6.2965768153874,
34.5811261320365));
#152949=CARTESIAN_POINT('Ctrl Pts',(-3.25355202745786,-6.21336537748145,
34.5727448316316));
#152950=CARTESIAN_POINT('Ctrl Pts',(-3.41432559772511,-6.12372495097707,
34.5643635312266));
#152951=CARTESIAN_POINT('Ctrl Pts',(-3.57489541102764,-6.03419813059084,
34.555992852893));
#152952=CARTESIAN_POINT('Ctrl Pts',(-3.73210939552516,-5.93825871759483,
34.5476221745593));
#152953=CARTESIAN_POINT('Ctrl Pts',(-3.88543996300208,-5.83617878893428,
34.5392514962257));
#152954=CARTESIAN_POINT('Ctrl Pts',(-4.03859652661053,-5.73421470346647,
34.5308903171748));
#152955=CARTESIAN_POINT('Ctrl Pts',(-4.18787818577808,-5.62612417165473,
34.5225291381239));
#152956=CARTESIAN_POINT('Ctrl Pts',(-4.33278251433605,-5.51222480002075,
34.514167959073));
#152957=CARTESIAN_POINT('Ctrl Pts',(-4.47749881243468,-5.39847322625713,
34.5058176296382));
#152958=CARTESIAN_POINT('Ctrl Pts',(-4.61784885310891,-5.27892804884745,
34.4974673002034));
#152959=CARTESIAN_POINT('Ctrl Pts',(-4.75335980002938,-5.1539496673876,
34.4891169707686));
#152960=CARTESIAN_POINT('Ctrl Pts',(-4.88876647938222,-5.02906744931628,
34.4807730664128));
#152961=CARTESIAN_POINT('Ctrl Pts',(-5.01934124519349,-4.89876057941237,
34.472429162057));
#152962=CARTESIAN_POINT('Ctrl Pts',(-5.14464404041121,-4.7634298840186,
34.4640852577012));
#152963=CARTESIAN_POINT('Ctrl Pts',(-5.26984619164242,-4.62820788708329,
34.4557480552214));
#152964=CARTESIAN_POINT('Ctrl Pts',(-5.38978459538553,-4.48797035194954,
34.4474108527416));
#152965=CARTESIAN_POINT('Ctrl Pts',(-5.50405569882937,-4.34315523861213,
34.4390736502618));
#152966=CARTESIAN_POINT('Ctrl Pts',(-5.54167311531509,-4.2954829026701,
34.4363290892262));
#152967=CARTESIAN_POINT('Ctrl Pts',(-5.57867667316407,-4.24731479163512,
34.4335845281906));
#152968=CARTESIAN_POINT('Ctrl Pts',(-5.61505288383928,-4.19866736884315,
34.430839967155));
#152969=CARTESIAN_POINT('Ctrl Pts',(-5.7255682370334,-4.05087058044642,
34.4225016568532));
#152970=CARTESIAN_POINT('Ctrl Pts',(-5.83019934000186,-3.89876854558231,
34.4141633465514));
#152971=CARTESIAN_POINT('Ctrl Pts',(-5.92862524298497,-3.74286378201792,
34.4058250362496));
#152972=CARTESIAN_POINT('Ctrl Pts',(-6.02711307220633,-3.58686092846663,
34.3974814797659));
#152973=CARTESIAN_POINT('Ctrl Pts',(-6.119387739315,-3.42705085103788,34.3891379232822));
#152974=CARTESIAN_POINT('Ctrl Pts',(-6.20517366432427,-3.26396175805975,
34.3807943667985));
#152975=CARTESIAN_POINT('Ctrl Pts',(-6.29102485489143,-3.10074858761046,
34.3724444625734));
#152976=CARTESIAN_POINT('Ctrl Pts',(-6.37037730408053,-2.93425171523097,
34.3640945583483));
#152977=CARTESIAN_POINT('Ctrl Pts',(-6.44300289213029,-2.76502084883654,
34.3557446541232));
#152978=CARTESIAN_POINT('Ctrl Pts',(-6.51573741318775,-2.59553614866579,
34.3473822256597));
#152979=CARTESIAN_POINT('Ctrl Pts',(-6.5817247811968,-2.42330956117124,
34.3390197971961));
#152980=CARTESIAN_POINT('Ctrl Pts',(-6.64078572320307,-2.24890896681086,
34.3306573687326));
#152981=CARTESIAN_POINT('Ctrl Pts',(-6.699897170366,-2.07435923616785,34.3222877892528));
#152982=CARTESIAN_POINT('Ctrl Pts',(-6.75207028098247,-1.89763210282481,
34.3139182097729));
#152983=CARTESIAN_POINT('Ctrl Pts',(-6.79717641353081,-1.71930781590747,
34.3055486302931));
#152984=CARTESIAN_POINT('Ctrl Pts',(-6.84235211679289,-1.54070848550448,
34.2971661417566));
#152985=CARTESIAN_POINT('Ctrl Pts',(-6.88043899300769,-1.36050739883639,
34.2887836532202));
#152986=CARTESIAN_POINT('Ctrl Pts',(-6.91135973017388,-1.1792935353977,
34.2804011646837));
#152987=CARTESIAN_POINT('Ctrl Pts',(-6.92147750204344,-1.11999738990093,
34.2776582770787));
#152988=CARTESIAN_POINT('Ctrl Pts',(-6.93082840628247,-1.06059283284357,
34.2749153894737));
#152989=CARTESIAN_POINT('Ctrl Pts',(-6.93941094439624,-1.00110054804385,
34.2721725018687));
#152990=CARTESIAN_POINT('Ctrl Pts',(-6.96566293201507,-0.819127487944901,
34.2637826467358));
#152991=CARTESIAN_POINT('Ctrl Pts',(-6.98477516963711,-0.635966017424542,
34.255392791603));
#152992=CARTESIAN_POINT('Ctrl Pts',(-6.99665206940579,-0.452201705193195,
34.2470029364702));
#152993=CARTESIAN_POINT('Ctrl Pts',(-7.00851800933787,-0.268606968093,34.238620823378));
#152994=CARTESIAN_POINT('Ctrl Pts',(-7.01316190024741,-0.0844108247111611,
34.2302387102859));
#152995=CARTESIAN_POINT('Ctrl Pts',(-7.01053975293831,0.0997944636322941,
34.2218565971937));
#152996=CARTESIAN_POINT('Ctrl Pts',(-7.00791963985978,0.283856847713138,
34.2134809868448));
#152997=CARTESIAN_POINT('Ctrl Pts',(-6.99804473149739,0.467928035097267,
34.2051053764959));
#152998=CARTESIAN_POINT('Ctrl Pts',(-6.98092305719494,0.651413718019586,
34.196729766147));
#152999=CARTESIAN_POINT('Ctrl Pts',(-6.96381215267988,0.834783985722573,
34.1883594241814));
#153000=CARTESIAN_POINT('Ctrl Pts',(-6.93946360157599,1.01756915684159,
34.1799890822158));
#153001=CARTESIAN_POINT('Ctrl Pts',(-6.90793744792243,1.19917754235601,
34.1716187402501));
#153002=CARTESIAN_POINT('Ctrl Pts',(-6.87642650330757,1.38069831524898,
34.1632524363558));
#153003=CARTESIAN_POINT('Ctrl Pts',(-6.83774491737662,1.56104311134469,
34.1548861324614));
#153004=CARTESIAN_POINT('Ctrl Pts',(-6.79200432149817,1.73962750589032,
34.146519828567));
#153005=CARTESIAN_POINT('Ctrl Pts',(-6.74627651798235,1.91816195538625,
34.1381558644934));
#153006=CARTESIAN_POINT('Ctrl Pts',(-6.69349372113455,2.09493666658613,
34.1297919004197));
#153007=CARTESIAN_POINT('Ctrl Pts',(-6.63381833132013,2.26937897001383,
34.1214279363461));
#153008=CARTESIAN_POINT('Ctrl Pts',(-6.5741521245565,2.44379442966994,34.1130652593475));
#153009=CARTESIAN_POINT('Ctrl Pts',(-6.50759554590933,2.61587788629101,
34.1047025823489));
#153010=CARTESIAN_POINT('Ctrl Pts',(-6.43436051071591,2.78507295786657,
34.0963399053503));
#153011=CARTESIAN_POINT('Ctrl Pts',(-6.36112698329804,2.95426454602481,
34.087977400524));
#153012=CARTESIAN_POINT('Ctrl Pts',(-6.28121540442131,3.12056756626644,
34.0796148956976));
#153013=CARTESIAN_POINT('Ctrl Pts',(-6.19488554339137,3.28344630941038,
34.0712523908713));
#153014=CARTESIAN_POINT('Ctrl Pts',(-6.10854595257947,3.44634340975584,
34.0628889435512));
#153015=CARTESIAN_POINT('Ctrl Pts',(-6.01578679179923,3.60581517344633,
34.0545254962312));
#153016=CARTESIAN_POINT('Ctrl Pts',(-5.91691362816744,3.76135077855104,
34.0461620489112));
#153017=CARTESIAN_POINT('Ctrl Pts',(-5.81798224523829,3.916977967391,34.0377936769584));
#153018=CARTESIAN_POINT('Ctrl Pts',(-5.71292984129663,4.06866408812234,
34.0294253050055));
#153019=CARTESIAN_POINT('Ctrl Pts',(-5.60210571350595,4.21592672341492,
34.0210569330527));
#153020=CARTESIAN_POINT('Ctrl Pts',(-5.49124837991019,4.36323348244173,
34.0126860537169));
#153021=CARTESIAN_POINT('Ctrl Pts',(-5.37461607605661,4.50611385375815,
34.0043151743811));
#153022=CARTESIAN_POINT('Ctrl Pts',(-5.25259863226846,4.64411823393758,
33.9959442950453));
#153023=CARTESIAN_POINT('Ctrl Pts',(-5.13047780441964,4.78223954373601,
33.987566323154));
#153024=CARTESIAN_POINT('Ctrl Pts',(-5.00296294130388,4.915476364326,33.9791883512626));
#153025=CARTESIAN_POINT('Ctrl Pts',(-4.87048179498309,5.04341487954722,
33.9708103793713));
#153026=CARTESIAN_POINT('Ctrl Pts',(-4.78628894770581,5.1247208477702,33.9654861100127));
#153027=CARTESIAN_POINT('Ctrl Pts',(-4.70009109629953,5.20388774031651,
33.9601618406542));
#153028=CARTESIAN_POINT('Ctrl Pts',(-4.61200508624403,5.28081770627989,
33.9548375712957));
#153029=CARTESIAN_POINT('Ctrl Pts',(-4.48192049048814,5.39442716046626,
33.9469747401064));
#153030=CARTESIAN_POINT('Ctrl Pts',(-4.34744573065238,5.50339217667764,
33.9391119089171));
#153031=CARTESIAN_POINT('Ctrl Pts',(-4.20896128643917,5.60734085389469,
33.9312490777279));
#153032=CARTESIAN_POINT('Ctrl Pts',(-4.07058324924164,5.71120966027432,
33.9233922880865));
#153033=CARTESIAN_POINT('Ctrl Pts',(-3.92820195746167,5.81006956527347,
33.9155354984452));
#153034=CARTESIAN_POINT('Ctrl Pts',(-3.78223311582231,5.90358697912355,
33.9076787088038));
#153035=CARTESIAN_POINT('Ctrl Pts',(-3.63634659369978,5.99705165357913,
33.8998263500199));
#153036=CARTESIAN_POINT('Ctrl Pts',(-3.48687686637915,6.08517962522162,
33.8919739912359));
#153037=CARTESIAN_POINT('Ctrl Pts',(-3.33427073828417,6.16767907776677,
33.884121632452));
#153038=CARTESIAN_POINT('Ctrl Pts',(-3.1817006422766,6.2501590512286,33.8762711277016));
#153039=CARTESIAN_POINT('Ctrl Pts',(-3.02599595045765,6.32701296201526,
33.8684206229512));
#153040=CARTESIAN_POINT('Ctrl Pts',(-2.86763027165357,6.39799368455425,
33.8605701182008));
#153041=CARTESIAN_POINT('Ctrl Pts',(-2.70929006889604,6.46896298853206,
33.8527208763492));
#153042=CARTESIAN_POINT('Ctrl Pts',(-2.54829008070091,6.53406083180059,
33.8448716344975));
#153043=CARTESIAN_POINT('Ctrl Pts',(-2.38512577786037,6.59308740927086,
33.8370223926459));
#153044=CARTESIAN_POINT('Ctrl Pts',(-2.22190650177241,6.65213387395047,
33.8291705062311));
#153045=CARTESIAN_POINT('Ctrl Pts',(-2.05652181359439,6.70510485710954,
33.8213186198162));
#153046=CARTESIAN_POINT('Ctrl Pts',(-1.88948448865828,6.75184974133902,
33.8134667334014));
#153047=CARTESIAN_POINT('Ctrl Pts',(-1.76683106002812,6.78617392800723,
33.8077011909374));
#153048=CARTESIAN_POINT('Ctrl Pts',(-1.64328693966225,6.81714216116094,
33.8019356484734));
#153049=CARTESIAN_POINT('Ctrl Pts',(-1.51905916836066,6.84471225147701,
33.7961701060094));
#153050=CARTESIAN_POINT('Ctrl Pts',(-1.31102029788735,6.89088268815237,
33.7865148016494));
#153051=CARTESIAN_POINT('Ctrl Pts',(-1.10117014471705,6.92749892086688,
33.7768594972894));
#153052=CARTESIAN_POINT('Ctrl Pts',(-0.890310616186968,6.95449304904425,
33.7672041929294));
#153053=CARTESIAN_POINT('Ctrl Pts',(-0.678282965425719,6.98163671962767,
33.7574953999946));
#153054=CARTESIAN_POINT('Ctrl Pts',(-0.465234778571069,6.99905142935194,
33.7477866070598));
#153055=CARTESIAN_POINT('Ctrl Pts',(-0.251976881838503,7.00672064617386,
33.738077814125));
#153056=CARTESIAN_POINT('Ctrl Pts',(-0.0376927699988857,7.01442676791832,
33.7283223016542));
#153057=CARTESIAN_POINT('Ctrl Pts',(0.176803030758819,7.01229340123778,
33.7185667891834));
#153058=CARTESIAN_POINT('Ctrl Pts',(0.390693177463751,7.00035609119874,
33.7088112767126));
#153059=CARTESIAN_POINT('Ctrl Pts',(0.604795108320485,6.98840696138623,
33.6990461047835));
#153060=CARTESIAN_POINT('Ctrl Pts',(0.818290147948013,6.96663448446964,
33.6892809328545));
#153061=CARTESIAN_POINT('Ctrl Pts',(1.03036436579813,6.93512623073246,33.6795157609255));
#153062=CARTESIAN_POINT('Ctrl Pts',(1.24214942526335,6.90366093778445,33.6697639035869));
#153063=CARTESIAN_POINT('Ctrl Pts',(1.45251749730597,6.86248640460992,33.6600120462483));
#153064=CARTESIAN_POINT('Ctrl Pts',(1.66066435004057,6.81174136906301,33.6502601889097));
#153065=CARTESIAN_POINT('Ctrl Pts',(1.75143145253539,6.7896128584366,33.6460076728474));
#153066=CARTESIAN_POINT('Ctrl Pts',(1.84177625504733,6.7656650905832,33.6417551567851));
#153067=CARTESIAN_POINT('Ctrl Pts',(1.93163247853303,6.73991265005537,33.6375026407228));
#153068=CARTESIAN_POINT('Ctrl Pts',(2.10137178816052,6.69126603096936,33.629469595124));
#153069=CARTESIAN_POINT('Ctrl Pts',(2.2694494660046,6.63615233030146,33.6214365495252));
#153070=CARTESIAN_POINT('Ctrl Pts',(2.43533104611058,6.57470830214923,33.6134035039265));
#153071=CARTESIAN_POINT('Ctrl Pts',(2.60110599114994,6.51330377258407,33.6053756222787));
#153072=CARTESIAN_POINT('Ctrl Pts',(2.76468730623457,6.44557714252613,33.597347740631));
#153073=CARTESIAN_POINT('Ctrl Pts',(2.92555509387023,6.37171515019543,33.5893198589832));
#153074=CARTESIAN_POINT('Ctrl Pts',(3.08635024811383,6.29788650728245,33.5812956020031));
#153075=CARTESIAN_POINT('Ctrl Pts',(3.24443398195006,6.21792817047563,33.5732713450231));
#153076=CARTESIAN_POINT('Ctrl Pts',(3.39930586596518,6.13207519459071,33.565247088043));
#153077=CARTESIAN_POINT('Ctrl Pts',(3.55415902439219,6.04623259920498,33.5572238012774));
#153078=CARTESIAN_POINT('Ctrl Pts',(3.70580078236128,5.95449695524091,33.5492005145117));
#153079=CARTESIAN_POINT('Ctrl Pts',(3.85375468587841,5.8571495954577,33.5411772277461));
#153080=CARTESIAN_POINT('Ctrl Pts',(4.00169646589286,5.75981021242229,33.5331545984172));
#153081=CARTESIAN_POINT('Ctrl Pts',(4.1459506892983,5.65686023438918,33.5251319690883));
#153082=CARTESIAN_POINT('Ctrl Pts',(4.28606956806187,5.54862453408355,33.5171093397594));
#153083=CARTESIAN_POINT('Ctrl Pts',(4.42624112154857,5.44034814486009,33.5090836944931));
#153084=CARTESIAN_POINT('Ctrl Pts',(4.5622739363716,5.32678229050574,33.5010580492267));
#153085=CARTESIAN_POINT('Ctrl Pts',(4.69375272997403,5.20829260625412,33.4930324039604));
#153086=CARTESIAN_POINT('Ctrl Pts',(4.77128063860812,5.13842386801091,33.4882999944524));
#153087=CARTESIAN_POINT('Ctrl Pts',(4.8472257603242,5.06684386173666,33.4835675849445));
#153088=CARTESIAN_POINT('Ctrl Pts',(4.92150891237664,4.99363360569208,33.4788351754365));
#153089=CARTESIAN_POINT('Ctrl Pts',(5.05853405375793,4.85858756351571,33.4701056174683));
#153090=CARTESIAN_POINT('Ctrl Pts',(5.18997071682224,4.7179250387306,33.4613760595001));
#153091=CARTESIAN_POINT('Ctrl Pts',(5.31538360554547,4.57212463614001,33.4526465015319));
#153092=CARTESIAN_POINT('Ctrl Pts',(5.44083371828673,4.42628095827788,33.4439143525284));
#153093=CARTESIAN_POINT('Ctrl Pts',(5.56025630903054,4.27529656607037,33.4351822035249));
#153094=CARTESIAN_POINT('Ctrl Pts',(5.67325609237645,4.11968346755105,33.4264500545214));
#153095=CARTESIAN_POINT('Ctrl Pts',(5.78630777788146,3.96399889406464,33.4177138947368));
#153096=CARTESIAN_POINT('Ctrl Pts',(5.89293059881551,3.80368158680107,33.4089777349523));
#153097=CARTESIAN_POINT('Ctrl Pts',(5.99277161017516,3.6392739647873,33.4002415751678));
#153098=CARTESIAN_POINT('Ctrl Pts',(6.09262680060904,3.47484299417315,33.3915041747041));
#153099=CARTESIAN_POINT('Ctrl Pts',(6.18569811946792,3.30632078499796,33.3827667742404));
#153100=CARTESIAN_POINT('Ctrl Pts',(6.27167754167765,3.1342762124159,33.3740293737768));
#153101=CARTESIAN_POINT('Ctrl Pts',(6.35767791546194,2.9621897157944,33.3652898441723));
#153102=CARTESIAN_POINT('Ctrl Pts',(6.43658281800373,2.78657938614114,33.3565503145678));
#153103=CARTESIAN_POINT('Ctrl Pts',(6.50813099130387,2.60803710911676,33.3478107849634));
#153104=CARTESIAN_POINT('Ctrl Pts',(6.52980024043262,2.55396337246626,33.3451639103398));
#153105=CARTESIAN_POINT('Ctrl Pts',(6.5507950217826,2.49962084380071,33.3425170357163));
#153106=CARTESIAN_POINT('Ctrl Pts',(6.57110895151813,2.44502632087639,33.3398701610928));
#153107=CARTESIAN_POINT('Origin',(0.,0.,50.));
#153108=CARTESIAN_POINT('',(6.57110895151815,2.44502632087633,31.3397623334207));
#153109=CARTESIAN_POINT('',(6.57110895151813,2.44502632087638,31.8871164994866));
#153110=CARTESIAN_POINT('',(6.57110895151814,2.44502632087636,50.));
#153111=CARTESIAN_POINT('',(7.01124984252467,-0.00148600059847291,33.7735343568733));
#153112=CARTESIAN_POINT('Ctrl Pts',(6.57110895151814,2.44502632087638,31.8871164994866));
#153113=CARTESIAN_POINT('Ctrl Pts',(6.50762598931832,2.6156393967432,31.8953699009264));
#153114=CARTESIAN_POINT('Ctrl Pts',(6.43748316425011,2.78380827029697,31.9036233023662));
#153115=CARTESIAN_POINT('Ctrl Pts',(6.36090066196278,2.94899463057184,31.911876703806));
#153116=CARTESIAN_POINT('Ctrl Pts',(6.28432000714449,3.11417700590656,31.9201299061415));
#153117=CARTESIAN_POINT('Ctrl Pts',(6.20130012895755,3.27637670157163,31.928383108477));
#153118=CARTESIAN_POINT('Ctrl Pts',(6.11210852405168,3.43507728482414,31.9366363108125));
#153119=CARTESIAN_POINT('Ctrl Pts',(6.02290496113898,3.59379914522106,31.9448906196631));
#153120=CARTESIAN_POINT('Ctrl Pts',(5.92752819059685,3.74902066080693,31.9531449285136));
#153121=CARTESIAN_POINT('Ctrl Pts',(5.82629077728874,3.90025157406291,31.9613992373641));
#153122=CARTESIAN_POINT('Ctrl Pts',(5.72499006368819,4.05157704683718,31.9696587073517));
#153123=CARTESIAN_POINT('Ctrl Pts',(5.61782157723185,4.19890664855539,31.9779181773393));
#153124=CARTESIAN_POINT('Ctrl Pts',(5.50514067103692,4.34177990628212,31.9861776473268));
#153125=CARTESIAN_POINT('Ctrl Pts',(5.39241852474357,4.48470545420964,31.9944401401988));
#153126=CARTESIAN_POINT('Ctrl Pts',(5.27418015407174,4.62317114316824,32.0027026330708));
#153127=CARTESIAN_POINT('Ctrl Pts',(5.15082027315724,4.75675068467252,32.0109651259428));
#153128=CARTESIAN_POINT('Ctrl Pts',(5.02735435984748,4.89044504274954,32.019234720734));
#153129=CARTESIAN_POINT('Ctrl Pts',(4.89875838211137,5.01924462032444,32.0275043155252));
#153130=CARTESIAN_POINT('Ctrl Pts',(4.76546346532463,5.14276039915882,32.0357739103165));
#153131=CARTESIAN_POINT('Ctrl Pts',(4.73024018932418,5.1753995310415,32.0379591565866));
#153132=CARTESIAN_POINT('Ctrl Pts',(4.69468897339523,5.20766992130522,32.0401444028568));
#153133=CARTESIAN_POINT('Ctrl Pts',(4.65881814938141,5.2395648687171,32.042329649127));
#153134=CARTESIAN_POINT('Ctrl Pts',(4.52974975206116,5.35432748870817,32.0501924803163));
#153135=CARTESIAN_POINT('Ctrl Pts',(4.39625003216115,5.46448492412669,32.0580553115057));
#153136=CARTESIAN_POINT('Ctrl Pts',(4.25869614464996,5.5696619026691,32.065918142695));
#153137=CARTESIAN_POINT('Ctrl Pts',(4.12124794914417,5.67475806658689,32.0737749323364));
#153138=CARTESIAN_POINT('Ctrl Pts',(3.9797520817573,5.77488115372705,32.0816317219779));
#153139=CARTESIAN_POINT('Ctrl Pts',(3.83462126202782,5.86969388804085,32.0894885116194));
#153140=CARTESIAN_POINT('Ctrl Pts',(3.68957228921087,5.96445315246049,32.0973408704034));
#153141=CARTESIAN_POINT('Ctrl Pts',(3.54089276005286,6.05390781349602,32.1051932291874));
#153142=CARTESIAN_POINT('Ctrl Pts',(3.38902686431709,6.13776209016259,32.1130455879714));
#153143=CARTESIAN_POINT('Ctrl Pts',(3.23719682589128,6.22159656785603,32.1208960927218));
#153144=CARTESIAN_POINT('Ctrl Pts',(3.0821822476397,6.29983310144248,32.1287465974723));
#153145=CARTESIAN_POINT('Ctrl Pts',(2.92445452038378,6.37222036033806,32.1365971022228));
#153146=CARTESIAN_POINT('Ctrl Pts',(2.76675216654805,6.44459597440511,32.1444463440744));
#153147=CARTESIAN_POINT('Ctrl Pts',(2.60633788058183,6.51112403055832,32.1522955859261));
#153148=CARTESIAN_POINT('Ctrl Pts',(2.44370533552698,6.57160032226679,32.1601448277778));
#153149=CARTESIAN_POINT('Ctrl Pts',(2.2810179963844,6.63209698962167,32.1679967141927));
#153150=CARTESIAN_POINT('Ctrl Pts',(2.11611126323491,6.68653768674299,32.1758486006076));
#153151=CARTESIAN_POINT('Ctrl Pts',(1.94949655071189,6.73476723883331,32.1837004870225));
#153152=CARTESIAN_POINT('Ctrl Pts',(1.8271534411247,6.77018159863009,32.1894660294862));
#153153=CARTESIAN_POINT('Ctrl Pts',(1.70388980936199,6.80224806436027,32.1952315719499));
#153154=CARTESIAN_POINT('Ctrl Pts',(1.5799123125686,6.83092260584865,32.2009971144136));
#153155=CARTESIAN_POINT('Ctrl Pts',(1.37229256597395,6.87894261908909,32.2106524187732));
#153156=CARTESIAN_POINT('Ctrl Pts',(1.16277658247089,6.91742492590143,32.2203077231329));
#153157=CARTESIAN_POINT('Ctrl Pts',(0.952165633372154,6.94629449196656,
32.2299630274926));
#153158=CARTESIAN_POINT('Ctrl Pts',(0.740387939123326,6.97532399001214,
32.2396718204272));
#153159=CARTESIAN_POINT('Ctrl Pts',(0.52750316803832,6.99463399454275,32.2493806133618));
#153160=CARTESIAN_POINT('Ctrl Pts',(0.314321967100086,7.00420075836625,
32.2590894062964));
#153161=CARTESIAN_POINT('Ctrl Pts',(0.100114920123539,7.0138135582695,32.2688449187669));
#153162=CARTESIAN_POINT('Ctrl Pts',(-0.114391372164453,7.01358914327749,
32.2786004312374));
#153163=CARTESIAN_POINT('Ctrl Pts',(-0.328379282832671,7.00355578325084,
32.2883559437079));
#153164=CARTESIAN_POINT('Ctrl Pts',(-0.542579074453864,6.99351248865416,
32.2981211156366));
#153165=CARTESIAN_POINT('Ctrl Pts',(-0.756259420008023,6.97364083503563,
32.3078862875653));
#153166=CARTESIAN_POINT('Ctrl Pts',(-0.968605641862296,6.94402114578092,
32.317651459494));
#153167=CARTESIAN_POINT('Ctrl Pts',(-1.18066233446117,6.91444184230044,
32.3274033168324));
#153168=CARTESIAN_POINT('Ctrl Pts',(-1.39138850140542,6.87514107285008,
32.3371551741707));
#153169=CARTESIAN_POINT('Ctrl Pts',(-1.59997870798422,6.82625041267145,
32.346907031509));
#153170=CARTESIAN_POINT('Ctrl Pts',(-1.69093914489552,6.80493054399847,
32.3511595475727));
#153171=CARTESIAN_POINT('Ctrl Pts',(-1.78149348870259,6.78178773195593,
32.3554120636363));
#153172=CARTESIAN_POINT('Ctrl Pts',(-1.87157533319403,6.75683597068034,
32.3596645796999));
#153173=CARTESIAN_POINT('Ctrl Pts',(-2.04174084311919,6.70970184276628,
32.3676976252988));
#153174=CARTESIAN_POINT('Ctrl Pts',(-2.2103023397027,6.65608610196862,32.3757306708977));
#153175=CARTESIAN_POINT('Ctrl Pts',(-2.37672416113583,6.59612074058482,
32.3837637164966));
#153176=CARTESIAN_POINT('Ctrl Pts',(-2.54303900021432,6.53619392724419,
32.3917915981445));
#153177=CARTESIAN_POINT('Ctrl Pts',(-2.70721655861343,6.46992574194481,
32.3998194797924));
#153178=CARTESIAN_POINT('Ctrl Pts',(-2.86873529758317,6.39749828877667,
32.4078473614403));
#153179=CARTESIAN_POINT('Ctrl Pts',(-3.03018110924926,6.32510353731797,
32.4158716184204));
#153180=CARTESIAN_POINT('Ctrl Pts',(-3.18897015799944,6.24655520489625,
32.4238958754005));
#153181=CARTESIAN_POINT('Ctrl Pts',(-3.34459994240831,6.16208388353667,
32.4319201323807));
#153182=CARTESIAN_POINT('Ctrl Pts',(-3.50021090959193,6.07762277561976,
32.4399434191465));
#153183=CARTESIAN_POINT('Ctrl Pts',(-3.65266304762526,5.98724027320072,
32.4479667059122));
#153184=CARTESIAN_POINT('Ctrl Pts',(-3.80147741771086,5.89121345778053,
32.455989992678));
#153185=CARTESIAN_POINT('Ctrl Pts',(-3.95027959378598,5.79519451090147,
32.464012622007));
#153186=CARTESIAN_POINT('Ctrl Pts',(-4.09544428977,5.69353237444891,32.472035251336));
#153187=CARTESIAN_POINT('Ctrl Pts',(-4.23652084421534,5.58654792327328,
32.480057880665));
#153188=CARTESIAN_POINT('Ctrl Pts',(-4.37765043340174,5.47952325356036,
32.4880835259314));
#153189=CARTESIAN_POINT('Ctrl Pts',(-4.51468852047096,5.3671724962097,32.4961091711979));
#153190=CARTESIAN_POINT('Ctrl Pts',(-4.64721658540546,5.24985757624266,
32.5041348164644));
#153191=CARTESIAN_POINT('Ctrl Pts',(-4.72536320834495,5.18068155061841,
32.5088672259717));
#153192=CARTESIAN_POINT('Ctrl Pts',(-4.80194233617012,5.10978023899885,
32.5135996354791));
#153193=CARTESIAN_POINT('Ctrl Pts',(-4.87687406826338,5.03723395176363,
32.5183320449864));
#153194=CARTESIAN_POINT('Ctrl Pts',(-5.01510337395136,4.90340516341685,
32.527062093821));
#153195=CARTESIAN_POINT('Ctrl Pts',(-5.14779378229039,4.76390974366043,
32.5357921426555));
#153196=CARTESIAN_POINT('Ctrl Pts',(-5.27450568218276,4.61922248556202,
32.54452219149));
#153197=CARTESIAN_POINT('Ctrl Pts',(-5.40125422097954,4.47449339096188,
32.5532547646291));
#153198=CARTESIAN_POINT('Ctrl Pts',(-5.52202062028321,4.32456966757488,
32.5619873377682));
#153199=CARTESIAN_POINT('Ctrl Pts',(-5.63640499889543,4.16995986202824,
32.5707199109073));
#153200=CARTESIAN_POINT('Ctrl Pts',(-5.75241439019912,4.01315357738816,
32.5795765441878));
#153201=CARTESIAN_POINT('Ctrl Pts',(-5.86185887281638,3.85152728226869,
32.5884331774682));
#153202=CARTESIAN_POINT('Ctrl Pts',(-5.96436600366898,3.68564305607282,
32.5972898107487));
#153203=CARTESIAN_POINT('Ctrl Pts',(-6.06550159581761,3.52197834996995,
32.6060279428553));
#153204=CARTESIAN_POINT('Ctrl Pts',(-6.15988419962545,3.35416919531648,
32.6147660749619));
#153205=CARTESIAN_POINT('Ctrl Pts',(-6.24720130009147,3.18278219151664,
32.6235042070686));
#153206=CARTESIAN_POINT('Ctrl Pts',(-6.33629461178435,3.00790881999889,
32.6324200909359));
#153207=CARTESIAN_POINT('Ctrl Pts',(-6.41803174921255,2.82931074059938,
32.6413359748033));
#153208=CARTESIAN_POINT('Ctrl Pts',(-6.49213095548987,2.64761443931519,
32.6502518586706));
#153209=CARTESIAN_POINT('Ctrl Pts',(-6.56623016176718,2.46591813803099,
32.659167742538));
#153210=CARTESIAN_POINT('Ctrl Pts',(-6.63269132832819,2.28112389718056,
32.6680836264054));
#153211=CARTESIAN_POINT('Ctrl Pts',(-6.69128520431699,2.0938789069544,32.6769995102727));
#153212=CARTESIAN_POINT('Ctrl Pts',(-6.74872769583583,1.91031332810334,
32.685740194769));
#153213=CARTESIAN_POINT('Ctrl Pts',(-6.79861531624983,1.72437292502866,
32.6944808792653));
#153214=CARTESIAN_POINT('Ctrl Pts',(-6.84077743513127,1.53668169947419,
32.7032215637616));
#153215=CARTESIAN_POINT('Ctrl Pts',(-6.88293196834713,1.34902424268907,
32.7119606756636));
#153216=CARTESIAN_POINT('Ctrl Pts',(-6.9173637158717,1.15961685954915,32.7206997875655));
#153217=CARTESIAN_POINT('Ctrl Pts',(-6.94395283789062,0.969095221147462,
32.7294388994675));
#153218=CARTESIAN_POINT('Ctrl Pts',(-6.97088646025336,0.776105100714336,
32.7382912391418));
#153219=CARTESIAN_POINT('Ctrl Pts',(-6.98977275377,0.581971929352691,32.7471435788161));
#153220=CARTESIAN_POINT('Ctrl Pts',(-7.00054105897722,0.387364742941425,
32.7559959184904));
#153221=CARTESIAN_POINT('Ctrl Pts',(-7.01116618111522,0.195345192533053,
32.7647305511403));
#153222=CARTESIAN_POINT('Ctrl Pts',(-7.01388785773924,0.00286443576630693,
32.7734651837901));
#153223=CARTESIAN_POINT('Ctrl Pts',(-7.0086904969564,-0.189430938268088,
32.78219981644));
#153224=CARTESIAN_POINT('Ctrl Pts',(-7.00338807751271,-0.38561334176364,
32.7911110096265));
#153225=CARTESIAN_POINT('Ctrl Pts',(-6.98984304867562,-0.581602497256222,
32.8000222028131));
#153226=CARTESIAN_POINT('Ctrl Pts',(-6.96809478004038,-0.776712108103157,
32.8089333959996));
#153227=CARTESIAN_POINT('Ctrl Pts',(-6.94634651140514,-0.971821718950125,
32.8178445891861));
#153228=CARTESIAN_POINT('Ctrl Pts',(-6.91639502316164,-1.16605148239483,
32.8267557823727));
#153229=CARTESIAN_POINT('Ctrl Pts',(-6.87833604413308,-1.35871992201471,
32.8356669755592));
#153230=CARTESIAN_POINT('Ctrl Pts',(-6.84405908436904,-1.53224240005324,
32.8436926404116));
#153231=CARTESIAN_POINT('Ctrl Pts',(-6.80318963512244,-1.70457808617821,
32.8517183052639));
#153232=CARTESIAN_POINT('Ctrl Pts',(-6.75583514478471,-1.87518480662354,
32.8597439701162));
#153233=CARTESIAN_POINT('Ctrl Pts',(-6.70849568360071,-2.04573738068047,
32.8677670878194));
#153234=CARTESIAN_POINT('Ctrl Pts',(-6.65467537691853,-2.21456172873366,
32.8757902055225));
#153235=CARTESIAN_POINT('Ctrl Pts',(-6.59453233375685,-2.3811278549325,
32.8838133232257));
#153236=CARTESIAN_POINT('Ctrl Pts',(-6.53439687515926,-2.54767297568509,
32.8918354291435));
#153237=CARTESIAN_POINT('Ctrl Pts',(-6.46794039333055,-2.71196009735109,
32.8998575350613));
#153238=CARTESIAN_POINT('Ctrl Pts',(-6.39537020827451,-2.87347637220403,
32.9078796409791));
#153239=CARTESIAN_POINT('Ctrl Pts',(-6.32277305589253,-3.03505266705039,
32.9159047279386));
#153240=CARTESIAN_POINT('Ctrl Pts',(-6.24405780943784,-3.19385572224353,
32.9239298148981));
#153241=CARTESIAN_POINT('Ctrl Pts',(-6.15947929165377,-3.34939418674309,
32.9319549018575));
#153242=CARTESIAN_POINT('Ctrl Pts',(-6.07488411655371,-3.50496328376517,
32.9399815693177));
#153243=CARTESIAN_POINT('Ctrl Pts',(-5.98442355254028,-3.65726619141962,
32.9480082367779));
#153244=CARTESIAN_POINT('Ctrl Pts',(-5.8883972550525,-3.80583819009561,
32.9560349042381));
#153245=CARTESIAN_POINT('Ctrl Pts',(-5.79229386799168,-3.95452946184827,
32.9640680154786));
#153246=CARTESIAN_POINT('Ctrl Pts',(-5.69061603018767,-4.09948353977782,
32.9721011267192));
#153247=CARTESIAN_POINT('Ctrl Pts',(-5.58370576002964,-4.24026609399833,
32.9801342379597));
#153248=CARTESIAN_POINT('Ctrl Pts',(-5.52071034512014,-4.32322028915685,
32.9848676389217));
#153249=CARTESIAN_POINT('Ctrl Pts',(-5.45589900390423,-4.40472675175332,
32.9896010398836));
#153250=CARTESIAN_POINT('Ctrl Pts',(-5.38934796350373,-4.48470234137989,
32.9943344408456));
#153251=CARTESIAN_POINT('Ctrl Pts',(-5.25225074908031,-4.6494545450072,
33.00408539414));
#153252=CARTESIAN_POINT('Ctrl Pts',(-5.10768840988505,-4.80780577014889,
33.0138363474343));
#153253=CARTESIAN_POINT('Ctrl Pts',(-4.95623241000825,-4.95917199343639,
33.0235873007287));
#153254=CARTESIAN_POINT('Ctrl Pts',(-4.80455820934961,-5.11075628816571,
33.0333523021006));
#153255=CARTESIAN_POINT('Ctrl Pts',(-4.64597050918983,-5.25533542435829,
33.0431173034725));
#153256=CARTESIAN_POINT('Ctrl Pts',(-4.48107791694203,-5.39236193748106,
33.0528823048444));
#153257=CARTESIAN_POINT('Ctrl Pts',(-4.31646016648299,-5.52916005579566,
33.0626310299821));
#153258=CARTESIAN_POINT('Ctrl Pts',(-4.14555855621277,-5.65843068642626,
33.0723797551198));
#153259=CARTESIAN_POINT('Ctrl Pts',(-3.96901263390927,-5.77966826680984,
33.0821284802576));
#153260=CARTESIAN_POINT('Ctrl Pts',(-3.79295126170702,-5.90057309704499,
33.0918504489248));
#153261=CARTESIAN_POINT('Ctrl Pts',(-3.61127653653412,-6.01348886887274,
33.1015724175921));
#153262=CARTESIAN_POINT('Ctrl Pts',(-3.42465619383811,-6.11795362163741,
33.1112943862594));
#153263=CARTESIAN_POINT('Ctrl Pts',(-3.23927066920705,-6.22172715841779,
33.1209520271993));
#153264=CARTESIAN_POINT('Ctrl Pts',(-3.04900478506897,-6.31716109486227,
33.1306096681391));
#153265=CARTESIAN_POINT('Ctrl Pts',(-2.85454578800082,-6.40384219876683,
33.140267309079));
#153266=CARTESIAN_POINT('Ctrl Pts',(-2.76907436399434,-6.4419415281724,
33.1445121747634));
#153267=CARTESIAN_POINT('Ctrl Pts',(-2.6827932943079,-6.47835041455719,
33.1487570404477));
#153268=CARTESIAN_POINT('Ctrl Pts',(-2.59576293581742,-6.51303626149406,
33.1530019061321));
#153269=CARTESIAN_POINT('Ctrl Pts',(-2.43478044279226,-6.57719564460401,
33.160853753146));
#153270=CARTESIAN_POINT('Ctrl Pts',(-2.27129897621931,-6.63542977659479,
33.1687056001598));
#153271=CARTESIAN_POINT('Ctrl Pts',(-2.10581350796627,-6.68753886210516,
33.1765574471737));
#153272=CARTESIAN_POINT('Ctrl Pts',(-1.94037497005416,-6.73963316990016,
33.1844070674672));
#153273=CARTESIAN_POINT('Ctrl Pts',(-1.77293392443771,-6.78560577197313,
33.1922566877607));
#153274=CARTESIAN_POINT('Ctrl Pts',(-1.60400279985007,-6.82530596974034,
33.2001063080542));
#153275=CARTESIAN_POINT('Ctrl Pts',(-1.43508516225289,-6.86500299795434,
33.207955301656));
#153276=CARTESIAN_POINT('Ctrl Pts',(-1.26467805402748,-6.89842853222061,
33.2158042952577));
#153277=CARTESIAN_POINT('Ctrl Pts',(-1.09330619583859,-6.9254825192647,
33.2236532888594));
#153278=CARTESIAN_POINT('Ctrl Pts',(-0.921847577095081,-6.95255020295039,
33.2315062561767));
#153279=CARTESIAN_POINT('Ctrl Pts',(-0.74942360978009,-6.97323983468652,
33.2393592234941));
#153280=CARTESIAN_POINT('Ctrl Pts',(-0.576566617006927,-6.98750295160247,
33.2472121908115));
#153281=CARTESIAN_POINT('Ctrl Pts',(-0.403665724365122,-7.00176969087091,
33.2550671525187));
#153282=CARTESIAN_POINT('Ctrl Pts',(-0.23033196829142,-7.00960664652511,
33.262922114226));
#153283=CARTESIAN_POINT('Ctrl Pts',(-0.0570991721866667,-7.01101749013905,
33.2707770759332));
#153284=CARTESIAN_POINT('Ctrl Pts',(0.116305571947877,-7.0124297341332,
33.2786398343465));
#153285=CARTESIAN_POINT('Ctrl Pts',(0.289608774828138,-7.00740313774596,
33.2865025927598));
#153286=CARTESIAN_POINT('Ctrl Pts',(0.462279656661582,-6.99599343063849,
33.2943653511731));
#153287=CARTESIAN_POINT('Ctrl Pts',(0.588948537902381,-6.9876234332235,
33.3001333579215));
#153288=CARTESIAN_POINT('Ctrl Pts',(0.715277210139274,-6.97581946807651,
33.30590136467));
#153289=CARTESIAN_POINT('Ctrl Pts',(0.841059499435936,-6.96062105568954,
33.3116693714184));
#153290=CARTESIAN_POINT('Ctrl Pts',(1.02375907362051,-6.9385452651557,33.3200474378595));
#153291=CARTESIAN_POINT('Ctrl Pts',(1.20571028047133,-6.90925737613366,
33.3284255043006));
#153292=CARTESIAN_POINT('Ctrl Pts',(1.38632299124725,-6.8728258472363,33.3368035707416));
#153293=CARTESIAN_POINT('Ctrl Pts',(1.56681220119751,-6.83641922978552,
33.3451759083604));
#153294=CARTESIAN_POINT('Ctrl Pts',(1.74596441859894,-6.7928787759688,33.3535482459792));
#153295=CARTESIAN_POINT('Ctrl Pts',(1.92319734510185,-6.74232441627464,
33.3619205835979));
#153296=CARTESIAN_POINT('Ctrl Pts',(2.10033507316078,-6.69179721122085,
33.3702884241206));
#153297=CARTESIAN_POINT('Ctrl Pts',(2.27555525047526,-6.63426370215943,
33.3786562646432));
#153298=CARTESIAN_POINT('Ctrl Pts',(2.44828798851151,-6.56989440461643,
33.3870241051658));
#153299=CARTESIAN_POINT('Ctrl Pts',(2.62095324941777,-6.50555025259886,
33.3953886768358));
#153300=CARTESIAN_POINT('Ctrl Pts',(2.79113270119787,-6.43437575180299,
33.4037532485058));
#153301=CARTESIAN_POINT('Ctrl Pts',(2.95827334529808,-6.35659070390716,
33.4121178201758));
#153302=CARTESIAN_POINT('Ctrl Pts',(3.12537316214558,-6.27882465647543,
33.4204803486415));
#153303=CARTESIAN_POINT('Ctrl Pts',(3.28943535406032,-6.19445142109821,
33.4288428771072));
#153304=CARTESIAN_POINT('Ctrl Pts',(3.44992815628357,-6.10373838552914,
33.4372054055729));
#153305=CARTESIAN_POINT('Ctrl Pts',(3.61043376633267,-6.01301811077708,
33.4455686013944));
#153306=CARTESIAN_POINT('Ctrl Pts',(3.76736912850284,-5.91595718150947,
33.4539317972159));
#153307=CARTESIAN_POINT('Ctrl Pts',(3.92022761570562,-5.81286865528192,
33.4622949930375));
#153308=CARTESIAN_POINT('Ctrl Pts',(4.07309652755098,-5.70977309862342,
33.4706587592122));
#153309=CARTESIAN_POINT('Ctrl Pts',(4.22188773728259,-5.60064930899922,
33.4790225253869));
#153310=CARTESIAN_POINT('Ctrl Pts',(4.36612398131493,-5.48585343791526,
33.4873862915617));
#153311=CARTESIAN_POINT('Ctrl Pts',(4.51038929205391,-5.37103443299327,
33.4957517432153));
#153312=CARTESIAN_POINT('Ctrl Pts',(4.65009754948598,-5.25054127210444,
33.5041171948688));
#153313=CARTESIAN_POINT('Ctrl Pts',(4.78480460374487,-5.12477038182999,
33.5124826465224));
#153314=CARTESIAN_POINT('Ctrl Pts',(4.91955677113244,-4.99895737113069,
33.5208508997494));
#153315=CARTESIAN_POINT('Ctrl Pts',(5.04930415533888,-4.86786333088658,
33.5292191529763));
#153316=CARTESIAN_POINT('Ctrl Pts',(5.17363919570639,-4.73192181202844,
33.5375874062033));
#153317=CARTESIAN_POINT('Ctrl Pts',(5.29808951239366,-4.59585425598923,
33.5459634179948));
#153318=CARTESIAN_POINT('Ctrl Pts',(5.41711723562476,-4.45493048323752,
33.5543394297862));
#153319=CARTESIAN_POINT('Ctrl Pts',(5.53035406856111,-4.30961836348065,
33.5627154415777));
#153320=CARTESIAN_POINT('Ctrl Pts',(5.64364643423984,-4.16423498086432,
33.5710955610689));
#153321=CARTESIAN_POINT('Ctrl Pts',(5.75114204946101,-4.01445922273378,
33.5794756805601));
#153322=CARTESIAN_POINT('Ctrl Pts',(5.85251540366539,-3.86078878111187,
33.5878558000513));
#153323=CARTESIAN_POINT('Ctrl Pts',(5.95400458976775,-3.70694275154522,
33.5962454948905));
#153324=CARTESIAN_POINT('Ctrl Pts',(6.04935736084891,-3.54919342420882,
33.6046351897297));
#153325=CARTESIAN_POINT('Ctrl Pts',(6.1382930230822,-3.38806513002339,33.613024884569));
#153326=CARTESIAN_POINT('Ctrl Pts',(6.1947567402894,-3.28576755660341,33.6183513570431));
#153327=CARTESIAN_POINT('Ctrl Pts',(6.24863480532729,-3.18210848943555,
33.6236778295173));
#153328=CARTESIAN_POINT('Ctrl Pts',(6.299865374172,-3.07722648334644,33.6290043019914));
#153329=CARTESIAN_POINT('Ctrl Pts',(6.38140366550722,-2.91029685985858,
33.6374818862576));
#153330=CARTESIAN_POINT('Ctrl Pts',(6.45639289574677,-2.73994110069037,
33.6459594705238));
#153331=CARTESIAN_POINT('Ctrl Pts',(6.52454701389006,-2.56669297463455,
33.65443705479));
#153332=CARTESIAN_POINT('Ctrl Pts',(6.59260653858626,-2.39368530561771,
33.6629028727251));
#153333=CARTESIAN_POINT('Ctrl Pts',(6.6538497482956,-2.21779356304895,33.6713686906602));
#153334=CARTESIAN_POINT('Ctrl Pts',(6.70803706498751,-2.03957478344232,
33.6798345085954));
#153335=CARTESIAN_POINT('Ctrl Pts',(6.76212856497949,-1.86167113911769,
33.6882853568515));
#153336=CARTESIAN_POINT('Ctrl Pts',(6.80918896995622,-1.68144896544347,
33.6967362051076));
#153337=CARTESIAN_POINT('Ctrl Pts',(6.84902733914818,-1.49948360114435,
33.7051870533637));
#153338=CARTESIAN_POINT('Ctrl Pts',(6.88882413540738,-1.31770812498592,
33.7136290828215));
#153339=CARTESIAN_POINT('Ctrl Pts',(6.92141385003952,-1.13419338926625,
33.7220711122792));
#153340=CARTESIAN_POINT('Ctrl Pts',(6.94665528797605,-0.949529816558885,
33.7305131417369));
#153341=CARTESIAN_POINT('Ctrl Pts',(6.97186394570614,-0.76510606022219,
33.7389442078149));
#153342=CARTESIAN_POINT('Ctrl Pts',(6.98974332037367,-0.579536753288603,
33.747375273893));
#153343=CARTESIAN_POINT('Ctrl Pts',(7.00020323955213,-0.393422377939883,
33.755806339971));
#153344=CARTESIAN_POINT('Ctrl Pts',(7.00753460280148,-0.262974707329013,
33.7617156789384));
#153345=CARTESIAN_POINT('Ctrl Pts',(7.0112221257058,-0.132259529340179,
33.7676250179058));
#153346=CARTESIAN_POINT('Ctrl Pts',(7.01124984252467,-0.00148600059851424,
33.7735343568733));
#153347=CARTESIAN_POINT('Ctrl Pts',(7.01124984252485,-0.00148599977195217,
33.7735343569106));
#153348=CARTESIAN_POINT('Ctrl Pts',(7.0112719456076,0.102800850313519,33.778246827033));
#153349=CARTESIAN_POINT('Ctrl Pts',(7.008966713201,0.207099752356633,33.7829592971554));
#153350=CARTESIAN_POINT('Ctrl Pts',(7.00433593370125,0.31129518204029,33.7876717672778));
#153351=CARTESIAN_POINT('Ctrl Pts',(6.99614033435056,0.495701283843723,
33.7960119435002));
#153352=CARTESIAN_POINT('Ctrl Pts',(6.98066136702986,0.679707727527018,
33.8043521197226));
#153353=CARTESIAN_POINT('Ctrl Pts',(6.9579693378657,0.862722003788445,33.8126922959449));
#153354=CARTESIAN_POINT('Ctrl Pts',(6.9352661934101,1.04582592637477,33.821036557456));
#153355=CARTESIAN_POINT('Ctrl Pts',(6.90534298778614,1.22793638792556,33.829380818967));
#153356=CARTESIAN_POINT('Ctrl Pts',(6.86832139437408,1.40847001603985,33.8377250804781));
#153357=CARTESIAN_POINT('Ctrl Pts',(6.83125253035464,1.58923415649754,33.8460799962661));
#153358=CARTESIAN_POINT('Ctrl Pts',(6.78706723451658,1.76841711894936,33.8544349120541));
#153359=CARTESIAN_POINT('Ctrl Pts',(6.73593781222904,1.94544811092022,33.8627898278421));
#153360=CARTESIAN_POINT('Ctrl Pts',(6.68723243189414,2.11408607726602,33.8707486377194));
#153361=CARTESIAN_POINT('Ctrl Pts',(6.63222621110177,2.28077116823723,33.8787074475966));
#153362=CARTESIAN_POINT('Ctrl Pts',(6.57110895151815,2.44502632087633,33.8866662574739));
#153363=CARTESIAN_POINT('',(7.01124989960866,0.00118648116847724,33.2264656430502));
#153364=CARTESIAN_POINT('Ctrl Pts',(6.57110895151813,2.44502632087639,33.3398701610928));
#153365=CARTESIAN_POINT('Ctrl Pts',(6.62151232165559,2.30956518744441,33.3333026774452));
#153366=CARTESIAN_POINT('Ctrl Pts',(6.66772295152383,2.17255230094966,33.3267351937976));
#153367=CARTESIAN_POINT('Ctrl Pts',(6.70965433379238,2.03424808799741,33.32016771015));
#153368=CARTESIAN_POINT('Ctrl Pts',(6.76495279892197,1.8518546088549,33.3115066132381));
#153369=CARTESIAN_POINT('Ctrl Pts',(6.81281612487184,1.66718451890023,33.3028455163263));
#153370=CARTESIAN_POINT('Ctrl Pts',(6.85308001335555,1.48085140815909,33.2941844194144));
#153371=CARTESIAN_POINT('Ctrl Pts',(6.8933350640091,1.29455919710369,33.2855252235932));
#153372=CARTESIAN_POINT('Ctrl Pts',(6.92599394708551,1.10660497441285,33.276866027772));
#153373=CARTESIAN_POINT('Ctrl Pts',(6.95094321879609,0.917613715880841,
33.2682068319508));
#153374=CARTESIAN_POINT('Ctrl Pts',(6.97588795117122,0.728656842910447,
33.2595492116063));
#153375=CARTESIAN_POINT('Ctrl Pts',(6.99312583458587,0.53866359506697,33.2508915912618));
#153376=CARTESIAN_POINT('Ctrl Pts',(7.0025950358404,0.348266171948085,33.2422339709172));
#153377=CARTESIAN_POINT('Ctrl Pts',(7.00834386225785,0.232674401700854,
33.2369778616413));
#153378=CARTESIAN_POINT('Ctrl Pts',(7.01123031221648,0.116933788887199,
33.2317217523655));
#153379=CARTESIAN_POINT('Ctrl Pts',(7.01124989960851,0.00118648203690645,
33.2264656430896));
#153380=CARTESIAN_POINT('Ctrl Pts',(7.01124989960866,0.00118648116847724,
33.2264656430502));
#153381=CARTESIAN_POINT('Ctrl Pts',(7.01128401231658,-0.200395074715246,
33.2173117826749));
#153382=CARTESIAN_POINT('Ctrl Pts',(7.00262022694572,-0.401968332958667,
33.2081579222996));
#153383=CARTESIAN_POINT('Ctrl Pts',(6.98528696967019,-0.602820465690959,
33.1990040619243));
#153384=CARTESIAN_POINT('Ctrl Pts',(6.96796416524755,-0.803551474172744,
33.1898557218015));
#153385=CARTESIAN_POINT('Ctrl Pts',(6.94198235289239,-1.00356203552825,
33.1807073816787));
#153386=CARTESIAN_POINT('Ctrl Pts',(6.90742184977378,-1.20214389811195,
33.1715590415559));
#153387=CARTESIAN_POINT('Ctrl Pts',(6.8947551776495,-1.27492557419297,33.1682061093251));
#153388=CARTESIAN_POINT('Ctrl Pts',(6.88093665415477,-1.34751538291487,
33.1648531770944));
#153389=CARTESIAN_POINT('Ctrl Pts',(6.865971977599,-1.4198786445768,33.1615002448636));
#153390=CARTESIAN_POINT('Ctrl Pts',(6.83015214277981,-1.59308920947274,
33.1534745800109));
#153391=CARTESIAN_POINT('Ctrl Pts',(6.78775064118185,-1.76505436076465,
33.1454489151583));
#153392=CARTESIAN_POINT('Ctrl Pts',(6.73887974192064,-1.93523290237419,
33.1374232503056));
#153393=CARTESIAN_POINT('Ctrl Pts',(6.69002435308418,-2.10535743348863,
33.1294001326021));
#153394=CARTESIAN_POINT('Ctrl Pts',(6.63470375542867,-2.27369613190525,
33.1213770148986));
#153395=CARTESIAN_POINT('Ctrl Pts',(6.57308076831546,-2.43972042982418,
33.1133538971951));
#153396=CARTESIAN_POINT('Ctrl Pts',(6.51146555240038,-2.60572379062571,
33.105331791277));
#153397=CARTESIAN_POINT('Ctrl Pts',(6.4435496582257,-2.76941298893526,33.0973096853589));
#153398=CARTESIAN_POINT('Ctrl Pts',(6.36954496158249,-2.93027704234244,
33.0892875794408));
#153399=CARTESIAN_POINT('Ctrl Pts',(6.29551276454375,-3.09120087337585,
33.081262492481));
#153400=CARTESIAN_POINT('Ctrl Pts',(6.21538739565959,-3.24929712768591,
33.0732374055212));
#153401=CARTESIAN_POINT('Ctrl Pts',(6.12942804027358,-3.4040767414393,33.0652123185614));
#153402=CARTESIAN_POINT('Ctrl Pts',(6.04345175562286,-3.55888683826276,
33.0571856511009));
#153403=CARTESIAN_POINT('Ctrl Pts',(5.9516393811973,-3.71037867707376,33.0491589836404));
#153404=CARTESIAN_POINT('Ctrl Pts',(5.85429469625917,-3.85809022339445,
33.0411323161799));
#153405=CARTESIAN_POINT('Ctrl Pts',(5.75687186335079,-4.00592035202432,
33.033099204939));
#153406=CARTESIAN_POINT('Ctrl Pts',(5.65390805893699,-4.14996382599031,
33.0250660936982));
#153407=CARTESIAN_POINT('Ctrl Pts',(5.54574915310466,-4.28978937633761,
33.0170329824573));
#153408=CARTESIAN_POINT('Ctrl Pts',(5.48201799672505,-4.3721796700122,33.0122995814972));
#153409=CARTESIAN_POINT('Ctrl Pts',(5.41648386978901,-4.45310612794275,
33.0075661805371));
#153410=CARTESIAN_POINT('Ctrl Pts',(5.34922373629297,-4.53248629138356,
33.0028327795771));
#153411=CARTESIAN_POINT('Ctrl Pts',(5.21066576797738,-4.69601189859285,
32.9930818262833));
#153412=CARTESIAN_POINT('Ctrl Pts',(5.06469993487682,-4.85307034624515,
32.9833308729896));
#153413=CARTESIAN_POINT('Ctrl Pts',(4.91190287586367,-5.00308271974213,
32.9735799196959));
#153414=CARTESIAN_POINT('Ctrl Pts',(4.75888568402282,-5.15331121420491,
32.9638149183247));
#153415=CARTESIAN_POINT('Ctrl Pts',(4.59901760761635,-5.29647330207611,
32.9540499169535));
#153416=CARTESIAN_POINT('Ctrl Pts',(4.43291210201972,-5.43202695669555,
32.9442849155823));
#153417=CARTESIAN_POINT('Ctrl Pts',(4.26708345988466,-5.56735467145881,
32.9345361904451));
#153418=CARTESIAN_POINT('Ctrl Pts',(4.09503819631533,-5.69509927453355,
32.9247874653079));
#153419=CARTESIAN_POINT('Ctrl Pts',(3.91742033292767,-5.81476091491859,
32.9150387401707));
#153420=CARTESIAN_POINT('Ctrl Pts',(3.74028996170514,-5.9340941304986,32.9053167715041));
#153421=CARTESIAN_POINT('Ctrl Pts',(3.55761755700346,-6.04538864900124,
32.8955948028374));
#153422=CARTESIAN_POINT('Ctrl Pts',(3.37007493896457,-6.14818847045721,
32.8858728341707));
#153423=CARTESIAN_POINT('Ctrl Pts',(3.18377324144409,-6.25030809234538,
32.8762151932314));
#153424=CARTESIAN_POINT('Ctrl Pts',(2.99266559446705,-6.34404501225384,
32.8665575522921));
#153425=CARTESIAN_POINT('Ctrl Pts',(2.79744289488201,-6.42899213037115,
32.8568999113528));
#153426=CARTESIAN_POINT('Ctrl Pts',(2.71163579726229,-6.46632931335396,
32.8526550456654));
#153427=CARTESIAN_POINT('Ctrl Pts',(2.62503412982007,-6.50196891495713,
32.8484101799781));
#153428=CARTESIAN_POINT('Ctrl Pts',(2.53769853712739,-6.53587887717953,
32.8441653142908));
#153429=CARTESIAN_POINT('Ctrl Pts',(2.37615144395421,-6.59860308454728,
32.8363134672768));
#153430=CARTESIAN_POINT('Ctrl Pts',(2.21215820690979,-6.65538003626377,
32.8284616202628));
#153431=CARTESIAN_POINT('Ctrl Pts',(2.04621555630433,-6.70601434979364,
32.8206097732488));
#153432=CARTESIAN_POINT('Ctrl Pts',(1.88031996569292,-6.75663430384158,
32.8127601529552));
#153433=CARTESIAN_POINT('Ctrl Pts',(1.71247642570658,-6.80111497362436,
32.8049105326615));
#153434=CARTESIAN_POINT('Ctrl Pts',(1.54319868590164,-6.83931022679418,
32.7970609123679));
#153435=CARTESIAN_POINT('Ctrl Pts',(1.37393446075989,-6.87750243056139,
32.789211918766));
#153436=CARTESIAN_POINT('Ctrl Pts',(1.20323663601684,-6.90941013345148,
32.7813629251642));
#153437=CARTESIAN_POINT('Ctrl Pts',(1.03163080196475,-6.93493795581024,
32.7735139315624));
#153438=CARTESIAN_POINT('Ctrl Pts',(0.859938088903061,-6.96047870215808,
32.7656609642449));
#153439=CARTESIAN_POINT('Ctrl Pts',(0.687336825835717,-6.97963305817761,
32.7578079969274));
#153440=CARTESIAN_POINT('Ctrl Pts',(0.514359746082859,-6.99235730023213,
32.7499550296099));
#153441=CARTESIAN_POINT('Ctrl Pts',(0.34133873596433,-7.00508477381656,
32.7421000679026));
#153442=CARTESIAN_POINT('Ctrl Pts',(0.167942100270191,-7.01137886621337,
32.7342451061953));
#153443=CARTESIAN_POINT('Ctrl Pts',(-0.00529639141246658,-7.01124799951749,
32.726390144488));
#153444=CARTESIAN_POINT('Ctrl Pts',(-0.178706836779513,-7.01111700292548,
32.7185273860745));
#153445=CARTESIAN_POINT('Ctrl Pts',(-0.351958443599177,-7.00454832457666,
32.7106646276611));
#153446=CARTESIAN_POINT('Ctrl Pts',(-0.524520949053849,-6.99160241550559,
32.7028018692477));
#153447=CARTESIAN_POINT('Ctrl Pts',(-0.651110326921706,-6.98210548237448,
32.6970338624999));
#153448=CARTESIAN_POINT('Ctrl Pts',(-0.77732894927321,-6.96917774512589,
32.6912658557521));
#153449=CARTESIAN_POINT('Ctrl Pts',(-0.902971002042146,-6.9528605574951,
32.6854978490043));
#153450=CARTESIAN_POINT('Ctrl Pts',(-1.08546688179907,-6.92915973881047,
32.6771197825633));
#153451=CARTESIAN_POINT('Ctrl Pts',(-1.26715024107038,-6.89825376719693,
32.6687417161223));
#153452=CARTESIAN_POINT('Ctrl Pts',(-1.44743158371919,-6.86021635030209,
32.6603636496813));
#153453=CARTESIAN_POINT('Ctrl Pts',(-1.6275896521276,-6.82220494294106,
32.6519913120625));
#153454=CARTESIAN_POINT('Ctrl Pts',(-1.8063472946246,-6.77707188003955,
32.6436189744438));
#153455=CARTESIAN_POINT('Ctrl Pts',(-1.98312330321943,-6.72494226939742,
32.6352466368251));
#153456=CARTESIAN_POINT('Ctrl Pts',(-2.15980435879847,-6.6728406595218,
32.6268787963025));
#153457=CARTESIAN_POINT('Ctrl Pts',(-2.33450558821199,-6.61375008798809,
32.61851095578));
#153458=CARTESIAN_POINT('Ctrl Pts',(-2.50665864296621,-6.54784613519154,
32.6101431152574));
#153459=CARTESIAN_POINT('Ctrl Pts',(-2.67874444704001,-6.48196792742563,
32.6017785435875));
#153460=CARTESIAN_POINT('Ctrl Pts',(-2.8482837549517,-6.40928176337756,
32.5934139719175));
#153461=CARTESIAN_POINT('Ctrl Pts',(-3.01472554613214,-6.33001235733378,
32.5850494002476));
#153462=CARTESIAN_POINT('Ctrl Pts',(-3.18112668076744,-6.25076231433675,
32.576686871782));
#153463=CARTESIAN_POINT('Ctrl Pts',(-3.34443151126597,-6.16493237783986,
32.5683243433164));
#153464=CARTESIAN_POINT('Ctrl Pts',(-3.50411067349647,-6.07279465735407,
32.5599618148507));
#153465=CARTESIAN_POINT('Ctrl Pts',(-3.66380257862292,-5.98064958399037,
32.5515986190292));
#153466=CARTESIAN_POINT('Ctrl Pts',(-3.81986794972493,-5.88219587998511,
32.5432354232077));
#153467=CARTESIAN_POINT('Ctrl Pts',(-3.97180296577638,-5.77775109913451,
32.5348722273862));
#153468=CARTESIAN_POINT('Ctrl Pts',(-4.12374834349135,-5.67329919535922,
32.5265084612115));
#153469=CARTESIAN_POINT('Ctrl Pts',(-4.27156253338215,-5.56285558611907,
32.5181446950368));
#153470=CARTESIAN_POINT('Ctrl Pts',(-4.41477146026969,-5.44678065613884,
32.5097809288621));
#153471=CARTESIAN_POINT('Ctrl Pts',(-4.5580092468382,-5.33068233456201,
32.5014154772085));
#153472=CARTESIAN_POINT('Ctrl Pts',(-4.69663966441671,-5.2089506363984,
32.4930500255549));
#153473=CARTESIAN_POINT('Ctrl Pts',(-4.83022210865503,-5.08198592516352,
32.4846845739013));
#153474=CARTESIAN_POINT('Ctrl Pts',(-4.96384928939157,-4.95497869369621,
32.4763163206744));
#153475=CARTESIAN_POINT('Ctrl Pts',(-5.09242488755258,-4.82273518098884,
32.4679480674475));
#153476=CARTESIAN_POINT('Ctrl Pts',(-5.21554521692894,-4.6856925478172,
32.4595798142205));
#153477=CARTESIAN_POINT('Ctrl Pts',(-5.33877969641471,-4.54852285657442,
32.4512038024291));
#153478=CARTESIAN_POINT('Ctrl Pts',(-5.45654858014128,-4.40654539832958,
32.4428277906376));
#153479=CARTESIAN_POINT('Ctrl Pts',(-5.56848774957778,-4.26023130185465,
32.4344517788462));
#153480=CARTESIAN_POINT('Ctrl Pts',(-5.68048181536616,-4.11384545113887,
32.426071659355));
#153481=CARTESIAN_POINT('Ctrl Pts',(-5.78664027108274,-3.96311898599499,
32.4176915398639));
#153482=CARTESIAN_POINT('Ctrl Pts',(-5.88664204818,-3.80855247556066,32.4093114203727));
#153483=CARTESIAN_POINT('Ctrl Pts',(-5.98675808997502,-3.6538093533089,
32.4009217255335));
#153484=CARTESIAN_POINT('Ctrl Pts',(-6.08070322304552,-3.49521769779045,
32.3925320306944));
#153485=CARTESIAN_POINT('Ctrl Pts',(-6.16820143086998,-3.3333043171474,
32.3841423358552));
#153486=CARTESIAN_POINT('Ctrl Pts',(-6.22375253308335,-3.23050830587529,
32.3788158633806));
#153487=CARTESIAN_POINT('Ctrl Pts',(-6.27670596914686,-3.12637386532124,
32.3734893909061));
#153488=CARTESIAN_POINT('Ctrl Pts',(-6.32700113052968,-3.02104009519505,
32.3681629184315));
#153489=CARTESIAN_POINT('Ctrl Pts',(-6.40614147312532,-2.85529551012004,
32.3597816180266));
#153490=CARTESIAN_POINT('Ctrl Pts',(-6.47885731027182,-2.6862460912205,
32.3514003176217));
#153491=CARTESIAN_POINT('Ctrl Pts',(-6.54487131078258,-2.51441565533529,
32.3430190172168));
#153492=CARTESIAN_POINT('Ctrl Pts',(-6.61080164821146,-2.34280298937334,
32.3346483388832));
#153493=CARTESIAN_POINT('Ctrl Pts',(-6.67004695930937,-2.16841663382883,
32.3262776605496));
#153494=CARTESIAN_POINT('Ctrl Pts',(-6.72237646680245,-1.9918035046361,
32.317906982216));
#153495=CARTESIAN_POINT('Ctrl Pts',(-6.77464658928913,-1.81539080102177,
32.3095458031651));
#153496=CARTESIAN_POINT('Ctrl Pts',(-6.82001645808053,-1.63675667260096,
32.3011846241143));
#153497=CARTESIAN_POINT('Ctrl Pts',(-6.85830378523821,-1.45646687291105,
32.2928234450634));
#153498=CARTESIAN_POINT('Ctrl Pts',(-6.89654143007242,-1.27641102050369,
32.2844731156287));
#153499=CARTESIAN_POINT('Ctrl Pts',(-6.92771479682381,-1.0947041010865,
32.2761227861939));
#153500=CARTESIAN_POINT('Ctrl Pts',(-6.95169173340734,-0.91192576790882,
32.2677724567592));
#153501=CARTESIAN_POINT('Ctrl Pts',(-6.9756502211722,-0.729288071726782,
32.2594285524035));
#153502=CARTESIAN_POINT('Ctrl Pts',(-6.99242327101026,-0.545580928129063,
32.2510846480479));
#153503=CARTESIAN_POINT('Ctrl Pts',(-7.00192979954321,-0.361394029791344,
32.2427407436922));
#153504=CARTESIAN_POINT('Ctrl Pts',(-7.01142869237322,-0.177355071517599,
32.2344035412125));
#153505=CARTESIAN_POINT('Ctrl Pts',(-7.01367268715593,0.00716254671880051,
32.2260663387328));
#153506=CARTESIAN_POINT('Ctrl Pts',(-7.00863251950209,0.191564007782966,
32.2177291362531));
#153507=CARTESIAN_POINT('Ctrl Pts',(-7.00697332413152,0.252267950892913,
32.2149845752171));
#153508=CARTESIAN_POINT('Ctrl Pts',(-7.00452516987978,0.312959274457857,
32.212240014181));
#153509=CARTESIAN_POINT('Ctrl Pts',(-7.00128824767276,0.373616695958923,
32.209495453145));
#153510=CARTESIAN_POINT('Ctrl Pts',(-6.99145408423799,0.557901321422113,
32.2011571428431));
#153511=CARTESIAN_POINT('Ctrl Pts',(-6.97434365674282,0.741721695672878,
32.1928188325413));
#153512=CARTESIAN_POINT('Ctrl Pts',(-6.95003248498712,0.924486354752603,
32.1844805222394));
#153513=CARTESIAN_POINT('Ctrl Pts',(-6.92570601746714,1.10736600315381,
32.1761369657556));
#153514=CARTESIAN_POINT('Ctrl Pts',(-6.89416981231609,1.28918828672469,
32.1677934092719));
#153515=CARTESIAN_POINT('Ctrl Pts',(-6.85555068412416,1.46937108311846,
32.1594498527881));
#153516=CARTESIAN_POINT('Ctrl Pts',(-6.81690217466752,1.64969096179987,
32.1510999485629));
#153517=CARTESIAN_POINT('Ctrl Pts',(-6.77116006214715,1.82836854530606,
32.1427500443377));
#153518=CARTESIAN_POINT('Ctrl Pts',(-6.71850137597883,2.00483561008641,
32.1344001401125));
#153519=CARTESIAN_POINT('Ctrl Pts',(-6.66576370567854,2.1815673624036,32.1260377116489));
#153520=CARTESIAN_POINT('Ctrl Pts',(-6.60608882429062,2.35608165611188,
32.1176752831853));
#153521=CARTESIAN_POINT('Ctrl Pts',(-6.53970290914599,2.52782760935304,
32.1093128547217));
#153522=CARTESIAN_POINT('Ctrl Pts',(-6.47326022499415,2.69972042879672,
32.1009432752418));
#153523=CARTESIAN_POINT('Ctrl Pts',(-6.4000951863851,2.86883988437988,32.0925736957619));
#153524=CARTESIAN_POINT('Ctrl Pts',(-6.32048077044012,3.03465803559424,
32.084204116282));
#153525=CARTESIAN_POINT('Ctrl Pts',(-6.2407435589583,3.20073194110455,32.0758216277455));
#153526=CARTESIAN_POINT('Ctrl Pts',(-6.15453724537031,3.36349407820791,
32.067439139209));
#153527=CARTESIAN_POINT('Ctrl Pts',(-6.06217981162978,3.52244268852857,
32.0590566506724));
#153528=CARTESIAN_POINT('Ctrl Pts',(-6.03195894594133,3.5744532783568,32.0563137630678));
#153529=CARTESIAN_POINT('Ctrl Pts',(-6.00107981224043,3.62605579680324,
32.0535708754633));
#153530=CARTESIAN_POINT('Ctrl Pts',(-5.96955451152326,3.67723340249872,
32.0508279878587));
#153531=CARTESIAN_POINT('Ctrl Pts',(-5.87312595003434,3.83377379340367,
32.0424381327259));
#153532=CARTESIAN_POINT('Ctrl Pts',(-5.77045400655895,3.98665241824335,
32.034048277593));
#153533=CARTESIAN_POINT('Ctrl Pts',(-5.66184044539724,4.13535842864485,
32.0256584224602));
#153534=CARTESIAN_POINT('Ctrl Pts',(-5.55332711130731,4.28392721522439,
32.0172763093681));
#153535=CARTESIAN_POINT('Ctrl Pts',(-5.43888328252145,4.42833079901656,
32.008894196276));
#153536=CARTESIAN_POINT('Ctrl Pts',(-5.31885462928466,4.56808625083165,
32.0005120831839));
#153537=CARTESIAN_POINT('Ctrl Pts',(-5.19891909284367,4.70773328203619,
31.9921364728351));
#153538=CARTESIAN_POINT('Ctrl Pts',(-5.07340758332518,4.842739121977,31.9837608624862));
#153539=CARTESIAN_POINT('Ctrl Pts',(-4.94270702263677,4.97265259704287,
31.9753852521374));
#153540=CARTESIAN_POINT('Ctrl Pts',(-4.81208867454161,5.10248435460403,
31.9670149101718));
#153541=CARTESIAN_POINT('Ctrl Pts',(-4.67628801592536,5.22722990298551,
31.9586445682062));
#153542=CARTESIAN_POINT('Ctrl Pts',(-4.53573022854585,5.34647340368915,
31.9502742262406));
#153543=CARTESIAN_POINT('Ctrl Pts',(-4.39524024990846,5.46565937821839,
31.9419079223462));
#153544=CARTESIAN_POINT('Ctrl Pts',(-4.24999796925914,5.57934838595688,
31.9335416184519));
#153545=CARTESIAN_POINT('Ctrl Pts',(-4.1004635238077,5.68716321661534,31.9251753145575));
#153546=CARTESIAN_POINT('Ctrl Pts',(-3.95097089894964,5.79494789448741,
31.9168113504839));
#153547=CARTESIAN_POINT('Ctrl Pts',(-3.79718876837405,5.8968614778718,31.9084473864103));
#153548=CARTESIAN_POINT('Ctrl Pts',(-3.63960871914783,5.99256830866392,
31.9000834223367));
#153549=CARTESIAN_POINT('Ctrl Pts',(-3.48205291887242,6.08826041176529,
31.8917207453381));
#153550=CARTESIAN_POINT('Ctrl Pts',(-3.32070064602085,6.17774749602488,
31.8833580683396));
#153551=CARTESIAN_POINT('Ctrl Pts',(-3.1560710710089,6.26073813198099,31.874995391341));
#153552=CARTESIAN_POINT('Ctrl Pts',(-2.99144488541913,6.34372705931151,
31.8666328865147));
#153553=CARTESIAN_POINT('Ctrl Pts',(-2.82354182586127,6.42021965745607,
31.8582703816884));
#153554=CARTESIAN_POINT('Ctrl Pts',(-2.65290456117458,6.48997102857934,
31.8499078768621));
#153555=CARTESIAN_POINT('Ctrl Pts',(-2.48224806486497,6.55973026101045,
31.8415444295421));
#153556=CARTESIAN_POINT('Ctrl Pts',(-2.30885705345371,6.62274662780922,
31.8331809822221));
#153557=CARTESIAN_POINT('Ctrl Pts',(-2.13329341539225,6.67882368133372,
31.8248175349022));
#153558=CARTESIAN_POINT('Ctrl Pts',(-1.95762640052625,6.73493375460345,
31.8164491629493));
#153559=CARTESIAN_POINT('Ctrl Pts',(-1.77978451576621,6.78409624865335,
31.8080807909965));
#153560=CARTESIAN_POINT('Ctrl Pts',(-1.60034502804635,6.82616454194501,
31.7997124190437));
#153561=CARTESIAN_POINT('Ctrl Pts',(-1.4208517755662,6.86824543999682,31.7913415397079));
#153562=CARTESIAN_POINT('Ctrl Pts',(-1.23976028689496,6.90322782899965,
31.7829706603722));
#153563=CARTESIAN_POINT('Ctrl Pts',(-1.05765792791444,6.93101625088412,
31.7745997810364));
#153564=CARTESIAN_POINT('Ctrl Pts',(-0.875401275574798,6.95882821759789,
31.7662218091451));
#153565=CARTESIAN_POINT('Ctrl Pts',(-0.692132367449455,6.97943399325733,
31.7578438372538));
#153566=CARTESIAN_POINT('Ctrl Pts',(-0.508444758329448,6.99278989318479,
31.7494658653626));
#153567=CARTESIAN_POINT('Ctrl Pts',(-0.391709786961072,7.0012776763461,
31.7441415960036));
#153568=CARTESIAN_POINT('Ctrl Pts',(-0.274805793214833,7.00683849559473,
31.7388173266447));
#153569=CARTESIAN_POINT('Ctrl Pts',(-0.157885183101994,7.00947207936924,
31.7334930572857));
#153570=CARTESIAN_POINT('Ctrl Pts',(0.0147820803083811,7.01336133125448,
31.7256302260964));
#153571=CARTESIAN_POINT('Ctrl Pts',(0.187844607514974,7.0108718598126,31.7177673949071));
#153572=CARTESIAN_POINT('Ctrl Pts',(0.360771993997862,7.00196187727745,
31.7099045637178));
#153573=CARTESIAN_POINT('Ctrl Pts',(0.533566508610325,6.99305874088779,
31.7020477740764));
#153574=CARTESIAN_POINT('Ctrl Pts',(0.706225710690218,6.97774492350381,
31.694190984435));
#153575=CARTESIAN_POINT('Ctrl Pts',(0.878216694434533,6.95603062098755,
31.6863341947936));
#153576=CARTESIAN_POINT('Ctrl Pts',(1.05011068340587,6.93432856430999,31.6784818360096));
#153577=CARTESIAN_POINT('Ctrl Pts',(1.22133682657994,6.9062332503719,31.6706294772256));
#153578=CARTESIAN_POINT('Ctrl Pts',(1.39136510250798,6.87180687403415,31.6627771184416));
#153579=CARTESIAN_POINT('Ctrl Pts',(1.56135323277611,6.83738862616555,31.6549266136912));
#153580=CARTESIAN_POINT('Ctrl Pts',(1.73014368368552,6.79664235836334,31.6470761089407));
#153581=CARTESIAN_POINT('Ctrl Pts',(1.89721448512012,6.749681752494,31.6392256041903));
#153582=CARTESIAN_POINT('Ctrl Pts',(2.06425841012786,6.70272870110622,31.6313763623386));
#153583=CARTESIAN_POINT('Ctrl Pts',(2.22958286988284,6.64956340787834,31.623527120487));
#153584=CARTESIAN_POINT('Ctrl Pts',(2.39267942529673,6.59034989437296,31.6156778786353));
#153585=CARTESIAN_POINT('Ctrl Pts',(2.5558309311327,6.53111643067581,31.6078259922204));
#153586=CARTESIAN_POINT('Ctrl Pts',(2.716752674362,6.46583080670773,31.5999741058056));
#153587=CARTESIAN_POINT('Ctrl Pts',(2.87495444244162,6.39470589756755,31.5921222193907));
#153588=CARTESIAN_POINT('Ctrl Pts',(2.99112003164114,6.34247976206145,31.5863566769269));
#153589=CARTESIAN_POINT('Ctrl Pts',(3.10581943799112,6.28710623658754,31.5805911344631));
#153590=CARTESIAN_POINT('Ctrl Pts',(3.21886666312162,6.22868557301974,31.5748255919993));
#153591=CARTESIAN_POINT('Ctrl Pts',(3.40818195696215,6.1308510169134,31.5651702876393));
#153592=CARTESIAN_POINT('Ctrl Pts',(3.59276685959477,6.02452017000735,31.5555149832794));
#153593=CARTESIAN_POINT('Ctrl Pts',(3.77196215332,5.91015465757213,31.5458596789194));
#153594=CARTESIAN_POINT('Ctrl Pts',(3.95215015534536,5.79515558165942,31.5361508859852));
#153595=CARTESIAN_POINT('Ctrl Pts',(4.12688865788375,5.67203264406426,31.5264420930509));
#153596=CARTESIAN_POINT('Ctrl Pts',(4.29554450562247,5.54129262561694,31.5167333001167));
#153597=CARTESIAN_POINT('Ctrl Pts',(4.46501193962845,5.409923475094,31.506977787646));
#153598=CARTESIAN_POINT('Ctrl Pts',(4.62833801798703,5.27086380472715,31.4972222751754));
#153599=CARTESIAN_POINT('Ctrl Pts',(4.78491794612142,5.12466455598659,31.4874667627048));
#153600=CARTESIAN_POINT('Ctrl Pts',(4.94165291247532,4.97832054749623,31.4777015907758));
#153601=CARTESIAN_POINT('Ctrl Pts',(5.09162834723011,4.82482285479086,31.4679364188469));
#153602=CARTESIAN_POINT('Ctrl Pts',(5.2342754070601,4.66476017878153,31.458171246918));
#153603=CARTESIAN_POINT('Ctrl Pts',(5.37672797085845,4.5049157446016,31.4484193895796));
#153604=CARTESIAN_POINT('Ctrl Pts',(5.51187210507935,4.33852424571791,31.4386675322412));
#153605=CARTESIAN_POINT('Ctrl Pts',(5.63917919484042,4.16620745654594,31.4289156749028));
#153606=CARTESIAN_POINT('Ctrl Pts',(5.69469430600281,4.09106485667988,31.4246631588394));
#153607=CARTESIAN_POINT('Ctrl Pts',(5.74871962058488,4.01479596187637,31.4204106427761));
#153608=CARTESIAN_POINT('Ctrl Pts',(5.80121359253963,3.93745443354376,31.4161581267128));
#153609=CARTESIAN_POINT('Ctrl Pts',(5.90037610655681,3.79135422238041,31.4081250103752));
#153610=CARTESIAN_POINT('Ctrl Pts',(5.99411941724529,3.64135298941197,31.4000918940376));
#153611=CARTESIAN_POINT('Ctrl Pts',(6.08212076048457,3.48789816614285,31.3920587777));
#153612=CARTESIAN_POINT('Ctrl Pts',(6.17006761570061,3.33453835790041,31.3840306352482));
#153613=CARTESIAN_POINT('Ctrl Pts',(6.25227939740905,3.17772953174599,31.3760024927963));
#153614=CARTESIAN_POINT('Ctrl Pts',(6.32847653303838,3.01794819923778,31.3679743503445));
#153615=CARTESIAN_POINT('Ctrl Pts',(6.40463678429455,2.85824421129435,31.3599500940361));
#153616=CARTESIAN_POINT('Ctrl Pts',(6.47478803089947,2.69557091309334,31.3519258377278));
#153617=CARTESIAN_POINT('Ctrl Pts',(6.53869663140437,2.53042939537168,31.3439015814194));
#153618=CARTESIAN_POINT('Ctrl Pts',(6.54968554371298,2.50203375468457,31.3425218320865));
#153619=CARTESIAN_POINT('Ctrl Pts',(6.5604899992243,2.47356519257603,31.3411420827536));
#153620=CARTESIAN_POINT('Ctrl Pts',(6.57110895151815,2.44502632087633,31.3397623334207));
#153621=CARTESIAN_POINT('Origin',(0.,0.,50.));
#153622=CARTESIAN_POINT('',(6.57110895151813,2.4450263208764,29.3400595704968));
#153623=CARTESIAN_POINT('',(6.57110895151814,2.44502632087637,29.8870331279755));
#153624=CARTESIAN_POINT('',(6.57110895151814,2.44502632087636,50.));
#153625=CARTESIAN_POINT('',(7.0112494081677,-0.00288079295652949,31.7735343569381));
#153626=CARTESIAN_POINT('Ctrl Pts',(6.57110895151814,2.44502632087637,29.8870331279755));
#153627=CARTESIAN_POINT('Ctrl Pts',(6.51063509439985,2.6075523028872,29.894884053626));
#153628=CARTESIAN_POINT('Ctrl Pts',(6.44409497257938,2.76792041289768,29.9027349792766));
#153629=CARTESIAN_POINT('Ctrl Pts',(6.37167987579692,2.92563191855445,29.9105859049271));
#153630=CARTESIAN_POINT('Ctrl Pts',(6.29927905469288,3.08331233347408,29.9184352828715));
#153631=CARTESIAN_POINT('Ctrl Pts',(6.22100572524205,3.23833684075603,29.9262846608159));
#153632=CARTESIAN_POINT('Ctrl Pts',(6.13709891967929,3.39022763432948,29.9341340387603));
#153633=CARTESIAN_POINT('Ctrl Pts',(6.05316317315262,3.54217081776507,29.941986124096));
#153634=CARTESIAN_POINT('Ctrl Pts',(5.96359025085054,3.69097779240164,29.9498382094318));
#153635=CARTESIAN_POINT('Ctrl Pts',(5.86866479683627,3.83619604098575,29.9576902947676));
#153636=CARTESIAN_POINT('Ctrl Pts',(5.78016253938773,3.97158799624028,29.9650110633129));
#153637=CARTESIAN_POINT('Ctrl Pts',(5.68700818700101,4.10386050920121,29.9723318318582));
#153638=CARTESIAN_POINT('Ctrl Pts',(5.58946555198157,4.23267071784605,29.9796526004035));
#153639=CARTESIAN_POINT('Ctrl Pts',(5.4608173337849,4.40255749427359,29.9893079047635));
#153640=CARTESIAN_POINT('Ctrl Pts',(5.32460260862027,4.56633595418709,29.9989632091234));
#153641=CARTESIAN_POINT('Ctrl Pts',(5.18138853132814,4.72343513239265,30.0086185134833));
#153642=CARTESIAN_POINT('Ctrl Pts',(5.037381074914,4.88140461057452,30.0183273064181));
#153643=CARTESIAN_POINT('Ctrl Pts',(4.88629657359023,5.0326206001273,30.0280360993529));
#153644=CARTESIAN_POINT('Ctrl Pts',(4.72874223923885,5.17654550809112,30.0377448922877));
#153645=CARTESIAN_POINT('Ctrl Pts',(4.5704297400526,5.32116299493275,30.0475004047585));
#153646=CARTESIAN_POINT('Ctrl Pts',(4.40558503937709,5.4584190492802,30.0572559172293));
#153647=CARTESIAN_POINT('Ctrl Pts',(4.23485403431082,5.58781154572892,30.0670114297));
#153648=CARTESIAN_POINT('Ctrl Pts',(4.06395397928303,5.71733216065581,30.076776601629));
#153649=CARTESIAN_POINT('Ctrl Pts',(3.88715599914691,5.83897362939123,30.086541773558));
#153650=CARTESIAN_POINT('Ctrl Pts',(3.70513707577017,5.9522756834889,30.096306945487));
#153651=CARTESIAN_POINT('Ctrl Pts',(3.52336633106581,6.06542325280641,30.1060588028256));
#153652=CARTESIAN_POINT('Ctrl Pts',(3.33638890295605,6.1702541132167,30.1158106601642));
#153653=CARTESIAN_POINT('Ctrl Pts',(3.14490751213805,6.26635326985302,30.1255625175028));
#153654=CARTESIAN_POINT('Ctrl Pts',(3.06140775800607,6.30825946197511,30.1298150335652));
#153655=CARTESIAN_POINT('Ctrl Pts',(2.97705189745367,6.34850579990758,30.1340675496276));
#153656=CARTESIAN_POINT('Ctrl Pts',(2.89189988376014,6.38706048388522,30.13832006569));
#153657=CARTESIAN_POINT('Ctrl Pts',(2.73104687373191,6.45989066956716,30.1463531112888));
#153658=CARTESIAN_POINT('Ctrl Pts',(2.56727285395661,6.52671653460236,30.1543861568876));
#153659=CARTESIAN_POINT('Ctrl Pts',(2.4010736769296,6.58729624052659,30.1624192024864));
#153660=CARTESIAN_POINT('Ctrl Pts',(2.23498133913274,6.64783700348336,30.1704470841342));
#153661=CARTESIAN_POINT('Ctrl Pts',(2.06646729024776,6.70213947481297,30.178474965782));
#153662=CARTESIAN_POINT('Ctrl Pts',(1.8960486441547,6.75000934084532,30.1865028474298));
#153663=CARTESIAN_POINT('Ctrl Pts',(1.72570694376052,6.79785759316122,30.1945271044099));
#153664=CARTESIAN_POINT('Ctrl Pts',(1.5534627105848,6.83927892421778,30.20255136139));
#153665=CARTESIAN_POINT('Ctrl Pts',(1.37984950628901,6.87412844675556,30.21057561837));
#153666=CARTESIAN_POINT('Ctrl Pts',(1.20625729359781,6.90897375563113,30.2185989051357));
#153667=CARTESIAN_POINT('Ctrl Pts',(1.03129679715255,6.93724875903307,30.2266221919014));
#153668=CARTESIAN_POINT('Ctrl Pts',(0.855513271446454,6.95885936090671,
30.2346454786671));
#153669=CARTESIAN_POINT('Ctrl Pts',(0.679744149632396,6.98046819198429,
30.242668107996));
#153670=CARTESIAN_POINT('Ctrl Pts',(0.503152497286794,6.99541366853891,
30.2506907373249));
#153671=CARTESIAN_POINT('Ctrl Pts',(0.326289914370252,7.00365343619173,
30.2587133666538));
#153672=CARTESIAN_POINT('Ctrl Pts',(0.1493608437137,7.01189630141059,30.2667390119202));
#153673=CARTESIAN_POINT('Ctrl Pts',(-0.0278389944188127,7.01342840779966,
30.2747646571866));
#153674=CARTESIAN_POINT('Ctrl Pts',(-0.204756378974013,7.00825951201648,
30.282790302453));
#153675=CARTESIAN_POINT('Ctrl Pts',(-0.309077649721913,7.00521161608573,
30.2875227119608));
#153676=CARTESIAN_POINT('Ctrl Pts',(-0.413300719792258,6.99983476989188,
30.2922551214686));
#153677=CARTESIAN_POINT('Ctrl Pts',(-0.517312787694124,6.99213944670643,
30.2969875309764));
#153678=CARTESIAN_POINT('Ctrl Pts',(-0.709187652006507,6.97794360268724,
30.305717579811));
#153679=CARTESIAN_POINT('Ctrl Pts',(-0.900440130699299,6.95584821871191,
30.3144476286457));
#153680=CARTESIAN_POINT('Ctrl Pts',(-1.09042849719771,6.92593620061571,
30.3231776774803));
#153681=CARTESIAN_POINT('Ctrl Pts',(-1.28047179906911,6.8960155334222,30.3319102506195));
#153682=CARTESIAN_POINT('Ctrl Pts',(-1.46924998854034,6.85827376325242,
30.3406428237586));
#153683=CARTESIAN_POINT('Ctrl Pts',(-1.65613021921757,6.81284516626456,
30.3493753968978));
#153684=CARTESIAN_POINT('Ctrl Pts',(-1.84566538188862,6.76677118353879,
30.3582320301782));
#153685=CARTESIAN_POINT('Ctrl Pts',(-2.03324796605332,6.7127903705848,30.3670886634586));
#153686=CARTESIAN_POINT('Ctrl Pts',(-2.21823189569185,6.65109568563221,
30.3759452967391));
#153687=CARTESIAN_POINT('Ctrl Pts',(-2.40074075245821,6.59022647152664,
30.3846834288458));
#153688=CARTESIAN_POINT('Ctrl Pts',(-2.5807198063312,6.52184863553396,30.3934215609525));
#153689=CARTESIAN_POINT('Ctrl Pts',(-2.75756609906262,6.44619700069743,
30.4021596930593));
#153690=CARTESIAN_POINT('Ctrl Pts',(-2.9380098127859,6.36900645444226,30.4110755769265));
#153691=CARTESIAN_POINT('Ctrl Pts',(-3.11519167258611,6.28424312418134,
30.4199914607938));
#153692=CARTESIAN_POINT('Ctrl Pts',(-3.28849396900906,6.19220752060935,
30.428907344661));
#153693=CARTESIAN_POINT('Ctrl Pts',(-3.46179626543201,6.10017191703736,
30.4378232285283));
#153694=CARTESIAN_POINT('Ctrl Pts',(-3.6312187342459,6.00086418736742,30.4467391123955));
#153695=CARTESIAN_POINT('Ctrl Pts',(-3.79617071624401,5.89463437845227,
30.4556549962628));
#153696=CARTESIAN_POINT('Ctrl Pts',(-3.95788135011287,5.79049201212634,
30.464395680759));
#153697=CARTESIAN_POINT('Ctrl Pts',(-4.11531273400632,5.6796860216251,30.4731363652552));
#153698=CARTESIAN_POINT('Ctrl Pts',(-4.2679340745091,5.56258620590676,30.4818770497515));
#153699=CARTESIAN_POINT('Ctrl Pts',(-4.4205279558975,5.44550745839044,30.4906161616534));
#153700=CARTESIAN_POINT('Ctrl Pts',(-4.56831330503308,5.32213731368012,
30.4993552735553));
#153701=CARTESIAN_POINT('Ctrl Pts',(-4.71079085000666,5.19288707079151,
30.5080943854572));
#153702=CARTESIAN_POINT('Ctrl Pts',(-4.85511439663588,5.06196220498313,
30.5169467251315));
#153703=CARTESIAN_POINT('Ctrl Pts',(-4.99399141362478,4.92500398340368,
30.5257990648058));
#153704=CARTESIAN_POINT('Ctrl Pts',(-5.12693901451052,4.78248083153397,
30.5346514044802));
#153705=CARTESIAN_POINT('Ctrl Pts',(-5.25811884923516,4.64185276918352,
30.5433860371299));
#153706=CARTESIAN_POINT('Ctrl Pts',(-5.38352579062743,4.49580706298467,
30.5521206697797));
#153707=CARTESIAN_POINT('Ctrl Pts',(-5.50273361492177,4.34483018375978,
30.5608553024295));
#153708=CARTESIAN_POINT('Ctrl Pts',(-5.6243510880585,4.19080148084457,30.5697664956161));
#153709=CARTESIAN_POINT('Ctrl Pts',(-5.73951596194569,4.03164034017232,
30.5786776888027));
#153710=CARTESIAN_POINT('Ctrl Pts',(-5.84781877346367,3.86789893291253,
30.5875888819893));
#153711=CARTESIAN_POINT('Ctrl Pts',(-5.95612158498165,3.70415752565273,
30.596500075176));
#153712=CARTESIAN_POINT('Ctrl Pts',(-6.05756215566455,3.53583609720128,
30.6054112683626));
#153713=CARTESIAN_POINT('Ctrl Pts',(-6.15177738397854,3.3635192255241,30.6143224615492));
#153714=CARTESIAN_POINT('Ctrl Pts',(-6.23663020117184,3.20832592744051,
30.6223481264016));
#153715=CARTESIAN_POINT('Ctrl Pts',(-6.315660867571,3.04982023554652,30.630373791254));
#153716=CARTESIAN_POINT('Ctrl Pts',(-6.38860452752384,2.88848727769431,
30.6383994561063));
#153717=CARTESIAN_POINT('Ctrl Pts',(-6.4615250369482,2.72720552296571,30.6464225738096));
#153718=CARTESIAN_POINT('Ctrl Pts',(-6.52836223525133,2.56309862234801,
30.6544456915128));
#153719=CARTESIAN_POINT('Ctrl Pts',(-6.5888979667776,2.39667481020977,30.662468809216));
#153720=CARTESIAN_POINT('Ctrl Pts',(-6.6494260642183,2.23027198557082,30.6704909151338));
#153721=CARTESIAN_POINT('Ctrl Pts',(-6.70365415305941,2.06155317599891,
30.6785130210517));
#153722=CARTESIAN_POINT('Ctrl Pts',(-6.75141284886433,1.89104497743699,
30.6865351269695));
#153723=CARTESIAN_POINT('Ctrl Pts',(-6.79918929196198,1.72047341745238,
30.6945602139291));
#153724=CARTESIAN_POINT('Ctrl Pts',(-6.84049143764329,1.54811149263829,
30.7025853008886));
#153725=CARTESIAN_POINT('Ctrl Pts',(-6.87520014708154,1.37449972719894,
30.7106103878481));
#153726=CARTESIAN_POINT('Ctrl Pts',(-6.90991569222643,1.2008537697912,30.7186370553083));
#153727=CARTESIAN_POINT('Ctrl Pts',(-6.93803515099065,1.02595784256382,
30.7266637227685));
#153728=CARTESIAN_POINT('Ctrl Pts',(-6.95949086975134,0.850360744829992,
30.7346903902288));
#153729=CARTESIAN_POINT('Ctrl Pts',(-6.98096381308744,0.674622678364829,
30.7427235014694));
#153730=CARTESIAN_POINT('Ctrl Pts',(-6.99576229664982,0.498182682066907,
30.7507566127099));
#153731=CARTESIAN_POINT('Ctrl Pts',(-7.00387066355227,0.321593362387762,
30.7587897239505));
#153732=CARTESIAN_POINT('Ctrl Pts',(-7.00864840788377,0.217540520274141,
30.7635231249122));
#153733=CARTESIAN_POINT('Ctrl Pts',(-7.01110433567621,0.113435852690615,
30.768256525874));
#153734=CARTESIAN_POINT('Ctrl Pts',(-7.01124370937302,0.00939203265171227,
30.7729899268357));
#153735=CARTESIAN_POINT('Ctrl Pts',(-7.01153082352604,-0.204941474683194,
30.7827408801298));
#153736=CARTESIAN_POINT('Ctrl Pts',(-7.00198517742529,-0.419142924389543,
30.792491833424));
#153737=CARTESIAN_POINT('Ctrl Pts',(-6.98267138124105,-0.632397773633994,
30.8022427867182));
#153738=CARTESIAN_POINT('Ctrl Pts',(-6.96332975991021,-0.84595985649458,
30.8120077880898));
#153739=CARTESIAN_POINT('Ctrl Pts',(-6.93419184213379,-1.05857257250479,
30.8217727894614));
#153740=CARTESIAN_POINT('Ctrl Pts',(-6.89537417949784,-1.26942565249582,
30.8315377908331));
#153741=CARTESIAN_POINT('Ctrl Pts',(-6.85662121786268,-1.47992728409023,
30.8412865159707));
#153742=CARTESIAN_POINT('Ctrl Pts',(-6.80822076380325,-1.68867510415602,
30.8510352411083));
#153743=CARTESIAN_POINT('Ctrl Pts',(-6.75033997080507,-1.89487119378904,
30.8607839662459));
#153744=CARTESIAN_POINT('Ctrl Pts',(-6.69261803814045,-2.10050135510829,
30.870505934913));
#153745=CARTESIAN_POINT('Ctrl Pts',(-6.62546772171576,-2.30359372891132,
30.8802279035802));
#153746=CARTESIAN_POINT('Ctrl Pts',(-6.54910575246193,-2.50336581537138,
30.8899498722473));
#153747=CARTESIAN_POINT('Ctrl Pts',(-6.47324905041402,-2.70181606211292,
30.8996075131871));
#153748=CARTESIAN_POINT('Ctrl Pts',(-6.38830218450866,-2.89698976132389,
30.9092651541268));
#153749=CARTESIAN_POINT('Ctrl Pts',(-6.29452808559151,-3.08812932731123,
30.9189227950665));
#153750=CARTESIAN_POINT('Ctrl Pts',(-6.25331114067329,-3.17214174709414,
30.9231676607517));
#153751=CARTESIAN_POINT('Ctrl Pts',(-6.21038951751227,-3.25537493916658,
30.9274125264369));
#153752=CARTESIAN_POINT('Ctrl Pts',(-6.16578867531316,-3.33776520652366,
30.9316573921221));
#153753=CARTESIAN_POINT('Ctrl Pts',(-6.08328924762561,-3.49016479291804,
30.939509239136));
#153754=CARTESIAN_POINT('Ctrl Pts',(-5.99507492550315,-3.63961591340342,
30.9473610861499));
#153755=CARTESIAN_POINT('Ctrl Pts',(-5.90139775178298,-3.78564804726361,
30.9552129331638));
#153756=CARTESIAN_POINT('Ctrl Pts',(-5.8077471441519,-3.93163876759131,
30.9630625534573));
#153757=CARTESIAN_POINT('Ctrl Pts',(-5.70863697235183,-4.07421210922496,
30.9709121737509));
#153758=CARTESIAN_POINT('Ctrl Pts',(-5.6043641378185,-4.21292406449889,
30.9787617940445));
#153759=CARTESIAN_POINT('Ctrl Pts',(-5.50009962813733,-4.35162494539737,
30.9866107876462));
#153760=CARTESIAN_POINT('Ctrl Pts',(-5.39067350605877,-4.48646474917287,
30.994459781248));
#153761=CARTESIAN_POINT('Ctrl Pts',(-5.27642455801112,-4.61703047922765,
31.0023087748498));
#153762=CARTESIAN_POINT('Ctrl Pts',(-5.16211776906659,-4.74766231088826,
31.0101617421672));
#153763=CARTESIAN_POINT('Ctrl Pts',(-5.04298352713106,-4.87401545791966,
31.0180147094846));
#153764=CARTESIAN_POINT('Ctrl Pts',(-4.91939950847132,-4.99571166487339,
31.0258676768021));
#153765=CARTESIAN_POINT('Ctrl Pts',(-4.79578410362338,-5.11743877857459,
31.0337226385093));
#153766=CARTESIAN_POINT('Ctrl Pts',(-4.66771695222961,-5.23450633856665,
31.0415776002165));
#153767=CARTESIAN_POINT('Ctrl Pts',(-4.5356102836231,-5.3465751577615,31.0494325619238));
#153768=CARTESIAN_POINT('Ctrl Pts',(-4.40337248810524,-5.45875521462721,
31.0572953203371));
#153769=CARTESIAN_POINT('Ctrl Pts',(-4.26708746699066,-5.56592638528403,
31.0651580787504));
#153770=CARTESIAN_POINT('Ctrl Pts',(-4.12719846489199,-5.66779140352688,
31.0730208371638));
#153771=CARTESIAN_POINT('Ctrl Pts',(-4.02457790023861,-5.74251811923491,
31.078788843912));
#153772=CARTESIAN_POINT('Ctrl Pts',(-3.92001850282062,-5.81439022392568,
31.0845568506602));
#153773=CARTESIAN_POINT('Ctrl Pts',(-3.81370389557021,-5.88330597193556,
31.0903248574085));
#153774=CARTESIAN_POINT('Ctrl Pts',(-3.65928125321288,-5.98340653368293,
31.0987029238495));
#153775=CARTESIAN_POINT('Ctrl Pts',(-3.50081262185188,-6.07749008693342,
31.1070809902906));
#153776=CARTESIAN_POINT('Ctrl Pts',(-3.33879497014469,-6.16523111568711,
31.1154590567316));
#153777=CARTESIAN_POINT('Ctrl Pts',(-3.17688810418275,-6.25291214816782,
31.1238313943504));
#153778=CARTESIAN_POINT('Ctrl Pts',(-3.01143734428889,-6.33425914669135,
31.1322037319691));
#153779=CARTESIAN_POINT('Ctrl Pts',(-2.84296662347145,-6.40899113280143,
31.1405760695879));
#153780=CARTESIAN_POINT('Ctrl Pts',(-2.67458639458861,-6.48368297756252,
31.1489439101105));
#153781=CARTESIAN_POINT('Ctrl Pts',(-2.50318973897938,-6.55176676160134,
31.1573117506331));
#153782=CARTESIAN_POINT('Ctrl Pts',(-2.32932346968383,-6.61300829699163,
31.1656795911557));
#153783=CARTESIAN_POINT('Ctrl Pts',(-2.15552512032786,-6.67422590869965,
31.1740441628256));
#153784=CARTESIAN_POINT('Ctrl Pts',(-1.97925939070246,-6.72860649283356,
31.1824087344955));
#153785=CARTESIAN_POINT('Ctrl Pts',(-1.80109170178626,-6.77596452501463,
31.1907733061655));
#153786=CARTESIAN_POINT('Ctrl Pts',(-1.6229675336869,-6.82331098910354,
31.1991358346311));
#153787=CARTESIAN_POINT('Ctrl Pts',(-1.44294265028617,-6.86363823819933,
31.2074983630967));
#153788=CARTESIAN_POINT('Ctrl Pts',(-1.26159665606641,-6.8968108890923,
31.2158608915623));
#153789=CARTESIAN_POINT('Ctrl Pts',(-1.08023618986904,-6.92998618726657,
31.2242240873838));
#153790=CARTESIAN_POINT('Ctrl Pts',(-0.897554724438878,-6.9560056814588,
31.2325872832053));
#153791=CARTESIAN_POINT('Ctrl Pts',(-0.714141822607698,-6.97478515939398,
31.2409504790269));
#153792=CARTESIAN_POINT('Ctrl Pts',(-0.530716412384352,-6.99356591805191,
31.2493142452016));
#153793=CARTESIAN_POINT('Ctrl Pts',(-0.346559793382873,-7.00510564218847,
31.2576780113763));
#153794=CARTESIAN_POINT('Ctrl Pts',(-0.162266591852918,-7.00937202006488,
31.266041777551));
#153795=CARTESIAN_POINT('Ctrl Pts',(0.0220637487227761,-7.01363925770824,
31.2744072292046));
#153796=CARTESIAN_POINT('Ctrl Pts',(0.20653039801308,-7.01063021878234,
31.2827726808582));
#153797=CARTESIAN_POINT('Ctrl Pts',(0.390538351795674,-7.00036473037489,
31.2911381325117));
#153798=CARTESIAN_POINT('Ctrl Pts',(0.574607929480229,-6.99009580407556,
31.2995063857386));
#153799=CARTESIAN_POINT('Ctrl Pts',(0.758218177199506,-6.97256560077253,
31.3078746389655));
#153800=CARTESIAN_POINT('Ctrl Pts',(0.940778399872127,-6.94784589386049,
31.3162428921924));
#153801=CARTESIAN_POINT('Ctrl Pts',(1.12350788191618,-6.9231032682535,31.3246189039839));
#153802=CARTESIAN_POINT('Ctrl Pts',(1.30518506737711,-6.8911578631517,31.3329949157754));
#153803=CARTESIAN_POINT('Ctrl Pts',(1.48522742137247,-6.85213295764927,
31.3413709275669));
#153804=CARTESIAN_POINT('Ctrl Pts',(1.66535807036304,-6.81308891385094,
31.349751047058));
#153805=CARTESIAN_POINT('Ctrl Pts',(1.84385196932977,-6.76695852205919,
31.3581311665492));
#153806=CARTESIAN_POINT('Ctrl Pts',(2.02014032894375,-6.71391537136678,
31.3665112860404));
#153807=CARTESIAN_POINT('Ctrl Pts',(2.19663012033953,-6.66081161215557,
31.3749009808796));
#153808=CARTESIAN_POINT('Ctrl Pts',(2.37090902367499,-6.60077941179378,
31.3832906757188));
#153809=CARTESIAN_POINT('Ctrl Pts',(2.5424255937145,-6.53404152595662,31.3916803705581));
#153810=CARTESIAN_POINT('Ctrl Pts',(2.65131850421169,-6.49167079391852,
31.3970068430325));
#153811=CARTESIAN_POINT('Ctrl Pts',(2.75909838701318,-6.44659813077163,
31.402333315507));
#153812=CARTESIAN_POINT('Ctrl Pts',(2.86562898909525,-6.39889029905631,
31.4076597879814));
#153813=CARTESIAN_POINT('Ctrl Pts',(3.033256810818,-6.32382116630708,31.4160410883863));
#153814=CARTESIAN_POINT('Ctrl Pts',(3.19812844818045,-6.24207373702027,
31.4244223887911));
#153815=CARTESIAN_POINT('Ctrl Pts',(3.35969339087501,-6.15386763603271,
31.4328036891959));
#153816=CARTESIAN_POINT('Ctrl Pts',(3.52105357365609,-6.06577332336571,
31.4411743675294));
#153817=CARTESIAN_POINT('Ctrl Pts',(3.67911512824899,-5.97123680742495,
31.4495450458629));
#153818=CARTESIAN_POINT('Ctrl Pts',(3.83334806603012,-5.87052545920407,
31.4579157241964));
#153819=CARTESIAN_POINT('Ctrl Pts',(3.98740597590764,-5.76992840107195,
31.4662769032472));
#153820=CARTESIAN_POINT('Ctrl Pts',(4.13764365600859,-5.66317065517934,
31.474638082298));
#153821=CARTESIAN_POINT('Ctrl Pts',(4.28355587357753,-5.55056534421851,
31.4829992613488));
#153822=CARTESIAN_POINT('Ctrl Pts',(4.42927875283216,-5.43810615193172,
31.4913495907835));
#153823=CARTESIAN_POINT('Ctrl Pts',(4.57068710670983,-5.31981472869339,
31.4996999202181));
#153824=CARTESIAN_POINT('Ctrl Pts',(4.70730491029333,-5.19604725190488,
31.5080502496528));
#153825=CARTESIAN_POINT('Ctrl Pts',(4.84381759464959,-5.07237500678587,
31.5163941540085));
#153826=CARTESIAN_POINT('Ctrl Pts',(4.97554683253056,-4.94323532389461,
31.5247380583642));
#153827=CARTESIAN_POINT('Ctrl Pts',(5.10204901722773,-4.80902509749175,
31.5330819627199));
#153828=CARTESIAN_POINT('Ctrl Pts',(5.22844959458117,-4.6749226695798,31.5414191651996));
#153829=CARTESIAN_POINT('Ctrl Pts',(5.34963126777935,-4.53575805829959,
31.5497563676793));
#153830=CARTESIAN_POINT('Ctrl Pts',(5.46518660244469,-4.39196561495637,
31.558093570159));
#153831=CARTESIAN_POINT('Ctrl Pts',(5.50322678076923,-4.34462993631947,
31.5608381311952));
#153832=CARTESIAN_POINT('Ctrl Pts',(5.5406575368276,-4.29679303929625,31.5635826922315));
#153833=CARTESIAN_POINT('Ctrl Pts',(5.57746523610436,-4.24847126653192,
31.5663272532677));
#153834=CARTESIAN_POINT('Ctrl Pts',(5.68929150413603,-4.10166384256667,
31.5746655635697));
#153835=CARTESIAN_POINT('Ctrl Pts',(5.79527206873142,-3.9504989767829,31.5830038738716));
#153836=CARTESIAN_POINT('Ctrl Pts',(5.89508152077292,-3.79547631081286,
31.5913421841736));
#153837=CARTESIAN_POINT('Ctrl Pts',(5.9949537695349,-3.64035610984164,31.5996857406574));
#153838=CARTESIAN_POINT('Ctrl Pts',(6.08864698393497,-3.48137354282746,
31.6080292971413));
#153839=CARTESIAN_POINT('Ctrl Pts',(6.17588089420329,-3.31905434470645,
31.6163728536251));
#153840=CARTESIAN_POINT('Ctrl Pts',(6.26318117165118,-3.15661165484542,
31.6247227578504));
#153841=CARTESIAN_POINT('Ctrl Pts',(6.34401218779013,-2.99082755869547,
31.6330726620758));
#153842=CARTESIAN_POINT('Ctrl Pts',(6.41814093986457,-2.82224971229236,
31.6414225663011));
#153843=CARTESIAN_POINT('Ctrl Pts',(6.49238087958084,-2.65341901159613,
31.6497849947648));
#153844=CARTESIAN_POINT('Ctrl Pts',(6.5598983343723,-2.48178648706626,31.6581474232285));
#153845=CARTESIAN_POINT('Ctrl Pts',(6.62050898463268,-2.30791840126508,
31.6665098516922));
#153846=CARTESIAN_POINT('Ctrl Pts',(6.68117146526149,-2.13390163454882,
31.6748794311722));
#153847=CARTESIAN_POINT('Ctrl Pts',(6.73491526150781,-1.95764580486575,
31.6832490106522));
#153848=CARTESIAN_POINT('Ctrl Pts',(6.78160657312031,-1.77972999354158,
31.6916185901322));
#153849=CARTESIAN_POINT('Ctrl Pts',(6.82836990039218,-1.60153976875538,
31.7000010786688));
#153850=CARTESIAN_POINT('Ctrl Pts',(6.86805893587711,-1.42168476537843,
31.7083835672054));
#153851=CARTESIAN_POINT('Ctrl Pts',(6.9005911291171,-1.24075325155743,31.716766055742));
#153852=CARTESIAN_POINT('Ctrl Pts',(6.91123619581566,-1.18154949550305,
31.7195089433461));
#153853=CARTESIAN_POINT('Ctrl Pts',(6.92111539004135,-1.12223050757922,
31.7222518309502));
#153854=CARTESIAN_POINT('Ctrl Pts',(6.93022702928683,-1.0628169574495,31.7249947185543));
#153855=CARTESIAN_POINT('Ctrl Pts',(6.97711648276298,-0.757068582255461,
31.7391099065285));
#153856=CARTESIAN_POINT('Ctrl Pts',(7.00374762286509,-0.448352345442656,
31.7532250945026));
#153857=CARTESIAN_POINT('Ctrl Pts',(7.00987641222234,-0.138777692259644,
31.7673402824768));
#153858=CARTESIAN_POINT('Ctrl Pts',(7.010772897567,-0.0934948274911753,
31.7694049739547));
#153859=CARTESIAN_POINT('Ctrl Pts',(7.01123078995131,-0.048193640247624,
31.7714696654327));
#153860=CARTESIAN_POINT('Ctrl Pts',(7.01124940816745,-0.00288079356036475,
31.7735343569106));
#153861=CARTESIAN_POINT('Ctrl Pts',(7.0112494081677,-0.00288079295658086,
31.7735343569381));
#153862=CARTESIAN_POINT('Ctrl Pts',(7.01132401614023,0.178699456341272,
31.7818081075562));
#153863=CARTESIAN_POINT('Ctrl Pts',(7.00434040300367,0.360449743185088,
31.7900818581744));
#153864=CARTESIAN_POINT('Ctrl Pts',(6.99028539102326,0.541790286500964,
31.7983556087925));
#153865=CARTESIAN_POINT('Ctrl Pts',(6.97624480014575,0.722944765896102,
31.8066208701536));
#153866=CARTESIAN_POINT('Ctrl Pts',(6.95514730409161,0.903690000783933,
31.8148861315147));
#153867=CARTESIAN_POINT('Ctrl Pts',(6.92703176507304,1.08344703985431,31.8231513928758));
#153868=CARTESIAN_POINT('Ctrl Pts',(6.89893310426121,1.26309616790559,31.8314116924687));
#153869=CARTESIAN_POINT('Ctrl Pts',(6.86382484659498,1.44175794545868,31.8396719920615));
#153870=CARTESIAN_POINT('Ctrl Pts',(6.82179765978736,1.61885862613749,31.8479322916543));
#153871=CARTESIAN_POINT('Ctrl Pts',(6.77979130111409,1.79587153799204,31.8561884975487));
#153872=CARTESIAN_POINT('Ctrl Pts',(6.73087292716555,1.97132456327243,31.864444703443));
#153873=CARTESIAN_POINT('Ctrl Pts',(6.67518430983552,2.14465404954405,31.8727009093374));
#153874=CARTESIAN_POINT('Ctrl Pts',(6.64277296198895,2.24553359263494,31.8775061060538));
#153875=CARTESIAN_POINT('Ctrl Pts',(6.60806924282777,2.345694015534,31.8823113027702));
#153876=CARTESIAN_POINT('Ctrl Pts',(6.57110895151814,2.44502632087638,31.8871164994866));
#153877=CARTESIAN_POINT('',(7.01124987764386,-0.00130986217405227,31.2264656430654));
#153878=CARTESIAN_POINT('Ctrl Pts',(6.57110895151815,2.44502632087633,31.3397623334207));
#153879=CARTESIAN_POINT('Ctrl Pts',(6.63285687696087,2.27907622776285,31.3317392576425));
#153880=CARTESIAN_POINT('Ctrl Pts',(6.68832843807726,2.11074736469941,31.3237161818643));
#153881=CARTESIAN_POINT('Ctrl Pts',(6.73734652205013,1.94056393976572,31.3156931060861));
#153882=CARTESIAN_POINT('Ctrl Pts',(6.78636203415064,1.77038944398654,31.3076704512613));
#153883=CARTESIAN_POINT('Ctrl Pts',(6.82892464653872,1.59836093374321,31.2996477964365));
#153884=CARTESIAN_POINT('Ctrl Pts',(6.86490740091012,1.42501682075319,31.2916251416116));
#153885=CARTESIAN_POINT('Ctrl Pts',(6.90090345642949,1.25160863052012,31.2835995211851));
#153886=CARTESIAN_POINT('Ctrl Pts',(6.93031472605805,1.07688422620562,31.2755739007585));
#153887=CARTESIAN_POINT('Ctrl Pts',(6.95306549893561,0.901391551996848,
31.2675482803319));
#153888=CARTESIAN_POINT('Ctrl Pts',(6.96256917139311,0.828083058111971,
31.2641957406968));
#153889=CARTESIAN_POINT('Ctrl Pts',(6.97091122194759,0.754640578532504,
31.2608432010616));
#153890=CARTESIAN_POINT('Ctrl Pts',(6.97808881553906,0.681104283460815,
31.2574906614265));
#153891=CARTESIAN_POINT('Ctrl Pts',(6.99876795302476,0.46924119361102,31.2478317657035));
#153892=CARTESIAN_POINT('Ctrl Pts',(7.00978401741194,0.256539866432542,
31.2381728699806));
#153893=CARTESIAN_POINT('Ctrl Pts',(7.0111131591244,0.0438044798241868,
31.2285139742577));
#153894=CARTESIAN_POINT('Ctrl Pts',(7.01120711473708,0.0287664418181586,
31.2278311972017));
#153895=CARTESIAN_POINT('Ctrl Pts',(7.01125268710363,0.0137282333579481,
31.2271484201457));
#153896=CARTESIAN_POINT('Ctrl Pts',(7.01124987764396,-0.00130986163894219,
31.2264656430897));
#153897=CARTESIAN_POINT('Ctrl Pts',(7.01124987764386,-0.00130986217404309,
31.2264656430654));
#153898=CARTESIAN_POINT('Ctrl Pts',(7.01121431189105,-0.19168132644035,
31.2178221767256));
#153899=CARTESIAN_POINT('Ctrl Pts',(7.00342087638219,-0.382039512845058,
31.2091787103858));
#153900=CARTESIAN_POINT('Ctrl Pts',(6.98789859162277,-0.571751550672562,
31.200535244046));
#153901=CARTESIAN_POINT('Ctrl Pts',(6.97237161482203,-0.76152093422815,
31.1918891649787));
#153902=CARTESIAN_POINT('Ctrl Pts',(6.94911114148364,-0.950643490621212,
31.1832430859113));
#153903=CARTESIAN_POINT('Ctrl Pts',(6.91819815905292,-1.13849057728942,
31.174597006844));
#153904=CARTESIAN_POINT('Ctrl Pts',(6.88728354559609,-1.32634757511729,
31.1659504715935));
#153905=CARTESIAN_POINT('Ctrl Pts',(6.84871566768912,-1.51292868433962,
31.157303936343));
#153906=CARTESIAN_POINT('Ctrl Pts',(6.80262687431758,-1.69761425869135,
31.1486574010926));
#153907=CARTESIAN_POINT('Ctrl Pts',(6.75652405074711,-1.88235605441837,
31.1400082336923));
#153908=CARTESIAN_POINT('Ctrl Pts',(6.70289580584609,-2.06520088150153,
31.131359066292));
#153909=CARTESIAN_POINT('Ctrl Pts',(6.64192504571639,-2.24554186101825,
31.1227098988917));
#153910=CARTESIAN_POINT('Ctrl Pts',(6.58579669808265,-2.41155982060071,
31.1147476646412));
#153911=CARTESIAN_POINT('Ctrl Pts',(6.52344643640313,-2.57545584263654,
31.1067854303906));
#153912=CARTESIAN_POINT('Ctrl Pts',(6.45505378653801,-2.73676947794317,
31.0988231961401));
#153913=CARTESIAN_POINT('Ctrl Pts',(6.37997453672923,-2.91385439491354,
31.0900825116438));
#153914=CARTESIAN_POINT('Ctrl Pts',(6.29760020324757,-3.08785749071656,
31.0813418271476));
#153915=CARTESIAN_POINT('Ctrl Pts',(6.20820478069621,-3.25819274498006,
31.0726011426514));
#153916=CARTESIAN_POINT('Ctrl Pts',(6.11882544186649,-3.42849735310156,
31.0638620307495));
#153917=CARTESIAN_POINT('Ctrl Pts',(6.02242766388431,-3.5951351952172,31.0551229188476));
#153918=CARTESIAN_POINT('Ctrl Pts',(5.91933170364109,-3.75754424388715,
31.0463838069457));
#153919=CARTESIAN_POINT('Ctrl Pts',(5.81489998685208,-3.92205753552982,
31.0375314672714));
#153920=CARTESIAN_POINT('Ctrl Pts',(5.70359544243871,-4.08223143695854,
31.028679127597));
#153921=CARTESIAN_POINT('Ctrl Pts',(5.58579740980158,-4.2375103373507,31.0198267879227));
#153922=CARTESIAN_POINT('Ctrl Pts',(5.46956570385669,-4.39072453868989,
31.0110921552729));
#153923=CARTESIAN_POINT('Ctrl Pts',(5.34701230226747,-4.53917289000252,
31.0023575226231));
#153924=CARTESIAN_POINT('Ctrl Pts',(5.21854397658004,-4.68235254193875,
30.9936228899733));
#153925=CARTESIAN_POINT('Ctrl Pts',(5.08747881168255,-4.8284264055979,30.9847116967867));
#153926=CARTESIAN_POINT('Ctrl Pts',(4.95025722691191,-4.96901606933813,
30.9758005036001));
#153927=CARTESIAN_POINT('Ctrl Pts',(4.80735358884143,-5.10362400989272,
30.9668893104135));
#153928=CARTESIAN_POINT('Ctrl Pts',(4.66444995077095,-5.23823195044731,
30.9579781172268));
#153929=CARTESIAN_POINT('Ctrl Pts',(4.51586447081601,-5.36685795016344,
30.9490669240402));
#153930=CARTESIAN_POINT('Ctrl Pts',(4.36211134490397,-5.48904465068013,
30.9401557308536));
#153931=CARTESIAN_POINT('Ctrl Pts',(4.22363706511502,-5.59908934247726,
30.9321300660012));
#153932=CARTESIAN_POINT('Ctrl Pts',(4.08090719246041,-5.703961092946,30.9241044011488));
#153933=CARTESIAN_POINT('Ctrl Pts',(3.93435465838164,-5.80331629196365,
30.9160787362964));
#153934=CARTESIAN_POINT('Ctrl Pts',(3.78784863648236,-5.90263995807824,
30.9080556185932));
#153935=CARTESIAN_POINT('Ctrl Pts',(3.63752267161901,-5.99645035300017,
30.90003250089));
#153936=CARTESIAN_POINT('Ctrl Pts',(3.48384041782166,-6.08444594894656,
30.8920093831867));
#153937=CARTESIAN_POINT('Ctrl Pts',(3.33017754470146,-6.17243044787821,
30.8839872772689));
#153938=CARTESIAN_POINT('Ctrl Pts',(3.17315954404523,-6.25460142689658,
30.875965171351));
#153939=CARTESIAN_POINT('Ctrl Pts',(3.01327646961216,-6.33070228965015,
30.8679430654331));
#153940=CARTESIAN_POINT('Ctrl Pts',(2.85333398208868,-6.40683143174133,
30.8599179784736));
#153941=CARTESIAN_POINT('Ctrl Pts',(2.6905246239216,-6.47688579104044,30.8518928915141));
#153942=CARTESIAN_POINT('Ctrl Pts',(2.52536073116679,-6.54065591053227,
30.8438678045545));
#153943=CARTESIAN_POINT('Ctrl Pts',(2.36016431020983,-6.60443858923002,
30.8358411370943));
#153944=CARTESIAN_POINT('Ctrl Pts',(2.19261277600286,-6.66193443870541,
30.827814469634));
#153945=CARTESIAN_POINT('Ctrl Pts',(2.02323538745976,-6.7129833255737,30.8197878021738));
#153946=CARTESIAN_POINT('Ctrl Pts',(1.85372202334592,-6.76407319430851,
30.8117546909332));
#153947=CARTESIAN_POINT('Ctrl Pts',(1.68238023093686,-6.80870566660739,
30.8037215796926));
#153948=CARTESIAN_POINT('Ctrl Pts',(1.50975187643278,-6.84677119773311,
30.795688468452));
#153949=CARTESIAN_POINT('Ctrl Pts',(1.40803297889223,-6.86920079147817,
30.7909550674904));
#153950=CARTESIAN_POINT('Ctrl Pts',(1.30586757525944,-6.88935131738097,
30.7862216665288));
#153951=CARTESIAN_POINT('Ctrl Pts',(1.20336758864659,-6.90720877121105,
30.7814882655671));
#153952=CARTESIAN_POINT('Ctrl Pts',(0.992214426213876,-6.94399568186168,
30.771737312273));
#153953=CARTESIAN_POINT('Ctrl Pts',(0.779516735558681,-6.97107099913154,
30.7619863589789));
#153954=CARTESIAN_POINT('Ctrl Pts',(0.566088162933685,-6.98835966119993,
30.7522354056848));
#153955=CARTESIAN_POINT('Ctrl Pts',(0.352352106411399,-7.00567323082932,
30.7424704043132));
#153956=CARTESIAN_POINT('Ctrl Pts',(0.137883100171667,-7.0131719389632,
30.7327054029416));
#153957=CARTESIAN_POINT('Ctrl Pts',(-0.0765005744095588,-7.0108326341894,
30.72294040157));
#153958=CARTESIAN_POINT('Ctrl Pts',(-0.290526915824577,-7.00849722855196,
30.7131916764325));
#153959=CARTESIAN_POINT('Ctrl Pts',(-0.504468171934545,-6.9963565832212,
30.7034429512949));
#153960=CARTESIAN_POINT('Ctrl Pts',(-0.717509612978354,-6.97443951280558,
30.6936942261573));
#153961=CARTESIAN_POINT('Ctrl Pts',(-0.92996633787348,-6.95258259624988,
30.6839722574902));
#153962=CARTESIAN_POINT('Ctrl Pts',(-1.14152813821791,-6.92100282538834,
30.6742502888231));
#153963=CARTESIAN_POINT('Ctrl Pts',(-1.35138703432115,-6.87978049402513,
30.6645283201559));
#153964=CARTESIAN_POINT('Ctrl Pts',(-1.55985734892056,-6.83883092006196,
30.6548706792163));
#153965=CARTESIAN_POINT('Ctrl Pts',(-1.76664716877632,-6.7883659490976,
30.6452130382766));
#153966=CARTESIAN_POINT('Ctrl Pts',(-1.97096519584124,-6.72851564308819,
30.6355553973369));
#153967=CARTESIAN_POINT('Ctrl Pts',(-2.06077000297908,-6.70220937307606,
30.6313105316515));
#153968=CARTESIAN_POINT('Ctrl Pts',(-2.15009729756754,-6.6740906170634,
30.6270656659661));
#153969=CARTESIAN_POINT('Ctrl Pts',(-2.23887997716637,-6.64417361380206,
30.6228208002807));
#153970=CARTESIAN_POINT('Ctrl Pts',(-2.4031037876147,-6.5888352944928,30.6149689532668));
#153971=CARTESIAN_POINT('Ctrl Pts',(-2.56539553607136,-6.52736341128647,
30.6071171062529));
#153972=CARTESIAN_POINT('Ctrl Pts',(-2.72524864978274,-6.45992618838306,
30.599265259239));
#153973=CARTESIAN_POINT('Ctrl Pts',(-2.88505643044338,-6.39250809013089,
30.5914156389454));
#153974=CARTESIAN_POINT('Ctrl Pts',(-3.04242660090272,-6.31912816543368,
30.5835660186518));
#153975=CARTESIAN_POINT('Ctrl Pts',(-3.1968710740518,-6.24000335724196,
30.5757163983582));
#153976=CARTESIAN_POINT('Ctrl Pts',(-3.35130321678492,-6.16088486615423,
30.5678674047564));
#153977=CARTESIAN_POINT('Ctrl Pts',(-3.50280978803967,-6.07602257922963,
30.5600184111546));
#153978=CARTESIAN_POINT('Ctrl Pts',(-3.65092612509904,-5.98567999408332,
30.5521694175528));
#153979=CARTESIAN_POINT('Ctrl Pts',(-3.79911744912295,-5.89529167113142,
30.5443164502354));
#153980=CARTESIAN_POINT('Ctrl Pts',(-3.94391478345556,-5.79941770523523,
30.536463482918));
#153981=CARTESIAN_POINT('Ctrl Pts',(-4.08488107547273,-5.69836583256505,
30.5286105156005));
#153982=CARTESIAN_POINT('Ctrl Pts',(-4.22588316819149,-5.59728829611463,
30.5207555538933));
#153983=CARTESIAN_POINT('Ctrl Pts',(-4.36305197863703,-5.49103046671003,
30.512900592186));
#153984=CARTESIAN_POINT('Ctrl Pts',(-4.49598306688087,-5.37994078264998,
30.5050456304787));
#153985=CARTESIAN_POINT('Ctrl Pts',(-4.62904610034134,-5.26874083279265,
30.4971828720654));
#153986=CARTESIAN_POINT('Ctrl Pts',(-4.75786272725996,-5.1526997046112,
30.489320113652));
#153987=CARTESIAN_POINT('Ctrl Pts',(-4.88206453378519,-5.03220353825805,
30.4814573552387));
#153988=CARTESIAN_POINT('Ctrl Pts',(-4.97317719686141,-4.94380927963927,
30.4756893484905));
#153989=CARTESIAN_POINT('Ctrl Pts',(-5.06180716553638,-4.85301833475441,
30.4699213417424));
#153990=CARTESIAN_POINT('Ctrl Pts',(-5.14782290711501,-4.75999431506824,
30.4641533349943));
#153991=CARTESIAN_POINT('Ctrl Pts',(-5.27276131814498,-4.62487633556926,
30.4557752685533));
#153992=CARTESIAN_POINT('Ctrl Pts',(-5.39245971855703,-4.48474669895984,
30.4473972021123));
#153993=CARTESIAN_POINT('Ctrl Pts',(-5.50651270748305,-4.34003967318592,
30.4390191356713));
#153994=CARTESIAN_POINT('Ctrl Pts',(-5.62048770833041,-4.19543159635682,
30.4306467980525));
#153995=CARTESIAN_POINT('Ctrl Pts',(-5.72882479108331,-4.04625262793735,
30.4222744604338));
#153996=CARTESIAN_POINT('Ctrl Pts',(-5.83115784931125,-3.89297119163703,
30.4139021228151));
#153997=CARTESIAN_POINT('Ctrl Pts',(-5.93343594062039,-3.73977208853781,
30.4055342822925));
#153998=CARTESIAN_POINT('Ctrl Pts',(-6.02971625560733,-3.58247518408994,
30.3971664417699));
#153999=CARTESIAN_POINT('Ctrl Pts',(-6.11967489796566,-3.42157941683501,
30.3887986012473));
#154000=CARTESIAN_POINT('Ctrl Pts',(-6.20959839845578,-3.26074650266123,
30.3804340295774));
#154001=CARTESIAN_POINT('Ctrl Pts',(-6.29320499072888,-3.09631781568865,
30.3720694579075));
#154002=CARTESIAN_POINT('Ctrl Pts',(-6.37021556185225,-2.92881891861471,
30.3637048862376));
#154003=CARTESIAN_POINT('Ctrl Pts',(-6.44720732169168,-2.76136093630438,
30.355342357772));
#154004=CARTESIAN_POINT('Ctrl Pts',(-6.51760613671886,-2.59083453803814,
30.3469798293064));
#154005=CARTESIAN_POINT('Ctrl Pts',(-6.58117988695108,-2.41778780253574,
30.3386173008408));
#154006=CARTESIAN_POINT('Ctrl Pts',(-6.64475871056746,-2.24472725736247,
30.3302541050193));
#154007=CARTESIAN_POINT('Ctrl Pts',(-6.70151126222156,-2.06914627954793,
30.3218909091978));
#154008=CARTESIAN_POINT('Ctrl Pts',(-6.75125414920415,-1.89161147579352,
30.3135277133763));
#154009=CARTESIAN_POINT('Ctrl Pts',(-6.80100042855192,-1.71406456452137,
30.3051639472016));
#154010=CARTESIAN_POINT('Ctrl Pts',(-6.84373600107348,-1.53456387818199,
30.2968001810269));
#154011=CARTESIAN_POINT('Ctrl Pts',(-6.8793277539502,-1.35368985230387,
30.2884364148522));
#154012=CARTESIAN_POINT('Ctrl Pts',(-6.91492667933099,-1.17277937641747,
30.2800709631986));
#154013=CARTESIAN_POINT('Ctrl Pts',(-6.94337885093577,-0.990495331733168,
30.2717055115451));
#154014=CARTESIAN_POINT('Ctrl Pts',(-6.96460246864214,-0.807427406200588,
30.2633400598915));
#154015=CARTESIAN_POINT('Ctrl Pts',(-6.98583319409635,-0.62429817157966,
30.2549718066647));
#154016=CARTESIAN_POINT('Ctrl Pts',(-6.99983050060385,-0.440384859104023,
30.2466035534378));
#154017=CARTESIAN_POINT('Ctrl Pts',(-7.00656450931262,-0.256281757721546,
30.2382353002109));
#154018=CARTESIAN_POINT('Ctrl Pts',(-7.01330476140818,-0.0720079664988862,
30.2298592884195));
#154019=CARTESIAN_POINT('Ctrl Pts',(-7.01276824690753,0.112455636350494,
30.221483276628));
#154020=CARTESIAN_POINT('Ctrl Pts',(-7.00497722994792,0.296514030715599,
30.2131072648365));
#154021=CARTESIAN_POINT('Ctrl Pts',(-6.99718239217732,0.480662689591468,
30.2047271453454));
#154022=CARTESIAN_POINT('Ctrl Pts',(-6.98212597764208,0.664405415695956,
30.1963470258542));
#154023=CARTESIAN_POINT('Ctrl Pts',(-6.95988216650108,0.847152165151158,
30.1879669063631));
#154024=CARTESIAN_POINT('Ctrl Pts',(-6.93761293898814,1.0301077259168,30.1795772115239));
#154025=CARTESIAN_POINT('Ctrl Pts',(-6.90813995077994,1.21206471037733,
30.1711875166847));
#154026=CARTESIAN_POINT('Ctrl Pts',(-6.87158878422795,1.39244179159226,
30.1627978218455));
#154027=CARTESIAN_POINT('Ctrl Pts',(-6.8483830793379,1.50696008773605,30.1574713493708));
#154028=CARTESIAN_POINT('Ctrl Pts',(-6.82232535479647,1.62084179431224,
30.1521448768961));
#154029=CARTESIAN_POINT('Ctrl Pts',(-6.79345819193923,1.73394127838109,
30.1468184044215));
#154030=CARTESIAN_POINT('Ctrl Pts',(-6.74803519108937,1.91190535425455,
30.1384371040166));
#154031=CARTESIAN_POINT('Ctrl Pts',(-6.69556204792646,2.08829092126232,
30.1300558036117));
#154032=CARTESIAN_POINT('Ctrl Pts',(-6.63616141893694,2.26251810695801,
30.1216745032068));
#154033=CARTESIAN_POINT('Ctrl Pts',(-6.57683607154906,2.43652448520081,
30.1133038248732));
#154034=CARTESIAN_POINT('Ctrl Pts',(-6.51060083998953,2.6083776259555,30.1049331465396));
#154035=CARTESIAN_POINT('Ctrl Pts',(-6.43762892445247,2.7775097467971,30.0965624682061));
#154036=CARTESIAN_POINT('Ctrl Pts',(-6.3647398195109,2.94644993172011,30.0882012891553));
#154037=CARTESIAN_POINT('Ctrl Pts',(-6.28512939688715,3.11267495222,30.0798401101044));
#154038=CARTESIAN_POINT('Ctrl Pts',(-6.19902015630494,3.27563362789935,
30.0714789310536));
#154039=CARTESIAN_POINT('Ctrl Pts',(-6.11302265261986,3.43838084547435,
30.0631286016189));
#154040=CARTESIAN_POINT('Ctrl Pts',(-6.02054330380952,3.59786988397599,
30.0547782721842));
#154041=CARTESIAN_POINT('Ctrl Pts',(-5.92185200977382,3.75357101129547,
30.0464279427494));
#154042=CARTESIAN_POINT('Ctrl Pts',(-5.8232366527853,3.90915233591134,30.0380840383937));
#154043=CARTESIAN_POINT('Ctrl Pts',(-5.71841905035115,4.0609512819887,30.029740134038));
#154044=CARTESIAN_POINT('Ctrl Pts',(-5.60771474562497,4.20846312734237,
30.0213962296822));
#154045=CARTESIAN_POINT('Ctrl Pts',(-5.49709935928672,4.35585649026193,
30.0130590272025));
#154046=CARTESIAN_POINT('Ctrl Pts',(-5.38060689655022,4.49896935857856,
30.0047218247228));
#154047=CARTESIAN_POINT('Ctrl Pts',(-5.25859597101388,4.6373262744966,29.9963846222431));
#154048=CARTESIAN_POINT('Ctrl Pts',(-5.21843064781213,4.68287260750423,
29.9936400612071));
#154049=CARTESIAN_POINT('Ctrl Pts',(-5.17766763597383,4.7279037864933,29.9908955001711));
#154050=CARTESIAN_POINT('Ctrl Pts',(-5.13632071722715,4.77240359276992,
29.988150939135));
#154051=CARTESIAN_POINT('Ctrl Pts',(-5.01070374824296,4.90759941761722,
29.9798126288331));
#154052=CARTESIAN_POINT('Ctrl Pts',(-4.87979739535233,5.03777707888049,
29.9714743185312));
#154053=CARTESIAN_POINT('Ctrl Pts',(-4.74403857862696,5.16253082576744,
29.9631360082293));
#154054=CARTESIAN_POINT('Ctrl Pts',(-4.60819434706087,5.28736306347862,
29.9547924517455));
#154055=CARTESIAN_POINT('Ctrl Pts',(-4.46749180331662,5.40676435837349,
29.9464488952617));
#154056=CARTESIAN_POINT('Ctrl Pts',(-4.32240126740431,5.52036899546051,
29.9381053387779));
#154057=CARTESIAN_POINT('Ctrl Pts',(-4.17720034724476,5.63406006246019,
29.9297554345527));
#154058=CARTESIAN_POINT('Ctrl Pts',(-4.02760503365489,5.74194547323107,
29.9214055303275));
#154059=CARTESIAN_POINT('Ctrl Pts',(-3.87411529770678,5.84370235574797,
29.9130556261023));
#154060=CARTESIAN_POINT('Ctrl Pts',(-3.72039533851287,5.94561186605871,
29.9046931976387));
#154061=CARTESIAN_POINT('Ctrl Pts',(-3.56276955744135,6.04137429772846,
29.896330769175));
#154062=CARTESIAN_POINT('Ctrl Pts',(-3.40176455166731,6.1307115816616,29.8879683407114));
#154063=CARTESIAN_POINT('Ctrl Pts',(-3.24062186466519,6.22012526115094,
29.8795987612314));
#154064=CARTESIAN_POINT('Ctrl Pts',(-3.07609447912067,6.30310268300638,
29.8712291817515));
#154065=CARTESIAN_POINT('Ctrl Pts',(-2.90873022784017,6.37941337617723,
29.8628596022715));
#154066=CARTESIAN_POINT('Ctrl Pts',(-2.74110783759349,6.4558417692947,29.8544771137349));
#154067=CARTESIAN_POINT('Ctrl Pts',(-2.57064014068247,6.52558276216785,
29.8460946251984));
#154068=CARTESIAN_POINT('Ctrl Pts',(-2.39789275106961,6.588454820128,29.8377121366618));
#154069=CARTESIAN_POINT('Ctrl Pts',(-2.34136697455426,6.60902758771239,
29.8349692490574));
#154070=CARTESIAN_POINT('Ctrl Pts',(-2.28459721094064,6.62886529793537,
29.832226361453));
#154071=CARTESIAN_POINT('Ctrl Pts',(-2.22760354135085,6.64796277253876,
29.8294834738486));
#154072=CARTESIAN_POINT('Ctrl Pts',(-2.05327316391254,6.7063775049062,29.8210936187158));
#154073=CARTESIAN_POINT('Ctrl Pts',(-1.87649502487367,6.75798071670244,
29.812703763583));
#154074=CARTESIAN_POINT('Ctrl Pts',(-1.6978281097707,6.80257350362144,29.8043139084503));
#154075=CARTESIAN_POINT('Ctrl Pts',(-1.51932606599218,6.84712514094184,
29.7959317953582));
#154076=CARTESIAN_POINT('Ctrl Pts',(-1.33893903809313,6.88467917035211,
29.7875496822661));
#154077=CARTESIAN_POINT('Ctrl Pts',(-1.15724183614367,6.91508625363262,
29.779167569174));
#154078=CARTESIAN_POINT('Ctrl Pts',(-0.975685592713515,6.94546974746107,
29.7707919588251));
#154079=CARTESIAN_POINT('Ctrl Pts',(-0.792821524714185,6.96871729517118,
29.7624163484762));
#154080=CARTESIAN_POINT('Ctrl Pts',(-0.609235770880054,6.98473036974085,
29.7540407381274));
#154081=CARTESIAN_POINT('Ctrl Pts',(-0.425765495211278,7.00073337184883,
29.7456703961618));
#154082=CARTESIAN_POINT('Ctrl Pts',(-0.241574765484927,7.009510945796,29.7373000541962));
#154083=CARTESIAN_POINT('Ctrl Pts',(-0.0572564586337002,7.01101620740137,
29.7289297122306));
#154084=CARTESIAN_POINT('Ctrl Pts',(0.126972928259185,7.01252074282929,
29.7205634083363));
#154085=CARTESIAN_POINT('Ctrl Pts',(0.311329441416462,7.00675995946011,
29.712197104442));
#154086=CARTESIAN_POINT('Ctrl Pts',(0.495218112667432,6.99373902740059,
29.7038308005477));
#154087=CARTESIAN_POINT('Ctrl Pts',(0.679055355411382,6.98072173693079,
29.695466836474));
#154088=CARTESIAN_POINT('Ctrl Pts',(0.862424689500081,6.96044836823139,
29.6871028724004));
#154089=CARTESIAN_POINT('Ctrl Pts',(1.04473362048138,6.93297614482668,29.6787389083268));
#154090=CARTESIAN_POINT('Ctrl Pts',(1.2270144971478,6.90550814894063,29.6703762313283));
#154091=CARTESIAN_POINT('Ctrl Pts',(1.40823497115759,6.87084355600778,29.6620135543297));
#154092=CARTESIAN_POINT('Ctrl Pts',(1.58780970527041,6.829091220825,29.6536508773312));
#154093=CARTESIAN_POINT('Ctrl Pts',(1.76738074226754,6.78733974524652,29.6452883725049));
#154094=CARTESIAN_POINT('Ctrl Pts',(1.94530578691105,6.73850089320938,29.6369258676786));
#154095=CARTESIAN_POINT('Ctrl Pts',(2.12101127109405,6.68273430194498,29.6285633628523));
#154096=CARTESIAN_POINT('Ctrl Pts',(2.29673655811301,6.62696142552298,29.6201999155323));
#154097=CARTESIAN_POINT('Ctrl Pts',(2.47024147285925,6.56425935313404,29.6118364682123));
#154098=CARTESIAN_POINT('Ctrl Pts',(2.64096873086428,6.49483723622826,29.6034730208923));
#154099=CARTESIAN_POINT('Ctrl Pts',(2.81179651787647,6.42537424162919,29.5951046489395));
#154100=CARTESIAN_POINT('Ctrl Pts',(2.97984307477428,6.34918341861954,29.5867362769867));
#154101=CARTESIAN_POINT('Ctrl Pts',(3.14457123150864,6.26652202840365,29.5783679050339));
#154102=CARTESIAN_POINT('Ctrl Pts',(3.30934874510399,6.18383587067488,29.5699970256981));
#154103=CARTESIAN_POINT('Ctrl Pts',(3.47080558453469,6.09467543208002,29.5616261463624));
#154104=CARTESIAN_POINT('Ctrl Pts',(3.62842960468568,5.99934372797063,29.5532552670266));
#154105=CARTESIAN_POINT('Ctrl Pts',(3.78618717796451,5.9039312503392,29.5448772951353));
#154106=CARTESIAN_POINT('Ctrl Pts',(3.94010516420754,5.80233723384743,29.536499323244));
#154107=CARTESIAN_POINT('Ctrl Pts',(4.08969983617666,5.69490841124566,29.5281213513527));
#154108=CARTESIAN_POINT('Ctrl Pts',(4.18476846836697,5.62663651968609,29.5227970819937));
#154109=CARTESIAN_POINT('Ctrl Pts',(4.27809165190787,5.55600897634346,29.5174728126348));
#154110=CARTESIAN_POINT('Ctrl Pts',(4.36955219335547,5.48312321510674,29.5121485432758));
#154111=CARTESIAN_POINT('Ctrl Pts',(4.50462026549713,5.37548620464291,29.5042857120865));
#154112=CARTESIAN_POINT('Ctrl Pts',(4.63590515167403,5.26269828661749,29.4964228808972));
#154113=CARTESIAN_POINT('Ctrl Pts',(4.76297282760709,5.14506719159008,29.4885600497079));
#154114=CARTESIAN_POINT('Ctrl Pts',(4.88994286880393,5.02752648053207,29.4807032600665));
#154115=CARTESIAN_POINT('Ctrl Pts',(5.01270186571746,4.90515025023247,29.4728464704251));
#154116=CARTESIAN_POINT('Ctrl Pts',(5.13084717804913,4.77828774751011,29.4649896807837));
#154117=CARTESIAN_POINT('Ctrl Pts',(5.2489258620171,4.65149678923421,29.4571373219998));
#154118=CARTESIAN_POINT('Ctrl Pts',(5.36239577814475,4.52022486952118,29.4492849632159));
#154119=CARTESIAN_POINT('Ctrl Pts',(5.47088981512912,4.38485931281911,29.4414326044319));
#154120=CARTESIAN_POINT('Ctrl Pts',(5.57935823540567,4.24952571750415,29.4335820996815));
#154121=CARTESIAN_POINT('Ctrl Pts',(5.68285287002689,4.1101007008737,29.4257315949311));
#154122=CARTESIAN_POINT('Ctrl Pts',(5.78104577594338,3.96700596154673,29.4178810901807));
#154123=CARTESIAN_POINT('Ctrl Pts',(5.87922288571611,3.8239342416533,29.410031848329));
#154124=CARTESIAN_POINT('Ctrl Pts',(5.97209975122812,3.6771942905496,29.4021826064774));
#154125=CARTESIAN_POINT('Ctrl Pts',(6.05939107001984,3.52723778941311,29.3943333646257));
#154126=CARTESIAN_POINT('Ctrl Pts',(6.14671179896544,3.37723076499623,29.3864814782109));
#154127=CARTESIAN_POINT('Ctrl Pts',(6.2284430301416,3.224005355905,29.378629591796));
#154128=CARTESIAN_POINT('Ctrl Pts',(6.30434475482012,3.06803907649039,29.3707777053812));
#154129=CARTESIAN_POINT('Ctrl Pts',(6.36007844652168,2.95351497878972,29.3650121629172));
#154130=CARTESIAN_POINT('Ctrl Pts',(6.41266993519047,2.83751361474207,29.3592466204533));
#154131=CARTESIAN_POINT('Ctrl Pts',(6.46204063733937,2.7202311232457,29.3534810779893));
#154132=CARTESIAN_POINT('Ctrl Pts',(6.50035037448015,2.62922448925273,29.3490072421585));
#154133=CARTESIAN_POINT('Ctrl Pts',(6.53671425519462,2.53746348401301,29.3445334063276));
#154134=CARTESIAN_POINT('Ctrl Pts',(6.57110895151813,2.4450263208764,29.3400595704968));
#154135=CARTESIAN_POINT('Origin',(0.,0.,50.));
#154136=CARTESIAN_POINT('',(6.57110895151815,2.44502632087633,27.3397910544677));
#154137=CARTESIAN_POINT('',(6.57110895151815,2.44502632087634,27.8869594752573));
#154138=CARTESIAN_POINT('',(6.57110895151814,2.44502632087636,50.));
#154139=CARTESIAN_POINT('',(7.01124999898235,0.000119457237031912,29.7735343568796));
#154140=CARTESIAN_POINT('Ctrl Pts',(6.57110895151814,2.44502632087635,27.8869594752573));
#154141=CARTESIAN_POINT('Ctrl Pts',(6.49449213640473,2.65093716745085,27.8969648340648));
#154142=CARTESIAN_POINT('Ctrl Pts',(6.40816968419754,2.85330601056279,27.9069701928724));
#154143=CARTESIAN_POINT('Ctrl Pts',(6.31245749192074,3.05131233655189,27.9169755516799));
#154144=CARTESIAN_POINT('Ctrl Pts',(6.23561263111062,3.21028652989345,27.9250085972787));
#154145=CARTESIAN_POINT('Ctrl Pts',(6.15267817288181,3.36652193378537,27.9330416428775));
#154146=CARTESIAN_POINT('Ctrl Pts',(6.063879900354,3.51951518203612,27.9410746884763));
#154147=CARTESIAN_POINT('Ctrl Pts',(5.9751387107748,3.67241008033615,27.9491025701241));
#154148=CARTESIAN_POINT('Ctrl Pts',(5.88054139339257,3.82206665589529,27.9571304517719));
#154149=CARTESIAN_POINT('Ctrl Pts',(5.78036050396136,3.96800441112955,27.9651583334197));
#154150=CARTESIAN_POINT('Ctrl Pts',(5.68022484718948,4.11387627402842,27.9731825903997));
#154151=CARTESIAN_POINT('Ctrl Pts',(5.57451084507305,4.25603235826394,27.9812068473798));
#154152=CARTESIAN_POINT('Ctrl Pts',(5.46353534836288,4.39401957889235,27.9892311043599));
#154153=CARTESIAN_POINT('Ctrl Pts',(5.35257326972032,4.53199011546066,27.9972543911256));
#154154=CARTESIAN_POINT('Ctrl Pts',(5.23635118721347,4.66579250210413,28.0052776778913));
#154155=CARTESIAN_POINT('Ctrl Pts',(5.11522747005976,4.79500516079452,28.013300964657));
#154156=CARTESIAN_POINT('Ctrl Pts',(4.99411367791395,4.92420723166043,28.0213235939859));
#154157=CARTESIAN_POINT('Ctrl Pts',(4.86809930484048,5.04882005895622,28.0293462233148));
#154158=CARTESIAN_POINT('Ctrl Pts',(4.73758074168348,5.16845772726544,28.0373688526438));
#154159=CARTESIAN_POINT('Ctrl Pts',(4.60701311283887,5.28814037082046,28.0453944979101));
#154160=CARTESIAN_POINT('Ctrl Pts',(4.47193818378545,5.40284387349322,28.0534201431765));
#154161=CARTESIAN_POINT('Ctrl Pts',(4.33278697619247,5.51222129285799,28.0614457884429));
#154162=CARTESIAN_POINT('Ctrl Pts',(4.25073494473848,5.57671688444728,28.0661781979507));
#154163=CARTESIAN_POINT('Ctrl Pts',(4.16726621787055,5.63936136101981,28.0709106074586));
#154164=CARTESIAN_POINT('Ctrl Pts',(4.08247411608823,5.70009049524388,28.0756430169664));
#154165=CARTESIAN_POINT('Ctrl Pts',(3.92605502595416,5.8121197493877,28.084373065801));
#154166=CARTESIAN_POINT('Ctrl Pts',(3.76505279119581,5.91768488095134,28.0931031146357));
#154167=CARTESIAN_POINT('Ctrl Pts',(3.60001325395084,6.01643840938128,28.1018331634704));
#154168=CARTESIAN_POINT('Ctrl Pts',(3.43492599531807,6.11522049251699,28.1105657366095));
#154169=CARTESIAN_POINT('Ctrl Pts',(3.26579933909619,6.20718690046475,28.1192983097487));
#154170=CARTESIAN_POINT('Ctrl Pts',(3.09320522066855,6.29203528481277,28.1280308828878));
#154171=CARTESIAN_POINT('Ctrl Pts',(2.91815912727661,6.37808907590394,28.1368875161683));
#154172=CARTESIAN_POINT('Ctrl Pts',(2.73954655923852,6.45682092833929,28.1457441494487));
#154173=CARTESIAN_POINT('Ctrl Pts',(2.55798720584053,6.52796507475769,28.1546007827291));
#154174=CARTESIAN_POINT('Ctrl Pts',(2.37885710470831,6.59815731715325,28.1633389148358));
#154175=CARTESIAN_POINT('Ctrl Pts',(2.1968588511512,6.66096355880477,28.1720770469426));
#154176=CARTESIAN_POINT('Ctrl Pts',(2.01260584967943,6.71617780112589,28.1808151790494));
#154177=CARTESIAN_POINT('Ctrl Pts',(1.82460475937334,6.77251521584304,28.1897310629166));
#154178=CARTESIAN_POINT('Ctrl Pts',(1.63425648870766,6.82094836000736,28.1986469467838));
#154179=CARTESIAN_POINT('Ctrl Pts',(1.44222785267097,6.86131222023019,28.2075628306511));
#154180=CARTESIAN_POINT('Ctrl Pts',(1.25019921663424,6.90167608045302,28.2164787145183));
#154181=CARTESIAN_POINT('Ctrl Pts',(1.05649051242281,6.93397060048049,28.2253945983855));
#154182=CARTESIAN_POINT('Ctrl Pts',(0.861779521940682,6.95808613183709,
28.2343104822528));
#154183=CARTESIAN_POINT('Ctrl Pts',(0.670894651624785,6.98172778690857,
28.243051166749));
#154184=CARTESIAN_POINT('Ctrl Pts',(0.479026245877058,6.99751141897453,
28.2517918512452));
#154185=CARTESIAN_POINT('Ctrl Pts',(0.28681877544978,7.00538089989042,28.2605325357414));
#154186=CARTESIAN_POINT('Ctrl Pts',(0.0946458863390992,7.01324896495598,
28.2692716476433));
#154187=CARTESIAN_POINT('Ctrl Pts',(-0.0978656721553102,7.01320571128652,
28.2780107595452));
#154188=CARTESIAN_POINT('Ctrl Pts',(-0.2900690439721,7.00524707003466,28.286749871447));
#154189=CARTESIAN_POINT('Ctrl Pts',(-0.484762687099649,6.99718531313089,
28.2956022111214));
#154190=CARTESIAN_POINT('Ctrl Pts',(-0.679139816174599,6.9810016176754,
28.3044545507957));
#154191=CARTESIAN_POINT('Ctrl Pts',(-0.872529556733192,6.95674627502879,
28.3133068904701));
#154192=CARTESIAN_POINT('Ctrl Pts',(-1.06334784931464,6.93281344872459,
28.3220415231198));
#154193=CARTESIAN_POINT('Ctrl Pts',(-1.25320457131862,6.90102234370817,
28.3307761557696));
#154194=CARTESIAN_POINT('Ctrl Pts',(-1.44146079353006,6.86147340905841,
28.3395107884193));
#154195=CARTESIAN_POINT('Ctrl Pts',(-1.63352239840614,6.82112503825429,
28.348421981606));
#154196=CARTESIAN_POINT('Ctrl Pts',(-1.82391782121114,6.77270190480895,
28.3573331747926));
#154197=CARTESIAN_POINT('Ctrl Pts',(-2.01197890935735,6.7163656415357,28.3662443679792));
#154198=CARTESIAN_POINT('Ctrl Pts',(-2.20003999750359,6.66002937826244,
28.3751555611659));
#154199=CARTESIAN_POINT('Ctrl Pts',(-2.38576645674396,6.5957800592414,28.3840667543525));
#154200=CARTESIAN_POINT('Ctrl Pts',(-2.56850496940774,6.52383390228689,
28.3929779475392));
#154201=CARTESIAN_POINT('Ctrl Pts',(-2.73308428303568,6.45903722118701,
28.4010036123916));
#154202=CARTESIAN_POINT('Ctrl Pts',(-2.89531542892217,6.38796714380733,
28.409029277244));
#154203=CARTESIAN_POINT('Ctrl Pts',(-3.05468423894557,6.3108264722489,28.4170549420963));
#154204=CARTESIAN_POINT('Ctrl Pts',(-3.21400246921774,6.23371028324748,
28.4250780597996));
#154205=CARTESIAN_POINT('Ctrl Pts',(-3.37045984267823,6.15052749538051,
28.4331011775028));
#154206=CARTESIAN_POINT('Ctrl Pts',(-3.523563244396,6.06152857167576,28.441124295206));
#154207=CARTESIAN_POINT('Ctrl Pts',(-3.67664733843497,5.97254087151414,
28.4491464011239));
#154208=CARTESIAN_POINT('Ctrl Pts',(-3.82637798670055,5.87773868117624,
28.4571685070418));
#154209=CARTESIAN_POINT('Ctrl Pts',(-3.9722877577215,5.77741780836006,28.4651906129596));
#154210=CARTESIAN_POINT('Ctrl Pts',(-4.11825174930623,5.67705965596866,
28.4732156999191));
#154211=CARTESIAN_POINT('Ctrl Pts',(-4.2603917231887,5.57117892973248,28.4812407868787));
#154212=CARTESIAN_POINT('Ctrl Pts',(-4.39826990371879,5.46011432266226,
28.4892658738382));
#154213=CARTESIAN_POINT('Ctrl Pts',(-4.53617523866651,5.3490278419735,28.4972925412984));
#154214=CARTESIAN_POINT('Ctrl Pts',(-4.66981682822056,5.23275568338216,
28.5053192087587));
#154215=CARTESIAN_POINT('Ctrl Pts',(-4.79879112615074,5.11167587881674,
28.5133458762189));
#154216=CARTESIAN_POINT('Ctrl Pts',(-4.92786896419288,4.99049887181083,
28.5213789874595));
#154217=CARTESIAN_POINT('Ctrl Pts',(-5.05227176630182,4.86450676794351,
28.5294120987001));
#154218=CARTESIAN_POINT('Ctrl Pts',(-5.17163347093701,4.73411383521605,
28.5374452099407));
#154219=CARTESIAN_POINT('Ctrl Pts',(-5.24196572335827,4.65728158247163,
28.5421786109023));
#154220=CARTESIAN_POINT('Ctrl Pts',(-5.31054845581914,4.57892201252761,
28.546912011864));
#154221=CARTESIAN_POINT('Ctrl Pts',(-5.37731352235279,4.49912500880136,
28.5516454128256));
#154222=CARTESIAN_POINT('Ctrl Pts',(-5.51485163727835,4.33474069767834,
28.5613963661197));
#154223=CARTESIAN_POINT('Ctrl Pts',(-5.64475541595091,4.16415819944942,
28.5711473194139));
#154224=CARTESIAN_POINT('Ctrl Pts',(-5.76655261146059,3.98804432545039,
28.580898272708));
#154225=CARTESIAN_POINT('Ctrl Pts',(-5.88852527867925,3.81167672637735,
28.5906632740796));
#154226=CARTESIAN_POINT('Ctrl Pts',(-6.00236797921543,3.6297618429951,28.6004282754512));
#154227=CARTESIAN_POINT('Ctrl Pts',(-6.10765108552397,3.44299648271646,
28.6101932768228));
#154228=CARTESIAN_POINT('Ctrl Pts',(-6.21275870670836,3.25654242159665,
28.6199420019604));
#154229=CARTESIAN_POINT('Ctrl Pts',(-6.30933522912802,3.0652540747158,28.629690727098));
#154230=CARTESIAN_POINT('Ctrl Pts',(-6.39699779056177,2.86985118604569,
28.6394394522356));
#154231=CARTESIAN_POINT('Ctrl Pts',(-6.48441975225538,2.67498460253787,
28.6491614209027));
#154232=CARTESIAN_POINT('Ctrl Pts',(-6.56297657772261,2.4760260579487,28.6588833895698));
#154233=CARTESIAN_POINT('Ctrl Pts',(-6.6323333495813,2.27371522019176,28.668605358237));
#154234=CARTESIAN_POINT('Ctrl Pts',(-6.70123120579561,2.07274302040754,
28.6782629991767));
#154235=CARTESIAN_POINT('Ctrl Pts',(-6.7610503122403,1.86846277810626,28.6879206401164));
#154236=CARTESIAN_POINT('Ctrl Pts',(-6.81150718628199,1.66162463081433,
28.697578281056));
#154237=CARTESIAN_POINT('Ctrl Pts',(-6.8336847195478,1.57071214407534,28.7018231467414));
#154238=CARTESIAN_POINT('Ctrl Pts',(-6.85405414701578,1.4793058181311,28.7060680124267));
#154239=CARTESIAN_POINT('Ctrl Pts',(-6.87259420767519,1.38747087145262,
28.7103128781121));
#154240=CARTESIAN_POINT('Ctrl Pts',(-6.90688827743316,1.21760119705035,
28.718164725126));
#154241=CARTESIAN_POINT('Ctrl Pts',(-6.93490536937299,1.04633401805437,
28.7260165721399));
#154242=CARTESIAN_POINT('Ctrl Pts',(-6.95653755564094,0.874192083844924,
28.7338684191538));
#154243=CARTESIAN_POINT('Ctrl Pts',(-6.97816360719576,0.702098967696304,
28.7417180394474));
#154244=CARTESIAN_POINT('Ctrl Pts',(-6.99340830737022,0.529131967908664,
28.749567659741));
#154245=CARTESIAN_POINT('Ctrl Pts',(-7.00221515756077,0.355822216459495,
28.7574172800346));
#154246=CARTESIAN_POINT('Ctrl Pts',(-7.01102130463699,0.182526301577319,
28.7652662736364));
#154247=CARTESIAN_POINT('Ctrl Pts',(-7.01339060631142,0.0088880705190284,
28.7731152672382));
#154248=CARTESIAN_POINT('Ctrl Pts',(-7.00931859181233,-0.164558320889845,
28.78096426084));
#154249=CARTESIAN_POINT('Ctrl Pts',(-7.00524451577152,-0.338092523127861,
28.7888172281574));
#154250=CARTESIAN_POINT('Ctrl Pts',(-6.9947226167812,-0.51143430980403,
28.7966701954748));
#154251=CARTESIAN_POINT('Ctrl Pts',(-6.97780054194222,-0.684051284167264,
28.8045231627923));
#154252=CARTESIAN_POINT('Ctrl Pts',(-6.96087416946482,-0.856712097441932,
28.8123781244995));
#154253=CARTESIAN_POINT('Ctrl Pts',(-6.93754443419944,-1.02864735363224,
28.8202330862068));
#154254=CARTESIAN_POINT('Ctrl Pts',(-6.9079105436122,-1.19933251600692,
28.828088047914));
#154255=CARTESIAN_POINT('Ctrl Pts',(-6.87824723891148,-1.37018709767266,
28.8359508063274));
#154256=CARTESIAN_POINT('Ctrl Pts',(-6.84226736039405,-1.53978873428667,
28.8438135647407));
#154257=CARTESIAN_POINT('Ctrl Pts',(-6.80012078706305,-1.70762520590818,
28.8516763231541));
#154258=CARTESIAN_POINT('Ctrl Pts',(-6.76920266563492,-1.83074763317909,
28.8574443299022));
#154259=CARTESIAN_POINT('Ctrl Pts',(-6.73496700950739,-1.95292040784697,
28.8632123366503));
#154260=CARTESIAN_POINT('Ctrl Pts',(-6.69748962124275,-2.07394776593957,
28.8689803433985));
#154261=CARTESIAN_POINT('Ctrl Pts',(-6.64305347672562,-2.24974077235539,
28.8773584098395));
#154262=CARTESIAN_POINT('Ctrl Pts',(-6.58165583125913,-2.42350599110958,
28.8857364762805));
#154263=CARTESIAN_POINT('Ctrl Pts',(-6.51346971504031,-2.59467509213634,
28.8941145427215));
#154264=CARTESIAN_POINT('Ctrl Pts',(-6.44533022367758,-2.76572714976562,
28.9024868803403));
#154265=CARTESIAN_POINT('Ctrl Pts',(-6.37041163735338,-2.93418632446769,
28.910859217959));
#154266=CARTESIAN_POINT('Ctrl Pts',(-6.28893622386575,-3.099501207396,28.9192315555777));
#154267=CARTESIAN_POINT('Ctrl Pts',(-6.20750457387462,-3.26472729350828,
28.9275993961003));
#154268=CARTESIAN_POINT('Ctrl Pts',(-6.11952326408598,-3.426812161188,28.9359672366229));
#154269=CARTESIAN_POINT('Ctrl Pts',(-6.02526210732891,-3.58522566939466,
28.9443350771455));
#154270=CARTESIAN_POINT('Ctrl Pts',(-5.93103777319457,-3.74357729420153,
28.9526996488154));
#154271=CARTESIAN_POINT('Ctrl Pts',(-5.8305386519412,-3.89826013745946,
28.9610642204853));
#154272=CARTESIAN_POINT('Ctrl Pts',(-5.72408002124771,-4.04876950107718,
28.9694287921552));
#154273=CARTESIAN_POINT('Ctrl Pts',(-5.61764739508189,-4.19924209994522,
28.9777913206208));
#154274=CARTESIAN_POINT('Ctrl Pts',(-5.50525835252799,-4.345542984347,28.9861538490864));
#154275=CARTESIAN_POINT('Ctrl Pts',(-5.38727118564399,-4.48719686829428,
28.994516377552));
#154276=CARTESIAN_POINT('Ctrl Pts',(-5.26927460301499,-4.62886205666461,
29.0028795733735));
#154277=CARTESIAN_POINT('Ctrl Pts',(-5.14567920922331,-4.76587924727605,
29.011242769195));
#154278=CARTESIAN_POINT('Ctrl Pts',(-5.01688372631647,-4.89780606385359,
29.0196059650165));
#154279=CARTESIAN_POINT('Ctrl Pts',(-4.88807945981585,-5.02974187757559,
29.0279697311912));
#154280=CARTESIAN_POINT('Ctrl Pts',(-4.75407462659777,-5.15658638959434,
29.0363334973659));
#154281=CARTESIAN_POINT('Ctrl Pts',(-4.61530508773846,-5.27793382959615,
29.0446972635406));
#154282=CARTESIAN_POINT('Ctrl Pts',(-4.47650758383102,-5.39930572371829,
29.0530627151942));
#154283=CARTESIAN_POINT('Ctrl Pts',(-4.33294370715091,-5.51517812046617,
29.0614281668478));
#154284=CARTESIAN_POINT('Ctrl Pts',(-4.18508301291899,-5.62518504028773,
29.0697936185013));
#154285=CARTESIAN_POINT('Ctrl Pts',(-4.03717280043112,-5.73522880121059,
29.0781618717282));
#154286=CARTESIAN_POINT('Ctrl Pts',(-3.8849631646743,-5.83940297208849,
29.0865301249551));
#154287=CARTESIAN_POINT('Ctrl Pts',(-3.7289536328408,-5.93738421921837,
29.094898378182));
#154288=CARTESIAN_POINT('Ctrl Pts',(-3.57279945791429,-6.03545630894279,
29.1032743899734));
#154289=CARTESIAN_POINT('Ctrl Pts',(-3.41283862552856,-6.12732382619703,
29.1116504017649));
#154290=CARTESIAN_POINT('Ctrl Pts',(-3.24959739566591,-6.21270821209087,
29.1200264135564));
#154291=CARTESIAN_POINT('Ctrl Pts',(-3.08627611028722,-6.29813447154251,
29.1284065330475));
#154292=CARTESIAN_POINT('Ctrl Pts',(-2.91967151346045,-6.37707111278823,
29.1367866525387));
#154293=CARTESIAN_POINT('Ctrl Pts',(-2.75033154339166,-6.44928701205993,
29.1451667720298));
#154294=CARTESIAN_POINT('Ctrl Pts',(-2.58079808095614,-6.5215854271444,
29.153556466869));
#154295=CARTESIAN_POINT('Ctrl Pts',(-2.40852330489872,-6.5871476324327,
29.1619461617082));
#154296=CARTESIAN_POINT('Ctrl Pts',(-2.23407333608442,-6.64579136683485,
29.1703358565475));
#154297=CARTESIAN_POINT('Ctrl Pts',(-2.12331806132192,-6.68302326180712,
29.1756623290221));
#154298=CARTESIAN_POINT('Ctrl Pts',(-2.01168633077783,-6.71746748972033,
29.1809888014967));
#154299=CARTESIAN_POINT('Ctrl Pts',(-1.89932553437362,-6.74908801816782,
29.1863152739714));
#154300=CARTESIAN_POINT('Ctrl Pts',(-1.72252379684822,-6.79884348938106,
29.1946965743762));
#154301=CARTESIAN_POINT('Ctrl Pts',(-1.54355969267688,-6.84170545877291,
29.2030778747811));
#154302=CARTESIAN_POINT('Ctrl Pts',(-1.36299661903062,-6.87748986033503,
29.211459175186));
#154303=CARTESIAN_POINT('Ctrl Pts',(-1.18266238264766,-6.91322891040663,
29.2198298535196));
#154304=CARTESIAN_POINT('Ctrl Pts',(-1.00073353410862,-6.94190820531127,
29.2282005318531));
#154305=CARTESIAN_POINT('Ctrl Pts',(-0.817788303416799,-6.96339348689234,
29.2365712101867));
#154306=CARTESIAN_POINT('Ctrl Pts',(-0.635050684151665,-6.98485438636766,
29.2449323892375));
#154307=CARTESIAN_POINT('Ctrl Pts',(-0.45129930506122,-6.9991375062249,
29.2532935682883));
#154308=CARTESIAN_POINT('Ctrl Pts',(-0.267122700120177,-7.00615957751324,
29.2616547473392));
#154309=CARTESIAN_POINT('Ctrl Pts',(-0.0831850860494773,-7.01317253683577,
29.2700050767739));
#154310=CARTESIAN_POINT('Ctrl Pts',(0.101176327419426,-7.01294322847668,
29.2783554062086));
#154311=CARTESIAN_POINT('Ctrl Pts',(0.285367848513169,-7.00544015416126,
29.2867057356433));
#154312=CARTESIAN_POINT('Ctrl Pts',(0.469417645249815,-6.99794285301269,
29.2950496399991));
#154313=CARTESIAN_POINT('Ctrl Pts',(0.653297484127329,-6.98318295244637,
29.3033935443548));
#154314=CARTESIAN_POINT('Ctrl Pts',(0.836412478337948,-6.96118098662724,
29.3117374487106));
#154315=CARTESIAN_POINT('Ctrl Pts',(1.01938039344278,-6.93919669292432,
29.3200746511903));
#154316=CARTESIAN_POINT('Ctrl Pts',(1.20158436470146,-6.90998197386488,
29.32841185367));
#154317=CARTESIAN_POINT('Ctrl Pts',(1.38243328121407,-6.87360929828658,
29.3367490561497));
#154318=CARTESIAN_POINT('Ctrl Pts',(1.44196774626718,-6.86163561425871,
29.3394936171857));
#154319=CARTESIAN_POINT('Ctrl Pts',(1.50135540542682,-6.84888664744455,
29.3422381782218));
#154320=CARTESIAN_POINT('Ctrl Pts',(1.56057531963233,-6.83536621069087,
29.3449827392578));
#154321=CARTESIAN_POINT('Ctrl Pts',(1.74049262306095,-6.79428947907898,
29.3533210495597));
#154322=CARTESIAN_POINT('Ctrl Pts',(1.91871320861433,-6.74612185920696,
29.3616593598616));
#154323=CARTESIAN_POINT('Ctrl Pts',(2.09466711579002,-6.69103850209576,
29.3699976701635));
#154324=CARTESIAN_POINT('Ctrl Pts',(2.27073172719311,-6.63592048840553,
29.3783412266473));
#154325=CARTESIAN_POINT('Ctrl Pts',(2.44452650296433,-6.57387815646015,
29.3866847831311));
#154326=CARTESIAN_POINT('Ctrl Pts',(2.61549942395021,-6.50513561163917,
29.3950283396149));
#154327=CARTESIAN_POINT('Ctrl Pts',(2.78660242038971,-6.4363407677895,29.4033782438401));
#154328=CARTESIAN_POINT('Ctrl Pts',(2.95487897611399,-6.36083566531951,
29.4117281480654));
#154329=CARTESIAN_POINT('Ctrl Pts',(3.11979931998863,-6.27889152362887,
29.4200780522906));
#154330=CARTESIAN_POINT('Ctrl Pts',(3.28496703217464,-6.19682447178973,
29.4284404807543));
#154331=CARTESIAN_POINT('Ctrl Pts',(3.44676817917632,-6.10829922676537,
29.4368029092179));
#154332=CARTESIAN_POINT('Ctrl Pts',(3.60469844876366,-6.01363248427944,
29.4451653376816));
#154333=CARTESIAN_POINT('Ctrl Pts',(3.76276377026057,-5.9188847888237,29.4535349171615));
#154334=CARTESIAN_POINT('Ctrl Pts',(3.9169513362688,-5.81798529615717,29.4619044966415));
#154335=CARTESIAN_POINT('Ctrl Pts',(4.06678741138989,-5.71129291080932,
29.4702740761214));
#154336=CARTESIAN_POINT('Ctrl Pts',(4.21685459040094,-5.60443596545639,
29.478656564658));
#154337=CARTESIAN_POINT('Ctrl Pts',(4.36255660796396,-5.49176847300578,
29.4870390531946));
#154338=CARTESIAN_POINT('Ctrl Pts',(4.50345319323985,-5.37368922610881,
29.4954215417311));
#154339=CARTESIAN_POINT('Ctrl Pts',(4.54955686466963,-5.33505176168087,
29.4981644293355));
#154340=CARTESIAN_POINT('Ctrl Pts',(4.59514631446224,-5.2958351468955,29.5009073169399));
#154341=CARTESIAN_POINT('Ctrl Pts',(4.64020700827224,-5.25605417427191,
29.5036502045443));
#154342=CARTESIAN_POINT('Ctrl Pts',(4.77571791990833,-5.13642095493618,
29.5118988835671));
#154343=CARTESIAN_POINT('Ctrl Pts',(4.90674524486949,-5.01141517077875,
29.52014756259));
#154344=CARTESIAN_POINT('Ctrl Pts',(5.03284519947687,-4.88140305246378,
29.5283962416128));
#154345=CARTESIAN_POINT('Ctrl Pts',(5.15882230318774,-4.75151759640924,
29.5366368844899));
#154346=CARTESIAN_POINT('Ctrl Pts',(5.27988136223031,-4.6166357707436,29.544877527367));
#154347=CARTESIAN_POINT('Ctrl Pts',(5.39561293035008,-4.47716290393135,
29.5531181702441));
#154348=CARTESIAN_POINT('Ctrl Pts',(5.51125271317169,-4.33780065135232,
29.5613522775677));
#154349=CARTESIAN_POINT('Ctrl Pts',(5.62157320513941,-4.1938548782192,29.5695863848912));
#154350=CARTESIAN_POINT('Ctrl Pts',(5.72620281943154,-4.04576665580633,
29.5778204922147));
#154351=CARTESIAN_POINT('Ctrl Pts',(5.83076368565356,-3.89777573643299,
29.586049189225));
#154352=CARTESIAN_POINT('Ctrl Pts',(5.92964092982658,-3.74564807526189,
29.5942778862353));
#154353=CARTESIAN_POINT('Ctrl Pts',(6.02250405524087,-3.58985674743537,
29.6025065832456));
#154354=CARTESIAN_POINT('Ctrl Pts',(6.11533308220262,-3.43412262469619,
29.610732258757));
#154355=CARTESIAN_POINT('Ctrl Pts',(6.20215221349858,-3.27472781168244,
29.6189579342683));
#154356=CARTESIAN_POINT('Ctrl Pts',(6.28267476045562,-3.11217358398176,
29.6271836097797));
#154357=CARTESIAN_POINT('Ctrl Pts',(6.3631809559691,-2.94965236562295,29.6354076149307));
#154358=CARTESIAN_POINT('Ctrl Pts',(6.43739296194922,-2.78397332036744,
29.6436316200817));
#154359=CARTESIAN_POINT('Ctrl Pts',(6.50507036382054,-2.61566169912007,
29.6518556252327));
#154360=CARTESIAN_POINT('Ctrl Pts',(6.57274512885284,-2.44735663561043,
29.660079309961));
#154361=CARTESIAN_POINT('Ctrl Pts',(6.63388566909423,-2.27641952117878,
29.6683029946893));
#154362=CARTESIAN_POINT('Ctrl Pts',(6.68829989246451,-2.10339513904528,
29.6765266794176));
#154363=CARTESIAN_POINT('Ctrl Pts',(6.74274013189878,-1.93028803197112,
29.6847542959838));
#154364=CARTESIAN_POINT('Ctrl Pts',(6.79044752185053,-1.75509199202338,
29.69298191255));
#154365=CARTESIAN_POINT('Ctrl Pts',(6.83127976266757,-1.57836731044091,
29.7012095291163));
#154366=CARTESIAN_POINT('Ctrl Pts',(6.87212112187813,-1.40160316383868,
29.7094389830209));
#154367=CARTESIAN_POINT('Ctrl Pts',(6.90608420006113,-1.22331003323168,
29.7176684369256));
#154368=CARTESIAN_POINT('Ctrl Pts',(6.93307788002744,-1.04405827039217,
29.7258978908303));
#154369=CARTESIAN_POINT('Ctrl Pts',(6.96009610059357,-0.86464354548948,
29.7341348263283));
#154370=CARTESIAN_POINT('Ctrl Pts',(6.98013221510365,-0.684268789542715,
29.7423717618262));
#154371=CARTESIAN_POINT('Ctrl Pts',(6.99314691492785,-0.503510465368024,
29.7506086973242));
#154372=CARTESIAN_POINT('Ctrl Pts',(7.00522141267682,-0.335810402528576,
29.7582505838427));
#154373=CARTESIAN_POINT('Ctrl Pts',(7.01125285965042,-0.16778045001463,
29.7658924703612));
#154374=CARTESIAN_POINT('Ctrl Pts',(7.01124999898235,0.000119457236979679,
29.7735343568796));
#154375=CARTESIAN_POINT('Ctrl Pts',(7.01124999898234,0.000119457914987822,
29.7735343569105));
#154376=CARTESIAN_POINT('Ctrl Pts',(7.01124407803179,0.347633178975341,
29.7893512829794));
#154377=CARTESIAN_POINT('Ctrl Pts',(6.98539996000983,0.694636108610281,
29.8051682090482));
#154378=CARTESIAN_POINT('Ctrl Pts',(6.93395267227691,1.0382325852736,29.820985135117));
#154379=CARTESIAN_POINT('Ctrl Pts',(6.90837589769859,1.20904994060521,29.8288484447376));
#154380=CARTESIAN_POINT('Ctrl Pts',(6.87644550131219,1.37917031431264,29.8367117543582));
#154381=CARTESIAN_POINT('Ctrl Pts',(6.83821065173588,1.54806383750348,29.8445750639788));
#154382=CARTESIAN_POINT('Ctrl Pts',(6.80000851446076,1.7168128617395,29.8524316460471));
#154383=CARTESIAN_POINT('Ctrl Pts',(6.75551274019734,1.88433675449325,29.8602882281153));
#154384=CARTESIAN_POINT('Ctrl Pts',(6.70482413161581,2.05011217415103,29.8681448101836));
#154385=CARTESIAN_POINT('Ctrl Pts',(6.66420330613044,2.18296124182378,29.8744409161142));
#154386=CARTESIAN_POINT('Ctrl Pts',(6.61960639339951,2.31468744814057,29.8807370220449));
#154387=CARTESIAN_POINT('Ctrl Pts',(6.57110895151814,2.44502632087637,29.8870331279755));
#154388=CARTESIAN_POINT('',(7.01124997488654,0.000593425250984153,29.2264656431291));
#154389=CARTESIAN_POINT('Ctrl Pts',(6.57110895151813,2.4450263208764,29.3400595704968));
#154390=CARTESIAN_POINT('Ctrl Pts',(6.64399555118415,2.24914058196973,29.3305789610997));
#154391=CARTESIAN_POINT('Ctrl Pts',(6.70803579118306,2.05021802406892,29.3210983517026));
#154392=CARTESIAN_POINT('Ctrl Pts',(6.76304630522514,1.84900817626114,29.3116177423055));
#154393=CARTESIAN_POINT('Ctrl Pts',(6.81821243560133,1.6472291365553,29.3021103137138));
#154394=CARTESIAN_POINT('Ctrl Pts',(6.864297702838,1.44314996512382,29.2926028851222));
#154395=CARTESIAN_POINT('Ctrl Pts',(6.90116951794474,1.23753216002269,29.2830954565305));
#154396=CARTESIAN_POINT('Ctrl Pts',(6.93813914256544,1.03136891452158,29.2735628076733));
#154397=CARTESIAN_POINT('Ctrl Pts',(6.96584637654926,0.823658970759291,
29.264030158816));
#154398=CARTESIAN_POINT('Ctrl Pts',(6.98420988671341,0.615173813515072,
29.2544975099588));
#154399=CARTESIAN_POINT('Ctrl Pts',(7.00220990185979,0.410815498865802,
29.2451535543489));
#154400=CARTESIAN_POINT('Ctrl Pts',(7.01123261381448,0.205712462309202,
29.235809598739));
#154401=CARTESIAN_POINT('Ctrl Pts',(7.01124997488654,0.000593425251026187,
29.2264656431291));
#154402=CARTESIAN_POINT('Ctrl Pts',(7.01124997488661,0.000593424383951388,
29.2264656430896));
#154403=CARTESIAN_POINT('Ctrl Pts',(7.01126957801832,-0.231015623751386,
29.2159149662941));
#154404=CARTESIAN_POINT('Ctrl Pts',(6.9998102786117,-0.46267258523056,29.2053642894985));
#154405=CARTESIAN_POINT('Ctrl Pts',(6.97687299454424,-0.693447748932306,
29.1948136127029));
#154406=CARTESIAN_POINT('Ctrl Pts',(6.95940906759447,-0.869154715321837,
29.186780567104));
#154407=CARTESIAN_POINT('Ctrl Pts',(6.93528503923172,-1.04438501249477,
29.1787475215051));
#154408=CARTESIAN_POINT('Ctrl Pts',(6.90453974263472,-1.21858832461075,
29.1707144759062));
#154409=CARTESIAN_POINT('Ctrl Pts',(6.8738142102982,-1.39267965213017,29.1626865942583));
#154410=CARTESIAN_POINT('Ctrl Pts',(6.83647594565298,-1.56574494922353,
29.1546587126104));
#154411=CARTESIAN_POINT('Ctrl Pts',(6.79261556688361,-1.73723928203066,
29.1466308309625));
#154412=CARTESIAN_POINT('Ctrl Pts',(6.74877499150779,-1.90865618345534,
29.1386065739824));
#154413=CARTESIAN_POINT('Ctrl Pts',(6.69841825607998,-2.07850317850176,
29.1305823170023));
#154414=CARTESIAN_POINT('Ctrl Pts',(6.64168700062609,-2.24624583432321,
29.1225580600221));
#154415=CARTESIAN_POINT('Ctrl Pts',(6.5849626045586,-2.41396820834972,29.1145347732563));
#154416=CARTESIAN_POINT('Ctrl Pts',(6.52186533372496,-2.57958640042939,
29.1065114864905));
#154417=CARTESIAN_POINT('Ctrl Pts',(6.45258665145337,-2.74258127828253,
29.0984881997248));
#154418=CARTESIAN_POINT('Ctrl Pts',(6.3833136459519,-2.90556280015916,29.0904655703958));
#154419=CARTESIAN_POINT('Ctrl Pts',(6.30786038505268,-3.06592110012482,
29.0824429410668));
#154420=CARTESIAN_POINT('Ctrl Pts',(6.22646630163365,-3.2231574514939,29.0744203117378));
#154421=CARTESIAN_POINT('Ctrl Pts',(6.14504161983387,-3.3804529125371,29.0663946664714));
#154422=CARTESIAN_POINT('Ctrl Pts',(6.05767182536901,-3.53462375608389,
29.0583690212049));
#154423=CARTESIAN_POINT('Ctrl Pts',(5.9646422756733,-3.68519593586974,29.0503433759384));
#154424=CARTESIAN_POINT('Ctrl Pts',(5.90978638423711,-3.77398246847858,
29.0456109664311));
#154425=CARTESIAN_POINT('Ctrl Pts',(5.85296344717681,-3.86151824762984,
29.0408785569238));
#154426=CARTESIAN_POINT('Ctrl Pts',(5.79423899333342,-3.94771086208635,
29.0361461474164));
#154427=CARTESIAN_POINT('Ctrl Pts',(5.68590784636769,-4.10671352916862,
29.0274160985818));
#154428=CARTESIAN_POINT('Ctrl Pts',(5.57104950672835,-4.26122332955139,
29.0186860497472));
#154429=CARTESIAN_POINT('Ctrl Pts',(5.45005695877084,-4.41072621102847,
29.0099560009125));
#154430=CARTESIAN_POINT('Ctrl Pts',(5.32902942566769,-4.56027232144957,
29.0012234277734));
#154431=CARTESIAN_POINT('Ctrl Pts',(5.20186431615247,-4.70480841022049,
28.9924908546343));
#154432=CARTESIAN_POINT('Ctrl Pts',(5.06899464155256,-4.84385382587165,
28.9837582814952));
#154433=CARTESIAN_POINT('Ctrl Pts',(4.9342373411241,-4.98487460361137,28.9749016482147));
#154434=CARTESIAN_POINT('Ctrl Pts',(4.79361235562339,-5.12024730212231,
28.9660450149343));
#154435=CARTESIAN_POINT('Ctrl Pts',(4.64761012012673,-5.24950918980009,
28.9571883816539));
#154436=CARTESIAN_POINT('Ctrl Pts',(4.50356138498687,-5.37704156187942,
28.9484502495472));
#154437=CARTESIAN_POINT('Ctrl Pts',(4.35427862404699,-5.49862546531161,
28.9397121174405));
#154438=CARTESIAN_POINT('Ctrl Pts',(4.20026693293569,-5.61385645119173,
28.9309739853338));
#154439=CARTESIAN_POINT('Ctrl Pts',(4.04312232406658,-5.73143147471801,
28.9220581014665));
#154440=CARTESIAN_POINT('Ctrl Pts',(3.88105456659959,-5.84239216861101,
28.9131422175992));
#154441=CARTESIAN_POINT('Ctrl Pts',(3.71463300634061,-5.94635419317626,
28.9042263337319));
#154442=CARTESIAN_POINT('Ctrl Pts',(3.54821144608166,-6.0503162177415,28.8953104498646));
#154443=CARTESIAN_POINT('Ctrl Pts',(3.37743634273424,-6.14727941791697,
28.8863945659973));
#154444=CARTESIAN_POINT('Ctrl Pts',(3.20290638631692,-6.23690766670393,
28.87747868213));
#154445=CARTESIAN_POINT('Ctrl Pts',(3.03180598764778,-6.32477469775273,
28.8687379976338));
#154446=CARTESIAN_POINT('Ctrl Pts',(2.85707876118365,-6.40560170126986,
28.8599973131376));
#154447=CARTESIAN_POINT('Ctrl Pts',(2.67931053116122,-6.4791142635478,28.8512566286414));
#154448=CARTESIAN_POINT('Ctrl Pts',(2.50157428459663,-6.55261359969453,
28.8425175167395));
#154449=CARTESIAN_POINT('Ctrl Pts',(2.32079838005193,-6.61880101814192,
28.8337784048377));
#154450=CARTESIAN_POINT('Ctrl Pts',(2.13758879097322,-6.67745016628396,
28.8250392929358));
#154451=CARTESIAN_POINT('Ctrl Pts',(1.95200545798299,-6.73685919855116,
28.8161869532615));
#154452=CARTESIAN_POINT('Ctrl Pts',(1.76392520166172,-6.7885331522239,28.8073346135871));
#154453=CARTESIAN_POINT('Ctrl Pts',(1.57399524887777,-6.8322884540255,28.7984822739128));
#154454=CARTESIAN_POINT('Ctrl Pts',(1.38659074026424,-6.87546195411422,
28.789747641263));
#154455=CARTESIAN_POINT('Ctrl Pts',(1.19738569637837,-6.91092602912531,
28.7810130086133));
#154456=CARTESIAN_POINT('Ctrl Pts',(1.00701460402804,-6.93855519180861,
28.7722783759635));
#154457=CARTESIAN_POINT('Ctrl Pts',(0.81279537934934,-6.96674284618735,
28.7633671827769));
#154458=CARTESIAN_POINT('Ctrl Pts',(0.617362747733219,-6.98677540412211,
28.7544559895902));
#154459=CARTESIAN_POINT('Ctrl Pts',(0.421399684115591,-6.99857477410417,
28.7455447964036));
#154460=CARTESIAN_POINT('Ctrl Pts',(0.225436620497963,-7.01037414408624,
28.7366336032169));
#154461=CARTESIAN_POINT('Ctrl Pts',(0.028943426650755,-7.01394029444683,
28.7277224100303));
#154462=CARTESIAN_POINT('Ctrl Pts',(-0.167392073522051,-7.00925149043905,
28.7188112168436));
#154463=CARTESIAN_POINT('Ctrl Pts',(-0.34421720681354,-7.00502862502284,
28.7107855519912));
#154464=CARTESIAN_POINT('Ctrl Pts',(-0.520995680481737,-6.99410746015789,
28.7027598871388));
#154465=CARTESIAN_POINT('Ctrl Pts',(-0.697174942039755,-6.97650153462979,
28.6947342222864));
#154466=CARTESIAN_POINT('Ctrl Pts',(-0.873298288621336,-6.95890119679064,
28.6867111045832));
#154467=CARTESIAN_POINT('Ctrl Pts',(-1.04882243739377,-6.9346203585602,
28.67868798688));
#154468=CARTESIAN_POINT('Ctrl Pts',(-1.22319820765172,-6.90372455326092,
28.6706648691767));
#154469=CARTESIAN_POINT('Ctrl Pts',(-1.39755198759884,-6.8728326441931,
28.6626427632589));
#154470=CARTESIAN_POINT('Ctrl Pts',(-1.57075731675442,-6.83532749421448,
28.654620657341));
#154471=CARTESIAN_POINT('Ctrl Pts',(-1.74227353068216,-6.79132604921781,
28.6465985514231));
#154472=CARTESIAN_POINT('Ctrl Pts',(-1.91385348061453,-6.7473082531355,
28.6385734644636));
#154473=CARTESIAN_POINT('Ctrl Pts',(-2.08374270526097,-6.69678942780656,
28.6305483775041));
#154474=CARTESIAN_POINT('Ctrl Pts',(-2.2514136324211,-6.63993698902696,
28.6225232905446));
#154475=CARTESIAN_POINT('Ctrl Pts',(-2.41911758153125,-6.58307335344406,
28.6144966230843));
#154476=CARTESIAN_POINT('Ctrl Pts',(-2.58460201849207,-6.51987374548824,
28.6064699556241));
#154477=CARTESIAN_POINT('Ctrl Pts',(-2.74735797780886,-6.45055429434324,
28.5984432881638));
#154478=CARTESIAN_POINT('Ctrl Pts',(-2.91024459703649,-6.38117919378703,
28.5904101769232));
#154479=CARTESIAN_POINT('Ctrl Pts',(-3.07039803027066,-6.30567458973652,
28.5823770656826));
#154480=CARTESIAN_POINT('Ctrl Pts',(-3.22733204274069,-6.2243035311912,
28.574343954442));
#154481=CARTESIAN_POINT('Ctrl Pts',(-3.31980326382667,-6.17635674753153,
28.5696105534804));
#154482=CARTESIAN_POINT('Ctrl Pts',(-3.41115718156983,-6.12637399944188,
28.5648771525187));
#154483=CARTESIAN_POINT('Ctrl Pts',(-3.50129888771244,-6.07441624038093,
28.5601437515571));
#154484=CARTESIAN_POINT('Ctrl Pts',(-3.68699360776096,-5.96738163968337,
28.550392798263));
#154485=CARTESIAN_POINT('Ctrl Pts',(-3.86765228366181,-5.85190080475005,
28.5406418449689));
#154486=CARTESIAN_POINT('Ctrl Pts',(-4.04260209639738,-5.72843738315289,
28.5308908916748));
#154487=CARTESIAN_POINT('Ctrl Pts',(-4.21780395715782,-5.60479608933586,
28.5211258903033));
#154488=CARTESIAN_POINT('Ctrl Pts',(-4.38728047139096,-5.47314922691908,
28.5113608889317));
#154489=CARTESIAN_POINT('Ctrl Pts',(-4.55038851875762,-5.33400327060819,
28.5015958875602));
#154490=CARTESIAN_POINT('Ctrl Pts',(-4.71322469880496,-5.19508924177572,
28.4918471624226));
#154491=CARTESIAN_POINT('Ctrl Pts',(-4.86971359804892,-5.04870112494837,
28.4820984372851));
#154492=CARTESIAN_POINT('Ctrl Pts',(-5.01924811634967,-4.89538301964415,
28.4723497121475));
#154493=CARTESIAN_POINT('Ctrl Pts',(-5.16837222038109,-4.74248571308847,
28.4626277434803));
#154494=CARTESIAN_POINT('Ctrl Pts',(-5.31058001982027,-4.58269641722677,
28.4529057748131));
#154495=CARTESIAN_POINT('Ctrl Pts',(-5.44530257865017,-4.41659443343464,
28.4431838061459));
#154496=CARTESIAN_POINT('Ctrl Pts',(-5.57913371349427,-4.2515915030878,
28.4335261652063));
#154497=CARTESIAN_POINT('Ctrl Pts',(-5.70557828425975,-4.0803591655633,
28.4238685242666));
#154498=CARTESIAN_POINT('Ctrl Pts',(-5.82411204843313,-3.90350424744178,
28.414210883327));
#154499=CARTESIAN_POINT('Ctrl Pts',(-5.87621171865758,-3.82577042218146,
28.4099660176416));
#154500=CARTESIAN_POINT('Ctrl Pts',(-5.92678353746462,-3.74695087422018,
28.4057211519561));
#154501=CARTESIAN_POINT('Ctrl Pts',(-5.97578510504653,-3.66709952698369,
28.4014762862707));
#154502=CARTESIAN_POINT('Ctrl Pts',(-6.06642467779386,-3.51939625229324,
28.3936244392568));
#154503=CARTESIAN_POINT('Ctrl Pts',(-6.15165117836221,-3.36822136137917,
28.3857725922429));
#154504=CARTESIAN_POINT('Ctrl Pts',(-6.23118342980562,-3.21402856655256,
28.377920745229));
#154505=CARTESIAN_POINT('Ctrl Pts',(-6.31069312654532,-3.05987949955634,
28.3700711249354));
#154506=CARTESIAN_POINT('Ctrl Pts',(-6.38451161166455,-2.90271456977397,
28.3622215046419));
#154507=CARTESIAN_POINT('Ctrl Pts',(-6.45240311453528,-2.74301305320179,
28.3543718843483));
#154508=CARTESIAN_POINT('Ctrl Pts',(-6.5202891971378,-2.58332428675323,
28.3465228907465));
#154509=CARTESIAN_POINT('Ctrl Pts',(-6.58224909094005,-2.42109968801649,
28.3386738971447));
#154510=CARTESIAN_POINT('Ctrl Pts',(-6.63809483719985,-2.25683927093638,
28.330824903543));
#154511=CARTESIAN_POINT('Ctrl Pts',(-6.69396885652599,-2.09249569361617,
28.3229719362255));
#154512=CARTESIAN_POINT('Ctrl Pts',(-6.74372242056868,-1.92611460024439,
28.3151189689081));
#154513=CARTESIAN_POINT('Ctrl Pts',(-6.78721711244265,-1.75821228270811,
28.3072660015906));
#154514=CARTESIAN_POINT('Ctrl Pts',(-6.83072285050694,-1.59026732362469,
28.2994110398834));
#154515=CARTESIAN_POINT('Ctrl Pts',(-6.86796646777074,-1.42080074331452,
28.2915560781761));
#154516=CARTESIAN_POINT('Ctrl Pts',(-6.89886066458123,-1.25033919125723,
28.2837011164688));
#154517=CARTESIAN_POINT('Ctrl Pts',(-6.92978552646445,-1.07970844186098,
28.2758383580555));
#154518=CARTESIAN_POINT('Ctrl Pts',(-6.95434832651521,-0.908081125695903,
28.2679755996421));
#154519=CARTESIAN_POINT('Ctrl Pts',(-6.97251358096026,-0.735989759320567,
28.2601128412287));
#154520=CARTESIAN_POINT('Ctrl Pts',(-6.98583935096519,-0.609746002312418,
28.2543448344806));
#154521=CARTESIAN_POINT('Ctrl Pts',(-6.99572338168541,-0.483252631113423,
28.2485768277325));
#154522=CARTESIAN_POINT('Ctrl Pts',(-7.00216950191021,-0.356719538319117,
28.2428088209843));
#154523=CARTESIAN_POINT('Ctrl Pts',(-7.01153253248354,-0.172929417276127,
28.2344307545433));
#154524=CARTESIAN_POINT('Ctrl Pts',(-7.01366137701737,0.011351591344907,
28.2260526881023));
#154525=CARTESIAN_POINT('Ctrl Pts',(-7.008522986763,0.195530321215718,28.2176746216613));
#154526=CARTESIAN_POINT('Ctrl Pts',(-7.00338811007882,0.37958311185948,
28.2093022840425));
#154527=CARTESIAN_POINT('Ctrl Pts',(-6.99099591495653,0.563533435637692,
28.2009299464238));
#154528=CARTESIAN_POINT('Ctrl Pts',(-6.97136540613618,0.746787075830669,
28.1925576088051));
#154529=CARTESIAN_POINT('Ctrl Pts',(-6.95174544159739,0.929942283629653,
28.1841897682825));
#154530=CARTESIAN_POINT('Ctrl Pts',(-6.92489495053835,1.11240122786889,
28.1758219277599));
#154531=CARTESIAN_POINT('Ctrl Pts',(-6.89088489724653,1.29357330499653,
28.1674540872373));
#154532=CARTESIAN_POINT('Ctrl Pts',(-6.85688812980253,1.4746746082085,28.1590895155674));
#154533=CARTESIAN_POINT('Ctrl Pts',(-6.81573743799202,1.65448972418672,
28.1507249438975));
#154534=CARTESIAN_POINT('Ctrl Pts',(-6.76755522877617,1.8324362984738,28.1423603722277));
#154535=CARTESIAN_POINT('Ctrl Pts',(-6.71938478897285,2.01033940595693,
28.133997843762));
#154536=CARTESIAN_POINT('Ctrl Pts',(-6.66418634327921,2.18637456510496,
28.1256353152964));
#154537=CARTESIAN_POINT('Ctrl Pts',(-6.60213280590384,2.3599722404529,28.1172727868308));
#154538=CARTESIAN_POINT('Ctrl Pts',(-6.54007431646243,2.5335837694374,28.1089095910093));
#154539=CARTESIAN_POINT('Ctrl Pts',(-6.471159747336,2.70475711447586,28.1005463951878));
#154540=CARTESIAN_POINT('Ctrl Pts',(-6.39561129658887,2.87293973230293,
28.0921831993663));
#154541=CARTESIAN_POINT('Ctrl Pts',(-6.32005769358875,3.04113381984761,
28.0838194331916));
#154542=CARTESIAN_POINT('Ctrl Pts',(-6.23786944137973,3.20633647343993,
28.0754556670168));
#154543=CARTESIAN_POINT('Ctrl Pts',(-6.14931620338209,3.36801674481029,
28.0670919008421));
#154544=CARTESIAN_POINT('Ctrl Pts',(-6.06074512000138,3.5297295982346,28.0587264491886));
#154545=CARTESIAN_POINT('Ctrl Pts',(-5.96580665108505,3.68791836564707,
28.050360997535));
#154546=CARTESIAN_POINT('Ctrl Pts',(-5.86481578643275,3.84207786929276,
28.0419955458814));
#154547=CARTESIAN_POINT('Ctrl Pts',(-5.7637911001383,3.99628900065335,28.0336272926545));
#154548=CARTESIAN_POINT('Ctrl Pts',(-5.65671015643922,4.14646790260694,
28.0252590394276));
#154549=CARTESIAN_POINT('Ctrl Pts',(-5.54393075874577,4.2921391292376,28.0168907862007));
#154550=CARTESIAN_POINT('Ctrl Pts',(-5.4310467984613,4.43794541387715,28.0085147744092));
#154551=CARTESIAN_POINT('Ctrl Pts',(-5.31245402809585,4.57923541154522,
28.0001387626178));
#154552=CARTESIAN_POINT('Ctrl Pts',(-5.18855075561073,4.71556652152754,
27.9917627508263));
#154553=CARTESIAN_POINT('Ctrl Pts',(-5.06458671942991,4.85196448997062,
27.9833826313352));
#154554=CARTESIAN_POINT('Ctrl Pts',(-4.93530721340992,4.98339848229445,
27.975002511844));
#154555=CARTESIAN_POINT('Ctrl Pts',(-4.80114721922023,5.10946297979287,
27.9666223923529));
#154556=CARTESIAN_POINT('Ctrl Pts',(-4.66683393024254,5.23567152194885,
27.9582326975136));
#154557=CARTESIAN_POINT('Ctrl Pts',(-4.5276292540479,5.35649808919911,27.9498430026744));
#154558=CARTESIAN_POINT('Ctrl Pts',(-4.38400205492107,5.47157678781426,
27.9414533078352));
#154559=CARTESIAN_POINT('Ctrl Pts',(-4.29281562473338,5.54463826768128,
27.9361268353606));
#154560=CARTESIAN_POINT('Ctrl Pts',(-4.19984721973464,5.61538375356261,
27.930800362886));
#154561=CARTESIAN_POINT('Ctrl Pts',(-4.10522283754282,5.68372870716196,
27.9254738904114));
#154562=CARTESIAN_POINT('Ctrl Pts',(-3.95632966733273,5.79127072300983,
27.9170925900065));
#154563=CARTESIAN_POINT('Ctrl Pts',(-3.80303460730463,5.89308390277139,
27.9087112896016));
#154564=CARTESIAN_POINT('Ctrl Pts',(-3.64580334336836,5.98880159497575,
27.9003299891967));
#154565=CARTESIAN_POINT('Ctrl Pts',(-3.48877134704259,6.08439797901702,
27.8919593108632));
#154566=CARTESIAN_POINT('Ctrl Pts',(-3.32781336609644,6.17391410190386,
27.8835886325296));
#154567=CARTESIAN_POINT('Ctrl Pts',(-3.16342614885495,6.25702497703507,
27.8752179541961));
#154568=CARTESIAN_POINT('Ctrl Pts',(-2.99922548288099,6.34004153559252,
27.8668567751452));
#154569=CARTESIAN_POINT('Ctrl Pts',(-2.83160362761403,6.41666718708988,
27.8584955960944));
#154570=CARTESIAN_POINT('Ctrl Pts',(-2.661084547777,6.48662127706578,27.8501344170436));
#154571=CARTESIAN_POINT('Ctrl Pts',(-2.49078673655989,6.5564845933584,27.8417840876088));
#154572=CARTESIAN_POINT('Ctrl Pts',(-2.3175995011781,6.619693491938,27.8334337581741));
#154573=CARTESIAN_POINT('Ctrl Pts',(-2.14206945953442,6.67601415464572,
27.8250834287393));
#154574=CARTESIAN_POINT('Ctrl Pts',(-1.96667447775937,6.732291481972,27.8167395243836));
#154575=CARTESIAN_POINT('Ctrl Pts',(-1.78894059273396,6.78169103585329,
27.8083956200279));
#154576=CARTESIAN_POINT('Ctrl Pts',(-1.60943344470827,6.82402744349365,
27.8000517156722));
#154577=CARTESIAN_POINT('Ctrl Pts',(-1.43007047794205,6.86632984626767,
27.7917145131925));
#154578=CARTESIAN_POINT('Ctrl Pts',(-1.24893740670868,6.9015803421214,27.7833773107128));
#154579=CARTESIAN_POINT('Ctrl Pts',(-1.06661419244611,6.92964362193126,
27.775040108233));
#154580=CARTESIAN_POINT('Ctrl Pts',(-1.0065943967124,6.93888189873884,27.772295547197));
#154581=CARTESIAN_POINT('Ctrl Pts',(-0.946445732511336,6.94734171020539,
27.769550986161));
#154582=CARTESIAN_POINT('Ctrl Pts',(-0.886189172523352,6.95501943297087,
27.766806425125));
#154583=CARTESIAN_POINT('Ctrl Pts',(-0.703122413097995,6.97834528872371,
27.7584681148231));
#154584=CARTESIAN_POINT('Ctrl Pts',(-0.519209392208376,6.99442936365961,
27.7501298045212));
#154585=CARTESIAN_POINT('Ctrl Pts',(-0.335045536708833,7.00324003949825,
27.7417914942192));
#154586=CARTESIAN_POINT('Ctrl Pts',(-0.150765811561441,7.01205625871512,
27.7334479377355));
#154587=CARTESIAN_POINT('Ctrl Pts',(0.0337647357046807,7.01358993542549,
27.7251043812517));
#154588=CARTESIAN_POINT('Ctrl Pts',(0.217950683148152,7.00786158983004,
27.7167608247679));
#154589=CARTESIAN_POINT('Ctrl Pts',(0.402276758457761,7.00212888613423,
27.7084109205427));
#154590=CARTESIAN_POINT('Ctrl Pts',(0.586257383878938,6.98912314990432,
27.7000610163175));
#154591=CARTESIAN_POINT('Ctrl Pts',(0.769301819297712,6.96891679339948,
27.6917111120923));
#154592=CARTESIAN_POINT('Ctrl Pts',(0.952620807823779,6.94868012885521,
27.6833486836287));
#154593=CARTESIAN_POINT('Ctrl Pts',(1.13500047432767,6.92122129742725,27.674986255165));
#154594=CARTESIAN_POINT('Ctrl Pts',(1.31585833882374,6.8866641703112,27.6666238267014));
#154595=CARTESIAN_POINT('Ctrl Pts',(1.4968708614489,6.85207749214056,27.6582542472215));
#154596=CARTESIAN_POINT('Ctrl Pts',(1.67635866714702,6.81038048100691,27.6498846677415));
#154597=CARTESIAN_POINT('Ctrl Pts',(1.85375346569482,6.76174715964184,27.6415150882616));
#154598=CARTESIAN_POINT('Ctrl Pts',(2.03142187410601,6.71303882730393,27.633132599725));
#154599=CARTESIAN_POINT('Ctrl Pts',(2.20699051272182,6.65737290494878,27.6247501111885));
#154600=CARTESIAN_POINT('Ctrl Pts',(2.37990879091184,6.59497238124926,27.6163676226519));
#154601=CARTESIAN_POINT('Ctrl Pts',(2.43649048497056,6.57455390740123,27.6136247350475));
#154602=CARTESIAN_POINT('Ctrl Pts',(2.49278858441337,6.55341473033929,27.6108818474431));
#154603=CARTESIAN_POINT('Ctrl Pts',(2.54878435310499,6.53156373955481,27.6081389598386));
#154604=CARTESIAN_POINT('Ctrl Pts',(2.72007692581268,6.46472096705356,27.5997483923835));
#154605=CARTESIAN_POINT('Ctrl Pts',(2.88888454541639,6.3910788444342,27.5913578249283));
#154606=CARTESIAN_POINT('Ctrl Pts',(3.0546504413274,6.31084283149235,27.5829672574732));
#154607=CARTESIAN_POINT('Ctrl Pts',(3.22026085090869,6.23068207892354,27.574584560265));
#154608=CARTESIAN_POINT('Ctrl Pts',(3.38283493013489,6.14393990895742,27.5662018630568));
#154609=CARTESIAN_POINT('Ctrl Pts',(3.54183554505036,6.05086998160742,27.5578191658486));
#154610=CARTESIAN_POINT('Ctrl Pts',(3.70071039710015,5.95787366869457,27.5494430990048));
#154611=CARTESIAN_POINT('Ctrl Pts',(3.85601713748993,5.85855974291226,27.541067032161));
#154612=CARTESIAN_POINT('Ctrl Pts',(4.00724251775276,5.75322813439677,27.5326909653173));
#154613=CARTESIAN_POINT('Ctrl Pts',(4.15835538266826,5.64797489515037,27.5243211304702));
#154614=CARTESIAN_POINT('Ctrl Pts',(4.30539267594718,5.53671309200644,27.5159512956232));
#154615=CARTESIAN_POINT('Ctrl Pts',(4.44786923437015,5.41978651207255,27.5075814607761));
#154616=CARTESIAN_POINT('Ctrl Pts',(4.59028295293201,5.30291150307864,27.4992153174785));
#154617=CARTESIAN_POINT('Ctrl Pts',(4.72813969320088,5.18037690635018,27.4908491741808));
#154618=CARTESIAN_POINT('Ctrl Pts',(4.86098597337318,5.05256785497921,27.4824830308832));
#154619=CARTESIAN_POINT('Ctrl Pts',(4.99379138380543,4.9247981236607,27.4741194614032));
#154620=CARTESIAN_POINT('Ctrl Pts',(5.12158917111287,4.79175740083689,27.4657558919233));
#154621=CARTESIAN_POINT('Ctrl Pts',(5.24396113443014,4.65386916265231,27.4573923224433));
#154622=CARTESIAN_POINT('Ctrl Pts',(5.36631176667809,4.51600496023122,27.4490302108453));
#154623=CARTESIAN_POINT('Ctrl Pts',(5.48323824341888,4.37329517355471,27.4406680992473));
#154624=CARTESIAN_POINT('Ctrl Pts',(5.59436095381705,4.22619830118124,27.4323059876494));
#154625=CARTESIAN_POINT('Ctrl Pts',(5.70550116287917,4.07907826523726,27.4239425592568));
#154626=CARTESIAN_POINT('Ctrl Pts',(5.81083557781614,3.92757002288179,27.4155791308643));
#154627=CARTESIAN_POINT('Ctrl Pts',(5.91002597127305,3.77216377976593,27.4072157024717));
#154628=CARTESIAN_POINT('Ctrl Pts',(6.00922162718179,3.61674929171991,27.3988518303654));
#154629=CARTESIAN_POINT('Ctrl Pts',(6.10227243811671,3.45743666978052,27.3904879582592));
#154630=CARTESIAN_POINT('Ctrl Pts',(6.18888447304698,3.29474362307266,27.3821240861529));
#154631=CARTESIAN_POINT('Ctrl Pts',(6.27553806438576,3.13197251632713,27.3737562010652));
#154632=CARTESIAN_POINT('Ctrl Pts',(6.35574655392168,2.965818035204,27.3653883159775));
#154633=CARTESIAN_POINT('Ctrl Pts',(6.42926236551352,2.7968217672729,27.3570204308899));
#154634=CARTESIAN_POINT('Ctrl Pts',(6.4797184276934,2.68083466166572,27.3512773054158));
#154635=CARTESIAN_POINT('Ctrl Pts',(6.52702289263795,2.56350942008527,27.3455341799418));
#154636=CARTESIAN_POINT('Ctrl Pts',(6.57110895151815,2.44502632087633,27.3397910544677));
#154637=CARTESIAN_POINT('Origin',(0.,0.,50.));
#154638=CARTESIAN_POINT('',(6.57110895151814,2.44502632087636,25.3397663899914));
#154639=CARTESIAN_POINT('',(6.57110895151813,2.4450263208764,25.8869210003222));
#154640=CARTESIAN_POINT('',(6.57110895151814,2.44502632087636,50.));
#154641=CARTESIAN_POINT('',(7.01125,3.98146142790989E-12,27.7735343569105));
#154642=CARTESIAN_POINT('Ctrl Pts',(6.57110895151813,2.4450263208764,25.8869210003222));
#154643=CARTESIAN_POINT('Ctrl Pts',(6.50449838733137,2.62404495591359,25.895592809261));
#154644=CARTESIAN_POINT('Ctrl Pts',(6.43056821795849,2.8003399071602,25.9042646181997));
#154645=CARTESIAN_POINT('Ctrl Pts',(6.3495651145922,2.97332295892218,25.9129364271385));
#154646=CARTESIAN_POINT('Ctrl Pts',(6.26856213015488,3.14630575670998,25.9216082233453));
#154647=CARTESIAN_POINT('Ctrl Pts',(6.18048635294261,3.31597640754702,25.9302800195521));
#154648=CARTESIAN_POINT('Ctrl Pts',(6.08563165071554,3.48176879966337,25.9389518157589));
#154649=CARTESIAN_POINT('Ctrl Pts',(5.99077708581931,3.64756095174514,25.9476235994107));
#154650=CARTESIAN_POINT('Ctrl Pts',(5.88914375658037,3.80947460983848,25.9562953830625));
#154651=CARTESIAN_POINT('Ctrl Pts',(5.78107076500122,3.9669695452005,25.9649671667142));
#154652=CARTESIAN_POINT('Ctrl Pts',(5.67299792768767,4.12446425575102,25.9736389379877));
#154653=CARTESIAN_POINT('Ctrl Pts',(5.55848560711277,4.27754002202627,25.9823107092612));
#154654=CARTESIAN_POINT('Ctrl Pts',(5.43791587524801,4.42568610457471,25.9909824805347));
#154655=CARTESIAN_POINT('Ctrl Pts',(5.3173463130282,4.57383197867751,25.9996542396067));
#154656=CARTESIAN_POINT('Ctrl Pts',(5.19071953583764,4.71704796266913,26.0083259986788));
#154657=CARTESIAN_POINT('Ctrl Pts',(5.05845803451533,4.85485621574392,26.0169977577508));
#154658=CARTESIAN_POINT('Ctrl Pts',(4.92619671659181,4.99266427772857,26.0256695047983));
#154659=CARTESIAN_POINT('Ctrl Pts',(4.78830088681791,5.12506441890887,26.0343412518458));
#154660=CARTESIAN_POINT('Ctrl Pts',(4.64523063400501,5.25161488681352,26.0430129988932));
#154661=CARTESIAN_POINT('Ctrl Pts',(4.49652806262435,5.38314733060852,26.0520261309662));
#154662=CARTESIAN_POINT('Ctrl Pts',(4.34223563524006,5.50835996364229,26.0610392630392));
#154663=CARTESIAN_POINT('Ctrl Pts',(4.18290943344607,5.62680151010216,26.0700523951122));
#154664=CARTESIAN_POINT('Ctrl Pts',(4.02607270355511,5.74339240739859,26.0789246969966));
#154665=CARTESIAN_POINT('Ctrl Pts',(3.86435862820459,5.85342208902587,26.087796998881));
#154666=CARTESIAN_POINT('Ctrl Pts',(3.69833198496527,5.95650628233387,26.0966693007653));
#154667=CARTESIAN_POINT('Ctrl Pts',(3.53489950802656,6.05797978512143,26.1054029729328));
#154668=CARTESIAN_POINT('Ctrl Pts',(3.36728850947157,6.15272311279868,26.1141366451002));
#154669=CARTESIAN_POINT('Ctrl Pts',(3.19606623001045,6.24041562845671,26.1228703172676));
#154670=CARTESIAN_POINT('Ctrl Pts',(3.02603797481171,6.32749661743928,26.1315430848816));
#154671=CARTESIAN_POINT('Ctrl Pts',(2.85244891335412,6.40762471321573,26.1402158524956));
#154672=CARTESIAN_POINT('Ctrl Pts',(2.67587836095206,6.48053250588935,26.1488886201096));
#154673=CARTESIAN_POINT('Ctrl Pts',(2.49930871513515,6.55343992422466,26.1575613431941));
#154674=CARTESIAN_POINT('Ctrl Pts',(2.31975787165042,6.61912700519397,26.1662340662785));
#154675=CARTESIAN_POINT('Ctrl Pts',(2.13782503580156,6.67737453486024,26.174906789363));
#154676=CARTESIAN_POINT('Ctrl Pts',(1.95589311921898,6.73562177021466,26.1835794686261));
#154677=CARTESIAN_POINT('Ctrl Pts',(1.77157950497104,6.78642944284875,26.1922521478892));
#154678=CARTESIAN_POINT('Ctrl Pts',(1.5854992866886,6.82962799678064,26.2009248271524));
#154679=CARTESIAN_POINT('Ctrl Pts',(1.39941999343939,6.87282633596591,26.2095974633023));
#154680=CARTESIAN_POINT('Ctrl Pts',(1.21157439050707,6.90841556788906,26.2182700994522));
#154681=CARTESIAN_POINT('Ctrl Pts',(1.02258935229166,6.93627692491294,26.2269427356021));
#154682=CARTESIAN_POINT('Ctrl Pts',(0.833605238124551,6.96413814570784,
26.2356153293469));
#154683=CARTESIAN_POINT('Ctrl Pts',(0.643481980915828,6.98427152577621,
26.2442879230917));
#154684=CARTESIAN_POINT('Ctrl Pts',(0.452854049807141,6.99660987708142,
26.2529605168364));
#154685=CARTESIAN_POINT('Ctrl Pts',(0.262227035220992,7.00894816906491,
26.2616330688842));
#154686=CARTESIAN_POINT('Ctrl Pts',(0.0710956351212699,7.01349148893088,
26.2703056209319));
#154687=CARTESIAN_POINT('Ctrl Pts',(-0.11990232315709,7.01022467510147,
26.2789781729796));
#154688=CARTESIAN_POINT('Ctrl Pts',(-0.31089937872256,7.006957876712,26.2876506840382));
#154689=CARTESIAN_POINT('Ctrl Pts',(-0.501762709652909,6.99588102335283,
26.2963231950969));
#154690=CARTESIAN_POINT('Ctrl Pts',(-0.691855389205306,6.97703107940101,
26.3049957061555));
#154691=CARTESIAN_POINT('Ctrl Pts',(-0.881947185837381,6.95818122300121,
26.3136681769331));
#154692=CARTESIAN_POINT('Ctrl Pts',(-1.0712680555302,6.93155837629127,26.3223406477107));
#154693=CARTESIAN_POINT('Ctrl Pts',(-1.25918622472477,6.89725138109112,
26.3310131184883));
#154694=CARTESIAN_POINT('Ctrl Pts',(-1.44710353643495,6.86294454243631,
26.3396855496928));
#154695=CARTESIAN_POINT('Ctrl Pts',(-1.63361788097034,6.8209536764805,26.3483579808972));
#154696=CARTESIAN_POINT('Ctrl Pts',(-1.81810685596641,6.77141890764321,
26.3570304121017));
#154697=CARTESIAN_POINT('Ctrl Pts',(-2.0025950041816,6.72188436079425,26.365702804441));
#154698=CARTESIAN_POINT('Ctrl Pts',(-2.18505752664097,6.6648060523869,26.3743751967802));
#154699=CARTESIAN_POINT('Ctrl Pts',(-2.36488554744894,6.60037445225399,
26.3830475891195));
#154700=CARTESIAN_POINT('Ctrl Pts',(-2.54471277703887,6.53594313561107,
26.3917199433015));
#154701=CARTESIAN_POINT('Ctrl Pts',(-2.72190526072999,6.46415868780901,
26.4003922974834));
#154702=CARTESIAN_POINT('Ctrl Pts',(-2.89587171389957,6.38526065083771,
26.4090646516654));
#154703=CARTESIAN_POINT('Ctrl Pts',(-3.06983741583694,6.30636295456856,
26.4177369683979));
#154704=CARTESIAN_POINT('Ctrl Pts',(-3.24057685640863,6.22035184793722,
26.4264092851304));
#154705=CARTESIAN_POINT('Ctrl Pts',(-3.40752028946867,6.12751434428018,
26.4350816018629));
#154706=CARTESIAN_POINT('Ctrl Pts',(-3.57446301524634,6.03467723394397,
26.4437538818537));
#154707=CARTESIAN_POINT('Ctrl Pts',(-3.73760951742251,5.93501392252102,
26.4524261618445));
#154708=CARTESIAN_POINT('Ctrl Pts',(-3.89641539158944,5.82885697703117,
26.4610984418354));
#154709=CARTESIAN_POINT('Ctrl Pts',(-4.05522060590818,5.72270047262997,
26.4697706857924));
#154710=CARTESIAN_POINT('Ctrl Pts',(-4.20968499214218,5.61005054602491,
26.4784429297494));
#154711=CARTESIAN_POINT('Ctrl Pts',(-4.35929312156039,5.49128309621862,
26.4871151737063));
#154712=CARTESIAN_POINT('Ctrl Pts',(-4.50890064155473,5.37251613020767,
26.4957873823372));
#154713=CARTESIAN_POINT('Ctrl Pts',(-4.65365172183414,5.24763186748313,
26.5044595909681));
#154714=CARTESIAN_POINT('Ctrl Pts',(-4.79306334971054,5.1170470281366,26.513131799599));
#154715=CARTESIAN_POINT('Ctrl Pts',(-4.93247442107311,4.98646271006846,
26.5218039736115));
#154716=CARTESIAN_POINT('Ctrl Pts',(-5.06654587536718,4.85017805510722,
26.530476147624));
#154717=CARTESIAN_POINT('Ctrl Pts',(-5.19483033978618,4.70864782111988,
26.5391483216365));
#154718=CARTESIAN_POINT('Ctrl Pts',(-5.32311430257632,4.56711814055615,
26.5478204617383));
#154719=CARTESIAN_POINT('Ctrl Pts',(-5.44561113000617,4.42034313247767,
26.5564926018402));
#154720=CARTESIAN_POINT('Ctrl Pts',(-5.56191207495191,4.26881255538401,
26.565164741942));
#154721=CARTESIAN_POINT('Ctrl Pts',(-5.6782125746164,4.11728255845523,26.5738368488408));
#154722=CARTESIAN_POINT('Ctrl Pts',(-5.78831706632251,3.96099725427966,
26.5825089557396));
#154723=CARTESIAN_POINT('Ctrl Pts',(-5.89185815647341,3.80047813130109,
26.5911810626385));
#154724=CARTESIAN_POINT('Ctrl Pts',(-5.99539885864402,3.63995960980598,
26.5998531370419));
#154725=CARTESIAN_POINT('Ctrl Pts',(-6.09237605450623,3.47520753995039,
26.6085252114454));
#154726=CARTESIAN_POINT('Ctrl Pts',(-6.18246615568043,3.30677165772994,
26.6171972858488));
#154727=CARTESIAN_POINT('Ctrl Pts',(-6.2725559266266,3.13833639291638,26.6258693284645));
#154728=CARTESIAN_POINT('Ctrl Pts',(-6.3557585194383,2.96621759322364,26.6345413710802));
#154729=CARTESIAN_POINT('Ctrl Pts',(-6.43179631013632,2.79098957135581,
26.6432134136959));
#154730=CARTESIAN_POINT('Ctrl Pts',(-6.50783382831866,2.61576217749653,
26.6518854252314));
#154731=CARTESIAN_POINT('Ctrl Pts',(-6.57670648270564,2.43742584432176,
26.6605574367669));
#154732=CARTESIAN_POINT('Ctrl Pts',(-6.63818446599434,2.25657562645958,
26.6692294483025));
#154733=CARTESIAN_POINT('Ctrl Pts',(-6.69966223396433,2.07572604200197,
26.6779014294654));
#154734=CARTESIAN_POINT('Ctrl Pts',(-6.75374529124721,1.89236285939279,
26.6865734106283));
#154735=CARTESIAN_POINT('Ctrl Pts',(-6.80025318023369,1.70709790206118,
26.6952453917912));
#154736=CARTESIAN_POINT('Ctrl Pts',(-6.8467609101261,1.52183357848343,26.703917343289));
#154737=CARTESIAN_POINT('Ctrl Pts',(-6.88569345442265,1.33466776867936,
26.7125892947869));
#154738=CARTESIAN_POINT('Ctrl Pts',(-6.91692090874659,1.14622497994254,
26.7212612462847));
#154739=CARTESIAN_POINT('Ctrl Pts',(-6.94814825879519,0.957782820457667,
26.729933168825));
#154740=CARTESIAN_POINT('Ctrl Pts',(-6.97167052392495,0.76806397077221,
26.7386050913653));
#154741=CARTESIAN_POINT('Ctrl Pts',(-6.98740921903147,0.577701452563602,
26.7472770139055));
#154742=CARTESIAN_POINT('Ctrl Pts',(-7.00314786286679,0.387339554489842,
26.7559489081957));
#154743=CARTESIAN_POINT('Ctrl Pts',(-7.01110296401741,0.196334275138949,
26.7646208024859));
#154744=CARTESIAN_POINT('Ctrl Pts',(-7.01124797942392,0.00532292438054067,
26.773292696776));
#154745=CARTESIAN_POINT('Ctrl Pts',(-7.01139299436986,-0.185687819710631,
26.7819645635236));
#154746=CARTESIAN_POINT('Ctrl Pts',(-7.00372797299446,-0.376704351159606,
26.7906364302711));
#154747=CARTESIAN_POINT('Ctrl Pts',(-6.98827849031214,-0.567089326597393,
26.7993082970187));
#154748=CARTESIAN_POINT('Ctrl Pts',(-6.97282905543841,-0.757473712886903,
26.807980136931));
#154749=CARTESIAN_POINT('Ctrl Pts',(-6.94959523043391,-0.947226263999834,
26.8166519768434));
#154750=CARTESIAN_POINT('Ctrl Pts',(-6.91865453650915,-1.13571385786268,
26.8253238167557));
#154751=CARTESIAN_POINT('Ctrl Pts',(-6.88771393580715,-1.3242008838219,
26.8339956305403));
#154752=CARTESIAN_POINT('Ctrl Pts',(-6.84906655865545,-1.51142267990603,
26.8426674443248));
#154753=CARTESIAN_POINT('Ctrl Pts',(-6.8028413538356,-1.69675457183538,
26.8513392581094));
#154754=CARTESIAN_POINT('Ctrl Pts',(-6.7566162845193,-1.88208592048689,
26.8600110464736));
#154755=CARTESIAN_POINT('Ctrl Pts',(-6.70281350071529,-2.06552710051335,
26.8686828348377));
#154756=CARTESIAN_POINT('Ctrl Pts',(-6.64161251687691,-2.24646605542217,
26.8773546232019));
#154757=CARTESIAN_POINT('Ctrl Pts',(-6.58041170745033,-2.42740449468745,
26.8860263868531));
#154758=CARTESIAN_POINT('Ctrl Pts',(-6.51181283117406,-2.60584045408293,
26.8946981505042));
#154759=CARTESIAN_POINT('Ctrl Pts',(-6.43604476876361,-2.78117858056086,
26.9033699141553));
#154760=CARTESIAN_POINT('Ctrl Pts',(-6.35684774728392,-2.96445180845019,
26.9124341271007));
#154761=CARTESIAN_POINT('Ctrl Pts',(-6.26981768815816,-3.14433998861945,
26.9214983400461));
#154762=CARTESIAN_POINT('Ctrl Pts',(-6.17527181578263,-3.32018742900167,
26.9305625529914));
#154763=CARTESIAN_POINT('Ctrl Pts',(-6.08368050191884,-3.49053963687194,
26.9393435092823));
#154764=CARTESIAN_POINT('Ctrl Pts',(-5.98503618716775,-3.65709956718355,
26.9481244655731));
#154765=CARTESIAN_POINT('Ctrl Pts',(-5.87967633130269,-3.81929742251359,
26.9569054218639));
#154766=CARTESIAN_POINT('Ctrl Pts',(-5.77561495477872,-3.97949631379242,
26.9655781596094));
#154767=CARTESIAN_POINT('Ctrl Pts',(-5.66500279405408,-4.13543980257367,
26.9742508973549));
#154768=CARTESIAN_POINT('Ctrl Pts',(-5.54820899034767,-4.28660746534194,
26.9829236351004));
#154769=CARTESIAN_POINT('Ctrl Pts',(-5.4314163636855,-4.43777360464733,
26.9915962854423));
#154770=CARTESIAN_POINT('Ctrl Pts',(-5.30844239242882,-4.58416378940367,
27.0002689357842));
#154771=CARTESIAN_POINT('Ctrl Pts',(-5.17969746407295,-4.72528948776435,
27.0089415861261));
#154772=CARTESIAN_POINT('Ctrl Pts',(-5.05095379117012,-4.86641380994122,
27.0176141518969));
#154773=CARTESIAN_POINT('Ctrl Pts',(-4.91643946527151,-5.00227353854657,
27.0262867176676));
#154774=CARTESIAN_POINT('Ctrl Pts',(-4.77660337748139,-5.13241529269928,
27.0349592834384));
#154775=CARTESIAN_POINT('Ctrl Pts',(-4.63676860764736,-5.26255582026506,
27.0436317674702));
#154776=CARTESIAN_POINT('Ctrl Pts',(-4.49161238427182,-5.3869782876605,
27.052304251502));
#154777=CARTESIAN_POINT('Ctrl Pts',(-4.34161910267806,-5.50526748939241,
27.0609767355338));
#154778=CARTESIAN_POINT('Ctrl Pts',(-4.19162718580731,-5.62355561486281,
27.0696491406584));
#154779=CARTESIAN_POINT('Ctrl Pts',(-4.03679852186557,-5.73571041041281,
27.0783215457831));
#154780=CARTESIAN_POINT('Ctrl Pts',(-3.8776497743179,-5.84135761533501,
27.0869939509077));
#154781=CARTESIAN_POINT('Ctrl Pts',(-3.71850242284481,-5.94700389350549,
27.0956662799569));
#154782=CARTESIAN_POINT('Ctrl Pts',(-3.55503530028666,-6.04614253816331,
27.104338609006));
#154783=CARTESIAN_POINT('Ctrl Pts',(-3.38779388709622,-6.13844272931282,
27.1130109380551));
#154784=CARTESIAN_POINT('Ctrl Pts',(-3.22055388638227,-6.23074214091948,
27.1216831938601));
#154785=CARTESIAN_POINT('Ctrl Pts',(-3.04953990753783,-6.31620307732865,
27.130355449665));
#154786=CARTESIAN_POINT('Ctrl Pts',(-2.87532260481446,-6.39454036508825,
27.13902770547));
#154787=CARTESIAN_POINT('Ctrl Pts',(-2.70110671662283,-6.47287701679978,
27.1476998908618));
#154788=CARTESIAN_POINT('Ctrl Pts',(-2.52368781567789,-6.54409001910875,
27.1563720762537));
#154789=CARTESIAN_POINT('Ctrl Pts',(-2.34365791912572,-6.60794174615813,
27.1650442616455));
#154790=CARTESIAN_POINT('Ctrl Pts',(-2.16362942554482,-6.6717929756116,
27.1737163794551));
#154791=CARTESIAN_POINT('Ctrl Pts',(-1.9809902447887,-6.72828294965036,
27.1823884972647));
#154792=CARTESIAN_POINT('Ctrl Pts',(-1.79634980371343,-6.77722317363083,
27.1910606150743));
#154793=CARTESIAN_POINT('Ctrl Pts',(-1.61171074128322,-6.82616303219191,
27.1997326681322));
#154794=CARTESIAN_POINT('Ctrl Pts',(-1.42507072299827,-6.86755318072487,
27.2084047211902));
#154795=CARTESIAN_POINT('Ctrl Pts',(-1.23705251634051,-6.90125551144975,
27.2170767742481));
#154796=CARTESIAN_POINT('Ctrl Pts',(-1.04903565219333,-6.93495760152914,
27.2257487653848));
#154797=CARTESIAN_POINT('Ctrl Pts',(-0.859640898942888,-6.96097193353372,
27.2344207565215));
#154798=CARTESIAN_POINT('Ctrl Pts',(-0.669500206864174,-6.97921170588118,
27.2430927476582));
#154799=CARTESIAN_POINT('Ctrl Pts',(-0.479360810406287,-6.99745135394262,
27.2517646797038));
#154800=CARTESIAN_POINT('Ctrl Pts',(-0.288475768017,-7.00791652123609,27.2604366117495));
#154801=CARTESIAN_POINT('Ctrl Pts',(-0.0974819939226111,-7.01057228929,
27.2691085437951));
#154802=CARTESIAN_POINT('Ctrl Pts',(0.0935105410567989,-7.01322804011402,
27.2777804195797));
#154803=CARTESIAN_POINT('Ctrl Pts',(0.284611522343041,-7.00807448913608,
27.2864522953642));
#154804=CARTESIAN_POINT('Ctrl Pts',(0.475183323465242,-6.99512883166569,
27.2951241711487));
#154805=CARTESIAN_POINT('Ctrl Pts',(0.665753950389365,-6.98218325395928,
27.303795993502));
#154806=CARTESIAN_POINT('Ctrl Pts',(0.855795120321891,-6.96144568508307,
27.3124678158552));
#154807=CARTESIAN_POINT('Ctrl Pts',(1.04467275075859,-6.93298531704218,
27.3211396382084));
#154808=CARTESIAN_POINT('Ctrl Pts',(1.23354927905871,-6.90452511507291,
27.32981140996));
#154809=CARTESIAN_POINT('Ctrl Pts',(1.42126200062285,-6.86834224643213,
27.3384831817115));
#154810=CARTESIAN_POINT('Ctrl Pts',(1.60718460924098,-6.82455743578431,
27.347154953463));
#154811=CARTESIAN_POINT('Ctrl Pts',(1.7976338940525,-6.7797065920087,27.3560378577015));
#154812=CARTESIAN_POINT('Ctrl Pts',(1.98620448431277,-6.72687898191044,
27.36492076194));
#154813=CARTESIAN_POINT('Ctrl Pts',(2.17223623427263,-6.66625954377814,
27.3738036661785));
#154814=CARTESIAN_POINT('Ctrl Pts',(2.35386532185444,-6.60707473666823,
27.3824763459348));
#154815=CARTESIAN_POINT('Ctrl Pts',(2.5330741022709,-6.5404628369675,27.3911490256911));
#154816=CARTESIAN_POINT('Ctrl Pts',(2.70926451773662,-6.46664614274149,
27.3998217054475));
#154817=CARTESIAN_POINT('Ctrl Pts',(2.88545151535583,-6.39283088045563,
27.408494216966));
#154818=CARTESIAN_POINT('Ctrl Pts',(3.05862000313812,-6.31181121311306,
27.4171667284846));
#154819=CARTESIAN_POINT('Ctrl Pts',(3.22819210343652,-6.22385751008248,
27.4258392400031));
#154820=CARTESIAN_POINT('Ctrl Pts',(3.39776113570525,-6.13590539837837,
27.4345115946118));
#154821=CARTESIAN_POINT('Ctrl Pts',(3.56373365850634,-6.04101963284236,
27.4431839492206));
#154822=CARTESIAN_POINT('Ctrl Pts',(3.72555582774813,-5.93951684371986,
27.4518563038293));
#154823=CARTESIAN_POINT('Ctrl Pts',(3.8873752804605,-5.83801575853765,27.4605285128542));
#154824=CARTESIAN_POINT('Ctrl Pts',(4.04504427838494,-5.72989802299959,
27.469200721879));
#154825=CARTESIAN_POINT('Ctrl Pts',(4.19803670362804,-5.61552440983848,
27.4778729309038));
#154826=CARTESIAN_POINT('Ctrl Pts',(4.35102676029652,-5.5011525673692,27.4865450056686));
#154827=CARTESIAN_POINT('Ctrl Pts',(4.49934016166036,-5.38052521116288,
27.4952170804333));
#154828=CARTESIAN_POINT('Ctrl Pts',(4.64248202336259,-5.25404484423717,
27.5038891551981));
#154829=CARTESIAN_POINT('Ctrl Pts',(4.7856218558408,-5.12756627033689,27.5125611070247));
#154830=CARTESIAN_POINT('Ctrl Pts',(4.92359008252016,-4.99523503982615,
27.5212330588514));
#154831=CARTESIAN_POINT('Ctrl Pts',(5.05592635131787,-4.85749269608814,
27.5299050106781));
#154832=CARTESIAN_POINT('Ctrl Pts',(5.18826091679903,-4.71975212524894,
27.5385768508871));
#154833=CARTESIAN_POINT('Ctrl Pts',(5.31496347269061,-4.57660078535814,
27.547248691096));
#154834=CARTESIAN_POINT('Ctrl Pts',(5.43561126741474,-4.42851631046493,
27.5559205313049));
#154835=CARTESIAN_POINT('Ctrl Pts',(5.56176013705229,-4.27367975368109,
27.5649877740385));
#154836=CARTESIAN_POINT('Ctrl Pts',(5.68128895686198,-4.11344992041542,
27.574055016772));
#154837=CARTESIAN_POINT('Ctrl Pts',(5.79376175353724,-3.94841123817531,
27.5831222595056));
#154838=CARTESIAN_POINT('Ctrl Pts',(5.90133874236041,-3.79055649463233,
27.591794815884));
#154839=CARTESIAN_POINT('Ctrl Pts',(6.00246078173934,-3.62830291662156,
27.6004673722625));
#154840=CARTESIAN_POINT('Ctrl Pts',(6.09679041553024,-3.46219196342413,
27.6091399286409));
#154841=CARTESIAN_POINT('Ctrl Pts',(6.19111669178468,-3.29608692272269,
27.6178121763313));
#154842=CARTESIAN_POINT('Ctrl Pts',(6.27865090596041,-3.12612502861305,
27.6264844240218));
#154843=CARTESIAN_POINT('Ctrl Pts',(6.35910096685864,-2.95287342359905,
27.6351566717122));
#154844=CARTESIAN_POINT('Ctrl Pts',(6.43954858436819,-2.77962708049541,
27.6438286560135));
#154845=CARTESIAN_POINT('Ctrl Pts',(6.51291235951768,-2.60309148404424,
27.6525006403149));
#154846=CARTESIAN_POINT('Ctrl Pts',(6.57894750102292,-2.42385567666153,
27.6611726246162));
#154847=CARTESIAN_POINT('Ctrl Pts',(6.64498098170959,-2.24462437715371,
27.6698443908125));
#154848=CARTESIAN_POINT('Ctrl Pts',(6.70368609940726,-2.06269326910442,
27.6785161570089));
#154849=CARTESIAN_POINT('Ctrl Pts',(6.7548669838925,-1.87866936750964,27.6871879232052));
#154850=CARTESIAN_POINT('Ctrl Pts',(6.80605126222379,-1.69463326314033,
27.6958602644334));
#154851=CARTESIAN_POINT('Ctrl Pts',(6.84971023276513,-1.50850436118443,
27.7045326056616));
#154852=CARTESIAN_POINT('Ctrl Pts',(6.88569820761627,-1.32090376490116,
27.7132049468899));
#154853=CARTESIAN_POINT('Ctrl Pts',(6.92168406448144,-1.1333142094012,27.7218767777282));
#154854=CARTESIAN_POINT('Ctrl Pts',(6.94999977553719,-0.944253411833958,
27.7305486085666));
#154855=CARTESIAN_POINT('Ctrl Pts',(6.97055086371791,-0.754352184872193,
27.7392204394049));
#154856=CARTESIAN_POINT('Ctrl Pts',(6.99110229107969,-0.564447823726136,
27.7478924133657));
#154857=CARTESIAN_POINT('Ctrl Pts',(7.00388880856458,-0.373703287800228,
27.7565643873264));
#154858=CARTESIAN_POINT('Ctrl Pts',(7.00886775178444,-0.18275502864788,
27.7652363612872));
#154859=CARTESIAN_POINT('Ctrl Pts',(7.01045582731889,-0.121850486194973,
27.7680023598283));
#154860=CARTESIAN_POINT('Ctrl Pts',(7.01125000000004,-0.0609252433299691,
27.7707683583694));
#154861=CARTESIAN_POINT('Ctrl Pts',(7.01125,3.98146195391879E-12,27.7735343569105));
#154862=CARTESIAN_POINT('Ctrl Pts',(7.01124849188977,0.0045986382217964,
27.7735343569106));
#154863=CARTESIAN_POINT('Ctrl Pts',(7.01110746258416,0.219616967251206,
27.7832889411837));
#154864=CARTESIAN_POINT('Ctrl Pts',(7.00107121144239,0.43435405131007,27.7930435254568));
#154865=CARTESIAN_POINT('Ctrl Pts',(6.98124137501422,0.647993384448971,
27.8027981097299));
#154866=CARTESIAN_POINT('Ctrl Pts',(6.96133438247261,0.862463969054885,
27.8125906482147));
#154867=CARTESIAN_POINT('Ctrl Pts',(6.93155750156275,1.07582822248848,27.8223831866996));
#154868=CARTESIAN_POINT('Ctrl Pts',(6.89206436059057,1.2872744120728,27.8321757251844));
#154869=CARTESIAN_POINT('Ctrl Pts',(6.85246177079178,1.49930659043311,27.8419954020994));
#154870=CARTESIAN_POINT('Ctrl Pts',(6.80308901990283,1.70941004109375,27.8518150790144));
#154871=CARTESIAN_POINT('Ctrl Pts',(6.74415134707051,1.91678093957212,27.8616347559293));
#154872=CARTESIAN_POINT('Ctrl Pts',(6.69348504934856,2.09504918764271,27.8700763290386));
#154873=CARTESIAN_POINT('Ctrl Pts',(6.63575095573061,2.2712982718579,27.878517902148));
#154874=CARTESIAN_POINT('Ctrl Pts',(6.57110895151814,2.44502632087635,27.8869594752573));
#154875=CARTESIAN_POINT('',(7.01124919374723,0.00336239182502676,27.2264656430545));
#154876=CARTESIAN_POINT('Ctrl Pts',(6.57110895151815,2.44502632087633,27.3397910544677));
#154877=CARTESIAN_POINT('Ctrl Pts',(6.63541756143711,2.27219428275467,27.3314135214061));
#154878=CARTESIAN_POINT('Ctrl Pts',(6.69287570619621,2.09689805609267,27.3230359883445));
#154879=CARTESIAN_POINT('Ctrl Pts',(6.7433182271924,1.91970983466637,27.3146584552828));
#154880=CARTESIAN_POINT('Ctrl Pts',(6.7911953837239,1.75153290684378,27.3067069799438));
#154881=CARTESIAN_POINT('Ctrl Pts',(6.83275269263724,1.58165188370494,27.2987555046048));
#154882=CARTESIAN_POINT('Ctrl Pts',(6.867891461695,1.41056493394559,27.2908040292657));
#154883=CARTESIAN_POINT('Ctrl Pts',(6.90680224734355,1.22111243438856,27.281998992527));
#154884=CARTESIAN_POINT('Ctrl Pts',(6.93790954720012,1.02985490892179,27.2731939557883));
#154885=CARTESIAN_POINT('Ctrl Pts',(6.96105872276864,0.837429412348653,
27.2643889190496));
#154886=CARTESIAN_POINT('Ctrl Pts',(6.98414320400172,0.64554168177873,27.2556084894939));
#154887=CARTESIAN_POINT('Ctrl Pts',(6.99931389611967,0.452492746196682,
27.2468280599383));
#154888=CARTESIAN_POINT('Ctrl Pts',(7.00646718374326,0.258928881411138,
27.2380476303826));
#154889=CARTESIAN_POINT('Ctrl Pts',(7.00961240899805,0.173820887999565,
27.2341869679516));
#154890=CARTESIAN_POINT('Ctrl Pts',(7.01120830977233,0.0886135121272676,
27.2303263055206));
#154891=CARTESIAN_POINT('Ctrl Pts',(7.01124919374686,0.00336239260024742,
27.2264656430896));
#154892=CARTESIAN_POINT('Ctrl Pts',(7.01124919374723,0.00336239182502279,
27.2264656430545));
#154893=CARTESIAN_POINT('Ctrl Pts',(7.01133243824318,-0.170218777617792,
27.2186048864649));
#154894=CARTESIAN_POINT('Ctrl Pts',(7.00496446246311,-0.343967021434672,
27.2107441298753));
#154895=CARTESIAN_POINT('Ctrl Pts',(6.99213931214691,-0.517314606433853,
27.2028833732857));
#154896=CARTESIAN_POINT('Ctrl Pts',(6.97984637489577,-0.683468681239413,
27.1953488192945));
#154897=CARTESIAN_POINT('Ctrl Pts',(6.96162145168017,-0.849254241412167,
27.1878142653033));
#154898=CARTESIAN_POINT('Ctrl Pts',(6.93751249916856,-1.01417300613852,
27.1802797113122));
#154899=CARTESIAN_POINT('Ctrl Pts',(6.91340523989964,-1.17908018813461,
27.1727456864949));
#154900=CARTESIAN_POINT('Ctrl Pts',(6.88341483877647,-1.34312029690605,
27.1652116616776));
#154901=CARTESIAN_POINT('Ctrl Pts',(6.84764077591788,-1.50580289762199,
27.1576776368603));
#154902=CARTESIAN_POINT('Ctrl Pts',(6.81185484725471,-1.66853945810081,
27.1501411131022));
#154903=CARTESIAN_POINT('Ctrl Pts',(6.77028152667223,-1.82991722014581,
27.1426045893441));
#154904=CARTESIAN_POINT('Ctrl Pts',(6.72307070525454,-1.98945893515002,
27.135068065586));
#154905=CARTESIAN_POINT('Ctrl Pts',(6.71694946583952,-2.01014472296088,
27.1340908983838));
#154906=CARTESIAN_POINT('Ctrl Pts',(6.71073352178257,-2.03079966839598,
27.1331137311815));
#154907=CARTESIAN_POINT('Ctrl Pts',(6.70442326004343,-2.05142275328336,
27.1321365639793));
#154908=CARTESIAN_POINT('Ctrl Pts',(6.64207211118979,-2.25519766608262,
27.1224812596194));
#154909=CARTESIAN_POINT('Ctrl Pts',(6.57051491078361,-2.45584014003303,
27.1128259552595));
#154910=CARTESIAN_POINT('Ctrl Pts',(6.49008777157213,-2.65261894734052,
27.1031706508996));
#154911=CARTESIAN_POINT('Ctrl Pts',(6.40921508109799,-2.85048787232372,
27.093461857965));
#154912=CARTESIAN_POINT('Ctrl Pts',(6.31937397250988,-3.04445018114414,
27.0837530650303));
#154913=CARTESIAN_POINT('Ctrl Pts',(6.22094965134369,-3.23379220079876,
27.0740442720957));
#154914=CARTESIAN_POINT('Ctrl Pts',(6.12205170398593,-3.42404535033072,
27.064288759625));
#154915=CARTESIAN_POINT('Ctrl Pts',(6.01448778024528,-3.6096336099399,27.0545332471543));
#154916=CARTESIAN_POINT('Ctrl Pts',(5.89869161118943,-3.78986330077795,
27.0447777346835));
#154917=CARTESIAN_POINT('Ctrl Pts',(5.78278078611118,-3.97027144673792,
27.0350125627546));
#154918=CARTESIAN_POINT('Ctrl Pts',(5.65862144160521,-4.14531038488499,
27.0252473908257));
#154919=CARTESIAN_POINT('Ctrl Pts',(5.52669089582952,-4.31431504464557,
27.0154822188968));
#154920=CARTESIAN_POINT('Ctrl Pts',(5.39494023436033,-4.48308927038622,
27.0057303615582));
#154921=CARTESIAN_POINT('Ctrl Pts',(5.25543957231355,-4.64584563187324,
26.9959785042197));
#154922=CARTESIAN_POINT('Ctrl Pts',(5.10870597069337,-4.80195271400104,
26.9862266468812));
#154923=CARTESIAN_POINT('Ctrl Pts',(5.0447194934325,-4.87002670762308,26.9819741308184));
#154924=CARTESIAN_POINT('Ctrl Pts',(4.9793581400238,-4.93683667999793,26.9777216147556));
#154925=CARTESIAN_POINT('Ctrl Pts',(4.91266726452488,-5.00233214716553,
26.9734690986928));
#154926=CARTESIAN_POINT('Ctrl Pts',(4.78668753017544,-5.12605374315805,
26.965436053094));
#154927=CARTESIAN_POINT('Ctrl Pts',(4.6558994660757,-5.24514239954555,26.9574030074952));
#154928=CARTESIAN_POINT('Ctrl Pts',(4.5206854613145,-5.35920045551197,26.9493699618964));
#154929=CARTESIAN_POINT('Ctrl Pts',(4.38555837732173,-5.47318519056842,
26.9413420802486));
#154930=CARTESIAN_POINT('Ctrl Pts',(4.2460112950641,-5.58214552691869,26.9333141986008));
#154931=CARTESIAN_POINT('Ctrl Pts',(4.10246291679174,-5.68572111335481,
26.925286316953));
#154932=CARTESIAN_POINT('Ctrl Pts',(3.95897935202721,-5.78924993439265,
26.9172620599729));
#154933=CARTESIAN_POINT('Ctrl Pts',(3.81149838509464,-5.88739863240532,
26.9092378029927));
#154934=CARTESIAN_POINT('Ctrl Pts',(3.66047116581132,-5.97984760731943,
26.9012135460126));
#154935=CARTESIAN_POINT('Ctrl Pts',(3.50946220725726,-6.07228540421074,
26.8931902592469));
#154936=CARTESIAN_POINT('Ctrl Pts',(3.35490815884217,-6.15902465283727,
26.8851669724813));
#154937=CARTESIAN_POINT('Ctrl Pts',(3.19728862275171,-6.23978942155282,
26.8771436857156));
#154938=CARTESIAN_POINT('Ctrl Pts',(3.03968200217577,-6.32054757231625,
26.8691210563866));
#154939=CARTESIAN_POINT('Ctrl Pts',(2.87901072240415,-6.39533205469342,
26.8610984270577));
#154940=CARTESIAN_POINT('Ctrl Pts',(2.71577814400141,-6.46391333752737,
26.8530757977287));
#154941=CARTESIAN_POINT('Ctrl Pts',(2.55248420177032,-6.53252040204112,
26.8450501524623));
#154942=CARTESIAN_POINT('Ctrl Pts',(2.38662737676646,-6.59491946921344,
26.8370245071959));
#154943=CARTESIAN_POINT('Ctrl Pts',(2.21873047899309,-6.65092938047662,
26.8289988619295));
#154944=CARTESIAN_POINT('Ctrl Pts',(2.11972823693536,-6.68395623723245,
26.8242664524218));
#154945=CARTESIAN_POINT('Ctrl Pts',(2.02001699361798,-6.71476251525415,
26.8195340429141));
#154946=CARTESIAN_POINT('Ctrl Pts',(1.91970626837255,-6.74331924245554,
26.8148016334064));
#154947=CARTESIAN_POINT('Ctrl Pts',(1.73465940617455,-6.79599888115151,
26.8060715845718));
#154948=CARTESIAN_POINT('Ctrl Pts',(1.54747933220458,-6.84104703880416,
26.7973415357371));
#154949=CARTESIAN_POINT('Ctrl Pts',(1.35879712463937,-6.87832079337478,
26.7886114869024));
#154950=CARTESIAN_POINT('Ctrl Pts',(1.1700603593783,-6.91560532569806,26.7798789137632));
#154951=CARTESIAN_POINT('Ctrl Pts',(0.979820862296732,-6.94511091476232,
26.771146340624));
#154952=CARTESIAN_POINT('Ctrl Pts',(0.788719045892941,-6.96674592827568,
26.7624137674848));
#154953=CARTESIAN_POINT('Ctrl Pts',(0.594902323132202,-6.98868830169187,
26.7535571342044));
#154954=CARTESIAN_POINT('Ctrl Pts',(0.400198881071557,-7.00253473439903,
26.744700500924));
#154955=CARTESIAN_POINT('Ctrl Pts',(0.205281742193317,-7.00824414306623,
26.7358438676436));
#154956=CARTESIAN_POINT('Ctrl Pts',(0.0129725818766674,-7.01387716021912,
26.7271057355369));
#154957=CARTESIAN_POINT('Ctrl Pts',(-0.179544313956954,-7.01158956178497,
26.7183676034302));
#154958=CARTESIAN_POINT('Ctrl Pts',(-0.371622006393339,-7.00139440732089,
26.7096294713234));
#154959=CARTESIAN_POINT('Ctrl Pts',(-0.567606958134552,-6.99099186223461,
26.7007135874562));
#154960=CARTESIAN_POINT('Ctrl Pts',(-0.763134350466151,-6.97235661479738,
26.691797703589));
#154961=CARTESIAN_POINT('Ctrl Pts',(-0.957520795717108,-6.94555832804457,
26.6828818197217));
#154962=CARTESIAN_POINT('Ctrl Pts',(-1.15190724096807,-6.91876004129176,
26.6739659358545));
#154963=CARTESIAN_POINT('Ctrl Pts',(-1.34515244039036,-6.88379876254957,
26.6650500519873));
#154964=CARTESIAN_POINT('Ctrl Pts',(-1.53658136398352,-6.84079997327495,
26.65613416812));
#154965=CARTESIAN_POINT('Ctrl Pts',(-1.72424866085428,-6.7986461210753,
26.6473934836238));
#154966=CARTESIAN_POINT('Ctrl Pts',(-1.91019033201925,-6.74876322731641,
26.6386527991276));
#154967=CARTESIAN_POINT('Ctrl Pts',(-2.09378076403657,-6.69131591502378,
26.6299121146314));
#154968=CARTESIAN_POINT('Ctrl Pts',(-2.27733816508554,-6.63387893845688,
26.6211730027295));
#154969=CARTESIAN_POINT('Ctrl Pts',(-2.45854491059668,-6.56888034304077,
26.6124338908276));
#154970=CARTESIAN_POINT('Ctrl Pts',(-2.63679070772815,-6.49653456283721,
26.6036947789258));
#154971=CARTESIAN_POINT('Ctrl Pts',(-2.81734593570198,-6.42325143892735,
26.5948424392514));
#154972=CARTESIAN_POINT('Ctrl Pts',(-2.99486268119414,-6.34242950269776,
26.5859900995771));
#154973=CARTESIAN_POINT('Ctrl Pts',(-3.16872638396559,-6.25434246472484,
26.5771377599027));
#154974=CARTESIAN_POINT('Ctrl Pts',(-3.34027827089012,-6.16742669486049,
26.568403127253));
#154975=CARTESIAN_POINT('Ctrl Pts',(-3.50827341437775,-6.07343796674531,
26.5596684946033));
#154976=CARTESIAN_POINT('Ctrl Pts',(-3.6721442503273,-5.97268642800609,
26.5509338619535));
#154977=CARTESIAN_POINT('Ctrl Pts',(-3.83932754645015,-5.86989831297471,
26.5420226687669));
#154978=CARTESIAN_POINT('Ctrl Pts',(-4.00221776425247,-5.76007120419847,
26.5331114755802));
#154979=CARTESIAN_POINT('Ctrl Pts',(-4.16024047493792,-5.64358270544415,
26.5242002823936));
#154980=CARTESIAN_POINT('Ctrl Pts',(-4.31826318562334,-5.52709420668986,
26.5152890892069));
#154981=CARTESIAN_POINT('Ctrl Pts',(-4.47141813719785,-5.40394448697886,
26.5063778960203));
#154982=CARTESIAN_POINT('Ctrl Pts',(-4.61916328400845,-5.27455752818834,
26.4974667028336));
#154983=CARTESIAN_POINT('Ctrl Pts',(-4.75222661313107,-5.15802808642069,
26.4894410379812));
#154984=CARTESIAN_POINT('Ctrl Pts',(-4.88096269756848,-5.03638549043477,
26.4814153731288));
#154985=CARTESIAN_POINT('Ctrl Pts',(-5.00495595374457,-4.90999414089028,
26.4733897082764));
#154986=CARTESIAN_POINT('Ctrl Pts',(-5.12890985750245,-4.78364290486,26.4653665905732));
#154987=CARTESIAN_POINT('Ctrl Pts',(-5.24812367342016,-4.65254617720502,
26.4573434728699));
#154988=CARTESIAN_POINT('Ctrl Pts',(-5.36221771831204,-4.51710612050685,
26.4493203551667));
#154989=CARTESIAN_POINT('Ctrl Pts',(-5.47629737494666,-4.38168314398478,
26.4412982492488));
#154990=CARTESIAN_POINT('Ctrl Pts',(-5.5852583109627,-4.24191821009367,
26.4332761433309));
#154991=CARTESIAN_POINT('Ctrl Pts',(-5.68876032072398,-4.09824750056124,
26.425254037413));
#154992=CARTESIAN_POINT('Ctrl Pts',(-5.79230079218135,-3.95452340250834,
26.4172289504535));
#154993=CARTESIAN_POINT('Ctrl Pts',(-5.89037806806708,-3.80689092532794,
26.409203863494));
#154994=CARTESIAN_POINT('Ctrl Pts',(-5.98269432984447,-3.65581661440324,
26.4011787765344));
#154995=CARTESIAN_POINT('Ctrl Pts',(-6.07502877284792,-3.50471255014858,
26.3931521090742));
#154996=CARTESIAN_POINT('Ctrl Pts',(-6.16159975781025,-3.35016561913782,
26.3851254416139));
#154997=CARTESIAN_POINT('Ctrl Pts',(-6.24215496202924,-3.19266784876124,
26.3770987741536));
#154998=CARTESIAN_POINT('Ctrl Pts',(-6.32277483568218,-3.03504363972989,
26.369065662913));
#154999=CARTESIAN_POINT('Ctrl Pts',(-6.39736912435996,-2.87446419052744,
26.3610325516724));
#155000=CARTESIAN_POINT('Ctrl Pts',(-6.46573301858075,-2.71144299127506,
26.3529994404318));
#155001=CARTESIAN_POINT('Ctrl Pts',(-6.50601550850889,-2.61538497860908,
26.3482660394702));
#155002=CARTESIAN_POINT('Ctrl Pts',(-6.54413573015374,-2.51847954999399,
26.3435326385087));
#155003=CARTESIAN_POINT('Ctrl Pts',(-6.58005986285852,-2.42083431149228,
26.3387992375471));
#155004=CARTESIAN_POINT('Ctrl Pts',(-6.65406469426429,-2.21968208125537,
26.329048284253));
#155005=CARTESIAN_POINT('Ctrl Pts',(-6.71879150752572,-2.01527117141818,
26.3192973309588));
#155006=CARTESIAN_POINT('Ctrl Pts',(-6.77402074923731,-1.80838863395079,
26.3095463776647));
#155007=CARTESIAN_POINT('Ctrl Pts',(-6.82932955903277,-1.60120804337632,
26.299781376293));
#155008=CARTESIAN_POINT('Ctrl Pts',(-6.8751134172199,-1.39154873976351,
26.2900163749214));
#155009=CARTESIAN_POINT('Ctrl Pts',(-6.91120301163579,-1.1802116312155,
26.2802513735497));
#155010=CARTESIAN_POINT('Ctrl Pts',(-6.94723245217505,-0.969226777841337,
26.2705026484122));
#155011=CARTESIAN_POINT('Ctrl Pts',(-6.97359991649955,-0.75656974607434,
26.2607539232746));
#155012=CARTESIAN_POINT('Ctrl Pts',(-6.99018785445479,-0.54304725570876,
26.2510051981371));
#155013=CARTESIAN_POINT('Ctrl Pts',(-7.00673026495205,-0.330110801789158,
26.2412832294701));
#155014=CARTESIAN_POINT('Ctrl Pts',(-7.01354672967217,-0.116313671079241,
26.2315612608032));
#155015=CARTESIAN_POINT('Ctrl Pts',(-7.01057155428194,0.0975348388676593,
26.2218392921362));
#155016=CARTESIAN_POINT('Ctrl Pts',(-7.00761606485012,0.309968369083623,
26.2121816511964));
#155017=CARTESIAN_POINT('Ctrl Pts',(-6.99499805624369,0.522452553789386,
26.2025240102567));
#155018=CARTESIAN_POINT('Ctrl Pts',(-6.97270378507736,0.73418559511063,
26.1928663693169));
#155019=CARTESIAN_POINT('Ctrl Pts',(-6.96290468535469,0.827249556296496,
26.1886215036315));
#155020=CARTESIAN_POINT('Ctrl Pts',(-6.95123688691085,0.920168297558035,
26.1843766379461));
#155021=CARTESIAN_POINT('Ctrl Pts',(-6.93770238185817,1.01287325132982,
26.1801317722607));
#155022=CARTESIAN_POINT('Ctrl Pts',(-6.91266722857905,1.18435220223187,
26.1722799252468));
#155023=CARTESIAN_POINT('Ctrl Pts',(-6.88125167260407,1.35502869998381,
26.1644280782329));
#155024=CARTESIAN_POINT('Ctrl Pts',(-6.84353050352254,1.52437423550011,
26.156576231219));
#155025=CARTESIAN_POINT('Ctrl Pts',(-6.80582003185968,1.69367174599126,
26.1487266109254));
#155026=CARTESIAN_POINT('Ctrl Pts',(-6.76180758702288,1.86163867308816,
26.1408769906318));
#155027=CARTESIAN_POINT('Ctrl Pts',(-6.71161920016561,2.02775597014738,
26.1330273703382));
#155028=CARTESIAN_POINT('Ctrl Pts',(-6.66143482020923,2.19386000486471,
26.1251783767365));
#155029=CARTESIAN_POINT('Ctrl Pts',(-6.60507559084176,2.35811433856822,
26.1173293831347));
#155030=CARTESIAN_POINT('Ctrl Pts',(-6.5427175400908,2.52001463350676,26.1094803895329));
#155031=CARTESIAN_POINT('Ctrl Pts',(-6.48032791928435,2.68199689382481,
26.1016274222155));
#155032=CARTESIAN_POINT('Ctrl Pts',(-6.41193354624725,2.84162237770336,
26.093774454898));
#155033=CARTESIAN_POINT('Ctrl Pts',(-6.33775891677217,2.99840598908401,
26.0859214875806));
#155034=CARTESIAN_POINT('Ctrl Pts',(-6.26356544943364,3.15522941823366,
26.0780665258733));
#155035=CARTESIAN_POINT('Ctrl Pts',(-6.18358897692535,3.30920919844509,
26.070211564166));
#155036=CARTESIAN_POINT('Ctrl Pts',(-6.09809987939284,3.45988503038022,
26.0623566024587));
#155037=CARTESIAN_POINT('Ctrl Pts',(-6.01252592678512,3.61071042067329,
26.0544938440454));
#155038=CARTESIAN_POINT('Ctrl Pts',(-5.92142862103876,3.75822498838122,
26.0466310856321));
#155039=CARTESIAN_POINT('Ctrl Pts',(-5.82512188613292,3.90199712636943,
26.0387683272187));
#155040=CARTESIAN_POINT('Ctrl Pts',(-5.75447264732586,4.00746630378949,
26.0330003204706));
#155041=CARTESIAN_POINT('Ctrl Pts',(-5.68102087203422,4.1109221094603,26.0272323137224));
#155042=CARTESIAN_POINT('Ctrl Pts',(-5.60490397254878,4.21220583791996,
26.0214643069743));
#155043=CARTESIAN_POINT('Ctrl Pts',(-5.49434369253848,4.35932109687934,
26.0130862405333));
#155044=CARTESIAN_POINT('Ctrl Pts',(-5.37791440519695,4.50217851939109,
26.0047081740923));
#155045=CARTESIAN_POINT('Ctrl Pts',(-5.2559707608116,4.64030149063545,25.9963301076512));
#155046=CARTESIAN_POINT('Ctrl Pts',(-5.1341105000411,4.77833001503352,25.9879577700325));
#155047=CARTESIAN_POINT('Ctrl Pts',(-5.00674361665911,4.91163029686316,
25.9795854324137));
#155048=CARTESIAN_POINT('Ctrl Pts',(-4.87426540130525,5.03975826405777,
25.971213094795));
#155049=CARTESIAN_POINT('Ctrl Pts',(-4.74185834496274,5.16781740892225,
25.9628452542723));
#155050=CARTESIAN_POINT('Ctrl Pts',(-4.60434566665319,5.29070955068675,
25.9544774137497));
#155051=CARTESIAN_POINT('Ctrl Pts',(-4.46216023742309,5.40802668059805,
25.946109573227));
#155052=CARTESIAN_POINT('Ctrl Pts',(-4.32003035217989,5.52529798119222,
25.9377450015571));
#155053=CARTESIAN_POINT('Ctrl Pts',(-4.1732316092692,5.63699840398083,25.9293804298871));
#155054=CARTESIAN_POINT('Ctrl Pts',(-4.02223109316899,5.74275923190626,
25.9210158582172));
#155055=CARTESIAN_POINT('Ctrl Pts',(-3.87126746179278,5.84849422575477,
25.9126533297516));
#155056=CARTESIAN_POINT('Ctrl Pts',(-3.71610437327031,5.94829233005975,
25.9042908012861));
#155057=CARTESIAN_POINT('Ctrl Pts',(-3.5572394794681,6.0418270289883,25.8959282728205));
#155058=CARTESIAN_POINT('Ctrl Pts',(-3.39836190775007,6.1353691922786,25.887565076999));
#155059=CARTESIAN_POINT('Ctrl Pts',(-3.23578222071404,6.22264677962363,
25.8792018811775));
#155060=CARTESIAN_POINT('Ctrl Pts',(-3.07002502461718,6.30337789686802,
25.870838685356));
#155061=CARTESIAN_POINT('Ctrl Pts',(-2.90425652421129,6.38411451981303,
25.8624749191813));
#155062=CARTESIAN_POINT('Ctrl Pts',(-2.7353103781694,6.45830363823885,25.8541111530066));
#155063=CARTESIAN_POINT('Ctrl Pts',(-2.56373380198316,6.52571034869531,
25.8457473868319));
#155064=CARTESIAN_POINT('Ctrl Pts',(-2.39212264942504,6.5931306430543,25.8373819351783));
#155065=CARTESIAN_POINT('Ctrl Pts',(-2.21788031573532,6.6537656837975,25.8290164835247));
#155066=CARTESIAN_POINT('Ctrl Pts',(-2.04157230816241,6.70742939381731,
25.8206510318712));
#155067=CARTESIAN_POINT('Ctrl Pts',(-1.86520525538438,6.7611110757081,25.8122827786443));
#155068=CARTESIAN_POINT('Ctrl Pts',(-1.68677146368532,6.8078166757492,25.8039145254174));
#155069=CARTESIAN_POINT('Ctrl Pts',(-1.5068502648184,6.84741037487288,25.7955462721905));
#155070=CARTESIAN_POINT('Ctrl Pts',(-1.32676225333157,6.8870407830043,25.7871702603991));
#155071=CARTESIAN_POINT('Ctrl Pts',(-1.14518440037874,6.91954604321055,
25.7787942486076));
#155072=CARTESIAN_POINT('Ctrl Pts',(-0.962706094642602,6.94484150559521,
25.7704182368161));
#155073=CARTESIAN_POINT('Ctrl Pts',(-0.780138299290921,6.97014937318714,
25.762038117325));
#155074=CARTESIAN_POINT('Ctrl Pts',(-0.596669496892935,6.98824035330412,
25.7536579978338));
#155075=CARTESIAN_POINT('Ctrl Pts',(-0.412893477279431,6.99908176398305,
25.7452778783427));
#155076=CARTESIAN_POINT('Ctrl Pts',(-0.228907470283813,7.00993556234702,
25.7368881835035));
#155077=CARTESIAN_POINT('Ctrl Pts',(-0.0446138732810691,7.0135232261692,
25.7284984886643));
#155078=CARTESIAN_POINT('Ctrl Pts',(0.139392895001137,7.00986420576913,
25.720108793825));
#155079=CARTESIAN_POINT('Ctrl Pts',(0.256215616824345,7.00754115685993,
25.7147823213505));
#155080=CARTESIAN_POINT('Ctrl Pts',(0.372922769241343,7.00229819252713,
25.709455848876));
#155081=CARTESIAN_POINT('Ctrl Pts',(0.489363448129637,6.99415112634369,
25.7041293764015));
#155082=CARTESIAN_POINT('Ctrl Pts',(0.67258495425426,6.9813315709196,25.6957480759965));
#155083=CARTESIAN_POINT('Ctrl Pts',(0.855515982903206,6.96129316380636,
25.6873667755916));
#155084=CARTESIAN_POINT('Ctrl Pts',(1.03756407028496,6.9340527372204,25.6789854751867));
#155085=CARTESIAN_POINT('Ctrl Pts',(1.21938143836511,6.90684683388755,25.6706147968532));
#155086=CARTESIAN_POINT('Ctrl Pts',(1.40031777380958,6.87245714934698,25.6622441185196));
#155087=CARTESIAN_POINT('Ctrl Pts',(1.57978345622306,6.8309524075303,25.6538734401861));
#155088=CARTESIAN_POINT('Ctrl Pts',(1.75904547589867,6.78949476646981,25.6455122611353));
#155089=CARTESIAN_POINT('Ctrl Pts',(1.93683985163729,6.74093823461556,25.6371510820845));
#155090=CARTESIAN_POINT('Ctrl Pts',(2.11258446831307,6.68540301154257,25.6287899030338));
#155091=CARTESIAN_POINT('Ctrl Pts',(2.28810103561878,6.62993985197216,25.6204395735991));
#155092=CARTESIAN_POINT('Ctrl Pts',(2.46157283817462,6.56751616194645,25.6120892441644));
#155093=CARTESIAN_POINT('Ctrl Pts',(2.63243037417588,6.49830261588488,25.6037389147297));
#155094=CARTESIAN_POINT('Ctrl Pts',(2.80315644552294,6.42914232550703,25.595395010374));
#155095=CARTESIAN_POINT('Ctrl Pts',(2.97127195652179,6.35320271284423,25.5870511060183));
#155096=CARTESIAN_POINT('Ctrl Pts',(3.13622383737408,6.27070383644345,25.5787072016627));
#155097=CARTESIAN_POINT('Ctrl Pts',(3.30104322784797,6.18827122365419,25.570369999183));
#155098=CARTESIAN_POINT('Ctrl Pts',(3.46270376373737,6.09929000042067,25.5620327967032));
#155099=CARTESIAN_POINT('Ctrl Pts',(3.62067345367302,6.00402784007266,25.5536955942235));
#155100=CARTESIAN_POINT('Ctrl Pts',(3.67267620362997,5.97266806271945,25.5509510331874));
#155101=CARTESIAN_POINT('Ctrl Pts',(3.72427915896482,5.94062800628429,25.5482064721512));
#155102=CARTESIAN_POINT('Ctrl Pts',(3.77546389517242,5.90791832532826,25.545461911115));
#155103=CARTESIAN_POINT('Ctrl Pts',(3.93096935036048,5.80854233547277,25.5371236008131));
#155104=CARTESIAN_POINT('Ctrl Pts',(4.08248496436116,5.70306382850009,25.5287852905112));
#155105=CARTESIAN_POINT('Ctrl Pts',(4.22953330315354,5.59184000128895,25.5204469802093));
#155106=CARTESIAN_POINT('Ctrl Pts',(4.37667415977078,5.48054619581996,25.5121034237255));
#155107=CARTESIAN_POINT('Ctrl Pts',(4.51934187365447,5.36350005767804,25.5037598672417));
#155108=CARTESIAN_POINT('Ctrl Pts',(4.65709241826652,5.24109881324752,25.4954163107579));
#155109=CARTESIAN_POINT('Ctrl Pts',(4.79494776289289,5.11860444648338,25.4870664065326));
#155110=CARTESIAN_POINT('Ctrl Pts',(4.9278782316006,4.9907470642378,25.4787165023074));
#155111=CARTESIAN_POINT('Ctrl Pts',(5.05547663845835,4.85796073682177,25.4703665980822));
#155112=CARTESIAN_POINT('Ctrl Pts',(5.18326643348369,4.72497523974123,25.4620041696185));
#155113=CARTESIAN_POINT('Ctrl Pts',(5.30570795752275,4.58704626030353,25.4536417411548));
#155114=CARTESIAN_POINT('Ctrl Pts',(5.42243333523086,4.44464208766883,25.4452793126912));
#155115=CARTESIAN_POINT('Ctrl Pts',(5.53925852904966,4.30211614005307,25.4369097332112));
#155116=CARTESIAN_POINT('Ctrl Pts',(5.65035762646628,4.1551076243623,25.4285401537312));
#155117=CARTESIAN_POINT('Ctrl Pts',(5.7554057779623,4.00411424580995,25.4201705742511));
#155118=CARTESIAN_POINT('Ctrl Pts',(5.86061595343287,3.8528879783683,25.4117880857145));
#155119=CARTESIAN_POINT('Ctrl Pts',(5.95975635714806,3.69766484179189,25.4034055971779));
#155120=CARTESIAN_POINT('Ctrl Pts',(6.05254710073434,3.53896879837791,25.3950231086413));
#155121=CARTESIAN_POINT('Ctrl Pts',(6.08290975250043,3.48704085258712,25.3922802210371));
#155122=CARTESIAN_POINT('Ctrl Pts',(6.11259292136257,3.43474123219163,25.3895373334329));
#155123=CARTESIAN_POINT('Ctrl Pts',(6.1415879167107,3.38208876640061,25.3867944458286));
#155124=CARTESIAN_POINT('Ctrl Pts',(6.23396022342135,3.21434844912426,25.3780561497189));
#155125=CARTESIAN_POINT('Ctrl Pts',(6.31951401861006,3.04271762722003,25.3693178536093));
#155126=CARTESIAN_POINT('Ctrl Pts',(6.39793694776335,2.86775685422328,25.3605795574996));
#155127=CARTESIAN_POINT('Ctrl Pts',(6.46020040433268,2.72884770343746,25.3536418349969));
#155128=CARTESIAN_POINT('Ctrl Pts',(6.51796974249906,2.58784013399584,25.3467041124941));
#155129=CARTESIAN_POINT('Ctrl Pts',(6.57110895151814,2.44502632087636,25.3397663899914));
#155130=CARTESIAN_POINT('Origin',(0.,0.,50.));
#155131=CARTESIAN_POINT('',(6.57110895151814,2.44502632087637,23.3397812382711));
#155132=CARTESIAN_POINT('',(6.57110895151814,2.44502632087635,23.8869833201214));
#155133=CARTESIAN_POINT('',(6.57110895151814,2.44502632087636,50.));
#155134=CARTESIAN_POINT('',(7.01124974356013,-0.001896293246826,25.7735343569105));
#155135=CARTESIAN_POINT('Ctrl Pts',(6.57110895151814,2.44502632087635,23.8869833201214));
#155136=CARTESIAN_POINT('Ctrl Pts',(6.50404482602339,2.62526392061162,23.8957163741572));
#155137=CARTESIAN_POINT('Ctrl Pts',(6.42955178260845,2.8027657603483,23.9044494281931));
#155138=CARTESIAN_POINT('Ctrl Pts',(6.34787351276833,2.97693272150956,23.9131824822289));
#155139=CARTESIAN_POINT('Ctrl Pts',(6.26622575892236,3.15103461177769,23.9219122734896));
#155140=CARTESIAN_POINT('Ctrl Pts',(6.17739825529668,3.32180386372133,23.9306420647503));
#155141=CARTESIAN_POINT('Ctrl Pts',(6.08168209537615,3.48866298935297,23.939371856011));
#155142=CARTESIAN_POINT('Ctrl Pts',(6.04178272988089,3.55821836271232,23.9430108771804));
#155143=CARTESIAN_POINT('Ctrl Pts',(6.00068692045035,3.62709456677471,23.9466498983498));
#155144=CARTESIAN_POINT('Ctrl Pts',(5.95841812638918,3.69525100549569,23.9502889195193));
#155145=CARTESIAN_POINT('Ctrl Pts',(5.8651965816224,3.84556635383936,23.9583145843718));
#155146=CARTESIAN_POINT('Ctrl Pts',(5.76622355083788,3.99244807418705,23.9663402492242));
#155147=CARTESIAN_POINT('Ctrl Pts',(5.66179063331389,4.13542662696597,23.9743659140767));
#155148=CARTESIAN_POINT('Ctrl Pts',(5.55739086023635,4.27835980185925,23.98238903178));
#155149=CARTESIAN_POINT('Ctrl Pts',(5.44753486628551,4.41739197979333,23.9904121494833));
#155150=CARTESIAN_POINT('Ctrl Pts',(5.33255737110211,4.55208286901772,23.9984352671866));
#155151=CARTESIAN_POINT('Ctrl Pts',(5.21759437558721,4.68675677254207,24.0064573731045));
#155152=CARTESIAN_POINT('Ctrl Pts',(5.09751140371063,4.8170901995232,24.0144794790224));
#155153=CARTESIAN_POINT('Ctrl Pts',(4.97268318748858,4.94267624666723,24.0225015849403));
#155154=CARTESIAN_POINT('Ctrl Pts',(4.84780858467955,5.06830896201076,24.0305266718999));
#155155=CARTESIAN_POINT('Ctrl Pts',(4.71818547144416,5.18919051097218,24.0385517588595));
#155156=CARTESIAN_POINT('Ctrl Pts',(4.58422546121499,5.30495084644978,24.0465768458191));
#155157=CARTESIAN_POINT('Ctrl Pts',(4.45023906823207,5.42073398034625,24.0546035132794));
#155158=CARTESIAN_POINT('Ctrl Pts',(4.31191435980095,5.53139365845925,24.0626301807397));
#155159=CARTESIAN_POINT('Ctrl Pts',(4.1696955226784,5.63660055447038,24.0706568482));
#155160=CARTESIAN_POINT('Ctrl Pts',(4.0273625127746,5.74189191020686,24.0786899594406));
#155161=CARTESIAN_POINT('Ctrl Pts',(3.88112943055859,5.84172153043871,24.0867230706813));
#155162=CARTESIAN_POINT('Ctrl Pts',(3.73146940048094,5.93580345663285,24.094756181922));
#155163=CARTESIAN_POINT('Ctrl Pts',(3.64328427407108,5.99123994525314,24.0994895828831));
#155164=CARTESIAN_POINT('Ctrl Pts',(3.55390981728491,6.04468168798134,24.1042229838443));
#155165=CARTESIAN_POINT('Ctrl Pts',(3.46344666393083,6.09607773643073,24.1089563848055));
#155166=CARTESIAN_POINT('Ctrl Pts',(3.27708975260619,6.20195519579622,24.1187073380996));
#155167=CARTESIAN_POINT('Ctrl Pts',(3.08600197741005,6.29921177699002,24.1284582913937));
#155168=CARTESIAN_POINT('Ctrl Pts',(2.89092393910911,6.38750227716483,24.1382092446878));
#155169=CARTESIAN_POINT('Ctrl Pts',(2.69556485429831,6.47591997636801,24.1479742460593));
#155170=CARTESIAN_POINT('Ctrl Pts',(2.49620404244238,6.55534574017783,24.1577392474308));
#155171=CARTESIAN_POINT('Ctrl Pts',(2.29360398337489,6.62548166776929,24.1675042488024));
#155172=CARTESIAN_POINT('Ctrl Pts',(2.09134161662808,6.69550069330128,24.1772529739399));
#155173=CARTESIAN_POINT('Ctrl Pts',(1.8858508292091,6.7562608169052,24.1870016990774));
#155174=CARTESIAN_POINT('Ctrl Pts',(1.67790829217237,6.80751425452486,24.1967504242149));
#155175=CARTESIAN_POINT('Ctrl Pts',(1.47053647677048,6.85862702133169,24.206472392882));
#155176=CARTESIAN_POINT('Ctrl Pts',(1.26072638407638,6.90028518134357,24.2161943615491));
#155177=CARTESIAN_POINT('Ctrl Pts',(1.04926570122329,6.93229168823243,24.2259163302161));
#155178=CARTESIAN_POINT('Ctrl Pts',(0.839204198477849,6.96408641642489,
24.2355739711558));
#155179=CARTESIAN_POINT('Ctrl Pts',(0.627513918248232,6.9863567587275,24.2452316120954));
#155180=CARTESIAN_POINT('Ctrl Pts',(0.414983637284344,6.99895814698776,
24.2548892530351));
#155181=CARTESIAN_POINT('Ctrl Pts',(0.321569261820565,7.004496890968,24.2591341187208));
#155182=CARTESIAN_POINT('Ctrl Pts',(0.227992819303063,7.00816832190326,
24.2633789844064));
#155183=CARTESIAN_POINT('Ctrl Pts',(0.134322281303897,7.00996320156143,
24.2676238500921));
#155184=CARTESIAN_POINT('Ctrl Pts',(-0.038942737790631,7.0132832407636,
24.275475697106));
#155185=CARTESIAN_POINT('Ctrl Pts',(-0.212458611611713,7.01017750829807,
24.28332754412));
#155186=CARTESIAN_POINT('Ctrl Pts',(-0.385691713600459,7.00063343309446,
24.2911793911339));
#155187=CARTESIAN_POINT('Ctrl Pts',(-0.558875688082151,6.99109206451341,
24.2990290114275));
#155188=CARTESIAN_POINT('Ctrl Pts',(-0.731776669736127,6.97511600610969,
24.3068786317211));
#155189=CARTESIAN_POINT('Ctrl Pts',(-0.903861994681407,6.95274478584325,
24.3147282520147));
#155190=CARTESIAN_POINT('Ctrl Pts',(-1.07593358081459,6.93037535163261,
24.3225772456165));
#155191=CARTESIAN_POINT('Ctrl Pts',(-1.2471892616903,6.90161182188765,24.3304262392183));
#155192=CARTESIAN_POINT('Ctrl Pts',(-1.41710271542319,6.86654545287805,
24.3382752328201));
#155193=CARTESIAN_POINT('Ctrl Pts',(-1.58710219136203,6.83146133079269,
24.3461282001375));
#155194=CARTESIAN_POINT('Ctrl Pts',(-1.7557577083443,6.7900680709802,24.3539811674549));
#155195=CARTESIAN_POINT('Ctrl Pts',(-1.92255400821172,6.74250789009617,
24.3618341347724));
#155196=CARTESIAN_POINT('Ctrl Pts',(-2.08939266873477,6.69493563052426,
24.3696890964796));
#155197=CARTESIAN_POINT('Ctrl Pts',(-2.25437080870463,6.64119344782899,
24.3775440581869));
#155198=CARTESIAN_POINT('Ctrl Pts',(-2.41699013617812,6.58147287802037,
24.3853990198941));
#155199=CARTESIAN_POINT('Ctrl Pts',(-2.57977087692747,6.52169303055417,
24.3932617783075));
#155200=CARTESIAN_POINT('Ctrl Pts',(-2.74018777617318,6.4559230888124,24.4011245367208));
#155201=CARTESIAN_POINT('Ctrl Pts',(-2.89776373374651,6.38440223559602,
24.4089872951342));
#155202=CARTESIAN_POINT('Ctrl Pts',(-3.01335919514051,6.33193556394028,
24.4147553018822));
#155203=CARTESIAN_POINT('Ctrl Pts',(-3.12742626232211,6.27637504553989,
24.4205233086303));
#155204=CARTESIAN_POINT('Ctrl Pts',(-3.23978591027477,6.21783031435284,
24.4262913153784));
#155205=CARTESIAN_POINT('Ctrl Pts',(-3.40298901265464,6.13279372041702,
24.4346693818195));
#155206=CARTESIAN_POINT('Ctrl Pts',(-3.56295046482453,6.04127128635174,
24.4430474482605));
#155207=CARTESIAN_POINT('Ctrl Pts',(-3.7191421093381,5.94353501992275,24.4514255147015));
#155208=CARTESIAN_POINT('Ctrl Pts',(-3.87522695186101,5.84586558439145,
24.4597978523202));
#155209=CARTESIAN_POINT('Ctrl Pts',(-4.02754684822184,5.74199096145221,
24.468170189939));
#155210=CARTESIAN_POINT('Ctrl Pts',(-4.17559910596323,5.63222857035997,
24.4765425275577));
#155211=CARTESIAN_POINT('Ctrl Pts',(-4.32357183929128,5.52252513675943,
24.4849103680803));
#155212=CARTESIAN_POINT('Ctrl Pts',(-4.46728124116798,5.4069404361491,24.4932782086029));
#155213=CARTESIAN_POINT('Ctrl Pts',(-4.60625405735026,5.2858348556916,24.5016460491255));
#155214=CARTESIAN_POINT('Ctrl Pts',(-4.74517258453623,5.16477658448919,
24.5100106207954));
#155215=CARTESIAN_POINT('Ctrl Pts',(-4.87935796838042,5.03820194985158,
24.5183751924653));
#155216=CARTESIAN_POINT('Ctrl Pts',(-5.00837012799503,4.90651151262352,
24.5267397641352));
#155217=CARTESIAN_POINT('Ctrl Pts',(-5.13735077395742,4.77485324326747,
24.5351022926008));
#155218=CARTESIAN_POINT('Ctrl Pts',(-5.26116048622341,4.63808189827305,
24.5434648210664));
#155219=CARTESIAN_POINT('Ctrl Pts',(-5.37939582343168,4.49663509052556,
24.551827349532));
#155220=CARTESIAN_POINT('Ctrl Pts',(-5.49764059618969,4.35517699488037,
24.5601905453535));
#155221=CARTESIAN_POINT('Ctrl Pts',(-5.61030988971127,4.20904293934588,
24.568553741175));
#155222=CARTESIAN_POINT('Ctrl Pts',(-5.71703988042991,4.05870441989485,
24.5769169369966));
#155223=CARTESIAN_POINT('Ctrl Pts',(-5.82377714991998,3.90835564765814,
24.5852807031713));
#155224=CARTESIAN_POINT('Ctrl Pts',(-5.92457411840601,3.75380210774675,
24.593644469346));
#155225=CARTESIAN_POINT('Ctrl Pts',(-6.01910962728124,3.59554527954666,
24.6020082355207));
#155226=CARTESIAN_POINT('Ctrl Pts',(-6.11366418709565,3.43725655919045,
24.6103736871743));
#155227=CARTESIAN_POINT('Ctrl Pts',(-6.20195460260338,3.27526334468759,
24.6187391388278));
#155228=CARTESIAN_POINT('Ctrl Pts',(-6.28370489657797,3.11009313931625,
24.6271045904814));
#155229=CARTESIAN_POINT('Ctrl Pts',(-6.36548256856545,2.94486761876756,
24.6354728437083));
#155230=CARTESIAN_POINT('Ctrl Pts',(-6.44071560576633,2.77646328031728,
24.6438410969352));
#155231=CARTESIAN_POINT('Ctrl Pts',(-6.50917535471592,2.60542947785176,
24.652209350162));
#155232=CARTESIAN_POINT('Ctrl Pts',(-6.57769857561956,2.43423710265091,
24.6605853619535));
#155233=CARTESIAN_POINT('Ctrl Pts',(-6.63943583704474,2.2604106973618,24.668961373745));
#155234=CARTESIAN_POINT('Ctrl Pts',(-6.69420732377659,2.08451789841101,
24.6773373855365));
#155235=CARTESIAN_POINT('Ctrl Pts',(-6.74900567112229,1.90853883945832,
24.6857175050276));
#155236=CARTESIAN_POINT('Ctrl Pts',(-6.79683133996421,1.73049168161851,
24.6940976245188));
#155237=CARTESIAN_POINT('Ctrl Pts',(-6.83755506548899,1.55095689459954,
24.7024777440099));
#155238=CARTESIAN_POINT('Ctrl Pts',(-6.8783253230288,1.37121696634411,24.7108674388492));
#155239=CARTESIAN_POINT('Ctrl Pts',(-6.91197735568175,1.18998633447894,
24.7192571336884));
#155240=CARTESIAN_POINT('Ctrl Pts',(-6.93843322754209,1.00785460729208,
24.7276468285276));
#155241=CARTESIAN_POINT('Ctrl Pts',(-6.95522960404399,0.892222316701829,
24.7329733010022));
#155242=CARTESIAN_POINT('Ctrl Pts',(-6.9691264230549,0.776226943854541,
24.7382997734768));
#155243=CARTESIAN_POINT('Ctrl Pts',(-6.98011462870249,0.660019948693604,
24.7436262459514));
#155244=CARTESIAN_POINT('Ctrl Pts',(-6.99740476826154,0.477166148126987,
24.7520075463562));
#155245=CARTESIAN_POINT('Ctrl Pts',(-7.0075256093269,0.293419399643907,
24.7603888467611));
#155246=CARTESIAN_POINT('Ctrl Pts',(-7.01039695250101,0.109366955085041,
24.768770147166));
#155247=CARTESIAN_POINT('Ctrl Pts',(-7.01326465666798,-0.0744522299437054,
24.7771408254996));
#155248=CARTESIAN_POINT('Ctrl Pts',(-7.00890116796093,-0.258576013994685,
24.7855115038331));
#155249=CARTESIAN_POINT('Ctrl Pts',(-6.99727794590954,-0.442411471582774,
24.7938821821667));
#155250=CARTESIAN_POINT('Ctrl Pts',(-6.98566791421957,-0.626038307489429,
24.8022433612175));
#155251=CARTESIAN_POINT('Ctrl Pts',(-6.96681459007259,-0.80937714407093,
24.8106045402683));
#155252=CARTESIAN_POINT('Ctrl Pts',(-6.94074144317052,-0.991834049403023,
24.8189657193191));
#155253=CARTESIAN_POINT('Ctrl Pts',(-6.91470212925214,-1.17405419537787,
24.8273160487539));
#155254=CARTESIAN_POINT('Ctrl Pts',(-6.8814617253198,-1.35539436992544,
24.8356663781886));
#155255=CARTESIAN_POINT('Ctrl Pts',(-6.84109555852682,-1.53526483761095,
24.8440167076233));
#155256=CARTESIAN_POINT('Ctrl Pts',(-6.80076045108455,-1.71499690573115,
24.852360611979));
#155257=CARTESIAN_POINT('Ctrl Pts',(-6.75331057854142,-1.89326120222885,
24.8607045163347));
#155258=CARTESIAN_POINT('Ctrl Pts',(-6.69887267339629,-2.0694761337412,
24.8690484206904));
#155259=CARTESIAN_POINT('Ctrl Pts',(-6.64447849311608,-2.24554952832158,
24.8773856231701));
#155260=CARTESIAN_POINT('Ctrl Pts',(-6.58310757065704,-2.41957652860795,
24.8857228256499));
#155261=CARTESIAN_POINT('Ctrl Pts',(-6.51493705749792,-2.59098855638932,
24.8940600281296));
#155262=CARTESIAN_POINT('Ctrl Pts',(-6.49249570085809,-2.64741644976337,
24.8968045891656));
#155263=CARTESIAN_POINT('Ctrl Pts',(-6.46931788325442,-2.70356107538801,
24.8995491502017));
#155264=CARTESIAN_POINT('Ctrl Pts',(-6.44541110559393,-2.75940251547079,
24.9022937112378));
#155265=CARTESIAN_POINT('Ctrl Pts',(-6.37277940681515,-2.92905560352234,
24.9106320215397));
#155266=CARTESIAN_POINT('Ctrl Pts',(-6.29347528529428,-3.09576958922512,
24.9189703318416));
#155267=CARTESIAN_POINT('Ctrl Pts',(-6.20777312731114,-3.25901509084167,
24.9273086421435));
#155268=CARTESIAN_POINT('Ctrl Pts',(-6.12201704843831,-3.42236330098845,
24.9356521986273));
#155269=CARTESIAN_POINT('Ctrl Pts',(-6.02985505618818,-3.58223838417279,
24.9439957551111));
#155270=CARTESIAN_POINT('Ctrl Pts',(-5.93160648698461,-3.73813737656364,
24.9523393115949));
#155271=CARTESIAN_POINT('Ctrl Pts',(-5.83328317069781,-3.89415497622842,
24.9606892158201));
#155272=CARTESIAN_POINT('Ctrl Pts',(-5.72886421533329,-4.04619017434361,
24.9690391200453));
#155273=CARTESIAN_POINT('Ctrl Pts',(-5.61871132564573,-4.19377033247654,
24.9773890242705));
#155274=CARTESIAN_POINT('Ctrl Pts',(-5.50839321477503,-4.34157184992565,
24.9857514527342));
#155275=CARTESIAN_POINT('Ctrl Pts',(-5.39232417927697,-4.48490471139241,
24.9941138811978));
#155276=CARTESIAN_POINT('Ctrl Pts',(-5.27090610601988,-4.62332946955139,
25.0024763096615));
#155277=CARTESIAN_POINT('Ctrl Pts',(-5.14938420375849,-4.76187259974862,
25.0108458891414));
#155278=CARTESIAN_POINT('Ctrl Pts',(-5.02250436218446,-4.89549901530344,
25.0192154686214));
#155279=CARTESIAN_POINT('Ctrl Pts',(-4.89070451907986,-5.02380691005854,
25.0275850481013));
#155280=CARTESIAN_POINT('Ctrl Pts',(-4.75870139077554,-5.15231270410847,
25.0359675366379));
#155281=CARTESIAN_POINT('Ctrl Pts',(-4.62176333998194,-5.27548336628875,
25.0443500251745));
#155282=CARTESIAN_POINT('Ctrl Pts',(-4.48036155510013,-5.39295715707818,
25.052732513711));
#155283=CARTESIAN_POINT('Ctrl Pts',(-4.43409257408121,-5.43139650634665,
25.0554754013154));
#155284=CARTESIAN_POINT('Ctrl Pts',(-4.38734588961209,-5.46922623405847,
25.0582182889198));
#155285=CARTESIAN_POINT('Ctrl Pts',(-4.34013865785327,-5.50643468980679,
25.0609611765242));
#155286=CARTESIAN_POINT('Ctrl Pts',(-4.19574271722335,-5.62024670053037,
25.069351031657));
#155287=CARTESIAN_POINT('Ctrl Pts',(-4.04674420327156,-5.72847259738455,
25.0777408867898));
#155288=CARTESIAN_POINT('Ctrl Pts',(-3.89360220379027,-5.83073652647241,
25.0861307419226));
#155289=CARTESIAN_POINT('Ctrl Pts',(-3.74060152159914,-5.9329060878402,
25.0945128550146));
#155290=CARTESIAN_POINT('Ctrl Pts',(-3.58346524817898,-6.02912446724261,
25.1028949681067));
#155291=CARTESIAN_POINT('Ctrl Pts',(-3.42268409254566,-6.11905713040293,
25.1112770811988));
#155292=CARTESIAN_POINT('Ctrl Pts',(-3.26202766901266,-6.20892002487724,
25.1196526915477));
#155293=CARTESIAN_POINT('Ctrl Pts',(-3.09773228661755,-6.29250676523397,
25.1280283018966));
#155294=CARTESIAN_POINT('Ctrl Pts',(-2.93031646352881,-6.36952682591667,
25.1364039122455));
#155295=CARTESIAN_POINT('Ctrl Pts',(-2.7630059474789,-6.44649843983745,
25.144774254211));
#155296=CARTESIAN_POINT('Ctrl Pts',(-2.59257920225916,-6.51691147297294,
25.1531445961766));
#155297=CARTESIAN_POINT('Ctrl Pts',(-2.41957851455754,-6.58052174028713,
25.1615149381422));
#155298=CARTESIAN_POINT('Ctrl Pts',(-2.24666128689977,-6.64410132034932,
25.1698812420365));
#155299=CARTESIAN_POINT('Ctrl Pts',(-2.07117290096369,-6.70088456585396,
25.1782475459308));
#155300=CARTESIAN_POINT('Ctrl Pts',(-1.8936751763582,-6.75067558759453,
25.1866138498251));
#155301=CARTESIAN_POINT('Ctrl Pts',(-1.716227092891,-6.80045268418197,25.1949778138988));
#155302=CARTESIAN_POINT('Ctrl Pts',(-1.53677110705684,-6.84324136622329,
25.2033417779724));
#155303=CARTESIAN_POINT('Ctrl Pts',(-1.3558842738562,-6.87889557984488,
25.211705742046));
#155304=CARTESIAN_POINT('Ctrl Pts',(-1.17502527613319,-6.9145443068755,
25.2200684190445));
#155305=CARTESIAN_POINT('Ctrl Pts',(-0.992736192405863,-6.9430606908922,
25.2284310960431));
#155306=CARTESIAN_POINT('Ctrl Pts',(-0.80960476180415,-6.96434969628637,
25.2367937730416));
#155307=CARTESIAN_POINT('Ctrl Pts',(-0.626477101543896,-6.98563826337883,
25.2451562778679));
#155308=CARTESIAN_POINT('Ctrl Pts',(-0.442507455486583,-6.99969971100276,
25.2535187826942));
#155309=CARTESIAN_POINT('Ctrl Pts',(-0.258289619027391,-7.00649077892797,
25.2618812875205));
#155310=CARTESIAN_POINT('Ctrl Pts',(-0.0740510203503235,-7.01328261223853,
25.2702447348405));
#155311=CARTESIAN_POINT('Ctrl Pts',(0.11043549606457,-7.01280242061977,
25.2786081821605));
#155312=CARTESIAN_POINT('Ctrl Pts',(0.294574756225263,-7.00505904868009,
25.2869716294805));
#155313=CARTESIAN_POINT('Ctrl Pts',(0.478822442757081,-6.99731111722541,
25.2953400014333));
#155314=CARTESIAN_POINT('Ctrl Pts',(0.662722135695841,-6.98229147231855,
25.3037083733861));
#155315=CARTESIAN_POINT('Ctrl Pts',(0.845681362469007,-6.96006103390427,
25.3120767453389));
#155316=CARTESIAN_POINT('Ctrl Pts',(1.02869540860835,-6.93782393466963,
25.3204476246747));
#155317=CARTESIAN_POINT('Ctrl Pts',(1.21076810101937,-6.90837177876169,
25.3288185040105));
#155318=CARTESIAN_POINT('Ctrl Pts',(1.3913150859135,-6.87181700092556,25.3371893833462));
#155319=CARTESIAN_POINT('Ctrl Pts',(1.5720150463155,-6.83523125062147,25.3455673552375));
#155320=CARTESIAN_POINT('Ctrl Pts',(1.75118639481871,-6.79153092394558,
25.3539453271288));
#155321=CARTESIAN_POINT('Ctrl Pts',(1.92825677762194,-6.74087919800193,
25.3623232990201));
#155322=CARTESIAN_POINT('Ctrl Pts',(2.0407864477829,-6.70868961370619,25.3676475683791));
#155323=CARTESIAN_POINT('Ctrl Pts',(2.15246788626999,-6.67369357446904,
25.3729718377381));
#155324=CARTESIAN_POINT('Ctrl Pts',(2.26315789621798,-6.63594325618342,
25.3782961070971));
#155325=CARTESIAN_POINT('Ctrl Pts',(2.42662386757984,-6.58019393923352,
25.3861589382864));
#155326=CARTESIAN_POINT('Ctrl Pts',(2.58826656138555,-6.51831926484871,
25.3940217694757));
#155327=CARTESIAN_POINT('Ctrl Pts',(2.74757357211185,-6.45046246623702,
25.4018846006649));
#155328=CARTESIAN_POINT('Ctrl Pts',(2.90675817642854,-6.38265780661813,
25.4097413903063));
#155329=CARTESIAN_POINT('Ctrl Pts',(3.06361031810499,-6.3088803119669,25.4175981799477));
#155330=CARTESIAN_POINT('Ctrl Pts',(3.21763312647164,-6.22932288663322,
25.4254549695891));
#155331=CARTESIAN_POINT('Ctrl Pts',(3.3715690732653,-6.14981032792144,25.4333073283731));
#155332=CARTESIAN_POINT('Ctrl Pts',(3.52267852308861,-6.06452449706262,
25.441159687157));
#155333=CARTESIAN_POINT('Ctrl Pts',(3.67048520232198,-5.97370613120828,
25.4490120459409));
#155334=CARTESIAN_POINT('Ctrl Pts',(3.81825698267394,-5.88290920862968,
25.4568625506914));
#155335=CARTESIAN_POINT('Ctrl Pts',(3.9627272155274,-5.78658254317813,25.4647130554418));
#155336=CARTESIAN_POINT('Ctrl Pts',(4.10344489977226,-5.68501244651523,
25.4725635601922));
#155337=CARTESIAN_POINT('Ctrl Pts',(4.24413994697689,-5.58345868927958,
25.4804128020438));
#155338=CARTESIAN_POINT('Ctrl Pts',(4.38108333969664,-5.47666340573365,
25.4882620438955));
#155339=CARTESIAN_POINT('Ctrl Pts',(4.51385409985741,-5.36495551963858,
25.4961112857471));
#155340=CARTESIAN_POINT('Ctrl Pts',(4.6466695930859,-5.25320999697032,25.503963172162));
#155341=CARTESIAN_POINT('Ctrl Pts',(4.77530935347403,-5.13654881153163,
25.5118150585768));
#155342=CARTESIAN_POINT('Ctrl Pts',(4.89938632362559,-5.01534048837869,
25.5196669449917));
#155343=CARTESIAN_POINT('Ctrl Pts',(4.9904944984531,-4.92633872533693,25.5254324874556));
#155344=CARTESIAN_POINT('Ctrl Pts',(5.07914321494458,-4.83488608072877,
25.5311980299196));
#155345=CARTESIAN_POINT('Ctrl Pts',(5.16519231646852,-4.74114067460507,
25.5369635723836));
#155346=CARTESIAN_POINT('Ctrl Pts',(5.30929502151379,-4.58414930143849,
25.5466188767435));
#155347=CARTESIAN_POINT('Ctrl Pts',(5.44603316626756,-4.4208075889074,25.5562741811034));
#155348=CARTESIAN_POINT('Ctrl Pts',(5.5749465792256,-4.25177577034359,25.5659294854633));
#155349=CARTESIAN_POINT('Ctrl Pts',(5.70457414830735,-4.0818075472152,25.5756382783981));
#155350=CARTESIAN_POINT('Ctrl Pts',(5.8262900652624,-3.90608606988243,25.5853470713328));
#155351=CARTESIAN_POINT('Ctrl Pts',(5.93967416463933,-3.72530500501852,
25.5950558642676));
#155352=CARTESIAN_POINT('Ctrl Pts',(6.05360387793019,-3.54365400631993,
25.6048113767383));
#155353=CARTESIAN_POINT('Ctrl Pts',(6.15912139122199,-3.3568946580016,25.6145668892091));
#155354=CARTESIAN_POINT('Ctrl Pts',(6.25584836090517,-3.16575233520566,
25.6243224016798));
#155355=CARTESIAN_POINT('Ctrl Pts',(6.35267110516921,-2.97442075210404,
25.6340875736087));
#155356=CARTESIAN_POINT('Ctrl Pts',(6.44068588851664,-2.77869755315185,
25.6438527455376));
#155357=CARTESIAN_POINT('Ctrl Pts',(6.51956111423719,-2.57933120018085,
25.6536179174666));
#155358=CARTESIAN_POINT('Ctrl Pts',(6.59832879537709,-2.38023667870864,
25.6633697748051));
#155359=CARTESIAN_POINT('Ctrl Pts',(6.66798181118765,-2.17750896648122,
25.6731216321437));
#155360=CARTESIAN_POINT('Ctrl Pts',(6.72823771591766,-1.97191374065986,
25.6828734894822));
#155361=CARTESIAN_POINT('Ctrl Pts',(6.75451365431931,-1.88225933229006,
25.6871260055448));
#155362=CARTESIAN_POINT('Ctrl Pts',(6.77900326126279,-1.79205989726403,
25.6913785216074));
#155363=CARTESIAN_POINT('Ctrl Pts',(6.80168598724666,-1.70138011431673,
25.69563103767));
#155364=CARTESIAN_POINT('Ctrl Pts',(6.84497028679044,-1.5283404677396,25.7037458991376));
#155365=CARTESIAN_POINT('Ctrl Pts',(6.88169100112746,-1.35347215330042,
25.7118607606052));
#155366=CARTESIAN_POINT('Ctrl Pts',(6.91169686818472,-1.17731600041179,
25.7199756220728));
#155367=CARTESIAN_POINT('Ctrl Pts',(6.94168248721917,-1.00127871806913,
25.7280850076147));
#155368=CARTESIAN_POINT('Ctrl Pts',(6.96496221977847,-0.823955678787677,
25.7361943931566));
#155369=CARTESIAN_POINT('Ctrl Pts',(6.98143534720324,-0.64590018990645,
25.7443037786985));
#155370=CARTESIAN_POINT('Ctrl Pts',(6.9978989439945,-0.46794771617018,25.7524084725034));
#155371=CARTESIAN_POINT('Ctrl Pts',(7.00756374903863,-0.289263992872046,
25.7605131663082));
#155372=CARTESIAN_POINT('Ctrl Pts',(7.01038060736483,-0.110409702395602,
25.7686178601131));
#155373=CARTESIAN_POINT('Ctrl Pts',(7.01095019807662,-0.0742439706399554,
25.7702566923789));
#155374=CARTESIAN_POINT('Ctrl Pts',(7.01123995951459,-0.0380712819292277,
25.7718955246447));
#155375=CARTESIAN_POINT('Ctrl Pts',(7.01124974356013,-0.001896293246826,
25.7735343569105));
#155376=CARTESIAN_POINT('Ctrl Pts',(7.01125,3.93647490780448E-12,25.7735343569105));
#155377=CARTESIAN_POINT('Ctrl Pts',(7.01124999999989,0.191008754744065,
25.7822061308426));
#155378=CARTESIAN_POINT('Ctrl Pts',(7.00344012880997,0.382017367486861,
25.7908779047747));
#155379=CARTESIAN_POINT('Ctrl Pts',(6.98784644419148,0.572388534913533,
25.7995496787068));
#155380=CARTESIAN_POINT('Ctrl Pts',(6.97225169663166,0.762772678964236,
25.8082220437492));
#155381=CARTESIAN_POINT('Ctrl Pts',(6.94887209704279,0.952519007630594,
25.8168944087915));
#155382=CARTESIAN_POINT('Ctrl Pts',(6.91778566246047,1.14099434299926,25.8255667738339));
#155383=CARTESIAN_POINT('Ctrl Pts',(6.88670108297135,1.32945843104044,25.83423862135));
#155384=CARTESIAN_POINT('Ctrl Pts',(6.84791063501091,1.51665139731177,25.8429104688661));
#155385=CARTESIAN_POINT('Ctrl Pts',(6.80154374572902,1.70194865887149,25.8515823163823));
#155386=CARTESIAN_POINT('Ctrl Pts',(6.75517597619818,1.88724943819406,25.8602543285285));
#155387=CARTESIAN_POINT('Ctrl Pts',(6.70123154646039,2.07065416525621,25.8689263406747));
#155388=CARTESIAN_POINT('Ctrl Pts',(6.63989045285471,2.25155087363996,25.8775983528209));
#155389=CARTESIAN_POINT('Ctrl Pts',(6.61790934153598,2.31637382429903,25.880705901988));
#155390=CARTESIAN_POINT('Ctrl Pts',(6.59497889661491,2.3808748601913,25.8838134511551));
#155391=CARTESIAN_POINT('Ctrl Pts',(6.57110895151813,2.4450263208764,25.8869210003222));
#155392=CARTESIAN_POINT('',(7.01124976619934,0.00181065449874002,25.226465446522));
#155393=CARTESIAN_POINT('Ctrl Pts',(6.57110895151814,2.44502632087636,25.3397663899914));
#155394=CARTESIAN_POINT('Ctrl Pts',(6.63790538062555,2.26550816620888,25.3310456149202));
#155395=CARTESIAN_POINT('Ctrl Pts',(6.69738434870032,2.08313550795474,25.3223248398489));
#155396=CARTESIAN_POINT('Ctrl Pts',(6.74931780320426,1.89850882374829,25.3136040647777));
#155397=CARTESIAN_POINT('Ctrl Pts',(6.8011622294282,1.71419864065453,25.3048982395227));
#155398=CARTESIAN_POINT('Ctrl Pts',(6.84548688543691,1.52764241001528,25.2961924142678));
#155399=CARTESIAN_POINT('Ctrl Pts',(6.88211327509476,1.33945639393918,25.2874865890128));
#155400=CARTESIAN_POINT('Ctrl Pts',(6.91869907638936,1.15147892045898,25.2787904113153));
#155401=CARTESIAN_POINT('Ctrl Pts',(6.94760357468004,0.961875534795149,
25.2700942336178));
#155402=CARTESIAN_POINT('Ctrl Pts',(6.96869864591293,0.771275401495021,
25.2613980559203));
#155403=CARTESIAN_POINT('Ctrl Pts',(6.98976139966878,0.580967266044245,
25.2527152006961));
#155404=CARTESIAN_POINT('Ctrl Pts',(7.00303857133397,0.389665704772105,
25.2440323454718));
#155405=CARTESIAN_POINT('Ctrl Pts',(7.00845342637586,0.198007911004861,
25.2353494902476));
#155406=CARTESIAN_POINT('Ctrl Pts',(7.01030015932765,0.132643139375614,
25.2323882078616));
#155407=CARTESIAN_POINT('Ctrl Pts',(7.01123282932787,0.0672370078704981,
25.2294269254756));
#155408=CARTESIAN_POINT('Ctrl Pts',(7.0112497650765,0.00181499715977043,
25.2264656430896));
#155409=CARTESIAN_POINT('Ctrl Pts',(7.01124976619934,0.00181065449874002,
25.226465446522));
#155410=CARTESIAN_POINT('Ctrl Pts',(7.01130034097044,-0.194025907512635,
25.2176010389394));
#155411=CARTESIAN_POINT('Ctrl Pts',(7.00314147806038,-0.389720306454623,
25.2087366313568));
#155412=CARTESIAN_POINT('Ctrl Pts',(6.98683502308065,-0.584604928779768,
25.1998722237742));
#155413=CARTESIAN_POINT('Ctrl Pts',(6.97050530574478,-0.779767568337832,
25.1909951704629));
#155414=CARTESIAN_POINT('Ctrl Pts',(6.94600479014023,-0.974117878634766,
25.1821181171515));
#155415=CARTESIAN_POINT('Ctrl Pts',(6.91344697393,-1.16699507332213,25.1732410638402));
#155416=CARTESIAN_POINT('Ctrl Pts',(6.88082450327225,-1.3602552902731,25.1643463821666));
#155417=CARTESIAN_POINT('Ctrl Pts',(6.84011276527309,-1.55203629727069,
25.1554517004931));
#155418=CARTESIAN_POINT('Ctrl Pts',(6.79147657483599,-1.74168668133912,
25.1465570188195));
#155419=CARTESIAN_POINT('Ctrl Pts',(6.74279912605188,-1.93149794686815,
25.1376547917387));
#155420=CARTESIAN_POINT('Ctrl Pts',(6.68618386337597,-2.11917474334998,
25.1287525646579));
#155421=CARTESIAN_POINT('Ctrl Pts',(6.62184551843366,-2.304080834628,25.1198503375771));
#155422=CARTESIAN_POINT('Ctrl Pts',(6.55742811921313,-2.48921412506071,
25.1109371720872));
#155423=CARTESIAN_POINT('Ctrl Pts',(6.48526874591048,-2.67156967222017,
25.1020240065974));
#155424=CARTESIAN_POINT('Ctrl Pts',(6.40563111334279,-2.85052917934105,
25.0931108411075));
#155425=CARTESIAN_POINT('Ctrl Pts',(6.33519090890342,-3.008820477833,25.0852270658235));
#155426=CARTESIAN_POINT('Ctrl Pts',(6.25890078141443,-3.1644550562951,25.0773432905396));
#155427=CARTESIAN_POINT('Ctrl Pts',(6.17697358078289,-3.31702034133199,
25.0694595152557));
#155428=CARTESIAN_POINT('Ctrl Pts',(6.0952640285474,-3.46918032032493,25.0615966840664));
#155429=CARTESIAN_POINT('Ctrl Pts',(6.00780935259729,-3.61854067465449,
25.0537338528771));
#155430=CARTESIAN_POINT('Ctrl Pts',(5.91483458551074,-3.76461928865935,
25.0458710216878));
#155431=CARTESIAN_POINT('Ctrl Pts',(5.82193125726022,-3.91058566053142,
25.0380142320465));
#155432=CARTESIAN_POINT('Ctrl Pts',(5.72351647602592,-4.0532749870423,25.0301574424051));
#155433=CARTESIAN_POINT('Ctrl Pts',(5.61986173967537,-4.19222859460609,
25.0223006527637));
#155434=CARTESIAN_POINT('Ctrl Pts',(5.51626545968907,-4.33110383891333,
25.0144482939797));
#155435=CARTESIAN_POINT('Ctrl Pts',(5.40743533019381,-4.46624725046369,
25.0065959351958));
#155436=CARTESIAN_POINT('Ctrl Pts',(5.29368667357636,-4.59722829153612,
24.9987435764118));
#155437=CARTESIAN_POINT('Ctrl Pts',(5.17996487434422,-4.72817840645615,
24.9908930716614));
#155438=CARTESIAN_POINT('Ctrl Pts',(5.06132710274201,-4.85496781377019,
24.983042566911));
#155439=CARTESIAN_POINT('Ctrl Pts',(4.9381295137889,-4.97719835525439,24.9751920621605));
#155440=CARTESIAN_POINT('Ctrl Pts',(4.81495174344497,-5.09940923369686,
24.9673428203089));
#155441=CARTESIAN_POINT('Ctrl Pts',(4.68721588895584,-5.2170624396675,24.9594935784573));
#155442=CARTESIAN_POINT('Ctrl Pts',(4.55531523916441,-5.3297963970809,24.9516443366056));
#155443=CARTESIAN_POINT('Ctrl Pts',(4.42337014946246,-5.44256833677102,
24.9437924501908));
#155444=CARTESIAN_POINT('Ctrl Pts',(4.28725775193319,-5.55041746926412,
24.935940563776));
#155445=CARTESIAN_POINT('Ctrl Pts',(4.14740486204788,-5.65302215392454,
24.9280886773611));
#155446=CARTESIAN_POINT('Ctrl Pts',(4.04471262571944,-5.72836349677554,
24.9223231348972));
#155447=CARTESIAN_POINT('Ctrl Pts',(3.94000430801992,-5.80087797357664,
24.9165575924333));
#155448=CARTESIAN_POINT('Ctrl Pts',(3.83345880483282,-5.87045314725786,
24.9107920499693));
#155449=CARTESIAN_POINT('Ctrl Pts',(3.6550316632605,-5.98696767854257,24.9011367456094));
#155450=CARTESIAN_POINT('Ctrl Pts',(3.47154285546835,-6.09517901204503,
24.8914814412495));
#155451=CARTESIAN_POINT('Ctrl Pts',(3.28371893132749,-6.19474103918327,
24.8818261368895));
#155452=CARTESIAN_POINT('Ctrl Pts',(3.09485449788327,-6.2948546212737,24.8721173439548));
#155453=CARTESIAN_POINT('Ctrl Pts',(2.90160685089553,-6.38622282673731,
24.8624085510201));
#155454=CARTESIAN_POINT('Ctrl Pts',(2.70472898748495,-6.46854447822373,
24.8526997580854));
#155455=CARTESIAN_POINT('Ctrl Pts',(2.50690373107783,-6.5512622684874,24.8429442456146));
#155456=CARTESIAN_POINT('Ctrl Pts',(2.3054132855391,-6.62484623516559,24.8331887331439));
#155457=CARTESIAN_POINT('Ctrl Pts',(2.10103509685722,-6.68904164169085,
24.8234332206731));
#155458=CARTESIAN_POINT('Ctrl Pts',(1.89645454232499,-6.75330061154502,
24.8136680487442));
#155459=CARTESIAN_POINT('Ctrl Pts',(1.68898056530443,-6.80815242605906,
24.8039028768152));
#155460=CARTESIAN_POINT('Ctrl Pts',(1.47940575001441,-6.8533922395646,24.7941377048862));
#155461=CARTESIAN_POINT('Ctrl Pts',(1.27011668523058,-6.89857036961076,
24.7843858475476));
#155462=CARTESIAN_POINT('Ctrl Pts',(1.05873254427478,-6.93416268435699,
24.774633990209));
#155463=CARTESIAN_POINT('Ctrl Pts',(0.846054864332172,-6.96001564143644,
24.7648821328705));
#155464=CARTESIAN_POINT('Ctrl Pts',(0.753311993030767,-6.97128940308283,
24.7606296168079));
#155465=CARTESIAN_POINT('Ctrl Pts',(0.660323296768818,-6.98071178572341,
24.7563771007454));
#155466=CARTESIAN_POINT('Ctrl Pts',(0.567155942728443,-6.98827308418381,
24.7521245846828));
#155467=CARTESIAN_POINT('Ctrl Pts',(0.391161874200898,-7.0025564530001,
24.744091539084));
#155468=CARTESIAN_POINT('Ctrl Pts',(0.214444101747245,-7.01020201969531,
24.7360584934852));
#155469=CARTESIAN_POINT('Ctrl Pts',(0.0375509995440148,-7.01114944106409,
24.7280254478864));
#155470=CARTESIAN_POINT('Ctrl Pts',(-0.139228388962544,-7.01209625339393,
24.7199975662386));
#155471=CARTESIAN_POINT('Ctrl Pts',(-0.316182517834179,-7.00635348929287,
24.7119696845908));
#155472=CARTESIAN_POINT('Ctrl Pts',(-0.492759034396457,-6.99391271725067,
24.7039418029429));
#155473=CARTESIAN_POINT('Ctrl Pts',(-0.669255824920628,-6.98147756233971,
24.6959175459628));
#155474=CARTESIAN_POINT('Ctrl Pts',(-0.845374977707885,-6.96235044675952,
24.6878932889827));
#155475=CARTESIAN_POINT('Ctrl Pts',(-1.02056533453558,-6.93657501656576,
24.6798690320026));
#155476=CARTESIAN_POINT('Ctrl Pts',(-1.1957345090647,-6.91080270288405,
24.6718457452369));
#155477=CARTESIAN_POINT('Ctrl Pts',(-1.36997474774258,-6.87838372141819,
24.6638224584712));
#155478=CARTESIAN_POINT('Ctrl Pts',(-1.54274102339802,-6.83941347611218,
24.6557991717055));
#155479=CARTESIAN_POINT('Ctrl Pts',(-1.71549314239819,-6.80044642407017,
24.6477765423766));
#155480=CARTESIAN_POINT('Ctrl Pts',(-1.88677118217955,-6.75492926207253,
24.6397539130477));
#155481=CARTESIAN_POINT('Ctrl Pts',(-2.05604160109105,-6.70300824235529,
24.6317312837188));
#155482=CARTESIAN_POINT('Ctrl Pts',(-2.22537565362933,-6.65106770403101,
24.6237056384524));
#155483=CARTESIAN_POINT('Ctrl Pts',(-2.3927002278046,-6.5927186092541,24.615679993186));
#155484=CARTESIAN_POINT('Ctrl Pts',(-2.5574978394213,-6.52815681213736,
24.6076543479196));
#155485=CARTESIAN_POINT('Ctrl Pts',(-2.65467255350088,-6.49008724235576,
24.6029219384119));
#155486=CARTESIAN_POINT('Ctrl Pts',(-2.75096898407471,-6.44985844336345,
24.5981895289042));
#155487=CARTESIAN_POINT('Ctrl Pts',(-2.84628447904216,-6.40751833605365,
24.5934571193964));
#155488=CARTESIAN_POINT('Ctrl Pts',(-3.02211645732037,-6.32941199215503,
24.5847270705618));
#155489=CARTESIAN_POINT('Ctrl Pts',(-3.19469706244835,-6.24407939971261,
24.5759970217271));
#155490=CARTESIAN_POINT('Ctrl Pts',(-3.36345017752334,-6.15181513586179,
24.5672669728924));
#155491=CARTESIAN_POINT('Ctrl Pts',(-3.53225208777275,-6.05952419368361,
24.5585343997532));
#155492=CARTESIAN_POINT('Ctrl Pts',(-3.69722405852661,-5.96029771081905,
24.549801826614));
#155493=CARTESIAN_POINT('Ctrl Pts',(-3.8578156658095,-5.85447562563333,
24.5410692534748));
#155494=CARTESIAN_POINT('Ctrl Pts',(-4.02068873322492,-5.74715016880462,
24.5322126201944));
#155495=CARTESIAN_POINT('Ctrl Pts',(-4.17905578646859,-5.63304043873814,
24.523355986914));
#155496=CARTESIAN_POINT('Ctrl Pts',(-4.33237374851257,-5.51254607832888,
24.5144993536336));
#155497=CARTESIAN_POINT('Ctrl Pts',(-4.48364032625899,-5.3936639245756,
24.5057612215268));
#155498=CARTESIAN_POINT('Ctrl Pts',(-4.62999188266194,-5.26856712115267,
24.4970230894201));
#155499=CARTESIAN_POINT('Ctrl Pts',(-4.77094005590083,-5.13768017158533,
24.4882849573133));
#155500=CARTESIAN_POINT('Ctrl Pts',(-4.914755407802,-5.00413070954728,24.4793690734461));
#155501=CARTESIAN_POINT('Ctrl Pts',(-5.05294497010798,-4.86455320968231,
24.4704531895789));
#155502=CARTESIAN_POINT('Ctrl Pts',(-5.18502865944739,-4.7194389881859,
24.4615373057117));
#155503=CARTESIAN_POINT('Ctrl Pts',(-5.31711234878681,-4.57432476668949,
24.4526214218445));
#155504=CARTESIAN_POINT('Ctrl Pts',(-5.44308996609738,-4.4236740512991,
24.4437055379772));
#155505=CARTESIAN_POINT('Ctrl Pts',(-5.56252360649249,-4.26801566184027,
24.43478965411));
#155506=CARTESIAN_POINT('Ctrl Pts',(-5.6796103456734,-4.11541599906859,
24.4260489696138));
#155507=CARTESIAN_POINT('Ctrl Pts',(-5.79042033807267,-3.95798743193461,
24.4173082851176));
#155508=CARTESIAN_POINT('Ctrl Pts',(-5.8945786984682,-3.79625717385756,
24.4085676006214));
#155509=CARTESIAN_POINT('Ctrl Pts',(-5.99871831904458,-3.63455601374034,
24.3998284887195));
#155510=CARTESIAN_POINT('Ctrl Pts',(-6.09620854940289,-3.4685549384139,
24.3910893768176));
#155511=CARTESIAN_POINT('Ctrl Pts',(-6.18671818027138,-3.29880959141318,
24.3823502649158));
#155512=CARTESIAN_POINT('Ctrl Pts',(-6.27840049367379,-3.12686494913601,
24.3734979252414));
#155513=CARTESIAN_POINT('Ctrl Pts',(-6.36291990525879,-2.95107857488779,
24.3646455855671));
#155514=CARTESIAN_POINT('Ctrl Pts',(-6.43997990604259,-2.77205435954413,
24.3557932458927));
#155515=CARTESIAN_POINT('Ctrl Pts',(-6.51601526207242,-2.59541057790436,
24.347058613243));
#155516=CARTESIAN_POINT('Ctrl Pts',(-6.58478824835879,-2.41561478928434,
24.3383239805932));
#155517=CARTESIAN_POINT('Ctrl Pts',(-6.64606178443819,-2.23326875228448,
24.3295893479435));
#155518=CARTESIAN_POINT('Ctrl Pts',(-6.70857389446358,-2.04723680020555,
24.3206781547568));
#155519=CARTESIAN_POINT('Ctrl Pts',(-6.7632800266861,-1.8585506693559,24.3117669615702));
#155520=CARTESIAN_POINT('Ctrl Pts',(-6.80998104715273,-1.66786831012541,
24.3028557683836));
#155521=CARTESIAN_POINT('Ctrl Pts',(-6.85668206761938,-1.47718595089489,
24.2939445751969));
#155522=CARTESIAN_POINT('Ctrl Pts',(-6.89537789113301,-1.28450765450624,
24.2850333820103));
#155523=CARTESIAN_POINT('Ctrl Pts',(-6.92592396116732,-1.09050623410796,
24.2761221888236));
#155524=CARTESIAN_POINT('Ctrl Pts',(-6.95343458915158,-0.915783237041549,
24.2680965239712));
#155525=CARTESIAN_POINT('Ctrl Pts',(-6.97434683907059,-0.739906637125955,
24.2600708591188));
#155526=CARTESIAN_POINT('Ctrl Pts',(-6.9885750816751,-0.563422479396998,
24.2520451942664));
#155527=CARTESIAN_POINT('Ctrl Pts',(-7.00279880858434,-0.386994333411741,
24.2440220765632));
#155528=CARTESIAN_POINT('Ctrl Pts',(-7.0103427221453,-0.209959378457967,
24.23599895886));
#155529=CARTESIAN_POINT('Ctrl Pts',(-7.01117295096849,-0.0328696532956069,
24.2279758411568));
#155530=CARTESIAN_POINT('Ctrl Pts',(-7.01200307509257,0.144197739303647,
24.2199537352389));
#155531=CARTESIAN_POINT('Ctrl Pts',(-7.00612119979062,0.321319521888407,
24.211931629321));
#155532=CARTESIAN_POINT('Ctrl Pts',(-6.9935455602307,0.497942827518838,
24.2039095234031));
#155533=CARTESIAN_POINT('Ctrl Pts',(-6.98096524752066,0.674631766966055,
24.1958844364435));
#155534=CARTESIAN_POINT('Ctrl Pts',(-6.96168622452858,0.85082149321643,
24.187859349484));
#155535=CARTESIAN_POINT('Ctrl Pts',(-6.9357787249994,1.02596298195681,24.1798342625244));
#155536=CARTESIAN_POINT('Ctrl Pts',(-6.90986612311783,1.201138963937,24.1718075950642));
#155537=CARTESIAN_POINT('Ctrl Pts',(-6.87732250639086,1.37526593580663,
24.1637809276039));
#155538=CARTESIAN_POINT('Ctrl Pts',(-6.83826936653071,1.54780445575909,
24.1557542601437));
#155539=CARTESIAN_POINT('Ctrl Pts',(-6.79918487494756,1.72048148902712,
24.1477211489031));
#155540=CARTESIAN_POINT('Ctrl Pts',(-6.75358051292866,1.89156716807226,
24.1396880376624));
#155541=CARTESIAN_POINT('Ctrl Pts',(-6.70162800408928,2.06053601213529,
24.1316549264218));
#155542=CARTESIAN_POINT('Ctrl Pts',(-6.67101569860373,2.16009859318383,
24.1269215254603));
#155543=CARTESIAN_POINT('Ctrl Pts',(-6.63820025694798,2.25892652538069,
24.1221881244987));
#155544=CARTESIAN_POINT('Ctrl Pts',(-6.60322465143547,2.35691551931225,
24.1174547235371));
#155545=CARTESIAN_POINT('Ctrl Pts',(-6.5311738155657,2.55877589643372,24.1077037702429));
#155546=CARTESIAN_POINT('Ctrl Pts',(-6.44991144028197,2.75719415864556,
24.0979528169488));
#155547=CARTESIAN_POINT('Ctrl Pts',(-6.35977319226589,2.95142533455213,
24.0882018636546));
#155548=CARTESIAN_POINT('Ctrl Pts',(-6.26950508319346,3.14593633690568,
24.0784368622829));
#155549=CARTESIAN_POINT('Ctrl Pts',(-6.17033553916897,3.33624815156836,
24.0686718609112));
#155550=CARTESIAN_POINT('Ctrl Pts',(-6.0626476800497,3.52163735641364,24.0589068595395));
#155551=CARTESIAN_POINT('Ctrl Pts',(-5.95513931428039,3.7067175558641,24.0491581344019));
#155552=CARTESIAN_POINT('Ctrl Pts',(-5.83914102902578,3.88689151112113,
24.0394094092644));
#155553=CARTESIAN_POINT('Ctrl Pts',(-5.71507941112824,4.0614645002755,24.0296606841268));
#155554=CARTESIAN_POINT('Ctrl Pts',(-5.59135829426732,4.23555835426478,
24.0199387154597));
#155555=CARTESIAN_POINT('Ctrl Pts',(-5.45961804826436,4.40408189824422,
24.0102167467926));
#155556=CARTESIAN_POINT('Ctrl Pts',(-5.32032672708516,4.56637165368341,
24.0004947781255));
#155557=CARTESIAN_POINT('Ctrl Pts',(-5.1819570601973,4.72758758019861,23.9908371371859));
#155558=CARTESIAN_POINT('Ctrl Pts',(-5.03613592331542,4.88265188598419,
23.9811794962462));
#155559=CARTESIAN_POINT('Ctrl Pts',(-4.88336645422707,5.03094013443112,
23.9715218553065));
#155560=CARTESIAN_POINT('Ctrl Pts',(-4.81621901303099,5.09611792487628,
23.9672769896213));
#155561=CARTESIAN_POINT('Ctrl Pts',(-4.7477297973509,5.15998698885246,23.963032123936));
#155562=CARTESIAN_POINT('Ctrl Pts',(-4.67794426613782,5.22249595551862,
23.9587872582507));
#155563=CARTESIAN_POINT('Ctrl Pts',(-4.54886001342004,5.33812054287933,
23.9509354112368));
#155564=CARTESIAN_POINT('Ctrl Pts',(-4.41539090845914,5.44904124456702,
23.9430835642229));
#155565=CARTESIAN_POINT('Ctrl Pts',(-4.27793297718134,5.55490017959319,
23.935231717209));
#155566=CARTESIAN_POINT('Ctrl Pts',(-4.14051402786141,5.66072909388133,
23.9273820969154));
#155567=CARTESIAN_POINT('Ctrl Pts',(-3.99910880430221,5.76149886439373,
23.9195324766218));
#155568=CARTESIAN_POINT('Ctrl Pts',(-3.85414661408788,5.8568917046173,23.9116828563283));
#155569=CARTESIAN_POINT('Ctrl Pts',(-3.70919599725087,5.95227692894233,
23.9038338627265));
#155570=CARTESIAN_POINT('Ctrl Pts',(-3.56068929815195,6.04228586848726,
23.8959848691247));
#155571=CARTESIAN_POINT('Ctrl Pts',(-3.40908478908445,6.12664406207289,
23.8881358755229));
#155572=CARTESIAN_POINT('Ctrl Pts',(-3.25740352709307,6.21104496374189,
23.8802829082055));
#155573=CARTESIAN_POINT('Ctrl Pts',(-3.10262165529976,6.28978921769403,
23.8724299408881));
#155574=CARTESIAN_POINT('Ctrl Pts',(-2.94522233259348,6.36264818877271,
23.8645769735707));
#155575=CARTESIAN_POINT('Ctrl Pts',(-2.7877830357479,6.43552566358196,23.8567220118634));
#155576=CARTESIAN_POINT('Ctrl Pts',(-2.62772531559183,6.50251473050419,
23.8488670501562));
#155577=CARTESIAN_POINT('Ctrl Pts',(-2.46555167507444,6.56343519051096,
23.8410120884489));
#155578=CARTESIAN_POINT('Ctrl Pts',(-2.30321706366306,6.62441611916651,
23.8331493300356));
#155579=CARTESIAN_POINT('Ctrl Pts',(-2.13876269887763,6.67931628950445,
23.8252865716223));
#155580=CARTESIAN_POINT('Ctrl Pts',(-1.97270613491372,6.72800543012368,
23.817423813209));
#155581=CARTESIAN_POINT('Ctrl Pts',(-1.85088942235821,6.7637230850348,23.8116558064608));
#155582=CARTESIAN_POINT('Ctrl Pts',(-1.72821079585807,6.79609933591454,
23.8058877997125));
#155583=CARTESIAN_POINT('Ctrl Pts',(-1.60487744077216,6.82510036282256,
23.8001197929643));
#155584=CARTESIAN_POINT('Ctrl Pts',(-1.42573495907763,6.86722453862539,
23.7917417265233));
#155585=CARTESIAN_POINT('Ctrl Pts',(-1.24481405199267,6.90231937438808,
23.7833636600822));
#155586=CARTESIAN_POINT('Ctrl Pts',(-1.06269237914367,6.93024613342196,
23.7749855936412));
#155587=CARTESIAN_POINT('Ctrl Pts',(-0.880695238931423,6.9581537964697,
23.7666132560225));
#155588=CARTESIAN_POINT('Ctrl Pts',(-0.6974992938152,6.9789031051554,23.7582409184038));
#155589=CARTESIAN_POINT('Ctrl Pts',(-0.513692558391576,6.99240634674167,
23.749868580785));
#155590=CARTESIAN_POINT('Ctrl Pts',(-0.329984552450935,7.00590233523104,
23.7415007402625));
#155591=CARTESIAN_POINT('Ctrl Pts',(-0.145666737467837,7.01215999313698,
23.7331328997399));
#155592=CARTESIAN_POINT('Ctrl Pts',(0.0386671219871292,7.01114337438461,
23.7247650592174));
#155593=CARTESIAN_POINT('Ctrl Pts',(0.222928972394616,7.01012715276899,
23.7164004875475));
#155594=CARTESIAN_POINT('Ctrl Pts',(0.407206526552163,7.00184232297608,
23.7080359158776));
#155595=CARTESIAN_POINT('Ctrl Pts',(0.590904923462759,6.98630502726065,
23.6996713442077));
#155596=CARTESIAN_POINT('Ctrl Pts',(0.774558448575304,6.97077152682275,
23.6913088157421));
#155597=CARTESIAN_POINT('Ctrl Pts',(0.957632771375497,6.9479891214706,23.6829462872766));
#155598=CARTESIAN_POINT('Ctrl Pts',(1.13953659797897,6.91802593984487,23.6745837588111));
#155599=CARTESIAN_POINT('Ctrl Pts',(1.32145494107814,6.8880603670633,23.6662205629896));
#155600=CARTESIAN_POINT('Ctrl Pts',(1.50220227608055,6.8509129205959,23.6578573671681));
#155601=CARTESIAN_POINT('Ctrl Pts',(1.68119520104314,6.80670325917691,23.6494941713466));
#155602=CARTESIAN_POINT('Ctrl Pts',(1.86020033296453,6.7624905827476,23.6411304051719));
#155603=CARTESIAN_POINT('Ctrl Pts',(2.0374504969865,6.71121480962573,23.6327666389972));
#155604=CARTESIAN_POINT('Ctrl Pts',(2.21237503715055,6.65304616378792,23.6244028728225));
#155605=CARTESIAN_POINT('Ctrl Pts',(2.38733482837268,6.59486579571656,23.616037421169));
#155606=CARTESIAN_POINT('Ctrl Pts',(2.55996774922694,6.52978988886511,23.6076719695155));
#155607=CARTESIAN_POINT('Ctrl Pts',(2.72972038080205,6.45803787578967,23.5993065178619));
#155608=CARTESIAN_POINT('Ctrl Pts',(2.89952986220081,6.38626183310566,23.5909382646351));
#155609=CARTESIAN_POINT('Ctrl Pts',(3.06645682815355,6.30780535387567,23.5825700114082));
#155610=CARTESIAN_POINT('Ctrl Pts',(3.22996944406444,6.22293531646522,23.5742017581813));
#155611=CARTESIAN_POINT('Ctrl Pts',(3.39363365949794,6.13798659242204,23.5658257463898));
#155612=CARTESIAN_POINT('Ctrl Pts',(3.55387690697908,6.04661257937223,23.5574497345983));
#155613=CARTESIAN_POINT('Ctrl Pts',(3.7101924127613,5.94912588728701,23.5490737228068));
#155614=CARTESIAN_POINT('Ctrl Pts',(3.86658457759864,5.85159138652367,23.5406936033157));
#155615=CARTESIAN_POINT('Ctrl Pts',(4.01904488415931,5.74793840808889,23.5323134838245));
#155616=CARTESIAN_POINT('Ctrl Pts',(4.16709647387925,5.63852228335432,23.5239333643334));
#155617=CARTESIAN_POINT('Ctrl Pts',(4.31531723129459,5.52898113683716,23.5155436694942));
#155618=CARTESIAN_POINT('Ctrl Pts',(4.45911894529113,5.41366388626498,23.507153974655));
#155619=CARTESIAN_POINT('Ctrl Pts',(4.59805767416841,5.2929662938206,23.4987642798158));
#155620=CARTESIAN_POINT('Ctrl Pts',(4.68626747550549,5.21633747522254,23.493437807341));
#155621=CARTESIAN_POINT('Ctrl Pts',(4.77251783042629,5.13754074700647,23.4881113348662));
#155622=CARTESIAN_POINT('Ctrl Pts',(4.85670300396736,5.05668493123256,23.4827848623915));
#155623=CARTESIAN_POINT('Ctrl Pts',(4.9891814242929,4.9294457714459,23.4744028322823));
#155624=CARTESIAN_POINT('Ctrl Pts',(5.1168110448189,4.79684904428586,23.4660208021732));
#155625=CARTESIAN_POINT('Ctrl Pts',(5.23914763292184,4.65928735354984,23.457638772064));
#155626=CARTESIAN_POINT('Ctrl Pts',(5.36132838271575,4.52190089560071,23.4492674193934));
#155627=CARTESIAN_POINT('Ctrl Pts',(5.47822932135505,4.37956232150529,23.4408960667228));
#155628=CARTESIAN_POINT('Ctrl Pts',(5.58944166541492,4.23270226113575,23.4325247140521));
#155629=CARTESIAN_POINT('Ctrl Pts',(5.70048456162258,4.08606596299347,23.4241661163301));
#155630=CARTESIAN_POINT('Ctrl Pts',(5.80585595371169,3.93492217855557,23.415807518608));
#155631=CARTESIAN_POINT('Ctrl Pts',(5.90518623718454,3.77973571386497,23.407448920886));
#155632=CARTESIAN_POINT('Ctrl Pts',(6.00442800788643,3.62468753513838,23.3990977714729));
#155633=CARTESIAN_POINT('Ctrl Pts',(6.09763922092593,3.46560412870264,23.3907466220599));
#155634=CARTESIAN_POINT('Ctrl Pts',(6.18449185087015,3.30298154839241,23.3823954726469));
#155635=CARTESIAN_POINT('Ctrl Pts',(6.2712577169811,3.14052142439988,23.3740526658452));
#155636=CARTESIAN_POINT('Ctrl Pts',(6.35167751446895,2.9745294654463,23.3657098590435));
#155637=CARTESIAN_POINT('Ctrl Pts',(6.4254676812057,2.80552876304647,23.3573670522418));
#155638=CARTESIAN_POINT('Ctrl Pts',(6.47731514597153,2.68678315844126,23.3515051142516));
#155639=CARTESIAN_POINT('Ctrl Pts',(6.52589050575783,2.56655275647024,23.3456431762613));
#155640=CARTESIAN_POINT('Ctrl Pts',(6.57110895151814,2.44502632087637,23.3397812382711));
#155641=CARTESIAN_POINT('Origin',(0.,0.,50.));
#155642=CARTESIAN_POINT('',(6.57110895151816,2.44502632087631,21.3399745565681));
#155643=CARTESIAN_POINT('',(6.57110895151813,2.44502632087638,21.886801314899));
#155644=CARTESIAN_POINT('',(6.57110895151814,2.44502632087636,50.));
#155645=CARTESIAN_POINT('',(7.01124999042383,0.000366444892493489,23.7735343569435));
#155646=CARTESIAN_POINT('Ctrl Pts',(6.57110895151813,2.44502632087638,21.886801314899));
#155647=CARTESIAN_POINT('Ctrl Pts',(6.56903774075831,2.45059278510957,21.8870715001979));
#155648=CARTESIAN_POINT('Ctrl Pts',(6.56695953073157,2.45615641900482,21.8873416854967));
#155649=CARTESIAN_POINT('Ctrl Pts',(6.56487433029739,2.46171720347857,21.8876118707956));
#155650=CARTESIAN_POINT('Ctrl Pts',(6.48961971012513,2.66240521244526,21.8973628240897));
#155651=CARTESIAN_POINT('Ctrl Pts',(6.40520950384978,2.85950492703563,21.9071137773838));
#155652=CARTESIAN_POINT('Ctrl Pts',(6.31199119297193,3.0522768128636,21.9168647306779));
#155653=CARTESIAN_POINT('Ctrl Pts',(6.21863858362937,3.2453264227574,21.9266297320495));
#155654=CARTESIAN_POINT('Ctrl Pts',(6.11645250331447,3.434035697175,21.9363947334211));
#155655=CARTESIAN_POINT('Ctrl Pts',(6.00582753770331,3.61768740355832,21.9461597347927));
#155656=CARTESIAN_POINT('Ctrl Pts',(5.89538696098912,3.80103300059845,21.9559084599303));
#155657=CARTESIAN_POINT('Ctrl Pts',(5.77653563050745,3.97933784511388,21.9656571850678));
#155658=CARTESIAN_POINT('Ctrl Pts',(5.64971113660622,4.15191409297058,21.9754059102054));
#155659=CARTESIAN_POINT('Ctrl Pts',(5.52323472676498,4.32401668594277,21.9851278788725));
#155660=CARTESIAN_POINT('Ctrl Pts',(5.38882886346775,4.49042203803086,21.9948498475396));
#155661=CARTESIAN_POINT('Ctrl Pts',(5.24697210164763,4.6504742045335,22.0045718162067));
#155662=CARTESIAN_POINT('Ctrl Pts',(5.10605396896906,4.80946734765424,22.0142294571464));
#155663=CARTESIAN_POINT('Ctrl Pts',(4.957783222508,4.96219104795769,22.0238870980861));
#155664=CARTESIAN_POINT('Ctrl Pts',(4.80267287516415,5.10802895613,22.0335447390258));
#155665=CARTESIAN_POINT('Ctrl Pts',(4.73449653738069,5.17212973766682,22.0377896047112));
#155666=CARTESIAN_POINT('Ctrl Pts',(4.66499942543247,5.23490060216006,22.0420344703966));
#155667=CARTESIAN_POINT('Ctrl Pts',(4.59422781015614,5.29629090882364,22.0462793360821));
#155668=CARTESIAN_POINT('Ctrl Pts',(4.46331957011812,5.40984627942447,22.054131183096));
#155669=CARTESIAN_POINT('Ctrl Pts',(4.32810190270302,5.51862856870388,22.0619830301099));
#155670=CARTESIAN_POINT('Ctrl Pts',(4.18897647988422,5.62228624435619,22.0698348771238));
#155671=CARTESIAN_POINT('Ctrl Pts',(4.04989051191047,5.72591452352978,22.0776844974174));
#155672=CARTESIAN_POINT('Ctrl Pts',(3.9068992985402,5.82442085224993,22.085534117711));
#155673=CARTESIAN_POINT('Ctrl Pts',(3.7604371510249,5.91749431733498,22.0933837380046));
#155674=CARTESIAN_POINT('Ctrl Pts',(3.61398669663878,6.01056035169428,22.1012327316064));
#155675=CARTESIAN_POINT('Ctrl Pts',(3.46406618211453,6.09819418192184,22.1090817252082));
#155676=CARTESIAN_POINT('Ctrl Pts',(3.31113819015592,6.18012867569851,22.1169307188101));
#155677=CARTESIAN_POINT('Ctrl Pts',(3.15813277523306,6.26210465051015,22.1247836861275));
#155678=CARTESIAN_POINT('Ctrl Pts',(3.0021171773325,6.3383753432974,22.1326366534449));
#155679=CARTESIAN_POINT('Ctrl Pts',(2.84357813321102,6.40871983806627,22.1404896207624));
#155680=CARTESIAN_POINT('Ctrl Pts',(2.68499882549949,6.47908219797313,22.1483445824696));
#155681=CARTESIAN_POINT('Ctrl Pts',(2.523895149032,6.54351521976674,22.1561995441769));
#155682=CARTESIAN_POINT('Ctrl Pts',(2.36077241124134,6.6018467253354,22.1640545058842));
#155683=CARTESIAN_POINT('Ctrl Pts',(2.19748776049796,6.66023612979928,22.1719172642975));
#155684=CARTESIAN_POINT('Ctrl Pts',(2.03218040931206,6.71251180716714,22.1797800227109));
#155685=CARTESIAN_POINT('Ctrl Pts',(1.86536991978293,6.75855174019324,22.1876427811242));
#155686=CARTESIAN_POINT('Ctrl Pts',(1.74300013825431,6.79232597442694,22.1934107878723));
#155687=CARTESIAN_POINT('Ctrl Pts',(1.61982173543324,6.82274550924742,22.1991787946204));
#155688=CARTESIAN_POINT('Ctrl Pts',(1.49604240872844,6.84977982666494,22.2049468013685));
#155689=CARTESIAN_POINT('Ctrl Pts',(1.31625215042091,6.88904734444081,22.2133248678095));
#155690=CARTESIAN_POINT('Ctrl Pts',(1.1347955745208,6.92125810630837,22.2217029342505));
#155691=CARTESIAN_POINT('Ctrl Pts',(0.952252475682128,6.94628258747492,
22.2300810006915));
#155692=CARTESIAN_POINT('Ctrl Pts',(0.769834197645309,6.97128995719861,
22.2384533383103));
#155693=CARTESIAN_POINT('Ctrl Pts',(0.586331202535501,6.98912079856643,
22.246825675929));
#155694=CARTESIAN_POINT('Ctrl Pts',(0.402332826542288,6.99969676908839,
22.2551980135478));
#155695=CARTESIAN_POINT('Ctrl Pts',(0.218433282969056,7.01026705886043,
22.2635658540703));
#155696=CARTESIAN_POINT('Ctrl Pts',(0.0340392165147784,7.01359022894086,
22.2719336945929));
#155697=CARTESIAN_POINT('Ctrl Pts',(-0.150255111329594,7.00963978846412,
22.2803015351155));
#155698=CARTESIAN_POINT('Ctrl Pts',(-0.334477445569004,7.00569089120608,
22.2886661067855));
#155699=CARTESIAN_POINT('Ctrl Pts',(-0.518599790742253,6.99447405657695,
22.2970306784554));
#155700=CARTESIAN_POINT('Ctrl Pts',(-0.702027618134933,6.97601489289378,
22.3053952501253));
#155701=CARTESIAN_POINT('Ctrl Pts',(-0.88541063982203,6.95756023820941,
22.3137577785909));
#155702=CARTESIAN_POINT('Ctrl Pts',(-1.06809915534767,6.9318668157454,22.3221203070565));
#155703=CARTESIAN_POINT('Ctrl Pts',(-1.24950303009968,6.89901215684331,
22.3304828355221));
#155704=CARTESIAN_POINT('Ctrl Pts',(-1.43092138144848,6.86615487603664,
22.3388460313436));
#155705=CARTESIAN_POINT('Ctrl Pts',(-1.61105456272152,6.82613526966641,
22.3472092271651));
#155706=CARTESIAN_POINT('Ctrl Pts',(-1.78932115042715,6.77908226702804,
22.3555724229866));
#155707=CARTESIAN_POINT('Ctrl Pts',(-1.96759989555667,6.73202605546923,
22.3639361891613));
#155708=CARTESIAN_POINT('Ctrl Pts',(-2.14401147529566,6.67793557489219,
22.372299955336));
#155709=CARTESIAN_POINT('Ctrl Pts',(-2.31798801534422,6.61699011055786,
22.3806637215107));
#155710=CARTESIAN_POINT('Ctrl Pts',(-2.49199961540934,6.55603236440101,
22.3890291731643));
#155711=CARTESIAN_POINT('Ctrl Pts',(-2.66357488699754,6.48821698860045,
22.3973946248178));
#155712=CARTESIAN_POINT('Ctrl Pts',(-2.83216397390128,6.41377219640951,
22.4057600764714));
#155713=CARTESIAN_POINT('Ctrl Pts',(-3.00080952095862,6.3393024728041,22.4141283296982));
#155714=CARTESIAN_POINT('Ctrl Pts',(-3.16646658852308,6.25819903846777,
22.4224965829251));
#155715=CARTESIAN_POINT('Ctrl Pts',(-3.32860765713966,6.17073720290625,
22.430864836152));
#155716=CARTESIAN_POINT('Ctrl Pts',(-3.49089905365884,6.08319427774534,
22.4392408479434));
#155717=CARTESIAN_POINT('Ctrl Pts',(-3.64966764744425,5.98928132735308,
22.4476168597349));
#155718=CARTESIAN_POINT('Ctrl Pts',(-3.80441170460284,5.8893189881667,22.4559928715264));
#155719=CARTESIAN_POINT('Ctrl Pts',(-3.95923165015915,5.78930762621401,
22.4643729910175));
#155720=CARTESIAN_POINT('Ctrl Pts',(-4.11002285073835,5.6832411430872,22.4727531105087));
#155721=CARTESIAN_POINT('Ctrl Pts',(-4.25631416381568,5.57148241506711,
22.4811332299998));
#155722=CARTESIAN_POINT('Ctrl Pts',(-4.40277263324938,5.45959598854343,
22.4895229248391));
#155723=CARTESIAN_POINT('Ctrl Pts',(-4.5447206836691,5.34200452537568,22.4979126196783));
#155724=CARTESIAN_POINT('Ctrl Pts',(-4.68172072876112,5.21911080361286,
22.5063023145175));
#155725=CARTESIAN_POINT('Ctrl Pts',(-4.76869969321592,5.14108770041062,
22.5116287869921));
#155726=CARTESIAN_POINT('Ctrl Pts',(-4.85368495392768,5.06092814974724,
22.5169552594667));
#155727=CARTESIAN_POINT('Ctrl Pts',(-4.93657252139366,4.97874264282871,
22.5222817319414));
#155728=CARTESIAN_POINT('Ctrl Pts',(-5.066997602171,4.8494222669717,22.5306630323462));
#155729=CARTESIAN_POINT('Ctrl Pts',(-5.19249008304699,4.71482309815738,
22.5390443327511));
#155730=CARTESIAN_POINT('Ctrl Pts',(-5.31261214947924,4.57534465496378,
22.547425633156));
#155731=CARTESIAN_POINT('Ctrl Pts',(-5.43258197877688,4.43604298027876,
22.5557963114895));
#155732=CARTESIAN_POINT('Ctrl Pts',(-5.54719474562594,4.29187460107555,
22.5641669898231));
#155733=CARTESIAN_POINT('Ctrl Pts',(-5.65604866497901,4.14327648870905,
22.5725376681566));
#155734=CARTESIAN_POINT('Ctrl Pts',(-5.76477905382293,3.99484700968703,
22.5808988472075));
#155735=CARTESIAN_POINT('Ctrl Pts',(-5.86776342830181,3.84199807955139,
22.5892600262583));
#155736=CARTESIAN_POINT('Ctrl Pts',(-5.96463929270588,3.68520076392171,
22.5976212053091));
#155737=CARTESIAN_POINT('Ctrl Pts',(-6.06138944924839,3.5286069113049,22.6059715347438));
#155738=CARTESIAN_POINT('Ctrl Pts',(-6.15204673458099,3.36807516997443,
22.6143218641785));
#155739=CARTESIAN_POINT('Ctrl Pts',(-6.23629115844561,3.20410660708928,
22.6226721936132));
#155740=CARTESIAN_POINT('Ctrl Pts',(-6.32047076126546,3.04026420820486,
22.6310160979689));
#155741=CARTESIAN_POINT('Ctrl Pts',(-6.39824718670623,2.87299054782822,
22.6393600023246));
#155742=CARTESIAN_POINT('Ctrl Pts',(-6.46934513065601,2.7028133755325,22.6477039066804));
#155743=CARTESIAN_POINT('Ctrl Pts',(-6.54038596829378,2.53277289060295,
22.6560411091601));
#155744=CARTESIAN_POINT('Ctrl Pts',(-6.60475889662637,2.35983384628395,
22.6643783116398));
#155745=CARTESIAN_POINT('Ctrl Pts',(-6.66223566239289,2.18454630100633,
22.6727155141195));
#155746=CARTESIAN_POINT('Ctrl Pts',(-6.68115669641936,2.12684260866413,
22.6754600751556));
#155747=CARTESIAN_POINT('Ctrl Pts',(-6.69933078347864,2.06888458268803,
22.6782046361917));
#155748=CARTESIAN_POINT('Ctrl Pts',(-6.71675092208239,2.01069232186463,
22.6809491972278));
#155749=CARTESIAN_POINT('Ctrl Pts',(-6.76967542231021,1.83389715442881,
22.6892875075297));
#155750=CARTESIAN_POINT('Ctrl Pts',(-6.81559374010498,1.6550838305122,22.6976258178316));
#155751=CARTESIAN_POINT('Ctrl Pts',(-6.85437739256016,1.47483460864606,
22.7059641281335));
#155752=CARTESIAN_POINT('Ctrl Pts',(-6.89318544637344,1.29447198008583,
22.7143076846173));
#155753=CARTESIAN_POINT('Ctrl Pts',(-6.92484981227702,1.11267197191541,
22.7226512411012));
#155754=CARTESIAN_POINT('Ctrl Pts',(-6.94929344594818,0.930025356967012,
22.730994797585));
#155755=CARTESIAN_POINT('Ctrl Pts',(-6.9737556762293,0.747239785270095,
22.7393447018102));
#155756=CARTESIAN_POINT('Ctrl Pts',(-6.9909861731223,0.563606646424557,
22.7476946060354));
#155757=CARTESIAN_POINT('Ctrl Pts',(-7.00095985196023,0.379720573239007,
22.7560445102606));
#155758=CARTESIAN_POINT('Ctrl Pts',(-7.01094849057836,0.195558684551334,
22.7644069387243));
#155759=CARTESIAN_POINT('Ctrl Pts',(-7.01365854234677,0.0111434308513623,
22.772769367188));
#155760=CARTESIAN_POINT('Ctrl Pts',(-7.00911703962814,-0.1729302960572,
22.7811317956516));
#155761=CARTESIAN_POINT('Ctrl Pts',(-7.00457165330559,-0.357161431095265,
22.7895013751316));
#155762=CARTESIAN_POINT('Ctrl Pts',(-6.99276236071042,-0.541050130422998,
22.7978709546116));
#155763=CARTESIAN_POINT('Ctrl Pts',(-6.9737679902753,-0.724007306808131,
22.8062405340916));
#155764=CARTESIAN_POINT('Ctrl Pts',(-6.95474432333805,-0.9072466723465,
22.8146230226281));
#155765=CARTESIAN_POINT('Ctrl Pts',(-6.92851347977865,-1.08955132018455,
22.8230055111647));
#155766=CARTESIAN_POINT('Ctrl Pts',(-6.89520548792601,-1.27034162404253,
22.8313879997013));
#155767=CARTESIAN_POINT('Ctrl Pts',(-6.88430656720839,-1.32949917388767,
22.8341308873056));
#155768=CARTESIAN_POINT('Ctrl Pts',(-6.87265029112042,-1.38849469943956,
22.8368737749099));
#155769=CARTESIAN_POINT('Ctrl Pts',(-6.86024236830183,-1.44730826386657,
22.8396166625142));
#155770=CARTESIAN_POINT('Ctrl Pts',(-6.8222894187228,-1.62720527627531,
22.848006517647));
#155771=CARTESIAN_POINT('Ctrl Pts',(-6.77722367748968,-1.80576193640548,
22.8563963727798));
#155772=CARTESIAN_POINT('Ctrl Pts',(-6.72515683921751,-1.98239553329449,
22.8647862279126));
#155773=CARTESIAN_POINT('Ctrl Pts',(-6.67313804749378,-2.1588661351765,
22.8731683410047));
#155774=CARTESIAN_POINT('Ctrl Pts',(-6.61413113025516,-2.33341689764163,
22.8815504540967));
#155775=CARTESIAN_POINT('Ctrl Pts',(-6.5482985336932,-2.50547657664796,
22.8899325671888));
#155776=CARTESIAN_POINT('Ctrl Pts',(-6.48251700927337,-2.6774027738103,
22.8983081775377));
#155777=CARTESIAN_POINT('Ctrl Pts',(-6.4099204797556,-2.84684143451612,
22.9066837878866));
#155778=CARTESIAN_POINT('Ctrl Pts',(-6.3307209387802,-3.01323728866314,
22.9150593982354));
#155779=CARTESIAN_POINT('Ctrl Pts',(-6.25157121549219,-3.17952847734691,
22.923429740201));
#155780=CARTESIAN_POINT('Ctrl Pts',(-6.16582690315162,-3.3427803797026,
22.9318000821666));
#155781=CARTESIAN_POINT('Ctrl Pts',(-6.07374793431425,-3.50245807868037,
22.9401704241322));
#155782=CARTESIAN_POINT('Ctrl Pts',(-5.98171338677288,-3.66205874497174,
22.9485367280265));
#155783=CARTESIAN_POINT('Ctrl Pts',(-5.88335044082126,-3.81808836213549,
22.9569030319208));
#155784=CARTESIAN_POINT('Ctrl Pts',(-5.77896496849237,-3.97003658112088,
22.9652693358151));
#155785=CARTESIAN_POINT('Ctrl Pts',(-5.67460868985427,-4.12194230444839,
22.9736332998887));
#155786=CARTESIAN_POINT('Ctrl Pts',(-5.5642334281146,-4.26976863416818,
22.9819972639624));
#155787=CARTESIAN_POINT('Ctrl Pts',(-5.44818868139861,-4.41303372459129,
22.990361228036));
#155788=CARTESIAN_POINT('Ctrl Pts',(-5.3321617920407,-4.55627676889777,
22.9987239050345));
#155789=CARTESIAN_POINT('Ctrl Pts',(-5.21046736398084,-4.69495971803971,
23.0070865820331));
#155790=CARTESIAN_POINT('Ctrl Pts',(-5.08349578478654,-4.82863305383185,
23.0154492590316));
#155791=CARTESIAN_POINT('Ctrl Pts',(-4.95652681970505,-4.96230363753426,
23.0238117638579));
#155792=CARTESIAN_POINT('Ctrl Pts',(-4.82428114676228,-5.09096457553647,
23.0321742686842));
#155793=CARTESIAN_POINT('Ctrl Pts',(-4.68718697469135,-5.2142022234263,
23.0405367735105));
#155794=CARTESIAN_POINT('Ctrl Pts',(-4.55007735146155,-5.33745376077946,
23.0489002208305));
#155795=CARTESIAN_POINT('Ctrl Pts',(-4.40811838440423,-5.45528057010076,
23.0572636681505));
#155796=CARTESIAN_POINT('Ctrl Pts',(-4.26177272291521,-5.56730813057046,
23.0656271154704));
#155797=CARTESIAN_POINT('Ctrl Pts',(-4.11534088898789,-5.67940165601611,
23.0739954874233));
#155798=CARTESIAN_POINT('Ctrl Pts',(-3.96451745982217,-5.78568890835989,
23.0823638593761));
#155799=CARTESIAN_POINT('Ctrl Pts',(-3.80979637388184,-5.88583708167808,
23.0907322313289));
#155800=CARTESIAN_POINT('Ctrl Pts',(-3.65502892946048,-5.9860152620064,
23.0991031106646));
#155801=CARTESIAN_POINT('Ctrl Pts',(-3.4963617784528,-6.08005052135353,
23.1074739900004));
#155802=CARTESIAN_POINT('Ctrl Pts',(-3.3343156297423,-6.16765480906286,
23.1158448693361));
#155803=CARTESIAN_POINT('Ctrl Pts',(-3.17213218108231,-6.25533332293784,
23.1242228412274));
#155804=CARTESIAN_POINT('Ctrl Pts',(-3.00656430585668,-6.33656982562772,
23.1326008131187));
#155805=CARTESIAN_POINT('Ctrl Pts',(-2.83815600844423,-6.41112291523349,
23.14097878501));
#155806=CARTESIAN_POINT('Ctrl Pts',(-2.73113116408414,-6.45850201076629,
23.146303054369));
#155807=CARTESIAN_POINT('Ctrl Pts',(-2.62295958427795,-6.50318283201215,
23.151627323728));
#155808=CARTESIAN_POINT('Ctrl Pts',(-2.5137846452561,-6.5451136980021,23.1569515930871));
#155809=CARTESIAN_POINT('Ctrl Pts',(-2.3525561164677,-6.60703680869905,
23.1648144242763));
#155810=CARTESIAN_POINT('Ctrl Pts',(-2.18880317525843,-6.66308866001819,
23.1726772554656));
#155811=CARTESIAN_POINT('Ctrl Pts',(-2.02301101936965,-6.71305094409457,
23.1805400866549));
#155812=CARTESIAN_POINT('Ctrl Pts',(-1.85734625286848,-6.76297483875054,
23.1883968762963));
#155813=CARTESIAN_POINT('Ctrl Pts',(-1.68964575032468,-6.80681836178494,
23.1962536659377));
#155814=CARTESIAN_POINT('Ctrl Pts',(-1.52041460455554,-6.84441129628796,
23.204110455579));
#155815=CARTESIAN_POINT('Ctrl Pts',(-1.3512788971414,-6.88198303015552,
23.211962814363));
#155816=CARTESIAN_POINT('Ctrl Pts',(-1.18061463466396,-6.91331110517384,
23.219815173147));
#155817=CARTESIAN_POINT('Ctrl Pts',(-1.00894174041677,-6.93827522709678,
23.2276675319309));
#155818=CARTESIAN_POINT('Ctrl Pts',(-0.837309380143093,-6.96323345469923,
23.2355180366813));
#155819=CARTESIAN_POINT('Ctrl Pts',(-0.664669237830203,-6.98183065663853,
23.2433685414318));
#155820=CARTESIAN_POINT('Ctrl Pts',(-0.491551030538751,-6.99399772282464,
23.2512190461822));
#155821=CARTESIAN_POINT('Ctrl Pts',(-0.318460672510607,-7.00616283171328,
23.2590682880338));
#155822=CARTESIAN_POINT('Ctrl Pts',(-0.144892783401678,-7.01189984029918,
23.2669175298855));
#155823=CARTESIAN_POINT('Ctrl Pts',(0.0286186714169425,-7.0111915916017,
23.2747667717371));
#155824=CARTESIAN_POINT('Ctrl Pts',(0.202188585640859,-7.01048310428137,
23.282618658152));
#155825=CARTESIAN_POINT('Ctrl Pts',(0.37570164573594,-7.00332502373086,
23.2904705445668));
#155826=CARTESIAN_POINT('Ctrl Pts',(0.548624559625237,-6.98975233145467,
23.2983224309817));
#155827=CARTESIAN_POINT('Ctrl Pts',(0.675599702965492,-6.9797860724522,
23.3040879734456));
#155828=CARTESIAN_POINT('Ctrl Pts',(0.802256653223391,-6.96636228414092,
23.3098535159095));
#155829=CARTESIAN_POINT('Ctrl Pts',(0.928386492953912,-6.94951257874973,
23.3156190583735));
#155830=CARTESIAN_POINT('Ctrl Pts',(1.13961067508076,-6.92129510659616,
23.3252743627334));
#155831=CARTESIAN_POINT('Ctrl Pts',(1.34924873525073,-6.88348348125073,
23.3349296670933));
#155832=CARTESIAN_POINT('Ctrl Pts',(1.5565243537746,-6.83628981967606,23.3445849714532));
#155833=CARTESIAN_POINT('Ctrl Pts',(1.76494824034017,-6.78883471406981,
23.3542937643879));
#155834=CARTESIAN_POINT('Ctrl Pts',(1.97098340393757,-6.73189339868861,
23.3640025573226));
#155835=CARTESIAN_POINT('Ctrl Pts',(2.17386282224807,-6.66572929187405,
23.3737113502573));
#155836=CARTESIAN_POINT('Ctrl Pts',(2.37771851354603,-6.59924679775948,
23.383466862728));
#155837=CARTESIAN_POINT('Ctrl Pts',(2.57838798136036,-6.52345257316277,
23.3932223751987));
#155838=CARTESIAN_POINT('Ctrl Pts',(2.77511600001003,-6.43866117675005,
23.4029778876694));
#155839=CARTESIAN_POINT('Ctrl Pts',(2.97203880966447,-6.35378582380986,
23.4127430595983));
#155840=CARTESIAN_POINT('Ctrl Pts',(3.16501233319539,-6.25989550529004,
23.4225082315272));
#155841=CARTESIAN_POINT('Ctrl Pts',(3.35330244682744,-6.15735245560956,
23.4322734034561));
#155842=CARTESIAN_POINT('Ctrl Pts',(3.54133583116123,-6.05494922105097,
23.4420252607947));
#155843=CARTESIAN_POINT('Ctrl Pts',(3.72469853505676,-5.94391685308443,
23.4517771181332));
#155844=CARTESIAN_POINT('Ctrl Pts',(3.90268314413615,-5.82466229398543,
23.4615289754717));
#155845=CARTESIAN_POINT('Ctrl Pts',(3.98029732395359,-5.77265866939207,
23.4657814915344));
#155846=CARTESIAN_POINT('Ctrl Pts',(4.05688911734959,-5.71909211161391,
23.4700340075972));
#155847=CARTESIAN_POINT('Ctrl Pts',(4.13240130821906,-5.66399911637788,
23.4742865236599));
#155848=CARTESIAN_POINT('Ctrl Pts',(4.27504459599879,-5.55992789445181,
23.4823195692587));
#155849=CARTESIAN_POINT('Ctrl Pts',(4.41390286247934,-5.45035596546787,
23.4903526148575));
#155850=CARTESIAN_POINT('Ctrl Pts',(4.54852131076749,-5.33559560386599,
23.4983856604564));
#155851=CARTESIAN_POINT('Ctrl Pts',(4.68305322113387,-5.22090901464315,
23.5064135421042));
#155852=CARTESIAN_POINT('Ctrl Pts',(4.81335046072091,-5.10104086866477,
23.514441423752));
#155853=CARTESIAN_POINT('Ctrl Pts',(4.9389891074563,-4.9763453617015,23.5224693053999));
#155854=CARTESIAN_POINT('Ctrl Pts',(5.06457102710433,-4.8517061559887,23.53049356238));
#155855=CARTESIAN_POINT('Ctrl Pts',(5.18549828237431,-4.72224418681631,
23.5385178193601));
#155856=CARTESIAN_POINT('Ctrl Pts',(5.30138185290725,-4.58835231996909,
23.5465420763403));
#155857=CARTESIAN_POINT('Ctrl Pts',(5.417251411936,-4.45447664201253,23.554565363106));
#155858=CARTESIAN_POINT('Ctrl Pts',(5.5280782553281,-4.31617240520948,23.5625886498717));
#155859=CARTESIAN_POINT('Ctrl Pts',(5.6335117953184,-4.17386768052228,23.5706119366374));
#155860=CARTESIAN_POINT('Ctrl Pts',(5.73893669597062,-4.03157461643784,
23.5786345659664));
#155861=CARTESIAN_POINT('Ctrl Pts',(5.83896895847041,-3.88528201441365,
23.5866571952953));
#155862=CARTESIAN_POINT('Ctrl Pts',(5.9332998899645,-3.73544896608791,23.5946798246243));
#155863=CARTESIAN_POINT('Ctrl Pts',(6.02766628317316,-3.58555959120303,
23.6027054698907));
#155864=CARTESIAN_POINT('Ctrl Pts',(6.11632687089674,-3.43212742323012,
23.6107311151571));
#155865=CARTESIAN_POINT('Ctrl Pts',(6.19901750484803,-3.27563864568236,
23.6187567604235));
#155866=CARTESIAN_POINT('Ctrl Pts',(6.24777694154283,-3.18336332648741,
23.6234891699311));
#155867=CARTESIAN_POINT('Ctrl Pts',(6.29446148932374,-3.09002570380697,
23.6282215794388));
#155868=CARTESIAN_POINT('Ctrl Pts',(6.33902467059575,-2.99572909123613,
23.6329539889464));
#155869=CARTESIAN_POINT('Ctrl Pts',(6.42123645572228,-2.82176725481528,
23.6416845109259));
#155870=CARTESIAN_POINT('Ctrl Pts',(6.49626706470883,-2.6444536424203,23.6504150329054));
#155871=CARTESIAN_POINT('Ctrl Pts',(6.56387238010522,-2.46438753855636,
23.6591455548849));
#155872=CARTESIAN_POINT('Ctrl Pts',(6.6314977521916,-2.28426801389257,23.6678786669769));
#155873=CARTESIAN_POINT('Ctrl Pts',(6.69169333708936,-2.10139462394241,
23.6766117790689));
#155874=CARTESIAN_POINT('Ctrl Pts',(6.74426407861609,-1.91638425175869,
23.6853448911609));
#155875=CARTESIAN_POINT('Ctrl Pts',(6.7968591561174,-1.73128823483065,23.694082045973));
#155876=CARTESIAN_POINT('Ctrl Pts',(6.84182226067417,-1.54405352189869,
23.7028192007851));
#155877=CARTESIAN_POINT('Ctrl Pts',(6.87900855322177,-1.35531099279898,
23.7115563555972));
#155878=CARTESIAN_POINT('Ctrl Pts',(6.91620003221789,-1.16654213939147,
23.7202947289982));
#155879=CARTESIAN_POINT('Ctrl Pts',(6.94561248434305,-0.976265319218672,
23.7290331023993));
#155880=CARTESIAN_POINT('Ctrl Pts',(6.96715235187015,-0.785120798559216,
23.7377714758003));
#155881=CARTESIAN_POINT('Ctrl Pts',(6.98869753821513,-0.593929078774995,
23.7465120069591));
#155882=CARTESIAN_POINT('Ctrl Pts',(7.00236622588051,-0.401869502479807,
23.7552525381179));
#155883=CARTESIAN_POINT('Ctrl Pts',(7.00811668633663,-0.209587865083013,
23.7639930692767));
#155884=CARTESIAN_POINT('Ctrl Pts',(7.01020911436883,-0.139622078649738,
23.7671734984879));
#155885=CARTESIAN_POINT('Ctrl Pts',(7.01125364863884,-0.0696269189312333,
23.7703539276992));
#155886=CARTESIAN_POINT('Ctrl Pts',(7.01124999042387,0.000366444167520355,
23.7735343569105));
#155887=CARTESIAN_POINT('Ctrl Pts',(7.01124999042383,0.000366444892447644,
23.7735343569434));
#155888=CARTESIAN_POINT('Ctrl Pts',(7.01124305565533,0.133050503538856,
23.7795633893733));
#155889=CARTESIAN_POINT('Ctrl Pts',(7.00746885027521,0.265723050043453,
23.785592421803));
#155890=CARTESIAN_POINT('Ctrl Pts',(6.99993417826157,0.398180941916439,
23.7916214542327));
#155891=CARTESIAN_POINT('Ctrl Pts',(6.98901051473158,0.590216566040994,
23.8003622622672));
#155892=CARTESIAN_POINT('Ctrl Pts',(6.97017950023319,0.781812626957233,
23.8091030703016));
#155893=CARTESIAN_POINT('Ctrl Pts',(6.94350132643035,0.972324993178723,
23.8178438783361));
#155894=CARTESIAN_POINT('Ctrl Pts',(6.91682833312505,1.16280036478232,23.826582989038));
#155895=CARTESIAN_POINT('Ctrl Pts',(6.88231126202484,1.35219219094782,23.8353220997399));
#155896=CARTESIAN_POINT('Ctrl Pts',(6.84006194747097,1.53986334369634,23.8440612104418));
#155897=CARTESIAN_POINT('Ctrl Pts',(6.79782233411896,1.72749140377562,23.8527983144869));
#155898=CARTESIAN_POINT('Ctrl Pts',(6.7478540829149,1.91339931244425,23.8615354185319));
#155899=CARTESIAN_POINT('Ctrl Pts',(6.69031993997926,2.09696105429165,23.870272522577));
#155900=CARTESIAN_POINT('Ctrl Pts',(6.65363953994698,2.21398927054781,23.8758427884251));
#155901=CARTESIAN_POINT('Ctrl Pts',(6.61388493874407,2.33006409320201,23.8814130542733));
#155902=CARTESIAN_POINT('Ctrl Pts',(6.57110895151814,2.44502632087635,23.8869833201214));
#155903=CARTESIAN_POINT('',(7.01124707280511,-0.00640676063125135,23.2264656431175));
#155904=CARTESIAN_POINT('Ctrl Pts',(6.57110895151814,2.44502632087637,23.3397812382711));
#155905=CARTESIAN_POINT('Ctrl Pts',(6.61138542398337,2.33678164208002,23.3345599578824));
#155906=CARTESIAN_POINT('Ctrl Pts',(6.64899878954924,2.22750884430548,23.3293386774937));
#155907=CARTESIAN_POINT('Ctrl Pts',(6.68389688264738,2.11734480532496,23.324117397105));
#155908=CARTESIAN_POINT('Ctrl Pts',(6.73828743675399,1.94564822849709,23.3159797509394));
#155909=CARTESIAN_POINT('Ctrl Pts',(6.78605493295745,1.77186261854152,23.3078421047737));
#155910=CARTESIAN_POINT('Ctrl Pts',(6.82705109833992,1.59655875656229,23.2997044586081));
#155911=CARTESIAN_POINT('Ctrl Pts',(6.86695367326194,1.42593120099738,23.2917838876771));
#155912=CARTESIAN_POINT('Ctrl Pts',(6.90044152218367,1.25386574377418,23.283863316746));
#155913=CARTESIAN_POINT('Ctrl Pts',(6.9274298551555,1.08089877620446,23.275942745815));
#155914=CARTESIAN_POINT('Ctrl Pts',(6.95552767229742,0.900821176323035,
23.2676965620321));
#155915=CARTESIAN_POINT('Ctrl Pts',(6.97658018198758,0.719766819360145,
23.2594503782491));
#155916=CARTESIAN_POINT('Ctrl Pts',(6.99055149854557,0.53834590059025,23.2512041944662));
#155917=CARTESIAN_POINT('Ctrl Pts',(7.00452281510356,0.356924981820356,
23.2429580106833));
#155918=CARTESIAN_POINT('Ctrl Pts',(7.01141296534021,0.175137957219189,
23.2347118269004));
#155919=CARTESIAN_POINT('Ctrl Pts',(7.01124707280511,-0.00640676063126676,
23.2264656431175));
#155920=CARTESIAN_POINT('Ctrl Pts',(7.01124707280455,-0.00640676124481819,
23.2264656430896));
#155921=CARTESIAN_POINT('Ctrl Pts',(7.01104249227252,-0.230289718879575,
23.2162963578778));
#155922=CARTESIAN_POINT('Ctrl Pts',(7.00010998406549,-0.453798136458237,
23.206127072666));
#155923=CARTESIAN_POINT('Ctrl Pts',(6.97858319956031,-0.676020036178396,
23.1959577874541));
#155924=CARTESIAN_POINT('Ctrl Pts',(6.95705641505512,-0.898241935898589,
23.1857885022423));
#155925=CARTESIAN_POINT('Ctrl Pts',(6.92493548555938,-1.11917735600806,
23.1756192170305));
#155926=CARTESIAN_POINT('Ctrl Pts',(6.88240943016724,-1.33793385413669,
23.1654499318186));
#155927=CARTESIAN_POINT('Ctrl Pts',(6.84732461971334,-1.51841215624182,
23.1570600766858));
#155928=CARTESIAN_POINT('Ctrl Pts',(6.80510658490061,-1.69766348663097,
23.148670221553));
#155929=CARTESIAN_POINT('Ctrl Pts',(6.75585773147409,-1.87510343036906,
23.1402803664202));
#155930=CARTESIAN_POINT('Ctrl Pts',(6.70665432419899,-2.05237963501495,
23.1318982533281));
#155931=CARTESIAN_POINT('Ctrl Pts',(6.65043311950308,-2.22784746996435,
23.123516140236));
#155932=CARTESIAN_POINT('Ctrl Pts',(6.58734745079217,-2.40093317796267,
23.1151340271439));
#155933=CARTESIAN_POINT('Ctrl Pts',(6.52431072318973,-2.57388460813557,
23.106758416795));
#155934=CARTESIAN_POINT('Ctrl Pts',(6.45442026090144,-2.74445728801398,
23.0983828064462));
#155935=CARTESIAN_POINT('Ctrl Pts',(6.37787919275471,-2.91209264363731,
23.0900071960973));
#155936=CARTESIAN_POINT('Ctrl Pts',(6.30138627007631,-3.07962255413295,
23.0816368541317));
#155937=CARTESIAN_POINT('Ctrl Pts',(6.21825121890737,-3.24421852610303,
23.0732665121661));
#155938=CARTESIAN_POINT('Ctrl Pts',(6.12872542486748,-3.40534157304123,
23.0648961702005));
#155939=CARTESIAN_POINT('Ctrl Pts',(6.03924282040576,-3.56638689001897,
23.0565298663062));
#155940=CARTESIAN_POINT('Ctrl Pts',(5.94337578057158,-3.72396233620873,
23.0481635624119));
#155941=CARTESIAN_POINT('Ctrl Pts',(5.841422015679,-3.87755275879526,23.0397972585176));
#155942=CARTESIAN_POINT('Ctrl Pts',(5.73949676439662,-4.03110022644583,
23.031433294444));
#155943=CARTESIAN_POINT('Ctrl Pts',(5.63148836278843,-4.18066461841331,
23.0230693303703));
#155944=CARTESIAN_POINT('Ctrl Pts',(5.51773859540824,-4.32575858725869,
23.0147053662967));
#155945=CARTESIAN_POINT('Ctrl Pts',(5.40400633222695,-4.47083022855345,
23.0063426892982));
#155946=CARTESIAN_POINT('Ctrl Pts',(5.28453466751206,-4.61143255973544,
22.9979800122996));
#155947=CARTESIAN_POINT('Ctrl Pts',(5.1597067846208,-4.74710990595731,22.9896173353011));
#155948=CARTESIAN_POINT('Ctrl Pts',(5.03488147170754,-4.88278445883057,
22.9812548304748));
#155949=CARTESIAN_POINT('Ctrl Pts',(4.90470038332,-5.01353398734206,22.9728923256485));
#155950=CARTESIAN_POINT('Ctrl Pts',(4.769585090175,-5.13893808389246,22.9645298208222));
#155951=CARTESIAN_POINT('Ctrl Pts',(4.6344545689001,-5.26435631407518,22.9561663735022));
#155952=CARTESIAN_POINT('Ctrl Pts',(4.49438897538875,-5.38442768800414,
22.9478029261822));
#155953=CARTESIAN_POINT('Ctrl Pts',(4.34984493936847,-5.49877036854154,
22.9394394788622));
#155954=CARTESIAN_POINT('Ctrl Pts',(4.20521579175774,-5.61318037726256,
22.9310711069094));
#155955=CARTESIAN_POINT('Ctrl Pts',(4.05610318965071,-5.72185474723528,
22.9227027349566));
#155956=CARTESIAN_POINT('Ctrl Pts',(3.90299571183461,-5.82445285292109,
22.9143343630038));
#155957=CARTESIAN_POINT('Ctrl Pts',(3.74984235901648,-5.92708169968091,
22.9059634836681));
#155958=CARTESIAN_POINT('Ctrl Pts',(3.59269201978674,-6.02363047331074,
22.8975926043323));
#155959=CARTESIAN_POINT('Ctrl Pts',(3.43206075230852,-6.11380287177821,
22.8892217249966));
#155960=CARTESIAN_POINT('Ctrl Pts',(3.27129338369452,-6.20405167234373,
22.8808437531053));
#155961=CARTESIAN_POINT('Ctrl Pts',(3.10703948294594,-6.28791314600656,
22.872465781214));
#155962=CARTESIAN_POINT('Ctrl Pts',(2.93983914325539,-6.36513726279987,
22.8640878093227));
#155963=CARTESIAN_POINT('Ctrl Pts',(2.83358196586494,-6.41421381786019,
22.8587635399637));
#155964=CARTESIAN_POINT('Ctrl Pts',(2.72613525119984,-6.46061069245768,
22.8534392706047));
#155965=CARTESIAN_POINT('Ctrl Pts',(2.61764153474794,-6.50427393012183,
22.8481150012457));
#155966=CARTESIAN_POINT('Ctrl Pts',(2.45741902907789,-6.56875539110413,
22.8402521700565));
#155967=CARTESIAN_POINT('Ctrl Pts',(2.29457898084835,-6.62740651627266,
22.8323893388672));
#155968=CARTESIAN_POINT('Ctrl Pts',(2.1296030516401,-6.68000130276523,22.8245265076779));
#155969=CARTESIAN_POINT('Ctrl Pts',(1.96475388465679,-6.73255567710685,
22.8166697180365));
#155970=CARTESIAN_POINT('Ctrl Pts',(1.79777246125311,-6.77906285186108,
22.8088129283952));
#155971=CARTESIAN_POINT('Ctrl Pts',(1.62916110100544,-6.81934459236889,
22.8009561387538));
#155972=CARTESIAN_POINT('Ctrl Pts',(1.46064482958318,-6.85960361588191,
22.7931037799698));
#155973=CARTESIAN_POINT('Ctrl Pts',(1.29050081951073,-6.8936441007166,22.7852514211859));
#155974=CARTESIAN_POINT('Ctrl Pts',(1.11924701355631,-6.92133749250427,
22.7773990624019));
#155975=CARTESIAN_POINT('Ctrl Pts',(0.948033642623864,-6.94902434555898,
22.7695485576515));
#155976=CARTESIAN_POINT('Ctrl Pts',(0.775711372026825,-6.97036701910334,
22.7616980529011));
#155977=CARTESIAN_POINT('Ctrl Pts',(0.602808751732648,-6.98528798055846,
22.7538475481506));
#155978=CARTESIAN_POINT('Ctrl Pts',(0.429933946020593,-7.00020654170116,
22.745998306299));
#155979=CARTESIAN_POINT('Ctrl Pts',(0.2564793568388,-7.00870541744943,22.7381490644474));
#155980=CARTESIAN_POINT('Ctrl Pts',(0.082978608838857,-7.01075895413437,
22.7302998225957));
#155981=CARTESIAN_POINT('Ctrl Pts',(-0.0905805949590776,-7.012813182696,
22.7224479361809));
#155982=CARTESIAN_POINT('Ctrl Pts',(-0.264185606802933,-7.00841773011439,
22.714596049766));
#155983=CARTESIAN_POINT('Ctrl Pts',(-0.437302645387597,-6.99759908531755,
22.7067441633512));
#155984=CARTESIAN_POINT('Ctrl Pts',(-0.564420332075718,-6.98965508910021,
22.7009786208872));
#155985=CARTESIAN_POINT('Ctrl Pts',(-0.691274897765848,-6.97824893703722,
22.6952130784233));
#155986=CARTESIAN_POINT('Ctrl Pts',(-0.817656948321552,-6.96340891211779,
22.6894475359593));
#155987=CARTESIAN_POINT('Ctrl Pts',(-1.02930349699858,-6.93855696484626,
22.6797922315994));
#155988=CARTESIAN_POINT('Ctrl Pts',(-1.23951683001374,-6.90408683421205,
22.6701369272395));
#155989=CARTESIAN_POINT('Ctrl Pts',(-1.44751734985819,-6.86019825401275,
22.6604816228796));
#155990=CARTESIAN_POINT('Ctrl Pts',(-1.65667015356232,-6.8160665393125,
22.6507728299448));
#155991=CARTESIAN_POINT('Ctrl Pts',(-1.86358552418146,-6.76241179639087,
22.64106403701));
#155992=CARTESIAN_POINT('Ctrl Pts',(-2.06749234386089,-6.69948520190743,
22.6313552440753));
#155993=CARTESIAN_POINT('Ctrl Pts',(-2.27238038047024,-6.63625579930827,
22.6215997316045));
#155994=CARTESIAN_POINT('Ctrl Pts',(-2.47423080740267,-6.56366513225861,
22.6118442191338));
#155995=CARTESIAN_POINT('Ctrl Pts',(-2.67228348797172,-6.48201569902555,
22.6020887066631));
#155996=CARTESIAN_POINT('Ctrl Pts',(-2.87053227116404,-6.4002854202922,
22.5923235347341));
#155997=CARTESIAN_POINT('Ctrl Pts',(-3.06497575524139,-6.30947845912893,
22.5825583628052));
#155998=CARTESIAN_POINT('Ctrl Pts',(-3.25487414391858,-6.20994531938489,
22.5727931908763));
#155999=CARTESIAN_POINT('Ctrl Pts',(-3.44451361045146,-6.11054789081856,
22.5630413335377));
#156000=CARTESIAN_POINT('Ctrl Pts',(-3.62962033383856,-6.00244808104336,
22.5532894761991));
#156001=CARTESIAN_POINT('Ctrl Pts',(-3.80948051221595,-5.88604152122179,
22.5435376188606));
#156002=CARTESIAN_POINT('Ctrl Pts',(-3.88791257607909,-5.83527983057753,
22.539285102798));
#156003=CARTESIAN_POINT('Ctrl Pts',(-3.96534725946363,-5.78293913191706,
22.5350325867355));
#156004=CARTESIAN_POINT('Ctrl Pts',(-4.041726772628,-5.72905500566385,22.5307800706729));
#156005=CARTESIAN_POINT('Ctrl Pts',(-4.18600844094843,-5.62726734939705,
22.5227470250741));
#156006=CARTESIAN_POINT('Ctrl Pts',(-4.32659311946212,-5.51991943857312,
22.5147139794753));
#156007=CARTESIAN_POINT('Ctrl Pts',(-4.46302109857033,-5.40731626929812,
22.5066809338765));
#156008=CARTESIAN_POINT('Ctrl Pts',(-4.59936137652064,-5.29478548567592,
22.4986530522287));
#156009=CARTESIAN_POINT('Ctrl Pts',(-4.73154999238677,-5.17700640052288,
22.4906251705809));
#156010=CARTESIAN_POINT('Ctrl Pts',(-4.85915744023882,-5.05432641738459,
22.4825972889331));
#156011=CARTESIAN_POINT('Ctrl Pts',(-4.98670727207014,-4.93170182546813,
22.474573031953));
#156012=CARTESIAN_POINT('Ctrl Pts',(-5.10967979068683,-4.80418099503689,
22.4665487749729));
#156013=CARTESIAN_POINT('Ctrl Pts',(-5.22767977195964,-4.67215055026527,
22.4585245179928));
#156014=CARTESIAN_POINT('Ctrl Pts',(-5.3456654858329,-4.54013606931913,
22.4505012312271));
#156015=CARTESIAN_POINT('Ctrl Pts',(-5.45867961003044,-4.40361332811601,
22.4424779444614));
#156016=CARTESIAN_POINT('Ctrl Pts',(-5.56636478780507,-4.26300476326075,
22.4344546576957));
#156017=CARTESIAN_POINT('Ctrl Pts',(-5.67404114174001,-4.12240772002305,
22.4264320283668));
#156018=CARTESIAN_POINT('Ctrl Pts',(-5.77638919929735,-3.97772581354571,
22.4184093990379));
#156019=CARTESIAN_POINT('Ctrl Pts',(-5.87309299959403,-3.82941316400041,
22.4103867697089));
#156020=CARTESIAN_POINT('Ctrl Pts',(-5.96983315363501,-3.68104475945767,
22.4023611244425));
#156021=CARTESIAN_POINT('Ctrl Pts',(-6.06092461385538,-3.52904319413968,
22.3943354791761));
#156022=CARTESIAN_POINT('Ctrl Pts',(-6.14609552708751,-3.37389038565495,
22.3863098339097));
#156023=CARTESIAN_POINT('Ctrl Pts',(-6.19631748758872,-3.28240283522638,
22.381577424402));
#156024=CARTESIAN_POINT('Ctrl Pts',(-6.2444817301707,-3.18982009090364,
22.3768450148942));
#156025=CARTESIAN_POINT('Ctrl Pts',(-6.29054013873481,-3.09624471343373,
22.3721126053864));
#156026=CARTESIAN_POINT('Ctrl Pts',(-6.37550576889667,-2.92362279352308,
22.3633825565517));
#156027=CARTESIAN_POINT('Ctrl Pts',(-6.45334528794889,-2.74753552574655,
22.3546525077171));
#156028=CARTESIAN_POINT('Ctrl Pts',(-6.52380507287605,-2.568578193012,22.3459224588824));
#156029=CARTESIAN_POINT('Ctrl Pts',(-6.59428523133781,-2.38956911454171,
22.3371898857432));
#156030=CARTESIAN_POINT('Ctrl Pts',(-6.65738129601697,-2.20768856951921,
22.3284573126041));
#156031=CARTESIAN_POINT('Ctrl Pts',(-6.71288843299581,-2.02355020907588,
22.3197247394649));
#156032=CARTESIAN_POINT('Ctrl Pts',(-6.76918413746143,-1.83679586928257,
22.3108681061845));
#156033=CARTESIAN_POINT('Ctrl Pts',(-6.81767356152658,-1.64771935090213,
22.3020114729041));
#156034=CARTESIAN_POINT('Ctrl Pts',(-6.85819576343518,-1.45697544004688,
22.2931548396237));
#156035=CARTESIAN_POINT('Ctrl Pts',(-6.89817578093431,-1.26878367023517,
22.2844167075169));
#156036=CARTESIAN_POINT('Ctrl Pts',(-6.93040041898989,-1.07896912656069,
22.2756785754102));
#156037=CARTESIAN_POINT('Ctrl Pts',(-6.9547666744769,-0.888170628925281,
22.2669404433034));
#156038=CARTESIAN_POINT('Ctrl Pts',(-6.97962859022127,-0.693490893465223,
22.2580245594362));
#156039=CARTESIAN_POINT('Ctrl Pts',(-6.9963089458876,-0.49778703725925,
22.249108675569));
#156040=CARTESIAN_POINT('Ctrl Pts',(-7.00475389972531,-0.301743876131736,
22.2401927917017));
#156041=CARTESIAN_POINT('Ctrl Pts',(-7.01319885356303,-0.10570071500419,
22.2312769078345));
#156042=CARTESIAN_POINT('Ctrl Pts',(-7.01340839863455,0.0906814486510902,
22.2223610239673));
#156043=CARTESIAN_POINT('Ctrl Pts',(-7.00538510597693,0.286716025810481,
22.2134451401));
#156044=CARTESIAN_POINT('Ctrl Pts',(-6.99751947304751,0.478898473990961,
22.2047044556038));
#156045=CARTESIAN_POINT('Ctrl Pts',(-6.98174071831608,0.670767280899435,
22.1959637711076));
#156046=CARTESIAN_POINT('Ctrl Pts',(-6.95809877101642,0.861677465923196,
22.1872230866114));
#156047=CARTESIAN_POINT('Ctrl Pts',(-6.9344610772958,1.05255330303345,22.1784839747095));
#156048=CARTESIAN_POINT('Ctrl Pts',(-6.90296304994579,1.24247059107705,
22.1697448628077));
#156049=CARTESIAN_POINT('Ctrl Pts',(-6.86370636760827,1.4307905023985,22.1610057509058));
#156050=CARTESIAN_POINT('Ctrl Pts',(-6.8239410584508,1.62155036921092,22.1521534112314));
#156051=CARTESIAN_POINT('Ctrl Pts',(-6.77621467986645,1.81067089452022,
22.1433010715571));
#156052=CARTESIAN_POINT('Ctrl Pts',(-6.72068646462487,1.99749843722293,
22.1344487318827));
#156053=CARTESIAN_POINT('Ctrl Pts',(-6.66589659215342,2.1818417876134,22.125714099233));
#156054=CARTESIAN_POINT('Ctrl Pts',(-6.60351116548751,2.36395248962728,
22.1169794665832));
#156055=CARTESIAN_POINT('Ctrl Pts',(-6.53373368135293,2.54321661359277,
22.1082448339335));
#156056=CARTESIAN_POINT('Ctrl Pts',(-6.46254572575882,2.72610435531557,
22.0993336407469));
#156057=CARTESIAN_POINT('Ctrl Pts',(-6.38366377114866,2.90602893427757,
22.0904224475602));
#156058=CARTESIAN_POINT('Ctrl Pts',(-6.29735645066384,3.08235758726702,
22.0815112543736));
#156059=CARTESIAN_POINT('Ctrl Pts',(-6.21104913017901,3.25868624025649,
22.0726000611869));
#156060=CARTESIAN_POINT('Ctrl Pts',(-6.11731656498246,3.43141868908508,
22.0636888680003));
#156061=CARTESIAN_POINT('Ctrl Pts',(-6.01647881569159,3.59994572498453,
22.0547776748136));
#156062=CARTESIAN_POINT('Ctrl Pts',(-5.92566157457379,3.75172579308185,
22.0467520099612));
#156063=CARTESIAN_POINT('Ctrl Pts',(-5.82903892465932,3.90016421168691,
22.0387263451088));
#156064=CARTESIAN_POINT('Ctrl Pts',(-5.72689495485971,4.04478685946521,
22.0307006802564));
#156065=CARTESIAN_POINT('Ctrl Pts',(-5.62478340305075,4.18936360756237,
22.0226775625532));
#156066=CARTESIAN_POINT('Ctrl Pts',(-5.51715423130696,4.33012669681961,
22.0146544448499));
#156067=CARTESIAN_POINT('Ctrl Pts',(-5.40433510896315,4.46663056369433,
22.0066313271467));
#156068=CARTESIAN_POINT('Ctrl Pts',(-5.29153021409795,4.60311721623688,
21.9986092212288));
#156069=CARTESIAN_POINT('Ctrl Pts',(-5.17353690623727,4.73534543418988,
21.9905871153109));
#156070=CARTESIAN_POINT('Ctrl Pts',(-5.05072339345024,4.86290240138074,
21.9825650093931));
#156071=CARTESIAN_POINT('Ctrl Pts',(-4.92786424274702,4.99050676917146,
21.9745399224335));
#156072=CARTESIAN_POINT('Ctrl Pts',(-4.80018156118176,5.1134361521193,21.966514835474));
#156073=CARTESIAN_POINT('Ctrl Pts',(-4.66808102018971,5.23131399855186,
21.9584897485145));
#156074=CARTESIAN_POINT('Ctrl Pts',(-4.53595446265715,5.3492150604364,21.9504630810542));
#156075=CARTESIAN_POINT('Ctrl Pts',(-4.39940859173352,5.4620623663669,21.942436413594));
#156076=CARTESIAN_POINT('Ctrl Pts',(-4.25888229618446,5.56951956184253,
21.9344097461337));
#156077=CARTESIAN_POINT('Ctrl Pts',(-4.11824318662046,5.67706302357608,
21.9263766348931));
#156078=CARTESIAN_POINT('Ctrl Pts',(-3.9736175670563,5.77920751718783,21.9183435236525));
#156079=CARTESIAN_POINT('Ctrl Pts',(-3.82547395054926,5.87565958988172,
21.9103104124119));
#156080=CARTESIAN_POINT('Ctrl Pts',(-3.73818235009383,5.93249265492502,
21.9055770114503));
#156081=CARTESIAN_POINT('Ctrl Pts',(-3.64966982054114,5.98735015674246,
21.9008436104887));
#156082=CARTESIAN_POINT('Ctrl Pts',(-3.56003617203163,6.04017955166288,
21.8961102095271));
#156083=CARTESIAN_POINT('Ctrl Pts',(-3.37538806651734,6.14900974935908,
21.886359256233));
#156084=CARTESIAN_POINT('Ctrl Pts',(-3.18587248217942,6.24929545974911,
21.8766083029389));
#156085=CARTESIAN_POINT('Ctrl Pts',(-2.99222443154627,6.3406797359398,21.8668573496447));
#156086=CARTESIAN_POINT('Ctrl Pts',(-2.79829739456872,6.4321956683236,21.8570923482732));
#156087=CARTESIAN_POINT('Ctrl Pts',(-2.60022601729658,6.51478449787464,
21.8473273469016));
#156088=CARTESIAN_POINT('Ctrl Pts',(-2.39876794143634,6.5881362254918,21.83756234553));
#156089=CARTESIAN_POINT('Ctrl Pts',(-2.1976456544473,6.66136569097718,21.8278136203924));
#156090=CARTESIAN_POINT('Ctrl Pts',(-1.99314798640384,6.72538881257968,
21.8180648952549));
#156091=CARTESIAN_POINT('Ctrl Pts',(-1.78604756611937,6.77994547574382,
21.8083161701173));
#156092=CARTESIAN_POINT('Ctrl Pts',(-1.57951555618622,6.8343524020217,21.7985942014502));
#156093=CARTESIAN_POINT('Ctrl Pts',(-1.37039509354959,6.87934472802108,
21.7888722327832));
#156094=CARTESIAN_POINT('Ctrl Pts',(-1.15947062927344,6.9147128951499,21.7791502641161));
#156095=CARTESIAN_POINT('Ctrl Pts',(-0.949941797086738,6.94984704035452,
21.7694926231764));
#156096=CARTESIAN_POINT('Ctrl Pts',(-0.738632798821536,6.97548393061858,
21.7598349822368));
#156097=CARTESIAN_POINT('Ctrl Pts',(-0.526330010289526,6.99146646153499,
21.7501773412971));
#156098=CARTESIAN_POINT('Ctrl Pts',(-0.433015625586685,6.99849133411802,
21.7459324756116));
#156099=CARTESIAN_POINT('Ctrl Pts',(-0.339509473265604,7.00365170974,21.7416876099262));
#156100=CARTESIAN_POINT('Ctrl Pts',(-0.245879369247645,7.00693726946934,
21.7374427442407));
#156101=CARTESIAN_POINT('Ctrl Pts',(-0.0726891420124154,7.01301466137321,
21.7295908972268));
#156102=CARTESIAN_POINT('Ctrl Pts',(0.100854183988949,7.01267108832776,
21.7217390502129));
#156103=CARTESIAN_POINT('Ctrl Pts',(0.274217249882488,7.00588548738608,
21.713887203199));
#156104=CARTESIAN_POINT('Ctrl Pts',(0.447531151412028,6.99910181078597,
21.7060375829054));
#156105=CARTESIAN_POINT('Ctrl Pts',(0.620664513724713,6.98587975522486,
21.6981879626118));
#156106=CARTESIAN_POINT('Ctrl Pts',(0.793084111268163,6.96625036550898,
21.6903383423182));
#156107=CARTESIAN_POINT('Ctrl Pts',(0.965489943311692,6.94662254294885,
21.6824893487164));
#156108=CARTESIAN_POINT('Ctrl Pts',(1.13718174509647,6.92058844847128,21.6746403551146));
#156109=CARTESIAN_POINT('Ctrl Pts',(1.30763180892856,6.88823094958192,21.6667913615129));
#156110=CARTESIAN_POINT('Ctrl Pts',(1.47816816663717,6.85585706903831,21.6589383941954));
#156111=CARTESIAN_POINT('Ctrl Pts',(1.64746115504819,6.81715345885381,21.651085426878));
#156112=CARTESIAN_POINT('Ctrl Pts',(1.8149933176821,6.77225411656041,21.6432324595606));
#156113=CARTESIAN_POINT('Ctrl Pts',(1.98256802785633,6.72734337134265,21.6353774978533));
#156114=CARTESIAN_POINT('Ctrl Pts',(2.14838065676238,6.67623387159824,21.627522536146));
#156115=CARTESIAN_POINT('Ctrl Pts',(2.31192992699491,6.61910919800885,21.6196675744388));
#156116=CARTESIAN_POINT('Ctrl Pts',(2.47564153354891,6.56192782340598,21.6118048160254));
#156117=CARTESIAN_POINT('Ctrl Pts',(2.63708493939628,6.49871948923473,21.603942057612));
#156118=CARTESIAN_POINT('Ctrl Pts',(2.79577929785132,6.42971575423097,21.5960792991987));
#156119=CARTESIAN_POINT('Ctrl Pts',(2.91219520208469,6.37909560437721,21.5903112924506));
#156120=CARTESIAN_POINT('Ctrl Pts',(3.02713214893815,6.32535767300183,21.5845432857024));
#156121=CARTESIAN_POINT('Ctrl Pts',(3.14040939108398,6.2686087307226,21.5787752789543));
#156122=CARTESIAN_POINT('Ctrl Pts',(3.304960287799,6.18617302552018,21.5703964495912));
#156123=CARTESIAN_POINT('Ctrl Pts',(3.46637260497444,6.09719951480489,21.5620176202281));
#156124=CARTESIAN_POINT('Ctrl Pts',(3.6241137781913,6.00195183962884,21.553638790865));
#156125=CARTESIAN_POINT('Ctrl Pts',(3.78174325263786,5.90677161068749,21.5452658946703));
#156126=CARTESIAN_POINT('Ctrl Pts',(3.93570648585905,5.80532624533494,21.5368929984755));
#156127=CARTESIAN_POINT('Ctrl Pts',(4.08549569848543,5.69792518906286,21.5285201022808));
#156128=CARTESIAN_POINT('Ctrl Pts',(4.2351917523392,5.59059092899329,21.5201524134619));
#156129=CARTESIAN_POINT('Ctrl Pts',(4.38071869727635,5.47730855774819,21.511784724643));
#156130=CARTESIAN_POINT('Ctrl Pts',(4.52159763341181,5.35843087144219,21.5034170358241));
#156131=CARTESIAN_POINT('Ctrl Pts',(4.66242521850144,5.23959651662126,21.4950523970678));
#156132=CARTESIAN_POINT('Ctrl Pts',(4.79860792169724,5.11517112458317,21.4866877583116));
#156133=CARTESIAN_POINT('Ctrl Pts',(4.92969933646971,4.98554821604506,21.4783231195553));
#156134=CARTESIAN_POINT('Ctrl Pts',(5.06076045028385,4.85595526902928,21.4699604142328));
#156135=CARTESIAN_POINT('Ctrl Pts',(5.18673238887386,4.72116743212467,21.4615977089103));
#156136=CARTESIAN_POINT('Ctrl Pts',(5.30720477662809,4.58161587449625,21.4532350035878));
#156137=CARTESIAN_POINT('Ctrl Pts',(5.42766537763979,4.44207797027265,21.4448731164532));
#156138=CARTESIAN_POINT('Ctrl Pts',(5.5426272867884,4.29777752399853,21.4365112293186));
#156139=CARTESIAN_POINT('Ctrl Pts',(5.65171939997368,4.14917996554273,21.4281493421841));
#156140=CARTESIAN_POINT('Ctrl Pts',(5.76083930437926,4.00054455185283,21.4197853248584));
#156141=CARTESIAN_POINT('Ctrl Pts',(5.86408622814664,3.84761010204599,21.4114213075328));
#156142=CARTESIAN_POINT('Ctrl Pts',(5.96113104311383,3.69087296575276,21.4030572902071));
#156143=CARTESIAN_POINT('Ctrl Pts',(6.05818750621396,3.53411701655336,21.3946922689619));
#156144=CARTESIAN_POINT('Ctrl Pts',(6.14904020684982,3.37355775255416,21.3863272477167));
#156145=CARTESIAN_POINT('Ctrl Pts',(6.23340485140487,3.20971813731085,21.3779622264715));
#156146=CARTESIAN_POINT('Ctrl Pts',(6.31781451050954,3.04579110195775,21.3695927418914));
#156147=CARTESIAN_POINT('Ctrl Pts',(6.39572904963281,2.87858051234587,21.3612232573113));
#156148=CARTESIAN_POINT('Ctrl Pts',(6.46691099881845,2.70863225556018,21.3528537727312));
#156149=CARTESIAN_POINT('Ctrl Pts',(6.50342331136282,2.62145841529419,21.3485607006768));
#156150=CARTESIAN_POINT('Ctrl Pts',(6.53816498276623,2.53356459390674,21.3442676286225));
#156151=CARTESIAN_POINT('Ctrl Pts',(6.57110895151816,2.44502632087631,21.3399745565681));
#156152=CARTESIAN_POINT('Origin',(0.,0.,50.));
#156153=CARTESIAN_POINT('',(6.57110895151814,2.44502632087635,19.3399454697435));
#156154=CARTESIAN_POINT('',(6.57110895151814,2.44502632087636,19.8869210003222));
#156155=CARTESIAN_POINT('',(6.57110895151814,2.44502632087636,50.));
#156156=CARTESIAN_POINT('',(7.01125,3.83823506831804E-12,21.7735343569105));
#156157=CARTESIAN_POINT('Ctrl Pts',(6.57110895151814,2.44502632087636,19.8869210003222));
#156158=CARTESIAN_POINT('Ctrl Pts',(6.50449838733151,2.6240449559132,19.8955928092609));
#156159=CARTESIAN_POINT('Ctrl Pts',(6.43056821795879,2.80033990715949,19.9042646181997));
#156160=CARTESIAN_POINT('Ctrl Pts',(6.34956511459268,2.97332295892115,19.9129364271385));
#156161=CARTESIAN_POINT('Ctrl Pts',(6.26856213015524,3.14630575670929,19.9216082233453));
#156162=CARTESIAN_POINT('Ctrl Pts',(6.18048635294281,3.31597640754666,19.9302800195521));
#156163=CARTESIAN_POINT('Ctrl Pts',(6.08563165071556,3.48176879966333,19.9389518157589));
#156164=CARTESIAN_POINT('Ctrl Pts',(5.99077708581969,3.64756095174446,19.9476235994107));
#156165=CARTESIAN_POINT('Ctrl Pts',(5.88914375658117,3.8094746098372,19.9562953830624));
#156166=CARTESIAN_POINT('Ctrl Pts',(5.78107076500248,3.96696954519866,19.9649671667141));
#156167=CARTESIAN_POINT('Ctrl Pts',(5.67299792768891,4.12446425574932,19.9736389379876));
#156168=CARTESIAN_POINT('Ctrl Pts',(5.55848560711398,4.27754002202472,19.9823107092611));
#156169=CARTESIAN_POINT('Ctrl Pts',(5.43791587524917,4.42568610457329,19.9909824805346));
#156170=CARTESIAN_POINT('Ctrl Pts',(5.31734631302946,4.57383197867604,19.9996542396066));
#156171=CARTESIAN_POINT('Ctrl Pts',(5.19071953583901,4.71704796266763,20.0083259986787));
#156172=CARTESIAN_POINT('Ctrl Pts',(5.0584580345168,4.85485621574238,20.0169977577507));
#156173=CARTESIAN_POINT('Ctrl Pts',(4.9261967165933,4.9926642777271,20.0256695047982));
#156174=CARTESIAN_POINT('Ctrl Pts',(4.78830088681942,5.12506441890746,20.0343412518457));
#156175=CARTESIAN_POINT('Ctrl Pts',(4.64523063400654,5.25161488681217,20.0430129988931));
#156176=CARTESIAN_POINT('Ctrl Pts',(4.49652806262589,5.38314733060724,20.0520261309661));
#156177=CARTESIAN_POINT('Ctrl Pts',(4.34223563524161,5.50835996364107,20.0610392630392));
#156178=CARTESIAN_POINT('Ctrl Pts',(4.18290943344762,5.626801510101,20.0700523951122));
#156179=CARTESIAN_POINT('Ctrl Pts',(4.02607270355667,5.7433924073975,20.0789246969965));
#156180=CARTESIAN_POINT('Ctrl Pts',(3.86435862820615,5.85342208902484,20.0877969988809));
#156181=CARTESIAN_POINT('Ctrl Pts',(3.69833198496683,5.9565062823329,20.0966693007653));
#156182=CARTESIAN_POINT('Ctrl Pts',(3.53489950802812,6.05797978512052,20.1054029729327));
#156183=CARTESIAN_POINT('Ctrl Pts',(3.36728850947313,6.15272311279783,20.1141366451001));
#156184=CARTESIAN_POINT('Ctrl Pts',(3.196066230012,6.24041562845592,20.1228703172675));
#156185=CARTESIAN_POINT('Ctrl Pts',(3.02603797481334,6.3274966174385,20.1315430848815));
#156186=CARTESIAN_POINT('Ctrl Pts',(2.85244891335583,6.40762471321497,20.1402158524955));
#156187=CARTESIAN_POINT('Ctrl Pts',(2.67587836095385,6.48053250588861,20.1488886201095));
#156188=CARTESIAN_POINT('Ctrl Pts',(2.49930871513683,6.55343992422402,20.157561343194));
#156189=CARTESIAN_POINT('Ctrl Pts',(2.319757871652,6.61912700519343,20.1662340662785));
#156190=CARTESIAN_POINT('Ctrl Pts',(2.13782503580303,6.67737453485978,20.1749067893629));
#156191=CARTESIAN_POINT('Ctrl Pts',(1.9558931192204,6.73562177021425,20.1835794686261));
#156192=CARTESIAN_POINT('Ctrl Pts',(1.7715795049724,6.7864294428484,20.1922521478892));
#156193=CARTESIAN_POINT('Ctrl Pts',(1.58549928668991,6.82962799678034,20.2009248271523));
#156194=CARTESIAN_POINT('Ctrl Pts',(1.39941999344073,6.87282633596564,20.2095974633022));
#156195=CARTESIAN_POINT('Ctrl Pts',(1.21157439050846,6.90841556788882,20.2182700994521));
#156196=CARTESIAN_POINT('Ctrl Pts',(1.02258935229308,6.93627692491273,20.226942735602));
#156197=CARTESIAN_POINT('Ctrl Pts',(0.833605238126011,6.96413814570766,
20.2356153293468));
#156198=CARTESIAN_POINT('Ctrl Pts',(0.643481980917327,6.98427152577607,
20.2442879230916));
#156199=CARTESIAN_POINT('Ctrl Pts',(0.452854049808676,6.99660987708132,
20.2529605168364));
#156200=CARTESIAN_POINT('Ctrl Pts',(0.262227035222496,7.00894816906485,
20.2616330688841));
#156201=CARTESIAN_POINT('Ctrl Pts',(0.071095635122742,7.01349148893086,
20.2703056209318));
#156202=CARTESIAN_POINT('Ctrl Pts',(-0.119902323155651,7.0102246751015,
20.2789781729795));
#156203=CARTESIAN_POINT('Ctrl Pts',(-0.310899378721189,7.00695787671206,
20.2876506840382));
#156204=CARTESIAN_POINT('Ctrl Pts',(-0.501762709651607,6.99588102335292,
20.2963231950968));
#156205=CARTESIAN_POINT('Ctrl Pts',(-0.691855389204073,6.97703107940113,
20.3049957061555));
#156206=CARTESIAN_POINT('Ctrl Pts',(-0.881947185836118,6.95818122300137,
20.3136681769331));
#156207=CARTESIAN_POINT('Ctrl Pts',(-1.07126805552891,6.93155837629147,
20.3223406477107));
#156208=CARTESIAN_POINT('Ctrl Pts',(-1.25918622472346,6.89725138109136,
20.3310131184882));
#156209=CARTESIAN_POINT('Ctrl Pts',(-1.44710353643374,6.86294454243657,
20.3396855496927));
#156210=CARTESIAN_POINT('Ctrl Pts',(-1.63361788096923,6.82095367648077,
20.3483579808972));
#156211=CARTESIAN_POINT('Ctrl Pts',(-1.81810685596541,6.77141890764348,
20.3570304121017));
#156212=CARTESIAN_POINT('Ctrl Pts',(-2.00259500418067,6.72188436079453,
20.3657028044409));
#156213=CARTESIAN_POINT('Ctrl Pts',(-2.1850575266401,6.66480605238719,20.3743751967802));
#156214=CARTESIAN_POINT('Ctrl Pts',(-2.36488554744815,6.60037445225427,
20.3830475891195));
#156215=CARTESIAN_POINT('Ctrl Pts',(-2.54471277703796,6.53594313561142,
20.3917199433014));
#156216=CARTESIAN_POINT('Ctrl Pts',(-2.72190526072897,6.46415868780944,
20.4003922974834));
#156217=CARTESIAN_POINT('Ctrl Pts',(-2.89587171389844,6.38526065083822,
20.4090646516653));
#156218=CARTESIAN_POINT('Ctrl Pts',(-3.06983741583579,6.30636295456912,
20.4177369683978));
#156219=CARTESIAN_POINT('Ctrl Pts',(-3.24057685640747,6.22035184793782,
20.4264092851303));
#156220=CARTESIAN_POINT('Ctrl Pts',(-3.4075202894675,6.12751434428083,20.4350816018628));
#156221=CARTESIAN_POINT('Ctrl Pts',(-3.57446301524516,6.03467723394467,
20.4437538818536));
#156222=CARTESIAN_POINT('Ctrl Pts',(-3.73760951742132,5.93501392252177,
20.4524261618445));
#156223=CARTESIAN_POINT('Ctrl Pts',(-3.89641539158824,5.82885697703197,
20.4610984418353));
#156224=CARTESIAN_POINT('Ctrl Pts',(-4.05522060590695,5.72270047263084,
20.4697706857923));
#156225=CARTESIAN_POINT('Ctrl Pts',(-4.20968499214093,5.61005054602585,
20.4784429297493));
#156226=CARTESIAN_POINT('Ctrl Pts',(-4.35929312155911,5.49128309621963,
20.4871151737063));
#156227=CARTESIAN_POINT('Ctrl Pts',(-4.50890064155348,5.37251613020872,
20.4957873823372));
#156228=CARTESIAN_POINT('Ctrl Pts',(-4.65365172183292,5.24763186748421,
20.504459590968));
#156229=CARTESIAN_POINT('Ctrl Pts',(-4.79306334970934,5.11704702813772,
20.5131317995989));
#156230=CARTESIAN_POINT('Ctrl Pts',(-4.93247442107197,4.98646271006959,
20.5218039736114));
#156231=CARTESIAN_POINT('Ctrl Pts',(-5.06654587536609,4.85017805510835,
20.5304761476239));
#156232=CARTESIAN_POINT('Ctrl Pts',(-5.19483033978515,4.70864782112102,
20.5391483216364));
#156233=CARTESIAN_POINT('Ctrl Pts',(-5.32311430257525,4.56711814055739,
20.5478204617383));
#156234=CARTESIAN_POINT('Ctrl Pts',(-5.44561113000508,4.42034313247902,
20.5564926018401));
#156235=CARTESIAN_POINT('Ctrl Pts',(-5.5619120749508,4.26881255538546,20.5651647419419));
#156236=CARTESIAN_POINT('Ctrl Pts',(-5.67821257461538,4.11728255845664,
20.5738368488408));
#156237=CARTESIAN_POINT('Ctrl Pts',(-5.78831706632159,3.96099725428101,
20.5825089557396));
#156238=CARTESIAN_POINT('Ctrl Pts',(-5.89185815647258,3.80047813130238,
20.5911810626384));
#156239=CARTESIAN_POINT('Ctrl Pts',(-5.99539885864335,3.6399596098071,20.5998531370419));
#156240=CARTESIAN_POINT('Ctrl Pts',(-6.0923760545057,3.47520753995133,20.6085252114453));
#156241=CARTESIAN_POINT('Ctrl Pts',(-6.18246615568003,3.30677165773069,
20.6171972858488));
#156242=CARTESIAN_POINT('Ctrl Pts',(-6.27255592662618,3.13833639291722,
20.6258693284645));
#156243=CARTESIAN_POINT('Ctrl Pts',(-6.35575851943786,2.96621759322458,
20.6345413710802));
#156244=CARTESIAN_POINT('Ctrl Pts',(-6.43179631013586,2.79098957135685,
20.6432134136958));
#156245=CARTESIAN_POINT('Ctrl Pts',(-6.50783382831831,2.61576217749741,
20.6518854252314));
#156246=CARTESIAN_POINT('Ctrl Pts',(-6.57670648270539,2.43742584432246,
20.6605574367669));
#156247=CARTESIAN_POINT('Ctrl Pts',(-6.63818446599417,2.2565756264601,20.6692294483024));
#156248=CARTESIAN_POINT('Ctrl Pts',(-6.69966223396417,2.07572604200249,
20.6779014294654));
#156249=CARTESIAN_POINT('Ctrl Pts',(-6.75374529124706,1.89236285939331,
20.6865734106283));
#156250=CARTESIAN_POINT('Ctrl Pts',(-6.80025318023355,1.7070979020617,20.6952453917912));
#156251=CARTESIAN_POINT('Ctrl Pts',(-6.84676091012601,1.52183357848386,
20.703917343289));
#156252=CARTESIAN_POINT('Ctrl Pts',(-6.88569345442259,1.3346677686797,20.7125892947869));
#156253=CARTESIAN_POINT('Ctrl Pts',(-6.91692090874655,1.14622497994278,
20.7212612462847));
#156254=CARTESIAN_POINT('Ctrl Pts',(-6.94814825879511,0.957782820458171,
20.729933168825));
#156255=CARTESIAN_POINT('Ctrl Pts',(-6.97167052392486,0.768063970772979,
20.7386050913652));
#156256=CARTESIAN_POINT('Ctrl Pts',(-6.98740921903138,0.577701452564639,
20.7472770139055));
#156257=CARTESIAN_POINT('Ctrl Pts',(-7.00314786286674,0.387339554490748,
20.7559489081957));
#156258=CARTESIAN_POINT('Ctrl Pts',(-7.01110296401739,0.196334275139723,
20.7646208024858));
#156259=CARTESIAN_POINT('Ctrl Pts',(-7.01124797942392,0.00532292438118208,
20.773292696776));
#156260=CARTESIAN_POINT('Ctrl Pts',(-7.01139299436988,-0.18568781970999,
20.7819645635235));
#156261=CARTESIAN_POINT('Ctrl Pts',(-7.00372797299449,-0.376704351158961,
20.7906364302711));
#156262=CARTESIAN_POINT('Ctrl Pts',(-6.98827849031219,-0.567089326596749,
20.7993082970186));
#156263=CARTESIAN_POINT('Ctrl Pts',(-6.97282905543853,-0.757473712885664,
20.807980136931));
#156264=CARTESIAN_POINT('Ctrl Pts',(-6.94959523043414,-0.947226263998012,
20.8166519768433));
#156265=CARTESIAN_POINT('Ctrl Pts',(-6.91865453650955,-1.13571385786028,
20.8253238167556));
#156266=CARTESIAN_POINT('Ctrl Pts',(-6.88771393580756,-1.3242008838198,
20.8339956305402));
#156267=CARTESIAN_POINT('Ctrl Pts',(-6.84906655865586,-1.51142267990424,
20.8426674443247));
#156268=CARTESIAN_POINT('Ctrl Pts',(-6.80284135383597,-1.69675457183389,
20.8513392581093));
#156269=CARTESIAN_POINT('Ctrl Pts',(-6.75661628451972,-1.88208592048537,
20.8600110464735));
#156270=CARTESIAN_POINT('Ctrl Pts',(-6.70281350071577,-2.06552710051182,
20.8686828348377));
#156271=CARTESIAN_POINT('Ctrl Pts',(-6.64161251687743,-2.24646605542062,
20.8773546232018));
#156272=CARTESIAN_POINT('Ctrl Pts',(-6.58041170745085,-2.42740449468607,
20.886026386853));
#156273=CARTESIAN_POINT('Ctrl Pts',(-6.51181283117455,-2.60584045408172,
20.8946981505041));
#156274=CARTESIAN_POINT('Ctrl Pts',(-6.43604476876406,-2.78117858055982,
20.9033699141553));
#156275=CARTESIAN_POINT('Ctrl Pts',(-6.3568477472844,-2.96445180844916,
20.9124341271007));
#156276=CARTESIAN_POINT('Ctrl Pts',(-6.26981768815867,-3.14433998861843,
20.921498340046));
#156277=CARTESIAN_POINT('Ctrl Pts',(-6.17527181578317,-3.32018742900067,
20.9305625529914));
#156278=CARTESIAN_POINT('Ctrl Pts',(-6.08368050191941,-3.49053963687095,
20.9393435092822));
#156279=CARTESIAN_POINT('Ctrl Pts',(-5.98503618716834,-3.65709956718258,
20.948124465573));
#156280=CARTESIAN_POINT('Ctrl Pts',(-5.87967633130331,-3.81929742251263,
20.9569054218639));
#156281=CARTESIAN_POINT('Ctrl Pts',(-5.77561495477929,-3.97949631379159,
20.9655781596094));
#156282=CARTESIAN_POINT('Ctrl Pts',(-5.66500279405459,-4.13543980257297,
20.9742508973548));
#156283=CARTESIAN_POINT('Ctrl Pts',(-5.54820899034813,-4.28660746534136,
20.9829236351003));
#156284=CARTESIAN_POINT('Ctrl Pts',(-5.43141636368597,-4.43777360464676,
20.9915962854423));
#156285=CARTESIAN_POINT('Ctrl Pts',(-5.3084423924293,-4.58416378940311,
21.0002689357842));
#156286=CARTESIAN_POINT('Ctrl Pts',(-5.17969746407345,-4.7252894877638,
21.0089415861261));
#156287=CARTESIAN_POINT('Ctrl Pts',(-5.05095379117065,-4.86641380994066,
21.0176141518968));
#156288=CARTESIAN_POINT('Ctrl Pts',(-4.91643946527209,-5.002273538546,21.0262867176676));
#156289=CARTESIAN_POINT('Ctrl Pts',(-4.776603377482,-5.13241529269871,21.0349592834384));
#156290=CARTESIAN_POINT('Ctrl Pts',(-4.63676860764796,-5.26255582026453,
21.0436317674702));
#156291=CARTESIAN_POINT('Ctrl Pts',(-4.49161238427241,-5.38697828766001,
21.052304251502));
#156292=CARTESIAN_POINT('Ctrl Pts',(-4.34161910267864,-5.50526748939195,
21.0609767355337));
#156293=CARTESIAN_POINT('Ctrl Pts',(-4.19162718580777,-5.62355561486247,
21.0696491406584));
#156294=CARTESIAN_POINT('Ctrl Pts',(-4.0367985218659,-5.73571041041258,
21.0783215457831));
#156295=CARTESIAN_POINT('Ctrl Pts',(-3.87764977431811,-5.84135761533488,
21.0869939509077));
#156296=CARTESIAN_POINT('Ctrl Pts',(-3.71850242284505,-5.94700389350534,
21.0956662799569));
#156297=CARTESIAN_POINT('Ctrl Pts',(-3.55503530028693,-6.04614253816315,
21.104338609006));
#156298=CARTESIAN_POINT('Ctrl Pts',(-3.38779388709652,-6.13844272931266,
21.1130109380551));
#156299=CARTESIAN_POINT('Ctrl Pts',(-3.22055388638266,-6.23074214091927,
21.1216831938601));
#156300=CARTESIAN_POINT('Ctrl Pts',(-3.04953990753832,-6.31620307732841,
21.130355449665));
#156301=CARTESIAN_POINT('Ctrl Pts',(-2.87532260481505,-6.39454036508799,
21.13902770547));
#156302=CARTESIAN_POINT('Ctrl Pts',(-2.7011067166233,-6.47287701679959,
21.1476998908618));
#156303=CARTESIAN_POINT('Ctrl Pts',(-2.52368781567824,-6.54409001910862,
21.1563720762537));
#156304=CARTESIAN_POINT('Ctrl Pts',(-2.34365791912595,-6.60794174615805,
21.1650442616455));
#156305=CARTESIAN_POINT('Ctrl Pts',(-2.16362942554496,-6.67179297561156,
21.1737163794551));
#156306=CARTESIAN_POINT('Ctrl Pts',(-1.98099024478875,-6.72828294965035,
21.1823884972647));
#156307=CARTESIAN_POINT('Ctrl Pts',(-1.79634980371338,-6.77722317363084,
21.1910606150743));
#156308=CARTESIAN_POINT('Ctrl Pts',(-1.61171074128287,-6.826163032192,21.1997326681323));
#156309=CARTESIAN_POINT('Ctrl Pts',(-1.42507072299763,-6.86755318072501,
21.2084047211902));
#156310=CARTESIAN_POINT('Ctrl Pts',(-1.23705251633957,-6.90125551144992,
21.2170767742482));
#156311=CARTESIAN_POINT('Ctrl Pts',(-1.04903565219215,-6.93495760152932,
21.2257487653849));
#156312=CARTESIAN_POINT('Ctrl Pts',(-0.859640898941481,-6.9609719335339,
21.2344207565216));
#156313=CARTESIAN_POINT('Ctrl Pts',(-0.669500206862531,-6.97921170588133,
21.2430927476583));
#156314=CARTESIAN_POINT('Ctrl Pts',(-0.479360810404673,-6.99745135394273,
21.2517646797039));
#156315=CARTESIAN_POINT('Ctrl Pts',(-0.288475768015417,-7.00791652123616,
21.2604366117496));
#156316=CARTESIAN_POINT('Ctrl Pts',(-0.0974819939210606,-7.01057228929003,
21.2691085437952));
#156317=CARTESIAN_POINT('Ctrl Pts',(0.0935105410582171,-7.013228040114,
21.2777804195797));
#156318=CARTESIAN_POINT('Ctrl Pts',(0.284611522344327,-7.00807448913602,
21.2864522953643));
#156319=CARTESIAN_POINT('Ctrl Pts',(0.475183323466393,-6.99512883166561,
21.2951241711488));
#156320=CARTESIAN_POINT('Ctrl Pts',(0.665753950390514,-6.98218325395917,
21.303795993502));
#156321=CARTESIAN_POINT('Ctrl Pts',(0.855795120323037,-6.96144568508293,
21.3124678158553));
#156322=CARTESIAN_POINT('Ctrl Pts',(1.04467275075973,-6.93298531704201,
21.3211396382085));
#156323=CARTESIAN_POINT('Ctrl Pts',(1.23354927906054,-6.9045251150726,21.32981140996));
#156324=CARTESIAN_POINT('Ctrl Pts',(1.42126200062534,-6.86834224643164,
21.3384831817116));
#156325=CARTESIAN_POINT('Ctrl Pts',(1.60718460924413,-6.82455743578357,
21.3471549534631));
#156326=CARTESIAN_POINT('Ctrl Pts',(1.79763389405557,-6.77970659200789,
21.3560378577016));
#156327=CARTESIAN_POINT('Ctrl Pts',(1.98620448431575,-6.72687898190956,
21.3649207619401));
#156328=CARTESIAN_POINT('Ctrl Pts',(2.17223623427553,-6.66625954377719,
21.3738036661786));
#156329=CARTESIAN_POINT('Ctrl Pts',(2.35386532185741,-6.60707473666718,
21.3824763459349));
#156330=CARTESIAN_POINT('Ctrl Pts',(2.53307410227393,-6.54046283696633,
21.3911490256913));
#156331=CARTESIAN_POINT('Ctrl Pts',(2.7092645177397,-6.4666461427402,21.3998217054476));
#156332=CARTESIAN_POINT('Ctrl Pts',(2.88545151535885,-6.39283088045427,
21.4084942169662));
#156333=CARTESIAN_POINT('Ctrl Pts',(3.05862000314107,-6.31181121311163,
21.4171667284847));
#156334=CARTESIAN_POINT('Ctrl Pts',(3.2281921034394,-6.22385751008099,21.4258392400032));
#156335=CARTESIAN_POINT('Ctrl Pts',(3.39776113570824,-6.13590539837672,
21.434511594612));
#156336=CARTESIAN_POINT('Ctrl Pts',(3.56373365850942,-6.04101963284054,
21.4431839492208));
#156337=CARTESIAN_POINT('Ctrl Pts',(3.7255558277513,-5.93951684371787,21.4518563038295));
#156338=CARTESIAN_POINT('Ctrl Pts',(3.88737528046358,-5.8380157585356,21.4605285128543));
#156339=CARTESIAN_POINT('Ctrl Pts',(4.04504427838794,-5.72989802299747,
21.4692007218791));
#156340=CARTESIAN_POINT('Ctrl Pts',(4.19803670363096,-5.6155244098363,21.477872930904));
#156341=CARTESIAN_POINT('Ctrl Pts',(4.35102676029949,-5.50115256736686,
21.4865450056687));
#156342=CARTESIAN_POINT('Ctrl Pts',(4.49934016166337,-5.38052521116037,
21.4952170804335));
#156343=CARTESIAN_POINT('Ctrl Pts',(4.64248202336562,-5.25404484423449,
21.5038891551982));
#156344=CARTESIAN_POINT('Ctrl Pts',(4.78562185584374,-5.12756627033415,
21.5125611070249));
#156345=CARTESIAN_POINT('Ctrl Pts',(4.92359008252299,-4.99523503982335,
21.5212330588516));
#156346=CARTESIAN_POINT('Ctrl Pts',(5.0559263513206,-4.85749269608529,21.5299050106783));
#156347=CARTESIAN_POINT('Ctrl Pts',(5.18826091680201,-4.71975212524569,
21.5385768508873));
#156348=CARTESIAN_POINT('Ctrl Pts',(5.3149634726938,-4.57660078535446,21.5472486910962));
#156349=CARTESIAN_POINT('Ctrl Pts',(5.43561126741811,-4.4285163104608,21.5559205313051));
#156350=CARTESIAN_POINT('Ctrl Pts',(5.56176013705541,-4.27367975367701,
21.5649877740387));
#156351=CARTESIAN_POINT('Ctrl Pts',(5.68128895686487,-4.11344992041142,
21.5740550167723));
#156352=CARTESIAN_POINT('Ctrl Pts',(5.79376175353991,-3.9484112381714,21.5831222595058));
#156353=CARTESIAN_POINT('Ctrl Pts',(5.90133874236296,-3.79055649462837,
21.5917948158842));
#156354=CARTESIAN_POINT('Ctrl Pts',(6.00246078174175,-3.62830291661756,
21.6004673722627));
#156355=CARTESIAN_POINT('Ctrl Pts',(6.09679041553253,-3.4621919634201,21.6091399286411));
#156356=CARTESIAN_POINT('Ctrl Pts',(6.19111669178686,-3.2960869227186,21.6178121763316));
#156357=CARTESIAN_POINT('Ctrl Pts',(6.27865090596248,-3.12612502860889,
21.626484424022));
#156358=CARTESIAN_POINT('Ctrl Pts',(6.35910096686059,-2.95287342359484,
21.6351566717124));
#156359=CARTESIAN_POINT('Ctrl Pts',(6.43954858437011,-2.77962708049096,
21.6438286560138));
#156360=CARTESIAN_POINT('Ctrl Pts',(6.51291235951956,-2.60309148403956,
21.6525006403151));
#156361=CARTESIAN_POINT('Ctrl Pts',(6.57894750102473,-2.42385567665661,
21.6611726246164));
#156362=CARTESIAN_POINT('Ctrl Pts',(6.64498098171129,-2.24462437714869,
21.6698443908128));
#156363=CARTESIAN_POINT('Ctrl Pts',(6.70368609940885,-2.06269326909929,
21.6785161570091));
#156364=CARTESIAN_POINT('Ctrl Pts',(6.75486698389396,-1.8786693675044,21.6871879232055));
#156365=CARTESIAN_POINT('Ctrl Pts',(6.80605126222514,-1.69463326313493,
21.6958602644337));
#156366=CARTESIAN_POINT('Ctrl Pts',(6.84971023276636,-1.50850436117886,
21.7045326056619));
#156367=CARTESIAN_POINT('Ctrl Pts',(6.88569820761737,-1.32090376489543,
21.7132049468901));
#156368=CARTESIAN_POINT('Ctrl Pts',(6.92168406448238,-1.13331420939547,
21.7218767777285));
#156369=CARTESIAN_POINT('Ctrl Pts',(6.94999977553796,-0.944253411828243,
21.7305486085668));
#156370=CARTESIAN_POINT('Ctrl Pts',(6.97055086371853,-0.754352184866494,
21.7392204394052));
#156371=CARTESIAN_POINT('Ctrl Pts',(6.99110229108013,-0.564447823720618,
21.7478924133659));
#156372=CARTESIAN_POINT('Ctrl Pts',(7.00388880856486,-0.373703287794897,
21.7565643873267));
#156373=CARTESIAN_POINT('Ctrl Pts',(7.00886775178458,-0.182755028642745,
21.7652363612874));
#156374=CARTESIAN_POINT('Ctrl Pts',(7.01045582731893,-0.121850486191596,
21.7680023598284));
#156375=CARTESIAN_POINT('Ctrl Pts',(7.01125000000004,-0.0609252433283521,
21.7707683583695));
#156376=CARTESIAN_POINT('Ctrl Pts',(7.01125,3.83823541218097E-12,21.7735343569105));
#156377=CARTESIAN_POINT('Ctrl Pts',(7.01124999865213,0.000137478978161555,
21.7735343569105));
#156378=CARTESIAN_POINT('Ctrl Pts',(7.01124653752022,0.176650728114333,
21.7815317420282));
#156379=CARTESIAN_POINT('Ctrl Pts',(7.00457296038423,0.353198568577369,
21.789529127146));
#156380=CARTESIAN_POINT('Ctrl Pts',(6.99124745647898,0.529231107150913,
21.7975265122637));
#156381=CARTESIAN_POINT('Ctrl Pts',(6.97791763612368,0.705320666882237,
21.8055264879262));
#156382=CARTESIAN_POINT('Ctrl Pts',(6.95793160765761,0.880894222625239,
21.8135264635886));
#156383=CARTESIAN_POINT('Ctrl Pts',(6.93135956303297,1.05540568998441,21.821526439251));
#156384=CARTESIAN_POINT('Ctrl Pts',(6.90478331956185,1.22994473319893,21.8295276790491));
#156385=CARTESIAN_POINT('Ctrl Pts',(6.87161905072997,1.40342099010502,21.8375289188472));
#156386=CARTESIAN_POINT('Ctrl Pts',(6.83198821305204,1.57529794617335,21.8455301586453));
#156387=CARTESIAN_POINT('Ctrl Pts',(6.7923256440326,1.74731251947895,21.8535378048201));
#156388=CARTESIAN_POINT('Ctrl Pts',(6.7461862551461,1.91772487634906,21.8615454509948));
#156389=CARTESIAN_POINT('Ctrl Pts',(6.69374175506267,2.0860124350134,21.8695530971696));
#156390=CARTESIAN_POINT('Ctrl Pts',(6.65608715443015,2.20684113588473,21.8753025030794));
#156391=CARTESIAN_POINT('Ctrl Pts',(6.61518326434292,2.3265747896752,21.8810519089892));
#156392=CARTESIAN_POINT('Ctrl Pts',(6.57110895151813,2.44502632087638,21.886801314899));
#156393=CARTESIAN_POINT('',(7.01124789938016,0.00542733243739705,21.2264656430542));
#156394=CARTESIAN_POINT('Ctrl Pts',(6.57110895151816,2.44502632087631,21.3399745565681));
#156395=CARTESIAN_POINT('Ctrl Pts',(6.63539956021585,2.2722426617783,21.3315965673332));
#156396=CARTESIAN_POINT('Ctrl Pts',(6.69284066714934,2.09700392013267,21.3232185780983));
#156397=CARTESIAN_POINT('Ctrl Pts',(6.74326910937081,1.91988236126734,21.3148405888634));
#156398=CARTESIAN_POINT('Ctrl Pts',(6.79372545835688,1.74266278450909,21.306457963305));
#156399=CARTESIAN_POINT('Ctrl Pts',(6.83716132020599,1.56355863023882,21.2980753377466));
#156400=CARTESIAN_POINT('Ctrl Pts',(6.87346441855802,1.3831534438799,21.2896927121881));
#156401=CARTESIAN_POINT('Ctrl Pts',(6.90980485689981,1.20256269959023,21.2813014645791));
#156402=CARTESIAN_POINT('Ctrl Pts',(6.93899782154279,1.02066857367475,21.27291021697));
#156403=CARTESIAN_POINT('Ctrl Pts',(6.9609826087011,0.838061861595461,21.2645189693609));
#156404=CARTESIAN_POINT('Ctrl Pts',(6.96367123658769,0.815729987520962,
21.2634927623678));
#156405=CARTESIAN_POINT('Ctrl Pts',(6.96625212254389,0.793387459064572,
21.2624665553746));
#156406=CARTESIAN_POINT('Ctrl Pts',(6.96872520897261,0.771035358676671,
21.2614403483814));
#156407=CARTESIAN_POINT('Ctrl Pts',(6.99682073277436,0.517104092395202,
21.2497821132842));
#156408=CARTESIAN_POINT('Ctrl Pts',(7.01104969501965,0.261475717700782,
21.2381238781869));
#156409=CARTESIAN_POINT('Ctrl Pts',(7.01124789937955,0.00542733321588756,
21.2264656430896));
#156410=CARTESIAN_POINT('Ctrl Pts',(7.01124789938016,0.00542733243739238,
21.2264656430541));
#156411=CARTESIAN_POINT('Ctrl Pts',(7.01138511315678,-0.171830982620558,
21.2183948281805));
#156412=CARTESIAN_POINT('Ctrl Pts',(7.00479604016339,-0.349336638244306,
21.2103240133068));
#156413=CARTESIAN_POINT('Ctrl Pts',(6.99145108150332,-0.526534269963628,
21.2022531984331));
#156414=CARTESIAN_POINT('Ctrl Pts',(6.97774366041824,-0.708544766595712,
21.1939631721549));
#156415=CARTESIAN_POINT('Ctrl Pts',(6.95690808489991,-0.890229896830883,
21.1856731458768));
#156416=CARTESIAN_POINT('Ctrl Pts',(6.92896952314784,-1.07098455161054,
21.1773831195986));
#156417=CARTESIAN_POINT('Ctrl Pts',(6.90182288203468,-1.2466157020749,21.1693280747402));
#156418=CARTESIAN_POINT('Ctrl Pts',(6.86797047923098,-1.42136801354171,
21.1612730298818));
#156419=CARTESIAN_POINT('Ctrl Pts',(6.82748809657842,-1.59468895198405,
21.1532179850234));
#156420=CARTESIAN_POINT('Ctrl Pts',(6.7852342884555,-1.77559405679175,21.1448104680353));
#156421=CARTESIAN_POINT('Ctrl Pts',(6.73575721398845,-1.95493929691785,
21.1364029510473));
#156422=CARTESIAN_POINT('Ctrl Pts',(6.67920292101102,-2.13210574373267,
21.1279954340592));
#156423=CARTESIAN_POINT('Ctrl Pts',(6.62264862803358,-2.30927219054752,
21.1195879170711));
#156424=CARTESIAN_POINT('Ctrl Pts',(6.55901722681694,-2.48425940783944,
21.1111804000831));
#156425=CARTESIAN_POINT('Ctrl Pts',(6.48851466909079,-2.6564645586745,21.102772883095));
#156426=CARTESIAN_POINT('Ctrl Pts',(6.41859245493036,-2.82725219850719,
21.0944345727931));
#156427=CARTESIAN_POINT('Ctrl Pts',(6.34195188302819,-2.995207309943,21.0860962624912));
#156428=CARTESIAN_POINT('Ctrl Pts',(6.25885887899983,-3.15979621103402,
21.0777579521894));
#156429=CARTESIAN_POINT('Ctrl Pts',(6.17571359567259,-3.32448866587731,
21.0694143957056));
#156430=CARTESIAN_POINT('Ctrl Pts',(6.08610793040353,-3.48581039346066,
21.0610708392217));
#156431=CARTESIAN_POINT('Ctrl Pts',(5.99035317373886,-3.64325341094697,
21.0527272827379));
#156432=CARTESIAN_POINT('Ctrl Pts',(5.89452556727291,-3.80081621039437,
21.0443773785127));
#156433=CARTESIAN_POINT('Ctrl Pts',(5.79253970798989,-3.95449413402541,
21.0360274742875));
#156434=CARTESIAN_POINT('Ctrl Pts',(5.68474973207407,-4.1038088462042,21.0276775700623));
#156435=CARTESIAN_POINT('Ctrl Pts',(5.57679807917088,-4.25334751940189,
21.0193151415987));
#156436=CARTESIAN_POINT('Ctrl Pts',(5.46302510476374,-4.39850963729829,
21.0109527131351));
#156437=CARTESIAN_POINT('Ctrl Pts',(5.34382565034685,-4.53884941160147,
21.0025902846714));
#156438=CARTESIAN_POINT('Ctrl Pts',(5.22452426414693,-4.67930919554309,
20.9942207051915));
#156439=CARTESIAN_POINT('Ctrl Pts',(5.09978736044891,-4.81493816732931,
20.9858511257115));
#156440=CARTESIAN_POINT('Ctrl Pts',(4.97004642620975,-4.94532760126361,
20.9774815462315));
#156441=CARTESIAN_POINT('Ctrl Pts',(4.84010538238685,-5.07591814501342,
20.969099057695));
#156442=CARTESIAN_POINT('Ctrl Pts',(4.70514512456409,-5.20125277943508,
20.9607165691584));
#156443=CARTESIAN_POINT('Ctrl Pts',(4.56563102382614,-5.32096231115917,
20.9523340806218));
#156444=CARTESIAN_POINT('Ctrl Pts',(4.51997972399048,-5.36013323149637,
20.9495911930174));
#156445=CARTESIAN_POINT('Ctrl Pts',(4.47384107817438,-5.39870221086967,
20.946848305413));
#156446=CARTESIAN_POINT('Ctrl Pts',(4.42723205493133,-5.43665732728195,
20.9441054178086));
#156447=CARTESIAN_POINT('Ctrl Pts',(4.28466589499679,-5.55275319928833,
20.9357155626758));
#156448=CARTESIAN_POINT('Ctrl Pts',(4.13740883337341,-5.66333692192345,
20.927325707543));
#156449=CARTESIAN_POINT('Ctrl Pts',(3.98591391741853,-5.76802538182949,
20.9189358524102));
#156450=CARTESIAN_POINT('Ctrl Pts',(3.83455879884845,-5.87261723669225,
20.9105537393182));
#156451=CARTESIAN_POINT('Ctrl Pts',(3.67897389091956,-5.97132448761094,
20.9021716262261));
#156452=CARTESIAN_POINT('Ctrl Pts',(3.51964451587096,-6.0638048323144,20.893789513134));
#156453=CARTESIAN_POINT('Ctrl Pts',(3.36043874664803,-6.1562134318713,20.8854139027851));
#156454=CARTESIAN_POINT('Ctrl Pts',(3.19749458510163,-6.24240459184712,
20.8770382924362));
#156455=CARTESIAN_POINT('Ctrl Pts',(3.03132585956567,-6.3220795704917,20.8686626820873));
#156456=CARTESIAN_POINT('Ctrl Pts',(2.86526165662619,-6.40170443239128,
20.8602923401217));
#156457=CARTESIAN_POINT('Ctrl Pts',(2.69597722959344,-6.47482114378974,
20.8519219981561));
#156458=CARTESIAN_POINT('Ctrl Pts',(2.52401090988896,-6.54117691927542,
20.8435516561905));
#156459=CARTESIAN_POINT('Ctrl Pts',(2.3521275512209,-6.60750068300487,20.8351853522961));
#156460=CARTESIAN_POINT('Ctrl Pts',(2.17756518609516,-6.66706989695571,
20.8268190484018));
#156461=CARTESIAN_POINT('Ctrl Pts',(2.00088244508062,-6.71967975453207,
20.8184527445074));
#156462=CARTESIAN_POINT('Ctrl Pts',(1.82424911727737,-6.77227489860562,
20.8100887804338));
#156463=CARTESIAN_POINT('Ctrl Pts',(1.64549691033531,-6.81791447217926,
20.8017248163601));
#156464=CARTESIAN_POINT('Ctrl Pts',(1.46520048148912,-6.85644325518297,
20.7933608522865));
#156465=CARTESIAN_POINT('Ctrl Pts',(1.28493179726724,-6.89496610924723,
20.784998175288));
#156466=CARTESIAN_POINT('Ctrl Pts',(1.10311968623601,-6.92638028575991,
20.7766354982894));
#156467=CARTESIAN_POINT('Ctrl Pts',(0.920350300438577,-6.95058140639923,
20.7682728212909));
#156468=CARTESIAN_POINT('Ctrl Pts',(0.737584677529384,-6.97478202878161,
20.7599103164646));
#156469=CARTESIAN_POINT('Ctrl Pts',(0.553862145010406,-6.99176984866476,
20.7515478116383));
#156470=CARTESIAN_POINT('Ctrl Pts',(0.369775734505855,-7.00149216015205,
20.743185306812));
#156471=CARTESIAN_POINT('Ctrl Pts',(0.18566857659615,-7.01121556738963,
20.734821859492));
#156472=CARTESIAN_POINT('Ctrl Pts',(0.00119778714406746,-7.01367181686933,
20.7264584121721));
#156473=CARTESIAN_POINT('Ctrl Pts',(-0.183041394477139,-7.00886027899029,
20.7180949648521));
#156474=CARTESIAN_POINT('Ctrl Pts',(-0.367389061307,-7.00404590794251,20.7097265928993));
#156475=CARTESIAN_POINT('Ctrl Pts',(-0.551504518878142,-6.99195520574972,
20.7013582209465));
#156476=CARTESIAN_POINT('Ctrl Pts',(-0.73479440003731,-6.9726396545479,
20.6929898489937));
#156477=CARTESIAN_POINT('Ctrl Pts',(-0.918139199635379,-6.9533183159021,
20.684618969658));
#156478=CARTESIAN_POINT('Ctrl Pts',(-1.1006576032259,-6.92676785149453,
20.6762480903222));
#156479=CARTESIAN_POINT('Ctrl Pts',(-1.2817635414756,-6.89309138095847,
20.6678772109864));
#156480=CARTESIAN_POINT('Ctrl Pts',(-1.46302292882833,-6.8593863767131,
20.6594992390951));
#156481=CARTESIAN_POINT('Ctrl Pts',(-1.64286713709922,-6.81854336718237,
20.6511212672038));
#156482=CARTESIAN_POINT('Ctrl Pts',(-1.82072128778139,-6.77071639892853,
20.6427432953125));
#156483=CARTESIAN_POINT('Ctrl Pts',(-1.93374904881,-6.74032197114721,20.6374190259536));
#156484=CARTESIAN_POINT('Ctrl Pts',(-2.04597335456467,-6.70710794305146,
20.6320947565947));
#156485=CARTESIAN_POINT('Ctrl Pts',(-2.15725019586194,-6.67112420473144,
20.6267704872357));
#156486=CARTESIAN_POINT('Ctrl Pts',(-2.32158279427387,-6.61798375655042,
20.6189076560465));
#156487=CARTESIAN_POINT('Ctrl Pts',(-2.48418984036692,-6.55868970666415,
20.6110448248572));
#156488=CARTESIAN_POINT('Ctrl Pts',(-2.64455671375529,-6.4933771144322,
20.6031819936679));
#156489=CARTESIAN_POINT('Ctrl Pts',(-2.80480036636881,-6.42811470630656,
20.5953252040265));
#156490=CARTESIAN_POINT('Ctrl Pts',(-2.96280691845738,-6.35684309511127,
20.5874684143852));
#156491=CARTESIAN_POINT('Ctrl Pts',(-3.11807649193003,-6.27974725231624,
20.5796116247438));
#156492=CARTESIAN_POINT('Ctrl Pts',(-3.27325850071401,-6.20269488792668,
20.5717592659599));
#156493=CARTESIAN_POINT('Ctrl Pts',(-3.42570626088162,-6.11982499477387,
20.5639069071759));
#156494=CARTESIAN_POINT('Ctrl Pts',(-3.5749397274518,-6.0313706989031,20.556054548392));
#156495=CARTESIAN_POINT('Ctrl Pts',(-3.72413795825914,-5.94293728812374,
20.5482040436415));
#156496=CARTESIAN_POINT('Ctrl Pts',(-3.87012307396475,-5.84892228586267,
20.5403535388911));
#156497=CARTESIAN_POINT('Ctrl Pts',(-4.01243957350879,-5.74960478915208,
20.5325030341407));
#156498=CARTESIAN_POINT('Ctrl Pts',(-4.15473317881393,-5.6503032694962,
20.5246537922891));
#156499=CARTESIAN_POINT('Ctrl Pts',(-4.29335903164857,-5.54570117428187,
20.5168045504374));
#156500=CARTESIAN_POINT('Ctrl Pts',(-4.42789097195009,-5.43612068510467,
20.5089553085858));
#156501=CARTESIAN_POINT('Ctrl Pts',(-4.56246823869516,-5.32650327611613,
20.5011034221709));
#156502=CARTESIAN_POINT('Ctrl Pts',(-4.69294854172649,-5.21190436398546,
20.4932515357561));
#156503=CARTESIAN_POINT('Ctrl Pts',(-4.81893900704827,-5.09268626648536,
20.4853996493412));
#156504=CARTESIAN_POINT('Ctrl Pts',(-4.91145223756234,-5.00514590136879,
20.4796341068773));
#156505=CARTESIAN_POINT('Ctrl Pts',(-5.0015453307585,-4.9151158191756,20.4738685644133));
#156506=CARTESIAN_POINT('Ctrl Pts',(-5.08907563104132,-4.8227518891232,
20.4681030219493));
#156507=CARTESIAN_POINT('Ctrl Pts',(-5.23565883552314,-4.66807401412598,
20.4584477175894));
#156508=CARTESIAN_POINT('Ctrl Pts',(-5.37497948782157,-4.50692938614802,
20.4487924132295));
#156509=CARTESIAN_POINT('Ctrl Pts',(-5.50656696611878,-4.33997083056435,
20.4391371088697));
#156510=CARTESIAN_POINT('Ctrl Pts',(-5.63888341436103,-4.17208735590279,
20.4294283159349));
#156511=CARTESIAN_POINT('Ctrl Pts',(-5.76338078437975,-3.99832542999536,
20.4197195230001));
#156512=CARTESIAN_POINT('Ctrl Pts',(-5.87962792320022,-3.81937194407984,
20.4100107300653));
#156513=CARTESIAN_POINT('Ctrl Pts',(-5.99643445312257,-3.6395573187962,
20.4002552175946));
#156514=CARTESIAN_POINT('Ctrl Pts',(-6.10491115573031,-3.45450109818584,
20.3904997051239));
#156515=CARTESIAN_POINT('Ctrl Pts',(-6.20466818990484,-3.26492254359625,
20.3807441926532));
#156516=CARTESIAN_POINT('Ctrl Pts',(-6.30452399889056,-3.07515627707146,
20.3709790207242));
#156517=CARTESIAN_POINT('Ctrl Pts',(-6.39564286188179,-2.88085875906645,
20.3612138487953));
#156518=CARTESIAN_POINT('Ctrl Pts',(-6.47768131127819,-2.68277307874096,
20.3514486768664));
#156519=CARTESIAN_POINT('Ctrl Pts',(-6.55960790311003,-2.48495748374668,
20.3416968195279));
#156520=CARTESIAN_POINT('Ctrl Pts',(-6.63247881191103,-2.28336408463178,
20.3319449621894));
#156521=CARTESIAN_POINT('Ctrl Pts',(-6.69599944080583,-2.07875396601617,
20.3221931048508));
#156522=CARTESIAN_POINT('Ctrl Pts',(-6.72369903538632,-1.98952913573145,
20.3179405887882));
#156523=CARTESIAN_POINT('Ctrl Pts',(-6.74962119971176,-1.89973091568127,
20.3136880727255));
#156524=CARTESIAN_POINT('Ctrl Pts',(-6.77374435742456,-1.80942364933117,
20.3094355566629));
#156525=CARTESIAN_POINT('Ctrl Pts',(-6.81931324488791,-1.63883231521045,
20.3014025110641));
#156526=CARTESIAN_POINT('Ctrl Pts',(-6.85848122771501,-1.46634030115633,
20.2933694654652));
#156527=CARTESIAN_POINT('Ctrl Pts',(-6.89109073719453,-1.29247631090546,
20.2853364198664));
#156528=CARTESIAN_POINT('Ctrl Pts',(-6.9236792840256,-1.1187240871228,20.2773085382186));
#156529=CARTESIAN_POINT('Ctrl Pts',(-6.94971768234484,-0.943602001488677,
20.2692806565709));
#156530=CARTESIAN_POINT('Ctrl Pts',(-6.96909872353552,-0.767651968092048,
20.2612527749231));
#156531=CARTESIAN_POINT('Ctrl Pts',(-6.98847101399519,-0.591781377868698,
20.253228517943));
#156532=CARTESIAN_POINT('Ctrl Pts',(-7.00119189229136,-0.415083947823816,
20.2452042609628));
#156533=CARTESIAN_POINT('Ctrl Pts',(-7.00720559944525,-0.23810974277255,
20.2371800039827));
#156534=CARTESIAN_POINT('Ctrl Pts',(-7.01321857948067,-0.0611569357055864,
20.229156717217));
#156535=CARTESIAN_POINT('Ctrl Pts',(-7.01252598353118,0.116072213828916,
20.2211334304513));
#156536=CARTESIAN_POINT('Ctrl Pts',(-7.00512407177512,0.293024404336646,
20.2131101436856));
#156537=CARTESIAN_POINT('Ctrl Pts',(-6.99772276653969,0.469962095190731,
20.2050875143566));
#156538=CARTESIAN_POINT('Ctrl Pts',(-6.9836132599218,0.646622506066317,
20.1970648850277));
#156539=CARTESIAN_POINT('Ctrl Pts',(-6.9628438952237,0.822454529591783,
20.1890422556988));
#156540=CARTESIAN_POINT('Ctrl Pts',(-6.94206672272314,0.998352653439866,
20.1810166104324));
#156541=CARTESIAN_POINT('Ctrl Pts',(-6.91462473673029,1.1734214039036,20.172990965166));
#156542=CARTESIAN_POINT('Ctrl Pts',(-6.88061795613055,1.34711658896841,
20.1649653198996));
#156543=CARTESIAN_POINT('Ctrl Pts',(-6.86056548601809,1.44953785454439,
20.1602329103919));
#156544=CARTESIAN_POINT('Ctrl Pts',(-6.83823141035492,1.55148170121444,
20.1555005008842));
#156545=CARTESIAN_POINT('Ctrl Pts',(-6.81364449281798,1.65283855472677,
20.1507680913764));
#156546=CARTESIAN_POINT('Ctrl Pts',(-6.76828810714593,1.83981524798255,
20.1420380425418));
#156547=CARTESIAN_POINT('Ctrl Pts',(-6.71524003955314,2.02488717757644,
20.1333079937072));
#156548=CARTESIAN_POINT('Ctrl Pts',(-6.65468693636266,2.20743478759943,
20.1245779448725));
#156549=CARTESIAN_POINT('Ctrl Pts',(-6.59411632416657,2.39003518149246,
20.1158453717334));
#156550=CARTESIAN_POINT('Ctrl Pts',(-6.52603643100342,2.57010953886378,
20.1071127985942));
#156551=CARTESIAN_POINT('Ctrl Pts',(-6.4506831321688,2.74705545827762,20.098380225455));
#156552=CARTESIAN_POINT('Ctrl Pts',(-6.37425931943792,2.92651517693516,
20.0895235921746));
#156553=CARTESIAN_POINT('Ctrl Pts',(-6.29035397886495,3.1027566245927,20.0806669588942));
#156554=CARTESIAN_POINT('Ctrl Pts',(-6.19926304082612,3.27517393631961,
20.0718103256138));
#156555=CARTESIAN_POINT('Ctrl Pts',(-6.10939089357683,3.44528431569942,
20.063072193507));
#156556=CARTESIAN_POINT('Ctrl Pts',(-6.01252439058699,3.61167202223607,
20.0543340614003));
#156557=CARTESIAN_POINT('Ctrl Pts',(-5.90899371920414,3.77378056978755,
20.0455959292935));
#156558=CARTESIAN_POINT('Ctrl Pts',(-5.80335701888056,3.93918674197647,
20.0366800454263));
#156559=CARTESIAN_POINT('Ctrl Pts',(-5.69078227619342,4.1001375447335,20.027764161559));
#156560=CARTESIAN_POINT('Ctrl Pts',(-5.57166689361946,4.25607267196472,
20.0188482776918));
#156561=CARTESIAN_POINT('Ctrl Pts',(-5.45255151104551,4.41200779919593,
20.0099323938245));
#156562=CARTESIAN_POINT('Ctrl Pts',(-5.32689567699348,4.56292701427444,
20.0010165099573));
#156563=CARTESIAN_POINT('Ctrl Pts',(-5.19514124450627,4.7083047917621,19.99210062609));
#156564=CARTESIAN_POINT('Ctrl Pts',(-5.06597581991149,4.85082585918546,
19.9833599415938));
#156565=CARTESIAN_POINT('Ctrl Pts',(-4.93093553144688,4.98803638595718,
19.9746192570976));
#156566=CARTESIAN_POINT('Ctrl Pts',(-4.79047193705921,5.1194731352697,19.9658785726013));
#156567=CARTESIAN_POINT('Ctrl Pts',(-4.65003361440603,5.25088623692714,
19.9571394606995));
#156568=CARTESIAN_POINT('Ctrl Pts',(-4.50417413431041,5.37652744868072,
19.9484003487976));
#156569=CARTESIAN_POINT('Ctrl Pts',(-4.35338084660384,5.49597141249141,
19.9396612368958));
#156570=CARTESIAN_POINT('Ctrl Pts',(-4.20063381482535,5.61696294476334,
19.9308088972214));
#156571=CARTESIAN_POINT('Ctrl Pts',(-4.04282444450216,5.73159532650693,
19.9219565575471));
#156572=CARTESIAN_POINT('Ctrl Pts',(-3.8804937669024,5.83946869907971,19.9131042178727));
#156573=CARTESIAN_POINT('Ctrl Pts',(-3.72032155381722,5.9459077103216,19.904369585223));
#156574=CARTESIAN_POINT('Ctrl Pts',(-3.5557477655038,6.04576619743504,19.8956349525732));
#156575=CARTESIAN_POINT('Ctrl Pts',(-3.38732197767626,6.13870315148496,
19.8869003199234));
#156576=CARTESIAN_POINT('Ctrl Pts',(-3.21549165657141,6.23351871899922,
19.8779891267368));
#156577=CARTESIAN_POINT('Ctrl Pts',(-3.03965219368265,6.32112979232151,
19.8690779335502));
#156578=CARTESIAN_POINT('Ctrl Pts',(-2.86041524351101,6.40122263299675,
19.8601667403635));
#156579=CARTESIAN_POINT('Ctrl Pts',(-2.68117829333937,6.481315473672,19.8512555471769));
#156580=CARTESIAN_POINT('Ctrl Pts',(-2.49854412714317,6.55388994572913,
19.8423443539902));
#156581=CARTESIAN_POINT('Ctrl Pts',(-2.31314879546395,6.61868334433244,
19.8334331608036));
#156582=CARTESIAN_POINT('Ctrl Pts',(-2.1461766778035,6.67703805519394,19.8254074959512));
#156583=CARTESIAN_POINT('Ctrl Pts',(-1.9768879904627,6.72910763299868,19.8173818310988));
#156584=CARTESIAN_POINT('Ctrl Pts',(-1.80580461755068,6.77471004883107,
19.8093561662464));
#156585=CARTESIAN_POINT('Ctrl Pts',(-1.63477554230475,6.82029799157525,
19.8013330485432));
#156586=CARTESIAN_POINT('Ctrl Pts',(-1.46195326926839,6.85942276441783,
19.79330993084));
#156587=CARTESIAN_POINT('Ctrl Pts',(-1.28787484800511,6.89195218630947,
19.7852868131368));
#156588=CARTESIAN_POINT('Ctrl Pts',(-1.11381837955452,6.92447750595626,
19.7772647072189));
#156589=CARTESIAN_POINT('Ctrl Pts',(-0.938506438753643,6.95040906463208,
19.7692426013011));
#156590=CARTESIAN_POINT('Ctrl Pts',(-0.762486221020042,6.96966579724269,
19.7612204953832));
#156591=CARTESIAN_POINT('Ctrl Pts',(-0.586400593578624,6.98892968572022,
19.7531954084237));
#156592=CARTESIAN_POINT('Ctrl Pts',(-0.409606527828915,7.00151375021644,
19.7451703214642));
#156593=CARTESIAN_POINT('Ctrl Pts',(-0.232656750402027,7.00738877178885,
19.7371452345047));
#156594=CARTESIAN_POINT('Ctrl Pts',(-0.0556721236026742,7.01326495041733,
19.7291185670444));
#156595=CARTESIAN_POINT('Ctrl Pts',(0.121467909313705,7.01242945049053,
19.7210918995842));
#156596=CARTESIAN_POINT('Ctrl Pts',(0.298210870223755,7.00490519845775,
19.713065232124));
#156597=CARTESIAN_POINT('Ctrl Pts',(0.475095719760626,6.99737490598193,
19.7050321208834));
#156598=CARTESIAN_POINT('Ctrl Pts',(0.65158249485985,6.9831451616253,19.6969990096428));
#156599=CARTESIAN_POINT('Ctrl Pts',(0.82712345741225,6.96229081184479,19.6889658984023));
#156600=CARTESIAN_POINT('Ctrl Pts',(0.930558569422978,6.95000267137836,
19.6842324974405));
#156601=CARTESIAN_POINT('Ctrl Pts',(1.03366543805472,6.93541544974664,19.6794990964788));
#156602=CARTESIAN_POINT('Ctrl Pts',(1.1363337643841,6.9185527488356,19.6747656955171));
#156603=CARTESIAN_POINT('Ctrl Pts',(1.34783371187111,6.88381506015708,19.6650147422229));
#156604=CARTESIAN_POINT('Ctrl Pts',(1.55759675625066,6.83939833325033,19.6552637889286));
#156605=CARTESIAN_POINT('Ctrl Pts',(1.76482985845557,6.78549940190136,19.6455128356344));
#156606=CARTESIAN_POINT('Ctrl Pts',(1.97236151881738,6.73152281903131,19.6357478342628));
#156607=CARTESIAN_POINT('Ctrl Pts',(2.17735590882976,6.6680367156351,19.6259828328913));
#156608=CARTESIAN_POINT('Ctrl Pts',(2.37903269260381,6.59528847056915,19.6162178315197));
#156609=CARTESIAN_POINT('Ctrl Pts',(2.58037332296702,6.52266148175417,19.6064691063821));
#156610=CARTESIAN_POINT('Ctrl Pts',(2.7784073631806,6.44080321856691,19.5967203812445));
#156611=CARTESIAN_POINT('Ctrl Pts',(2.97237492972121,6.35000896374681,19.5869716561069));
#156612=CARTESIAN_POINT('Ctrl Pts',(3.16581013049678,6.25946390395344,19.57724968744));
#156613=CARTESIAN_POINT('Ctrl Pts',(3.35520110233162,6.16003183127222,19.5675277187732));
#156614=CARTESIAN_POINT('Ctrl Pts',(3.53981127424797,6.05205442021195,19.5578057501063));
#156615=CARTESIAN_POINT('Ctrl Pts',(3.72319992887888,5.94479146747582,19.5481481091666));
#156616=CARTESIAN_POINT('Ctrl Pts',(3.90187078622064,5.82909588576575,19.5384904682269));
#156617=CARTESIAN_POINT('Ctrl Pts',(4.07511940342092,5.70535085777925,19.5288328272872));
#156618=CARTESIAN_POINT('Ctrl Pts',(4.15126813527024,5.65096065769506,19.5245879616017));
#156619=CARTESIAN_POINT('Ctrl Pts',(4.22636957634119,5.59501601051856,19.5203430959162));
#156620=CARTESIAN_POINT('Ctrl Pts',(4.30036504556353,5.5375524410515,19.5160982302307));
#156621=CARTESIAN_POINT('Ctrl Pts',(4.43723653858669,5.43126046628527,19.5082463832168));
#156622=CARTESIAN_POINT('Ctrl Pts',(4.57026540768506,5.31981216424165,19.5003945362029));
#156623=CARTESIAN_POINT('Ctrl Pts',(4.69902863801488,5.20353307106009,19.492542689189));
#156624=CARTESIAN_POINT('Ctrl Pts',(4.82775535213286,5.08728695368993,19.4846930688955));
#156625=CARTESIAN_POINT('Ctrl Pts',(4.95221855095236,4.96621302570285,19.4768434486019));
#156626=CARTESIAN_POINT('Ctrl Pts',(5.07202870601983,4.84067674688269,19.4689938283084));
#156627=CARTESIAN_POINT('Ctrl Pts',(5.19182929578005,4.71515049052748,19.4611448347065));
#156628=CARTESIAN_POINT('Ctrl Pts',(5.30697731848823,4.58516286903166,19.4532958411047));
#156629=CARTESIAN_POINT('Ctrl Pts',(5.41712068377745,4.45111559722847,19.4454468475029));
#156630=CARTESIAN_POINT('Ctrl Pts',(5.52731981142681,4.31700046121734,19.4375938801854));
#156631=CARTESIAN_POINT('Ctrl Pts',(5.63250897668519,4.17882186345816,19.429740912868));
#156632=CARTESIAN_POINT('Ctrl Pts',(5.73237671783214,4.0370142094568,19.4218879455506));
#156633=CARTESIAN_POINT('Ctrl Pts',(5.83226982203013,3.89517054107555,19.4140329838433));
#156634=CARTESIAN_POINT('Ctrl Pts',(5.92683860175204,3.74969630015664,19.406178022136));
#156635=CARTESIAN_POINT('Ctrl Pts',(6.01581578437549,3.60105359734602,19.3983230604287));
#156636=CARTESIAN_POINT('Ctrl Pts',(6.1048812842898,3.45226335422865,19.3904603020153));
#156637=CARTESIAN_POINT('Ctrl Pts',(6.18834391853178,3.300298702136,19.382597543602));
#156638=CARTESIAN_POINT('Ctrl Pts',(6.26598283970866,3.14564550052555,19.3747347851887));
#156639=CARTESIAN_POINT('Ctrl Pts',(6.32293763823132,3.03219413096644,19.3689667784406));
#156640=CARTESIAN_POINT('Ctrl Pts',(6.37675939458714,2.91729641313367,19.3631987716924));
#156641=CARTESIAN_POINT('Ctrl Pts',(6.42737773349486,2.80115012690761,19.3574307649443));
#156642=CARTESIAN_POINT('Ctrl Pts',(6.47852634438862,2.68378710534023,19.3516023332107));
#156643=CARTESIAN_POINT('Ctrl Pts',(6.52645943403865,2.56502373828055,19.3457739014771));
#156644=CARTESIAN_POINT('Ctrl Pts',(6.57110895151814,2.44502632087635,19.3399454697435));
#156645=CARTESIAN_POINT('Origin',(0.,0.,50.));
#156646=CARTESIAN_POINT('',(6.57110895151813,2.44502632087639,17.3396585048403));
#156647=CARTESIAN_POINT('',(6.57110895151814,2.44502632087637,17.886889234273));
#156648=CARTESIAN_POINT('',(6.57110895151814,2.44502632087636,50.));
#156649=CARTESIAN_POINT('',(7.01124873670978,-0.00420885798051574,19.7735343569105));
#156650=CARTESIAN_POINT('Ctrl Pts',(6.57110895151814,2.44502632087637,17.886889234273));
#156651=CARTESIAN_POINT('Ctrl Pts',(6.50720292022931,2.61677641234676,17.8952010218137));
#156652=CARTESIAN_POINT('Ctrl Pts',(6.43654999129877,2.7860443294507,17.9035128093544));
#156653=CARTESIAN_POINT('Ctrl Pts',(6.35937398010672,2.95228541026128,17.9118245968952));
#156654=CARTESIAN_POINT('Ctrl Pts',(6.28219796040125,3.11852650941021,17.9201363853528));
#156655=CARTESIAN_POINT('Ctrl Pts',(6.19849899777784,3.28174046743073,17.9284481738104));
#156656=CARTESIAN_POINT('Ctrl Pts',(6.10854821986263,3.44140454002622,17.936759962268));
#156657=CARTESIAN_POINT('Ctrl Pts',(6.01858428500979,3.6010919663969,17.9450729664759));
#156658=CARTESIAN_POINT('Ctrl Pts',(5.9223668763525,3.75722818017718,17.9533859706838));
#156659=CARTESIAN_POINT('Ctrl Pts',(5.82021223161276,3.90931658240738,17.9616989748917));
#156660=CARTESIAN_POINT('Ctrl Pts',(5.71802771142493,4.06144946337053,17.9700144102638));
#156661=CARTESIAN_POINT('Ctrl Pts',(5.60990268043997,4.20953189468716,17.978329845636));
#156662=CARTESIAN_POINT('Ctrl Pts',(5.49619589916734,4.35309742602622,17.9866452810082));
#156663=CARTESIAN_POINT('Ctrl Pts',(5.38238573978476,4.49679348197531,17.9949682764747));
#156664=CARTESIAN_POINT('Ctrl Pts',(5.26298389790001,4.63596416891988,18.0032912719412));
#156665=CARTESIAN_POINT('Ctrl Pts',(5.13838927820155,4.77017632673714,18.0116142674077));
#156666=CARTESIAN_POINT('Ctrl Pts',(5.01373525021222,4.9044524786091,18.0199412313838));
#156667=CARTESIAN_POINT('Ctrl Pts',(4.88388374072292,5.03376514662664,18.0282681953598));
#156668=CARTESIAN_POINT('Ctrl Pts',(4.74926986522116,5.15771871177579,18.0365951593359));
#156669=CARTESIAN_POINT('Ctrl Pts',(4.61449645450883,5.28181917826067,18.0449319918633));
#156670=CARTESIAN_POINT('Ctrl Pts',(4.47494965115375,5.40054762878076,18.0532688243908));
#156671=CARTESIAN_POINT('Ctrl Pts',(4.33109795261695,5.51354850231113,18.0616056569182));
#156672=CARTESIAN_POINT('Ctrl Pts',(4.22764270329482,5.59481645857174,18.0676013392526));
#156673=CARTESIAN_POINT('Ctrl Pts',(4.12196155486622,5.67312285929934,18.0735970215869));
#156674=CARTESIAN_POINT('Ctrl Pts',(4.0142377187002,5.74834951096962,18.0795927039213));
#156675=CARTESIAN_POINT('Ctrl Pts',(3.86365171675359,5.85350804521824,18.0879740043262));
#156676=CARTESIAN_POINT('Ctrl Pts',(3.70875556564004,5.95286840638979,18.0963553047311));
#156677=CARTESIAN_POINT('Ctrl Pts',(3.55002072808778,6.04607140155052,18.104736605136));
#156678=CARTESIAN_POINT('Ctrl Pts',(3.39148706370483,6.13915627555893,18.1131072834695));
#156679=CARTESIAN_POINT('Ctrl Pts',(3.2291246885253,6.22609917068576,18.1214779618031));
#156680=CARTESIAN_POINT('Ctrl Pts',(3.06343546059869,6.3065830479941,18.1298486401366));
#156681=CARTESIAN_POINT('Ctrl Pts',(2.89793426149854,6.38697558991999,18.1382098191875));
#156682=CARTESIAN_POINT('Ctrl Pts',(2.72911402738059,6.46092358098648,18.1465709982383));
#156683=CARTESIAN_POINT('Ctrl Pts',(2.55750312363193,6.52815474197058,18.1549321772891));
#156684=CARTESIAN_POINT('Ctrl Pts',(2.38611490527401,6.59529866259274,18.1632825067238));
#156685=CARTESIAN_POINT('Ctrl Pts',(2.21194354383317,6.65574301892446,18.1716328361585));
#156686=CARTESIAN_POINT('Ctrl Pts',(2.0355393095366,6.70926272267164,18.1799831655933));
#156687=CARTESIAN_POINT('Ctrl Pts',(1.85927080774591,6.76274124620831,18.188327069949));
#156688=CARTESIAN_POINT('Ctrl Pts',(1.68077316909132,6.80930564038414,18.1966709743047));
#156689=CARTESIAN_POINT('Ctrl Pts',(1.50061491265684,6.8487795589004,18.2050148786604));
#156690=CARTESIAN_POINT('Ctrl Pts',(1.32060136045763,6.88822177171909,18.2133520811402));
#156691=CARTESIAN_POINT('Ctrl Pts',(1.13893016972089,6.92058479704801,18.2216892836199));
#156692=CARTESIAN_POINT('Ctrl Pts',(0.95618338206577,6.94574257386216,18.2300264860996));
#156693=CARTESIAN_POINT('Ctrl Pts',(0.896024148307747,6.95402437512178,
18.2327710471356));
#156694=CARTESIAN_POINT('Ctrl Pts',(0.835748452853124,6.96152575851747,
18.2355156081717));
#156695=CARTESIAN_POINT('Ctrl Pts',(0.775377323396824,6.96824343495992,
18.2382601692078));
#156696=CARTESIAN_POINT('Ctrl Pts',(0.591962487993929,6.98865255319371,
18.2465984795097));
#156697=CARTESIAN_POINT('Ctrl Pts',(0.407816762156593,7.00180733844378,
18.2549367898116));
#156698=CARTESIAN_POINT('Ctrl Pts',(0.223536000565575,7.00768565354862,
18.2632751001135));
#156699=CARTESIAN_POINT('Ctrl Pts',(0.0391392957724966,7.01356766708986,
18.2716186565973));
#156700=CARTESIAN_POINT('Ctrl Pts',(-0.145392286753549,7.01216406843363,
18.2799622130811));
#156701=CARTESIAN_POINT('Ctrl Pts',(-0.329463727106422,7.00350485221658,
18.2883057695649));
#156702=CARTESIAN_POINT('Ctrl Pts',(-0.513675208208637,6.99483904810558,
18.2966556737901));
#156703=CARTESIAN_POINT('Ctrl Pts',(-0.697425521935273,6.97890663113029,
18.3050055780153));
#156704=CARTESIAN_POINT('Ctrl Pts',(-0.880125155554621,6.95578940689408,
18.3133554822406));
#156705=CARTESIAN_POINT('Ctrl Pts',(-1.0630988251048,6.93263750853218,18.3217179107042));
#156706=CARTESIAN_POINT('Ctrl Pts',(-1.24501833997801,6.90227930888075,
18.3300803391679));
#156707=CARTESIAN_POINT('Ctrl Pts',(-1.4253032655709,6.86484793448864,18.3384427676315));
#156708=CARTESIAN_POINT('Ctrl Pts',(-1.60574235935173,6.82738455116875,
18.3468123471115));
#156709=CARTESIAN_POINT('Ctrl Pts',(-1.78454375771095,6.78283600375344,
18.3551819265915));
#156710=CARTESIAN_POINT('Ctrl Pts',(-1.96114201224715,6.73138533812314,
18.3635515060714));
#156711=CARTESIAN_POINT('Ctrl Pts',(-2.13801264807444,6.6798553161098,18.371933994608));
#156712=CARTESIAN_POINT('Ctrl Pts',(-2.31267303959052,6.62140200642896,
18.3803164831446));
#156713=CARTESIAN_POINT('Ctrl Pts',(-2.48457621511136,6.55625713298395,
18.3886989716812));
#156714=CARTESIAN_POINT('Ctrl Pts',(-2.54082575094134,6.53494066293107,
18.3914418592855));
#156715=CARTESIAN_POINT('Ctrl Pts',(-2.59678025700478,6.51290809479449,
18.3941847468898));
#156716=CARTESIAN_POINT('Ctrl Pts',(-2.6524211410294,6.49016861515325,18.3969276344942));
#156717=CARTESIAN_POINT('Ctrl Pts',(-2.82261366211137,6.42061383657494,
18.405317489627));
#156718=CARTESIAN_POINT('Ctrl Pts',(-2.99021376345989,6.34430126921102,
18.4137073447597));
#156719=CARTESIAN_POINT('Ctrl Pts',(-3.15466815543368,6.26144515200706,
18.4220971998925));
#156720=CARTESIAN_POINT('Ctrl Pts',(-3.31897079120009,6.17866549326646,
18.4304793129846));
#156721=CARTESIAN_POINT('Ctrl Pts',(-3.48013321219892,6.08935446921592,
18.4388614260767));
#156722=CARTESIAN_POINT('Ctrl Pts',(-3.63762249876473,5.99377419652932,
18.4472435391688));
#156723=CARTESIAN_POINT('Ctrl Pts',(-3.79498960702314,5.89826807387661,
18.4556191495177));
#156724=CARTESIAN_POINT('Ctrl Pts',(-3.94868898201726,5.79650256908108,
18.4639947598666));
#156725=CARTESIAN_POINT('Ctrl Pts',(-4.09821229259012,5.68878568478047,
18.4723703702154));
#156726=CARTESIAN_POINT('Ctrl Pts',(-4.24764155078007,5.58113655599978,
18.480740712181));
#156727=CARTESIAN_POINT('Ctrl Pts',(-4.39289971613055,5.46754370358145,
18.4891110541466));
#156728=CARTESIAN_POINT('Ctrl Pts',(-4.53350706626756,5.34835864939909,
18.4974813961122));
#156729=CARTESIAN_POINT('Ctrl Pts',(-4.67404658375184,5.22923109319521,
18.5058477000065));
#156730=CARTESIAN_POINT('Ctrl Pts',(-4.80993950996139,5.10451692730062,
18.5142140039008));
#156731=CARTESIAN_POINT('Ctrl Pts',(-4.94073852006542,4.97460847090922,
18.5225803077952));
#156732=CARTESIAN_POINT('Ctrl Pts',(-5.07150094935249,4.84473634627187,
18.5309442718688));
#156733=CARTESIAN_POINT('Ctrl Pts',(-5.19717206921861,4.70967305816532,
18.5393082359424));
#156734=CARTESIAN_POINT('Ctrl Pts',(-5.31734040985135,4.56984874238326,
18.547672200016));
#156735=CARTESIAN_POINT('Ctrl Pts',(-5.43749025857343,4.43004594323979,
18.5560348770146));
#156736=CARTESIAN_POINT('Ctrl Pts',(-5.55213880223159,4.28548382634671,
18.5643975540131));
#156737=CARTESIAN_POINT('Ctrl Pts',(-5.66091369828726,4.13662696687092,
18.5727602310116));
#156738=CARTESIAN_POINT('Ctrl Pts',(-5.76968635486656,3.98777317208588,
18.581122735838));
#156739=CARTESIAN_POINT('Ctrl Pts',(-5.87258541139571,3.83462507661903,
18.5894852406643));
#156740=CARTESIAN_POINT('Ctrl Pts',(-5.96928059209804,3.67767804127845,
18.5978477454906));
#156741=CARTESIAN_POINT('Ctrl Pts',(-6.06598667080267,3.52071331726776,
18.6062111928106));
#156742=CARTESIAN_POINT('Ctrl Pts',(-6.15648730773891,3.35994907983606,
18.6145746401305));
#156743=CARTESIAN_POINT('Ctrl Pts',(-6.24049688580979,3.19590756760867,
18.6229380874505));
#156744=CARTESIAN_POINT('Ctrl Pts',(-6.32455593108116,3.0317694631288,18.6313064594033));
#156745=CARTESIAN_POINT('Ctrl Pts',(-6.40211612916342,2.86435052014575,
18.6396748313561));
#156746=CARTESIAN_POINT('Ctrl Pts',(-6.47293850667817,2.69419629041075,
18.6480432033089));
#156747=CARTESIAN_POINT('Ctrl Pts',(-6.54378210442819,2.52399107802149,
18.6564140826447));
#156748=CARTESIAN_POINT('Ctrl Pts',(-6.60788373468658,2.35104925020757,
18.6647849619805));
#156749=CARTESIAN_POINT('Ctrl Pts',(-6.66505324983363,2.1759346817821,18.6731558413162));
#156750=CARTESIAN_POINT('Ctrl Pts',(-6.72227120409265,2.00067174067645,
18.6815338132075));
#156751=CARTESIAN_POINT('Ctrl Pts',(-6.77254520996378,1.82323269477702,
18.6899117850988));
#156752=CARTESIAN_POINT('Ctrl Pts',(-6.81573518619107,1.6441959841263,18.6982897569901));
#156753=CARTESIAN_POINT('Ctrl Pts',(-6.84318276778077,1.5304166966065,18.7036140263491));
#156754=CARTESIAN_POINT('Ctrl Pts',(-6.86777033888593,1.41599240804873,
18.7089382957081));
#156755=CARTESIAN_POINT('Ctrl Pts',(-6.88947272927076,1.30107343187635,
18.7142625650671));
#156756=CARTESIAN_POINT('Ctrl Pts',(-6.92152261639967,1.13136216274959,
18.7221253962563));
#156757=CARTESIAN_POINT('Ctrl Pts',(-6.94734408917821,0.960218692717945,
18.7299882274456));
#156758=CARTESIAN_POINT('Ctrl Pts',(-6.96680925618418,0.788159470187608,
18.7378510586349));
#156759=CARTESIAN_POINT('Ctrl Pts',(-6.98625946677869,0.616232452458246,
18.7457078482763));
#156760=CARTESIAN_POINT('Ctrl Pts',(-6.99936304151817,0.443391457915472,
18.7535646379176));
#156761=CARTESIAN_POINT('Ctrl Pts',(-7.00604296529355,0.270163896479033,
18.761421427559));
#156762=CARTESIAN_POINT('Ctrl Pts',(-7.01271912190814,0.0970340271870361,
18.769273786343));
#156763=CARTESIAN_POINT('Ctrl Pts',(-7.01297881916429,-0.0764815955348706,
18.7771261451269));
#156764=CARTESIAN_POINT('Ctrl Pts',(-7.00679681341432,-0.249849911000555,
18.7849785039109));
#156765=CARTESIAN_POINT('Ctrl Pts',(-7.00061626730803,-0.423177292184107,
18.7928290086613));
#156766=CARTESIAN_POINT('Ctrl Pts',(-6.98799705047312,-0.596357054351083,
18.8006795134117));
#156767=CARTESIAN_POINT('Ctrl Pts',(-6.96896602986745,-0.768855667244176,
18.8085300181621));
#156768=CARTESIAN_POINT('Ctrl Pts',(-6.9499380707532,-0.941326530547105,
18.8163792600137));
#156769=CARTESIAN_POINT('Ctrl Pts',(-6.92450040602444,-1.11311608381016,
18.8242285018654));
#156770=CARTESIAN_POINT('Ctrl Pts',(-6.89273177670675,-1.28369592072148,
18.832077743717));
#156771=CARTESIAN_POINT('Ctrl Pts',(-6.86095244391603,-1.45433322931873,
18.8399296301318));
#156772=CARTESIAN_POINT('Ctrl Pts',(-6.82283795586274,-1.62375963204604,
18.8477815165467));
#156773=CARTESIAN_POINT('Ctrl Pts',(-6.77851822867546,-1.79145672178104,
18.8556334029615));
#156774=CARTESIAN_POINT('Ctrl Pts',(-6.74597480463827,-1.91459460749023,
18.8613989454255));
#156775=CARTESIAN_POINT('Ctrl Pts',(-6.71008672265903,-2.03680028130827,
18.8671644878895));
#156776=CARTESIAN_POINT('Ctrl Pts',(-6.67092249617087,-2.15787386391823,
18.8729300303535));
#156777=CARTESIAN_POINT('Ctrl Pts',(-6.60533586158689,-2.36063055114182,
18.8825853347134));
#156778=CARTESIAN_POINT('Ctrl Pts',(-6.53059419910574,-2.56010866816895,
18.8922406390733));
#156779=CARTESIAN_POINT('Ctrl Pts',(-6.44704521748711,-2.75558242957394,
18.9018959434332));
#156780=CARTESIAN_POINT('Ctrl Pts',(-6.36303339018411,-2.9521390789462,
18.9116047363679));
#156781=CARTESIAN_POINT('Ctrl Pts',(-6.27011646051596,-3.14464686117081,
18.9213135293026));
#156782=CARTESIAN_POINT('Ctrl Pts',(-6.16869094440121,-3.33239832477489,
18.9310223222373));
#156783=CARTESIAN_POINT('Ctrl Pts',(-6.06677736009053,-3.52105326436446,
18.9407778347081));
#156784=CARTESIAN_POINT('Ctrl Pts',(-5.9562731459008,-3.70490597291602,
18.9505333471788));
#156785=CARTESIAN_POINT('Ctrl Pts',(-5.83762301889833,-3.88326976293539,
18.9602888596495));
#156786=CARTESIAN_POINT('Ctrl Pts',(-5.71885541001622,-4.06181016054755,
18.9700540315785));
#156787=CARTESIAN_POINT('Ctrl Pts',(-5.59192578560676,-4.23485074290651,
18.9798192035074));
#156788=CARTESIAN_POINT('Ctrl Pts',(-5.45732198896148,-4.40173412092297,
18.9895843754363));
#156789=CARTESIAN_POINT('Ctrl Pts',(-5.32290172153903,-4.56838995723977,
18.9993362327749));
#156790=CARTESIAN_POINT('Ctrl Pts',(-5.18082821863161,-4.72890533870851,
19.0090880901134));
#156791=CARTESIAN_POINT('Ctrl Pts',(-5.03162852566511,-4.88265716001167,
19.018839947452));
#156792=CARTESIAN_POINT('Ctrl Pts',(-4.96656665397724,-4.94970408933509,
19.0230924635146));
#156793=CARTESIAN_POINT('Ctrl Pts',(-4.90015019910339,-5.01546527431112,
19.0273449795773));
#156794=CARTESIAN_POINT('Ctrl Pts',(-4.83242531288399,-5.07989095925277,
19.0315974956399));
#156795=CARTESIAN_POINT('Ctrl Pts',(-4.7044923218822,-5.20159172586942,
19.0396305412387));
#156796=CARTESIAN_POINT('Ctrl Pts',(-4.57182535042705,-5.31858360796435,
19.0476635868376));
#156797=CARTESIAN_POINT('Ctrl Pts',(-4.43481306853779,-5.43047508139265,
19.0556966324364));
#156798=CARTESIAN_POINT('Ctrl Pts',(-4.2978888634189,-5.54229462667351,
19.0637245140842));
#156799=CARTESIAN_POINT('Ctrl Pts',(-4.15662519080014,-5.64902005879922,
19.071752395732));
#156800=CARTESIAN_POINT('Ctrl Pts',(-4.01144643542351,-5.7502977364853,
19.0797802773798));
#156801=CARTESIAN_POINT('Ctrl Pts',(-3.86633322968604,-5.85152968630157,
19.0878045343599));
#156802=CARTESIAN_POINT('Ctrl Pts',(-3.71730876090025,-5.9473185699575,
19.09582879134));
#156803=CARTESIAN_POINT('Ctrl Pts',(-3.56482920864944,-6.03735200859283,
19.1038530483201));
#156804=CARTESIAN_POINT('Ctrl Pts',(-3.41236809272944,-6.12737456126846,
19.1118763350858));
#156805=CARTESIAN_POINT('Ctrl Pts',(-3.25645303698763,-6.21164286211121,
19.1198996218516));
#156806=CARTESIAN_POINT('Ctrl Pts',(-3.09756797472278,-6.28988864801849,
19.1279229086173));
#156807=CARTESIAN_POINT('Ctrl Pts',(-2.9386959316716,-6.36812802238152,
19.1359455379462));
#156808=CARTESIAN_POINT('Ctrl Pts',(-2.7768546975555,-6.44034570641755,
19.1439681672751));
#156809=CARTESIAN_POINT('Ctrl Pts',(-2.612551222509,-6.50632020978577,19.1519907966041));
#156810=CARTESIAN_POINT('Ctrl Pts',(-2.44818598105295,-6.57231951487041,
19.1600164418705));
#156811=CARTESIAN_POINT('Ctrl Pts',(-2.28135699108969,-6.63207081688275,
19.1680420871369));
#156812=CARTESIAN_POINT('Ctrl Pts',(-2.11258987980619,-6.68540130151066,
19.1760677324033));
#156813=CARTESIAN_POINT('Ctrl Pts',(-2.0130745068347,-6.71684820504616,
19.180800141911));
#156814=CARTESIAN_POINT('Ctrl Pts',(-1.91288556626571,-6.74606352631963,
19.1855325514187));
#156815=CARTESIAN_POINT('Ctrl Pts',(-1.81213302469172,-6.77302004007973,
19.1902649609264));
#156816=CARTESIAN_POINT('Ctrl Pts',(-1.62627112776042,-6.82274770653694,
19.198995009761));
#156817=CARTESIAN_POINT('Ctrl Pts',(-1.4383977557771,-6.86481090540057,
19.2077250585957));
#156818=CARTESIAN_POINT('Ctrl Pts',(-1.24914618179546,-6.89907677729461,
19.2164551074303));
#156819=CARTESIAN_POINT('Ctrl Pts',(-1.05983988548541,-6.93335255720821,
19.2251876805695));
#156820=CARTESIAN_POINT('Ctrl Pts',(-0.869154861291281,-6.95982646102874,
19.2339202537086));
#156821=CARTESIAN_POINT('Ctrl Pts',(-0.677732899052425,-6.97841706119963,
19.2426528268477));
#156822=CARTESIAN_POINT('Ctrl Pts',(-0.483591482272319,-6.99727177052219,
19.2515094601281));
#156823=CARTESIAN_POINT('Ctrl Pts',(-0.288692317585981,-7.00801745122277,
19.2603660934086));
#156824=CARTESIAN_POINT('Ctrl Pts',(-0.0937089961231848,-7.01062373733933,
19.269222726689));
#156825=CARTESIAN_POINT('Ctrl Pts',(0.0986654612588957,-7.01319515151821,
19.2779608587957));
#156826=CARTESIAN_POINT('Ctrl Pts',(0.29112155933783,-7.00784364703544,
19.2866989909025));
#156827=CARTESIAN_POINT('Ctrl Pts',(0.483012649013248,-6.99459257879923,
19.2954371230092));
#156828=CARTESIAN_POINT('Ctrl Pts',(0.678807202106398,-6.981071956306,19.3043530068765));
#156829=CARTESIAN_POINT('Ctrl Pts',(0.874013217916381,-6.95932695708988,
19.3132688907437));
#156830=CARTESIAN_POINT('Ctrl Pts',(1.06794850413261,-6.92943811250385,
19.322184774611));
#156831=CARTESIAN_POINT('Ctrl Pts',(1.26188379034882,-6.89954926791782,
19.3311006584782));
#156832=CARTESIAN_POINT('Ctrl Pts',(1.45454804901438,-6.86151663003711,
19.3400165423455));
#156833=CARTESIAN_POINT('Ctrl Pts',(1.64526833286464,-6.81547640854055,
19.3489324262128));
#156834=CARTESIAN_POINT('Ctrl Pts',(1.83224091494251,-6.7703408890307,19.357673110709));
#156835=CARTESIAN_POINT('Ctrl Pts',(2.01736507059274,-6.71750477296969,
19.3664137952052));
#156836=CARTESIAN_POINT('Ctrl Pts',(2.20001788584635,-6.65714262010783,
19.3751544797015));
#156837=CARTESIAN_POINT('Ctrl Pts',(2.38263783882449,-6.59679132739994,
19.3838935916034));
#156838=CARTESIAN_POINT('Ctrl Pts',(2.56278707950309,-6.52891678793202,
19.3926327035053));
#156839=CARTESIAN_POINT('Ctrl Pts',(2.73985880538999,-6.4537431223304,19.4013718154072));
#156840=CARTESIAN_POINT('Ctrl Pts',(2.91922475033559,-6.37759547369749,
19.4102241550815));
#156841=CARTESIAN_POINT('Ctrl Pts',(3.09543260616893,-6.29395832974499,
19.4190764947559));
#156842=CARTESIAN_POINT('Ctrl Pts',(3.26787224701603,-6.20311514802703,
19.4279288344302));
#156843=CARTESIAN_POINT('Ctrl Pts',(3.43801900736069,-6.11347988207089,
19.43666346708));
#156844=CARTESIAN_POINT('Ctrl Pts',(3.60449689805667,-6.01682916475391,
19.4453980997297));
#156845=CARTESIAN_POINT('Ctrl Pts',(3.76674336336508,-5.91348213805074,
19.4541327323795));
#156846=CARTESIAN_POINT('Ctrl Pts',(3.93226945406403,-5.80804607025709,
19.4630439255661));
#156847=CARTESIAN_POINT('Ctrl Pts',(4.09339097410259,-5.69564023118293,
19.4719551187527));
#156848=CARTESIAN_POINT('Ctrl Pts',(4.24953957758213,-5.57665131965978,
19.4808663119394));
#156849=CARTESIAN_POINT('Ctrl Pts',(4.40568818106166,-5.45766240813662,
19.489777505126));
#156850=CARTESIAN_POINT('Ctrl Pts',(4.5568636187103,-5.3320905971753,19.4986886983126));
#156851=CARTESIAN_POINT('Ctrl Pts',(4.70253066184799,-5.20036844241632,
19.5075998914992));
#156852=CARTESIAN_POINT('Ctrl Pts',(4.83372239383925,-5.08173585914821,
19.5156255563516));
#156853=CARTESIAN_POINT('Ctrl Pts',(4.96050604576484,-4.95805964397839,
19.523651221204));
#156854=CARTESIAN_POINT('Ctrl Pts',(5.08247188667733,-4.8297107660433,19.5316768860564));
#156855=CARTESIAN_POINT('Ctrl Pts',(5.20439901862358,-4.70140262289384,
19.5397000037596));
#156856=CARTESIAN_POINT('Ctrl Pts',(5.32151113154929,-4.56842503488184,
19.5477231214628));
#156857=CARTESIAN_POINT('Ctrl Pts',(5.43343499138747,-4.43118615687338,
19.555746239166));
#156858=CARTESIAN_POINT('Ctrl Pts',(5.54534473664729,-4.29396458588865,
19.5637683450839));
#156859=CARTESIAN_POINT('Ctrl Pts',(5.65206730092608,-4.15248307968907,
19.5717904510017));
#156860=CARTESIAN_POINT('Ctrl Pts',(5.75326946417137,-4.00718317963296,
19.5798125569196));
#156861=CARTESIAN_POINT('Ctrl Pts',(5.85450923448243,-3.8618292856431,19.5878376438791));
#156862=CARTESIAN_POINT('Ctrl Pts',(5.95022429354549,-3.7126544625929,19.5958627308386));
#156863=CARTESIAN_POINT('Ctrl Pts',(6.04012428632136,-3.56012993699541,
19.6038878177981));
#156864=CARTESIAN_POINT('Ctrl Pts',(6.13004198445088,-3.40757537245594,
19.6119144852583));
#156865=CARTESIAN_POINT('Ctrl Pts',(6.21414215622814,-3.25167011138713,
19.6199411527186));
#156866=CARTESIAN_POINT('Ctrl Pts',(6.29218034226967,-3.09291013494656,
19.6279678201788));
#156867=CARTESIAN_POINT('Ctrl Pts',(6.37028117709203,-2.93402270655622,
19.6360009314194));
#156868=CARTESIAN_POINT('Ctrl Pts',(6.44231015314334,-2.7722763185954,19.64403404266));
#156869=CARTESIAN_POINT('Ctrl Pts',(6.50807065985338,-2.60818765598941,
19.6520671539006));
#156870=CARTESIAN_POINT('Ctrl Pts',(6.54681913928817,-2.51150065513488,
19.6568005548623));
#156871=CARTESIAN_POINT('Ctrl Pts',(6.58339213644724,-2.41400076142861,
19.6615339558239));
#156872=CARTESIAN_POINT('Ctrl Pts',(6.61775754767034,-2.31579610560866,
19.6662673567856));
#156873=CARTESIAN_POINT('Ctrl Pts',(6.69106165164929,-2.10631791095802,
19.6763640704265));
#156874=CARTESIAN_POINT('Ctrl Pts',(6.75435454450432,-1.89353185208178,
19.6864607840674));
#156875=CARTESIAN_POINT('Ctrl Pts',(6.80741833042345,-1.67829742212602,
19.6965574977082));
#156876=CARTESIAN_POINT('Ctrl Pts',(6.86056137941349,-1.46274148963157,
19.7066692931326));
#156877=CARTESIAN_POINT('Ctrl Pts',(6.90344478032577,-1.24472979701641,
19.7167810885569));
#156878=CARTESIAN_POINT('Ctrl Pts',(6.93590123433321,-1.02513444487785,
19.7268928839812));
#156879=CARTESIAN_POINT('Ctrl Pts',(6.96825526148265,-0.806232097031962,
19.7369727683584));
#156880=CARTESIAN_POINT('Ctrl Pts',(6.99024806641376,-0.585755995177965,
19.7470526527356));
#156881=CARTESIAN_POINT('Ctrl Pts',(7.00176464560906,-0.364579771790776,
19.7571325371128));
#156882=CARTESIAN_POINT('Ctrl Pts',(7.0080111741597,-0.244615017441415,
19.7625998103787));
#156883=CARTESIAN_POINT('Ctrl Pts',(7.01117655918058,-0.124444468868163,
19.7680670836446));
#156884=CARTESIAN_POINT('Ctrl Pts',(7.01124873670978,-0.00420885798051574,
19.7735343569105));
#156885=CARTESIAN_POINT('Ctrl Pts',(7.01125,3.89288422118862E-12,19.7735343569105));
#156886=CARTESIAN_POINT('Ctrl Pts',(7.0112499999999,0.191008754744022,19.7822061308426));
#156887=CARTESIAN_POINT('Ctrl Pts',(7.00344012880997,0.382017367486818,
19.7908779047747));
#156888=CARTESIAN_POINT('Ctrl Pts',(6.98784644419149,0.57238853491349,19.7995496787068));
#156889=CARTESIAN_POINT('Ctrl Pts',(6.97225169663166,0.762772678964259,
19.8082220437492));
#156890=CARTESIAN_POINT('Ctrl Pts',(6.94887209704278,0.952519007630679,
19.8168944087915));
#156891=CARTESIAN_POINT('Ctrl Pts',(6.91778566246045,1.14099434299941,19.8255667738339));
#156892=CARTESIAN_POINT('Ctrl Pts',(6.8867010829714,1.3294584310401,19.83423862135));
#156893=CARTESIAN_POINT('Ctrl Pts',(6.84791063501108,1.51665139731095,19.8429104688661));
#156894=CARTESIAN_POINT('Ctrl Pts',(6.80154374572935,1.70194865887019,19.8515823163822));
#156895=CARTESIAN_POINT('Ctrl Pts',(6.75517597619855,1.88724943819274,19.8602543285284));
#156896=CARTESIAN_POINT('Ctrl Pts',(6.70123154646081,2.07065416525486,19.8689263406746));
#156897=CARTESIAN_POINT('Ctrl Pts',(6.63989045285517,2.2515508736386,19.8775983528208));
#156898=CARTESIAN_POINT('Ctrl Pts',(6.61790934153631,2.31637382429812,19.8807059019879));
#156899=CARTESIAN_POINT('Ctrl Pts',(6.59497889661509,2.38087486019083,19.8838134511551));
#156900=CARTESIAN_POINT('Ctrl Pts',(6.57110895151814,2.44502632087636,19.8869210003222));
#156901=CARTESIAN_POINT('',(7.01124999765299,-0.000181413711516228,19.2264656431264));
#156902=CARTESIAN_POINT('Ctrl Pts',(6.57110895151814,2.44502632087635,19.3399454697435));
#156903=CARTESIAN_POINT('Ctrl Pts',(6.64355296009685,2.25033006374781,19.3304888175255));
#156904=CARTESIAN_POINT('Ctrl Pts',(6.70735026907554,2.05238418768571,19.3210321653074));
#156905=CARTESIAN_POINT('Ctrl Pts',(6.76225087861329,1.85191512148745,19.3115755130893));
#156906=CARTESIAN_POINT('Ctrl Pts',(6.81648747471622,1.65387069418375,19.3022332374541));
#156907=CARTESIAN_POINT('Ctrl Pts',(6.86204130570839,1.4533639108226,19.292890961819));
#156908=CARTESIAN_POINT('Ctrl Pts',(6.89872045868837,1.251112543049,19.2835486861839));
#156909=CARTESIAN_POINT('Ctrl Pts',(6.93607320068683,1.04514695918164,19.2740348456743));
#156910=CARTESIAN_POINT('Ctrl Pts',(6.96422206952078,0.837372218825123,
19.2645210051647));
#156911=CARTESIAN_POINT('Ctrl Pts',(6.98301765280545,0.628562664423706,
19.2550071646552));
#156912=CARTESIAN_POINT('Ctrl Pts',(7.00181323609013,0.419753110022305,
19.2454933241456));
#156913=CARTESIAN_POINT('Ctrl Pts',(7.01125543366831,0.209908893479341,
19.235979483636));
#156914=CARTESIAN_POINT('Ctrl Pts',(7.01124999765299,-0.000181413711498942,
19.2264656431264));
#156915=CARTESIAN_POINT('Ctrl Pts',(7.01124999765297,-0.000181414524300546,
19.2264656430896));
#156916=CARTESIAN_POINT('Ctrl Pts',(7.01124516495315,-0.186954037711722,
19.2180077329065));
#156917=CARTESIAN_POINT('Ctrl Pts',(7.00377284192131,-0.373681608927717,
19.2095498227235));
#156918=CARTESIAN_POINT('Ctrl Pts',(6.98886978812648,-0.559754988466313,
19.2010919125404));
#156919=CARTESIAN_POINT('Ctrl Pts',(6.97396039576302,-0.745907508757027,
19.192630405038));
#156920=CARTESIAN_POINT('Ctrl Pts',(6.95161399222959,-0.931404968934443,
19.1841688975355));
#156921=CARTESIAN_POINT('Ctrl Pts',(6.92191919458265,-1.11564386170868,
19.1757073900331));
#156922=CARTESIAN_POINT('Ctrl Pts',(6.89220882192622,-1.29997938832901,
19.1672414444449));
#156923=CARTESIAN_POINT('Ctrl Pts',(6.85514241522061,-1.48305472035264,
19.1587754988566));
#156924=CARTESIAN_POINT('Ctrl Pts',(6.81085974217086,-1.66427645989969,
19.1503095532684));
#156925=CARTESIAN_POINT('Ctrl Pts',(6.7665494426539,-1.84561125758218,19.141838326062));
#156926=CARTESIAN_POINT('Ctrl Pts',(6.71501396877955,-2.02508985057409,
19.1333670988557));
#156927=CARTESIAN_POINT('Ctrl Pts',(6.65644314083335,-2.20213334640586,
19.1248958716493));
#156928=CARTESIAN_POINT('Ctrl Pts',(6.59780049088891,-2.37939394037492,
19.11641425667));
#156929=CARTESIAN_POINT('Ctrl Pts',(6.53210534447744,-2.55421317109245,
19.1079326416906));
#156930=CARTESIAN_POINT('Ctrl Pts',(6.45959646528243,-2.72603009304937,
19.0994510267112));
#156931=CARTESIAN_POINT('Ctrl Pts',(6.38703844263391,-2.89796346525362,
19.0909636632517));
#156932=CARTESIAN_POINT('Ctrl Pts',(6.30765760169667,-3.06689018248215,
19.0824762997922));
#156933=CARTESIAN_POINT('Ctrl Pts',(6.22173939182166,-3.23227249822082,
19.0739889363327));
#156934=CARTESIAN_POINT('Ctrl Pts',(6.13571527480889,-3.39785867257946,
19.0654911109191));
#156935=CARTESIAN_POINT('Ctrl Pts',(6.04313783782619,-3.55989144004833,
19.0569932855055));
#156936=CARTESIAN_POINT('Ctrl Pts',(5.94433741785836,-3.71785949507899,
19.0484954600919));
#156937=CARTESIAN_POINT('Ctrl Pts',(5.91178451919106,-3.76990702776921,
19.0456955848517));
#156938=CARTESIAN_POINT('Ctrl Pts',(5.87855640756592,-3.82151354934236,
19.0428957096116));
#156939=CARTESIAN_POINT('Ctrl Pts',(5.84466588621277,-3.87266151903838,
19.0400958343715));
#156940=CARTESIAN_POINT('Ctrl Pts',(5.74321613721404,-4.02577066225237,
19.0317145339666));
#156941=CARTESIAN_POINT('Ctrl Pts',(5.63562818842459,-4.17506946424774,
19.0233332335617));
#156942=CARTESIAN_POINT('Ctrl Pts',(5.52220866352554,-4.32005069865893,
19.0149519331568));
#156943=CARTESIAN_POINT('Ctrl Pts',(5.40893288127082,-4.46484819057929,
19.0065812548233));
#156944=CARTESIAN_POINT('Ctrl Pts',(5.28984045199139,-4.60533876384062,
18.9982105764897));
#156945=CARTESIAN_POINT('Ctrl Pts',(5.16528175072161,-4.74104323943183,
18.9898398981561));
#156946=CARTESIAN_POINT('Ctrl Pts',(5.04086440219207,-4.8765937137426,18.9814787191053));
#156947=CARTESIAN_POINT('Ctrl Pts',(4.91099336570416,-5.00736867584189,
18.9731175400545));
#156948=CARTESIAN_POINT('Ctrl Pts',(4.77606010814833,-5.13292084546939,
18.9647563610037));
#156949=CARTESIAN_POINT('Ctrl Pts',(4.64130194241101,-5.25831009634657,
18.9564060315689));
#156950=CARTESIAN_POINT('Ctrl Pts',(4.50149489657163,-5.37848985043261,
18.9480557021342));
#156951=CARTESIAN_POINT('Ctrl Pts',(4.35706814120457,-5.49304867768347,
18.9397053726995));
#156952=CARTESIAN_POINT('Ctrl Pts',(4.21275251358652,-5.60751935876939,
18.9313614683438));
#156953=CARTESIAN_POINT('Ctrl Pts',(4.06382451570365,-5.7163775291412,18.9230175639881));
#156954=CARTESIAN_POINT('Ctrl Pts',(3.91074819082601,-5.81925039420466,
18.9146736596324));
#156955=CARTESIAN_POINT('Ctrl Pts',(3.75779481780703,-5.92204063114144,
18.9063364571527));
#156956=CARTESIAN_POINT('Ctrl Pts',(3.60070003407538,-6.01885496828442,
18.8979992546729));
#156957=CARTESIAN_POINT('Ctrl Pts',(3.43995892618802,-6.10936241752275,
18.8896620521932));
#156958=CARTESIAN_POINT('Ctrl Pts',(3.38704384074103,-6.13915697022293,
18.8869174911572));
#156959=CARTESIAN_POINT('Ctrl Pts',(3.33373384921236,-6.16826839441706,
18.8841729301211));
#156960=CARTESIAN_POINT('Ctrl Pts',(3.28004730242159,-6.1966859091273,18.881428369085));
#156961=CARTESIAN_POINT('Ctrl Pts',(3.11694104233256,-6.28302177579195,
18.8730900587831));
#156962=CARTESIAN_POINT('Ctrl Pts',(2.95049105754875,-6.36287851805344,
18.8647517484812));
#156963=CARTESIAN_POINT('Ctrl Pts',(2.78124344501673,-6.43601673879516,
18.8564134381793));
#156964=CARTESIAN_POINT('Ctrl Pts',(2.61188934762992,-6.5092009756236,18.8480698816955));
#156965=CARTESIAN_POINT('Ctrl Pts',(2.4397344123806,-6.57565812955061,18.8397263252117));
#156966=CARTESIAN_POINT('Ctrl Pts',(2.26534310331881,-6.63519759967598,
18.8313827687279));
#156967=CARTESIAN_POINT('Ctrl Pts',(2.0908191181094,-6.69478236717065,18.8230328645027));
#156968=CARTESIAN_POINT('Ctrl Pts',(1.91405567502942,-6.7474388472641,18.8146829602774));
#156969=CARTESIAN_POINT('Ctrl Pts',(1.73563114144997,-6.79302665262908,
18.8063330560522));
#156970=CARTESIAN_POINT('Ctrl Pts',(1.55693898427338,-6.83868283632866,
18.7979706275886));
#156971=CARTESIAN_POINT('Ctrl Pts',(1.37658107549933,-6.87724907701198,
18.7896081991249));
#156972=CARTESIAN_POINT('Ctrl Pts',(1.1951461844033,-6.90863605644459,18.7812457706613));
#156973=CARTESIAN_POINT('Ctrl Pts',(1.01355614174206,-6.94004987602331,
18.7728761911813));
#156974=CARTESIAN_POINT('Ctrl Pts',(0.830887603227299,-6.96427214199749,
18.7645066117013));
#156975=CARTESIAN_POINT('Ctrl Pts',(0.647733730032479,-6.98126547106456,
18.7561370322213));
#156976=CARTESIAN_POINT('Ctrl Pts',(0.464297364303625,-6.99828501027126,
18.7477545436848));
#156977=CARTESIAN_POINT('Ctrl Pts',(0.280374494584013,-7.00805331469282,
18.7393720551482));
#156978=CARTESIAN_POINT('Ctrl Pts',(0.0965589714634512,-7.01058506314059,
18.7309895666116));
#156979=CARTESIAN_POINT('Ctrl Pts',(0.0364115203036668,-7.01141349271784,
18.7282466790073));
#156980=CARTESIAN_POINT('Ctrl Pts',(-0.0237244746506637,-7.01146751427345,
18.725503791403));
#156981=CARTESIAN_POINT('Ctrl Pts',(-0.0838283466072417,-7.01074884522368,
18.7227609037986));
#156982=CARTESIAN_POINT('Ctrl Pts',(-0.267672109595982,-7.00855060377677,
18.7143710486658));
#156983=CARTESIAN_POINT('Ctrl Pts',(-0.451586127756862,-6.99911472365721,
18.7059811935331));
#156984=CARTESIAN_POINT('Ctrl Pts',(-0.634977094670883,-6.98243730023717,
18.6975913384003));
#156985=CARTESIAN_POINT('Ctrl Pts',(-0.818198830971593,-6.96577526650966,
18.6892092253082));
#156986=CARTESIAN_POINT('Ctrl Pts',(-1.00089815242133,-6.94188504045475,
18.6808271122161));
#156987=CARTESIAN_POINT('Ctrl Pts',(-1.1824831180529,-6.91081473040769,
18.672444999124));
#156988=CARTESIAN_POINT('Ctrl Pts',(-1.36392721223693,-6.87976852433607,
18.6640693887751));
#156989=CARTESIAN_POINT('Ctrl Pts',(-1.54425835130521,-6.84155339484332,
18.6556937784263));
#156990=CARTESIAN_POINT('Ctrl Pts',(-1.72289061495748,-6.79626915972223,
18.6473181680774));
#156991=CARTESIAN_POINT('Ctrl Pts',(-1.90141051626331,-6.75101340905747,
18.6389478261118));
#156992=CARTESIAN_POINT('Ctrl Pts',(-2.07823335505521,-6.69869749940158,
18.6305774841462));
#156993=CARTESIAN_POINT('Ctrl Pts',(-2.25278384019998,-6.6394722329289,
18.6222071421806));
#156994=CARTESIAN_POINT('Ctrl Pts',(-2.42725011763826,-6.58027553826942,
18.6138408382863));
#156995=CARTESIAN_POINT('Ctrl Pts',(-2.59944591677695,-6.51417623927522,
18.605474534392));
#156996=CARTESIAN_POINT('Ctrl Pts',(-2.76881109924021,-6.44137498203794,
18.5971082304977));
#156997=CARTESIAN_POINT('Ctrl Pts',(-2.93812891500913,-6.36859408527174,
18.5887442664241));
#156998=CARTESIAN_POINT('Ctrl Pts',(-3.10461739038423,-6.28911509603682,
18.5803803023504));
#156999=CARTESIAN_POINT('Ctrl Pts',(-3.26773585023415,-6.20318700150129,
18.5720163382768));
#157000=CARTESIAN_POINT('Ctrl Pts',(-3.43082920886382,-6.11727212987154,
18.5636536612783));
#157001=CARTESIAN_POINT('Ctrl Pts',(-3.59055329523702,-6.0249102847418,
18.5552909842797));
#157002=CARTESIAN_POINT('Ctrl Pts',(-3.74639118127719,-5.92639685469582,
18.5469283072812));
#157003=CARTESIAN_POINT('Ctrl Pts',(-3.90222585890007,-5.82788545286134,
18.5385658024549));
#157004=CARTESIAN_POINT('Ctrl Pts',(-4.05417421814763,-5.72322289460059,
18.5302032976286));
#157005=CARTESIAN_POINT('Ctrl Pts',(-4.20174715382626,-5.61274865086732,
18.5218407928023));
#157006=CARTESIAN_POINT('Ctrl Pts',(-4.3493367216698,-5.50226195616646,
18.5134773454823));
#157007=CARTESIAN_POINT('Ctrl Pts',(-4.49254962002037,-5.38596246747935,
18.5051138981623));
#157008=CARTESIAN_POINT('Ctrl Pts',(-4.63092841241402,-5.26423105511114,
18.4967504508423));
#157009=CARTESIAN_POINT('Ctrl Pts',(-4.76938868612947,-5.14242796386633,
18.4883820788895));
#157010=CARTESIAN_POINT('Ctrl Pts',(-4.90300891833123,-5.01518677422067,
18.4800137069367));
#157011=CARTESIAN_POINT('Ctrl Pts',(-5.03136649664836,-4.88292716911736,
18.4716453349839));
#157012=CARTESIAN_POINT('Ctrl Pts',(-5.15976253425072,-4.7506279355796,
18.4632744556482));
#157013=CARTESIAN_POINT('Ctrl Pts',(-5.28289254867203,-4.61330752792642,
18.4549035763124));
#157014=CARTESIAN_POINT('Ctrl Pts',(-5.40037261365331,-4.47142060157656,
18.4465326969767));
#157015=CARTESIAN_POINT('Ctrl Pts',(-5.51795221822319,-4.32941345596842,
18.4381547250854));
#157016=CARTESIAN_POINT('Ctrl Pts',(-5.62987210217045,-4.18283231716381,
18.4297767531941));
#157017=CARTESIAN_POINT('Ctrl Pts',(-5.73578955921081,-4.03216377332919,
18.4213987813028));
#157018=CARTESIAN_POINT('Ctrl Pts',(-5.80310096564922,-3.93641268682348,
18.4160745119438));
#157019=CARTESIAN_POINT('Ctrl Pts',(-5.86798902647418,-3.83901142385793,
18.4107502425848));
#157020=CARTESIAN_POINT('Ctrl Pts',(-5.93037513265293,-3.74009055351763,
18.4054259732257));
#157021=CARTESIAN_POINT('Ctrl Pts',(-6.02250635073436,-3.59400513744734,
18.3975631420365));
#157022=CARTESIAN_POINT('Ctrl Pts',(-6.10937021996468,-3.44430041469862,
18.3897003108472));
#157023=CARTESIAN_POINT('Ctrl Pts',(-6.19065813649991,-3.29140978905506,
18.3818374796579));
#157024=CARTESIAN_POINT('Ctrl Pts',(-6.27188359400116,-3.138636639676,18.3739806900165));
#157025=CARTESIAN_POINT('Ctrl Pts',(-6.34754144109055,-2.98268278996627,
18.3661239003752));
#157026=CARTESIAN_POINT('Ctrl Pts',(-6.41736637059914,-2.82401052193565,
18.3582671107338));
#157027=CARTESIAN_POINT('Ctrl Pts',(-6.48715192215287,-2.66542773755293,
18.3504147519498));
#157028=CARTESIAN_POINT('Ctrl Pts',(-6.55111094658311,-2.50412993234406,
18.3425623931659));
#157029=CARTESIAN_POINT('Ctrl Pts',(-6.60902421618967,-2.34060365553814,
18.3347100343819));
#157030=CARTESIAN_POINT('Ctrl Pts',(-6.66692381179754,-2.17711598919423,
18.3268595296315));
#157031=CARTESIAN_POINT('Ctrl Pts',(-6.71878035852998,-2.01140125472944,
18.3190090248811));
#157032=CARTESIAN_POINT('Ctrl Pts',(-6.76442292621642,-1.84396557391339,
18.3111585201307));
#157033=CARTESIAN_POINT('Ctrl Pts',(-6.81005815145225,-1.67655682822124,
18.303309278279));
#157034=CARTESIAN_POINT('Ctrl Pts',(-6.84948129017765,-1.50742805618571,
18.2954600364274));
#157035=CARTESIAN_POINT('Ctrl Pts',(-6.88257154376019,-1.33709966252425,
18.2876107945758));
#157036=CARTESIAN_POINT('Ctrl Pts',(-6.91567294609685,-1.16671388189308,
18.2797589081609));
#157037=CARTESIAN_POINT('Ctrl Pts',(-6.94243712858477,-0.995128047173407,
18.2719070217461));
#157038=CARTESIAN_POINT('Ctrl Pts',(-6.9627945642581,-0.822872054719267,
18.2640551353312));
#157039=CARTESIAN_POINT('Ctrl Pts',(-6.97774277588914,-0.696386623487206,
18.2582895928673));
#157040=CARTESIAN_POINT('Ctrl Pts',(-6.9892376781199,-0.569540069083445,
18.2525240504033));
#157041=CARTESIAN_POINT('Ctrl Pts',(-6.99726959917371,-0.442543465638532,
18.2467585079393));
#157042=CARTESIAN_POINT('Ctrl Pts',(-7.01072030964093,-0.229867751844482,
18.2371032035794));
#157043=CARTESIAN_POINT('Ctrl Pts',(-7.01445165797877,-0.0168796950838728,
18.2274478992195));
#157044=CARTESIAN_POINT('Ctrl Pts',(-7.00852054170013,0.195617941578176,
18.2177925948596));
#157045=CARTESIAN_POINT('Ctrl Pts',(-7.00255656814998,0.409292775283142,
18.2080838019249));
#157046=CARTESIAN_POINT('Ctrl Pts',(-6.98682283297686,0.622471694535516,
18.1983750089902));
#157047=CARTESIAN_POINT('Ctrl Pts',(-6.9614283634964,0.834351066642706,
18.1886662160554));
#157048=CARTESIAN_POINT('Ctrl Pts',(-6.93591169367252,1.04725002027947,
18.1789107035847));
#157049=CARTESIAN_POINT('Ctrl Pts',(-6.90064111826093,1.25883684951397,
18.169155191114));
#157050=CARTESIAN_POINT('Ctrl Pts',(-6.85577812304805,1.46830953481742,
18.1593996786433));
#157051=CARTESIAN_POINT('Ctrl Pts',(-6.81087070656787,1.67798963030607,
18.1496345067144));
#157052=CARTESIAN_POINT('Ctrl Pts',(-6.7563518911328,1.88555135958048,18.1398693347854));
#157053=CARTESIAN_POINT('Ctrl Pts',(-6.69243403459657,2.09020411804049,
18.1301041628565));
#157054=CARTESIAN_POINT('Ctrl Pts',(-6.62860332860761,2.29457783710738,
18.1203523055179));
#157055=CARTESIAN_POINT('Ctrl Pts',(-6.55539920620729,2.49605047639107,
18.1106004481794));
#157056=CARTESIAN_POINT('Ctrl Pts',(-6.47308307807708,2.69384892427399,
18.1008485908409));
#157057=CARTESIAN_POINT('Ctrl Pts',(-6.43718728459529,2.78010337279462,
18.0965960747782));
#157058=CARTESIAN_POINT('Ctrl Pts',(-6.39955940009407,2.865659326623,18.0923435587156));
#157059=CARTESIAN_POINT('Ctrl Pts',(-6.36022408105815,2.95045355856146,
18.0880910426529));
#157060=CARTESIAN_POINT('Ctrl Pts',(-6.28591926790637,3.11063071524814,
18.0800579970541));
#157061=CARTESIAN_POINT('Ctrl Pts',(-6.20548203678741,3.26816635452103,
18.0720249514553));
#157062=CARTESIAN_POINT('Ctrl Pts',(-6.11913013039002,3.42255358027497,
18.0639919058564));
#157063=CARTESIAN_POINT('Ctrl Pts',(-6.03283373432293,3.57684155997572,
18.0559640242086));
#157064=CARTESIAN_POINT('Ctrl Pts',(-5.94063040950607,3.72798483623015,
18.0479361425608));
#157065=CARTESIAN_POINT('Ctrl Pts',(-5.84278502932592,3.87549863418695,
18.039908260913));
#157066=CARTESIAN_POINT('Ctrl Pts',(-5.74498382729946,4.02294582820981,
18.0318840039329));
#157067=CARTESIAN_POINT('Ctrl Pts',(-5.64154584436463,4.1667665020204,18.0238597469528));
#157068=CARTESIAN_POINT('Ctrl Pts',(-5.53278067960693,4.30650258491369,
18.0158354899726));
#157069=CARTESIAN_POINT('Ctrl Pts',(-5.42402866566543,4.44622177229134,
18.0078122032069));
#157070=CARTESIAN_POINT('Ctrl Pts',(-5.30995097180102,4.58185705861636,
17.9997889164412));
#157071=CARTESIAN_POINT('Ctrl Pts',(-5.19089921178639,4.71298121527929,
17.9917656296755));
#157072=CARTESIAN_POINT('Ctrl Pts',(-5.07185720700146,4.84409462748731,
17.9837430003466));
#157073=CARTESIAN_POINT('Ctrl Pts',(-4.94784219736173,4.97069737758333,
17.9757203710176));
#157074=CARTESIAN_POINT('Ctrl Pts',(-4.81924438107422,5.09239728988073,
17.9676977416887));
#157075=CARTESIAN_POINT('Ctrl Pts',(-4.69059822116308,5.21414295268094,
17.9596720964223));
#157076=CARTESIAN_POINT('Ctrl Pts',(-4.55736608149501,5.33098184579355,
17.9516464511559));
#157077=CARTESIAN_POINT('Ctrl Pts',(-4.41997340702905,5.44256021038408,
17.9436208058895));
#157078=CARTESIAN_POINT('Ctrl Pts',(-4.33895831386897,5.50835361339547,
17.9388883963818));
#157079=CARTESIAN_POINT('Ctrl Pts',(-4.25649724147723,5.57231868471863,
17.9341559868741));
#157080=CARTESIAN_POINT('Ctrl Pts',(-4.17268247625739,5.63438971982188,
17.9294235773664));
#157081=CARTESIAN_POINT('Ctrl Pts',(-4.01806631460727,5.74889442758001,
17.9206935285318));
#157082=CARTESIAN_POINT('Ctrl Pts',(-3.85876470267615,5.85700877924149,
17.9119634796971));
#157083=CARTESIAN_POINT('Ctrl Pts',(-3.69531788278139,5.95837665037182,
17.9032334308625));
#157084=CARTESIAN_POINT('Ctrl Pts',(-3.53182380203511,6.05977383214832,
17.8945008577234));
#157085=CARTESIAN_POINT('Ctrl Pts',(-3.36418235367525,6.15442049520198,
17.8857682845842));
#157086=CARTESIAN_POINT('Ctrl Pts',(-3.19296058830537,6.24200522620965,
17.8770357114451));
#157087=CARTESIAN_POINT('Ctrl Pts',(-3.01930634443635,6.33083423813319,
17.8681790781647));
#157088=CARTESIAN_POINT('Ctrl Pts',(-2.84196953804467,6.41239900471752,
17.8593224448842));
#157089=CARTESIAN_POINT('Ctrl Pts',(-2.66156554982998,6.48642392898107,
17.8504658116038));
#157090=CARTESIAN_POINT('Ctrl Pts',(-2.48357535517145,6.55945840460238,
17.8417276794971));
#157091=CARTESIAN_POINT('Ctrl Pts',(-2.30259981210677,6.62515346606341,
17.8329895473904));
#157092=CARTESIAN_POINT('Ctrl Pts',(-2.11924896866557,6.6832933776178,17.8242514152836));
#157093=CARTESIAN_POINT('Ctrl Pts',(-1.93216838815715,6.74261597575895,
17.8153355314164));
#157094=CARTESIAN_POINT('Ctrl Pts',(-1.7426151162702,6.79407266352937,17.8064196475491));
#157095=CARTESIAN_POINT('Ctrl Pts',(-1.55125325708798,6.83748783508051,
17.7975037636818));
#157096=CARTESIAN_POINT('Ctrl Pts',(-1.35989139790574,6.88090300663165,
17.7885878798146));
#157097=CARTESIAN_POINT('Ctrl Pts',(-1.16672124769152,6.91627660098644,
17.7796719959473));
#157098=CARTESIAN_POINT('Ctrl Pts',(-0.972418757270613,6.94348819564117,
17.77075611208));
#157099=CARTESIAN_POINT('Ctrl Pts',(-0.781934359886621,6.97016507558458,
17.7620154275838));
#157100=CARTESIAN_POINT('Ctrl Pts',(-0.590341479410634,6.98900058238697,
17.7532747430876));
#157101=CARTESIAN_POINT('Ctrl Pts',(-0.398283611592436,6.99992833729295,
17.7445340585913));
#157102=CARTESIAN_POINT('Ctrl Pts',(-0.206260298174957,7.01085412611431,
17.7357949466894));
#157103=CARTESIAN_POINT('Ctrl Pts',(-0.0137724377431587,7.01387498880377,
17.7270558347875));
#157104=CARTESIAN_POINT('Ctrl Pts',(0.178533260344289,7.00897656134267,
17.7183167228856));
#157105=CARTESIAN_POINT('Ctrl Pts',(0.373330555525936,7.00401466770375,
17.7094643832113));
#157106=CARTESIAN_POINT('Ctrl Pts',(0.567940649612334,6.99092682656728,
17.700612043537));
#157107=CARTESIAN_POINT('Ctrl Pts',(0.761691952660525,6.96975264494747,
17.6917597038626));
#157108=CARTESIAN_POINT('Ctrl Pts',(0.952867000139486,6.94886001035451,
17.6830250712129));
#157109=CARTESIAN_POINT('Ctrl Pts',(1.14320567516849,6.92009478765978,17.6742904385631));
#157110=CARTESIAN_POINT('Ctrl Pts',(1.33206753067108,6.88354724369869,17.6655558059133));
#157111=CARTESIAN_POINT('Ctrl Pts',(1.52474701101648,6.84626093323869,17.6566446127267));
#157112=CARTESIAN_POINT('Ctrl Pts',(1.71588904234259,6.80087436321998,17.6477334195401));
#157113=CARTESIAN_POINT('Ctrl Pts',(1.90482298407108,6.74753851132801,17.6388222263535));
#157114=CARTESIAN_POINT('Ctrl Pts',(2.09375692579957,6.69420265943603,17.6299110331668));
#157115=CARTESIAN_POINT('Ctrl Pts',(2.28048248254154,6.63291759505816,17.6209998399802));
#157116=CARTESIAN_POINT('Ctrl Pts',(2.46434297795406,6.56388911008623,17.6120886467936));
#157117=CARTESIAN_POINT('Ctrl Pts',(2.62993278000099,6.50172016435128,17.6040629819412));
#157118=CARTESIAN_POINT('Ctrl Pts',(2.79327456229531,6.43324124240267,17.5960373170888));
#157119=CARTESIAN_POINT('Ctrl Pts',(2.95385099394759,6.3586469368927,17.5880116522364));
#157120=CARTESIAN_POINT('Ctrl Pts',(3.11437646257926,6.28407630578556,17.5799885345332));
#157121=CARTESIAN_POINT('Ctrl Pts',(3.2721379958415,6.20339430946547,17.57196541683));
#157122=CARTESIAN_POINT('Ctrl Pts',(3.42663855477327,6.11684353056716,17.5639422991268));
#157123=CARTESIAN_POINT('Ctrl Pts',(3.58111962983246,6.03030366647952,17.5559201932089));
#157124=CARTESIAN_POINT('Ctrl Pts',(3.7323402302707,5.93789667363831,17.547898087291));
#157125=CARTESIAN_POINT('Ctrl Pts',(3.87982827560464,5.83991088239527,17.5398759813732));
#157126=CARTESIAN_POINT('Ctrl Pts',(4.02737112799429,5.74188867930132,17.5318508944136));
#157127=CARTESIAN_POINT('Ctrl Pts',(4.1711783471568,5.63828373694692,17.5238258074541));
#157128=CARTESIAN_POINT('Ctrl Pts',(4.31080682208906,5.52942773758103,17.5158007204946));
#157129=CARTESIAN_POINT('Ctrl Pts',(4.45046279615075,5.42055029957078,17.5077740530344));
#157130=CARTESIAN_POINT('Ctrl Pts',(4.58593810279121,5.30641997663847,17.4997473855741));
#157131=CARTESIAN_POINT('Ctrl Pts',(4.71682322995323,5.18740832978026,17.4917207181139));
#157132=CARTESIAN_POINT('Ctrl Pts',(4.84781343123415,5.06830114079129,17.4836876068733));
#157133=CARTESIAN_POINT('Ctrl Pts',(4.97420582830038,4.9443050546706,17.4756544956327));
#157134=CARTESIAN_POINT('Ctrl Pts',(5.09562781228434,4.81582846052207,17.4676213843921));
#157135=CARTESIAN_POINT('Ctrl Pts',(5.1671740561423,4.74012538408243,17.4628879834305));
#157136=CARTESIAN_POINT('Ctrl Pts',(5.23699531121069,4.6628673376765,17.4581545824688));
#157137=CARTESIAN_POINT('Ctrl Pts',(5.30502200952541,4.5841431086901,17.4534211815071));
#157138=CARTESIAN_POINT('Ctrl Pts',(5.44523849086005,4.42187690060242,17.4436647058287));
#157139=CARTESIAN_POINT('Ctrl Pts',(5.57791171544638,4.25328461661226,17.4339082301503));
#157140=CARTESIAN_POINT('Ctrl Pts',(5.70255807462325,4.07902659565357,17.4241517544719));
#157141=CARTESIAN_POINT('Ctrl Pts',(5.82731200848036,3.90461818321126,17.4143868585736));
#157142=CARTESIAN_POINT('Ctrl Pts',(5.94402521095326,3.72453429354533,17.4046219626753));
#157143=CARTESIAN_POINT('Ctrl Pts',(6.05225705726437,3.53946480068578,17.394857066777));
#157144=CARTESIAN_POINT('Ctrl Pts',(6.16027707130092,3.35475752738507,17.3851112828146));
#157145=CARTESIAN_POINT('Ctrl Pts',(6.25984888294183,3.1650841836814,17.3753654988522));
#157146=CARTESIAN_POINT('Ctrl Pts',(6.35057859735081,2.97115769379038,17.3656197148898));
#157147=CARTESIAN_POINT('Ctrl Pts',(6.43114174761781,2.79896130755009,17.3569659782066));
#157148=CARTESIAN_POINT('Ctrl Pts',(6.50473393484496,2.62341191226827,17.3483122415235));
#157149=CARTESIAN_POINT('Ctrl Pts',(6.57110895151813,2.44502632087639,17.3396585048403));
#157150=CARTESIAN_POINT('Origin',(0.,0.,50.));
#157151=CARTESIAN_POINT('',(6.57110895151814,2.44502632087634,15.3398759450547));
#157152=CARTESIAN_POINT('',(6.57110895151814,2.44502632087636,15.8871325193051));
#157153=CARTESIAN_POINT('',(6.57110895151814,2.44502632087636,50.));
#157154=CARTESIAN_POINT('',(7.01124960457286,0.00235475623571332,17.7735343569365));
#157155=CARTESIAN_POINT('Ctrl Pts',(6.57110895151814,2.44502632087636,15.8871325193051));
#157156=CARTESIAN_POINT('Ctrl Pts',(6.5069897366308,2.61734935204908,15.8955017124837));
#157157=CARTESIAN_POINT('Ctrl Pts',(6.43602216531024,2.78732527730889,15.9038709056622));
#157158=CARTESIAN_POINT('Ctrl Pts',(6.35839584537371,2.9543914493571,15.9122400988407));
#157159=CARTESIAN_POINT('Ctrl Pts',(6.27748822327716,3.12851958945502,15.9209630618705));
#157160=CARTESIAN_POINT('Ctrl Pts',(6.18934672976297,3.29948628853455,15.9296860249002));
#157161=CARTESIAN_POINT('Ctrl Pts',(6.09424340208908,3.46667332158566,15.93840898793));
#157162=CARTESIAN_POINT('Ctrl Pts',(6.00321710348158,3.62669313546637,15.9467580021749));
#157163=CARTESIAN_POINT('Ctrl Pts',(5.90581356536447,3.78325023446906,15.9551070164198));
#157164=CARTESIAN_POINT('Ctrl Pts',(5.80231996284411,3.9358238796065,15.9634560306648));
#157165=CARTESIAN_POINT('Ctrl Pts',(5.69890358042771,4.0882836843475,15.9717988154256));
#157166=CARTESIAN_POINT('Ctrl Pts',(5.58940637239973,4.23676568829624,15.9801416001865));
#157167=CARTESIAN_POINT('Ctrl Pts',(5.47416030766408,4.38077567201234,15.9884843849473));
#157168=CARTESIAN_POINT('Ctrl Pts',(5.3590020329863,4.52467595441383,15.9968208144928));
#157169=CARTESIAN_POINT('Ctrl Pts',(5.23810383945535,4.66411075531959,16.0051572440384));
#157170=CARTESIAN_POINT('Ctrl Pts',(5.11183979577424,4.79861651570938,16.0134936735839));
#157171=CARTESIAN_POINT('Ctrl Pts',(5.0945632853444,4.81702072726874,16.0146343341218));
#157172=CARTESIAN_POINT('Ctrl Pts',(5.07718637847166,4.83533270612563,16.0157749946598));
#157173=CARTESIAN_POINT('Ctrl Pts',(5.05971009278249,4.85355131213167,16.0169156551978));
#157174=CARTESIAN_POINT('Ctrl Pts',(4.93195719158946,4.98673062805503,16.0252539654997));
#157175=CARTESIAN_POINT('Ctrl Pts',(4.79899544814352,5.11480822757598,16.0335922758016));
#157176=CARTESIAN_POINT('Ctrl Pts',(4.66126818530316,5.23738536554077,16.0419305861035));
#157177=CARTESIAN_POINT('Ctrl Pts',(4.52345426914264,5.36003962488125,16.0502741425873));
#157178=CARTESIAN_POINT('Ctrl Pts',(4.3808690978533,5.47718630203073,16.0586176990712));
#157179=CARTESIAN_POINT('Ctrl Pts',(4.23398875277113,5.58846721417488,16.066961255555));
#157180=CARTESIAN_POINT('Ctrl Pts',(4.08699666176198,5.69983278835245,16.0753111597802));
#157181=CARTESIAN_POINT('Ctrl Pts',(3.93570313973195,5.80532349835782,16.0836610640055));
#157182=CARTESIAN_POINT('Ctrl Pts',(3.78061323341272,5.90462447085711,16.0920109682307));
#157183=CARTESIAN_POINT('Ctrl Pts',(3.62529070371132,6.00407438746646,16.1003733966944));
#157184=CARTESIAN_POINT('Ctrl Pts',(3.46616068690274,6.09731583709216,16.108735825158));
#157185=CARTESIAN_POINT('Ctrl Pts',(3.30375413934276,6.18407916744891,16.1170982536217));
#157186=CARTESIAN_POINT('Ctrl Pts',(3.14120871204524,6.27091669228075,16.1254678331017));
#157187=CARTESIAN_POINT('Ctrl Pts',(2.97538145768056,6.3512649022293,16.1338374125817));
#157188=CARTESIAN_POINT('Ctrl Pts',(2.8068238079514,6.42490207502163,16.1422069920616));
#157189=CARTESIAN_POINT('Ctrl Pts',(2.63800617858451,6.49865282418107,16.1505894805982));
#157190=CARTESIAN_POINT('Ctrl Pts',(2.46645004301298,6.56567173289311,16.1589719691348));
#157191=CARTESIAN_POINT('Ctrl Pts',(2.29272383294703,6.62578629208162,16.1673544576714));
#157192=CARTESIAN_POINT('Ctrl Pts',(2.23587777034313,6.64545676088272,16.1700973452756));
#157193=CARTESIAN_POINT('Ctrl Pts',(2.17879945109119,6.66438838201481,16.1728402328799));
#157194=CARTESIAN_POINT('Ctrl Pts',(2.12150903618929,6.68257629749689,16.1755831204842));
#157195=CARTESIAN_POINT('Ctrl Pts',(1.94627098386213,6.73820890009591,16.183972975617));
#157196=CARTESIAN_POINT('Ctrl Pts',(1.76869389559647,6.78699188517103,16.1923628307498));
#157197=CARTESIAN_POINT('Ctrl Pts',(1.58933985198005,6.82873527070775,16.2007526858825));
#157198=CARTESIAN_POINT('Ctrl Pts',(1.41015131376065,6.87044013603351,16.2091347989746));
#157199=CARTESIAN_POINT('Ctrl Pts',(1.22918940765239,6.90511827751886,16.2175169120667));
#157200=CARTESIAN_POINT('Ctrl Pts',(1.04703124785331,6.93262952482814,16.2258990251588));
#157201=CARTESIAN_POINT('Ctrl Pts',(0.865014404179025,6.96011942924032,
16.2342746355077));
#157202=CARTESIAN_POINT('Ctrl Pts',(0.681803480915807,6.98045347548991,
16.2426502458566));
#157203=CARTESIAN_POINT('Ctrl Pts',(0.497986110754245,6.99354247831497,
16.2510258562055));
#157204=CARTESIAN_POINT('Ctrl Pts',(0.314284364448098,7.00662324796289,
16.259396198171));
#157205=CARTESIAN_POINT('Ctrl Pts',(0.129977258900353,7.01246803762569,
16.2677665401366));
#157206=CARTESIAN_POINT('Ctrl Pts',(-0.0543416578270789,7.0110394055892,
16.2761368821022));
#157207=CARTESIAN_POINT('Ctrl Pts',(-0.238571654301916,7.00961146276208,
16.2845031859966));
#157208=CARTESIAN_POINT('Ctrl Pts',(-0.422813122465848,7.00091709807057,
16.2928694898909));
#157209=CARTESIAN_POINT('Ctrl Pts',(-0.606471251806126,6.98497095077945,
16.3012357937852));
#157210=CARTESIAN_POINT('Ctrl Pts',(-0.790078017115247,6.96902926317877,
16.3095997578588));
#157211=CARTESIAN_POINT('Ctrl Pts',(-0.973101441647726,6.94583986398603,
16.3179637219324));
#157212=CARTESIAN_POINT('Ctrl Pts',(-1.15495001680441,6.91546939991665,
16.326327686006));
#157213=CARTESIAN_POINT('Ctrl Pts',(-1.33677060848736,6.88510360935699,
16.3346903630046));
#157214=CARTESIAN_POINT('Ctrl Pts',(-1.51741638717926,6.84755901128605,
16.3430530400031));
#157215=CARTESIAN_POINT('Ctrl Pts',(-1.69630382237542,6.80295376323363,
16.3514157170017));
#157216=CARTESIAN_POINT('Ctrl Pts',(-1.87518757460608,6.75834943352178,
16.359778221828));
#157217=CARTESIAN_POINT('Ctrl Pts',(-2.05231273673844,6.70668482359164,
16.3681407266543));
#157218=CARTESIAN_POINT('Ctrl Pts',(-2.22710835418925,6.64812867965118,
16.3765032314806));
#157219=CARTESIAN_POINT('Ctrl Pts',(-2.40192367192968,6.58956593615741,
16.3848666788005));
#157220=CARTESIAN_POINT('Ctrl Pts',(-2.57440861009297,6.52411021501942,
16.3932301261205));
#157221=CARTESIAN_POINT('Ctrl Pts',(-2.74400928376474,6.45197951121305,
16.4015935734405));
#157222=CARTESIAN_POINT('Ctrl Pts',(-2.91370982307943,6.3798063348212,16.4099619453933));
#157223=CARTESIAN_POINT('Ctrl Pts',(-3.0805224010897,6.30095044972884,16.4183303173461));
#157224=CARTESIAN_POINT('Ctrl Pts',(-3.24391401049165,6.21567763442056,
16.4266986892989));
#157225=CARTESIAN_POINT('Ctrl Pts',(-3.40735457629014,6.13037926914814,
16.4350695686347));
#157226=CARTESIAN_POINT('Ctrl Pts',(-3.56737184065868,6.03866029666453,
16.4434404479705));
#157227=CARTESIAN_POINT('Ctrl Pts',(-3.72345854630337,5.94083184549609,
16.4518113273062));
#157228=CARTESIAN_POINT('Ctrl Pts',(-3.87967750252577,5.84292050533892,
16.4601892991975));
#157229=CARTESIAN_POINT('Ctrl Pts',(-4.03195896960979,5.73888952217155,
16.4685672710888));
#157230=CARTESIAN_POINT('Ctrl Pts',(-4.17982480036675,5.62909328406797,
16.4769452429801));
#157231=CARTESIAN_POINT('Ctrl Pts',(-4.27379473988855,5.55931688067919,
16.4822695123391));
#157232=CARTESIAN_POINT('Ctrl Pts',(-4.36598195812697,5.48721290535029,
16.4875937816981));
#157233=CARTESIAN_POINT('Ctrl Pts',(-4.45627082729048,5.41288064493758,
16.4929180510571));
#157234=CARTESIAN_POINT('Ctrl Pts',(-4.58960858476225,5.30310745802027,
16.5007808822463));
#157235=CARTESIAN_POINT('Ctrl Pts',(-4.71908165106864,5.18824423112787,
16.5086437134356));
#157236=CARTESIAN_POINT('Ctrl Pts',(-4.84426095490537,5.06860556398694,
16.5165065446249));
#157237=CARTESIAN_POINT('Ctrl Pts',(-4.96934407497058,4.94905882336958,
16.5243633342663));
#157238=CARTESIAN_POINT('Ctrl Pts',(-5.09013971963034,4.82474420115351,
16.5322201239076));
#157239=CARTESIAN_POINT('Ctrl Pts',(-5.20625085837897,4.69601730854223,
16.540076913549));
#157240=CARTESIAN_POINT('Ctrl Pts',(-5.32229651594179,4.56736301180475,
16.547929272333));
#157241=CARTESIAN_POINT('Ctrl Pts',(-5.43366266824448,4.43430167672755,
16.5557816311169));
#157242=CARTESIAN_POINT('Ctrl Pts',(-5.53998841533902,4.29722642182251,
16.5636339899009));
#157243=CARTESIAN_POINT('Ctrl Pts',(-5.64628905768406,4.16018353198454,
16.5714844946513));
#157244=CARTESIAN_POINT('Ctrl Pts',(-5.74755142330952,4.01912890439061,
16.5793349994017));
#157245=CARTESIAN_POINT('Ctrl Pts',(-5.84345432267586,3.87448940394742,
16.5871855041521));
#157246=CARTESIAN_POINT('Ctrl Pts',(-5.93934179428829,3.7298731714412,16.5950347460037));
#157247=CARTESIAN_POINT('Ctrl Pts',(-6.02987130763683,3.5816735337559,16.6028839878554));
#157248=CARTESIAN_POINT('Ctrl Pts',(-6.11476478558777,3.43034665586959,
16.610733229707));
#157249=CARTESIAN_POINT('Ctrl Pts',(-6.19968686581309,3.27896879299615,
16.6185851161218));
#157250=CARTESIAN_POINT('Ctrl Pts',(-6.27896893089106,3.12446191839945,
16.6264370025367));
#157251=CARTESIAN_POINT('Ctrl Pts',(-6.35237860285554,2.96730730604079,
16.6342888889515));
#157252=CARTESIAN_POINT('Ctrl Pts',(-6.40628241126751,2.85191063024941,
16.6400544314155));
#157253=CARTESIAN_POINT('Ctrl Pts',(-6.45702090177214,2.73508688812991,
16.6458199738795));
#157254=CARTESIAN_POINT('Ctrl Pts',(-6.50451862268238,2.61703344450889,
16.6515855163435));
#157255=CARTESIAN_POINT('Ctrl Pts',(-6.5840609995976,2.41933445330072,16.6612408207034));
#157256=CARTESIAN_POINT('Ctrl Pts',(-6.65447352736123,2.21828741597566,
16.6708961250633));
#157257=CARTESIAN_POINT('Ctrl Pts',(-6.71555819057391,2.01467236828117,
16.6805514294232));
#157258=CARTESIAN_POINT('Ctrl Pts',(-6.77698125136142,1.80992933142026,
16.690260222358));
#157259=CARTESIAN_POINT('Ctrl Pts',(-6.82897285094434,1.60258981369847,
16.6999690152927));
#157260=CARTESIAN_POINT('Ctrl Pts',(-6.87138419480713,1.39345104322139,
16.7096778082275));
#157261=CARTESIAN_POINT('Ctrl Pts',(-6.91399962565779,1.18330587922256,
16.7194333206982));
#157262=CARTESIAN_POINT('Ctrl Pts',(-6.94694239185566,0.971344151661304,
16.729188833169));
#157263=CARTESIAN_POINT('Ctrl Pts',(-6.97011401131694,0.758378026938607,
16.7389443456397));
#157264=CARTESIAN_POINT('Ctrl Pts',(-6.99330857424638,0.545201032988176,
16.7487095175686));
#157265=CARTESIAN_POINT('Ctrl Pts',(-7.00671264531666,0.331017691958229,
16.7584746894976));
#157266=CARTESIAN_POINT('Ctrl Pts',(-7.01027962605474,0.116645304328492,
16.7682398614265));
#157267=CARTESIAN_POINT('Ctrl Pts',(-7.01384174329551,-0.0974347914142347,
16.7779917187651));
#157268=CARTESIAN_POINT('Ctrl Pts',(-7.00759357668027,-0.311703380643881,
16.7877435761037));
#157269=CARTESIAN_POINT('Ctrl Pts',(-6.99154059236441,-0.525344370694879,
16.7974954334422));
#157270=CARTESIAN_POINT('Ctrl Pts',(-6.98454032859053,-0.618507314970021,
16.8017479495048));
#157271=CARTESIAN_POINT('Ctrl Pts',(-6.9756762554175,-0.711550891502383,
16.8060004655673));
#157272=CARTESIAN_POINT('Ctrl Pts',(-6.96495193175325,-0.804407328948929,
16.8102529816299));
#157273=CARTESIAN_POINT('Ctrl Pts',(-6.94469357652446,-0.979814072904426,
16.8182860272287));
#157274=CARTESIAN_POINT('Ctrl Pts',(-6.91778355046215,-1.15463820249878,
16.8263190728275));
#157275=CARTESIAN_POINT('Ctrl Pts',(-6.8842694409298,-1.32833008969161,
16.8343521184264));
#157276=CARTESIAN_POINT('Ctrl Pts',(-6.85077687555747,-1.50191032105159,
16.8423800000742));
#157277=CARTESIAN_POINT('Ctrl Pts',(-6.81068874636495,-1.67435940038211,
16.8504078817219));
#157278=CARTESIAN_POINT('Ctrl Pts',(-6.76410433349934,-1.84513390517747,
16.8584357633697));
#157279=CARTESIAN_POINT('Ctrl Pts',(-6.71754095395535,-2.01583130360049,
16.8664600203498));
#157280=CARTESIAN_POINT('Ctrl Pts',(-6.66448722721792,-2.18485528003029,
16.87448427733));
#157281=CARTESIAN_POINT('Ctrl Pts',(-6.60509328167289,-2.35167372373373,
16.8825085343101));
#157282=CARTESIAN_POINT('Ctrl Pts',(-6.54570651746083,-2.51847199738821,
16.8905318210758));
#157283=CARTESIAN_POINT('Ctrl Pts',(-6.4799811769894,-2.68306492176134,
16.8985551078415));
#157284=CARTESIAN_POINT('Ctrl Pts',(-6.40811696210377,-2.8449364777615,
16.9065783946072));
#157285=CARTESIAN_POINT('Ctrl Pts',(-6.33625863584952,-3.00679476983154,
16.9146010239361));
#157286=CARTESIAN_POINT('Ctrl Pts',(-6.25826258960548,-3.16593180423259,
16.922623653265));
#157287=CARTESIAN_POINT('Ctrl Pts',(-6.17437616390429,-3.32185272838977,
16.9306462825939));
#157288=CARTESIAN_POINT('Ctrl Pts',(-6.09045820287907,-3.47783226771412,
16.9386719278603));
#157289=CARTESIAN_POINT('Ctrl Pts',(-6.00064561527444,-3.63059295994871,
16.9466975731267));
#157290=CARTESIAN_POINT('Ctrl Pts',(-5.90523126753579,-3.77966536077172,
16.9547232183931));
#157291=CARTESIAN_POINT('Ctrl Pts',(-5.84896915384572,-3.8675675323207,
16.9594556279009));
#157292=CARTESIAN_POINT('Ctrl Pts',(-5.79076015132948,-3.95418780036338,
16.9641880374086));
#157293=CARTESIAN_POINT('Ctrl Pts',(-5.730671251391,-4.03943480835881,16.9689204469164));
#157294=CARTESIAN_POINT('Ctrl Pts',(-5.61982306083929,-4.19669308061732,
16.977650495751));
#157295=CARTESIAN_POINT('Ctrl Pts',(-5.50252001517797,-4.3493551652282,
16.9863805445857));
#157296=CARTESIAN_POINT('Ctrl Pts',(-5.37916323089467,-4.49691333003994,
16.9951105934203));
#157297=CARTESIAN_POINT('Ctrl Pts',(-5.25577077784348,-4.6445141614789,
17.0038431665595));
#157298=CARTESIAN_POINT('Ctrl Pts',(-5.12632126788788,-4.78700791715897,
17.0125757396987));
#157299=CARTESIAN_POINT('Ctrl Pts',(-4.99125530779404,-4.92392089852364,
17.0213083128378));
#157300=CARTESIAN_POINT('Ctrl Pts',(-4.8542705201311,-5.06277894734296,
17.0301649461182));
#157301=CARTESIAN_POINT('Ctrl Pts',(-4.71150868836064,-5.19589623937759,
17.0390215793986));
#157302=CARTESIAN_POINT('Ctrl Pts',(-4.56346755050197,-5.32281790765151,
17.0478782126791));
#157303=CARTESIAN_POINT('Ctrl Pts',(-4.41740719337916,-5.44804137231043,
17.0566163447858));
#157304=CARTESIAN_POINT('Ctrl Pts',(-4.26620815230103,-5.56723381445818,
17.0653544768926));
#157305=CARTESIAN_POINT('Ctrl Pts',(-4.11038189632529,-5.67999887577993,
17.0740926089993));
#157306=CARTESIAN_POINT('Ctrl Pts',(-3.95138581057447,-5.79505781271802,
17.0830084928666));
#157307=CARTESIAN_POINT('Ctrl Pts',(-3.78757247686869,-5.90342489858532,
17.0919243767338));
#157308=CARTESIAN_POINT('Ctrl Pts',(-3.61951728623572,-6.00472490436829,
17.100840260601));
#157309=CARTESIAN_POINT('Ctrl Pts',(-3.45146209560273,-6.10602491015128,
17.1097561444683));
#157310=CARTESIAN_POINT('Ctrl Pts',(-3.27916531018121,-6.20025768494112,
17.1186720283355));
#157311=CARTESIAN_POINT('Ctrl Pts',(-3.10323089411683,-6.2870966733699,
17.1275879122028));
#157312=CARTESIAN_POINT('Ctrl Pts',(-2.93075363378638,-6.37222925373202,
17.136328596699));
#157313=CARTESIAN_POINT('Ctrl Pts',(-2.75476205771371,-6.45026497194488,
17.1450692811952));
#157314=CARTESIAN_POINT('Ctrl Pts',(-2.5758462836326,-6.52093877333595,
17.1538099656915));
#157315=CARTESIAN_POINT('Ctrl Pts',(-2.39696269947126,-6.59159985933617,
17.1625490775933));
#157316=CARTESIAN_POINT('Ctrl Pts',(-2.21515622254328,-6.65490157315164,
17.1712881894952));
#157317=CARTESIAN_POINT('Ctrl Pts',(-2.03103635227476,-6.71062723582814,
17.1800273013971));
#157318=CARTESIAN_POINT('Ctrl Pts',(-1.84453094409265,-6.76707490466769,
17.1888796410715));
#157319=CARTESIAN_POINT('Ctrl Pts',(-1.65565204428361,-6.81574873246951,
17.1977319807458));
#157320=CARTESIAN_POINT('Ctrl Pts',(-1.46504971957287,-6.85647547079981,
17.2065843204201));
#157321=CARTESIAN_POINT('Ctrl Pts',(-1.27698177936859,-6.89666067735824,
17.2153189530699));
#157322=CARTESIAN_POINT('Ctrl Pts',(-1.08723623906643,-6.92910877720895,
17.2240535857197));
#157323=CARTESIAN_POINT('Ctrl Pts',(-0.896449502418545,-6.95370439780938,
17.2327882183694));
#157324=CARTESIAN_POINT('Ctrl Pts',(-0.701806231672854,-6.97879719054645,
17.2416994115561));
#157325=CARTESIAN_POINT('Ctrl Pts',(-0.506079508319231,-6.99571660669538,
17.2506106047427));
#157326=CARTESIAN_POINT('Ctrl Pts',(-0.309953463721105,-7.00439543521261,
17.2595217979293));
#157327=CARTESIAN_POINT('Ctrl Pts',(-0.113827419122962,-7.01307426372985,
17.2684329911159));
#157328=CARTESIAN_POINT('Ctrl Pts',(0.0826976444819196,-7.01351247775379,
17.2773441843025));
#157329=CARTESIAN_POINT('Ctrl Pts',(0.278933644378881,-7.00569929304231,
17.2862553774892));
#157330=CARTESIAN_POINT('Ctrl Pts',(0.455669164994588,-6.99866252472062,
17.2942810423415));
#157331=CARTESIAN_POINT('Ctrl Pts',(0.632251418391536,-6.98492904811914,
17.3023067071939));
#157332=CARTESIAN_POINT('Ctrl Pts',(0.80812813756787,-6.96452119501198,
17.3103323720463));
#157333=CARTESIAN_POINT('Ctrl Pts',(0.983949037787381,-6.94411981885684,
17.3183554897495));
#157334=CARTESIAN_POINT('Ctrl Pts',(1.15906448589412,-6.91704832570057,
17.3263786074527));
#157335=CARTESIAN_POINT('Ctrl Pts',(1.33292641381189,-6.88338098160073,
17.3344017251559));
#157336=CARTESIAN_POINT('Ctrl Pts',(1.50676641621861,-6.84971788324769,
17.3424238310738));
#157337=CARTESIAN_POINT('Ctrl Pts',(1.67935285364287,-6.80946066104088,
17.3504459369916));
#157338=CARTESIAN_POINT('Ctrl Pts',(1.85014699150703,-6.76273485154619,
17.3584680429094));
#157339=CARTESIAN_POINT('Ctrl Pts',(2.02100459705031,-6.71599167858271,
17.3664931298689));
#157340=CARTESIAN_POINT('Ctrl Pts',(2.19006821782699,-6.66277521032895,
17.3745182168285));
#157341=CARTESIAN_POINT('Ctrl Pts',(2.35681301314129,-6.60326123847814,
17.382543303788));
#157342=CARTESIAN_POINT('Ctrl Pts',(2.52359064800853,-6.54373554564842,
17.3905699712482));
#157343=CARTESIAN_POINT('Ctrl Pts',(2.68804820535844,-6.4779100099314,17.3985966387084));
#157344=CARTESIAN_POINT('Ctrl Pts',(2.84968022419069,-6.40600883408355,
17.4066233061687));
#157345=CARTESIAN_POINT('Ctrl Pts',(3.01144200063807,-6.33404993622512,
17.4146564174093));
#157346=CARTESIAN_POINT('Ctrl Pts',(3.17037337705654,-6.25600581409494,
17.4226895286498));
#157347=CARTESIAN_POINT('Ctrl Pts',(3.32599236708978,-6.17214722252803,
17.4307226398904));
#157348=CARTESIAN_POINT('Ctrl Pts',(3.41768872918733,-6.12273469404635,
17.4354560408521));
#157349=CARTESIAN_POINT('Ctrl Pts',(3.50823552404223,-6.07130424260402,
17.4401894418139));
#157350=CARTESIAN_POINT('Ctrl Pts',(3.59753882558523,-6.01791832454603,
17.4449228427756));
#157351=CARTESIAN_POINT('Ctrl Pts',(3.78150640606299,-5.90794167186893,
17.4546737960697));
#157352=CARTESIAN_POINT('Ctrl Pts',(3.96030414582063,-5.78960001110138,
17.4644247493639));
#157353=CARTESIAN_POINT('Ctrl Pts',(4.13326669071841,-5.6633676400087,17.4741757026581));
#157354=CARTESIAN_POINT('Ctrl Pts',(4.30647842060935,-5.53695340750466,
17.4839407040297));
#157355=CARTESIAN_POINT('Ctrl Pts',(4.47383810857436,-5.40262574800827,
17.4937057054013));
#157356=CARTESIAN_POINT('Ctrl Pts',(4.63471077704827,-5.26090130829429,
17.503470706773));
#157357=CARTESIAN_POINT('Ctrl Pts',(4.7953153041157,-5.11941309385686,17.5132194319106));
#157358=CARTESIAN_POINT('Ctrl Pts',(4.94945439307791,-4.97055276472544,
17.5229681570481));
#157359=CARTESIAN_POINT('Ctrl Pts',(5.09652968086165,-4.81487401440539,
17.5327168821857));
#157360=CARTESIAN_POINT('Ctrl Pts',(5.24320130400896,-4.65962254189043,
17.5424388508529));
#157361=CARTESIAN_POINT('Ctrl Pts',(5.38284780231951,-4.49759003650188,
17.5521608195201));
#157362=CARTESIAN_POINT('Ctrl Pts',(5.51490953229886,-4.32936478170403,
17.5618827881872));
#157363=CARTESIAN_POINT('Ctrl Pts',(5.64609744430358,-4.16225262947914,
17.571540429127));
#157364=CARTESIAN_POINT('Ctrl Pts',(5.76980057754607,-3.9890294274626,17.5811980700667));
#157365=CARTESIAN_POINT('Ctrl Pts',(5.8855044144789,-3.81031026947274,17.5908557110064));
#157366=CARTESIAN_POINT('Ctrl Pts',(5.93636023424994,-3.73175704661254,
17.5951005766916));
#157367=CARTESIAN_POINT('Ctrl Pts',(5.98567111523607,-3.65214255663833,
17.5993454423769));
#157368=CARTESIAN_POINT('Ctrl Pts',(6.03339552127299,-3.57152139100175,
17.6035903080621));
#157369=CARTESIAN_POINT('Ctrl Pts',(6.12167269252395,-3.42239416163723,
17.611442155076));
#157370=CARTESIAN_POINT('Ctrl Pts',(6.20448222130841,-3.26988191299991,
17.6192940020899));
#157371=CARTESIAN_POINT('Ctrl Pts',(6.28155018781221,-3.11444277528041,
17.6271458491038));
#157372=CARTESIAN_POINT('Ctrl Pts',(6.35859629846379,-2.9590477188437,17.6349954693974));
#157373=CARTESIAN_POINT('Ctrl Pts',(6.42990391644197,-2.80072776584618,
17.642845089691));
#157374=CARTESIAN_POINT('Ctrl Pts',(6.49524492938314,-2.63996588421567,
17.6506947099845));
#157375=CARTESIAN_POINT('Ctrl Pts',(6.56058072568014,-2.47921683736524,
17.6585437035863));
#157376=CARTESIAN_POINT('Ctrl Pts',(6.61995072229686,-2.31602660365896,
17.6663926971881));
#157377=CARTESIAN_POINT('Ctrl Pts',(6.67317494277457,-2.15089812534802,
17.6742416907899));
#157378=CARTESIAN_POINT('Ctrl Pts',(6.72642610911662,-1.98568604732373,
17.6820946581073));
#157379=CARTESIAN_POINT('Ctrl Pts',(6.77352516535617,-1.81853412759885,
17.6899476254247));
#157380=CARTESIAN_POINT('Ctrl Pts',(6.81434192970358,-1.64996079577172,
17.6978005927421));
#157381=CARTESIAN_POINT('Ctrl Pts',(6.85516906013767,-1.48134465198247,
17.7056555544494));
#157382=CARTESIAN_POINT('Ctrl Pts',(6.88971064413953,-1.31130675078587,
17.7135105161566));
#157383=CARTESIAN_POINT('Ctrl Pts',(6.91788777553333,-1.14037506445314,
17.7213654778639));
#157384=CARTESIAN_POINT('Ctrl Pts',(6.94609287508533,-0.969273714133762,
17.7292282362772));
#157385=CARTESIAN_POINT('Ctrl Pts',(6.96792085686429,-0.797277185065159,
17.7370909946906));
#157386=CARTESIAN_POINT('Ctrl Pts',(6.98334471739352,-0.624918491126651,
17.7449537531039));
#157387=CARTESIAN_POINT('Ctrl Pts',(6.99465944015861,-0.498478626452574,
17.7507217598521));
#157388=CARTESIAN_POINT('Ctrl Pts',(7.00252888663807,-0.371843959662768,
17.7564897666003));
#157389=CARTESIAN_POINT('Ctrl Pts',(7.00696022589238,-0.245224295823586,
17.7622577733485));
#157390=CARTESIAN_POINT('Ctrl Pts',(7.00984801535904,-0.162709527596158,
17.7660166345358));
#157391=CARTESIAN_POINT('Ctrl Pts',(7.01127732144656,-0.0801718186294929,
17.7697754957232));
#157392=CARTESIAN_POINT('Ctrl Pts',(7.01124960457305,0.00235475566585457,
17.7735343569105));
#157393=CARTESIAN_POINT('Ctrl Pts',(7.01124960457286,0.00235475623571418,
17.7735343569365));
#157394=CARTESIAN_POINT('Ctrl Pts',(7.0111881852894,0.185229705388182,17.7818638138947));
#157395=CARTESIAN_POINT('Ctrl Pts',(7.0039674730019,0.368245297451978,17.790193270853));
#157396=CARTESIAN_POINT('Ctrl Pts',(6.98958012196288,0.550814198402105,
17.7985227278113));
#157397=CARTESIAN_POINT('Ctrl Pts',(6.97520604982793,0.733214596136248,
17.8068444970403));
#157398=CARTESIAN_POINT('Ctrl Pts',(6.95367855695298,0.915168792105551,
17.8151662662693));
#157399=CARTESIAN_POINT('Ctrl Pts',(6.92504233787672,1.09609086353046,17.8234880354983));
#157400=CARTESIAN_POINT('Ctrl Pts',(6.89642175765243,1.27691412954095,17.8318052600311));
#157401=CARTESIAN_POINT('Ctrl Pts',(6.86070024019595,1.45670606423809,17.8401224845638));
#157402=CARTESIAN_POINT('Ctrl Pts',(6.81797423568344,1.63488650494671,17.8484397090966));
#157403=CARTESIAN_POINT('Ctrl Pts',(6.77526708842652,1.81298830516108,17.8567532627963));
#157404=CARTESIAN_POINT('Ctrl Pts',(6.72556169588046,1.98947970414347,17.865066816496));
#157405=CARTESIAN_POINT('Ctrl Pts',(6.66900552753703,2.16379107960555,17.8733803701958));
#157406=CARTESIAN_POINT('Ctrl Pts',(6.63837243453911,2.25820512375897,17.8778833248882));
#157407=CARTESIAN_POINT('Ctrl Pts',(6.60573038066985,2.35197980392451,17.8823862795806));
#157408=CARTESIAN_POINT('Ctrl Pts',(6.57110895151814,2.44502632087637,17.886889234273));
#157409=CARTESIAN_POINT('',(7.01124984869581,-0.00145659295646808,17.2264656431293));
#157410=CARTESIAN_POINT('Ctrl Pts',(6.57110895151813,2.44502632087639,17.3396585048403));
#157411=CARTESIAN_POINT('Ctrl Pts',(6.64521162053806,2.24587234548946,17.3299972645521));
#157412=CARTESIAN_POINT('Ctrl Pts',(6.71031798372647,2.04318290855153,17.3203360242638));
#157413=CARTESIAN_POINT('Ctrl Pts',(6.76612737026639,1.83770154590782,17.3106747839755));
#157414=CARTESIAN_POINT('Ctrl Pts',(6.79678406298721,1.72482843647281,17.3053677613906));
#157415=CARTESIAN_POINT('Ctrl Pts',(6.82463624788957,1.61111333633684,17.3000607388057));
#157416=CARTESIAN_POINT('Ctrl Pts',(6.84963993305301,1.49668278203018,17.2947537162207));
#157417=CARTESIAN_POINT('Ctrl Pts',(6.88499295409668,1.3348879998611,17.287250051065));
#157418=CARTESIAN_POINT('Ctrl Pts',(6.91464614817789,1.17167025084036,17.2797463859093));
#157419=CARTESIAN_POINT('Ctrl Pts',(6.93848291677126,1.00751246948778,17.2722427207536));
#157420=CARTESIAN_POINT('Ctrl Pts',(6.96271946392455,0.840601514559226,
17.2646132078162));
#157421=CARTESIAN_POINT('Ctrl Pts',(6.98094261072084,0.672719122730744,
17.2569836948789));
#157422=CARTESIAN_POINT('Ctrl Pts',(6.99308397869091,0.504383811671779,
17.2493541819415));
#157423=CARTESIAN_POINT('Ctrl Pts',(7.00522534666098,0.336048500612814,
17.2417246690041));
#157424=CARTESIAN_POINT('Ctrl Pts',(7.01128489985525,0.167260710847184,
17.2340951560667));
#157425=CARTESIAN_POINT('Ctrl Pts',(7.01124984869581,-0.00145659295646722,
17.2264656431293));
#157426=CARTESIAN_POINT('Ctrl Pts',(7.01124984869562,-0.00145659383538793,
17.2264656430896));
#157427=CARTESIAN_POINT('Ctrl Pts',(7.01121141547279,-0.186453208016376,
17.2180999685));
#157428=CARTESIAN_POINT('Ctrl Pts',(7.00384680112655,-0.37131131097293,
17.2097342939103));
#157429=CARTESIAN_POINT('Ctrl Pts',(6.98921446351228,-0.555434735617764,
17.2013686193206));
#157430=CARTESIAN_POINT('Ctrl Pts',(6.97456974963572,-0.739713894763606,
17.1929958689113));
#157431=CARTESIAN_POINT('Ctrl Pts',(6.95264508443871,-0.923256813949637,
17.1846231185019));
#157432=CARTESIAN_POINT('Ctrl Pts',(6.92355038038466,-1.10547577665705,
17.1762503680925));
#157433=CARTESIAN_POINT('Ctrl Pts',(6.89440752844861,-1.28799628761518,
17.1678637618901));
#157434=CARTESIAN_POINT('Ctrl Pts',(6.85807098344544,-1.46918814448098,
17.1594771556876));
#157435=CARTESIAN_POINT('Ctrl Pts',(6.81470140781121,-1.64847544260627,
17.1510905494852));
#157436=CARTESIAN_POINT('Ctrl Pts',(6.78883754642982,-1.75539513823031,
17.1460891166349));
#157437=CARTESIAN_POINT('Ctrl Pts',(6.76047337797917,-1.86163779181118,
17.1410876837846));
#157438=CARTESIAN_POINT('Ctrl Pts',(6.72965120968409,-1.96708443095296,
17.1360862509343));
#157439=CARTESIAN_POINT('Ctrl Pts',(6.67801997088463,-2.14372160177126,
17.1277081844933));
#157440=CARTESIAN_POINT('Ctrl Pts',(6.61939583769859,-2.31844204455275,
17.1193301180522));
#157441=CARTESIAN_POINT('Ctrl Pts',(6.55394277257689,-2.49067474718945,
17.1109520516112));
#157442=CARTESIAN_POINT('Ctrl Pts',(6.48853446348344,-2.66278967915043,
17.1025797139925));
#157443=CARTESIAN_POINT('Ctrl Pts',(6.41630664854421,-2.83241995612727,
17.0942073763737));
#157444=CARTESIAN_POINT('Ctrl Pts',(6.33747279090054,-2.99901070139728,
17.085835038755));
#157445=CARTESIAN_POINT('Ctrl Pts',(6.25868127787468,-3.16551196453802,
17.0774671982324));
#157446=CARTESIAN_POINT('Ctrl Pts',(6.1732909375192,-3.32897665484439,17.0690993577098));
#157447=CARTESIAN_POINT('Ctrl Pts',(6.08156311049281,-3.48887040395499,
17.0607315171872));
#157448=CARTESIAN_POINT('Ctrl Pts',(5.98987111645723,-3.64870169141759,
17.0523669455172));
#157449=CARTESIAN_POINT('Ctrl Pts',(5.89184673599072,-3.80496453474687,
17.0440023738473));
#157450=CARTESIAN_POINT('Ctrl Pts',(5.7877971738053,-3.95714928166621,17.0356378021774));
#157451=CARTESIAN_POINT('Ctrl Pts',(5.68377302768726,-4.10929685459174,
17.0272752737118));
#157452=CARTESIAN_POINT('Ctrl Pts',(5.57372682060596,-4.25736804682712,
17.0189127452462));
#157453=CARTESIAN_POINT('Ctrl Pts',(5.45800923434146,-4.40088192983445,
17.0105502167806));
#157454=CARTESIAN_POINT('Ctrl Pts',(5.34228241345161,-4.54440726569856,
17.0021870209591));
#157455=CARTESIAN_POINT('Ctrl Pts',(5.22088351075938,-4.68337430608855,
16.9938238251376));
#157456=CARTESIAN_POINT('Ctrl Pts',(5.09420415672048,-4.81733438450684,
16.9854606293161));
#157457=CARTESIAN_POINT('Ctrl Pts',(4.9675161634036,-4.9513035987339,16.9770968631414));
#157458=CARTESIAN_POINT('Ctrl Pts',(4.83554722643299,-5.08026493103917,
16.9687330969667));
#157459=CARTESIAN_POINT('Ctrl Pts',(4.69872669322736,-5.20380572512586,
16.960369330792));
#157460=CARTESIAN_POINT('Ctrl Pts',(4.56187858774039,-5.32737141534072,
16.9520038791384));
#157461=CARTESIAN_POINT('Ctrl Pts',(4.42017718049494,-5.44551416882182,
16.9436384274849));
#157462=CARTESIAN_POINT('Ctrl Pts',(4.27408614211591,-5.55786057870048,
16.9352729758313));
#157463=CARTESIAN_POINT('Ctrl Pts',(4.12794617813501,-5.67024461317118,
16.9269047226044));
#157464=CARTESIAN_POINT('Ctrl Pts',(3.977413912167,-5.77682823291574,16.9185364693776));
#157465=CARTESIAN_POINT('Ctrl Pts',(3.82298366178426,-5.87728019446331,
16.9101682161507));
#157466=CARTESIAN_POINT('Ctrl Pts',(3.66841023252764,-5.97782528931019,
16.9017922043592));
#157467=CARTESIAN_POINT('Ctrl Pts',(3.50993187292332,-6.07222718633111,
16.8934161925677));
#157468=CARTESIAN_POINT('Ctrl Pts',(3.34807034260579,-6.16019898570359,
16.8850401807763));
#157469=CARTESIAN_POINT('Ctrl Pts',(3.18612943339389,-6.24821392753344,
16.8766600612851));
#157470=CARTESIAN_POINT('Ctrl Pts',(3.02080233661885,-6.3297923320713,16.868279941794));
#157471=CARTESIAN_POINT('Ctrl Pts',(2.8526332423941,-6.40469438356649,16.8598998223028));
#157472=CARTESIAN_POINT('Ctrl Pts',(2.6842719936766,-6.47968202014363,16.8515101274636));
#157473=CARTESIAN_POINT('Ctrl Pts',(2.51306256168837,-6.5479779323654,16.8431204326244));
#157474=CARTESIAN_POINT('Ctrl Pts',(2.33956809462149,-6.60939087156518,
16.8347307377852));
#157475=CARTESIAN_POINT('Ctrl Pts',(2.22941945143073,-6.64838088687561,
16.8294042653106));
#157476=CARTESIAN_POINT('Ctrl Pts',(2.11835009357165,-6.68459753836778,
16.824077792836));
#157477=CARTESIAN_POINT('Ctrl Pts',(2.00650681878506,-6.71800245226727,
16.8187513203614));
#157478=CARTESIAN_POINT('Ctrl Pts',(1.83051941084748,-6.77056568613866,
16.8103700199566));
#157479=CARTESIAN_POINT('Ctrl Pts',(1.65226018973763,-6.81627070874301,
16.8019887195517));
#157480=CARTESIAN_POINT('Ctrl Pts',(1.47228955157064,-6.85492451007565,
16.7936074191468));
#157481=CARTESIAN_POINT('Ctrl Pts',(1.29254699984151,-6.89352932337367,
16.7852367408132));
#157482=CARTESIAN_POINT('Ctrl Pts',(1.11109767133741,-6.92510065645303,
16.7768660624797));
#157483=CARTESIAN_POINT('Ctrl Pts',(0.928517585893615,-6.94949506476451,
16.7684953841461));
#157484=CARTESIAN_POINT('Ctrl Pts',(0.746144697499774,-6.97386178961082,
16.7601342050953));
#157485=CARTESIAN_POINT('Ctrl Pts',(0.562643932545363,-6.99106777960009,
16.7517730260445));
#157486=CARTESIAN_POINT('Ctrl Pts',(0.378602425101677,-7.00102040892663,
16.7434118469937));
#157487=CARTESIAN_POINT('Ctrl Pts',(0.194799733223228,-7.01096012354261,
16.735061517559));
#157488=CARTESIAN_POINT('Ctrl Pts',(0.0104580240532623,-7.01366523329991,
16.7267111881243));
#157489=CARTESIAN_POINT('Ctrl Pts',(-0.173829587183502,-7.00909479441673,
16.7183608586895));
#157490=CARTESIAN_POINT('Ctrl Pts',(-0.357975400127153,-7.00452787221287,
16.7100169543338));
#157491=CARTESIAN_POINT('Ctrl Pts',(-0.542066871929678,-6.99269656545033,
16.7016730499781));
#157492=CARTESIAN_POINT('Ctrl Pts',(-0.725508864308825,-6.97361193717498,
16.6933291456224));
#157493=CARTESIAN_POINT('Ctrl Pts',(-0.908803514935531,-6.95454263779209,
16.6849919431427));
#157494=CARTESIAN_POINT('Ctrl Pts',(-1.09144940157904,-6.92823166965606,
16.676654740663));
#157495=CARTESIAN_POINT('Ctrl Pts',(-1.27285433476826,-6.89474208400588,
16.6683175381833));
#157496=CARTESIAN_POINT('Ctrl Pts',(-1.33257183744352,-6.88371749726781,
16.6655729771472));
#157497=CARTESIAN_POINT('Ctrl Pts',(-1.39215489261315,-6.87191538931628,
16.6628284161111));
#157498=CARTESIAN_POINT('Ctrl Pts',(-1.45158250318175,-6.85933923923847,
16.660083855075));
#157499=CARTESIAN_POINT('Ctrl Pts',(-1.63213081342386,-6.82113136542065,
16.6517455447731));
#157500=CARTESIAN_POINT('Ctrl Pts',(-1.81109548287068,-6.77580649576908,
16.6434072344712));
#157501=CARTESIAN_POINT('Ctrl Pts',(-1.98790383542801,-6.7235306873391,
16.6350689241693));
#157502=CARTESIAN_POINT('Ctrl Pts',(-2.16482342980106,-6.67122198874435,
16.6267253676855));
#157503=CARTESIAN_POINT('Ctrl Pts',(-2.33958368701016,-6.61195372118975,
16.6183818112017));
#157504=CARTESIAN_POINT('Ctrl Pts',(-2.51162909085513,-6.54594117545142,
16.6100382547179));
#157505=CARTESIAN_POINT('Ctrl Pts',(-2.68380538609342,-6.47987840765602,
16.6016883504927));
#157506=CARTESIAN_POINT('Ctrl Pts',(-2.85326240251176,-6.40706124421282,
16.5933384462675));
#157507=CARTESIAN_POINT('Ctrl Pts',(-3.0194661192203,-6.32775243806051,
16.5849885420423));
#157508=CARTESIAN_POINT('Ctrl Pts',(-3.18591912920494,-6.24832467456777,
16.5766261135786));
#157509=CARTESIAN_POINT('Ctrl Pts',(-3.34910879232073,-6.16238595203878,
16.568263685115));
#157510=CARTESIAN_POINT('Ctrl Pts',(-3.50852581953311,-6.07024489919225,
16.5599012566513));
#157511=CARTESIAN_POINT('Ctrl Pts',(-3.66807917003529,-5.97802505318498,
16.5515316771713));
#157512=CARTESIAN_POINT('Ctrl Pts',(-3.82385317136701,-5.8795924689408,
16.5431620976914));
#157513=CARTESIAN_POINT('Ctrl Pts',(-3.97536843563536,-5.77529846531364,
16.5347925182115));
#157514=CARTESIAN_POINT('Ctrl Pts',(-4.12711739373861,-5.6708436008928,
16.5264100296749));
#157515=CARTESIAN_POINT('Ctrl Pts',(-4.27459422694588,-5.56050944732146,
16.5180275411383));
#157516=CARTESIAN_POINT('Ctrl Pts',(-4.41735237280503,-5.44468773916134,
16.5096450526017));
#157517=CARTESIAN_POINT('Ctrl Pts',(-4.4640651773608,-5.40678897840034,
16.5069021649974));
#157518=CARTESIAN_POINT('Ctrl Pts',(-4.51027304346737,-5.36830295603565,
16.504159277393));
#157519=CARTESIAN_POINT('Ctrl Pts',(-4.55596120317526,-5.3292442313767,
16.5014163897886));
#157520=CARTESIAN_POINT('Ctrl Pts',(-4.69571065576761,-5.2097726784636,
16.4930265346558));
#157521=CARTESIAN_POINT('Ctrl Pts',(-4.83087709247391,-5.08469895501282,
16.484636679523));
#157522=CARTESIAN_POINT('Ctrl Pts',(-4.96100246275852,-4.95440017832672,
16.4762468243903));
#157523=CARTESIAN_POINT('Ctrl Pts',(-5.09100775517568,-4.82422163952509,
16.4678647112982));
#157524=CARTESIAN_POINT('Ctrl Pts',(-5.21598102341111,-4.68882789082997,
16.4594825982061));
#157525=CARTESIAN_POINT('Ctrl Pts',(-5.33549858863682,-4.54863511101456,
16.451100485114));
#157526=CARTESIAN_POINT('Ctrl Pts',(-5.45492343356298,-4.40855109108324,
16.4427248747651));
#157527=CARTESIAN_POINT('Ctrl Pts',(-5.5689008012334,-4.26367571188172,
16.4343492644162));
#157528=CARTESIAN_POINT('Ctrl Pts',(-5.67704476441904,-4.11446099814816,
16.4259736540673));
#157529=CARTESIAN_POINT('Ctrl Pts',(-5.7851207034458,-3.96534014268552,
16.4176033121018));
#157530=CARTESIAN_POINT('Ctrl Pts',(-5.88737036182711,-3.81188566056653,
16.4092329701362));
#157531=CARTESIAN_POINT('Ctrl Pts',(-5.98344863786708,-3.65458191322983,
16.4008626281706));
#157532=CARTESIAN_POINT('Ctrl Pts',(-6.07948056324105,-3.49735405332319,
16.3924963242763));
#157533=CARTESIAN_POINT('Ctrl Pts',(-6.16934687232379,-3.33628091136447,
16.384130020382));
#157534=CARTESIAN_POINT('Ctrl Pts',(-6.25274603156381,-3.17187541168676,
16.3757637164876));
#157535=CARTESIAN_POINT('Ctrl Pts',(-6.33612186639654,-3.00751589161928,
16.367399752414));
#157536=CARTESIAN_POINT('Ctrl Pts',(-6.41303400803017,-2.8398261643493,
16.3590357883404));
#157537=CARTESIAN_POINT('Ctrl Pts',(-6.48322683788039,-2.6693438015901,
16.3506718242668));
#157538=CARTESIAN_POINT('Ctrl Pts',(-6.55340886622055,-2.49888767323347,
16.3423091472682));
#157539=CARTESIAN_POINT('Ctrl Pts',(-6.61687351925621,-2.32564007002177,
16.3339464702697));
#157540=CARTESIAN_POINT('Ctrl Pts',(-6.67341313985151,-2.15015897722873,
16.3255837932712));
#157541=CARTESIAN_POINT('Ctrl Pts',(-6.72995159639933,-1.97468149727072,
16.3172212884448));
#157542=CARTESIAN_POINT('Ctrl Pts',(-6.77956520439417,-1.79697093235842,
16.3088587836185));
#157543=CARTESIAN_POINT('Ctrl Pts',(-6.82209591187667,-1.61760128945783,
16.3004962787922));
#157544=CARTESIAN_POINT('Ctrl Pts',(-6.86463141277021,-1.4382114307537,
16.2921328314723));
#157545=CARTESIAN_POINT('Ctrl Pts',(-6.90008234631887,-1.25716244115872,
16.2837693841523));
#157546=CARTESIAN_POINT('Ctrl Pts',(-6.92834149969731,-1.07503982534234,
16.2754059368323));
#157547=CARTESIAN_POINT('Ctrl Pts',(-6.95661729285943,-0.892809970611502,
16.2670375648795));
#157548=CARTESIAN_POINT('Ctrl Pts',(-6.97769279247257,-0.709505551373533,
16.2586691929267));
#157549=CARTESIAN_POINT('Ctrl Pts',(-6.99151239034034,-0.525719562331074,
16.2503008209739));
#157550=CARTESIAN_POINT('Ctrl Pts',(-7.0053361289208,-0.341878506202975,
16.2419299416381));
#157551=CARTESIAN_POINT('Ctrl Pts',(-7.0118996113659,-0.157555920751295,
16.2335590623024));
#157552=CARTESIAN_POINT('Ctrl Pts',(-7.01119933913227,0.0266531321092605,
16.2251881829666));
#157553=CARTESIAN_POINT('Ctrl Pts',(-7.01049847356555,0.211018263308303,
16.2168102110753));
#157554=CARTESIAN_POINT('Ctrl Pts',(-7.00252156216052,0.395269340809793,
16.208432239184));
#157555=CARTESIAN_POINT('Ctrl Pts',(-6.9873172140908,0.578813192809563,
16.2000542672927));
#157556=CARTESIAN_POINT('Ctrl Pts',(-6.97765472708303,0.695456805358571,
16.1947299979337));
#157557=CARTESIAN_POINT('Ctrl Pts',(-6.9650743382028,0.811814874612261,
16.1894057285747));
#157558=CARTESIAN_POINT('Ctrl Pts',(-6.94959934240933,0.92773678513023,
16.1840814592157));
#157559=CARTESIAN_POINT('Ctrl Pts',(-6.92674601336555,1.09892917831777,
16.1762186280265));
#157560=CARTESIAN_POINT('Ctrl Pts',(-6.89752954876172,1.26952587813066,
16.1683557968372));
#157561=CARTESIAN_POINT('Ctrl Pts',(-6.86199066830943,1.43899639698447,
16.1604929656479));
#157562=CARTESIAN_POINT('Ctrl Pts',(-6.82647909479571,1.60833670011434,
16.1526361760065));
#157563=CARTESIAN_POINT('Ctrl Pts',(-6.78465484389676,1.77655217235836,
16.1447793863651));
#157564=CARTESIAN_POINT('Ctrl Pts',(-6.73661038061155,1.94311789203246,
16.1369225967237));
#157565=CARTESIAN_POINT('Ctrl Pts',(-6.68859301212934,2.10958967652546,
16.1290702379398));
#157566=CARTESIAN_POINT('Ctrl Pts',(-6.63436251462591,2.27441319399734,
16.1212178791558));
#157567=CARTESIAN_POINT('Ctrl Pts',(-6.57406228090848,2.43707441192024,
16.1133655203719));
#157568=CARTESIAN_POINT('Ctrl Pts',(-6.5137762847798,2.59969722363173,16.1055150156215));
#157569=CARTESIAN_POINT('Ctrl Pts',(-6.44742352927106,2.76015839181329,
16.097664510871));
#157570=CARTESIAN_POINT('Ctrl Pts',(-6.37519703030243,2.91795979878461,
16.0898140061206));
#157571=CARTESIAN_POINT('Ctrl Pts',(-6.30298215030111,3.07573582048299,
16.081964764269));
#157572=CARTESIAN_POINT('Ctrl Pts',(-6.22489556937921,3.23085258707242,
16.0741155224173));
#157573=CARTESIAN_POINT('Ctrl Pts',(-6.14117794584862,3.38283313214273,
16.0662662805657));
#157574=CARTESIAN_POINT('Ctrl Pts',(-6.05743211621199,3.5348648824335,16.0584143941509));
#157575=CARTESIAN_POINT('Ctrl Pts',(-5.96805163865196,3.68375796612744,
16.050562507736));
#157576=CARTESIAN_POINT('Ctrl Pts',(-5.87332261961546,3.82906097736944,
16.0427106213211));
#157577=CARTESIAN_POINT('Ctrl Pts',(-5.80376428000561,3.93575516997383,
16.0369450788572));
#157578=CARTESIAN_POINT('Ctrl Pts',(-5.73132307943551,4.04051419632107,
16.0311795363932));
#157579=CARTESIAN_POINT('Ctrl Pts',(-5.65612682125047,4.14316979430376,
16.0254139939293));
#157580=CARTESIAN_POINT('Ctrl Pts',(-5.53019890309862,4.3150826800325,16.0157586895694));
#157581=CARTESIAN_POINT('Ctrl Pts',(-5.39660821342972,4.48100845535577,
16.0061033852096));
#157582=CARTESIAN_POINT('Ctrl Pts',(-5.2559127474701,4.64036720028505,15.9964480808497));
#157583=CARTESIAN_POINT('Ctrl Pts',(-5.11443785502317,4.80060876276595,
15.986739287915));
#157584=CARTESIAN_POINT('Ctrl Pts',(-4.9657793222305,4.95421033392937,15.9770304949802));
#157585=CARTESIAN_POINT('Ctrl Pts',(-4.81053572745499,5.10062472422537,
15.9673217020455));
#157586=CARTESIAN_POINT('Ctrl Pts',(-4.65454508731951,5.24774367299968,
15.9575661895748));
#157587=CARTESIAN_POINT('Ctrl Pts',(-4.49190590489966,5.3876060916009,15.9478106771041));
#157588=CARTESIAN_POINT('Ctrl Pts',(-4.32325600339384,5.51969963780812,
15.9380551646334));
#157589=CARTESIAN_POINT('Ctrl Pts',(-4.15443911253939,5.65192397694818,
15.9282899927045));
#157590=CARTESIAN_POINT('Ctrl Pts',(-3.97959963524236,5.77636404233737,
15.9185248207756));
#157591=CARTESIAN_POINT('Ctrl Pts',(-3.79940714174909,5.89254884864996,
15.9087596488467));
#157592=CARTESIAN_POINT('Ctrl Pts',(-3.61946033663232,6.00857523961526,
15.8990077915081));
#157593=CARTESIAN_POINT('Ctrl Pts',(-3.43417513474398,6.11636884739151,
15.8892559341696));
#157594=CARTESIAN_POINT('Ctrl Pts',(-3.24424756249647,6.21550354482529,
15.879504076831));
#157595=CARTESIAN_POINT('Ctrl Pts',(-3.16142538578677,6.25873345258309,
15.8752515607683));
#157596=CARTESIAN_POINT('Ctrl Pts',(-3.07772079202939,6.30031734263474,
15.8709990447056));
#157597=CARTESIAN_POINT('Ctrl Pts',(-2.99319322076793,6.34022246499671,
15.8667465286428));
#157598=CARTESIAN_POINT('Ctrl Pts',(-2.8335197887848,6.41560364235874,15.858713483044));
#157599=CARTESIAN_POINT('Ctrl Pts',(-2.67083014928502,6.48502775193635,
15.8506804374452));
#157600=CARTESIAN_POINT('Ctrl Pts',(-2.50561624272882,6.54824509366239,
15.8426473918463));
#157601=CARTESIAN_POINT('Ctrl Pts',(-2.34050854203324,6.61142179684701,
15.8346195101985));
#157602=CARTESIAN_POINT('Ctrl Pts',(-2.17288014523112,6.66839954381638,
15.8265916285507));
#157603=CARTESIAN_POINT('Ctrl Pts',(-2.00324500790262,6.71897581487039,
15.8185637469029));
#157604=CARTESIAN_POINT('Ctrl Pts',(-1.83368646251062,6.76952925023951,
15.8105394899228));
#157605=CARTESIAN_POINT('Ctrl Pts',(-1.66212333122726,6.81368686015267,
15.8025152329427));
#157606=CARTESIAN_POINT('Ctrl Pts',(-1.48908680202622,6.85129528326807,
15.7944909759626));
#157607=CARTESIAN_POINT('Ctrl Pts',(-1.31607119470399,6.88889915914207,
15.7864676891969));
#157608=CARTESIAN_POINT('Ctrl Pts',(-1.14158290066625,6.91995534013259,
15.7784444024312));
#157609=CARTESIAN_POINT('Ctrl Pts',(-0.966165607655633,6.94436106355966,
15.7704211156655));
#157610=CARTESIAN_POINT('Ctrl Pts',(-0.790762688527433,6.96876478715539,
15.7623984863365));
#157611=CARTESIAN_POINT('Ctrl Pts',(-0.614431285757129,6.98651909212234,
15.7543758570076));
#157612=CARTESIAN_POINT('Ctrl Pts',(-0.437722255297477,6.99757284990427,
15.7463532276787));
#157613=CARTESIAN_POINT('Ctrl Pts',(-0.260946794822806,7.00863076311217,
15.7383275824123));
#157614=CARTESIAN_POINT('Ctrl Pts',(-0.0837937893559116,7.01298307725086,
15.7303019371459));
#157615=CARTESIAN_POINT('Ctrl Pts',(0.0931834548376472,7.01063074239719,
15.7222762918795));
#157616=CARTESIAN_POINT('Ctrl Pts',(0.197540022473344,7.00924366242327,
15.7175438823718));
#157617=CARTESIAN_POINT('Ctrl Pts',(0.301835470615949,7.00552636419604,
15.7128114728641));
#157618=CARTESIAN_POINT('Ctrl Pts',(0.405956845365878,6.99948752425494,
15.7080790633564));
#157619=CARTESIAN_POINT('Ctrl Pts',(0.598033352021251,6.98834745543698,
15.6993490145218));
#157620=CARTESIAN_POINT('Ctrl Pts',(0.789613284952843,6.96929894113871,
15.6906189656871));
#157621=CARTESIAN_POINT('Ctrl Pts',(0.980053679305924,6.94241466265009,
15.6818889168525));
#157622=CARTESIAN_POINT('Ctrl Pts',(1.17054913973635,6.91552261053884,15.6731563437134));
#157623=CARTESIAN_POINT('Ctrl Pts',(1.35990413263774,6.88079031002813,15.6644237705742));
#157624=CARTESIAN_POINT('Ctrl Pts',(1.54748375457549,6.83834194756484,15.6556911974351));
#157625=CARTESIAN_POINT('Ctrl Pts',(1.73772824447685,6.79529053835231,15.6468345641546));
#157626=CARTESIAN_POINT('Ctrl Pts',(1.92614625230624,6.74430222229125,15.6379779308742));
#157627=CARTESIAN_POINT('Ctrl Pts',(2.11208871266556,6.68555964989699,15.6291212975938));
#157628=CARTESIAN_POINT('Ctrl Pts',(2.29554327507376,6.62760304927713,15.6203831654871));
#157629=CARTESIAN_POINT('Ctrl Pts',(2.4765878660588,6.56209851231269,15.6116450333804));
#157630=CARTESIAN_POINT('Ctrl Pts',(2.65461586619075,6.48927123531359,15.6029069012736));
#157631=CARTESIAN_POINT('Ctrl Pts',(2.83626532569898,6.41496250020148,15.5939910174064));
#157632=CARTESIAN_POINT('Ctrl Pts',(3.01477387672386,6.33303002306115,15.5850751335391));
#157633=CARTESIAN_POINT('Ctrl Pts',(3.18951910498039,6.24376444474526,15.5761592496718));
#157634=CARTESIAN_POINT('Ctrl Pts',(3.36426433323694,6.15449886642937,15.5672433658046));
#157635=CARTESIAN_POINT('Ctrl Pts',(3.53524597218369,6.05790032992673,15.5583274819373));
#157636=CARTESIAN_POINT('Ctrl Pts',(3.70186786591409,5.95430943651845,15.54941159807));
#157637=CARTESIAN_POINT('Ctrl Pts',(3.86521559732732,5.85275413034307,15.5406709135738));
#157638=CARTESIAN_POINT('Ctrl Pts',(4.02439068243854,5.74446793341385,15.5319302290776));
#157639=CARTESIAN_POINT('Ctrl Pts',(4.17885650916467,5.62981214946929,15.5231895445813));
#157640=CARTESIAN_POINT('Ctrl Pts',(4.33329454492248,5.51517699400501,15.5144504326795));
#157641=CARTESIAN_POINT('Ctrl Pts',(4.48302479459601,5.39417470329297,15.5057113207776));
#157642=CARTESIAN_POINT('Ctrl Pts',(4.62754150307941,5.2672085775843,15.4969722088757));
#157643=CARTESIAN_POINT('Ctrl Pts',(4.77393063351689,5.13859742298107,15.4881198692014));
#157644=CARTESIAN_POINT('Ctrl Pts',(4.91496995418404,5.00386698717785,15.479267529527));
#157645=CARTESIAN_POINT('Ctrl Pts',(5.05016918409218,4.86347795045333,15.4704151898527));
#157646=CARTESIAN_POINT('Ctrl Pts',(5.18357070857305,4.72495562653051,15.4616805572029));
#157647=CARTESIAN_POINT('Ctrl Pts',(5.31128630095293,4.58092446076588,15.4529459245531));
#157648=CARTESIAN_POINT('Ctrl Pts',(5.43288204854389,4.43186407836585,15.4442112919034));
#157649=CARTESIAN_POINT('Ctrl Pts',(5.55693571409598,4.27979061205085,15.4353000987167));
#157650=CARTESIAN_POINT('Ctrl Pts',(5.67461928824829,4.1224826553152,15.4263889055301));
#157651=CARTESIAN_POINT('Ctrl Pts',(5.78551457111583,3.96048579216066,15.4174777123435));
#157652=CARTESIAN_POINT('Ctrl Pts',(5.89640985398337,3.79848892900611,15.4085665191568));
#157653=CARTESIAN_POINT('Ctrl Pts',(6.00051666321702,3.63180340195692,15.3996553259702));
#157654=CARTESIAN_POINT('Ctrl Pts',(6.09746263884185,3.46100793562047,15.3907441327836));
#157655=CARTESIAN_POINT('Ctrl Pts',(6.18477556157925,3.30718358901897,15.3827184017805));
#157656=CARTESIAN_POINT('Ctrl Pts',(6.26631969761614,3.1499545437622,15.3746926707773));
#157657=CARTESIAN_POINT('Ctrl Pts',(6.34182249675829,2.98980166267102,15.3666669397742));
#157658=CARTESIAN_POINT('Ctrl Pts',(6.41729889345471,2.82970478516913,15.3586440152753));
#157659=CARTESIAN_POINT('Ctrl Pts',(6.4867380049896,2.66668643947756,15.3506210907764));
#157660=CARTESIAN_POINT('Ctrl Pts',(6.54991363018798,2.50125128677182,15.3425981662775));
#157661=CARTESIAN_POINT('Ctrl Pts',(6.55705890610752,2.48254027585327,15.3416907592033));
#157662=CARTESIAN_POINT('Ctrl Pts',(6.56412410946124,2.46379837162001,15.340783352129));
#157663=CARTESIAN_POINT('Ctrl Pts',(6.57110895151815,2.44502632087634,15.3398759450547));
#157664=CARTESIAN_POINT('Origin',(0.,0.,50.));
#157665=CARTESIAN_POINT('',(6.57110895151813,2.44502632087639,13.3398632123397));
#157666=CARTESIAN_POINT('',(6.57110895151813,2.44502632087639,13.8866662636617));
#157667=CARTESIAN_POINT('',(6.57110895151814,2.44502632087636,50.));
#157668=CARTESIAN_POINT('',(7.01124847424792,0.00462545740675339,15.7735343569468));
#157669=CARTESIAN_POINT('Ctrl Pts',(6.57110895151813,2.44502632087638,13.8866662636617));
#157670=CARTESIAN_POINT('Ctrl Pts',(6.50682343305336,2.61779629976374,13.8950331353048));
#157671=CARTESIAN_POINT('Ctrl Pts',(6.43577420808727,2.78788399297637,13.9034000069479));
#157672=CARTESIAN_POINT('Ctrl Pts',(6.35822606708258,2.95475681611392,13.911766878591));
#157673=CARTESIAN_POINT('Ctrl Pts',(6.28054885164576,3.12190738949285,13.920147676412));
#157674=CARTESIAN_POINT('Ctrl Pts',(6.19635124690865,3.28583210487158,13.928528474233));
#157675=CARTESIAN_POINT('Ctrl Pts',(6.10594367300422,3.44602356704067,13.936909272054));
#157676=CARTESIAN_POINT('Ctrl Pts',(6.04363046942621,3.55643514831101,13.9426857168607));
#157677=CARTESIAN_POINT('Ctrl Pts',(5.97836806944462,3.66507378318171,13.9484621616674));
#157678=CARTESIAN_POINT('Ctrl Pts',(5.91026961679952,3.77178202170227,13.9542386064741));
#157679=CARTESIAN_POINT('Ctrl Pts',(5.81136169478537,3.92676777723572,13.9626284616069));
#157680=CARTESIAN_POINT('Ctrl Pts',(5.70626946418082,4.07799285774942,13.9710183167397));
#157681=CARTESIAN_POINT('Ctrl Pts',(5.5953027819797,4.22495128261501,13.9794081718725));
#157682=CARTESIAN_POINT('Ctrl Pts',(5.48443849827716,4.3717740963065,13.9877902849646));
#157683=CARTESIAN_POINT('Ctrl Pts',(5.36771076659184,4.51433784210089,13.9961723980567));
#157684=CARTESIAN_POINT('Ctrl Pts',(5.24547289992488,4.65216515384543,14.0045545111488));
#157685=CARTESIAN_POINT('Ctrl Pts',(5.12332986393521,4.78988554080735,14.0129301214977));
#157686=CARTESIAN_POINT('Ctrl Pts',(4.99568543274421,4.92287657443647,14.0213057318465));
#157687=CARTESIAN_POINT('Ctrl Pts',(4.86293366035222,5.05069329671812,14.0296813421954));
#157688=CARTESIAN_POINT('Ctrl Pts',(4.73026539079616,5.17842962038364,14.038051684161));
#157689=CARTESIAN_POINT('Ctrl Pts',(4.59249642185694,5.30099789490473,14.0464220261266));
#157690=CARTESIAN_POINT('Ctrl Pts',(4.4500585001271,5.41798910186672,14.0547923680922));
#157691=CARTESIAN_POINT('Ctrl Pts',(4.30768929416612,5.53492386921882,14.0631586719865));
#157692=CARTESIAN_POINT('Ctrl Pts',(4.16065588068454,5.64628672608035,14.0715249758808));
#157693=CARTESIAN_POINT('Ctrl Pts',(4.0094243424729,5.75170783372085,14.0798912797751));
#157694=CARTESIAN_POINT('Ctrl Pts',(3.85823509948301,5.85709945803282,14.0882552438488));
#157695=CARTESIAN_POINT('Ctrl Pts',(3.70285034144664,5.95655245764888,14.0966192079224));
#157696=CARTESIAN_POINT('Ctrl Pts',(3.54376693566202,6.04973904133134,14.104983171996));
#157697=CARTESIAN_POINT('Ctrl Pts',(3.38470801016987,6.14291128514716,14.1133458489946));
#157698=CARTESIAN_POINT('Ctrl Pts',(3.22195185522551,6.2298188695767,14.1217085259932));
#157699=CARTESIAN_POINT('Ctrl Pts',(3.05602221401651,6.31017866545296,14.1300712029917));
#157700=CARTESIAN_POINT('Ctrl Pts',(2.89009598899557,6.39053680686788,14.138433707818));
#157701=CARTESIAN_POINT('Ctrl Pts',(2.72099670395211,6.46434728564727,14.1467962126444));
#157702=CARTESIAN_POINT('Ctrl Pts',(2.54927085689975,6.53137387236879,14.1551587174707));
#157703=CARTESIAN_POINT('Ctrl Pts',(2.37752565553506,6.59840801330253,14.1635221647907));
#157704=CARTESIAN_POINT('Ctrl Pts',(2.20315360830886,6.65865661884118,14.1718856121108));
#157705=CARTESIAN_POINT('Ctrl Pts',(2.02671965925461,6.71193220952736,14.1802490594308));
#157706=CARTESIAN_POINT('Ctrl Pts',(1.85018182093351,6.76523917037834,14.1886174313836));
#157707=CARTESIAN_POINT('Ctrl Pts',(1.6715799693897,6.81156481577389,14.1969858033364));
#157708=CARTESIAN_POINT('Ctrl Pts',(1.49149363213397,6.8507717308201,14.2053541752893));
#157709=CARTESIAN_POINT('Ctrl Pts',(1.31135333630524,6.88999039328269,14.213725054625));
#157710=CARTESIAN_POINT('Ctrl Pts',(1.12972799018647,6.92208600757216,14.2220959339608));
#157711=CARTESIAN_POINT('Ctrl Pts',(0.947206404613266,6.94697247652239,
14.2304668132965));
#157712=CARTESIAN_POINT('Ctrl Pts',(0.764530170474379,6.97188003150865,
14.2388447851878));
#157713=CARTESIAN_POINT('Ctrl Pts',(0.58095650614245,6.98956619671621,14.2472227570791));
#157714=CARTESIAN_POINT('Ctrl Pts',(0.397079586526947,6.99999674031807,
14.2556007289704));
#157715=CARTESIAN_POINT('Ctrl Pts',(0.280224306798269,7.00662543571315,
14.2609249983293));
#157716=CARTESIAN_POINT('Ctrl Pts',(0.163246613133867,7.01032484772516,
14.2662492676882));
#157717=CARTESIAN_POINT('Ctrl Pts',(0.0462988965612011,7.01109713059784,
14.2715735370471));
#157718=CARTESIAN_POINT('Ctrl Pts',(-0.126408397416553,7.01223763072076,
14.2794363682364));
#157719=CARTESIAN_POINT('Ctrl Pts',(-0.299409378148574,7.0069939243274,
14.2872991994256));
#157720=CARTESIAN_POINT('Ctrl Pts',(-0.472173043189139,6.99533267113048,
14.2951620306149));
#157721=CARTESIAN_POINT('Ctrl Pts',(-0.644803962157695,6.98368037806738,
14.3030188202563));
#157722=CARTESIAN_POINT('Ctrl Pts',(-0.817197550108498,6.96562036978901,
14.3108756098977));
#157723=CARTESIAN_POINT('Ctrl Pts',(-0.98882113102714,6.94117132286289,
14.3187323995391));
#157724=CARTESIAN_POINT('Ctrl Pts',(-1.16034792437023,6.91673606404191,
14.326584758323));
#157725=CARTESIAN_POINT('Ctrl Pts',(-1.33110519821472,6.88591898759986,
14.334437117107));
#157726=CARTESIAN_POINT('Ctrl Pts',(-1.50056398817736,6.84879071660722,
14.3422894758909));
#157727=CARTESIAN_POINT('Ctrl Pts',(-1.66998276694233,6.81167121203261,
14.3501399806413));
#157728=CARTESIAN_POINT('Ctrl Pts',(-1.83810329811438,6.76824355199754,
14.3579904853917));
#157729=CARTESIAN_POINT('Ctrl Pts',(-2.00440548711609,6.71862971190696,
14.3658409901422));
#157730=CARTESIAN_POINT('Ctrl Pts',(-2.17068092333709,6.66902385311951,
14.3736902319938));
#157731=CARTESIAN_POINT('Ctrl Pts',(-2.33513823495106,6.6132339073058,14.3815394738454));
#157732=CARTESIAN_POINT('Ctrl Pts',(-2.49727165792624,6.5514319678234,14.389388715697));
#157733=CARTESIAN_POINT('Ctrl Pts',(-2.65945970682528,6.48960920605785,
14.3972406021119));
#157734=CARTESIAN_POINT('Ctrl Pts',(-2.81932194634441,6.42177054070639,
14.4050924885267));
#157735=CARTESIAN_POINT('Ctrl Pts',(-2.97637161426586,6.34813662237136,
14.4129443749416));
#157736=CARTESIAN_POINT('Ctrl Pts',(-3.09169123066252,6.29406815264098,
14.4187099174055));
#157737=CARTESIAN_POINT('Ctrl Pts',(-3.20549475449589,6.23687602814435,
14.4244754598695));
#157738=CARTESIAN_POINT('Ctrl Pts',(-3.31759780661679,6.17666344849964,
14.4302410023335));
#157739=CARTESIAN_POINT('Ctrl Pts',(-3.50533193478854,6.07582804811839,
14.4398963066934));
#157740=CARTESIAN_POINT('Ctrl Pts',(-3.68820103973575,5.9665727244977,14.4495516110534));
#157741=CARTESIAN_POINT('Ctrl Pts',(-3.86555333472591,5.84936953687228,
14.4592069154133));
#157742=CARTESIAN_POINT('Ctrl Pts',(-4.0438881281576,5.73151706557566,14.468915708348));
#157743=CARTESIAN_POINT('Ctrl Pts',(-4.21664480894793,5.60562849866783,
14.4786245012827));
#157744=CARTESIAN_POINT('Ctrl Pts',(-4.38319836816824,5.47222063040109,
14.4883332942174));
#157745=CARTESIAN_POINT('Ctrl Pts',(-4.55055339725869,5.3381707921437,14.4980888066882));
#157746=CARTESIAN_POINT('Ctrl Pts',(-4.71164544247583,5.1965291571514,14.5078443191589));
#157747=CARTESIAN_POINT('Ctrl Pts',(-4.86587855491735,5.04785622331852,
14.5175998316297));
#157748=CARTESIAN_POINT('Ctrl Pts',(-5.02026438186789,4.89903608040883,
14.5273650035586));
#157749=CARTESIAN_POINT('Ctrl Pts',(-5.16777767184748,4.743170747589,14.5371301754875));
#157750=CARTESIAN_POINT('Ctrl Pts',(-5.30785902364905,4.5808579051928,14.5468953474164));
#157751=CARTESIAN_POINT('Ctrl Pts',(-5.447749377705,4.41876637267536,14.5566472047549));
#157752=CARTESIAN_POINT('Ctrl Pts',(-5.58022802160503,4.25024492945157,
14.5663990620934));
#157753=CARTESIAN_POINT('Ctrl Pts',(-5.70477630390394,4.07592368487391,
14.5761509194319));
#157754=CARTESIAN_POINT('Ctrl Pts',(-5.75908837520181,3.99990699729316,
14.5804034354945));
#157755=CARTESIAN_POINT('Ctrl Pts',(-5.8118929119634,3.9227878698017,14.5846559515572));
#157756=CARTESIAN_POINT('Ctrl Pts',(-5.86314922750659,3.84462061827808,
14.5889084676199));
#157757=CARTESIAN_POINT('Ctrl Pts',(-5.95997292291815,3.69696189422669,
14.5969415132187));
#157758=CARTESIAN_POINT('Ctrl Pts',(-6.05131610743908,3.54548896452417,
14.6049745588175));
#157759=CARTESIAN_POINT('Ctrl Pts',(-6.1368631875334,3.39065432918153,14.6130076044163));
#157760=CARTESIAN_POINT('Ctrl Pts',(-6.22235527467099,3.23591922750376,
14.6210354860642));
#157761=CARTESIAN_POINT('Ctrl Pts',(-6.30205849745976,3.07782704129155,
14.629063367712));
#157762=CARTESIAN_POINT('Ctrl Pts',(-6.37570092852195,2.9168586240242,14.6370912493598));
#157763=CARTESIAN_POINT('Ctrl Pts',(-6.44931010930046,2.75596288558427,
14.6451155063399));
#157764=CARTESIAN_POINT('Ctrl Pts',(-6.51686379486667,2.59219383449292,
14.65313976332));
#157765=CARTESIAN_POINT('Ctrl Pts',(-6.57813634697585,2.42605621598001,
14.6611640203001));
#157766=CARTESIAN_POINT('Ctrl Pts',(-6.63940149060938,2.2599386851974,14.6691873070659));
#157767=CARTESIAN_POINT('Ctrl Pts',(-6.69438687948556,2.09145349847771,
14.6772105938316));
#157768=CARTESIAN_POINT('Ctrl Pts',(-6.74291524803168,1.9211248060347,14.6852338805973));
#157769=CARTESIAN_POINT('Ctrl Pts',(-6.79143964011083,1.75081007050885,
14.6932565099262));
#157770=CARTESIAN_POINT('Ctrl Pts',(-6.83350796916813,1.57865248386803,
14.7012791392551));
#157771=CARTESIAN_POINT('Ctrl Pts',(-6.86899310809289,1.40519046519408,
14.709301768584));
#157772=CARTESIAN_POINT('Ctrl Pts',(-6.90449158690372,1.2316632371498,14.7173274138504));
#157773=CARTESIAN_POINT('Ctrl Pts',(-6.93340186115936,1.05683095744479,
14.7253530591169));
#157774=CARTESIAN_POINT('Ctrl Pts',(-6.95564803755869,0.881241703567202,
14.7333787043833));
#157775=CARTESIAN_POINT('Ctrl Pts',(-6.96876573877862,0.777703579601446,
14.738111113891));
#157776=CARTESIAN_POINT('Ctrl Pts',(-6.97956731078757,0.673902400168856,
14.7428435233987));
#157777=CARTESIAN_POINT('Ctrl Pts',(-6.98804566086226,0.56995122967162,
14.7475759329064));
#157778=CARTESIAN_POINT('Ctrl Pts',(-7.00368598321158,0.37818870502436,
14.756305981741));
#157779=CARTESIAN_POINT('Ctrl Pts',(-7.01142552498665,0.185819746789846,
14.7650360305757));
#157780=CARTESIAN_POINT('Ctrl Pts',(-7.01124697880516,-0.00650881674804643,
14.7737660794103));
#157781=CARTESIAN_POINT('Ctrl Pts',(-7.01106838099683,-0.198892992329736,
14.7824986525495));
#157782=CARTESIAN_POINT('Ctrl Pts',(-7.00296712547059,-0.39123647595842,
14.7912312256886));
#157783=CARTESIAN_POINT('Ctrl Pts',(-6.98697803043219,-0.582893270468943,
14.7999637988278));
#157784=CARTESIAN_POINT('Ctrl Pts',(-6.97076178477534,-0.777272855687614,
14.8088204321082));
#157785=CARTESIAN_POINT('Ctrl Pts',(-6.94643189688725,-0.970945803216331,
14.8176770653886));
#157786=CARTESIAN_POINT('Ctrl Pts',(-6.91407911602979,-1.1632439725959,
14.826533698669));
#157787=CARTESIAN_POINT('Ctrl Pts',(-6.88215921326288,-1.35296920505414,
14.8352718307758));
#157788=CARTESIAN_POINT('Ctrl Pts',(-6.84242984471826,-1.54135594971283,
14.8440099628825));
#157789=CARTESIAN_POINT('Ctrl Pts',(-6.79502978745293,-1.72777219277527,
14.8527480949893));
#157790=CARTESIAN_POINT('Ctrl Pts',(-6.74666551454929,-1.91798052950098,
14.8616639788565));
#157791=CARTESIAN_POINT('Ctrl Pts',(-6.69031520397961,-2.10613704971201,
14.8705798627238));
#157792=CARTESIAN_POINT('Ctrl Pts',(-6.62618024995159,-2.2915850099116,
14.879495746591));
#157793=CARTESIAN_POINT('Ctrl Pts',(-6.56204529592356,-2.4770329701112,
14.8884116304583));
#157794=CARTESIAN_POINT('Ctrl Pts',(-6.49012580302771,-2.65977208648433,
14.8973275143255));
#157795=CARTESIAN_POINT('Ctrl Pts',(-6.41067628819488,-2.83916468181681,
14.9062433981928));
#157796=CARTESIAN_POINT('Ctrl Pts',(-6.33278797640538,-3.01503216731855,
14.914984082689));
#157797=CARTESIAN_POINT('Ctrl Pts',(-6.24765455686902,-3.18770210982015,
14.9237247671852));
#157798=CARTESIAN_POINT('Ctrl Pts',(-6.15555931687582,-3.35659292421994,
14.9324654516814));
#157799=CARTESIAN_POINT('Ctrl Pts',(-6.06348064634596,-3.525453352357,14.9412045635833));
#157800=CARTESIAN_POINT('Ctrl Pts',(-5.96444278782203,-3.69053576996705,
14.9499436754852));
#157801=CARTESIAN_POINT('Ctrl Pts',(-5.85877490313842,-3.85128331817531,
14.9586827873871));
#157802=CARTESIAN_POINT('Ctrl Pts',(-5.75173793892643,-4.01411358222622,
14.9675351270615));
#157803=CARTESIAN_POINT('Ctrl Pts',(-5.63789808562857,-4.17249561437347,
14.9763874667358));
#157804=CARTESIAN_POINT('Ctrl Pts',(-5.51764347797401,-4.32587991193363,
14.9852398064101));
#157805=CARTESIAN_POINT('Ctrl Pts',(-5.39898786138609,-4.47722470243168,
14.9939744390599));
#157806=CARTESIAN_POINT('Ctrl Pts',(-5.27408720562648,-4.62370362732956,
15.0027090717097));
#157807=CARTESIAN_POINT('Ctrl Pts',(-5.14335623431666,-4.76482037535686,
15.0114437043594));
#157808=CARTESIAN_POINT('Ctrl Pts',(-5.0099826870218,-4.90878963588132,
15.0203548975461));
#157809=CARTESIAN_POINT('Ctrl Pts',(-4.87054078900852,-5.04717740252297,
15.0292660907327));
#157810=CARTESIAN_POINT('Ctrl Pts',(-4.72551276559025,-5.17949376529634,
15.0381772839193));
#157811=CARTESIAN_POINT('Ctrl Pts',(-4.58048474217196,-5.31181012806972,
15.0470884771059));
#157812=CARTESIAN_POINT('Ctrl Pts',(-4.42987080820157,-5.43805487271456,
15.0559996702926));
#157813=CARTESIAN_POINT('Ctrl Pts',(-4.27419237401628,-5.55777888300723,
15.0649108634792));
#157814=CARTESIAN_POINT('Ctrl Pts',(-4.1339841088214,-5.66560560848246,
15.0729365283316));
#157815=CARTESIAN_POINT('Ctrl Pts',(-3.98960312497885,-5.76819231375616,
15.0809621931839));
#157816=CARTESIAN_POINT('Ctrl Pts',(-3.84148776815999,-5.86520232298743,
15.0889878580363));
#157817=CARTESIAN_POINT('Ctrl Pts',(-3.69341941952229,-5.96218154362132,
15.0970109757395));
#157818=CARTESIAN_POINT('Ctrl Pts',(-3.54161936381376,-6.05358739132405,
15.1050340934427));
#157819=CARTESIAN_POINT('Ctrl Pts',(-3.38655599559884,-6.13912575625989,
15.1130572111459));
#157820=CARTESIAN_POINT('Ctrl Pts',(-3.23151218223137,-6.2246533340595,
15.1210793170638));
#157821=CARTESIAN_POINT('Ctrl Pts',(-3.07320619725014,-6.30431472647784,
15.1291014229817));
#157822=CARTESIAN_POINT('Ctrl Pts',(-2.91213211645322,-6.37786116961021,
15.1371235288995));
#157823=CARTESIAN_POINT('Ctrl Pts',(-2.75099817998405,-6.45143494284916,
15.145148615859));
#157824=CARTESIAN_POINT('Ctrl Pts',(-2.58709442533485,-6.51888907226617,
15.1531737028186));
#157825=CARTESIAN_POINT('Ctrl Pts',(-2.42093645748432,-6.58002228197772,
15.1611987897781));
#157826=CARTESIAN_POINT('Ctrl Pts',(-2.25474576565336,-6.64116753156906,
15.1692254572383));
#157827=CARTESIAN_POINT('Ctrl Pts',(-2.08630032324651,-6.69598926315759,
15.1772521246985));
#157828=CARTESIAN_POINT('Ctrl Pts',(-1.91613187089708,-6.74433578759484,
15.1852787921588));
#157829=CARTESIAN_POINT('Ctrl Pts',(-1.74582680791346,-6.79272112445162,
15.1933119033994));
#157830=CARTESIAN_POINT('Ctrl Pts',(-1.57379632742428,-6.83462078068159,
15.20134501464));
#157831=CARTESIAN_POINT('Ctrl Pts',(-1.40058397055772,-6.86993385003937,
15.2093781258806));
#157832=CARTESIAN_POINT('Ctrl Pts',(-1.29852095760964,-6.89074159332224,
15.2141115268423));
#157833=CARTESIAN_POINT('Ctrl Pts',(-1.19604776992183,-6.90926345064929,
15.2188449278039));
#157834=CARTESIAN_POINT('Ctrl Pts',(-1.09327653932694,-6.92548720098863,
15.2235783287656));
#157835=CARTESIAN_POINT('Ctrl Pts',(-0.881564605849781,-6.95890863160409,
15.2333292820597));
#157836=CARTESIAN_POINT('Ctrl Pts',(-0.668462914413408,-6.98259511557152,
15.2430802353539));
#157837=CARTESIAN_POINT('Ctrl Pts',(-0.454786202923141,-6.99648455098207,
15.2528311886481));
#157838=CARTESIAN_POINT('Ctrl Pts',(-0.240801650048419,-7.01039399672971,
15.2625961900196));
#157839=CARTESIAN_POINT('Ctrl Pts',(-0.0262404585796727,-7.01447815828849,
15.2723611913911));
#157840=CARTESIAN_POINT('Ctrl Pts',(0.188078825273883,-7.00872691135727,
15.2821261927625));
#157841=CARTESIAN_POINT('Ctrl Pts',(0.402040883290473,-7.00298525056296,
15.2918749179002));
#157842=CARTESIAN_POINT('Ctrl Pts',(0.615761801649108,-6.98744094642008,
15.3016236430378));
#157843=CARTESIAN_POINT('Ctrl Pts',(0.828427412422822,-6.96213577753597,
15.3113723681754));
#157844=CARTESIAN_POINT('Ctrl Pts',(1.04050933855961,-6.93690006152796,
15.3210943368427));
#157845=CARTESIAN_POINT('Ctrl Pts',(1.25154169966688,-6.90195696693144,
15.33081630551));
#157846=CARTESIAN_POINT('Ctrl Pts',(1.46071789640201,-6.85739963759084,
15.3405382741774));
#157847=CARTESIAN_POINT('Ctrl Pts',(1.66851002887363,-6.81313713246149,
15.3501959151171));
#157848=CARTESIAN_POINT('Ctrl Pts',(1.87447042763027,-6.75938718329948,
15.3598535560568));
#157849=CARTESIAN_POINT('Ctrl Pts',(2.07780996499439,-6.69629243028334,
15.3695111969966));
#157850=CARTESIAN_POINT('Ctrl Pts',(2.16718469221616,-6.66856011411384,
15.3737560626818));
#157851=CARTESIAN_POINT('Ctrl Pts',(2.25605311893811,-6.63902314187182,
15.3780009283669));
#157852=CARTESIAN_POINT('Ctrl Pts',(2.34434837785144,-6.60769681854164,
15.3822457940521));
#157853=CARTESIAN_POINT('Ctrl Pts',(2.50767059260672,-6.5497516404042,15.390097641066));
#157854=CARTESIAN_POINT('Ctrl Pts',(2.66896336522462,-6.48570442701368,
15.3979494880799));
#157855=CARTESIAN_POINT('Ctrl Pts',(2.82772286466298,-6.41573144412718,
15.4058013350938));
#157856=CARTESIAN_POINT('Ctrl Pts',(2.9864373411913,-6.3457783050127,15.4136509553874));
#157857=CARTESIAN_POINT('Ctrl Pts',(3.14261962487296,-6.26990289290201,
15.421500575681));
#157858=CARTESIAN_POINT('Ctrl Pts',(3.2957851434009,-6.18832989190443,15.4293501959745));
#157859=CARTESIAN_POINT('Ctrl Pts',(3.44893843362136,-6.10676340346756,
15.4371991895764));
#157860=CARTESIAN_POINT('Ctrl Pts',(3.59907510181574,-6.01950041166084,
15.4450481831782));
#157861=CARTESIAN_POINT('Ctrl Pts',(3.74573473808917,-5.9268117765264,15.45289717678));
#157862=CARTESIAN_POINT('Ctrl Pts',(3.89246862384126,-5.83407621585055,
15.4607501440974));
#157863=CARTESIAN_POINT('Ctrl Pts',(4.03572163758295,-5.7359097275759,15.4686031114148));
#157864=CARTESIAN_POINT('Ctrl Pts',(4.17506168013776,-5.63262696523969,
15.4764560787322));
#157865=CARTESIAN_POINT('Ctrl Pts',(4.31443711038153,-5.52931797255217,
15.4843110404394));
#157866=CARTESIAN_POINT('Ctrl Pts',(4.44989729178476,-5.42089035557746,
15.4921660021467));
#157867=CARTESIAN_POINT('Ctrl Pts',(4.581043381571,-5.30769894574519,15.5000209638539));
#157868=CARTESIAN_POINT('Ctrl Pts',(4.71231964481388,-5.19439518397696,
15.5078837222672));
#157869=CARTESIAN_POINT('Ctrl Pts',(4.83927298479952,-5.07631844508788,
15.5157464806806));
#157870=CARTESIAN_POINT('Ctrl Pts',(4.96154118034644,-4.95386068417618,
15.5236092390939));
#157871=CARTESIAN_POINT('Ctrl Pts',(5.05123537415605,-4.86402742793507,
15.5293772458421));
#157872=CARTESIAN_POINT('Ctrl Pts',(5.1384090411959,-4.77183730484334,15.5351452525903));
#157873=CARTESIAN_POINT('Ctrl Pts',(5.22293326955531,-4.67745599918079,
15.5409132593385));
#157874=CARTESIAN_POINT('Ctrl Pts',(5.3449247988286,-4.54123801723568,15.5492380672394));
#157875=CARTESIAN_POINT('Ctrl Pts',(5.46167769980065,-4.40014018445398,
15.5575628751404));
#157876=CARTESIAN_POINT('Ctrl Pts',(5.5727950877626,-4.25459533590553,15.5658876830414));
#157877=CARTESIAN_POINT('Ctrl Pts',(5.68827901390729,-4.10333106621026,
15.5745396277859));
#157878=CARTESIAN_POINT('Ctrl Pts',(5.79767526457732,-3.94726343442159,
15.5831915725305));
#157879=CARTESIAN_POINT('Ctrl Pts',(5.90058275068057,-3.78691824111254,
15.591843517275));
#157880=CARTESIAN_POINT('Ctrl Pts',(5.99945449149194,-3.63286134016663,
15.6001561568185));
#157881=CARTESIAN_POINT('Ctrl Pts',(6.09233650382568,-3.4748563019137,15.6084687963619));
#157882=CARTESIAN_POINT('Ctrl Pts',(6.17891585027054,-3.31340089300639,
15.6167814359053));
#157883=CARTESIAN_POINT('Ctrl Pts',(6.2654621520297,-3.15200710668529,15.6250909027688));
#157884=CARTESIAN_POINT('Ctrl Pts',(6.34571042458889,-2.98716586962572,
15.6334003696322));
#157885=CARTESIAN_POINT('Ctrl Pts',(6.41939286279622,-2.81940097105413,
15.6417098364956));
#157886=CARTESIAN_POINT('Ctrl Pts',(6.49305797317401,-2.65167552559558,
15.6500173492296));
#157887=CARTESIAN_POINT('Ctrl Pts',(6.5601601930512,-2.48102809613213,15.6583248619635));
#157888=CARTESIAN_POINT('Ctrl Pts',(6.62047905083359,-2.30800426775462,
15.6666323746975));
#157889=CARTESIAN_POINT('Ctrl Pts',(6.68079255755789,-2.13499578881493,
15.6749391504482));
#157890=CARTESIAN_POINT('Ctrl Pts',(6.73432379269518,-1.95961164803175,
15.683245926199));
#157891=CARTESIAN_POINT('Ctrl Pts',(6.78090141494034,-1.78241481237116,
15.6915527019498));
#157892=CARTESIAN_POINT('Ctrl Pts',(6.82749179049423,-1.60516945886351,
15.6998617521592));
#157893=CARTESIAN_POINT('Ctrl Pts',(6.86712466197352,-1.42611074264509,
15.7081708023686));
#157894=CARTESIAN_POINT('Ctrl Pts',(6.89967912188337,-1.2458148247419,15.716479852578));
#157895=CARTESIAN_POINT('Ctrl Pts',(6.93223858515478,-1.06549119679023,
15.7247901798224));
#157896=CARTESIAN_POINT('Ctrl Pts',(6.95771741333767,-0.883930318812309,
15.7331005070667));
#157897=CARTESIAN_POINT('Ctrl Pts',(6.97604620325943,-0.701716418854346,
15.7414108343111));
#157898=CARTESIAN_POINT('Ctrl Pts',(6.99438495527861,-0.519403481664143,
15.7497256783997));
#157899=CARTESIAN_POINT('Ctrl Pts',(7.00556587828336,-0.336437147572331,
15.7580405224883));
#157900=CARTESIAN_POINT('Ctrl Pts',(7.00957155226553,-0.15340539811163,
15.7663553665769));
#157901=CARTESIAN_POINT('Ctrl Pts',(7.01072437784235,-0.100729198529165,
15.7687483633547));
#157902=CARTESIAN_POINT('Ctrl Pts',(7.01128322367289,-0.0480475808299134,
15.7711413601326));
#157903=CARTESIAN_POINT('Ctrl Pts',(7.01124847424845,0.00462545660806772,
15.7735343569105));
#157904=CARTESIAN_POINT('Ctrl Pts',(7.01124847424792,0.00462545740675822,
15.7735343569468));
#157905=CARTESIAN_POINT('Ctrl Pts',(7.01109761289101,0.233300454373922,
15.7839233255262));
#157906=CARTESIAN_POINT('Ctrl Pts',(6.999755421247,0.461583810249137,15.7943122941056));
#157907=CARTESIAN_POINT('Ctrl Pts',(6.97735941040693,0.688536288445155,
15.804701262685));
#157908=CARTESIAN_POINT('Ctrl Pts',(6.95466206942866,0.918542329264845,
15.8152300110386));
#157909=CARTESIAN_POINT('Ctrl Pts',(6.9206114557263,1.14718165363006,15.8257587593922));
#157910=CARTESIAN_POINT('Ctrl Pts',(6.87540077452587,1.3734958143908,15.8362875077458));
#157911=CARTESIAN_POINT('Ctrl Pts',(6.84396755419799,1.5308432086266,15.8436077351343));
#157912=CARTESIAN_POINT('Ctrl Pts',(6.80714072868335,1.68706705157194,15.8509279625228));
#157913=CARTESIAN_POINT('Ctrl Pts',(6.76499934449847,1.84184973095942,15.8582481899113));
#157914=CARTESIAN_POINT('Ctrl Pts',(6.71673751112402,2.01911243901562,15.8666315783861));
#157915=CARTESIAN_POINT('Ctrl Pts',(6.66144805038815,2.1946837817458,15.8750149668608));
#157916=CARTESIAN_POINT('Ctrl Pts',(6.59926293776704,2.36798548152523,15.8833983553356));
#157917=CARTESIAN_POINT('Ctrl Pts',(6.59003002008751,2.39371640425486,15.8846430766588));
#157918=CARTESIAN_POINT('Ctrl Pts',(6.58064518186825,2.41939730899936,15.885887797982));
#157919=CARTESIAN_POINT('Ctrl Pts',(6.57110895151814,2.44502632087636,15.8871325193051));
#157920=CARTESIAN_POINT('',(7.01124961619472,-0.00231989425524781,15.2264656430654));
#157921=CARTESIAN_POINT('Ctrl Pts',(6.57110895151815,2.44502632087634,15.3398759450547));
#157922=CARTESIAN_POINT('Ctrl Pts',(6.63285964731569,2.27906878232018,15.3318538569744));
#157923=CARTESIAN_POINT('Ctrl Pts',(6.68832544267615,2.11075369790805,15.3238317688941));
#157924=CARTESIAN_POINT('Ctrl Pts',(6.7373341885473,1.9406067593234,15.3158096808138));
#157925=CARTESIAN_POINT('Ctrl Pts',(6.78636192543487,1.7703938883578,15.3077844841535));
#157926=CARTESIAN_POINT('Ctrl Pts',(6.82892751104394,1.59834809721087,15.2997592874933));
#157927=CARTESIAN_POINT('Ctrl Pts',(6.86490897642211,1.42500923082597,15.291734090833));
#157928=CARTESIAN_POINT('Ctrl Pts',(6.90089822560439,1.25163286636344,15.2837071580967));
#157929=CARTESIAN_POINT('Ctrl Pts',(6.93030045155082,1.07696323009593,15.2756802253604));
#157930=CARTESIAN_POINT('Ctrl Pts',(6.95304512735804,0.901548678343343,
15.2676532926241));
#157931=CARTESIAN_POINT('Ctrl Pts',(6.97580772661208,0.725995894970501,
15.2596200344382));
#157932=CARTESIAN_POINT('Ctrl Pts',(6.99190226173688,0.54969738842236,15.2515867762522));
#157933=CARTESIAN_POINT('Ctrl Pts',(7.00131017838675,0.373205504404982,
15.2435535180663));
#157934=CARTESIAN_POINT('Ctrl Pts',(7.00579043828701,0.289156129807543,
15.2397279012099));
#157935=CARTESIAN_POINT('Ctrl Pts',(7.0087550187039,0.205062904514265,15.2359022843535));
#157936=CARTESIAN_POINT('Ctrl Pts',(7.01020606780222,0.120985327412108,
15.2320766674971));
#157937=CARTESIAN_POINT('Ctrl Pts',(7.01091548471569,0.079879857370017,
15.230206326028));
#157938=CARTESIAN_POINT('Ctrl Pts',(7.01126321422435,0.0387764624478537,
15.2283359845588));
#157939=CARTESIAN_POINT('Ctrl Pts',(7.0112496161949,-0.0023198937239668,
15.2264656430896));
#157940=CARTESIAN_POINT('Ctrl Pts',(7.01124961619472,-0.00231989425526735,
15.2264656430654));
#157941=CARTESIAN_POINT('Ctrl Pts',(7.01117905493752,-0.215572108811857,
15.2167602945277));
#157942=CARTESIAN_POINT('Ctrl Pts',(7.00137487997501,-0.428703660272864,
15.2070549459899));
#157943=CARTESIAN_POINT('Ctrl Pts',(6.98189533488068,-0.640908804176824,
15.1973495974522));
#157944=CARTESIAN_POINT('Ctrl Pts',(6.96239982346777,-0.85328788104056,
15.1876362939706));
#157945=CARTESIAN_POINT('Ctrl Pts',(6.93321308995598,-1.06473897836569,
15.1779229904891));
#157946=CARTESIAN_POINT('Ctrl Pts',(6.89444527559506,-1.27446102503178,
15.1682096870075));
#157947=CARTESIAN_POINT('Ctrl Pts',(6.85576051130448,-1.48373379615792,
15.1585171917802));
#157948=CARTESIAN_POINT('Ctrl Pts',(6.80753568172825,-1.69128486360751,
15.1488246965529));
#157949=CARTESIAN_POINT('Ctrl Pts',(6.7499315107308,-1.89632570064939,15.1391322013256));
#157950=CARTESIAN_POINT('Ctrl Pts',(6.69249133156878,-2.10078281219675,
15.1294672994141));
#157951=CARTESIAN_POINT('Ctrl Pts',(6.62572512478436,-2.30274390398725,
15.1198023975026));
#157952=CARTESIAN_POINT('Ctrl Pts',(6.54984332309524,-2.50143538901262,
15.1101374955911));
#157953=CARTESIAN_POINT('Ctrl Pts',(6.47443174862118,-2.69889561513824,
15.1005324855088));
#157954=CARTESIAN_POINT('Ctrl Pts',(6.39001719368613,-2.89312656098337,
15.0909274754265));
#157955=CARTESIAN_POINT('Ctrl Pts',(6.29685686916809,-3.0833780390524,15.0813224653443));
#157956=CARTESIAN_POINT('Ctrl Pts',(6.27127292373383,-3.13562542503873,
15.0786847109664));
#157957=CARTESIAN_POINT('Ctrl Pts',(6.24502968962702,-3.18757274566128,
15.0760469565886));
#157958=CARTESIAN_POINT('Ctrl Pts',(6.21813317189115,-3.239204596676,15.0734092022107));
#157959=CARTESIAN_POINT('Ctrl Pts',(6.13806986340353,-3.39289798019031,
15.0655573551968));
#157960=CARTESIAN_POINT('Ctrl Pts',(6.05224545515072,-3.54373423243102,
15.0577055081829));
#157961=CARTESIAN_POINT('Ctrl Pts',(5.96090446899768,-3.69123888064475,
15.049853661169));
#157962=CARTESIAN_POINT('Ctrl Pts',(5.86958938640981,-3.83870169773283,
15.0420040408754));
#157963=CARTESIAN_POINT('Ctrl Pts',(5.77276103852661,-3.98283446619701,
15.0341544205818));
#157964=CARTESIAN_POINT('Ctrl Pts',(5.67070922212415,-4.12318850898382,
15.0263048002882));
#157965=CARTESIAN_POINT('Ctrl Pts',(5.56866555325388,-4.26353134629557,
15.0184558066864));
#157966=CARTESIAN_POINT('Ctrl Pts',(5.46139947098912,-4.40009575040983,
15.0106068130846));
#157967=CARTESIAN_POINT('Ctrl Pts',(5.34924314538045,-4.5324633847501,15.0027578194828));
#157968=CARTESIAN_POINT('Ctrl Pts',(5.23703003830839,-4.66489803294752,
14.9949048521654));
#157969=CARTESIAN_POINT('Ctrl Pts',(5.1199219880671,-4.79313137469256,14.987051884848));
#157970=CARTESIAN_POINT('Ctrl Pts',(4.99829060257687,-4.9167791911669,14.9791989175306));
#157971=CARTESIAN_POINT('Ctrl Pts',(4.87662832680158,-5.040458410032,14.9713439558233));
#157972=CARTESIAN_POINT('Ctrl Pts',(4.75044070460538,-5.15954952167867,
14.963488994116));
#157973=CARTESIAN_POINT('Ctrl Pts',(4.62013451442953,-5.27370682073596,
14.9556340324088));
#157974=CARTESIAN_POINT('Ctrl Pts',(4.4896989844677,-5.38797743045493,14.9477712739954));
#157975=CARTESIAN_POINT('Ctrl Pts',(4.35513701763923,-5.49730420614854,
14.9399085155821));
#157976=CARTESIAN_POINT('Ctrl Pts',(4.21688707096991,-5.60138286436366,
14.9320457571687));
#157977=CARTESIAN_POINT('Ctrl Pts',(4.1154688938625,-5.67773347459001,14.9262777504206));
#157978=CARTESIAN_POINT('Ctrl Pts',(4.01206669416725,-5.75126069484699,
14.9205097436725));
#157979=CARTESIAN_POINT('Ctrl Pts',(3.9068624521206,-5.82185986972464,14.9147417369243));
#157980=CARTESIAN_POINT('Ctrl Pts',(3.75405262227269,-5.92440561969234,
14.9063636704833));
#157981=CARTESIAN_POINT('Ctrl Pts',(3.59710154621272,-6.02099952136897,
14.8979856040423));
#157982=CARTESIAN_POINT('Ctrl Pts',(3.43650094856787,-6.11130818998618,
14.8896075376013));
#157983=CARTESIAN_POINT('Ctrl Pts',(3.27601016770342,-6.20155510660884,
14.8812351999825));
#157984=CARTESIAN_POINT('Ctrl Pts',(3.11187512615867,-6.28552519804157,
14.8728628623638));
#157985=CARTESIAN_POINT('Ctrl Pts',(2.94461521837787,-6.36292918223969,
14.8644905247451));
#157986=CARTESIAN_POINT('Ctrl Pts',(2.77744515215865,-6.44029158985855,
14.8561226842225));
#157987=CARTESIAN_POINT('Ctrl Pts',(2.60715386409951,-6.51109478480129,
14.8477548436999));
#157988=CARTESIAN_POINT('Ctrl Pts',(2.43428437051971,-6.57509590545594,
14.8393870031773));
#157989=CARTESIAN_POINT('Ctrl Pts',(2.26148240749429,-6.63907202441093,
14.8310224315074));
#157990=CARTESIAN_POINT('Ctrl Pts',(2.08610455518346,-6.69625125394265,
14.8226578598375));
#157991=CARTESIAN_POINT('Ctrl Pts',(1.90871321004138,-6.74643909364885,
14.8142932881676));
#157992=CARTESIAN_POINT('Ctrl Pts',(1.73136519607964,-6.79661467402903,
14.805930759702));
#157993=CARTESIAN_POINT('Ctrl Pts',(1.55200498623125,-6.83980218132074,
14.7975682312364));
#157994=CARTESIAN_POINT('Ctrl Pts',(1.37120995672951,-6.8758570241873,14.7892057027708));
#157995=CARTESIAN_POINT('Ctrl Pts',(1.19040049921894,-6.91191474434309,
14.7808425069493));
#157996=CARTESIAN_POINT('Ctrl Pts',(1.00815631443533,-6.94083859267118,
14.7724793111278));
#157997=CARTESIAN_POINT('Ctrl Pts',(0.825065550162284,-6.96253498378539,
14.7641161153063));
#157998=CARTESIAN_POINT('Ctrl Pts',(0.641962299466072,-6.98423285454999,
14.7557523491316));
#157999=CARTESIAN_POINT('Ctrl Pts',(0.458012680667262,-6.9987022463424,
14.7473885829569));
#158000=CARTESIAN_POINT('Ctrl Pts',(0.273810730400995,-7.00590138714622,
14.7390248167822));
#158001=CARTESIAN_POINT('Ctrl Pts',(0.0895716594778335,-7.01310197873182,
14.7306593651286));
#158002=CARTESIAN_POINT('Ctrl Pts',(-0.0949195157738741,-7.01302938503274,
14.722293913475));
#158003=CARTESIAN_POINT('Ctrl Pts',(-0.279067550926409,-7.00569396023834,
14.7139284618214));
#158004=CARTESIAN_POINT('Ctrl Pts',(-0.463277256893581,-6.99835607882461,
14.7055602085946));
#158005=CARTESIAN_POINT('Ctrl Pts',(-0.647143265221654,-6.9837505293066,
14.6971919553677));
#158006=CARTESIAN_POINT('Ctrl Pts',(-0.830073813274393,-6.96193967418679,
14.6888237021408));
#158007=CARTESIAN_POINT('Ctrl Pts',(-1.01317396404313,-6.94010859729263,
14.6804476903494));
#158008=CARTESIAN_POINT('Ctrl Pts',(-1.19533659459348,-6.91105890443767,
14.6720716785579));
#158009=CARTESIAN_POINT('Ctrl Pts',(-1.37597728166385,-6.87490458718119,
14.6636956667664));
#158010=CARTESIAN_POINT('Ctrl Pts',(-1.55670655715935,-6.83873253940077,
14.6553155472753));
#158011=CARTESIAN_POINT('Ctrl Pts',(-1.73591207984935,-6.79544898995672,
14.6469354277841));
#158012=CARTESIAN_POINT('Ctrl Pts',(-1.91302236952525,-6.745218452815,14.6385553082929));
#158013=CARTESIAN_POINT('Ctrl Pts',(-2.0903350301421,-6.69493052092178,
14.6301656134537));
#158014=CARTESIAN_POINT('Ctrl Pts',(-2.26554735932142,-6.63767983593482,
14.6217759186145));
#158015=CARTESIAN_POINT('Ctrl Pts',(-2.43810443619075,-6.57368034823165,
14.6133862237753));
#158016=CARTESIAN_POINT('Ctrl Pts',(-2.5476579465224,-6.53304817791146,
14.6080597513007));
#158017=CARTESIAN_POINT('Ctrl Pts',(-2.65614157544742,-6.4896967032418,
14.6027332788261));
#158018=CARTESIAN_POINT('Ctrl Pts',(-2.76341802457582,-6.44369050963417,
14.5974068063514));
#158019=CARTESIAN_POINT('Ctrl Pts',(-2.93221945005896,-6.37129893510762,
14.5890255059466));
#158020=CARTESIAN_POINT('Ctrl Pts',(-3.0983713354527,-6.29218604120259,
14.5806442055417));
#158021=CARTESIAN_POINT('Ctrl Pts',(-3.26131974452614,-6.20656266273563,
14.5722629051368));
#158022=CARTESIAN_POINT('Ctrl Pts',(-3.42406164034511,-6.12104779936646,
14.5638922268032));
#158023=CARTESIAN_POINT('Ctrl Pts',(-3.58360786318189,-6.02903904616635,
14.5555215484697));
#158024=CARTESIAN_POINT('Ctrl Pts',(-3.73942423593819,-5.93079530469381,
14.5471508701361));
#158025=CARTESIAN_POINT('Ctrl Pts',(-3.89506378386354,-5.83266305300036,
14.5387896910853));
#158026=CARTESIAN_POINT('Ctrl Pts',(-4.04698164254987,-5.72831008925468,
14.5304285120345));
#158027=CARTESIAN_POINT('Ctrl Pts',(-4.19466765942402,-5.61804145494515,
14.5220673329837));
#158028=CARTESIAN_POINT('Ctrl Pts',(-4.34216203627036,-5.50791590719583,
14.513717003549));
#158029=CARTESIAN_POINT('Ctrl Pts',(-4.48543526300853,-5.39189019513811,
14.5053666741143));
#158030=CARTESIAN_POINT('Ctrl Pts',(-4.62400570592323,-5.27031287440218,
14.4970163446796));
#158031=CARTESIAN_POINT('Ctrl Pts',(-4.76246952717136,-5.14882910014184,
14.4886724403239));
#158032=CARTESIAN_POINT('Ctrl Pts',(-4.89623753038195,-5.02180244495776,
14.4803285359682));
#158033=CARTESIAN_POINT('Ctrl Pts',(-5.02485984787179,-4.88962269216613,
14.4719846316124));
#158034=CARTESIAN_POINT('Ctrl Pts',(-5.15337885511394,-4.7575491069764,
14.4636474291327));
#158035=CARTESIAN_POINT('Ctrl Pts',(-5.27676019156735,-4.62033091296745,
14.455310226653));
#158036=CARTESIAN_POINT('Ctrl Pts',(-5.39458956111235,-4.47839592149217,
14.4469730241733));
#158037=CARTESIAN_POINT('Ctrl Pts',(-5.43337833916447,-4.43167170576036,
14.4442284631372));
#158038=CARTESIAN_POINT('Ctrl Pts',(-5.47156574979355,-4.38443663526283,
14.4414839021011));
#158039=CARTESIAN_POINT('Ctrl Pts',(-5.50913790009358,-4.33670683356075,
14.438739341065));
#158040=CARTESIAN_POINT('Ctrl Pts',(-5.62328666333548,-4.19169788968699,
14.4304010307631));
#158041=CARTESIAN_POINT('Ctrl Pts',(-5.73165981888653,-4.04223901281737,
14.4220627204612));
#158042=CARTESIAN_POINT('Ctrl Pts',(-5.83392404630276,-3.88882460191642,
14.4137244101593));
#158043=CARTESIAN_POINT('Ctrl Pts',(-5.93625261490078,-3.73531366787391,
14.4053808536755));
#158044=CARTESIAN_POINT('Ctrl Pts',(-6.03246440723192,-3.57784250843427,
14.3970372971916));
#158045=CARTESIAN_POINT('Ctrl Pts',(-6.12227082116779,-3.41693233102112,
14.3886937407078));
#158046=CARTESIAN_POINT('Ctrl Pts',(-6.212145559432,-3.25589973384628,14.3803438364826));
#158047=CARTESIAN_POINT('Ctrl Pts',(-6.29560503938939,-3.09142318563735,
14.3719939322574));
#158048=CARTESIAN_POINT('Ctrl Pts',(-6.37240757103098,-2.92404656446629,
14.3636440280321));
#158049=CARTESIAN_POINT('Ctrl Pts',(-6.44932530078655,-2.75641889074953,
14.3552815995685));
#158050=CARTESIAN_POINT('Ctrl Pts',(-6.51956599243058,-2.58588274966744,
14.3469191711048));
#158051=CARTESIAN_POINT('Ctrl Pts',(-6.58293633678555,-2.41300139832708,
14.3385567426412));
#158052=CARTESIAN_POINT('Ctrl Pts',(-6.64636087142363,-2.23997220986405,
14.3301871631612));
#158053=CARTESIAN_POINT('Ctrl Pts',(-6.70290323616088,-2.06459412080513,
14.3218175836812));
#158054=CARTESIAN_POINT('Ctrl Pts',(-6.75242043074529,-1.8874440094884,
14.3134480042012));
#158055=CARTESIAN_POINT('Ctrl Pts',(-6.80201399956923,-1.71002066570872,
14.3050655156647));
#158056=CARTESIAN_POINT('Ctrl Pts',(-6.84456067020032,-1.53082015623563,
14.2966830271281));
#158057=CARTESIAN_POINT('Ctrl Pts',(-6.87996853946572,-1.35042936078195,
14.2883005385915));
#158058=CARTESIAN_POINT('Ctrl Pts',(-6.8915545744813,-1.29140253663311,
14.2855576509872));
#158059=CARTESIAN_POINT('Ctrl Pts',(-6.90237666812968,-1.23224830520003,
14.2828147633829));
#158060=CARTESIAN_POINT('Ctrl Pts',(-6.91243280912787,-1.17298730674829,
14.2800718757786));
#158061=CARTESIAN_POINT('Ctrl Pts',(-6.94319220518833,-0.991721697739546,
14.2716820206458));
#158062=CARTESIAN_POINT('Ctrl Pts',(-6.96684353899493,-0.809090877999625,
14.2632921655131));
#158063=CARTESIAN_POINT('Ctrl Pts',(-6.98327672178247,-0.625677864009183,
14.2549023103803));
#158064=CARTESIAN_POINT('Ctrl Pts',(-6.99969474025931,-0.442434100976752,
14.2465201972882));
#158065=CARTESIAN_POINT('Ctrl Pts',(-7.00890785683722,-0.258409908431101,
14.2381380841961));
#158066=CARTESIAN_POINT('Ctrl Pts',(-7.01085739945251,-0.0741962737743869,
14.229755971104));
#158067=CARTESIAN_POINT('Ctrl Pts',(-7.01280542963592,0.109874450144695,
14.2213803607551));
#158068=CARTESIAN_POINT('Ctrl Pts',(-7.00750111685168,0.294133995638763,
14.2130047504063));
#158069=CARTESIAN_POINT('Ctrl Pts',(-6.99493774077801,0.477988038699149,
14.2046291400574));
#158070=CARTESIAN_POINT('Ctrl Pts',(-6.98238226725445,0.661726434836188,
14.1962587980918));
#158071=CARTESIAN_POINT('Ctrl Pts',(-6.96257685710581,0.845059510003589,
14.1878884561262));
#158072=CARTESIAN_POINT('Ctrl Pts',(-6.93556685367119,1.02739426743462,
14.1795181141607));
#158073=CARTESIAN_POINT('Ctrl Pts',(-6.90856988056661,1.2096410618236,14.1711518102663));
#158074=CARTESIAN_POINT('Ctrl Pts',(-6.87437529333594,1.39089017429796,
14.162785506372));
#158075=CARTESIAN_POINT('Ctrl Pts',(-6.83308018701918,1.57055459003051,
14.1544192024777));
#158076=CARTESIAN_POINT('Ctrl Pts',(-6.79179662978624,1.75016875866163,
14.1460552384041));
#158077=CARTESIAN_POINT('Ctrl Pts',(-6.74341658530399,1.92819879393217,
14.1376912743304));
#158078=CARTESIAN_POINT('Ctrl Pts',(-6.6880881936728,2.10406817288664,14.1293273102568));
#158079=CARTESIAN_POINT('Ctrl Pts',(-6.63276831616165,2.27991048846626,
14.1209646332583));
#158080=CARTESIAN_POINT('Ctrl Pts',(-6.57050232194391,2.45359249722821,
14.1126019562597));
#158081=CARTESIAN_POINT('Ctrl Pts',(-6.50148825500374,2.62455272999962,
14.1042392792612));
#158082=CARTESIAN_POINT('Ctrl Pts',(-6.43247560893708,2.79550944301226,
14.0958767744349));
#158083=CARTESIAN_POINT('Ctrl Pts',(-6.35671529057287,2.96374418716771,
14.0875142696086));
#158084=CARTESIAN_POINT('Ctrl Pts',(-6.27445369610554,3.12871497230534,
14.0791517647823));
#158085=CARTESIAN_POINT('Ctrl Pts',(-6.19218283036907,3.29370435042744,
14.0707883174623));
#158086=CARTESIAN_POINT('Ctrl Pts',(-6.10340937481897,3.45542874225665,
14.0624248701423));
#158087=CARTESIAN_POINT('Ctrl Pts',(-6.00842612691287,3.61336990078941,
14.0540614228224));
#158088=CARTESIAN_POINT('Ctrl Pts',(-5.91338695020106,3.77140405951497,
14.0456930508695));
#158089=CARTESIAN_POINT('Ctrl Pts',(-5.81213084330804,3.9256502510821,14.0373246789167));
#158090=CARTESIAN_POINT('Ctrl Pts',(-5.70499502510663,4.07561753922135,
14.0289563069639));
#158091=CARTESIAN_POINT('Ctrl Pts',(-5.59782710621405,4.22562976147958,
14.0205854276282));
#158092=CARTESIAN_POINT('Ctrl Pts',(-5.48477615858671,4.37136025948855,
14.0122145482924));
#158093=CARTESIAN_POINT('Ctrl Pts',(-5.36622073602281,4.51234989498585,
14.0038436689567));
#158094=CARTESIAN_POINT('Ctrl Pts',(-5.2475648627314,4.65345898947669,13.9954656970654));
#158095=CARTESIAN_POINT('Ctrl Pts',(-5.12339541103834,4.78981894673049,
13.9870877251741));
#158096=CARTESIAN_POINT('Ctrl Pts',(-4.99412973283141,4.92100546373902,
13.9787097532828));
#158097=CARTESIAN_POINT('Ctrl Pts',(-4.91198034171617,5.00437556355413,
13.9733854839238));
#158098=CARTESIAN_POINT('Ctrl Pts',(-4.82777348467621,5.08565699865715,
13.9680612145648));
#158099=CARTESIAN_POINT('Ctrl Pts',(-4.74162354313369,5.16474904886001,
13.9627369452057));
#158100=CARTESIAN_POINT('Ctrl Pts',(-4.61439811526017,5.28155144881852,
13.9548741140165));
#158101=CARTESIAN_POINT('Ctrl Pts',(-4.48266862771123,5.39381977872991,
13.9470112828272));
#158102=CARTESIAN_POINT('Ctrl Pts',(-4.34680621465619,5.5011728108401,13.9391484516379));
#158103=CARTESIAN_POINT('Ctrl Pts',(-4.21104819393207,5.60844335631546,
13.9312916619965));
#158104=CARTESIAN_POINT('Ctrl Pts',(-4.07116386007449,5.71080587976393,
13.9234348723551));
#158105=CARTESIAN_POINT('Ctrl Pts',(-3.92756051208506,5.80791657880949,
13.9155780827138));
#158106=CARTESIAN_POINT('Ctrl Pts',(-3.78403814958601,5.90497251201781,
13.9077257239298));
#158107=CARTESIAN_POINT('Ctrl Pts',(-3.63680125991078,5.99678229956816,
13.8998733651458));
#158108=CARTESIAN_POINT('Ctrl Pts',(-3.48628926875563,6.083043127996,13.8920210063619));
#158109=CARTESIAN_POINT('Ctrl Pts',(-3.33581281523772,6.16928358923578,
13.8841705016115));
#158110=CARTESIAN_POINT('Ctrl Pts',(-3.18206312560092,6.24997750223041,
13.876319996861));
#158111=CARTESIAN_POINT('Ctrl Pts',(-3.02550753064883,6.32486606533982,
13.8684694921106));
#158112=CARTESIAN_POINT('Ctrl Pts',(-2.86897712055763,6.39974258123977,
13.860620250259));
#158113=CARTESIAN_POINT('Ctrl Pts',(-2.70964204919594,6.46881544444567,
13.8527710084073));
#158114=CARTESIAN_POINT('Ctrl Pts',(-2.54799267681535,6.53187261674593,
13.8449217665557));
#158115=CARTESIAN_POINT('Ctrl Pts',(-2.38628884159724,6.59495103424177,
13.8370698801408));
#158116=CARTESIAN_POINT('Ctrl Pts',(-2.22226950364427,6.65200957363986,
13.829217993726));
#158117=CARTESIAN_POINT('Ctrl Pts',(-2.0564435429659,6.70288493986685,13.8213661073111));
#158118=CARTESIAN_POINT('Ctrl Pts',(-1.93467960403471,6.74024208805417,
13.8156005648472));
#158119=CARTESIAN_POINT('Ctrl Pts',(-1.81194197276822,6.77426641776532,
13.8098350223832));
#158120=CARTESIAN_POINT('Ctrl Pts',(-1.68843657932644,6.80491061514348,
13.8040694799193));
#158121=CARTESIAN_POINT('Ctrl Pts',(-1.48160744378032,6.85622912583037,
13.7944141755594));
#158122=CARTESIAN_POINT('Ctrl Pts',(-1.27273050459558,6.89804131974426,
13.7847588711995));
#158123=CARTESIAN_POINT('Ctrl Pts',(-1.0626057372995,6.93025941863349,13.7751035668396));
#158124=CARTESIAN_POINT('Ctrl Pts',(-0.85131691821211,6.96265599974643,
13.7653947739049));
#158125=CARTESIAN_POINT('Ctrl Pts',(-0.638766462176318,6.98535193935877,
13.7556859809701));
#158126=CARTESIAN_POINT('Ctrl Pts',(-0.425764535513677,6.99831059062106,
13.7459771880354));
#158127=CARTESIAN_POINT('Ctrl Pts',(-0.211737625493769,7.01133160001355,
13.7362216755647));
#158128=CARTESIAN_POINT('Ctrl Pts',(0.00274506599505633,7.01452140358415,
13.726466163094));
#158129=CARTESIAN_POINT('Ctrl Pts',(0.216865565637567,7.00789525385053,
13.7167106506233));
#158130=CARTESIAN_POINT('Ctrl Pts',(0.431198077516598,7.00126254320925,
13.7069454786944));
#158131=CARTESIAN_POINT('Ctrl Pts',(0.645167642239691,6.98479445079353,
13.6971803067655));
#158132=CARTESIAN_POINT('Ctrl Pts',(0.857958406906245,6.95855832299471,
13.6874151348366));
#158133=CARTESIAN_POINT('Ctrl Pts',(1.07045903619301,6.93235796756088,13.6776632774981));
#158134=CARTESIAN_POINT('Ctrl Pts',(1.28178404011654,6.89641620031286,13.6679114201595));
#158135=CARTESIAN_POINT('Ctrl Pts',(1.49112599177709,6.85085176012055,13.658159562821));
#158136=CARTESIAN_POINT('Ctrl Pts',(1.58241424396691,6.83098236426286,13.6539070467583));
#158137=CARTESIAN_POINT('Ctrl Pts',(1.67332546937911,6.80928379237649,13.6496545306955));
#158138=CARTESIAN_POINT('Ctrl Pts',(1.76379304747665,6.78576897987052,13.6454020146328));
#158139=CARTESIAN_POINT('Ctrl Pts',(1.93468721209668,6.74134926262031,13.637368969034));
#158140=CARTESIAN_POINT('Ctrl Pts',(2.10408073117804,6.69042322326471,13.6293359234352));
#158141=CARTESIAN_POINT('Ctrl Pts',(2.27143590991143,6.633114311518,13.6213028778363));
#158142=CARTESIAN_POINT('Ctrl Pts',(2.43868350629205,6.57584224014638,13.6132749961885));
#158143=CARTESIAN_POINT('Ctrl Pts',(2.60389502520306,6.51219558207775,13.6052471145407));
#158144=CARTESIAN_POINT('Ctrl Pts',(2.76654609550033,6.44234811726065,13.5972192328929));
#158145=CARTESIAN_POINT('Ctrl Pts',(2.92912372723587,6.37253218926251,13.5891949759128));
#158146=CARTESIAN_POINT('Ctrl Pts',(3.08914287609492,6.29652117343372,13.5811707189327));
#158147=CARTESIAN_POINT('Ctrl Pts',(3.24609743408801,6.21453763452336,13.5731464619526));
#158148=CARTESIAN_POINT('Ctrl Pts',(3.40303301467663,6.13256400825778,13.5651231751869));
#158149=CARTESIAN_POINT('Ctrl Pts',(3.55690441415735,6.04461946007117,13.5570998884212));
#158150=CARTESIAN_POINT('Ctrl Pts',(3.70722834423393,5.95097341333404,13.5490766016555));
#158151=CARTESIAN_POINT('Ctrl Pts',(3.85753995660528,5.85733504005514,13.5410539723266));
#158152=CARTESIAN_POINT('Ctrl Pts',(4.00430436951159,5.75799629609272,13.5330313429976));
#158153=CARTESIAN_POINT('Ctrl Pts',(4.14706587138744,5.65327084269572,13.5250087136687));
#158154=CARTESIAN_POINT('Ctrl Pts',(4.28988104142454,5.54850601998384,13.5169830684023));
#158155=CARTESIAN_POINT('Ctrl Pts',(4.42869000032998,5.43835066191202,13.5089574231359));
#158156=CARTESIAN_POINT('Ctrl Pts',(4.56306852052165,5.32315998627924,13.5009317778695));
#158157=CARTESIAN_POINT('Ctrl Pts',(4.64230628464827,5.2552365445539,13.4961993683618));
#158158=CARTESIAN_POINT('Ctrl Pts',(4.72000421274412,5.18556308634323,13.4914669588541));
#158159=CARTESIAN_POINT('Ctrl Pts',(4.79608113605262,5.11421864011505,13.4867345493464));
#158160=CARTESIAN_POINT('Ctrl Pts',(4.93641825604448,4.98261139739737,13.4780047967217));
#158161=CARTESIAN_POINT('Ctrl Pts',(5.07130774320044,4.84525047187811,13.4692750440971));
#158162=CARTESIAN_POINT('Ctrl Pts',(5.20030252992249,4.70260355120243,13.4605452914724));
#158163=CARTESIAN_POINT('Ctrl Pts',(5.32933520731001,4.55991472971133,13.451812974588));
#158164=CARTESIAN_POINT('Ctrl Pts',(5.45246954423712,4.41193701681353,13.4430806577035));
#158165=CARTESIAN_POINT('Ctrl Pts',(5.5692976497973,4.25917248423474,13.4343483408191));
#158166=CARTESIAN_POINT('Ctrl Pts',(5.68618189330382,4.10633454562842,13.4256118279039));
#158167=CARTESIAN_POINT('Ctrl Pts',(5.79675368208154,3.9487054074843,13.4168753149886));
#158168=CARTESIAN_POINT('Ctrl Pts',(5.90064667843867,3.78681863029255,13.4081388020733));
#158169=CARTESIAN_POINT('Ctrl Pts',(6.00455354455175,3.62491024115225,13.3994011228301));
#158170=CARTESIAN_POINT('Ctrl Pts',(6.10177969345145,3.45874331079357,13.3906634435869));
#158171=CARTESIAN_POINT('Ctrl Pts',(6.19200305242617,3.28887895205113,13.3819257643437));
#158172=CARTESIAN_POINT('Ctrl Pts',(6.28225097168962,3.11896835342424,13.3731857065599));
#158173=CARTESIAN_POINT('Ctrl Pts',(6.365492163762,2.94535855734084,13.3644456487761));
#158174=CARTESIAN_POINT('Ctrl Pts',(6.44145072079951,2.76863489359133,13.3557055909922));
#158175=CARTESIAN_POINT('Ctrl Pts',(6.48734531525382,2.66185744553822,13.3504247981081));
#158176=CARTESIAN_POINT('Ctrl Pts',(6.53058218404267,2.55394367782272,13.3451440052239));
#158177=CARTESIAN_POINT('Ctrl Pts',(6.57110895151813,2.44502632087638,13.3398632123397));
#158178=CARTESIAN_POINT('Origin',(0.,0.,50.));
#158179=CARTESIAN_POINT('',(6.57110895151813,2.44502632087638,11.3397782664936));
#158180=CARTESIAN_POINT('',(6.57110895151814,2.44502632087637,11.8871243640548));
#158181=CARTESIAN_POINT('',(6.57110895151814,2.44502632087636,50.));
#158182=CARTESIAN_POINT('',(7.0112496259069,-0.00229035375306598,13.7735343568827));
#158183=CARTESIAN_POINT('Ctrl Pts',(6.57110895151814,2.44502632087636,11.8871243640548));
#158184=CARTESIAN_POINT('Ctrl Pts',(6.50760538438029,2.61569477336292,11.8953815622089));
#158185=CARTESIAN_POINT('Ctrl Pts',(6.43743464203002,2.78392547564742,11.9036387603629));
#158186=CARTESIAN_POINT('Ctrl Pts',(6.36081519077275,2.9491789825873,11.911895958517));
#158187=CARTESIAN_POINT('Ctrl Pts',(6.28420124408154,3.11442061723063,11.9201525634498));
#158188=CARTESIAN_POINT('Ctrl Pts',(6.20113965574545,3.27668517334573,11.9284091683825));
#158189=CARTESIAN_POINT('Ctrl Pts',(6.11189630149514,3.43545486977635,11.9366657733153));
#158190=CARTESIAN_POINT('Ctrl Pts',(6.02264530226914,3.59423816711294,11.9449230855449));
#158191=CARTESIAN_POINT('Ctrl Pts',(5.92721164966669,3.74952571095857,11.9531803977745));
#158192=CARTESIAN_POINT('Ctrl Pts',(5.82590641104413,3.9008256885248,11.9614377100041));
#158193=CARTESIAN_POINT('Ctrl Pts',(5.72454044241862,4.0522163667123,11.9696999722896));
#158194=CARTESIAN_POINT('Ctrl Pts',(5.6172960445512,4.19961441816603,11.9779622345751));
#158195=CARTESIAN_POINT('Ctrl Pts',(5.50452724491788,4.3425575842419,11.9862244968607));
#158196=CARTESIAN_POINT('Ctrl Pts',(5.3917222526362,4.48554662729581,11.9944894108828));
#158197=CARTESIAN_POINT('Ctrl Pts',(5.27338954081468,4.62407767099775,12.0027543249049));
#158198=CARTESIAN_POINT('Ctrl Pts',(5.14992267951546,4.75772245486349,12.011019238927));
#158199=CARTESIAN_POINT('Ctrl Pts',(5.02634348688269,4.89148883003427,12.0192916724471));
#158200=CARTESIAN_POINT('Ctrl Pts',(4.89762104960985,5.02035981792788,12.0275641059672));
#158201=CARTESIAN_POINT('Ctrl Pts',(4.76418567851758,5.14394414657741,12.0358365394873));
#158202=CARTESIAN_POINT('Ctrl Pts',(4.68680150134963,5.21561533469727,12.0406340340039));
#158203=CARTESIAN_POINT('Ctrl Pts',(4.6078328794217,5.28550920289178,12.0454315285205));
#158204=CARTESIAN_POINT('Ctrl Pts',(4.52736870480114,5.35355575046037,12.050229023037));
#158205=CARTESIAN_POINT('Ctrl Pts',(4.3954923223182,5.46508032119157,12.0580918542263));
#158206=CARTESIAN_POINT('Ctrl Pts',(4.25930025509482,5.57189116622296,12.0659546854156));
#158207=CARTESIAN_POINT('Ctrl Pts',(4.11917885399977,5.67362248755248,12.0738175166048));
#158208=CARTESIAN_POINT('Ctrl Pts',(3.97916511770559,5.77527564178997,12.0816743062462));
#158209=CARTESIAN_POINT('Ctrl Pts',(3.83522835813943,5.87185681133711,12.0895310958876));
#158210=CARTESIAN_POINT('Ctrl Pts',(3.68778953694743,5.96303906524861,12.097387885529));
#158211=CARTESIAN_POINT('Ctrl Pts',(3.54043386427054,6.05416989668566,12.105240244313));
#158212=CARTESIAN_POINT('Ctrl Pts',(3.38958038194864,6.13990766924159,12.1130926030969));
#158213=CARTESIAN_POINT('Ctrl Pts',(3.23568048250117,6.21996771516227,12.1209449618809));
#158214=CARTESIAN_POINT('Ctrl Pts',(3.08181692061632,6.30000885797164,12.1287954666313));
#158215=CARTESIAN_POINT('Ctrl Pts',(2.92490870724261,6.37437475898552,12.1366459713818));
#158216=CARTESIAN_POINT('Ctrl Pts',(2.76543332458663,6.44282586213268,12.1444964761322));
#158217=CARTESIAN_POINT('Ctrl Pts',(2.60598359649338,6.51126595365479,12.1523457179838));
#158218=CARTESIAN_POINT('Ctrl Pts',(2.44396787301681,6.57379299375415,12.1601949598355));
#158219=CARTESIAN_POINT('Ctrl Pts',(2.27988474238346,6.63021508881477,12.1680442016871));
#158220=CARTESIAN_POINT('Ctrl Pts',(2.11574632893181,6.68665619358357,12.1758960881019));
#158221=CARTESIAN_POINT('Ctrl Pts',(1.9495394781173,6.7369881206579,12.1837479745168));
#158222=CARTESIAN_POINT('Ctrl Pts',(1.78177929761831,6.78106843329861,12.1915998609316));
#158223=CARTESIAN_POINT('Ctrl Pts',(1.65859508514715,6.81343605821399,12.1973654033956));
#158224=CARTESIAN_POINT('Ctrl Pts',(1.53457370881477,6.84243397803418,12.2031309458595));
#158225=CARTESIAN_POINT('Ctrl Pts',(1.40992285470066,6.86802330414602,12.2088964883235));
#158226=CARTESIAN_POINT('Ctrl Pts',(1.20117546575607,6.91087664076099,12.2185517926834));
#158227=CARTESIAN_POINT('Ctrl Pts',(0.990769093079809,6.94414815441213,
12.2282070970433));
#158228=CARTESIAN_POINT('Ctrl Pts',(0.779506623166767,6.96778271668536,
12.2378624014033));
#158229=CARTESIAN_POINT('Ctrl Pts',(0.567073798805806,6.99154820999944,
12.2475711943379));
#158230=CARTESIAN_POINT('Ctrl Pts',(0.353775418667275,7.00556973151011,
12.2572799872726));
#158231=CARTESIAN_POINT('Ctrl Pts',(0.14042246938709,7.00984365678659,12.2669887802072));
#158232=CARTESIAN_POINT('Ctrl Pts',(-0.0739571524036458,7.01413814855446,
12.2767442926779));
#158233=CARTESIAN_POINT('Ctrl Pts',(-0.288391826045461,7.0085910289728,
12.2864998051487));
#158234=CARTESIAN_POINT('Ctrl Pts',(-0.502064877858065,6.99325084784761,
12.2962553176194));
#158235=CARTESIAN_POINT('Ctrl Pts',(-0.715949498864964,6.97789547758307,
12.3060204895483));
#158236=CARTESIAN_POINT('Ctrl Pts',(-0.929070952183159,6.95272766417894,
12.3157856614773));
#158237=CARTESIAN_POINT('Ctrl Pts',(-1.14061680418228,6.91784792175407,
12.3255508334062));
#158238=CARTESIAN_POINT('Ctrl Pts',(-1.35187421821159,6.88301573706666,
12.3353026907448));
#158239=CARTESIAN_POINT('Ctrl Pts',(-1.56156028716068,6.83849809556149,
12.3450545480834));
#158240=CARTESIAN_POINT('Ctrl Pts',(-1.76887308924225,6.78444651807755,
12.3548064054219));
#158241=CARTESIAN_POINT('Ctrl Pts',(-1.85927648525571,6.76087611569348,
12.3590589214846));
#158242=CARTESIAN_POINT('Ctrl Pts',(-1.94922867856742,6.73549340807665,
12.3633114375472));
#158243=CARTESIAN_POINT('Ctrl Pts',(-2.03866363066502,6.70831403286278,
12.3675639536099));
#158244=CARTESIAN_POINT('Ctrl Pts',(-2.20760715439131,6.65697191981173,
12.3755969992087));
#158245=CARTESIAN_POINT('Ctrl Pts',(-2.37478632349617,6.59918999176792,
12.3836300448075));
#158246=CARTESIAN_POINT('Ctrl Pts',(-2.53966891637576,6.53511349233468,
12.3916630904063));
#158247=CARTESIAN_POINT('Ctrl Pts',(-2.70444551637603,6.47107818374247,
12.3996909720541));
#158248=CARTESIAN_POINT('Ctrl Pts',(-2.86692813856673,6.40075649043177,
12.4077188537019));
#158249=CARTESIAN_POINT('Ctrl Pts',(-3.02659992353144,6.32434340191767,
12.4157467353497));
#158250=CARTESIAN_POINT('Ctrl Pts',(-3.18619961511134,6.24796481466624,
12.4237709923298));
#158251=CARTESIAN_POINT('Ctrl Pts',(-3.34299066646071,6.16550046633553,
12.4317952493099));
#158252=CARTESIAN_POINT('Ctrl Pts',(-3.49647645280875,6.07719334705207,
12.43981950629));
#158253=CARTESIAN_POINT('Ctrl Pts',(-3.64994368116209,5.98889690499867,
12.4478427930557));
#158254=CARTESIAN_POINT('Ctrl Pts',(-3.80010611913558,5.8947592751385,12.4558660798214));
#158255=CARTESIAN_POINT('Ctrl Pts',(-3.94649185092404,5.7950693380744,12.4638893665871));
#158256=CARTESIAN_POINT('Ctrl Pts',(-4.09286558770762,5.69538756971136,
12.4719119959161));
#158257=CARTESIAN_POINT('Ctrl Pts',(-4.23546293395095,5.59015461008322,
12.479934625245));
#158258=CARTESIAN_POINT('Ctrl Pts',(-4.37384132918284,5.47970241798149,
12.4879572545739));
#158259=CARTESIAN_POINT('Ctrl Pts',(-4.51227174483931,5.3692087037193,12.4959828998403));
#158260=CARTESIAN_POINT('Ctrl Pts',(-4.6464797563193,5.25349206862029,12.5040085451067));
#158261=CARTESIAN_POINT('Ctrl Pts',(-4.77605595330646,5.13292471144726,
12.512034190373));
#158262=CARTESIAN_POINT('Ctrl Pts',(-4.85246197503441,5.06183085064536,
12.5167665998808));
#158263=CARTESIAN_POINT('Ctrl Pts',(-4.92725817294144,4.9890511310218,12.5214990093886));
#158264=CARTESIAN_POINT('Ctrl Pts',(-5.00036666383986,4.91466782088668,
12.5262314188964));
#158265=CARTESIAN_POINT('Ctrl Pts',(-5.13523256982751,4.77745020924604,
12.534961467731));
#158266=CARTESIAN_POINT('Ctrl Pts',(-5.26442067180707,4.63470515361891,
12.5436915165657));
#158267=CARTESIAN_POINT('Ctrl Pts',(-5.38750327559169,4.48691820941599,
12.5524215654003));
#158268=CARTESIAN_POINT('Ctrl Pts',(-5.51062146886518,4.33908853243327,
12.5611541385395));
#158269=CARTESIAN_POINT('Ctrl Pts',(-5.62763046477304,4.18621426739015,
12.5698867116787));
#158270=CARTESIAN_POINT('Ctrl Pts',(-5.73814312435743,4.02881372700321,
12.5786192848179));
#158271=CARTESIAN_POINT('Ctrl Pts',(-5.85022579268221,3.86917706068211,
12.5874759180983));
#158272=CARTESIAN_POINT('Ctrl Pts',(-5.95562596969656,3.70488477013143,
12.5963325513787));
#158273=CARTESIAN_POINT('Ctrl Pts',(-6.05398527447998,3.53650800350849,
12.6051891846591));
#158274=CARTESIAN_POINT('Ctrl Pts',(-6.15102853820277,3.37038410700311,
12.6139273167659));
#158275=CARTESIAN_POINT('Ctrl Pts',(-6.24121805231284,3.20028460720148,
12.6226654488726));
#158276=CARTESIAN_POINT('Ctrl Pts',(-6.32425545767368,3.02678368381104,
12.6314035809794));
#158277=CARTESIAN_POINT('Ctrl Pts',(-6.40898201636928,2.84975339119167,
12.6403194648466));
#158278=CARTESIAN_POINT('Ctrl Pts',(-6.48626224073296,2.66918207419653,
12.6492353487138));
#158279=CARTESIAN_POINT('Ctrl Pts',(-6.5558300063021,2.48570301745182,12.6581512325811));
#158280=CARTESIAN_POINT('Ctrl Pts',(-6.62539777187123,2.30222396070711,
12.6670671164483));
#158281=CARTESIAN_POINT('Ctrl Pts',(-6.68725297711931,2.1158374491383,12.6759830003155));
#158282=CARTESIAN_POINT('Ctrl Pts',(-6.74118250120182,1.92719616230169,
12.6848988841828));
#158283=CARTESIAN_POINT('Ctrl Pts',(-6.79405229650815,1.74226172442096,
12.693639568679));
#158284=CARTESIAN_POINT('Ctrl Pts',(-6.83931061792905,1.55514066064806,
12.7023802531752));
#158285=CARTESIAN_POINT('Ctrl Pts',(-6.87680237159827,1.3664610146215,12.7111209376714));
#158286=CARTESIAN_POINT('Ctrl Pts',(-6.91428737987839,1.17781531519662,
12.7198600495733));
#158287=CARTESIAN_POINT('Ctrl Pts',(-6.9440085576483,0.987611861976033,
12.7285991614752));
#158288=CARTESIAN_POINT('Ctrl Pts',(-6.9658618755799,0.796489104032495,
12.7373382733771));
#158289=CARTESIAN_POINT('Ctrl Pts',(-6.98799833469763,0.60289007568695,
12.7461906130514));
#158290=CARTESIAN_POINT('Ctrl Pts',(-7.00206157913035,0.408348035340911,
12.7550429527258));
#158291=CARTESIAN_POINT('Ctrl Pts',(-7.00799757267363,0.213533566214939,
12.7638952924001));
#158292=CARTESIAN_POINT('Ctrl Pts',(-7.01385463701134,0.0213094892736452,
12.7726299250499));
#158293=CARTESIAN_POINT('Ctrl Pts',(-7.01179924502979,-0.171179535379829,
12.7813645576996));
#158294=CARTESIAN_POINT('Ctrl Pts',(-7.00183185414267,-0.363286730851884,
12.7900991903494));
#158295=CARTESIAN_POINT('Ctrl Pts',(-6.991662983931,-0.5592771519767,12.799010383536));
#158296=CARTESIAN_POINT('Ctrl Pts',(-6.97325883762931,-0.754869851934066,
12.8079215767226));
#158297=CARTESIAN_POINT('Ctrl Pts',(-6.94667580252179,-0.949379722323063,
12.8168327699093));
#158298=CARTESIAN_POINT('Ctrl Pts',(-6.92009276741428,-1.14388959271204,
12.8257439630959));
#158299=CARTESIAN_POINT('Ctrl Pts',(-6.88533087119722,-1.33731633137024,
12.8346551562825));
#158300=CARTESIAN_POINT('Ctrl Pts',(-6.84250272341955,-1.52898104713437,
12.8435663494692));
#158301=CARTESIAN_POINT('Ctrl Pts',(-6.80393051955038,-1.70159954395467,
12.8515920143216));
#158302=CARTESIAN_POINT('Ctrl Pts',(-6.75879730526915,-1.87286802781277,
12.859617679174));
#158303=CARTESIAN_POINT('Ctrl Pts',(-6.7072239494188,-2.04224715811845,
12.8676433440264));
#158304=CARTESIAN_POINT('Ctrl Pts',(-6.65566696168666,-2.21157253164253,
12.8756664617296));
#158305=CARTESIAN_POINT('Ctrl Pts',(-6.59767400833211,-2.37900939517207,
12.8836895794328));
#158306=CARTESIAN_POINT('Ctrl Pts',(-6.53341630104245,-2.54403183937876,
12.891712697136));
#158307=CARTESIAN_POINT('Ctrl Pts',(-6.46916669721183,-2.70903347281152,
12.8997348030539));
#158308=CARTESIAN_POINT('Ctrl Pts',(-6.39865404663914,-2.87162095213325,
12.9077569089718));
#158309=CARTESIAN_POINT('Ctrl Pts',(-6.32209833132922,-3.03128673198435,
12.9157790148897));
#158310=CARTESIAN_POINT('Ctrl Pts',(-6.24551416765691,-3.19101184417854,
12.9238041018492));
#158311=CARTESIAN_POINT('Ctrl Pts',(-6.16288260913011,-3.34781275584398,
12.9318291888088));
#158312=CARTESIAN_POINT('Ctrl Pts',(-6.0744705924461,-3.50120459042421,
12.9398542757683));
#158313=CARTESIAN_POINT('Ctrl Pts',(-5.98604116345816,-3.65462663475809,
12.9478809432285));
#158314=CARTESIAN_POINT('Ctrl Pts',(-5.89182919905072,-3.80463795127912,
12.9559076106888));
#158315=CARTESIAN_POINT('Ctrl Pts',(-5.79214579397796,-3.95078139914163,
12.963934278149));
#158316=CARTESIAN_POINT('Ctrl Pts',(-5.69238236341871,-4.09704217044933,
12.9719673893896));
#158317=CARTESIAN_POINT('Ctrl Pts',(-5.58713893356198,-4.23942857387815,
12.9800005006302));
#158318=CARTESIAN_POINT('Ctrl Pts',(-5.47676819497516,-4.37751490014695,
12.9880336118708));
#158319=CARTESIAN_POINT('Ctrl Pts',(-5.41173374636398,-4.458880379844,12.9927670128324));
#158320=CARTESIAN_POINT('Ctrl Pts',(-5.34491985473411,-4.53875351224123,
12.997500413794));
#158321=CARTESIAN_POINT('Ctrl Pts',(-5.27640478678752,-4.61705307403605,
13.0022338147557));
#158322=CARTESIAN_POINT('Ctrl Pts',(-5.13526161448851,-4.77835260817588,
13.0119847680498));
#158323=CARTESIAN_POINT('Ctrl Pts',(-4.98681445036669,-4.93306789468406,
13.0217357213439));
#158324=CARTESIAN_POINT('Ctrl Pts',(-4.83164907454465,-5.08062927037113,
13.031486674638));
#158325=CARTESIAN_POINT('Ctrl Pts',(-4.67626015388893,-5.22840323590313,
13.0412516760096));
#158326=CARTESIAN_POINT('Ctrl Pts',(-4.5141336889914,-5.36900264785623,
13.0510166773813));
#158327=CARTESIAN_POINT('Ctrl Pts',(-4.34589168468698,-5.50189531229636,
13.0607816787529));
#158328=CARTESIAN_POINT('Ctrl Pts',(-4.17793010494584,-5.63456647219875,
13.0705304038905));
#158329=CARTESIAN_POINT('Ctrl Pts',(-4.0038733878872,-5.75955653413059,
13.080279129028));
#158330=CARTESIAN_POINT('Ctrl Pts',(-3.82437342942543,-5.8763759609818,
13.0900278541656));
#158331=CARTESIAN_POINT('Ctrl Pts',(-3.6453661287486,-5.992874763803,13.0997498228327));
#158332=CARTESIAN_POINT('Ctrl Pts',(-3.46094544458197,-6.10124767805766,
13.1094717914998));
#158333=CARTESIAN_POINT('Ctrl Pts',(-3.27179036988941,-6.20104945456807,
13.1191937601669));
#158334=CARTESIAN_POINT('Ctrl Pts',(-3.08388688492214,-6.30019086878977,
13.1288514011066));
#158335=CARTESIAN_POINT('Ctrl Pts',(-2.89131148259919,-6.39087414900364,
13.1385090420462));
#158336=CARTESIAN_POINT('Ctrl Pts',(-2.69476145185496,-6.47270324362987,
13.1481666829859));
#158337=CARTESIAN_POINT('Ctrl Pts',(-2.60837094653578,-6.50866994792293,
13.1524115486713));
#158338=CARTESIAN_POINT('Ctrl Pts',(-2.52121299160725,-6.54292663910667,
13.1566564143567));
#158339=CARTESIAN_POINT('Ctrl Pts',(-2.43334873421041,-6.57544222849054,
13.1609012800421));
#158340=CARTESIAN_POINT('Ctrl Pts',(-2.27082375504671,-6.63558722537181,
13.168753127056));
#158341=CARTESIAN_POINT('Ctrl Pts',(-2.10594760139337,-6.6897467859166,
13.1766049740699));
#158342=CARTESIAN_POINT('Ctrl Pts',(-1.93922005044379,-6.73773345854945,
13.1844568210838));
#158343=CARTESIAN_POINT('Ctrl Pts',(-1.77253978207964,-6.78570652254993,
13.1923064413773));
#158344=CARTESIAN_POINT('Ctrl Pts',(-1.60400952703719,-6.82751007543977,
13.2001560616709));
#158345=CARTESIAN_POINT('Ctrl Pts',(-1.43414529570925,-6.86300618047915,
13.2080056819645));
#158346=CARTESIAN_POINT('Ctrl Pts',(-1.2642946258674,-6.89849945160859,
13.2158546755663));
#158347=CARTESIAN_POINT('Ctrl Pts',(-1.09311056530598,-6.92768620006069,
13.2237036691681));
#158348=CARTESIAN_POINT('Ctrl Pts',(-0.921120155848448,-6.9504794238232,
13.2315526627699));
#158349=CARTESIAN_POINT('Ctrl Pts',(-0.749042672683,-6.97328418712746,13.2394056300873));
#158350=CARTESIAN_POINT('Ctrl Pts',(-0.576158403606521,-6.98968890816385,
13.2472585974048));
#158351=CARTESIAN_POINT('Ctrl Pts',(-0.40300071038223,-6.9996583480861,
13.2551115647222));
#158352=CARTESIAN_POINT('Ctrl Pts',(-0.229799040923113,-7.00963031991105,
13.2629665264294));
#158353=CARTESIAN_POINT('Ctrl Pts',(-0.0563241904046526,-7.01316374685499,
13.2708214881366));
#158354=CARTESIAN_POINT('Ctrl Pts',(0.116890273251932,-7.01027554569142,
13.2786764498438));
#158355=CARTESIAN_POINT('Ctrl Pts',(0.290276666743483,-7.00738447774676,
13.2865392082572));
#158356=CARTESIAN_POINT('Ctrl Pts',(0.463401776424912,-6.99805907169667,
13.2944019666705));
#158357=CARTESIAN_POINT('Ctrl Pts',(0.63573636881906,-6.982368210848,13.3022647250838));
#158358=CARTESIAN_POINT('Ctrl Pts',(0.762158552946482,-6.97085762047976,
13.3080327318321));
#158359=CARTESIAN_POINT('Ctrl Pts',(0.888155422117685,-6.95592256172403,
13.3138007385803));
#158360=CARTESIAN_POINT('Ctrl Pts',(1.01352184654488,-6.9376076589179,13.3195687453285));
#158361=CARTESIAN_POINT('Ctrl Pts',(1.19561737437144,-6.91100514625302,
13.3279468117695));
#158362=CARTESIAN_POINT('Ctrl Pts',(1.37678580379762,-6.87721132586113,
13.3363248782105));
#158363=CARTESIAN_POINT('Ctrl Pts',(1.55643888652931,-6.83630927877019,
13.3447029446515));
#158364=CARTESIAN_POINT('Ctrl Pts',(1.7359691246174,-6.79543520001312,13.3530752822702));
#158365=CARTESIAN_POINT('Ctrl Pts',(1.91398576233902,-6.74746265773913,
13.361447619889));
#158366=CARTESIAN_POINT('Ctrl Pts',(2.08990965660702,-6.69252599469892,
13.3698199575077));
#158367=CARTESIAN_POINT('Ctrl Pts',(2.26573905556167,-6.63761884019824,
13.3781877980302));
#158368=CARTESIAN_POINT('Ctrl Pts',(2.43947763931422,-6.57575512128009,
13.3865556385528));
#158369=CARTESIAN_POINT('Ctrl Pts',(2.61055992599276,-6.50711944221871,
13.3949234790754));
#158370=CARTESIAN_POINT('Ctrl Pts',(2.78157538028006,-6.43851057532266,
13.4032880507453));
#158371=CARTESIAN_POINT('Ctrl Pts',(2.94993630212466,-6.36313514586109,
13.4116526224152));
#158372=CARTESIAN_POINT('Ctrl Pts',(3.11509531742393,-6.28122660997544,
13.420017194085));
#158373=CARTESIAN_POINT('Ctrl Pts',(3.28021398952132,-6.19933808179322,
13.4283797225507));
#158374=CARTESIAN_POINT('Ctrl Pts',(3.4421320208106,-6.11091977595823,13.4367422510163));
#158375=CARTESIAN_POINT('Ctrl Pts',(3.60032444524996,-6.01625219313782,
13.4451047794819));
#158376=CARTESIAN_POINT('Ctrl Pts',(3.75852949393871,-5.92157705554871,
13.4534679753035));
#158377=CARTESIAN_POINT('Ctrl Pts',(3.91300805665509,-5.82065180820859,
13.461831171125));
#158378=CARTESIAN_POINT('Ctrl Pts',(4.06326143054084,-5.71380198375646,
13.4701943669465));
#158379=CARTESIAN_POINT('Ctrl Pts',(4.21352505140549,-5.60694487236049,
13.4785581331212));
#158380=CARTESIAN_POINT('Ctrl Pts',(4.35956264076597,-5.49416256856747,
13.4869218992959));
#158381=CARTESIAN_POINT('Ctrl Pts',(4.50090591956166,-5.37582295706944,
13.4952856654706));
#158382=CARTESIAN_POINT('Ctrl Pts',(4.64227768206981,-5.25745949759296,
13.5036511171242));
#158383=CARTESIAN_POINT('Ctrl Pts',(4.77895299557132,-5.13353670834518,
13.5120165687777));
#158384=CARTESIAN_POINT('Ctrl Pts',(4.91049768391706,-5.00446191500597,
13.5203820204313));
#158385=CARTESIAN_POINT('Ctrl Pts',(5.04208642632047,-4.87534389477207,
13.5287502736582));
#158386=CARTESIAN_POINT('Ctrl Pts',(5.16854088277218,-4.74107066013836,
13.5371185268851));
#158387=CARTESIAN_POINT('Ctrl Pts',(5.28946437627122,-4.60208574177597,
13.545486780112));
#158388=CARTESIAN_POINT('Ctrl Pts',(5.4104999831,-4.46297196456631,13.5538627919035));
#158389=CARTESIAN_POINT('Ctrl Pts',(5.52599416368704,-4.31913802255477,
13.562238803695));
#158390=CARTESIAN_POINT('Ctrl Pts',(5.6355903443491,-4.17106078032666,13.5706148154865));
#158391=CARTESIAN_POINT('Ctrl Pts',(5.74524027233254,-4.02291091918902,
13.5789949349776));
#158392=CARTESIAN_POINT('Ctrl Pts',(5.84898624206894,-3.87051387598069,
13.5873750544688));
#158393=CARTESIAN_POINT('Ctrl Pts',(5.94651519299269,-3.7143752667181,13.59575517396));
#158394=CARTESIAN_POINT('Ctrl Pts',(6.04415558309701,-3.55805824931611,
13.6041448687992));
#158395=CARTESIAN_POINT('Ctrl Pts',(6.13556459098721,-3.39799140545235,
13.6125345636384));
#158396=CARTESIAN_POINT('Ctrl Pts',(6.22047462004988,-3.23470586975312,
13.6209242584776));
#158397=CARTESIAN_POINT('Ctrl Pts',(6.27438253223083,-3.13103870091497,
13.6262507309522));
#158398=CARTESIAN_POINT('Ctrl Pts',(6.32567180420849,-3.02607461810334,
13.6315772034268));
#158399=CARTESIAN_POINT('Ctrl Pts',(6.37428404911066,-2.91995366808336,
13.6369036759013));
#158400=CARTESIAN_POINT('Ctrl Pts',(6.45225519315827,-2.74974198793713,
13.6454470203491));
#158401=CARTESIAN_POINT('Ctrl Pts',(6.52348723065363,-2.57622528567362,
13.6539903647969));
#158402=CARTESIAN_POINT('Ctrl Pts',(6.58770463527921,-2.3999529580433,13.6625337092447));
#158403=CARTESIAN_POINT('Ctrl Pts',(6.65182696371074,-2.22394160798015,
13.6710644049616));
#158404=CARTESIAN_POINT('Ctrl Pts',(6.70895526197059,-2.04518305176247,
13.6795951006784));
#158405=CARTESIAN_POINT('Ctrl Pts',(6.75886111797927,-1.86424862890337,
13.6881257963953));
#158406=CARTESIAN_POINT('Ctrl Pts',(6.80867084795871,-1.68366271239224,
13.6966400607357));
#158407=CARTESIAN_POINT('Ctrl Pts',(6.85128580808707,-1.50090958292236,
13.7051543250761));
#158408=CARTESIAN_POINT('Ctrl Pts',(6.88652671837764,-1.31657750230319,
13.7136685894165));
#158409=CARTESIAN_POINT('Ctrl Pts',(6.92172656359226,-1.13246021780667,
13.7221729323641));
#158410=CARTESIAN_POINT('Ctrl Pts',(6.9495694307345,-0.946767947700473,
13.7306772753118));
#158411=CARTESIAN_POINT('Ctrl Pts',(6.96992612818737,-0.760102841799044,
13.7391816182595));
#158412=CARTESIAN_POINT('Ctrl Pts',(6.9902529427843,-0.573711753158142,
13.7476734771559));
#158413=CARTESIAN_POINT('Ctrl Pts',(7.00311547628919,-0.386350979474767,
13.7561653360522));
#158414=CARTESIAN_POINT('Ctrl Pts',(7.00843577920027,-0.198631546652243,
13.7646571949486));
#158415=CARTESIAN_POINT('Ctrl Pts',(7.01028967994043,-0.133219256925804,
13.7676162489266));
#158416=CARTESIAN_POINT('Ctrl Pts',(7.01122823789861,-0.0677634995192813,
13.7705753029046));
#158417=CARTESIAN_POINT('Ctrl Pts',(7.0112496259069,-0.0022903537530466,
13.7735343568827));
#158418=CARTESIAN_POINT('Ctrl Pts',(7.01124962590711,-0.00229035313711163,
13.7735343569105));
#158419=CARTESIAN_POINT('Ctrl Pts',(7.01130271976769,0.160241050471527,
13.7808799516696));
#158420=CARTESIAN_POINT('Ctrl Pts',(7.00570090552392,0.322819188341013,
13.7882255464287));
#158421=CARTESIAN_POINT('Ctrl Pts',(6.99445468411544,0.485005396212896,
13.7955711411878));
#158422=CARTESIAN_POINT('Ctrl Pts',(6.98168692844655,0.669134251564195,
13.803910542994));
#158423=CARTESIAN_POINT('Ctrl Pts',(6.96164931566915,0.85268294976881,13.8122499448002));
#158424=CARTESIAN_POINT('Ctrl Pts',(6.93442680677069,1.03506107261361,13.8205893466064));
#158425=CARTESIAN_POINT('Ctrl Pts',(6.90719096826687,1.21752849760224,13.8289328318325));
#158426=CARTESIAN_POINT('Ctrl Pts',(6.87276327240065,1.39882388116677,13.8372763170586));
#158427=CARTESIAN_POINT('Ctrl Pts',(6.8312797859362,1.57836720973272,13.8456198022846));
#158428=CARTESIAN_POINT('Ctrl Pts',(6.78974908017936,1.75811490658233,13.8539727846264));
#158429=CARTESIAN_POINT('Ctrl Pts',(6.74114661530322,1.93610624538186,13.8623257669681));
#158430=CARTESIAN_POINT('Ctrl Pts',(6.6856586632065,2.11177527251172,13.8706787493098));
#158431=CARTESIAN_POINT('Ctrl Pts',(6.65025755758115,2.22385145390847,13.8760079207605));
#158432=CARTESIAN_POINT('Ctrl Pts',(6.61205478698717,2.33498270143529,13.8813370922111));
#158433=CARTESIAN_POINT('Ctrl Pts',(6.57110895151813,2.44502632087638,13.8866662636617));
#158434=CARTESIAN_POINT('',(7.0112498931807,0.00122387650393776,13.2264656430896));
#158435=CARTESIAN_POINT('Ctrl Pts',(6.57110895151813,2.44502632087638,13.3398632123397));
#158436=CARTESIAN_POINT('Ctrl Pts',(6.6012849092065,2.36392719159765,13.3359311695798));
#158437=CARTESIAN_POINT('Ctrl Pts',(6.62995846650225,2.28227170996608,13.3319991268199));
#158438=CARTESIAN_POINT('Ctrl Pts',(6.6571103512001,2.20011552752226,13.32806708406));
#158439=CARTESIAN_POINT('Ctrl Pts',(6.71682758851922,2.01942308945293,13.319419038694));
#158440=CARTESIAN_POINT('Ctrl Pts',(6.76919104950635,1.8362765019726,13.3107709933279));
#158441=CARTESIAN_POINT('Ctrl Pts',(6.81402159556527,1.65128321546308,13.3021229479618));
#158442=CARTESIAN_POINT('Ctrl Pts',(6.85884212225374,1.46633127389431,13.2934768353844));
#158443=CARTESIAN_POINT('Ctrl Pts',(6.89613302745317,1.27953373815494,13.2848307228069));
#158444=CARTESIAN_POINT('Ctrl Pts',(6.92576572928521,1.09151070794493,13.2761846102295));
#158445=CARTESIAN_POINT('Ctrl Pts',(6.95539404940694,0.90351548020988,13.2675397761302));
#158446=CARTESIAN_POINT('Ctrl Pts',(6.97736638061505,0.71429540499206,13.2588949420308));
#158447=CARTESIAN_POINT('Ctrl Pts',(6.99160555274134,0.524479129590983,
13.2502501079315));
#158448=CARTESIAN_POINT('Ctrl Pts',(7.00466426059404,0.350399115376199,
13.2423219529842));
#158449=CARTESIAN_POINT('Ctrl Pts',(7.01121941622546,0.175817921308749,
13.2343937980369));
#158450=CARTESIAN_POINT('Ctrl Pts',(7.0112498931807,0.00122387650393776,
13.2264656430896));
#158451=CARTESIAN_POINT('Ctrl Pts',(7.0112498931807,0.00122387650393776,
13.2264656430896));
#158452=CARTESIAN_POINT('Ctrl Pts',(7.01128645483302,-0.208227714535047,
13.216954639037));
#158453=CARTESIAN_POINT('Ctrl Pts',(7.00193253296366,-0.417672943101247,
13.2074436349843));
#158454=CARTESIAN_POINT('Ctrl Pts',(6.98321925767691,-0.626318897775246,
13.1979326309316));
#158455=CARTESIAN_POINT('Ctrl Pts',(6.96450598239015,-0.834964852449244,
13.1884216268789));
#158456=CARTESIAN_POINT('Ctrl Pts',(6.93643335324898,-1.04281133667803,
13.1789106228262));
#158457=CARTESIAN_POINT('Ctrl Pts',(6.89909079732579,-1.24906874620839,
13.1693996187735));
#158458=CARTESIAN_POINT('Ctrl Pts',(6.86758005073053,-1.42311481253751,
13.1613739539212));
#158459=CARTESIAN_POINT('Ctrl Pts',(6.82945876018241,-1.59607916667199,
13.1533482890688));
#158460=CARTESIAN_POINT('Ctrl Pts',(6.78482573095118,-1.76741799332325,
13.1453226242164));
#158461=CARTESIAN_POINT('Ctrl Pts',(6.74020686714869,-1.93870244123346,
13.1372995065132));
#158462=CARTESIAN_POINT('Ctrl Pts',(6.68908047149763,-2.10836203446348,
13.12927638881));
#158463=CARTESIAN_POINT('Ctrl Pts',(6.63159619730733,-2.27586432775746,
13.1212532711068));
#158464=CARTESIAN_POINT('Ctrl Pts',(6.57411917238709,-2.44334549754637,
13.113231165189));
#158465=CARTESIAN_POINT('Ctrl Pts',(6.51028598550464,-2.60866956286985,
13.1052090592711));
#158466=CARTESIAN_POINT('Ctrl Pts',(6.44029576765884,-2.77132044115719,
13.0971869533533));
#158467=CARTESIAN_POINT('Ctrl Pts',(6.37027954121157,-2.93403176106052,
13.0891618663938));
#158468=CARTESIAN_POINT('Ctrl Pts',(6.29410185542612,-3.09406757127754,
13.0811367794343));
#158469=CARTESIAN_POINT('Ctrl Pts',(6.21200968017546,-3.25093252712301,
13.0731116924748));
#158470=CARTESIAN_POINT('Ctrl Pts',(6.12990133728169,-3.40782837673656,
13.0650850250146));
#158471=CARTESIAN_POINT('Ctrl Pts',(6.04187636216168,-3.56155180721156,
13.0570583575544));
#158472=CARTESIAN_POINT('Ctrl Pts',(5.94822697558419,-3.71163338833897,
13.0490316900942));
#158473=CARTESIAN_POINT('Ctrl Pts',(5.8545024076091,-3.86183545443092,13.0409985788536));
#158474=CARTESIAN_POINT('Ctrl Pts',(5.75514461197914,-4.0083895258752,13.032965467613));
#158475=CARTESIAN_POINT('Ctrl Pts',(5.65048865074503,-4.15085588406797,
13.0249323563724));
#158476=CARTESIAN_POINT('Ctrl Pts',(5.58882155654904,-4.23480223769019,
13.0201989554107));
#158477=CARTESIAN_POINT('Ctrl Pts',(5.52531572324001,-4.3173299453401,13.0154655544489));
#158478=CARTESIAN_POINT('Ctrl Pts',(5.46004604497905,-4.39835466387247,
13.0107321534872));
#158479=CARTESIAN_POINT('Ctrl Pts',(5.32558847643832,-4.56526810570072,
13.000981200193));
#158480=CARTESIAN_POINT('Ctrl Pts',(5.18356484757897,-4.72590019857516,
12.9912302468989));
#158481=CARTESIAN_POINT('Ctrl Pts',(5.03453725449078,-4.87965789739859,
12.9814792936047));
#158482=CARTESIAN_POINT('Ctrl Pts',(4.8852949591962,-5.03363711303312,12.971714292233));
#158483=CARTESIAN_POINT('Ctrl Pts',(4.72902854254238,-5.18072209625207,
12.9619492908613));
#158484=CARTESIAN_POINT('Ctrl Pts',(4.56633782112557,-5.32035576497081,
12.9521842894896));
#158485=CARTESIAN_POINT('Ctrl Pts',(4.40391827143435,-5.45975669329375,
12.942435564352));
#158486=CARTESIAN_POINT('Ctrl Pts',(4.23509584666012,-5.59173110455787,
12.9326868392144));
#158487=CARTESIAN_POINT('Ctrl Pts',(4.06050196677742,-5.71576332087821,
12.9229381140768));
#158488=CARTESIAN_POINT('Ctrl Pts',(3.88638727939536,-5.83945511685885,
12.9132161454096));
#158489=CARTESIAN_POINT('Ctrl Pts',(3.7065327922419,-5.95524821140251,12.9034941767424));
#158490=CARTESIAN_POINT('Ctrl Pts',(3.52159880338043,-6.06267007435911,
12.8937722080752));
#158491=CARTESIAN_POINT('Ctrl Pts',(3.33788847442183,-6.16938115490519,
12.8841145671355));
#158492=CARTESIAN_POINT('Ctrl Pts',(3.14916566690129,-6.26783136979799,
12.8744569261958));
#158493=CARTESIAN_POINT('Ctrl Pts',(2.95611096312666,-6.35759660061743,
12.864799285256));
#158494=CARTESIAN_POINT('Ctrl Pts',(2.8712567743537,-6.3970515099891,12.8605544195709));
#158495=CARTESIAN_POINT('Ctrl Pts',(2.78556613652069,-6.43482907720547,
12.8563095538858));
#158496=CARTESIAN_POINT('Ctrl Pts',(2.69909888003669,-6.47089574929814,
12.8520646882007));
#158497=CARTESIAN_POINT('Ctrl Pts',(2.53915797259935,-6.53760928338389,
12.8442128411868));
#158498=CARTESIAN_POINT('Ctrl Pts',(2.37662409889338,-6.59843809185593,
12.8363609941729));
#158499=CARTESIAN_POINT('Ctrl Pts',(2.21198898804205,-6.6531745264408,12.828509147159));
#158500=CARTESIAN_POINT('Ctrl Pts',(2.04740056637714,-6.70789543821534,
12.8206595268654));
#158501=CARTESIAN_POINT('Ctrl Pts',(1.88071245452658,-6.75652729265902,
12.8128099065718));
#158502=CARTESIAN_POINT('Ctrl Pts',(1.7124346177168,-6.79891125420424,12.8049602862782));
#158503=CARTESIAN_POINT('Ctrl Pts',(1.5441702157396,-6.84129183193233,12.7971112926764));
#158504=CARTESIAN_POINT('Ctrl Pts',(1.37431671155877,-6.8774254173219,12.7892622990746));
#158505=CARTESIAN_POINT('Ctrl Pts',(1.20339716687151,-6.90720361805453,
12.7814133054728));
#158506=CARTESIAN_POINT('Ctrl Pts',(1.03239109062408,-6.93699689461816,
12.7735603381554));
#158507=CARTESIAN_POINT('Ctrl Pts',(0.860318271805542,-6.96042829214932,
12.7657073708379));
#158508=CARTESIAN_POINT('Ctrl Pts',(0.687710194737447,-6.97744088119378,
12.7578544035205));
#158509=CARTESIAN_POINT('Ctrl Pts',(0.515058281017167,-6.99445779086425,
12.7499994418132));
#158510=CARTESIAN_POINT('Ctrl Pts',(0.341871219025297,-7.00505262108919,
12.742144480106));
#158511=CARTESIAN_POINT('Ctrl Pts',(0.168682822978939,-7.00922054637546,
12.7342895183987));
#158512=CARTESIAN_POINT('Ctrl Pts',(-0.00467747702693838,-7.01339260867596,
12.7264267599853));
#158513=CARTESIAN_POINT('Ctrl Pts',(-0.178038732466307,-7.011125030057,
12.718564001572));
#158514=CARTESIAN_POINT('Ctrl Pts',(-0.350869343762094,-7.00246508496172,
12.7107012431586));
#158515=CARTESIAN_POINT('Ctrl Pts',(-0.477655400235681,-6.99611227350271,
12.7049332364105));
#158516=CARTESIAN_POINT('Ctrl Pts',(-0.604155947560724,-6.98632051437413,
12.6991652296624));
#158517=CARTESIAN_POINT('Ctrl Pts',(-0.730164208890093,-6.97312604149358,
12.6933972229143));
#158518=CARTESIAN_POINT('Ctrl Pts',(-0.913192008897945,-6.95396098582093,
12.6850191564733));
#158519=CARTESIAN_POINT('Ctrl Pts',(-1.09558632776216,-6.92757283386555,
12.6766410900323));
#158520=CARTESIAN_POINT('Ctrl Pts',(-1.27675602187481,-6.89402064278215,
12.6682630235912));
#158521=CARTESIAN_POINT('Ctrl Pts',(-1.4578018343029,-6.86049139428842,
12.6598906859725));
#158522=CARTESIAN_POINT('Ctrl Pts',(-1.6376243692774,-6.81980793286507,
12.6515183483538));
#158523=CARTESIAN_POINT('Ctrl Pts',(-1.81563949333761,-6.77208090565469,
12.6431460107351));
#158524=CARTESIAN_POINT('Ctrl Pts',(-1.99355899880669,-6.72437951441835,
12.6347781702125));
#158525=CARTESIAN_POINT('Ctrl Pts',(-2.16967271229991,-6.66964218599894,
12.6264103296899));
#158526=CARTESIAN_POINT('Ctrl Pts',(-2.34340810346346,-6.60803034368955,
12.6180424891673));
#158527=CARTESIAN_POINT('Ctrl Pts',(-2.51707562581395,-6.54644256972099,
12.6096779174974));
#158528=CARTESIAN_POINT('Ctrl Pts',(-2.68836636919932,-6.47798574682312,
12.6013133458275));
#158529=CARTESIAN_POINT('Ctrl Pts',(-2.85672390664315,-6.40287084702741,
12.5929487741577));
#158530=CARTESIAN_POINT('Ctrl Pts',(-3.02504031958462,-6.32777429546202,
12.5845862456921));
#158531=CARTESIAN_POINT('Ctrl Pts',(-3.19042465571586,-6.24602304455298,
12.5762237172265));
#158532=CARTESIAN_POINT('Ctrl Pts',(-3.35234096176165,-6.1578759843468,
12.567861188761));
#158533=CARTESIAN_POINT('Ctrl Pts',(-3.51427018923537,-6.06972188972936,
12.5594979929395));
#158534=CARTESIAN_POINT('Ctrl Pts',(-3.67273054214267,-5.97517111793979,
12.551134797118));
#158535=CARTESIAN_POINT('Ctrl Pts',(-3.82721047479072,-5.8745286231452,
12.5427716012965));
#158536=CARTESIAN_POINT('Ctrl Pts',(-3.98170094266064,-5.77387926473412,
12.5344078351218));
#158537=CARTESIAN_POINT('Ctrl Pts',(-4.13221017335271,-5.66713753422754,
12.5260440689471));
#158538=CARTESIAN_POINT('Ctrl Pts',(-4.27825529505239,-5.5546519416482,
12.5176803027724));
#158539=CARTESIAN_POINT('Ctrl Pts',(-4.4243298479869,-5.44214368080134,
12.5093148511188));
#158540=CARTESIAN_POINT('Ctrl Pts',(-4.56593823760468,-5.32388945041,12.5009493994652));
#158541=CARTESIAN_POINT('Ctrl Pts',(-4.7026300605774,-5.20027855752496,
12.4925839478117));
#158542=CARTESIAN_POINT('Ctrl Pts',(-4.83936766137271,-5.07662626759507,
12.4842156945848));
#158543=CARTESIAN_POINT('Ctrl Pts',(-4.97118516849557,-4.94761395844923,
12.4758474413579));
#158544=CARTESIAN_POINT('Ctrl Pts',(-5.0976681723013,-4.81366863915729,
12.467479188131));
#158545=CARTESIAN_POINT('Ctrl Pts',(-5.22426844389627,-4.67959913344503,
12.4591031763396));
#158546=CARTESIAN_POINT('Ctrl Pts',(-5.34552410293513,-4.54058771745697,
12.4507271645481));
#158547=CARTESIAN_POINT('Ctrl Pts',(-5.46105945238373,-4.39709633963487,
12.4423511527566));
#158548=CARTESIAN_POINT('Ctrl Pts',(-5.57665146179558,-4.2535345918677,
12.4339710332655));
#158549=CARTESIAN_POINT('Ctrl Pts',(-5.68651736631649,-4.10548876099445,
12.4255909137743));
#158550=CARTESIAN_POINT('Ctrl Pts',(-5.79032377510463,-3.95345129500264,
12.4172107942831));
#158551=CARTESIAN_POINT('Ctrl Pts',(-5.89424879586417,-3.80124010694706,
12.4088210994439));
#158552=CARTESIAN_POINT('Ctrl Pts',(-5.99210030578865,-3.64502844530348,
12.4004314046047));
#158553=CARTESIAN_POINT('Ctrl Pts',(-6.0835893010936,-3.48533610690842,
12.3920417097655));
#158554=CARTESIAN_POINT('Ctrl Pts',(-6.14167408541145,-3.38395019702961,
12.3867152372908));
#158555=CARTESIAN_POINT('Ctrl Pts',(-6.19719521531832,-3.28116181132902,
12.3813887648161));
#158556=CARTESIAN_POINT('Ctrl Pts',(-6.25008864931608,-3.17710850274118,
12.3760622923414));
#158557=CARTESIAN_POINT('Ctrl Pts',(-6.3333174206817,-3.01337874697112,
12.3676809919366));
#158558=CARTESIAN_POINT('Ctrl Pts',(-6.41020567117949,-2.84618575687497,
12.3592996915317));
#158559=CARTESIAN_POINT('Ctrl Pts',(-6.48046315699108,-2.67604630628494,
12.3509183911268));
#158560=CARTESIAN_POINT('Ctrl Pts',(-6.55063160172435,-2.50612248254191,
12.3425477127933));
#158561=CARTESIAN_POINT('Ctrl Pts',(-6.61418590507734,-2.33325994058392,
12.3341770344597));
#158562=CARTESIAN_POINT('Ctrl Pts',(-6.67088178962721,-2.15799970141799,
12.3258063561262));
#158563=CARTESIAN_POINT('Ctrl Pts',(-6.72751333408258,-1.982938352532,12.3174451770753));
#158564=CARTESIAN_POINT('Ctrl Pts',(-6.77730187212974,-1.8054850394893,
12.3090839980245));
#158565=CARTESIAN_POINT('Ctrl Pts',(-6.82005113331303,-1.62620081831723,
12.3007228189736));
#158566=CARTESIAN_POINT('Ctrl Pts',(-6.86274492228703,-1.44714923957134,
12.2923724895389));
#158567=CARTESIAN_POINT('Ctrl Pts',(-6.89841757807405,-1.2662718087306,
12.2840221601042));
#158568=CARTESIAN_POINT('Ctrl Pts',(-6.92692260572578,-1.08414472132883,
12.2756718306695));
#158569=CARTESIAN_POINT('Ctrl Pts',(-6.95540570046406,-0.902157769824967,
12.2673279263137));
#158570=CARTESIAN_POINT('Ctrl Pts',(-6.97673210713019,-0.718923400261605,
12.258984021958));
#158571=CARTESIAN_POINT('Ctrl Pts',(-6.99080613463866,-0.535029111729923,
12.2506401176022));
#158572=CARTESIAN_POINT('Ctrl Pts',(-7.00486885780036,-0.351282528239018,
12.2423029151225));
#158573=CARTESIAN_POINT('Ctrl Pts',(-7.01169079431758,-0.166877408640384,
12.2339657126428));
#158574=CARTESIAN_POINT('Ctrl Pts',(-7.01122792897932,0.0175923392535826,
12.2256285101631));
#158575=CARTESIAN_POINT('Ctrl Pts',(-7.01107555626492,0.0783187620109528,
12.2228839491271));
#158576=CARTESIAN_POINT('Ctrl Pts',(-7.01013415446048,0.139052146388286,
12.2201393880911));
#158577=CARTESIAN_POINT('Ctrl Pts',(-7.00840338632723,0.199771211682296,
12.217394827055));
#158578=CARTESIAN_POINT('Ctrl Pts',(-7.00314510219136,0.384243118488874,
12.2090565167531));
#158579=CARTESIAN_POINT('Ctrl Pts',(-6.9906012745149,0.568431470743603,
12.2007182064512));
#158580=CARTESIAN_POINT('Ctrl Pts',(-6.97083272321711,0.751743112655893,
12.1923798961493));
#158581=CARTESIAN_POINT('Ctrl Pts',(-6.95105173421761,0.935170088033341,
12.1840363396655));
#158582=CARTESIAN_POINT('Ctrl Pts',(-6.92403699006066,1.11771892707913,
12.1756927831817));
#158583=CARTESIAN_POINT('Ctrl Pts',(-6.88990082146475,1.2988045399056,12.1673492266979));
#158584=CARTESIAN_POINT('Ctrl Pts',(-6.85573868222082,1.48002792187567,
12.1589993224727));
#158585=CARTESIAN_POINT('Ctrl Pts',(-6.814444372126,1.65978553550783,12.1506494182475));
#158586=CARTESIAN_POINT('Ctrl Pts',(-6.76618076614808,1.83750493939686,
12.1422995140224));
#158587=CARTESIAN_POINT('Ctrl Pts',(-6.71784476833251,2.01549090924115,
12.1339370855587));
#158588=CARTESIAN_POINT('Ctrl Pts',(-6.66251867134186,2.19143224369496,
12.1255746570951));
#158589=CARTESIAN_POINT('Ctrl Pts',(-6.60041491324351,2.36477261814593,
12.1172122286315));
#158590=CARTESIAN_POINT('Ctrl Pts',(-6.53825804796553,2.5382612222481,12.1088426491515));
#158591=CARTESIAN_POINT('Ctrl Pts',(-6.46931207971429,2.70914412541343,
12.1004730696715));
#158592=CARTESIAN_POINT('Ctrl Pts',(-6.39383680120533,2.87688677602237,
12.0921034901915));
#158593=CARTESIAN_POINT('Ctrl Pts',(-6.31824511127568,3.044888149231,12.0837210016549));
#158594=CARTESIAN_POINT('Ctrl Pts',(-6.23610413273646,3.20973929851901,
12.0753385131184));
#158595=CARTESIAN_POINT('Ctrl Pts',(-6.14771929896308,3.37093072958447,
12.0669560245818));
#158596=CARTESIAN_POINT('Ctrl Pts',(-6.11879833308085,3.42367520710767,
12.0642131369774));
#158597=CARTESIAN_POINT('Ctrl Pts',(-6.08920917596683,3.47602807320811,
12.061470249373));
#158598=CARTESIAN_POINT('Ctrl Pts',(-6.05896350698819,3.52797219142744,
12.0587273617686));
#158599=CARTESIAN_POINT('Ctrl Pts',(-5.96644904131399,3.68685716584719,
12.0503375066358));
#158600=CARTESIAN_POINT('Ctrl Pts',(-5.8676022527814,3.84223642542365,12.041947651503));
#158601=CARTESIAN_POINT('Ctrl Pts',(-5.76271213654621,3.9935917910827,12.0335577963702));
#158602=CARTESIAN_POINT('Ctrl Pts',(-5.65791881144004,4.14480748813185,
12.0251756832781));
#158603=CARTESIAN_POINT('Ctrl Pts',(-5.5470934621099,4.29200642462559,12.0167935701861));
#158604=CARTESIAN_POINT('Ctrl Pts',(-5.43056966892561,4.43469724259111,
12.008411457094));
#158605=CARTESIAN_POINT('Ctrl Pts',(-5.31413627350797,4.57727736272478,
12.0000358467451));
#158606=CARTESIAN_POINT('Ctrl Pts',(-5.19201345511139,4.71535608326778,
11.9916602363962));
#158607=CARTESIAN_POINT('Ctrl Pts',(-5.06457682105126,4.8484727684262,11.9832846260474));
#158608=CARTESIAN_POINT('Ctrl Pts',(-4.93722034652608,4.98150572121318,
11.9749142840817));
#158609=CARTESIAN_POINT('Ctrl Pts',(-4.80455694765846,5.10958262515248,
11.9665439421161));
#158610=CARTESIAN_POINT('Ctrl Pts',(-4.66700135664109,5.23227721930043,
11.9581736001505));
#158611=CARTESIAN_POINT('Ctrl Pts',(-4.52951212602849,5.3549126223761,11.9498072962562));
#158612=CARTESIAN_POINT('Ctrl Pts',(-4.38713565460876,5.47217067521171,
11.9414409923618));
#158613=CARTESIAN_POINT('Ctrl Pts',(-4.2403225777862,5.58366286579129,11.9330746884675));
#158614=CARTESIAN_POINT('Ctrl Pts',(-4.09355056046649,5.69512387512997,
11.9247107243939));
#158615=CARTESIAN_POINT('Ctrl Pts',(-3.94234467250142,5.80082203787308,
11.9163467603203));
#158616=CARTESIAN_POINT('Ctrl Pts',(-3.78718802054721,5.90040960099583,
11.9079827962466));
#158617=CARTESIAN_POINT('Ctrl Pts',(-3.63205524462364,5.99998183924736,
11.8996201192481));
#158618=CARTESIAN_POINT('Ctrl Pts',(-3.47297319336155,6.0934451752122,11.8912574422496));
#158619=CARTESIAN_POINT('Ctrl Pts',(-3.31045364576519,6.18049538643465,
11.882894765251));
#158620=CARTESIAN_POINT('Ctrl Pts',(-3.1479374441493,6.26754380545233,11.8745322604248));
#158621=CARTESIAN_POINT('Ctrl Pts',(-2.98198417721538,6.34817920818327,
11.8661697555985));
#158622=CARTESIAN_POINT('Ctrl Pts',(-2.81313026979454,6.42214330637878,
11.8578072507722));
#158623=CARTESIAN_POINT('Ctrl Pts',(-2.64425733174284,6.49611574067661,
11.8494438034522));
#158624=CARTESIAN_POINT('Ctrl Pts',(-2.47248340266625,6.56341524002416,
11.8410803561322));
#158625=CARTESIAN_POINT('Ctrl Pts',(-2.29836532333641,6.62383147453079,
11.8327169088122));
#158626=CARTESIAN_POINT('Ctrl Pts',(-2.12414471838836,6.68428328381413,
11.8243485368594));
#158627=CARTESIAN_POINT('Ctrl Pts',(-1.94757751552225,6.73784362052027,
11.8159801649066));
#158628=CARTESIAN_POINT('Ctrl Pts',(-1.76923716564556,6.7843515839171,11.8076117929538));
#158629=CARTESIAN_POINT('Ctrl Pts',(-1.59084338033919,6.83087348231524,
11.7992409136181));
#158630=CARTESIAN_POINT('Ctrl Pts',(-1.41067570807971,6.87033871615299,
11.7908700342824));
#158631=CARTESIAN_POINT('Ctrl Pts',(-1.22931896518636,6.90263728181723,
11.7824991549466));
#158632=CARTESIAN_POINT('Ctrl Pts',(-1.04780856068579,6.93496321370691,
11.7741211830553));
#158633=CARTESIAN_POINT('Ctrl Pts',(-0.86510739717594,6.96011029163034,
11.7657432111641));
#158634=CARTESIAN_POINT('Ctrl Pts',(-0.681807762688048,6.97802011585223,
11.7573652392728));
#158635=CARTESIAN_POINT('Ctrl Pts',(-0.565319352356048,6.98940195498553,
11.7520409699138));
#158636=CARTESIAN_POINT('Ctrl Pts',(-0.448589341809831,6.99786192559897,
11.7467167005548));
#158637=CARTESIAN_POINT('Ctrl Pts',(-0.331770083393816,7.00339597440162,
11.7413924311957));
#158638=CARTESIAN_POINT('Ctrl Pts',(-0.159252495224037,7.01156860591114,
11.7335296000065));
#158639=CARTESIAN_POINT('Ctrl Pts',(0.0138185171071441,7.01337428630965,
11.7256667688172));
#158640=CARTESIAN_POINT('Ctrl Pts',(0.186913749324534,7.00875807920444,
11.7178039376279));
#158641=CARTESIAN_POINT('Ctrl Pts',(0.359875980703924,7.00414541904506,
11.7099471479865));
#158642=CARTESIAN_POINT('Ctrl Pts',(0.532862016288809,6.99312069419079,
11.7020903583451));
#158643=CARTESIAN_POINT('Ctrl Pts',(0.705338861365815,6.97568087380345,
11.6942335687038));
#158644=CARTESIAN_POINT('Ctrl Pts',(0.8777184376647,6.95825088864945,11.6863812099199));
#158645=CARTESIAN_POINT('Ctrl Pts',(1.04958901652641,6.93441304285293,11.6785288511361));
#158646=CARTESIAN_POINT('Ctrl Pts',(1.22041919639701,6.90421636013572,11.6706764923522));
#158647=CARTESIAN_POINT('Ctrl Pts',(1.3912090412712,6.87402680720722,11.6628259876018));
#158648=CARTESIAN_POINT('Ctrl Pts',(1.56095859948777,6.83748146354932,11.6549754828514));
#158649=CARTESIAN_POINT('Ctrl Pts',(1.72914324074419,6.79468102382214,11.6471249781009));
#158650=CARTESIAN_POINT('Ctrl Pts',(1.8973008263928,6.75188746933669,11.6392757362493));
#158651=CARTESIAN_POINT('Ctrl Pts',(2.06389362723065,6.70284091893477,11.6314264943976));
#158652=CARTESIAN_POINT('Ctrl Pts',(2.228409290684,6.647692727232,11.623577252546));
#158653=CARTESIAN_POINT('Ctrl Pts',(2.39298038268426,6.59252595502409,11.6157253661311));
#158654=CARTESIAN_POINT('Ctrl Pts',(2.55547257737388,6.53125355662401,11.6078734797163));
#158655=CARTESIAN_POINT('Ctrl Pts',(2.71539053085719,6.46407617741554,11.6000215933014));
#158656=CARTESIAN_POINT('Ctrl Pts',(2.8328162936427,6.41474866400218,11.5942560508374));
#158657=CARTESIAN_POINT('Ctrl Pts',(2.94885442458848,6.36223834779299,11.5884905083733));
#158658=CARTESIAN_POINT('Ctrl Pts',(3.06331649493972,6.30664083441655,11.5827249659093));
#158659=CARTESIAN_POINT('Ctrl Pts',(3.25500116881123,6.21353408571868,11.5730696615494));
#158660=CARTESIAN_POINT('Ctrl Pts',(3.44216773557614,6.11181628211994,11.5634143571894));
#158661=CARTESIAN_POINT('Ctrl Pts',(3.62414572571811,6.00193254887617,11.5537590528295));
#158662=CARTESIAN_POINT('Ctrl Pts',(3.80713183978237,5.89144008036685,11.5440502598949));
#158663=CARTESIAN_POINT('Ctrl Pts',(3.98487171840446,5.7726910273947,11.5343414669603));
#158664=CARTESIAN_POINT('Ctrl Pts',(4.15671982593661,5.64617630358507,11.5246326740258));
#158665=CARTESIAN_POINT('Ctrl Pts',(4.32939488115642,5.51905278018019,11.5148771615551));
#158666=CARTESIAN_POINT('Ctrl Pts',(4.49612130483396,5.38408871295277,11.5051216490844));
#158667=CARTESIAN_POINT('Ctrl Pts',(4.65628081751959,5.24181986631543,11.4953661366138));
#158668=CARTESIAN_POINT('Ctrl Pts',(4.8165989127633,5.09941015163187,11.4856009646848));
#158669=CARTESIAN_POINT('Ctrl Pts',(4.97033706978391,4.94968122399424,11.4758357927559));
#158670=CARTESIAN_POINT('Ctrl Pts',(5.11691201234755,4.79320748772608,11.466070620827));
#158671=CARTESIAN_POINT('Ctrl Pts',(5.2632871033026,4.63694709984714,11.4563187634885));
#158672=CARTESIAN_POINT('Ctrl Pts',(5.40251847437296,4.47396031134541,11.44656690615));
#158673=CARTESIAN_POINT('Ctrl Pts',(5.53406224469293,4.30485558809634,11.4368150488114));
#158674=CARTESIAN_POINT('Ctrl Pts',(5.59142485540756,4.23111368161041,11.4325625327485));
#158675=CARTESIAN_POINT('Ctrl Pts',(5.64732607623393,4.15620885907853,11.4283100166857));
#158676=CARTESIAN_POINT('Ctrl Pts',(5.70172304235996,4.08019373445936,11.4240575006228));
#158677=CARTESIAN_POINT('Ctrl Pts',(5.8044781167715,3.9366022744403,11.4160245598985));
#158678=CARTESIAN_POINT('Ctrl Pts',(5.90191268951564,3.78897669783169,11.4079916191741));
#158679=CARTESIAN_POINT('Ctrl Pts',(5.99369301470647,3.63775626010855,11.3999586784497));
#158680=CARTESIAN_POINT('Ctrl Pts',(6.08541671766824,3.48662911512809,11.3919306935044));
#158681=CARTESIAN_POINT('Ctrl Pts',(6.17149292580616,3.33191183475777,11.383902708559));
#158682=CARTESIAN_POINT('Ctrl Pts',(6.25163034420859,3.17407381796177,11.3758747236137));
#158683=CARTESIAN_POINT('Ctrl Pts',(6.33173144170547,3.01630733853015,11.3678503772143));
#158684=CARTESIAN_POINT('Ctrl Pts',(6.40589894333775,2.85542326519043,11.359826030815));
#158685=CARTESIAN_POINT('Ctrl Pts',(6.47388683555362,2.69191675260317,11.3518016844156));
#158686=CARTESIAN_POINT('Ctrl Pts',(6.50784377946204,2.610252484222,11.3477938784416));
#158687=CARTESIAN_POINT('Ctrl Pts',(6.54025990091052,2.52793441510125,11.3437860724676));
#158688=CARTESIAN_POINT('Ctrl Pts',(6.57110895151813,2.44502632087638,11.3397782664936));
#158689=CARTESIAN_POINT('Origin',(0.,0.,50.));
#158690=CARTESIAN_POINT('',(6.57110895151814,2.44502632087636,9.34006375887581));
#158691=CARTESIAN_POINT('',(6.57110895151814,2.44502632087636,9.88705365892876));
#158692=CARTESIAN_POINT('',(6.57110895151814,2.44502632087636,50.));
#158693=CARTESIAN_POINT('',(7.01124965431583,-0.00220167122712491,11.7735343569358));
#158694=CARTESIAN_POINT('Ctrl Pts',(6.57110895151814,2.44502632087636,9.88705365892876));
#158695=CARTESIAN_POINT('Ctrl Pts',(6.51065965303537,2.60748630054266,9.8949044975378));
#158696=CARTESIAN_POINT('Ctrl Pts',(6.44414243043556,2.7678078587859,9.90275533614685));
#158697=CARTESIAN_POINT('Ctrl Pts',(6.37174455141127,2.92549105861918,9.91060617475588));
#158698=CARTESIAN_POINT('Ctrl Pts',(6.29935684248814,3.08315210788516,9.91845591051738));
#158699=CARTESIAN_POINT('Ctrl Pts',(6.2210902739352,3.23817518699505,9.92630564627888));
#158700=CARTESIAN_POINT('Ctrl Pts',(6.13718012638381,3.39008062718567,9.93415538204038));
#158701=CARTESIAN_POINT('Ctrl Pts',(6.05327630085696,3.54197462239677,9.94200452638089));
#158702=CARTESIAN_POINT('Ctrl Pts',(5.96372993185385,3.69075111486342,9.9498536707214));
#158703=CARTESIAN_POINT('Ctrl Pts',(5.8688218592914,3.83595575396842,9.95770281506191));
#158704=CARTESIAN_POINT('Ctrl Pts',(5.77388295702589,3.98120756098849,9.96555450909901));
#158705=CARTESIAN_POINT('Ctrl Pts',(5.67357908796459,4.12288488234006,9.97340620313612));
#158706=CARTESIAN_POINT('Ctrl Pts',(5.56823396672836,4.26056299733645,9.98125789717322));
#158707=CARTESIAN_POINT('Ctrl Pts',(5.5400850383453,4.29735152017898,9.98335592288663));
#158708=CARTESIAN_POINT('Ctrl Pts',(5.51157639205649,4.33385468224104,9.98545394860006));
#158709=CARTESIAN_POINT('Ctrl Pts',(5.4827146855865,4.37006478658545,9.98755197431347));
#158710=CARTESIAN_POINT('Ctrl Pts',(5.34989049828849,4.53670696647608,9.99720727867339));
#158711=CARTESIAN_POINT('Ctrl Pts',(5.20965370605441,4.6970549548862,10.0068625830333));
#158712=CARTESIAN_POINT('Ctrl Pts',(5.0625854570575,4.85055203585014,10.0165178873932));
#158713=CARTESIAN_POINT('Ctrl Pts',(4.91470247755025,5.0048994618475,10.026226680328));
#158714=CARTESIAN_POINT('Ctrl Pts',(4.7599122137965,5.15231986845307,10.0359354732628));
#158715=CARTESIAN_POINT('Ctrl Pts',(4.59883503057595,5.2922908956375,10.0456442661976));
#158716=CARTESIAN_POINT('Ctrl Pts',(4.43698273027387,5.43293547528864,10.0553997786683));
#158717=CARTESIAN_POINT('Ctrl Pts',(4.26878290693983,5.56605879866049,10.065155291139));
#158718=CARTESIAN_POINT('Ctrl Pts',(4.0948937185639,5.69117492229557,10.0749108036097));
#158719=CARTESIAN_POINT('Ctrl Pts',(3.92083235313834,5.81641493014236,10.0846759755387));
#158720=CARTESIAN_POINT('Ctrl Pts',(3.74107039234043,5.93363186640219,10.0944411474676));
#158721=CARTESIAN_POINT('Ctrl Pts',(3.55629603071652,6.04238240302697,10.1042063193966));
#158722=CARTESIAN_POINT('Ctrl Pts',(3.37177360474307,6.15098466076206,10.1139581767351));
#158723=CARTESIAN_POINT('Ctrl Pts',(3.18225246996649,6.25114357144574,10.1237100340737));
#158724=CARTESIAN_POINT('Ctrl Pts',(2.98844542841549,6.34246170535405,10.1334618914122));
#158725=CARTESIAN_POINT('Ctrl Pts',(2.90393152212869,6.38228302531048,10.1377144074748));
#158726=CARTESIAN_POINT('Ctrl Pts',(2.81860296076509,6.42042375869067,10.1419669235373));
#158727=CARTESIAN_POINT('Ctrl Pts',(2.7325204682249,6.45685360320582,10.1462194395999));
#158728=CARTESIAN_POINT('Ctrl Pts',(2.56990977430587,6.52566994577636,10.1542524851987));
#158729=CARTESIAN_POINT('Ctrl Pts',(2.40452796168643,6.58841133439484,10.1622855307975));
#158730=CARTESIAN_POINT('Ctrl Pts',(2.23687673117688,6.64484830918054,10.1703185763963));
#158731=CARTESIAN_POINT('Ctrl Pts',(2.0693332733334,6.70124900410584,10.1783464580441));
#158732=CARTESIAN_POINT('Ctrl Pts',(1.89952364747798,6.75135323577297,10.1863743396919));
#158733=CARTESIAN_POINT('Ctrl Pts',(1.72796962997545,6.79497958204309,10.1944022213397));
#158734=CARTESIAN_POINT('Ctrl Pts',(1.55649307080299,6.83858623058781,10.2024264783198));
#158735=CARTESIAN_POINT('Ctrl Pts',(1.38327404273015,6.87572072725005,10.2104507353));
#158736=CARTESIAN_POINT('Ctrl Pts',(1.20884953836834,6.90625146921879,10.2184749922801));
#158737=CARTESIAN_POINT('Ctrl Pts',(1.03444612370561,6.93677851970986,10.2264982790458));
#158738=CARTESIAN_POINT('Ctrl Pts',(0.858837882611601,6.96070333514612,
10.2345215658114));
#158739=CARTESIAN_POINT('Ctrl Pts',(0.682572236592608,6.9779453784286,10.2425448525771));
#158740=CARTESIAN_POINT('Ctrl Pts',(0.506321033970898,6.99518600887944,
10.2505674819061));
#158741=CARTESIAN_POINT('Ctrl Pts',(0.329412899019472,7.00574492623494,
10.258590111235));
#158742=CARTESIAN_POINT('Ctrl Pts',(0.152400312836698,7.00959347659672,
10.2666127405639));
#158743=CARTESIAN_POINT('Ctrl Pts',(-0.0246788174764194,7.01344347373945,
10.2746383858303));
#158744=CARTESIAN_POINT('Ctrl Pts',(-0.201862110666864,7.01057805956247,
10.2826640310967));
#158745=CARTESIAN_POINT('Ctrl Pts',(-0.378596758129559,7.00102071538385,
10.2906896763631));
#158746=CARTESIAN_POINT('Ctrl Pts',(-0.482810275951469,6.99538512286033,
10.2954220858709));
#158747=CARTESIAN_POINT('Ctrl Pts',(-0.586867832603589,6.98742373395397,
10.3001544953786));
#158748=CARTESIAN_POINT('Ctrl Pts',(-0.690656921212897,6.97714981777522,
10.3048869048864));
#158749=CARTESIAN_POINT('Ctrl Pts',(-0.882120447473759,6.95819714898846,
10.313616953721));
#158750=CARTESIAN_POINT('Ctrl Pts',(-1.07276576003735,6.93136281656233,
10.3223470025557));
#158751=CARTESIAN_POINT('Ctrl Pts',(-1.26195338715803,6.89674562465083,
10.3310770513904));
#158752=CARTESIAN_POINT('Ctrl Pts',(-1.45119571811682,6.86211842313516,
10.3398096245295));
#158753=CARTESIAN_POINT('Ctrl Pts',(-1.63897925284441,6.81970391947392,
10.3485421976687));
#158754=CARTESIAN_POINT('Ctrl Pts',(-1.82467467174844,6.76965205197281,
10.3572747708079));
#158755=CARTESIAN_POINT('Ctrl Pts',(-2.01300819050361,6.71888911779606,
10.3661314040883));
#158756=CARTESIAN_POINT('Ctrl Pts',(-2.19919353136163,6.66027023944923,
10.3749880373687));
#158757=CARTESIAN_POINT('Ctrl Pts',(-2.3825896053187,6.59400434752111,10.3838446706491));
#158758=CARTESIAN_POINT('Ctrl Pts',(-2.56353185180905,6.52862508889005,
10.3925828027558));
#158759=CARTESIAN_POINT('Ctrl Pts',(-2.74175875492087,6.45580229510021,
10.4013209348626));
#158760=CARTESIAN_POINT('Ctrl Pts',(-2.91667336898161,6.37578567873588,
10.4100590669694));
#158761=CARTESIAN_POINT('Ctrl Pts',(-3.09514610967642,6.29414135816064,
10.4189749508366));
#158762=CARTESIAN_POINT('Ctrl Pts',(-3.27017008925038,6.20500752522851,
10.4278908347038));
#158763=CARTESIAN_POINT('Ctrl Pts',(-3.4411352453449,6.10869992598631,10.4368067185711));
#158764=CARTESIAN_POINT('Ctrl Pts',(-3.61210040143944,6.0123923267441,10.4457226024383));
#158765=CARTESIAN_POINT('Ctrl Pts',(-3.77900647355707,5.90891111491626,
10.4546384863055));
#158766=CARTESIAN_POINT('Ctrl Pts',(-3.94127167045108,5.79862088622802,
10.4635543701728));
#158767=CARTESIAN_POINT('Ctrl Pts',(-4.10034831522184,5.69049788840374,
10.472295054669));
#158768=CARTESIAN_POINT('Ctrl Pts',(-4.25498167604603,5.5758195038425,10.4810357391652));
#158769=CARTESIAN_POINT('Ctrl Pts',(-4.40465029916485,5.45496858877914,
10.4897764236614));
#158770=CARTESIAN_POINT('Ctrl Pts',(-4.55429199441221,5.33413941680285,
10.4985155355633));
#158771=CARTESIAN_POINT('Ctrl Pts',(-4.69897052287586,5.20714010410245,
10.5072546474651));
#158772=CARTESIAN_POINT('Ctrl Pts',(-4.8381969723823,5.07439421201495,10.515993759367));
#158773=CARTESIAN_POINT('Ctrl Pts',(-4.979227300924,4.93992840584069,10.5248460990414));
#158774=CARTESIAN_POINT('Ctrl Pts',(-5.11466306480168,4.79956625222048,
10.5336984387157));
#158775=CARTESIAN_POINT('Ctrl Pts',(-5.2440331497828,4.65378801477668,10.54255077839));
#158776=CARTESIAN_POINT('Ctrl Pts',(-5.37168303780633,4.50994814879311,
10.5512854110398));
#158777=CARTESIAN_POINT('Ctrl Pts',(-5.49342737628396,4.3608355561093,10.5600200436895));
#158778=CARTESIAN_POINT('Ctrl Pts',(-5.60885214401144,4.20694713410072,
10.5687546763393));
#158779=CARTESIAN_POINT('Ctrl Pts',(-5.72661009045162,4.04994803491747,
10.5776658695259));
#158780=CARTESIAN_POINT('Ctrl Pts',(-5.83779006784455,3.88797819357438,
10.5865770627126));
#158781=CARTESIAN_POINT('Ctrl Pts',(-5.94199644076384,3.72159977166404,
10.5954882558992));
#158782=CARTESIAN_POINT('Ctrl Pts',(-6.04620281368313,3.55522134975372,
10.6043994490859));
#158783=CARTESIAN_POINT('Ctrl Pts',(-6.14343540980711,3.38443459702493,
10.6133106422725));
#158784=CARTESIAN_POINT('Ctrl Pts',(-6.23334574516419,3.20983292146858,
10.6222218354592));
#158785=CARTESIAN_POINT('Ctrl Pts',(-6.31432145775723,3.05258186638172,
10.6302475003116));
#158786=CARTESIAN_POINT('Ctrl Pts',(-6.389394618327,2.89216390866958,10.638273165164));
#158787=CARTESIAN_POINT('Ctrl Pts',(-6.45831249077014,2.72907059895166,
10.6462988300164));
#158788=CARTESIAN_POINT('Ctrl Pts',(-6.527208490371,2.56602905104989,10.6543219477196));
#158789=CARTESIAN_POINT('Ctrl Pts',(-6.58995294864002,2.40031417886261,
10.6623450654229));
#158790=CARTESIAN_POINT('Ctrl Pts',(-6.64634038845737,2.23243947359392,
10.6703681831261));
#158791=CARTESIAN_POINT('Ctrl Pts',(-6.70272071732504,2.06458593879488,
10.678390289044));
#158792=CARTESIAN_POINT('Ctrl Pts',(-6.75274550846172,1.89457346103339,
10.6864123949619));
#158793=CARTESIAN_POINT('Ctrl Pts',(-6.79625849657452,1.7229326772218,10.6944345008797));
#158794=CARTESIAN_POINT('Ctrl Pts',(-6.83978765426074,1.55122811111492,
10.7024595878393));
#158795=CARTESIAN_POINT('Ctrl Pts',(-6.87680008183852,1.37789438511657,
10.7104846747988));
#158796=CARTESIAN_POINT('Ctrl Pts',(-6.90719008977021,1.20347481331362,
10.7185097617583));
#158797=CARTESIAN_POINT('Ctrl Pts',(-6.93758608286187,1.0290208904489,10.7265364292186));
#158798=CARTESIAN_POINT('Ctrl Pts',(-6.96135700378002,0.853481058385692,
10.7345630966788));
#158799=CARTESIAN_POINT('Ctrl Pts',(-6.97844883767682,0.677405626214464,
10.7425897641391));
#158800=CARTESIAN_POINT('Ctrl Pts',(-6.99555439283766,0.501188841306668,
10.7506228753797));
#158801=CARTESIAN_POINT('Ctrl Pts',(-7.0059701256658,0.324435963199458,
10.7586559866203));
#158802=CARTESIAN_POINT('Ctrl Pts',(-7.00969409651,0.147699816698825,10.7666890978609));
#158803=CARTESIAN_POINT('Ctrl Pts',(-7.011888395412,0.0435604588911374,
10.7714224988225));
#158804=CARTESIAN_POINT('Ctrl Pts',(-7.01176030669969,-0.0605730947154226,
10.7761558997841));
#158805=CARTESIAN_POINT('Ctrl Pts',(-7.00931788707195,-0.16458833638283,
10.7808893007457));
#158806=CARTESIAN_POINT('Ctrl Pts',(-7.00428642662564,-0.378862971387192,
10.7906402540398));
#158807=CARTESIAN_POINT('Ctrl Pts',(-6.98942851048065,-0.592761598645687,
10.8003912073339));
#158808=CARTESIAN_POINT('Ctrl Pts',(-6.96482894103385,-0.80547152937722,
10.810142160628));
#158809=CARTESIAN_POINT('Ctrl Pts',(-6.94019393129247,-1.01848790866763,
10.8199071619996));
#158810=CARTESIAN_POINT('Ctrl Pts',(-6.90578919919927,-1.23031212746868,
10.8296721633712));
#158811=CARTESIAN_POINT('Ctrl Pts',(-6.86175136652627,-1.44013705822569,
10.8394371647427));
#158812=CARTESIAN_POINT('Ctrl Pts',(-6.81778693579589,-1.6496122542979,
10.8491858898803));
#158813=CARTESIAN_POINT('Ctrl Pts',(-6.76422150246063,-1.85709478533727,
10.8589346150178));
#158814=CARTESIAN_POINT('Ctrl Pts',(-6.7012419681505,-2.06179112588993,
10.8686833401554));
#158815=CARTESIAN_POINT('Ctrl Pts',(-6.63843528824183,-2.26592565435847,
10.8784053088225));
#158816=CARTESIAN_POINT('Ctrl Pts',(-6.56626610055865,-2.46728922018291,
10.8881272774896));
#158817=CARTESIAN_POINT('Ctrl Pts',(-6.48497048630068,-2.66510494245707,
10.8978492461567));
#158818=CARTESIAN_POINT('Ctrl Pts',(-6.404212783889,-2.8616117697636,10.9075068870964));
#158819=CARTESIAN_POINT('Ctrl Pts',(-6.3144490211031,-3.05461749449963,
10.9171645280361));
#158820=CARTESIAN_POINT('Ctrl Pts',(-6.2159608466107,-3.24337128862897,
10.9268221689757));
#158821=CARTESIAN_POINT('Ctrl Pts',(-6.17267190317865,-3.32633507954867,
10.9310670346612));
#158822=CARTESIAN_POINT('Ctrl Pts',(-6.12769814221123,-3.40847758269322,
10.9353119003466));
#158823=CARTESIAN_POINT('Ctrl Pts',(-6.08106659565566,-3.48973575241749,
10.9395567660321));
#158824=CARTESIAN_POINT('Ctrl Pts',(-5.99481091721748,-3.64004126608645,
10.947408613046));
#158825=CARTESIAN_POINT('Ctrl Pts',(-5.90291526748711,-3.78725741194914,
10.9552604600599));
#158826=CARTESIAN_POINT('Ctrl Pts',(-5.80564328722662,-3.93092006837845,
10.9631123070738));
#158827=CARTESIAN_POINT('Ctrl Pts',(-5.70839889251332,-4.07454198323987,
10.9709619273674));
#158828=CARTESIAN_POINT('Ctrl Pts',(-5.60578141378705,-4.21461209767843,
10.978811547661));
#158829=CARTESIAN_POINT('Ctrl Pts',(-5.49809867869906,-4.35069390807808,
10.9866611679546));
#158830=CARTESIAN_POINT('Ctrl Pts',(-5.39042454070015,-4.48676485408572,
10.9945101615564));
#158831=CARTESIAN_POINT('Ctrl Pts',(-5.27768618867854,-4.61884783125907,
11.0023591551582));
#158832=CARTESIAN_POINT('Ctrl Pts',(-5.16023255287026,-4.74653837683823,
11.01020814876));
#158833=CARTESIAN_POINT('Ctrl Pts',(-5.0427194537255,-4.87429356840152,
11.0180611160774));
#158834=CARTESIAN_POINT('Ctrl Pts',(-4.92048655961227,-4.99765160406667,
11.0259140833949));
#158835=CARTESIAN_POINT('Ctrl Pts',(-4.79392081656102,-5.11624371654077,
11.0337670507123));
#158836=CARTESIAN_POINT('Ctrl Pts',(-4.66732293006375,-5.23486594742664,
11.0416220124196));
#158837=CARTESIAN_POINT('Ctrl Pts',(-4.5363902902682,-5.34871959341548,
11.0494769741268));
#158838=CARTESIAN_POINT('Ctrl Pts',(-4.40154341618671,-5.45747580094712,
11.0573319358341));
#158839=CARTESIAN_POINT('Ctrl Pts',(-4.2665626953109,-5.56633995810563,
11.0651946942474));
#158840=CARTESIAN_POINT('Ctrl Pts',(-4.12766028588765,-5.67009634324284,
11.0730574526608));
#158841=CARTESIAN_POINT('Ctrl Pts',(-3.98528667243108,-5.76845878038868,
11.0809202110741));
#158842=CARTESIAN_POINT('Ctrl Pts',(-3.88084343254005,-5.84061605286124,
11.0866882178222));
#158843=CARTESIAN_POINT('Ctrl Pts',(-3.77453279139432,-5.90987148297041,
11.0924562245704));
#158844=CARTESIAN_POINT('Ctrl Pts',(-3.66654084010936,-5.97612791281363,
11.0982242313185));
#158845=CARTESIAN_POINT('Ctrl Pts',(-3.50968184488422,-6.07236579803331,
11.1066022977595));
#158846=CARTESIAN_POINT('Ctrl Pts',(-3.34892741293879,-6.16248813004605,
11.1149803642005));
#158847=CARTESIAN_POINT('Ctrl Pts',(-3.18478243728188,-6.24618182489759,
11.1233584306416));
#158848=CARTESIAN_POINT('Ctrl Pts',(-3.02074970200894,-6.32981829099504,
11.1317307682603));
#158849=CARTESIAN_POINT('Ctrl Pts',(-2.85333133717546,-6.40703473506373,
11.140103105879));
#158850=CARTESIAN_POINT('Ctrl Pts',(-2.68305808668067,-6.47756326607448,
11.1484754434978));
#158851=CARTESIAN_POINT('Ctrl Pts',(-2.51287629632694,-6.54805391356932,
11.1568432840204));
#158852=CARTESIAN_POINT('Ctrl Pts',(-2.33984298092115,-6.61186368525468,
11.1652111245429));
#158853=CARTESIAN_POINT('Ctrl Pts',(-2.16451059628573,-6.66877203397048,
11.1735789650655));
#158854=CARTESIAN_POINT('Ctrl Pts',(-1.98924670431963,-6.72565815174066,
11.1819435367354));
#158855=CARTESIAN_POINT('Ctrl Pts',(-1.811685846297,-6.77564812142816,11.1903081084054));
#158856=CARTESIAN_POINT('Ctrl Pts',(-1.63239787270859,-6.81857050617477,
11.1986726800753));
#158857=CARTESIAN_POINT('Ctrl Pts',(-1.45315369358812,-6.86148240631963,
11.2070352085409));
#158858=CARTESIAN_POINT('Ctrl Pts',(-1.27218355970473,-6.8973300883243,
11.2153977370064));
#158859=CARTESIAN_POINT('Ctrl Pts',(-1.09007025647918,-6.92599259301072,
11.223760265472));
#158860=CARTESIAN_POINT('Ctrl Pts',(-0.907942420042187,-6.95465738505472,
11.2321234612935));
#158861=CARTESIAN_POINT('Ctrl Pts',(-0.724671555735195,-6.97613579714141,
11.240486657115));
#158862=CARTESIAN_POINT('Ctrl Pts',(-0.540849134503035,-6.99035827237827,
11.2488498529365));
#158863=CARTESIAN_POINT('Ctrl Pts',(-0.357014176950271,-7.00458171755943,
11.2572136191112));
#158864=CARTESIAN_POINT('Ctrl Pts',(-0.17262791529241,-7.01154821358821,
11.2655773852859));
#158865=CARTESIAN_POINT('Ctrl Pts',(0.0117144055303785,-7.01124021377125,
11.2739411514606));
#158866=CARTESIAN_POINT('Ctrl Pts',(0.196093875297651,-7.01093215188569,
11.2823066031142));
#158867=CARTESIAN_POINT('Ctrl Pts',(0.380429057787402,-7.003346671542,11.2906720547678));
#158868=CARTESIAN_POINT('Ctrl Pts',(0.564125623979578,-6.98851835819794,
11.2990375064214));
#158869=CARTESIAN_POINT('Ctrl Pts',(0.747883709790392,-6.97368507888092,
11.3074057596482));
#158870=CARTESIAN_POINT('Ctrl Pts',(0.931002425250959,-6.95160415627133,
11.3157740128751));
#158871=CARTESIAN_POINT('Ctrl Pts',(1.11289303815448,-6.92236199921149,
11.324142266102));
#158872=CARTESIAN_POINT('Ctrl Pts',(1.29495228960569,-6.89309273050021,
11.3325182778934));
#158873=CARTESIAN_POINT('Ctrl Pts',(1.47578083823409,-6.85664901190681,
11.3408942896849));
#158874=CARTESIAN_POINT('Ctrl Pts',(1.65479938758511,-6.81316853962589,
11.3492703014764));
#158875=CARTESIAN_POINT('Ctrl Pts',(1.83390572984466,-6.76966674398412,
11.3576504209675));
#158876=CARTESIAN_POINT('Ctrl Pts',(2.01119998494268,-6.71912139677779,
11.3660305404587));
#158877=CARTESIAN_POINT('Ctrl Pts',(2.18611784614132,-6.66172014762572,
11.3744106599498));
#158878=CARTESIAN_POINT('Ctrl Pts',(2.36123557315379,-6.6042533102753,11.382800354789));
#158879=CARTESIAN_POINT('Ctrl Pts',(2.53397117006586,-6.53991502628123,
11.3911900496282));
#158880=CARTESIAN_POINT('Ctrl Pts',(2.70377888891536,-6.46894166632809,
11.3995797444674));
#158881=CARTESIAN_POINT('Ctrl Pts',(2.81158687928558,-6.42388190486252,
11.4049062169421));
#158882=CARTESIAN_POINT('Ctrl Pts',(2.91821513877765,-6.37614866300158,
11.4102326894167));
#158883=CARTESIAN_POINT('Ctrl Pts',(3.02352911297256,-6.32581206372015,
11.4155591618913));
#158884=CARTESIAN_POINT('Ctrl Pts',(3.18924254879002,-6.24660651784591,
11.4239404622962));
#158885=CARTESIAN_POINT('Ctrl Pts',(3.35203493321813,-6.16079312393665,
11.4323217627011));
#158886=CARTESIAN_POINT('Ctrl Pts',(3.51136137524599,-6.06860509960325,
11.440703063106));
#158887=CARTESIAN_POINT('Ctrl Pts',(3.67048589433233,-5.97653391009532,
11.4490737414396));
#158888=CARTESIAN_POINT('Ctrl Pts',(3.826152943663,-5.87810435335717,11.4574444197731));
#158889=CARTESIAN_POINT('Ctrl Pts',(3.9778393323686,-5.77359686922817,11.4658150981067));
#158890=CARTESIAN_POINT('Ctrl Pts',(4.12935358306614,-5.66920798315071,
11.4741762771575));
#158891=CARTESIAN_POINT('Ctrl Pts',(4.27689590857438,-5.55875510173029,
11.4825374562083));
#158892=CARTESIAN_POINT('Ctrl Pts',(4.41996900155504,-5.44256378812344,
11.4908986352591));
#158893=CARTESIAN_POINT('Ctrl Pts',(4.56285644032072,-5.32652324645188,
11.4992489646939));
#158894=CARTESIAN_POINT('Ctrl Pts',(4.70128596084793,-5.2047593305936,11.5075992941286));
#158895=CARTESIAN_POINT('Ctrl Pts',(4.83479052300556,-5.07763992039172,
11.5159496235633));
#158896=CARTESIAN_POINT('Ctrl Pts',(4.96819236138863,-4.95061832097192,
11.524293527919));
#158897=CARTESIAN_POINT('Ctrl Pts',(5.09667655682613,-4.81824966405888,
11.5326374322748));
#158898=CARTESIAN_POINT('Ctrl Pts',(5.21980948776443,-4.68094172938998,
11.5409813366305));
#158899=CARTESIAN_POINT('Ctrl Pts',(5.34284351756477,-4.54374408131044,
11.5493185391102));
#158900=CARTESIAN_POINT('Ctrl Pts',(5.46053463683438,-4.40161531083358,
11.5576557415899));
#158901=CARTESIAN_POINT('Ctrl Pts',(5.57248631467415,-4.25499974562506,
11.5659929440696));
#158902=CARTESIAN_POINT('Ctrl Pts',(5.60934018906037,-4.20673471085718,
11.5687375051057));
#158903=CARTESIAN_POINT('Ctrl Pts',(5.64557239156457,-4.15798373428186,
11.5714820661417));
#158904=CARTESIAN_POINT('Ctrl Pts',(5.68116969739712,-4.10876349183994,
11.5742266271778));
#158905=CARTESIAN_POINT('Ctrl Pts',(5.7893186429094,-3.95922640768553,11.5825649374797));
#158906=CARTESIAN_POINT('Ctrl Pts',(5.89151555911645,-3.80547827912205,
11.5909032477815));
#158907=CARTESIAN_POINT('Ctrl Pts',(5.98744753524082,-3.64802666865782,
11.5992415580834));
#158908=CARTESIAN_POINT('Ctrl Pts',(6.08343986850949,-3.49047599498278,
11.6075851145673));
#158909=CARTESIAN_POINT('Ctrl Pts',(6.17315922902922,-3.32921747152846,
11.6159286710511));
#158910=CARTESIAN_POINT('Ctrl Pts',(6.25633847895222,-3.16478362598168,
11.6242722275349));
#158911=CARTESIAN_POINT('Ctrl Pts',(6.33958101128566,-3.00022467988263,
11.63262213176));
#158912=CARTESIAN_POINT('Ctrl Pts',(6.41627336041963,-2.83248588505753,
11.6409720359852));
#158913=CARTESIAN_POINT('Ctrl Pts',(6.48619618491797,-2.66212051065604,
11.6493219402104));
#158914=CARTESIAN_POINT('Ctrl Pts',(6.55622388847894,-2.49149960079956,
11.6576843686741));
#158915=CARTESIAN_POINT('Ctrl Pts',(6.61946165243177,-2.31824454203393,
11.6660467971377));
#158916=CARTESIAN_POINT('Ctrl Pts',(6.67573926520284,-2.14292599627917,
11.6744092256013));
#158917=CARTESIAN_POINT('Ctrl Pts',(6.7320650030048,-1.96745752926772,11.6827788050813));
#158918=CARTESIAN_POINT('Ctrl Pts',(6.78141862654025,-1.78992236943731,
11.6911483845613));
#158919=CARTESIAN_POINT('Ctrl Pts',(6.82368074612044,-1.61090273993349,
11.6995179640413));
#158920=CARTESIAN_POINT('Ctrl Pts',(6.86600804987073,-1.43160699446347,
11.7079004525778));
#158921=CARTESIAN_POINT('Ctrl Pts',(6.90122193019567,-1.25082252497166,
11.7162829411144));
#158922=CARTESIAN_POINT('Ctrl Pts',(6.92925445938158,-1.06913946688002,
11.7246654296509));
#158923=CARTESIAN_POINT('Ctrl Pts',(6.93842716227157,-1.00968979321814,
11.7274083172554));
#158924=CARTESIAN_POINT('Ctrl Pts',(6.94683136914179,-0.950143927580071,
11.7301512048598));
#158925=CARTESIAN_POINT('Ctrl Pts',(6.95446591090137,-0.890522575014692,
11.7328940924642));
#158926=CARTESIAN_POINT('Ctrl Pts',(6.99217189097099,-0.596060693431332,
11.7464408472796));
#158927=CARTESIAN_POINT('Ctrl Pts',(7.01115634495759,-0.299346418725676,
11.7599876020951));
#158928=CARTESIAN_POINT('Ctrl Pts',(7.01124965431565,-0.00220167178196738,
11.7735343569105));
#158929=CARTESIAN_POINT('Ctrl Pts',(7.01124965431583,-0.00220167122712958,
11.7735343569358));
#158930=CARTESIAN_POINT('Ctrl Pts',(7.01130668446778,0.179411563396666,
11.781814058953));
#158931=CARTESIAN_POINT('Ctrl Pts',(7.00430291895196,0.361201757753028,
11.7900937609703));
#158932=CARTESIAN_POINT('Ctrl Pts',(6.99022344746899,0.542588902351294,
11.7983734629875));
#158933=CARTESIAN_POINT('Ctrl Pts',(6.97615945174002,0.723776671367002,
11.8066440641922));
#158934=CARTESIAN_POINT('Ctrl Pts',(6.95503528430813,0.904561935256292,
11.8149146653968));
#158935=CARTESIAN_POINT('Ctrl Pts',(6.92688806918397,1.08436536254937,11.8231852666014));
#158936=CARTESIAN_POINT('Ctrl Pts',(6.89875892534549,1.26405335110059,11.8314505578528));
#158937=CARTESIAN_POINT('Ctrl Pts',(6.86361576914439,1.44276042284829,11.8397158491041));
#158938=CARTESIAN_POINT('Ctrl Pts',(6.82154754427712,1.61991223949535,11.8479811403555));
#158939=CARTESIAN_POINT('Ctrl Pts',(6.77950291415879,1.79696469724027,11.856241795864));
#158940=CARTESIAN_POINT('Ctrl Pts',(6.73054103683612,1.97246330740118,11.8645024513725));
#158941=CARTESIAN_POINT('Ctrl Pts',(6.67480198863536,2.14584365111008,11.8727631068811));
#158942=CARTESIAN_POINT('Ctrl Pts',(6.64250096825414,2.24631831288892,11.8775501926056));
#158943=CARTESIAN_POINT('Ctrl Pts',(6.60792495302767,2.34608180031525,11.8823372783302));
#158944=CARTESIAN_POINT('Ctrl Pts',(6.57110895151814,2.44502632087636,11.8871243640548));
#158945=CARTESIAN_POINT('',(7.0112498809707,-0.00129193205168586,11.2264656430533));
#158946=CARTESIAN_POINT('Ctrl Pts',(6.57110895151813,2.44502632087638,11.3397782664936));
#158947=CARTESIAN_POINT('Ctrl Pts',(6.63286227697798,2.27906171499445,11.3317554799954));
#158948=CARTESIAN_POINT('Ctrl Pts',(6.68833298419261,2.11073178541639,11.3237326934973));
#158949=CARTESIAN_POINT('Ctrl Pts',(6.7373471412283,1.94056179007081,11.3157099069992));
#158950=CARTESIAN_POINT('Ctrl Pts',(6.78858424553279,1.76267404644062,11.3073232617221));
#158951=CARTESIAN_POINT('Ctrl Pts',(6.83276533325641,1.58277584443963,11.298936616445));
#158952=CARTESIAN_POINT('Ctrl Pts',(6.8697504549464,1.40148323188821,11.2905499711678));
#158953=CARTESIAN_POINT('Ctrl Pts',(6.90673557663638,1.22019061933677,11.2821633258907));
#158954=CARTESIAN_POINT('Ctrl Pts',(6.93652466649385,1.03750404859929,11.2737766806136));
#158955=CARTESIAN_POINT('Ctrl Pts',(6.95903917973925,0.854049329578839,
11.2653900353364));
#158956=CARTESIAN_POINT('Ctrl Pts',(6.98457816243644,0.645950364981519,
11.2558767766536));
#158957=CARTESIAN_POINT('Ctrl Pts',(7.00076663815956,0.436802360120021,
11.2463635179709));
#158958=CARTESIAN_POINT('Ctrl Pts',(7.00756193005895,0.227381527148892,
11.2368502592881));
#158959=CARTESIAN_POINT('Ctrl Pts',(7.01003449670461,0.151180684833668,
11.2333887205553));
#158960=CARTESIAN_POINT('Ctrl Pts',(7.01126392857063,0.0749437292480127,
11.2299271818224));
#158961=CARTESIAN_POINT('Ctrl Pts',(7.01124988097084,-0.0012919312519414,
11.2264656430896));
#158962=CARTESIAN_POINT('Ctrl Pts',(7.0112498809707,-0.00129193205166578,
11.2264656430533));
#158963=CARTESIAN_POINT('Ctrl Pts',(7.01121483285703,-0.19149627172734,
11.2178292688864));
#158964=CARTESIAN_POINT('Ctrl Pts',(7.00343552236527,-0.381688380886737,
11.2091928947195));
#158965=CARTESIAN_POINT('Ctrl Pts',(6.98794071515853,-0.57123648686839,
11.2005565205526));
#158966=CARTESIAN_POINT('Ctrl Pts',(6.97244167909753,-0.760836324459489,
11.1919177893401));
#158967=CARTESIAN_POINT('Ctrl Pts',(6.94922296039208,-0.949791518269339,
11.1832790581275));
#158968=CARTESIAN_POINT('Ctrl Pts',(6.91836528355355,-1.13747455612029,
11.174640326915));
#158969=CARTESIAN_POINT('Ctrl Pts',(6.88750581762904,-1.32516847557757,
11.1660010948406));
#158970=CARTESIAN_POINT('Ctrl Pts',(6.84900656005112,-1.51158980612792,
11.1573618627662));
#158971=CARTESIAN_POINT('Ctrl Pts',(6.80299959257456,-1.69612001519068,
11.1487226306918));
#158972=CARTESIAN_POINT('Ctrl Pts',(6.75698038588684,-1.88069931473509,
11.1400811003267));
#158973=CARTESIAN_POINT('Ctrl Pts',(6.70344954877135,-2.06338620598536,
11.1314395699616));
#158974=CARTESIAN_POINT('Ctrl Pts',(6.64258968814643,-2.24357500374531,
11.1227980395966));
#158975=CARTESIAN_POINT('Ctrl Pts',(6.60485135574661,-2.35530750978073,
11.1174395497477));
#158976=CARTESIAN_POINT('Ctrl Pts',(6.56429595901887,-2.46607976288995,
11.1120810598989));
#158977=CARTESIAN_POINT('Ctrl Pts',(6.5209765531919,-2.57575063917715,11.10672257005));
#158978=CARTESIAN_POINT('Ctrl Pts',(6.45031461865842,-2.75464405039773,
11.0979818855538));
#158979=CARTESIAN_POINT('Ctrl Pts',(6.37228337420837,-2.9306376100954,11.0892412010576));
#158980=CARTESIAN_POINT('Ctrl Pts',(6.28714218852822,-3.1031386794226,11.0805005165614));
#158981=CARTESIAN_POINT('Ctrl Pts',(6.2020163211615,-3.27560871294231,11.0717614046595));
#158982=CARTESIAN_POINT('Ctrl Pts',(6.10978318835428,-3.44458726553878,
11.0630222927576));
#158983=CARTESIAN_POINT('Ctrl Pts',(6.01074900219863,-3.60950453595341,
11.0542831808556));
#158984=CARTESIAN_POINT('Ctrl Pts',(5.91043168562665,-3.77655854696298,
11.0454308411813));
#158985=CARTESIAN_POINT('Ctrl Pts',(5.8031359797634,-3.93944504673891,11.036578501507));
#158986=CARTESIAN_POINT('Ctrl Pts',(5.68922732024001,-4.09759918258664,
11.0277261618326));
#158987=CARTESIAN_POINT('Ctrl Pts',(5.57683327152893,-4.25365038819914,
11.0189915291829));
#158988=CARTESIAN_POINT('Ctrl Pts',(5.45800121360134,-4.40509407825301,
11.0102568965331));
#158989=CARTESIAN_POINT('Ctrl Pts',(5.33312531501383,-4.55141746457724,
11.0015222638833));
#158990=CARTESIAN_POINT('Ctrl Pts',(5.20572519399149,-4.70069860959371,
10.9926110706967));
#158991=CARTESIAN_POINT('Ctrl Pts',(5.0720344634497,-4.8446500091867,10.9836998775101));
#158992=CARTESIAN_POINT('Ctrl Pts',(4.93251499832045,-4.98276252232071,
10.9747886843235));
#158993=CARTESIAN_POINT('Ctrl Pts',(4.79299553319121,-5.12087503545471,
10.9658774911369));
#158994=CARTESIAN_POINT('Ctrl Pts',(4.64764753942393,-5.25314843929787,
10.9569662979502));
#158995=CARTESIAN_POINT('Ctrl Pts',(4.49697370569523,-5.37911275702469,
10.9480551047636));
#158996=CARTESIAN_POINT('Ctrl Pts',(4.36127272085424,-5.49255967443127,
10.9400294399112));
#158997=CARTESIAN_POINT('Ctrl Pts',(4.22118909179728,-5.60094084191295,
10.9320037750588));
#158998=CARTESIAN_POINT('Ctrl Pts',(4.07714709029428,-5.70390201236004,
10.9239781102064));
#158999=CARTESIAN_POINT('Ctrl Pts',(3.93315080418942,-5.80683050545712,
10.9159549925032));
#159000=CARTESIAN_POINT('Ctrl Pts',(3.78519894465811,-5.90434221331194,
10.9079318747999));
#159001=CARTESIAN_POINT('Ctrl Pts',(3.63374754083289,-5.99612419584442,
10.8999087570967));
#159002=CARTESIAN_POINT('Ctrl Pts',(3.48231523635535,-6.08789460386554,
10.8918866511788));
#159003=CARTESIAN_POINT('Ctrl Pts',(3.327384580363,-6.17393653641374,10.883864545261));
#159004=CARTESIAN_POINT('Ctrl Pts',(3.16943910852018,-6.25398131592051,
10.8758424393431));
#159005=CARTESIAN_POINT('Ctrl Pts',(3.0114349436063,-6.33405584033783,10.8678173523836));
#159006=CARTESIAN_POINT('Ctrl Pts',(2.85041405073292,-6.40812859121088,
10.859792265424));
#159007=CARTESIAN_POINT('Ctrl Pts',(2.68688341071867,-6.47597746287808,
10.8517671784645));
#159008=CARTESIAN_POINT('Ctrl Pts',(2.5233205641631,-6.54383969704107,10.8437405110042));
#159009=CARTESIAN_POINT('Ctrl Pts',(2.35724732772862,-6.6054754777394,10.835713843544));
#159010=CARTESIAN_POINT('Ctrl Pts',(2.18918882380095,-6.66071158782941,
10.8276871760837));
#159011=CARTESIAN_POINT('Ctrl Pts',(2.02099540309858,-6.71599204127395,
10.8196540648431));
#159012=CARTESIAN_POINT('Ctrl Pts',(1.85081388283077,-6.7648624573645,10.8116209536025));
#159013=CARTESIAN_POINT('Ctrl Pts',(1.67918324409768,-6.8071998791898,10.8035878423619));
#159014=CARTESIAN_POINT('Ctrl Pts',(1.57805223693432,-6.83214662611971,
10.7988544414003));
#159015=CARTESIAN_POINT('Ctrl Pts',(1.4764183082212,-6.8548260866022,10.7941210404387));
#159016=CARTESIAN_POINT('Ctrl Pts',(1.37439299910562,-6.87522148345124,
10.7893876394771));
#159017=CARTESIAN_POINT('Ctrl Pts',(1.16421768708872,-6.91723663570723,
10.779636686183));
#159018=CARTESIAN_POINT('Ctrl Pts',(0.952257338297864,-6.94958151096932,
10.7698857328889));
#159019=CARTESIAN_POINT('Ctrl Pts',(0.739323485861614,-6.97216088065626,
10.7601347795948));
#159020=CARTESIAN_POINT('Ctrl Pts',(0.526082862265363,-6.99477278016103,
10.7503697782232));
#159021=CARTESIAN_POINT('Ctrl Pts',(0.31186596799987,-7.00759102779102,
10.7406047768516));
#159022=CARTESIAN_POINT('Ctrl Pts',(0.0974902579981229,-7.01057217437318,
10.73083977548));
#159023=CARTESIAN_POINT('Ctrl Pts',(-0.116528132112505,-7.01354835200166,
10.7210910503425));
#159024=CARTESIAN_POINT('Ctrl Pts',(-0.330704771000217,-7.00672019781832,
10.711342325205));
#159025=CARTESIAN_POINT('Ctrl Pts',(-0.544224464764906,-6.99009630079954,
10.7015936000674));
#159026=CARTESIAN_POINT('Ctrl Pts',(-0.757158129762107,-6.97351802993218,
10.6918716314003));
#159027=CARTESIAN_POINT('Ctrl Pts',(-0.969438409336941,-6.94719769186674,
10.6821496627332));
#159028=CARTESIAN_POINT('Ctrl Pts',(-1.1802555801732,-6.91119550642073,
10.6724276940662));
#159029=CARTESIAN_POINT('Ctrl Pts',(-1.3896778288526,-6.87543153803253,
10.6627700531265));
#159030=CARTESIAN_POINT('Ctrl Pts',(-1.59765621594698,-6.83011340267927,
10.6531124121868));
#159031=CARTESIAN_POINT('Ctrl Pts',(-1.80339645969658,-6.77535148694545,
10.6434547712472));
#159032=CARTESIAN_POINT('Ctrl Pts',(-1.89382638003329,-6.75128173964155,
10.6392099055617));
#159033=CARTESIAN_POINT('Ctrl Pts',(-1.98382391000512,-6.72538821540239,
10.6349650398762));
#159034=CARTESIAN_POINT('Ctrl Pts',(-2.07332161451241,-6.69768348351097,
10.6307201741907));
#159035=CARTESIAN_POINT('Ctrl Pts',(-2.23886802656795,-6.64643726455113,
10.6228683271768));
#159036=CARTESIAN_POINT('Ctrl Pts',(-2.40263517021604,-6.58901142800171,
10.6150164801629));
#159037=CARTESIAN_POINT('Ctrl Pts',(-2.5641124543584,-6.52556157613306,
10.607164633149));
#159038=CARTESIAN_POINT('Ctrl Pts',(-2.72554394484851,-6.46212971812941,
10.5993150128554));
#159039=CARTESIAN_POINT('Ctrl Pts',(-2.88468651288333,-6.39267738239986,
10.5914653925618));
#159040=CARTESIAN_POINT('Ctrl Pts',(-3.04104683840681,-6.31740933366803,
10.5836157722682));
#159041=CARTESIAN_POINT('Ctrl Pts',(-3.1973946805583,-6.24214729412714,
10.5757667786664));
#159042=CARTESIAN_POINT('Ctrl Pts',(-3.35096037900238,-6.16107063202908,
10.5679177850646));
#159043=CARTESIAN_POINT('Ctrl Pts',(-3.50127287565162,-6.07443123368157,
10.5600687914628));
#159044=CARTESIAN_POINT('Ctrl Pts',(-3.65166147111628,-5.98774797234377,
10.5522158241453));
#159045=CARTESIAN_POINT('Ctrl Pts',(-3.79879324307088,-5.89549653849056,
10.5443628568279));
#159046=CARTESIAN_POINT('Ctrl Pts',(-3.94222363728072,-5.7979737284818,
10.5365098895105));
#159047=CARTESIAN_POINT('Ctrl Pts',(-4.08569045799139,-5.70042615095609,
10.5286549278032));
#159048=CARTESIAN_POINT('Ctrl Pts',(-4.22545372090009,-5.5976047562469,
10.5207999660959));
#159049=CARTESIAN_POINT('Ctrl Pts',(-4.36110046444042,-5.48984783956327,
10.5129450043887));
#159050=CARTESIAN_POINT('Ctrl Pts',(-4.49688184871228,-5.38198396513256,
10.5050822459753));
#159051=CARTESIAN_POINT('Ctrl Pts',(-4.62853826330783,-5.26917503243585,
10.4972194875619));
#159052=CARTESIAN_POINT('Ctrl Pts',(-4.75569182610824,-5.15179792088037,
10.4893567291486));
#159053=CARTESIAN_POINT('Ctrl Pts',(-4.84896985523238,-5.06569175610569,
10.4835887224005));
#159054=CARTESIAN_POINT('Ctrl Pts',(-4.93982542595319,-4.97712803729662,
10.4778207156524));
#159055=CARTESIAN_POINT('Ctrl Pts',(-5.02812298621066,-4.88626706167807,
10.4720527089043));
#159056=CARTESIAN_POINT('Ctrl Pts',(-5.15637575336667,-4.75429091742679,
10.4636746424633));
#159057=CARTESIAN_POINT('Ctrl Pts',(-5.27951448298945,-4.61717463325744,
10.4552965760223));
#159058=CARTESIAN_POINT('Ctrl Pts',(-5.39712312308619,-4.4753422837531,
10.4469185095812));
#159059=CARTESIAN_POINT('Ctrl Pts',(-5.51465134379223,-4.33360691752412,
10.4385461719625));
#159060=CARTESIAN_POINT('Ctrl Pts',(-5.62665680482521,-4.1871621674751,
10.4301738343438));
#159061=CARTESIAN_POINT('Ctrl Pts',(-5.73276188898709,-4.03646722849042,
10.421801496725));
#159062=CARTESIAN_POINT('Ctrl Pts',(-5.83880998013379,-3.88585323340221,
10.4134336562024));
#159063=CARTESIAN_POINT('Ctrl Pts',(-5.93896382489256,-3.73099386951696,
10.4050658156798));
#159064=CARTESIAN_POINT('Ctrl Pts',(-6.03288724599517,-3.57237988455999,
10.3966979751572));
#159065=CARTESIAN_POINT('Ctrl Pts',(-6.12677397640972,-3.41382786131795,
10.3883334034873));
#159066=CARTESIAN_POINT('Ctrl Pts',(-6.21443496943698,-3.25152442428541,
10.3799688318174));
#159067=CARTESIAN_POINT('Ctrl Pts',(-6.29557815673927,-3.0859880484032,
10.3716042601475));
#159068=CARTESIAN_POINT('Ctrl Pts',(-6.37670152328819,-2.92049210790181,
10.3632417316819));
#159069=CARTESIAN_POINT('Ctrl Pts',(-6.4513101149823,-2.75176509848021,
10.3548792032163));
#159070=CARTESIAN_POINT('Ctrl Pts',(-6.5191582832499,-2.58034917025472,
10.3465166747507));
#159071=CARTESIAN_POINT('Ctrl Pts',(-6.58701186601356,-2.40891956250198,
10.3381534789292));
#159072=CARTESIAN_POINT('Ctrl Pts',(-6.6481038209225,-2.23480091061489,
10.3297902831077));
#159073=CARTESIAN_POINT('Ctrl Pts',(-6.70223675191998,-2.05855509610823,
10.3214270872862));
#159074=CARTESIAN_POINT('Ctrl Pts',(-6.75637337467483,-1.88229726199034,
10.3130633211115));
#159075=CARTESIAN_POINT('Ctrl Pts',(-6.80354993042206,-1.70391229024975,
10.3046995549368));
#159076=CARTESIAN_POINT('Ctrl Pts',(-6.84361894436408,-1.52397713461885,
10.2963357887621));
#159077=CARTESIAN_POINT('Ctrl Pts',(-6.88369603307462,-1.3440057181822,
10.2879703371085));
#159078=CARTESIAN_POINT('Ctrl Pts',(-6.91666265244109,-1.16248381585892,
10.279604885455));
#159079=CARTESIAN_POINT('Ctrl Pts',(-6.94242239497191,-0.979998904230274,
10.2712394338014));
#159080=CARTESIAN_POINT('Ctrl Pts',(-6.96819076438986,-0.79745287876346,
10.2628711805746));
#159081=CARTESIAN_POINT('Ctrl Pts',(-6.98674739831039,-0.613943526323872,
10.2545029273477));
#159082=CARTESIAN_POINT('Ctrl Pts',(-6.99804768035543,-0.430064211452212,
10.2461346741208));
#159083=CARTESIAN_POINT('Ctrl Pts',(-7.00935843937408,-0.246014414222441,
10.2377586623293));
#159084=CARTESIAN_POINT('Ctrl Pts',(-7.0133993824308,-0.0615942976320604,
10.2293826505379));
#159085=CARTESIAN_POINT('Ctrl Pts',(-7.01017800193792,0.122600748960567,
10.2210066387464));
#159086=CARTESIAN_POINT('Ctrl Pts',(-7.00695504164024,0.306886127079898,
10.2126265192552));
#159087=CARTESIAN_POINT('Ctrl Pts',(-6.99646266769307,0.490945886679691,
10.2042463997641));
#159088=CARTESIAN_POINT('Ctrl Pts',(-6.97876039602519,0.674188324854724,
10.195866280273));
#159089=CARTESIAN_POINT('Ctrl Pts',(-6.96103789726951,0.857640140727379,
10.1874765854337));
#159090=CARTESIAN_POINT('Ctrl Pts',(-6.93608907723435,1.04027244237954,
10.1790868905945));
#159091=CARTESIAN_POINT('Ctrl Pts',(-6.90402505451619,1.22150096566184,
10.1706971957553));
#159092=CARTESIAN_POINT('Ctrl Pts',(-6.88366815981293,1.33655982768021,
10.1653707232807));
#159093=CARTESIAN_POINT('Ctrl Pts',(-6.86044432726521,1.45105306635647,
10.1600442508061));
#159094=CARTESIAN_POINT('Ctrl Pts',(-6.83439251135145,1.5648340369775,10.1547177783314));
#159095=CARTESIAN_POINT('Ctrl Pts',(-6.79339950964048,1.74387044422,10.1463364779266));
#159096=CARTESIAN_POINT('Ctrl Pts',(-6.74531936724476,1.92150377135524,
10.1379551775217));
#159097=CARTESIAN_POINT('Ctrl Pts',(-6.69026031388856,2.09715128088266,
10.1295738771168));
#159098=CARTESIAN_POINT('Ctrl Pts',(-6.63527103982242,2.2725761829047,10.1212031987833));
#159099=CARTESIAN_POINT('Ctrl Pts',(-6.57332057867011,2.44601997279038,
10.1128325204497));
#159100=CARTESIAN_POINT('Ctrl Pts',(-6.50456798830298,2.61691074514286,
10.1044618421162));
#159101=CARTESIAN_POINT('Ctrl Pts',(-6.43589342032166,2.78760758580926,
10.0961006630653));
#159102=CARTESIAN_POINT('Ctrl Pts',(-6.36043222998785,2.95575688132914,
10.0877394840145));
#159103=CARTESIAN_POINT('Ctrl Pts',(-6.27839317148616,3.12080209989932,
10.0793783049637));
#159104=CARTESIAN_POINT('Ctrl Pts',(-6.19646056834021,3.28563315282965,
10.071027975529));
#159105=CARTESIAN_POINT('Ctrl Pts',(-6.10796726725877,3.44736787087806,
10.0626776460943));
#159106=CARTESIAN_POINT('Ctrl Pts',(-6.01316994022668,3.60546998773451,
10.0543273166596));
#159107=CARTESIAN_POINT('Ctrl Pts',(-5.91844555406709,3.7634504544695,10.0459834123038));
#159108=CARTESIAN_POINT('Ctrl Pts',(-5.81742697603724,3.91780361026158,
10.0376395079481));
#159109=CARTESIAN_POINT('Ctrl Pts',(-5.71041712791927,4.06801705842862,
10.0292956035924));
#159110=CARTESIAN_POINT('Ctrl Pts',(-5.60349323077875,4.21810985421718,
10.0209584011127));
#159111=CARTESIAN_POINT('Ctrl Pts',(-5.49058785040465,4.36406930760973,
10.012621198633));
#159112=CARTESIAN_POINT('Ctrl Pts',(-5.3720476919304,4.5054112085497,10.0042839961533));
#159113=CARTESIAN_POINT('Ctrl Pts',(-5.33302492608617,4.55194018215114,
10.0015394351172));
#159114=CARTESIAN_POINT('Ctrl Pts',(-5.29339187257674,4.59796899144473,
9.99879487408112));
#159115=CARTESIAN_POINT('Ctrl Pts',(-5.25316190643485,4.64348108074985,
9.99605031304502));
#159116=CARTESIAN_POINT('Ctrl Pts',(-5.1309383753438,4.78175234457802,9.98771200274311));
#159117=CARTESIAN_POINT('Ctrl Pts',(-5.00330256798266,4.91513824112804,
9.97937369244119));
#159118=CARTESIAN_POINT('Ctrl Pts',(-4.87068120156059,5.04322230278066,
9.97103538213927));
#159119=CARTESIAN_POINT('Ctrl Pts',(-4.73797639427498,5.17138695057864,
9.96269182565545));
#159120=CARTESIAN_POINT('Ctrl Pts',(-4.60028000698162,5.29424288232457,
9.95434826917163));
#159121=CARTESIAN_POINT('Ctrl Pts',(-4.45805313999478,5.41141282508391,
9.94600471268782));
#159122=CARTESIAN_POINT('Ctrl Pts',(-4.31571806742758,5.52867191022492,
9.9376548084626));
#159123=CARTESIAN_POINT('Ctrl Pts',(-4.16884589258824,5.6402361695705,9.9293049042374));
#159124=CARTESIAN_POINT('Ctrl Pts',(-4.01792842083125,5.74577042419696,
9.92095500001219));
#159125=CARTESIAN_POINT('Ctrl Pts',(-3.86678458403449,5.85146297239585,
9.91259257154852));
#159126=CARTESIAN_POINT('Ctrl Pts',(-3.71158359400024,5.95110725406904,
9.90423014308485));
#159127=CARTESIAN_POINT('Ctrl Pts',(-3.55284498573029,6.04441221872492,
9.89586771462119));
#159128=CARTESIAN_POINT('Ctrl Pts',(-3.39397063431105,6.1377969718449,9.88749813514123));
#159129=CARTESIAN_POINT('Ctrl Pts',(-3.23155291681996,6.22483143729944,
9.87912855566126));
#159130=CARTESIAN_POINT('Ctrl Pts',(-3.06613377845246,6.30527162104321,
9.87075897618129));
#159131=CARTESIAN_POINT('Ctrl Pts',(-2.90045950121834,6.38583587396974,
9.86237648764471));
#159132=CARTESIAN_POINT('Ctrl Pts',(-2.73177485183306,6.45978538944467,
9.85399399910813));
#159133=CARTESIAN_POINT('Ctrl Pts',(-2.56064076548373,6.52692465351355,
9.84561151057155));
#159134=CARTESIAN_POINT('Ctrl Pts',(-2.50464288823322,6.54889372085846,
9.84286862296723));
#159135=CARTESIAN_POINT('Ctrl Pts',(-2.44838285924885,6.57013401149062,
9.8401257353629));
#159136=CARTESIAN_POINT('Ctrl Pts',(-2.39188062497575,6.59063985045197,
9.83738284775858));
#159137=CARTESIAN_POINT('Ctrl Pts',(-2.21905343384968,6.65336244177899,
9.82899299262579));
#159138=CARTESIAN_POINT('Ctrl Pts',(-2.04361021329538,6.70933634883603,
9.82060313749299));
#159139=CARTESIAN_POINT('Ctrl Pts',(-1.86610484110358,6.75834885785795,
9.8122132823602));
#159140=CARTESIAN_POINT('Ctrl Pts',(-1.68876326838071,6.80731613882366,
9.8038311692681));
#159141=CARTESIAN_POINT('Ctrl Pts',(-1.50936365283739,6.84933474068126,
9.79544905617602));
#159142=CARTESIAN_POINT('Ctrl Pts',(-1.32847692186159,6.88424110781872,
9.78706694308393));
#159143=CARTESIAN_POINT('Ctrl Pts',(-1.1477305206512,6.91912039501348,9.77869133273506));
#159144=CARTESIAN_POINT('Ctrl Pts',(-0.965499625721145,6.94689838581222,
9.77031572238618));
#159145=CARTESIAN_POINT('Ctrl Pts',(-0.782367750467858,6.96746203904462,
9.76194011203731));
#159146=CARTESIAN_POINT('Ctrl Pts',(-0.599351067883436,6.9880127574338,
9.75356977007172));
#159147=CARTESIAN_POINT('Ctrl Pts',(-0.415434860816468,7.00135814988574,
9.74519942810614));
#159148=CARTESIAN_POINT('Ctrl Pts',(-0.231210660255876,7.00743663496746,
9.73682908614055));
#159149=CARTESIAN_POINT('Ctrl Pts',(-0.0470753342545793,7.01351218762943,
9.72846278224624));
#159150=CARTESIAN_POINT('Ctrl Pts',(0.137367360980391,7.01232781312478,
9.72009647835192));
#159151=CARTESIAN_POINT('Ctrl Pts',(0.3215225121874,7.00387391638775,9.71173017445761));
#159152=CARTESIAN_POINT('Ctrl Pts',(0.505626160360471,6.99542238396868,
9.70336621038399));
#159153=CARTESIAN_POINT('Ctrl Pts',(0.689442096772502,6.97970539686829,
9.69500224631038));
#159154=CARTESIAN_POINT('Ctrl Pts',(0.872376589461687,6.95676545879328,
9.68663828223676));
#159155=CARTESIAN_POINT('Ctrl Pts',(1.05528293157237,6.93382905079353,9.67827560523823));
#159156=CARTESIAN_POINT('Ctrl Pts',(1.23730777438916,6.9036719487937,9.66991292823969));
#159157=CARTESIAN_POINT('Ctrl Pts',(1.4178632597763,6.86638844947448,9.66155025124115));
#159158=CARTESIAN_POINT('Ctrl Pts',(1.59841502785603,6.82910571775436,9.65318774641485));
#159159=CARTESIAN_POINT('Ctrl Pts',(1.77749717705043,6.784696948129,9.64482524158854));
#159160=CARTESIAN_POINT('Ctrl Pts',(1.95453235461456,6.73330749611696,9.63646273676223));
#159161=CARTESIAN_POINT('Ctrl Pts',(2.13158748487691,6.68191225227167,9.62809928944225));
#159162=CARTESIAN_POINT('Ctrl Pts',(2.30659486809438,6.62353484960426,9.61973584212229));
#159163=CARTESIAN_POINT('Ctrl Pts',(2.47899220149725,6.55837054666903,9.61137239480231));
#159164=CARTESIAN_POINT('Ctrl Pts',(2.65149104729497,6.4931678731609,9.60300402284951));
#159165=CARTESIAN_POINT('Ctrl Pts',(2.82137646415526,6.42117042921805,9.59463565089669));
#159166=CARTESIAN_POINT('Ctrl Pts',(2.98810506373554,6.34262206745586,9.58626727894389));
#159167=CARTESIAN_POINT('Ctrl Pts',(3.15488361956161,6.26405017055167,9.57789639960814));
#159168=CARTESIAN_POINT('Ctrl Pts',(3.31850317695768,6.17892358688459,9.56952552027242));
#159169=CARTESIAN_POINT('Ctrl Pts',(3.47844422946308,6.08753253009912,9.56115464093668));
#159170=CARTESIAN_POINT('Ctrl Pts',(3.63852079829292,5.9960640386594,9.55277666904538));
#159171=CARTESIAN_POINT('Ctrl Pts',(3.79491235148339,5.89832063598326,9.54439869715408));
#159172=CARTESIAN_POINT('Ctrl Pts',(3.94712670689393,5.79463694481584,9.53602072526279));
#159173=CARTESIAN_POINT('Ctrl Pts',(4.0438601692439,5.7287451147792,9.53069645590377));
#159174=CARTESIAN_POINT('Ctrl Pts',(4.13890717369984,5.66045504662206,9.52537218654476));
#159175=CARTESIAN_POINT('Ctrl Pts',(4.23214814517252,5.58986123618582,9.52004791718574));
#159176=CARTESIAN_POINT('Ctrl Pts',(4.36984553972143,5.48560895722712,9.51218508599645));
#159177=CARTESIAN_POINT('Ctrl Pts',(4.50388872818022,5.37611348052248,9.50432225480718));
#159178=CARTESIAN_POINT('Ctrl Pts',(4.63383618386604,5.26167167196832,9.49645942361791));
#159179=CARTESIAN_POINT('Ctrl Pts',(4.76368379208507,5.14731779683784,9.48860263397651));
#159180=CARTESIAN_POINT('Ctrl Pts',(4.88944164157285,5.02802539826285,9.48074584433512));
#159181=CARTESIAN_POINT('Ctrl Pts',(5.01069854977613,4.90413362437968,9.47288905469373));
#159182=CARTESIAN_POINT('Ctrl Pts',(5.13188707482306,4.78031171959238,9.46503669590978));
#159183=CARTESIAN_POINT('Ctrl Pts',(5.2485794420259,4.65189587085154,9.45718433712582));
#159184=CARTESIAN_POINT('Ctrl Pts',(5.36039904202615,4.51926417381692,9.44933197834187));
#159185=CARTESIAN_POINT('Ctrl Pts',(5.47219224011429,4.38666379267334,9.44148147359145));
#159186=CARTESIAN_POINT('Ctrl Pts',(5.5791147088633,4.24984983017525,9.43363096884102));
#159187=CARTESIAN_POINT('Ctrl Pts',(5.68082814214468,4.10923571749261,9.42578046409059));
#159188=CARTESIAN_POINT('Ctrl Pts',(5.78252521294037,3.96864422518894,9.41793122223895));
#159189=CARTESIAN_POINT('Ctrl Pts',(5.87901469524553,3.82425411056282,9.41008198038731));
#159190=CARTESIAN_POINT('Ctrl Pts',(5.9700001664025,3.67650983619711,9.40223273853567));
#159191=CARTESIAN_POINT('Ctrl Pts',(6.06101629234551,3.52871578389365,9.39438085212082));
#159192=CARTESIAN_POINT('Ctrl Pts',(6.14652450283271,3.37756563973237,9.38652896570598));
#159193=CARTESIAN_POINT('Ctrl Pts',(6.226273013965,3.22353081543688,9.37867707929113));
#159194=CARTESIAN_POINT('Ctrl Pts',(6.28483135307956,3.11042496118986,9.37291153682718));
#159195=CARTESIAN_POINT('Ctrl Pts',(6.34028511368452,2.99576432463116,9.36714599436324));
#159196=CARTESIAN_POINT('Ctrl Pts',(6.39255086948598,2.87974303428865,9.36138045189929));
#159197=CARTESIAN_POINT('Ctrl Pts',(6.45696418237184,2.7367561863678,9.35427488755813));
#159198=CARTESIAN_POINT('Ctrl Pts',(6.51651601396806,2.59174708930409,9.34716932321697));
#159199=CARTESIAN_POINT('Ctrl Pts',(6.57110895151814,2.44502632087636,9.34006375887581));
#159200=CARTESIAN_POINT('Origin',(0.,0.,50.));
#159201=CARTESIAN_POINT('',(6.57110895151814,2.44502632087637,7.33978485479521));
#159202=CARTESIAN_POINT('',(6.57110895151813,2.44502632087637,7.88693503181338));
#159203=CARTESIAN_POINT('',(6.57110895151814,2.44502632087636,50.));
#159204=CARTESIAN_POINT('',(7.01124998073505,0.000519752639607968,9.77353435687236));
#159205=CARTESIAN_POINT('Ctrl Pts',(6.57110895151814,2.44502632087637,7.88693503181337));
#159206=CARTESIAN_POINT('Ctrl Pts',(6.49628307728171,2.64612394007251,7.89670751236697));
#159207=CARTESIAN_POINT('Ctrl Pts',(6.41220863601586,2.84382046692177,7.90647999292057));
#159208=CARTESIAN_POINT('Ctrl Pts',(6.31918628001434,3.03735268300844,7.91625247347417));
#159209=CARTESIAN_POINT('Ctrl Pts',(6.29182779425026,3.09427177865692,7.91912662417941));
#159210=CARTESIAN_POINT('Ctrl Pts',(6.26369565058952,3.15083077630124,7.92200077488466));
#159211=CARTESIAN_POINT('Ctrl Pts',(6.23479831148065,3.20701053594434,7.9248749255899));
#159212=CARTESIAN_POINT('Ctrl Pts',(6.15403231604373,3.36402894493653,7.93290797118868));
#159213=CARTESIAN_POINT('Ctrl Pts',(6.06724655878222,3.51815830011378,7.94094101678745));
#159214=CARTESIAN_POINT('Ctrl Pts',(5.97467924385627,3.66890099287689,7.94897406238623));
#159215=CARTESIAN_POINT('Ctrl Pts',(5.88217143476448,3.81954678243306,7.95700194403399));
#159216=CARTESIAN_POINT('Ctrl Pts',(5.78388965702759,3.9668099320284,7.96502982568177));
#159217=CARTESIAN_POINT('Ctrl Pts',(5.68011830557492,4.11021685524896,7.97305770732953));
#159218=CARTESIAN_POINT('Ctrl Pts',(5.5763938079104,4.25355902883001,7.9810819643096));
#159219=CARTESIAN_POINT('Ctrl Pts',(5.46718488614912,4.39304814645702,7.98910622128966));
#159220=CARTESIAN_POINT('Ctrl Pts',(5.35281953635889,4.52823912505453,7.99713047826972));
#159221=CARTESIAN_POINT('Ctrl Pts',(5.2384680145043,4.66341375768576,8.00515376503539));
#159222=CARTESIAN_POINT('Ctrl Pts',(5.11896153718186,4.79429100174109,8.01317705180106));
#159223=CARTESIAN_POINT('Ctrl Pts',(4.99466882432703,4.92045830160115,8.02120033856673));
#159224=CARTESIAN_POINT('Ctrl Pts',(4.87038629615114,5.04661526317659,8.02922296789562));
#159225=CARTESIAN_POINT('Ctrl Pts',(4.7413185738181,5.16806279093765,8.03724559722452));
#159226=CARTESIAN_POINT('Ctrl Pts',(4.60787150224812,5.28442492436685,8.04526822655342));
#159227=CARTESIAN_POINT('Ctrl Pts',(4.47437426407975,5.40083080167404,8.05329387181978));
#159228=CARTESIAN_POINT('Ctrl Pts',(4.33649466631384,5.5121472268049,8.06131951708615));
#159229=CARTESIAN_POINT('Ctrl Pts',(4.1946722069539,5.6180380595639,8.06934516235251));
#159230=CARTESIAN_POINT('Ctrl Pts',(4.11104504267748,5.68047774723022,8.07407757186045));
#159231=CARTESIAN_POINT('Ctrl Pts',(4.02604755290439,5.7410317358922,8.0788099813684));
#159232=CARTESIAN_POINT('Ctrl Pts',(3.93977462314065,5.79963813365601,8.08354239087634));
#159233=CARTESIAN_POINT('Ctrl Pts',(3.78062379549445,5.90775149824227,8.09227243971103));
#159234=CARTESIAN_POINT('Ctrl Pts',(3.61705163562554,6.00928900419594,8.10100248854573));
#159235=CARTESIAN_POINT('Ctrl Pts',(3.44961244000387,6.10391682252228,8.10973253738042));
#159236=CARTESIAN_POINT('Ctrl Pts',(3.28212482912982,6.1985720026004,8.11846511051963));
#159237=CARTESIAN_POINT('Ctrl Pts',(3.11076818908985,6.28631337226274,8.12719768365884));
#159238=CARTESIAN_POINT('Ctrl Pts',(2.93612178165304,6.36685286823896,8.13593025679805));
#159239=CARTESIAN_POINT('Ctrl Pts',(2.75899424321187,6.44853655632009,8.14478689007845));
#159240=CARTESIAN_POINT('Ctrl Pts',(2.57848301538312,6.5228120615465,8.15364352335883));
#159241=CARTESIAN_POINT('Ctrl Pts',(2.39521419140986,6.58942907540318,8.16250015663922));
#159242=CARTESIAN_POINT('Ctrl Pts',(2.21439749230609,6.65515475797466,8.171238288746));
#159243=CARTESIAN_POINT('Ctrl Pts',(2.03089680065212,6.71342554354389,8.1799764208528));
#159244=CARTESIAN_POINT('Ctrl Pts',(1.84533044374377,6.76405071801598,8.18871455295959));
#159245=CARTESIAN_POINT('Ctrl Pts',(1.6559892816241,6.81570571371,8.19763043682679));
#159246=CARTESIAN_POINT('Ctrl Pts',(1.46449779898592,6.85940062961301,8.20654632069398));
#159247=CARTESIAN_POINT('Ctrl Pts',(1.27152670014793,6.89498704953903,8.21546220456118));
#159248=CARTESIAN_POINT('Ctrl Pts',(1.07855560130995,6.93057346946505,8.22437808842837));
#159249=CARTESIAN_POINT('Ctrl Pts',(0.884105184772854,6.95805134455219,
8.23329397229557));
#159250=CARTESIAN_POINT('Ctrl Pts',(0.688855744565208,6.97732787861367,
8.24220985616277));
#159251=CARTESIAN_POINT('Ctrl Pts',(0.497443005196463,6.99622562390973,
8.25095054065896));
#159252=CARTESIAN_POINT('Ctrl Pts',(0.305242022758536,7.00724336029941,
8.25969122515517));
#159253=CARTESIAN_POINT('Ctrl Pts',(0.112898462328194,7.01034096886192,
8.26843190965136));
#159254=CARTESIAN_POINT('Ctrl Pts',(-0.0794104923005177,7.01343802011321,
8.27717102155322));
#159255=CARTESIAN_POINT('Ctrl Pts',(-0.271861700031282,7.00861778488913,
8.28591013345508));
#159256=CARTESIAN_POINT('Ctrl Pts',(-0.463808403015683,6.99589224672536,
8.29464924535694));
#159257=CARTESIAN_POINT('Ctrl Pts',(-0.658242051797386,6.9830018308994,
8.30350158503129));
#159258=CARTESIAN_POINT('Ctrl Pts',(-0.852157745652109,6.96199983140085,
8.31235392470564));
#159259=CARTESIAN_POINT('Ctrl Pts',(-1.04488606462257,6.93295317122924,
8.32120626438));
#159260=CARTESIAN_POINT('Ctrl Pts',(-1.2350517303488,6.9042927361766,8.32994089702973));
#159261=CARTESIAN_POINT('Ctrl Pts',(-1.4240611257198,6.8678003025821,8.33867552967946));
#159262=CARTESIAN_POINT('Ctrl Pts',(-1.61127801080753,6.82359214302761,
8.3474101623292));
#159263=CARTESIAN_POINT('Ctrl Pts',(-1.80227926955795,6.77849036645446,
8.35632135551586));
#159264=CARTESIAN_POINT('Ctrl Pts',(-1.99141449157405,6.72535765834676,
8.36523254870253));
#159265=CARTESIAN_POINT('Ctrl Pts',(-2.17801974077083,6.66437218133206,
8.37414374188919));
#159266=CARTESIAN_POINT('Ctrl Pts',(-2.36462498996762,6.60338670431735,
8.38305493507585));
#159267=CARTESIAN_POINT('Ctrl Pts',(-2.54869997402684,6.53454853975444,
8.39196612826252));
#159268=CARTESIAN_POINT('Ctrl Pts',(-2.7295969416885,6.45809005034962,8.40087732144918));
#159269=CARTESIAN_POINT('Ctrl Pts',(-2.892517709408,6.38922943895561,8.40890298630158));
#159270=CARTESIAN_POINT('Ctrl Pts',(-3.05293536394447,6.31415563055696,
8.41692865115397));
#159271=CARTESIAN_POINT('Ctrl Pts',(-3.21034092784216,6.23308412341126,
8.42495431600637));
#159272=CARTESIAN_POINT('Ctrl Pts',(-3.36769653507477,6.15203834637339,
8.4329774337096));
#159273=CARTESIAN_POINT('Ctrl Pts',(-3.52204162940454,6.06499882797018,
8.44100055141283));
#159274=CARTESIAN_POINT('Ctrl Pts',(-3.6728894627452,5.97222819029509,8.44902366911607));
#159275=CARTESIAN_POINT('Ctrl Pts',(-3.82371827285366,5.87946925180945,
8.45704577503393));
#159276=CARTESIAN_POINT('Ctrl Pts',(-3.97105038861594,5.78098082615529,
8.46506788095178));
#159277=CARTESIAN_POINT('Ctrl Pts',(-4.11442586268289,5.6770702288228,8.47308998686965));
#159278=CARTESIAN_POINT('Ctrl Pts',(-4.2578546155606,5.57312101796113,8.48111507382918));
#159279=CARTESIAN_POINT('Ctrl Pts',(-4.3973234906917,5.46374582318037,8.48914016078872));
#159280=CARTESIAN_POINT('Ctrl Pts',(-4.53240325157572,5.3492940961968,8.49716524774825));
#159281=CARTESIAN_POINT('Ctrl Pts',(-4.66750961574264,5.23481982851836,
8.5051919152085));
#159282=CARTESIAN_POINT('Ctrl Pts',(-4.79822486962966,5.11526728056,8.51321858266876));
#159283=CARTESIAN_POINT('Ctrl Pts',(-4.92415497177501,4.99102438147155,
8.52124525012901));
#159284=CARTESIAN_POINT('Ctrl Pts',(-5.05018617016269,4.86668174062144,
8.52927836136961));
#159285=CARTESIAN_POINT('Ctrl Pts',(-5.17142428999715,4.73764149221596,
8.53731147261022));
#159286=CARTESIAN_POINT('Ctrl Pts',(-5.28751366212846,4.60432686017239,
8.54534458385083));
#159287=CARTESIAN_POINT('Ctrl Pts',(-5.35591773736397,4.52577303605498,
8.55007798481243));
#159288=CARTESIAN_POINT('Ctrl Pts',(-5.42253493239236,4.44573577773099,
8.55481138577402));
#159289=CARTESIAN_POINT('Ctrl Pts',(-5.4872993526033,4.36430663191984,8.55954478673562));
#159290=CARTESIAN_POINT('Ctrl Pts',(-5.62071607384052,4.19656005730543,
8.56929574002974));
#159291=CARTESIAN_POINT('Ctrl Pts',(-5.74634700732665,4.02280664304624,
8.57904669332387));
#159292=CARTESIAN_POINT('Ctrl Pts',(-5.8637365978661,3.84372471352278,8.58879764661799));
#159293=CARTESIAN_POINT('Ctrl Pts',(-5.98129531013271,3.66438478288451,
8.59856264798959));
#159294=CARTESIAN_POINT('Ctrl Pts',(-6.09058890837765,3.47970101358163,
8.60832764936119));
#159295=CARTESIAN_POINT('Ctrl Pts',(-6.19120518797151,3.29038065927556,
8.61809265073278));
#159296=CARTESIAN_POINT('Ctrl Pts',(-6.29165376107438,3.10137586277407,
8.62784137587034));
#159297=CARTESIAN_POINT('Ctrl Pts',(-6.38345390398281,2.90774996033089,
8.63759010100791));
#159298=CARTESIAN_POINT('Ctrl Pts',(-6.46624073214091,2.71023197466597,
8.64733882614547));
#159299=CARTESIAN_POINT('Ctrl Pts',(-6.54880034255623,2.5132560992843,8.65706079481259));
#159300=CARTESIAN_POINT('Ctrl Pts',(-6.62239600826602,2.31240950289493,
8.66678276347969));
#159301=CARTESIAN_POINT('Ctrl Pts',(-6.68671126918446,2.10843993631821,
8.6765047321468));
#159302=CARTESIAN_POINT('Ctrl Pts',(-6.75060097281963,1.90581998308961,
8.68616237308649));
#159303=CARTESIAN_POINT('Ctrl Pts',(-6.80533263618958,1.70011828665719,
8.69582001402617));
#159304=CARTESIAN_POINT('Ctrl Pts',(-6.85064147791335,1.49209178792499,
8.70547765496585));
#159305=CARTESIAN_POINT('Ctrl Pts',(-6.87055627373975,1.40065697981429,
8.70972252065125));
#159306=CARTESIAN_POINT('Ctrl Pts',(-6.88865126635412,1.30877335101945,
8.71396738633665));
#159307=CARTESIAN_POINT('Ctrl Pts',(-6.90490681962792,1.21650662750181,
8.71821225202205));
#159308=CARTESIAN_POINT('Ctrl Pts',(-6.93497517205461,1.04583828338241,
8.72606409903597));
#159309=CARTESIAN_POINT('Ctrl Pts',(-6.95873380167368,0.873928622337296,
8.73391594604989));
#159310=CARTESIAN_POINT('Ctrl Pts',(-6.97608778540275,0.701302910912703,
8.74176779306381));
#159311=CARTESIAN_POINT('Ctrl Pts',(-6.99343684768233,0.528726154744227,
8.7496174133574));
#159312=CARTESIAN_POINT('Ctrl Pts',(-7.00438483889631,0.355434131305913,
8.75746703365098));
#159313=CARTESIAN_POINT('Ctrl Pts',(-7.00888845738292,0.181959210991192,
8.76531665394457));
#159314=CARTESIAN_POINT('Ctrl Pts',(-7.01339171631319,0.00849814043011765,
8.77316564754637));
#159315=CARTESIAN_POINT('Ctrl Pts',(-7.01145161759505,-0.16514541658381,
8.78101464114818));
#159316=CARTESIAN_POINT('Ctrl Pts',(-7.00307694641226,-0.338437357762359,
8.78886363474999));
#159317=CARTESIAN_POINT('Ctrl Pts',(-6.99469803537867,-0.511817031576421,
8.79671660206742));
#159318=CARTESIAN_POINT('Ctrl Pts',(-6.97987806139873,-0.684844352360426,
8.80456956938485));
#159319=CARTESIAN_POINT('Ctrl Pts',(-6.95867786783105,-0.856988269615363,
8.81242253670229));
#159320=CARTESIAN_POINT('Ctrl Pts',(-6.93747229012655,-1.02917590564115,
8.82027749840955));
#159321=CARTESIAN_POINT('Ctrl Pts',(-6.90988332535711,-1.20047931451484,
8.8281324601168));
#159322=CARTESIAN_POINT('Ctrl Pts',(-6.87602316633129,-1.37037658275942,
8.83598742182406));
#159323=CARTESIAN_POINT('Ctrl Pts',(-6.8421293982673,-1.54044248824431,
8.84385018023741));
#159324=CARTESIAN_POINT('Ctrl Pts',(-6.80195209202671,-1.70909909458856,
8.85171293865077));
#159325=CARTESIAN_POINT('Ctrl Pts',(-6.75565379072281,-1.87583805868005,
8.85957569706412));
#159326=CARTESIAN_POINT('Ctrl Pts',(-6.72169002122761,-1.99815537017491,
8.86534370381225));
#159327=CARTESIAN_POINT('Ctrl Pts',(-6.68443330330044,-2.11944099994925,
8.87111171056036));
#159328=CARTESIAN_POINT('Ctrl Pts',(-6.64396427386324,-2.23950112527966,
8.87687971730848));
#159329=CARTESIAN_POINT('Ctrl Pts',(-6.58518275153944,-2.41388921996474,
8.88525778374951));
#159330=CARTESIAN_POINT('Ctrl Pts',(-6.51949218948711,-2.58607740822038,
8.89363585019053));
#159331=CARTESIAN_POINT('Ctrl Pts',(-6.44707966720527,-2.75550182856199,
8.90201391663155));
#159332=CARTESIAN_POINT('Ctrl Pts',(-6.37471665974576,-2.92481039849804,
8.91038625425029));
#159333=CARTESIAN_POINT('Ctrl Pts',(-6.29564098469207,-3.09135866697574,
8.91875859186902));
#159334=CARTESIAN_POINT('Ctrl Pts',(-6.21008852409888,-3.25460091030458,
8.92713092948775));
#159335=CARTESIAN_POINT('Ctrl Pts',(-6.12458201693686,-3.41775547010987,
8.93549877001035));
#159336=CARTESIAN_POINT('Ctrl Pts',(-6.03260581313219,-3.57760725501266,
8.94386661053294));
#159337=CARTESIAN_POINT('Ctrl Pts',(-5.93444279738993,-3.73363298236541,
8.95223445105553));
#159338=CARTESIAN_POINT('Ctrl Pts',(-5.83631812851099,-3.88959775909232,
8.96059902272545));
#159339=CARTESIAN_POINT('Ctrl Pts',(-5.73201164201706,-4.04173918095498,
8.96896359439538));
#159340=CARTESIAN_POINT('Ctrl Pts',(-5.62185104212056,-4.18956052858864,
8.9773281660653));
#159341=CARTESIAN_POINT('Ctrl Pts',(-5.51171735102767,-4.33734576807097,
8.98569069453087));
#159342=CARTESIAN_POINT('Ctrl Pts',(-5.39573259483072,-4.48081277470594,
8.99405322299644));
#159343=CARTESIAN_POINT('Ctrl Pts',(-5.27426674904245,-4.61949529953708,
9.00241575146201));
#159344=CARTESIAN_POINT('Ctrl Pts',(-5.15279120989962,-4.75818889166765,
9.01077894728352));
#159345=CARTESIAN_POINT('Ctrl Pts',(-5.02583391929153,-4.89209698795397,
9.01914214310503));
#159346=CARTESIAN_POINT('Ctrl Pts',(-4.89380445364757,-5.02078724225188,
9.02750533892654));
#159347=CARTESIAN_POINT('Ctrl Pts',(-4.76176598385867,-5.14948627296721,
9.03586910510124));
#159348=CARTESIAN_POINT('Ctrl Pts',(-4.6246548845979,-5.27296652245916,
9.04423287127595));
#159349=CARTESIAN_POINT('Ctrl Pts',(-4.48291695154482,-5.3908331608437,
9.05259663745066));
#159350=CARTESIAN_POINT('Ctrl Pts',(-4.34115045524832,-5.50872355189213,
9.06096208910422));
#159351=CARTESIAN_POINT('Ctrl Pts',(-4.19475551872438,-5.62099786585431,
9.06932754075776));
#159352=CARTESIAN_POINT('Ctrl Pts',(-4.04421063405157,-5.7273018874444,
9.07769299241132));
#159353=CARTESIAN_POINT('Ctrl Pts',(-3.89361533219282,-5.83364151004235,
9.0860612456382));
#159354=CARTESIAN_POINT('Ctrl Pts',(-3.7388675793336,-5.93400666375764,
9.09442949886508));
#159355=CARTESIAN_POINT('Ctrl Pts',(-3.58047477207803,-6.02808650974858,
9.10279775209195));
#159356=CARTESIAN_POINT('Ctrl Pts',(-3.421935112093,-6.12225358117866,9.11117376388342));
#159357=CARTESIAN_POINT('Ctrl Pts',(-3.25974392746319,-6.21012353197168,
9.11954977567489));
#159358=CARTESIAN_POINT('Ctrl Pts',(-3.09443422830602,-6.29143094766112,
9.12792578746637));
#159359=CARTESIAN_POINT('Ctrl Pts',(-2.92904345922981,-6.37277823751186,
9.13630590695752));
#159360=CARTESIAN_POINT('Ctrl Pts',(-2.76053142351737,-6.44755643510344,
9.14468602644866));
#159361=CARTESIAN_POINT('Ctrl Pts',(-2.58945162577646,-6.51554808441037,
9.15306614593981));
#159362=CARTESIAN_POINT('Ctrl Pts',(-2.41817634769534,-6.58361742278939,
9.16145584077902));
#159363=CARTESIAN_POINT('Ctrl Pts',(-2.24432775285461,-6.64488460241941,
9.16984553561824));
#159364=CARTESIAN_POINT('Ctrl Pts',(-2.06847631044044,-6.6991814660932,
9.17823523045745));
#159365=CARTESIAN_POINT('Ctrl Pts',(-1.95683126427435,-6.73365360785283,
9.18356170293207));
#159366=CARTESIAN_POINT('Ctrl Pts',(-1.84437920556129,-6.76531719248854,
9.1888881754067));
#159367=CARTESIAN_POINT('Ctrl Pts',(-1.73126837294955,-6.79413985603216,
9.19421464788132));
#159368=CARTESIAN_POINT('Ctrl Pts',(-1.55328643993816,-6.8394928364106,
9.20259594828622));
#159369=CARTESIAN_POINT('Ctrl Pts',(-1.37331386193084,-6.87790078047717,
9.21097724869112));
#159370=CARTESIAN_POINT('Ctrl Pts',(-1.1919184300458,-6.90919365907609,
9.21935854909601));
#159371=CARTESIAN_POINT('Ctrl Pts',(-1.01075289031636,-6.94044687853232,
9.22772922742957));
#159372=CARTESIAN_POINT('Ctrl Pts',(-0.828168410681715,-6.96460294782168,
9.23609990576311));
#159373=CARTESIAN_POINT('Ctrl Pts',(-0.644746374589701,-6.98154199836637,
9.24447058409667));
#159374=CARTESIAN_POINT('Ctrl Pts',(-0.46153249101654,-6.99846182599699,
9.2528317631475));
#159375=CARTESIAN_POINT('Ctrl Pts',(-0.277483269681747,-7.00818092866042,
9.26119294219835));
#159376=CARTESIAN_POINT('Ctrl Pts',(-0.0931891295821639,-7.01063066696768,
9.26955412124917));
#159377=CARTESIAN_POINT('Ctrl Pts',(0.0908658671312361,-7.01307722645052,
9.27790445068389));
#159378=CARTESIAN_POINT('Ctrl Pts',(0.275164822626464,-7.00827323207764,
9.28625478011861));
#159379=CARTESIAN_POINT('Ctrl Pts',(0.459113446337256,-6.99620192718109,
9.29460510955333));
#159380=CARTESIAN_POINT('Ctrl Pts',(0.64292053258566,-6.98413991043156,
9.30294901390906));
#159381=CARTESIAN_POINT('Ctrl Pts',(0.826377498673072,-6.96482174788353,
9.31129291826479));
#159382=CARTESIAN_POINT('Ctrl Pts',(1.00889015050328,-6.93828272894075,
9.31963682262052));
#159383=CARTESIAN_POINT('Ctrl Pts',(1.19125620703326,-6.9117650263035,9.32797402510024));
#159384=CARTESIAN_POINT('Ctrl Pts',(1.37267913868257,-6.87803808123059,
9.33631122757996));
#159385=CARTESIAN_POINT('Ctrl Pts',(1.55256981481071,-6.83718900811135,
9.34464843005967));
#159386=CARTESIAN_POINT('Ctrl Pts',(1.61178883241873,-6.82374171872212,
9.34739299109571));
#159387=CARTESIAN_POINT('Ctrl Pts',(1.67084185141757,-6.80952302812026,
9.35013755213173));
#159388=CARTESIAN_POINT('Ctrl Pts',(1.72970803380628,-6.79453726756179,
9.35288211316777));
#159389=CARTESIAN_POINT('Ctrl Pts',(1.90855065694367,-6.74900870397519,
9.36122042346967));
#159390=CARTESIAN_POINT('Ctrl Pts',(2.08552113087069,-6.69643353800162,
9.36955873377158));
#159391=CARTESIAN_POINT('Ctrl Pts',(2.26005401679439,-6.63700100976876,
9.37789704407349));
#159392=CARTESIAN_POINT('Ctrl Pts',(2.43469671288792,-6.57753108860572,
9.38624060055731));
#159393=CARTESIAN_POINT('Ctrl Pts',(2.60689845176619,-6.5111953051539,9.39458415704114));
#159394=CARTESIAN_POINT('Ctrl Pts',(2.77611294521756,-6.43823139362787,
9.40292771352497));
#159395=CARTESIAN_POINT('Ctrl Pts',(2.94545617631766,-6.36521197147612,
9.41127761775018));
#159396=CARTESIAN_POINT('Ctrl Pts',(3.11180732819729,-6.28555449239434,
9.41962752197539));
#159397=CARTESIAN_POINT('Ctrl Pts',(3.27464352290386,-6.19954323804615,
9.42797742620061));
#159398=CARTESIAN_POINT('Ctrl Pts',(3.43772395985251,-6.11340297318133,
9.43633985466426));
#159399=CARTESIAN_POINT('Ctrl Pts',(3.59727861419359,-6.02089004189167,
9.4447022831279));
#159400=CARTESIAN_POINT('Ctrl Pts',(3.75281118749222,-5.92233355642295,
9.45306471159156));
#159401=CARTESIAN_POINT('Ctrl Pts',(3.90847676234316,-5.82369279172396,
9.46143429107151));
#159402=CARTESIAN_POINT('Ctrl Pts',(4.06011312461653,-5.71899834694114,
9.46980387055147));
#159403=CARTESIAN_POINT('Ctrl Pts',(4.20725559066611,-5.60862077139369,
9.47817345003142));
#159404=CARTESIAN_POINT('Ctrl Pts',(4.35462500604198,-5.49807295188418,
9.48655593856799));
#159405=CARTESIAN_POINT('Ctrl Pts',(4.49748642076467,-5.38182469185198,
9.49493842710455));
#159406=CARTESIAN_POINT('Ctrl Pts',(4.63540959522959,-5.26028558606408,
9.50332091564112));
#159407=CARTESIAN_POINT('Ctrl Pts',(4.68054031791934,-5.22051599911428,
9.50606380324548));
#159408=CARTESIAN_POINT('Ctrl Pts',(4.72514260623293,-5.18018020006754,
9.50880669084984));
#159409=CARTESIAN_POINT('Ctrl Pts',(4.76920229736288,-5.13929333754444,
9.5115495784542));
#159410=CARTESIAN_POINT('Ctrl Pts',(4.90163784191209,-5.0163947478293,9.51979420759718));
#159411=CARTESIAN_POINT('Ctrl Pts',(5.02946326007933,-4.88824085956467,
9.52803883674016));
#159412=CARTESIAN_POINT('Ctrl Pts',(5.15224421891428,-4.75520830996544,
9.53628346588314));
#159413=CARTESIAN_POINT('Ctrl Pts',(5.27490518171818,-4.62230577546061,
9.54452003740233));
#159414=CARTESIAN_POINT('Ctrl Pts',(5.39253127495641,-4.48453433245291,
9.55275660892152));
#159415=CARTESIAN_POINT('Ctrl Pts',(5.50472345142624,-4.34230886577843,
9.56099318044071));
#159416=CARTESIAN_POINT('Ctrl Pts',(5.61682639527973,-4.20019651884993,
9.56922320096099));
#159417=CARTESIAN_POINT('Ctrl Pts',(5.72350382148417,-4.05363747813611,
9.57745322148126));
#159418=CARTESIAN_POINT('Ctrl Pts',(5.82439541115204,-3.90308143100437,
9.58568324200154));
#159419=CARTESIAN_POINT('Ctrl Pts',(5.92521986830862,-3.75262556274348,
9.59390778632754));
#159420=CARTESIAN_POINT('Ctrl Pts',(6.02026597205407,-3.5981782768221,9.60213233065354));
#159421=CARTESIAN_POINT('Ctrl Pts',(6.1092152791352,-3.44022023069469,9.61035687497954));
#159422=CARTESIAN_POINT('Ctrl Pts',(6.19813176112689,-3.28232047604994,
9.61857838419024));
#159423=CARTESIAN_POINT('Ctrl Pts',(6.2809557596573,-3.12091284334057,9.62679989340093));
#159424=CARTESIAN_POINT('Ctrl Pts',(6.35741332620368,-2.95650509255571,
9.63502140261163));
#159425=CARTESIAN_POINT('Ctrl Pts',(6.4338552822269,-2.79213090929226,9.64324123321724));
#159426=CARTESIAN_POINT('Ctrl Pts',(6.50393325101697,-2.62475814206892,
9.65146106382287));
#159427=CARTESIAN_POINT('Ctrl Pts',(6.56742014076435,-2.45491736259751,
9.65968089442848));
#159428=CARTESIAN_POINT('Ctrl Pts',(6.63090453343465,-2.28508326333237,
9.66790040173033));
#159429=CARTESIAN_POINT('Ctrl Pts',(6.68779824362939,-2.11278166948833,
9.67611990903217));
#159430=CARTESIAN_POINT('Ctrl Pts',(6.73792297411684,-1.93856146597638,
9.68433941633402));
#159431=CARTESIAN_POINT('Ctrl Pts',(6.78806944695646,-1.76426569184326,
9.6925624889702));
#159432=CARTESIAN_POINT('Ctrl Pts',(6.83144097603342,-1.58804997731326,
9.70078556160637));
#159433=CARTESIAN_POINT('Ctrl Pts',(6.86790944372065,-1.41047737853278,
9.70900863424255));
#159434=CARTESIAN_POINT('Ctrl Pts',(6.90438617357222,-1.2328645495456,9.71723356986837));
#159435=CARTESIAN_POINT('Ctrl Pts',(6.9339566615384,-1.05389456364962,9.72545850549418));
#159436=CARTESIAN_POINT('Ctrl Pts',(6.95654419597645,-0.874139240582622,
9.73368344112));
#159437=CARTESIAN_POINT('Ctrl Pts',(6.97914965908088,-0.694241238232732,
9.74191490521962));
#159438=CARTESIAN_POINT('Ctrl Pts',(6.99476105883144,-0.513556997444592,
9.75014636931923));
#159439=CARTESIAN_POINT('Ctrl Pts',(7.00335362096458,-0.332662925830885,
9.75837783341885));
#159440=CARTESIAN_POINT('Ctrl Pts',(7.0086274243415,-0.221636697453453,
9.76343000790335));
#159441=CARTESIAN_POINT('Ctrl Pts',(7.01125821309936,-0.110531466213418,
9.76848218238786));
#159442=CARTESIAN_POINT('Ctrl Pts',(7.01124998073505,0.000519752639607109,
9.77353435687236));
#159443=CARTESIAN_POINT('Ctrl Pts',(7.01124998073499,0.000519753478595656,
9.77353435691053));
#159444=CARTESIAN_POINT('Ctrl Pts',(7.01122549278315,0.330851649082017,
9.78856250690858));
#159445=CARTESIAN_POINT('Ctrl Pts',(6.98785181828166,0.660634656774128,
9.80359065690662));
#159446=CARTESIAN_POINT('Ctrl Pts',(6.94138454713677,0.987323215198966,
9.81861880690467));
#159447=CARTESIAN_POINT('Ctrl Pts',(6.93080397747084,1.06171000328255,9.82204070761214));
#159448=CARTESIAN_POINT('Ctrl Pts',(6.91902627410213,1.13593643056938,9.82546260831958));
#159449=CARTESIAN_POINT('Ctrl Pts',(6.90605482080883,1.20997246848147,9.82888450902704));
#159450=CARTESIAN_POINT('Ctrl Pts',(6.87624591910682,1.38011014901938,9.83674816929057));
#159451=CARTESIAN_POINT('Ctrl Pts',(6.84010208160346,1.54939332710809,9.8446118295541));
#159452=CARTESIAN_POINT('Ctrl Pts',(6.79768561947328,1.71729344647505,9.85247548981762));
#159453=CARTESIAN_POINT('Ctrl Pts',(6.75530637964033,1.88504622615753,9.86033224937598));
#159454=CARTESIAN_POINT('Ctrl Pts',(6.706665562064,2.05141799498684,9.86818900893433));
#159455=CARTESIAN_POINT('Ctrl Pts',(6.65187693518678,2.2158880390557,9.87604576849268));
#159456=CARTESIAN_POINT('Ctrl Pts',(6.62628932079653,2.29269952907191,9.87971506530471));
#159457=CARTESIAN_POINT('Ctrl Pts',(6.59936152799537,2.36909635782941,9.88338436211673));
#159458=CARTESIAN_POINT('Ctrl Pts',(6.57110895151814,2.44502632087636,9.88705365892876));
#159459=CARTESIAN_POINT('',(7.01124990260052,0.0011686677202812,9.22646564312219));
#159460=CARTESIAN_POINT('Ctrl Pts',(6.57110895151814,2.44502632087636,9.34006375887581));
#159461=CARTESIAN_POINT('Ctrl Pts',(6.6443561952353,2.24817133622682,9.33053023629209));
#159462=CARTESIAN_POINT('Ctrl Pts',(6.70867476342362,2.04823487019919,9.32099671370838));
#159463=CARTESIAN_POINT('Ctrl Pts',(6.76387515396249,1.84597385249871,9.31146319112466));
#159464=CARTESIAN_POINT('Ctrl Pts',(6.8192203234386,1.64318234697191,9.30190466412966));
#159465=CARTESIAN_POINT('Ctrl Pts',(6.86539944347675,1.43805418440369,9.29234613713465));
#159466=CARTESIAN_POINT('Ctrl Pts',(6.90227373070976,1.23135856226121,9.28278761013965));
#159467=CARTESIAN_POINT('Ctrl Pts',(6.93922415287218,1.02423617236859,9.2732093475014));
#159468=CARTESIAN_POINT('Ctrl Pts',(6.96683128480148,0.815539939704676,
9.26363108486317));
#159469=CARTESIAN_POINT('Ctrl Pts',(6.98500763070788,0.606048646110736,
9.25405282222492));
#159470=CARTESIAN_POINT('Ctrl Pts',(7.00245805043746,0.404924007432989,
9.24485709585735));
#159471=CARTESIAN_POINT('Ctrl Pts',(7.01121624930699,0.203066646850565,
9.23566136948977));
#159472=CARTESIAN_POINT('Ctrl Pts',(7.01124990260052,0.00116866772027653,
9.2264656431222));
#159473=CARTESIAN_POINT('Ctrl Pts',(7.01124990260064,0.00116866700544844,
9.22646564308963));
#159474=CARTESIAN_POINT('Ctrl Pts',(7.01127887818486,-0.172666190258528,
9.21854809093071));
#159475=CARTESIAN_POINT('Ctrl Pts',(7.00484218383645,-0.346555053651323,
9.21063053877179));
#159476=CARTESIAN_POINT('Ctrl Pts',(6.99193196050225,-0.520109625182228,
9.20271298661287));
#159477=CARTESIAN_POINT('Ctrl Pts',(6.97883341556641,-0.696195839585311,
9.19467994101399));
#159478=CARTESIAN_POINT('Ctrl Pts',(6.9590649918697,-0.871970795754378,
9.1866468954151));
#159479=CARTESIAN_POINT('Ctrl Pts',(6.93265185505888,-1.04688338369119,
9.17861384981622));
#159480=CARTESIAN_POINT('Ctrl Pts',(6.90625569762941,-1.22168353108165,
9.17058596816835));
#159481=CARTESIAN_POINT('Ctrl Pts',(6.8732233840713,-1.39562205276577,9.16255808652047));
#159482=CARTESIAN_POINT('Ctrl Pts',(6.83363198264051,-1.56815193407168,
9.15453020487261));
#159483=CARTESIAN_POINT('Ctrl Pts',(6.79405845711781,-1.74060391643517,
9.14650594789245));
#159484=CARTESIAN_POINT('Ctrl Pts',(6.74793182221218,-1.9116481682579,9.1384816909123));
#159485=CARTESIAN_POINT('Ctrl Pts',(6.69538041288335,-2.0807469065886,9.13045743393214));
#159486=CARTESIAN_POINT('Ctrl Pts',(6.64283535755508,-2.24982519915979,
9.12243414716638));
#159487=CARTESIAN_POINT('Ctrl Pts',(6.58386717645966,-2.41695809464307,
9.11441086040061));
#159488=CARTESIAN_POINT('Ctrl Pts',(6.518654392187,-2.58162186962405,9.10638757363485));
#159489=CARTESIAN_POINT('Ctrl Pts',(6.45344695152034,-2.74627215187738,
9.09836494430587));
#159490=CARTESIAN_POINT('Ctrl Pts',(6.38199606565139,-2.9084533772295,9.09034231497688));
#159491=CARTESIAN_POINT('Ctrl Pts',(6.30452871829496,-3.06766103125723,
9.0823196856479));
#159492=CARTESIAN_POINT('Ctrl Pts',(6.22703224873098,-3.22692853602856,
9.07429404038144));
#159493=CARTESIAN_POINT('Ctrl Pts',(6.14351496262899,-3.38321990785342,
9.06626839511497));
#159494=CARTESIAN_POINT('Ctrl Pts',(6.05425036654084,-3.53605416555518,
9.05824274984851));
#159495=CARTESIAN_POINT('Ctrl Pts',(6.00161452117611,-3.62617455714782,
9.05351034034116));
#159496=CARTESIAN_POINT('Ctrl Pts',(5.94698119959167,-3.71509339081393,
9.0487779308338));
#159497=CARTESIAN_POINT('Ctrl Pts',(5.89041361735245,-3.80271665773416,
9.04404552132645));
#159498=CARTESIAN_POINT('Ctrl Pts',(5.78606133029057,-3.96435850171983,
9.03531547249181));
#159499=CARTESIAN_POINT('Ctrl Pts',(5.67507237408558,-4.12167082863513,
9.02658542365718));
#159500=CARTESIAN_POINT('Ctrl Pts',(5.55782685636029,-4.27412999301851,
9.01785537482254));
#159501=CARTESIAN_POINT('Ctrl Pts',(5.44054743694793,-4.4266332411586,9.00912280168344));
#159502=CARTESIAN_POINT('Ctrl Pts',(5.31700801196676,-4.5742803085538,9.00039022854433));
#159503=CARTESIAN_POINT('Ctrl Pts',(5.18762953249469,-4.71657994696251,
8.99165765540523));
#159504=CARTESIAN_POINT('Ctrl Pts',(5.05641302519356,-4.86090117888916,
8.9828010221248));
#159505=CARTESIAN_POINT('Ctrl Pts',(4.91919048775539,-4.99972167185865,
8.97394438884436));
#159506=CARTESIAN_POINT('Ctrl Pts',(4.77644072199006,-5.13256666705997,
8.96508775556393));
#159507=CARTESIAN_POINT('Ctrl Pts',(4.63560093874928,-5.26363420491874,
8.95634962345722));
#159508=CARTESIAN_POINT('Ctrl Pts',(4.48938113564619,-5.38888498323262,
8.9476114913505));
#159509=CARTESIAN_POINT('Ctrl Pts',(4.33827621675964,-5.50790214415595,
8.93887335924379));
#159510=CARTESIAN_POINT('Ctrl Pts',(4.18409750990132,-5.6293403613915,8.92995747537649));
#159511=CARTESIAN_POINT('Ctrl Pts',(4.02483304193899,-5.74428844899757,
8.92104159150919));
#159512=CARTESIAN_POINT('Ctrl Pts',(3.86104244633639,-5.85234805783873,
8.91212570764189));
#159513=CARTESIAN_POINT('Ctrl Pts',(3.69725185073379,-5.96040766667988,
8.90320982377459));
#159514=CARTESIAN_POINT('Ctrl Pts',(3.52893538326675,-6.06157863529755,
8.89429393990729));
#159515=CARTESIAN_POINT('Ctrl Pts',(3.35668320892921,-6.15551008425725,
8.88537805604));
#159516=CARTESIAN_POINT('Ctrl Pts',(3.18781583334579,-6.24759575650828,
8.87663737154375));
#159517=CARTESIAN_POINT('Ctrl Pts',(3.01514805500628,-6.33273356531839,
8.86789668704751));
#159518=CARTESIAN_POINT('Ctrl Pts',(2.83925870844214,-6.41063464479419,
8.85915600255126));
#159519=CARTESIAN_POINT('Ctrl Pts',(2.66340100729269,-6.48852170857198,
8.85041689064932));
#159520=CARTESIAN_POINT('Ctrl Pts',(2.48432314570172,-6.55917453238893,
8.84167777874739));
#159521=CARTESIAN_POINT('Ctrl Pts',(2.30262529379728,-6.6223517966705,8.83293866684545));
#159522=CARTESIAN_POINT('Ctrl Pts',(2.11857328471429,-6.6863476133382,8.82408632717113));
#159523=CARTESIAN_POINT('Ctrl Pts',(1.93183318237887,-6.74267269199388,
8.81523398749681));
#159524=CARTESIAN_POINT('Ctrl Pts',(1.7430474591679,-6.79112745555466,8.80638164782249));
#159525=CARTESIAN_POINT('Ctrl Pts',(1.55677196563332,-6.83893793000617,
8.79764701517271));
#159526=CARTESIAN_POINT('Ctrl Pts',(1.36850518904379,-6.87908603184273,
8.78891238252292));
#159527=CARTESIAN_POINT('Ctrl Pts',(1.17887830698919,-6.91143056825505,
8.78017774987315));
#159528=CARTESIAN_POINT('Ctrl Pts',(0.985418335961838,-6.94442891221042,
8.77126655668655));
#159529=CARTESIAN_POINT('Ctrl Pts',(0.790542970508542,-6.96930478037182,
8.76235536349997));
#159530=CARTESIAN_POINT('Ctrl Pts',(0.594933037498019,-6.98596315788978,
8.75344417031337));
#159531=CARTESIAN_POINT('Ctrl Pts',(0.399323104487497,-7.00262153540775,
8.74453297712678));
#159532=CARTESIAN_POINT('Ctrl Pts',(0.202978904812929,-7.01106238313507,
8.73562178394019));
#159533=CARTESIAN_POINT('Ctrl Pts',(0.00658751125854588,-7.01124690530832,
8.72671059075359));
#159534=CARTESIAN_POINT('Ctrl Pts',(-0.170287961144563,-7.01141309103556,
8.71868492590123));
#159535=CARTESIAN_POINT('Ctrl Pts',(-0.347283000348599,-7.00488188201524,
8.71065926104888));
#159536=CARTESIAN_POINT('Ctrl Pts',(-0.523844888054318,-6.99165310178926,
8.70263359619653));
#159537=CARTESIAN_POINT('Ctrl Pts',(-0.700350739347519,-6.97842852005365,
8.69461047849335));
#159538=CARTESIAN_POINT('Ctrl Pts',(-0.876423347724347,-6.95851062642729,
8.68658736079017));
#159539=CARTESIAN_POINT('Ctrl Pts',(-1.05151207543291,-6.93195130664655,
8.67856424308699));
#159540=CARTESIAN_POINT('Ctrl Pts',(-1.22657872291956,-6.90539533622863,
8.67054213716921));
#159541=CARTESIAN_POINT('Ctrl Pts',(-1.40066137465016,-6.87219966348944,
8.66252003125144));
#159542=CARTESIAN_POINT('Ctrl Pts',(-1.57321663076453,-6.83246778222817,
8.65449792533366));
#159543=CARTESIAN_POINT('Ctrl Pts',(-1.74583600899621,-6.79272113646532,
8.64647283837417));
#159544=CARTESIAN_POINT('Ctrl Pts',(-1.91692649952479,-6.74643350945737,
8.63844775141469));
#159545=CARTESIAN_POINT('Ctrl Pts',(-2.08595653833109,-6.69375917423788,
8.6304226644552));
#159546=CARTESIAN_POINT('Ctrl Pts',(-2.2550198667579,-6.64107446507159,
8.62239599699498));
#159547=CARTESIAN_POINT('Ctrl Pts',(-2.42202158770787,-6.58200065935708,
8.61436932953476));
#159548=CARTESIAN_POINT('Ctrl Pts',(-2.5864475293609,-6.51674119022406,
8.60634266207454));
#159549=CARTESIAN_POINT('Ctrl Pts',(-2.75100547158014,-6.45142933101932,
8.59830955083399));
#159550=CARTESIAN_POINT('Ctrl Pts',(-2.91298316731429,-6.37992203423224,
8.59027643959342));
#159551=CARTESIAN_POINT('Ctrl Pts',(-3.07188800419658,-6.30247020240264,
8.58224332835287));
#159552=CARTESIAN_POINT('Ctrl Pts',(-3.16552050662644,-6.25683276949458,
8.57750992739096));
#159553=CARTESIAN_POINT('Ctrl Pts',(-3.25808657030887,-6.20913227422216,
8.57277652642905));
#159554=CARTESIAN_POINT('Ctrl Pts',(-3.34948980370665,-6.15942729621555,
8.56804312546714));
#159555=CARTESIAN_POINT('Ctrl Pts',(-3.53778330915515,-6.0570334946049,
8.55829217217283));
#159556=CARTESIAN_POINT('Ctrl Pts',(-3.72125190656563,-5.94607109475091,
8.54854121887851));
#159557=CARTESIAN_POINT('Ctrl Pts',(-3.89921147911015,-5.82698690608411,
8.5387902655842));
#159558=CARTESIAN_POINT('Ctrl Pts',(-4.07742743580522,-5.70773115430261,
8.52902526421232));
#159559=CARTESIAN_POINT('Ctrl Pts',(-4.250118459623,-5.58033022982944,8.51926026284045));
#159560=CARTESIAN_POINT('Ctrl Pts',(-4.41662906055381,-5.44527449298671,
8.50949526146857));
#159561=CARTESIAN_POINT('Ctrl Pts',(-4.5828621228114,-5.31044386607573,
8.49974653633082));
#159562=CARTESIAN_POINT('Ctrl Pts',(-4.74293532122369,-5.1679839507073,
8.48999781119308));
#159563=CARTESIAN_POINT('Ctrl Pts',(-4.89622824126452,-5.01842361423821,
8.48024908605532));
#159564=CARTESIAN_POINT('Ctrl Pts',(-5.0491004316789,-4.86927376290099,
8.47052711738802));
#159565=CARTESIAN_POINT('Ctrl Pts',(-5.19522946543464,-4.71306242276272,
8.46080514872073));
#159566=CARTESIAN_POINT('Ctrl Pts',(-5.33403220687575,-4.55035459920568,
8.45108318005343));
#159567=CARTESIAN_POINT('Ctrl Pts',(-5.47191652683011,-4.38872337082007,
8.44142553911356));
#159568=CARTESIAN_POINT('Ctrl Pts',(-5.60257113408197,-4.22068136269092,
8.43176789817369));
#159569=CARTESIAN_POINT('Ctrl Pts',(-5.72545688970472,-4.04682220595776,
8.42211025723382));
#159570=CARTESIAN_POINT('Ctrl Pts',(-5.77946940998658,-3.97040512098604,
8.41786539154946));
#159571=CARTESIAN_POINT('Ctrl Pts',(-5.83198149049903,-3.89286473541701,
8.4136205258651));
#159572=CARTESIAN_POINT('Ctrl Pts',(-5.88294940643042,-3.81425390396077,
8.40937566018074));
#159573=CARTESIAN_POINT('Ctrl Pts',(-5.97722618884602,-3.6688452460379,
8.40152381316689));
#159574=CARTESIAN_POINT('Ctrl Pts',(-6.06617771077686,-3.51983172051869,
8.39367196615304));
#159575=CARTESIAN_POINT('Ctrl Pts',(-6.14951162340794,-3.36765992286494,
8.3858201191392));
#159576=CARTESIAN_POINT('Ctrl Pts',(-6.23282190321506,-3.21553127990284,
8.37797049884569));
#159577=CARTESIAN_POINT('Ctrl Pts',(-6.31051755964291,-3.06024648067694,
8.37012087855218));
#159578=CARTESIAN_POINT('Ctrl Pts',(-6.38235100187401,-2.90227880317827,
8.36227125825867));
#159579=CARTESIAN_POINT('Ctrl Pts',(-6.45417870912356,-2.74432373737807,
8.35442226465694));
#159580=CARTESIAN_POINT('Ctrl Pts',(-6.520144976658,-2.5836865672631,8.34657327105521));
#159581=CARTESIAN_POINT('Ctrl Pts',(-6.58004949623077,-2.42086248879468,
8.33872427745347));
#159582=CARTESIAN_POINT('Ctrl Pts',(-6.63998434370778,-2.25795597726288,
8.3308713101361));
#159583=CARTESIAN_POINT('Ctrl Pts',(-6.69385117955146,-2.09286070367149,
8.32301834281873));
#159584=CARTESIAN_POINT('Ctrl Pts',(-6.74149881819546,-1.92608936624686,
8.31516537550136));
#159585=CARTESIAN_POINT('Ctrl Pts',(-6.78915855773862,-1.75927567450637,
8.30731041379416));
#159586=CARTESIAN_POINT('Ctrl Pts',(-6.8305958623034,-1.59078544138089,
8.29945545208697));
#159587=CARTESIAN_POINT('Ctrl Pts',(-6.86571039080206,-1.42114298792651,
8.29160049037977));
#159588=CARTESIAN_POINT('Ctrl Pts',(-6.90085977340539,-1.25133215015704,
8.2837377319665));
#159589=CARTESIAN_POINT('Ctrl Pts',(-6.92967378203492,-1.08036718384407,
8.27587497355323));
#159590=CARTESIAN_POINT('Ctrl Pts',(-6.95210372994142,-0.908779561078822,
8.26801221513996));
#159591=CARTESIAN_POINT('Ctrl Pts',(-6.96855801787632,-0.7829053431442,
8.2622442083914));
#159592=CARTESIAN_POINT('Ctrl Pts',(-6.98157782023741,-0.656696184326862,
8.25647620164285));
#159593=CARTESIAN_POINT('Ctrl Pts',(-6.99116175634591,-0.530362007600873,
8.25070819489429));
#159594=CARTESIAN_POINT('Ctrl Pts',(-7.00508248442126,-0.346860813423779,
8.24233012845327));
#159595=CARTESIAN_POINT('Ctrl Pts',(-7.0117834348992,-0.162689373237821,
8.23395206201226));
#159596=CARTESIAN_POINT('Ctrl Pts',(-7.01121685033776,0.0215601493483096,
8.22557399557124));
#159597=CARTESIAN_POINT('Ctrl Pts',(-7.01065065320011,0.205683684299958,
8.21720165795251));
#159598=CARTESIAN_POINT('Ctrl Pts',(-7.00282682965187,0.389884867529372,
8.20882932033377));
#159599=CARTESIAN_POINT('Ctrl Pts',(-6.98774963364724,0.573569193701026,
8.20045698271505));
#159600=CARTESIAN_POINT('Ctrl Pts',(-6.97268053616941,0.757154856139826,
8.1920891421925));
#159601=CARTESIAN_POINT('Ctrl Pts',(-6.95036586143784,0.940223888185467,
8.18372130166996));
#159602=CARTESIAN_POINT('Ctrl Pts',(-6.92086189661233,1.12218410722998,
8.17535346114742));
#159603=CARTESIAN_POINT('Ctrl Pts',(-6.89136945735466,1.30407324447717,
8.16698888947752));
#159604=CARTESIAN_POINT('Ctrl Pts',(-6.85469338100372,1.48485410849331,
8.15862431780762));
#159605=CARTESIAN_POINT('Ctrl Pts',(-6.81094158624654,1.66394148672285,
8.15025974613773));
#159606=CARTESIAN_POINT('Ctrl Pts',(-6.76720047869017,1.84298511948361,
8.14189721767218));
#159607=CARTESIAN_POINT('Ctrl Pts',(-6.71638717788505,2.02033577249617,
8.13353468920663));
#159608=CARTESIAN_POINT('Ctrl Pts',(-6.65866041230502,2.19541979495995,
8.12517216074108));
#159609=CARTESIAN_POINT('Ctrl Pts',(-6.60092903994836,2.37051778967687,
8.11680896491957));
#159610=CARTESIAN_POINT('Ctrl Pts',(-6.53628319774413,2.54334847843099,
8.10844576909806));
#159611=CARTESIAN_POINT('Ctrl Pts',(-6.46493130449214,2.71335397445626,
8.10008257327656));
#159612=CARTESIAN_POINT('Ctrl Pts',(-6.39357454518413,2.88337106451541,
8.09171880710187));
#159613=CARTESIAN_POINT('Ctrl Pts',(-6.31551094993941,3.05056227436935,
8.08335504092719));
#159614=CARTESIAN_POINT('Ctrl Pts',(-6.23099692415811,3.21439012778974,
8.0749912747525));
#159615=CARTESIAN_POINT('Ctrl Pts',(-6.14646586698207,3.3782509960478,8.06662582309896));
#159616=CARTESIAN_POINT('Ctrl Pts',(-6.05548193798342,3.53874686415457,
8.05826037144542));
#159617=CARTESIAN_POINT('Ctrl Pts',(-5.95834749445622,3.69536489372934,
8.04989491979188));
#159618=CARTESIAN_POINT('Ctrl Pts',(-5.8611805207953,3.85203537437359,8.04152666656507));
#159619=CARTESIAN_POINT('Ctrl Pts',(-5.7578590985367,4.00482514758256,8.03315841333824));
#159620=CARTESIAN_POINT('Ctrl Pts',(-5.64872912316993,4.15325003527983,
8.02479016011143));
#159621=CARTESIAN_POINT('Ctrl Pts',(-5.53949796874631,4.30181253402392,
8.01641414831997));
#159622=CARTESIAN_POINT('Ctrl Pts',(-5.4244476946266,4.44600179523599,8.0080381365285));
#159623=CARTESIAN_POINT('Ctrl Pts',(-5.30396550340238,4.585365470845,7.99966212473704));
#159624=CARTESIAN_POINT('Ctrl Pts',(-5.18342422622279,4.72479749212263,
7.99128200524589));
#159625=CARTESIAN_POINT('Ctrl Pts',(-5.05744593948409,4.85939896419983,
7.98290188575475));
#159626=CARTESIAN_POINT('Ctrl Pts',(-4.9264554283491,4.98875369957164,7.97452176626361));
#159627=CARTESIAN_POINT('Ctrl Pts',(-4.79531524396207,5.11825623911446,
7.9661320714244));
#159628=CARTESIAN_POINT('Ctrl Pts',(-4.65915162980593,5.24249983616411,
7.95774237658519));
#159629=CARTESIAN_POINT('Ctrl Pts',(-4.51842422648261,5.36110707522569,
7.94935268174598));
#159630=CARTESIAN_POINT('Ctrl Pts',(-4.42907882660513,5.43640876453474,
7.94402620927113));
#159631=CARTESIAN_POINT('Ctrl Pts',(-4.33789453138378,5.50943939103424,
7.93869973679628));
#159632=CARTESIAN_POINT('Ctrl Pts',(-4.24499520190079,5.58011131594516,
7.93337326432143));
#159633=CARTESIAN_POINT('Ctrl Pts',(-4.09881643320985,5.69131486307507,
7.92499196391622));
#159634=CARTESIAN_POINT('Ctrl Pts',(-3.94809497438731,5.79690056691332,
7.916610663511));
#159635=CARTESIAN_POINT('Ctrl Pts',(-3.79328726983628,5.89649033332524,
7.90822936310578));
#159636=CARTESIAN_POINT('Ctrl Pts',(-3.63867576138863,5.99595388428708,
7.8998586847719));
#159637=CARTESIAN_POINT('Ctrl Pts',(-3.47998860118254,6.08943646595476,
7.89148800643802));
#159638=CARTESIAN_POINT('Ctrl Pts',(-3.31771432034658,6.17660086544916,
7.88311732810414));
#159639=CARTESIAN_POINT('Ctrl Pts',(-3.15562419295871,6.26366634831526,
7.87475614905302));
#159640=CARTESIAN_POINT('Ctrl Pts',(-2.98995534531653,6.34442778560906,
7.86639497000189));
#159641=CARTESIAN_POINT('Ctrl Pts',(-2.82122461662683,6.41859160759109,
7.85803379095077));
#159642=CARTESIAN_POINT('Ctrl Pts',(-2.65271283596032,6.49265919326608,
7.84968346151571));
#159643=CARTESIAN_POINT('Ctrl Pts',(-2.48114739765742,6.56014610859907,
7.84133313208065));
#159644=CARTESIAN_POINT('Ctrl Pts',(-2.30706894932868,6.62080504361391,
7.8329828026456));
#159645=CARTESIAN_POINT('Ctrl Pts',(-2.13312444395439,6.68141730520625,
7.82463889828961));
#159646=CARTESIAN_POINT('Ctrl Pts',(-1.95667108997936,6.73521194883618,
7.81629499393363));
#159647=CARTESIAN_POINT('Ctrl Pts',(-1.77826975363068,6.78198962295154,
7.80795108957764));
#159648=CARTESIAN_POINT('Ctrl Pts',(-1.60001171034735,6.82872972494747,
7.79961388709764));
#159649=CARTESIAN_POINT('Ctrl Pts',(-1.41980912114422,6.8684640149127,7.79127668461763));
#159650=CARTESIAN_POINT('Ctrl Pts',(-1.23823841130986,6.90104283418505,
7.78293948213764));
#159651=CARTESIAN_POINT('Ctrl Pts',(-1.17846633592108,6.91176760165113,
7.78019492110342));
#159652=CARTESIAN_POINT('Ctrl Pts',(-1.11854611485407,6.92171734123032,
7.7774503600692));
#159653=CARTESIAN_POINT('Ctrl Pts',(-1.0584986244211,6.93088791026075,7.77470579903499));
#159654=CARTESIAN_POINT('Ctrl Pts',(-0.876067043632634,6.95874921458652,
7.76636748873373));
#159655=CARTESIAN_POINT('Ctrl Pts',(-0.692609763917193,6.97939196714889,
7.75802917843247));
#159656=CARTESIAN_POINT('Ctrl Pts',(-0.508721244209177,6.99276978444095,
7.74969086813121));
#159657=CARTESIAN_POINT('Ctrl Pts',(-0.324717028084998,7.00615601860165,
7.74134731164808));
#159658=CARTESIAN_POINT('Ctrl Pts',(-0.140281357570403,7.01226817658823,
7.73300375516494));
#159659=CARTESIAN_POINT('Ctrl Pts',(0.0439900195438079,7.01111199744239,
7.7246601986818));
#159660=CARTESIAN_POINT('Ctrl Pts',(0.228401589516582,7.0099549386805,7.71631029445735));
#159661=CARTESIAN_POINT('Ctrl Pts',(0.41264828949352,7.0015185148547,7.7079603902329));
#159662=CARTESIAN_POINT('Ctrl Pts',(0.596137764416577,6.98586045726197,
7.69961048600845));
#159663=CARTESIAN_POINT('Ctrl Pts',(0.779902459975568,6.97017891374139,
7.69124805754548));
#159664=CARTESIAN_POINT('Ctrl Pts',(0.962907334084302,6.94725411876133,
7.6828856290825));
#159665=CARTESIAN_POINT('Ctrl Pts',(1.14456701236412,6.9171954516775,7.67452320061952));
#159666=CARTESIAN_POINT('Ctrl Pts',(1.32638203443264,6.88711108033573,7.66615362114024));
#159667=CARTESIAN_POINT('Ctrl Pts',(1.50684924534435,6.84988073099078,7.65778404166098));
#159668=CARTESIAN_POINT('Ctrl Pts',(1.68539621165002,6.80566427119762,7.6494144621817));
#159669=CARTESIAN_POINT('Ctrl Pts',(1.86421856489746,6.76137961290245,7.64103197364581));
#159670=CARTESIAN_POINT('Ctrl Pts',(2.04111444101417,6.71008740311691,7.63264948510993));
#159671=CARTESIAN_POINT('Ctrl Pts',(2.21552788564968,6.65199689945874,7.62426699657404));
#159672=CARTESIAN_POINT('Ctrl Pts',(2.27259882275809,6.63298873476249,7.62152410896555));
#159673=CARTESIAN_POINT('Ctrl Pts',(2.32940413615168,6.61325305163047,7.61878122135707));
#159674=CARTESIAN_POINT('Ctrl Pts',(2.38592487487982,6.59279827189713,7.61603833374858));
#159675=CARTESIAN_POINT('Ctrl Pts',(2.5588208641615,6.53022744467304,7.60764788668033));
#159676=CARTESIAN_POINT('Ctrl Pts',(2.7294014515115,6.46079789610722,7.59925743961206));
#159677=CARTESIAN_POINT('Ctrl Pts',(2.89710496355616,6.38470119838339,7.5908669925438));
#159678=CARTESIAN_POINT('Ctrl Pts',(3.06465158322805,6.30867569172359,7.58248439502582));
#159679=CARTESIAN_POINT('Ctrl Pts',(3.22932619550739,6.22599560575943,7.57410179750785));
#159680=CARTESIAN_POINT('Ctrl Pts',(3.39058555648328,6.13690118436552,7.56571919998986));
#159681=CARTESIAN_POINT('Ctrl Pts',(3.55171776280078,6.04787701483576,7.55734321223591));
#159682=CARTESIAN_POINT('Ctrl Pts',(3.70943980023771,5.95244875244961,7.54896722448196));
#159683=CARTESIAN_POINT('Ctrl Pts',(3.86323114988645,5.85090348963705,7.54059123672801));
#159684=CARTESIAN_POINT('Ctrl Pts',(4.01690928358334,5.74943298098728,7.53222141509086));
#159685=CARTESIAN_POINT('Ctrl Pts',(4.16666222802708,5.64185463528875,7.52385159345374));
#159686=CARTESIAN_POINT('Ctrl Pts',(4.3119964399461,5.52850009174208,7.5154817718166));
#159687=CARTESIAN_POINT('Ctrl Pts',(4.45726703110845,5.41519516969702,7.5071156141095));
#159688=CARTESIAN_POINT('Ctrl Pts',(4.59812248720092,5.29611929235213,7.4987494564024));
#159689=CARTESIAN_POINT('Ctrl Pts',(4.73409990577678,5.17164622191274,7.49038329869531));
#159690=CARTESIAN_POINT('Ctrl Pts',(4.8700359395881,5.04721103488638,7.4820196872306));
#159691=CARTESIAN_POINT('Ctrl Pts',(5.00109665387081,4.91738215166125,7.47365607576589));
#159692=CARTESIAN_POINT('Ctrl Pts',(5.12685346072713,4.782572545684,7.46529246430118));
#159693=CARTESIAN_POINT('Ctrl Pts',(5.25258876091069,4.64778599457074,7.45693028316425));
#159694=CARTESIAN_POINT('Ctrl Pts',(5.37302173875201,4.50802065980671,7.44856810202733));
#159695=CARTESIAN_POINT('Ctrl Pts',(5.48776151230319,4.36372548937073,7.44020592089041));
#159696=CARTESIAN_POINT('Ctrl Pts',(5.60258692083858,4.21932262554947,7.43183749871581));
#159697=CARTESIAN_POINT('Ctrl Pts',(5.71171041313554,4.0703834153163,7.4234690765412));
#159698=CARTESIAN_POINT('Ctrl Pts',(5.81478108593368,3.91739039223408,7.4151006543666));
#159699=CARTESIAN_POINT('Ctrl Pts',(5.91780065474847,3.76447322538423,7.40673638138106));
#159700=CARTESIAN_POINT('Ctrl Pts',(6.01477323009914,3.60750654362712,7.39837210839551));
#159701=CARTESIAN_POINT('Ctrl Pts',(6.105392107819,3.44700069223688,7.39000783540997));
#159702=CARTESIAN_POINT('Ctrl Pts',(6.19607841426631,3.2863754098232,7.38163733864084));
#159703=CARTESIAN_POINT('Ctrl Pts',(6.28040140896109,3.1222059794816,7.37326684187171));
#159704=CARTESIAN_POINT('Ctrl Pts',(6.35809994547922,2.95502819712388,7.36489634510259));
#159705=CARTESIAN_POINT('Ctrl Pts',(6.43579848199734,2.78785041476615,7.35652584833346));
#159706=CARTESIAN_POINT('Ctrl Pts',(6.50687244152518,2.61766458747699,7.34815535156433));
#159707=CARTESIAN_POINT('Ctrl Pts',(6.57110895151815,2.44502632087633,7.33978485479521));
#159708=CARTESIAN_POINT('Origin',(0.,0.,50.));
#159709=CARTESIAN_POINT('',(6.57110895151814,2.44502632087637,5.33975062352345));
#159710=CARTESIAN_POINT('',(6.57110895151814,2.44502632087637,5.88692100032223));
#159711=CARTESIAN_POINT('',(6.57110895151814,2.44502632087636,50.));
#159712=CARTESIAN_POINT('',(7.01125,3.55178126493216E-12,7.77353435691053));
#159713=CARTESIAN_POINT('Ctrl Pts',(6.57110895151814,2.44502632087637,5.88692100032223));
#159714=CARTESIAN_POINT('Ctrl Pts',(6.5044983873315,2.62404495591324,5.895592809261));
#159715=CARTESIAN_POINT('Ctrl Pts',(6.43056821795877,2.80033990715955,5.90426461819976));
#159716=CARTESIAN_POINT('Ctrl Pts',(6.34956511459265,2.97332295892123,5.91293642713853));
#159717=CARTESIAN_POINT('Ctrl Pts',(6.26856213015506,3.14630575670966,5.92160822334536));
#159718=CARTESIAN_POINT('Ctrl Pts',(6.18048635294248,3.3159764075473,5.9302800195522));
#159719=CARTESIAN_POINT('Ctrl Pts',(6.08563165071504,3.48176879966423,5.93895181575904));
#159720=CARTESIAN_POINT('Ctrl Pts',(5.99077708581898,3.64756095174566,5.94762359941078));
#159721=CARTESIAN_POINT('Ctrl Pts',(5.88914375658023,3.80947460983867,5.95629538306252));
#159722=CARTESIAN_POINT('Ctrl Pts',(5.78107076500129,3.96696954520039,5.96496716671427));
#159723=CARTESIAN_POINT('Ctrl Pts',(5.6729979276878,4.12446425575084,5.97363893798774));
#159724=CARTESIAN_POINT('Ctrl Pts',(5.55848560711296,4.27754002202603,5.98231070926122));
#159725=CARTESIAN_POINT('Ctrl Pts',(5.43791587524826,4.4256861045744,5.99098248053469));
#159726=CARTESIAN_POINT('Ctrl Pts',(5.31734631302827,4.57383197867744,5.99965423960676));
#159727=CARTESIAN_POINT('Ctrl Pts',(5.19071953583751,4.7170479626693,6.00832599867883));
#159728=CARTESIAN_POINT('Ctrl Pts',(5.05845803451497,4.85485621574429,6.0169977577509));
#159729=CARTESIAN_POINT('Ctrl Pts',(4.92619671659114,4.99266427772924,6.02566950479839));
#159730=CARTESIAN_POINT('Ctrl Pts',(4.78830088681692,5.12506441890981,6.03434125184587));
#159731=CARTESIAN_POINT('Ctrl Pts',(4.64523063400368,5.25161488681471,6.04301299889335));
#159732=CARTESIAN_POINT('Ctrl Pts',(4.49652806262298,5.38314733060966,6.05202613096636));
#159733=CARTESIAN_POINT('Ctrl Pts',(4.34223563523867,5.50835996364338,6.06103926303936));
#159734=CARTESIAN_POINT('Ctrl Pts',(4.18290943344465,5.62680151010321,6.07005239511237));
#159735=CARTESIAN_POINT('Ctrl Pts',(4.02607270355366,5.7433924073996,6.07892469699674));
#159736=CARTESIAN_POINT('Ctrl Pts',(3.86435862820312,5.85342208902684,6.0877969988811));
#159737=CARTESIAN_POINT('Ctrl Pts',(3.69833198496378,5.9565062823348,6.09666930076547));
#159738=CARTESIAN_POINT('Ctrl Pts',(3.53489950802504,6.05797978512232,6.10540297293289));
#159739=CARTESIAN_POINT('Ctrl Pts',(3.36728850947003,6.15272311279952,6.11413664510032));
#159740=CARTESIAN_POINT('Ctrl Pts',(3.19606623000888,6.24041562845752,6.12287031726774));
#159741=CARTESIAN_POINT('Ctrl Pts',(3.02603797481024,6.32749661743998,6.13154308488173));
#159742=CARTESIAN_POINT('Ctrl Pts',(2.85244891335276,6.40762471321634,6.14021585249571));
#159743=CARTESIAN_POINT('Ctrl Pts',(2.6758783609508,6.48053250588987,6.1488886201097));
#159744=CARTESIAN_POINT('Ctrl Pts',(2.49930871513386,6.55343992422515,6.15756134319417));
#159745=CARTESIAN_POINT('Ctrl Pts',(2.3197578716491,6.61912700519444,6.16623406627865));
#159746=CARTESIAN_POINT('Ctrl Pts',(2.13782503580022,6.67737453486068,6.17490678936312));
#159747=CARTESIAN_POINT('Ctrl Pts',(1.95589311921758,6.73562177021507,6.18357946862625));
#159748=CARTESIAN_POINT('Ctrl Pts',(1.77157950496959,6.78642944284913,6.19225214788937));
#159749=CARTESIAN_POINT('Ctrl Pts',(1.58549928668711,6.82962799678099,6.2009248271525));
#159750=CARTESIAN_POINT('Ctrl Pts',(1.39941999343791,6.87282633596621,6.20959746330241));
#159751=CARTESIAN_POINT('Ctrl Pts',(1.21157439050561,6.90841556788932,6.21827009945232));
#159752=CARTESIAN_POINT('Ctrl Pts',(1.02258935229021,6.93627692491316,6.22694273560223));
#159753=CARTESIAN_POINT('Ctrl Pts',(0.833605238123156,6.96413814570801,
6.23561532934701));
#159754=CARTESIAN_POINT('Ctrl Pts',(0.643481980914484,6.98427152577633,
6.24428792309178));
#159755=CARTESIAN_POINT('Ctrl Pts',(0.452854049805853,6.9966098770815,6.25296051683656));
#159756=CARTESIAN_POINT('Ctrl Pts',(0.262227035219643,7.00894816906496,
6.26163306888427));
#159757=CARTESIAN_POINT('Ctrl Pts',(0.0710956351198641,7.01349148893089,
6.27030562093198));
#159758=CARTESIAN_POINT('Ctrl Pts',(-0.119902323158553,7.01022467510145,
6.27897817297969));
#159759=CARTESIAN_POINT('Ctrl Pts',(-0.310899378724106,7.00695787671193,
6.28765068403835));
#159760=CARTESIAN_POINT('Ctrl Pts',(-0.501762709654535,6.99588102335271,
6.29632319509701));
#159761=CARTESIAN_POINT('Ctrl Pts',(-0.69185538920701,6.97703107940084,
6.30499570615567));
#159762=CARTESIAN_POINT('Ctrl Pts',(-0.881947185839014,6.958181223001,6.31366817693325));
#159763=CARTESIAN_POINT('Ctrl Pts',(-1.07126805553177,6.93155837629103,
6.32234064771084));
#159764=CARTESIAN_POINT('Ctrl Pts',(-1.25918622472626,6.89725138109085,
6.33101311848842));
#159765=CARTESIAN_POINT('Ctrl Pts',(-1.44710353643658,6.86294454243597,
6.33968554969289));
#159766=CARTESIAN_POINT('Ctrl Pts',(-1.6336178809721,6.82095367648008,6.34835798089736));
#159767=CARTESIAN_POINT('Ctrl Pts',(-1.81810685596831,6.7714189076427,6.35703041210184));
#159768=CARTESIAN_POINT('Ctrl Pts',(-2.00259500418343,6.7218843607937,6.3657028044411));
#159769=CARTESIAN_POINT('Ctrl Pts',(-2.18505752664271,6.66480605238633,
6.37437519678037));
#159770=CARTESIAN_POINT('Ctrl Pts',(-2.36488554745062,6.60037445225339,
6.38304758911964));
#159771=CARTESIAN_POINT('Ctrl Pts',(-2.54471277704031,6.5359431356105,6.39171994330159));
#159772=CARTESIAN_POINT('Ctrl Pts',(-2.7219052607312,6.4641586878085,6.40039229748355));
#159773=CARTESIAN_POINT('Ctrl Pts',(-2.89587171390055,6.38526065083726,
6.4090646516655));
#159774=CARTESIAN_POINT('Ctrl Pts',(-3.06983741583796,6.30636295456807,
6.41773696839799));
#159775=CARTESIAN_POINT('Ctrl Pts',(-3.24057685640968,6.22035184793667,
6.42640928513048));
#159776=CARTESIAN_POINT('Ctrl Pts',(-3.40752028946975,6.12751434427958,
6.43508160186297));
#159777=CARTESIAN_POINT('Ctrl Pts',(-3.57446301524744,6.03467723394333,
6.44375388185381));
#159778=CARTESIAN_POINT('Ctrl Pts',(-3.73760951742361,5.93501392252033,
6.45242616184466));
#159779=CARTESIAN_POINT('Ctrl Pts',(-3.89641539159055,5.82885697703043,
6.4610984418355));
#159780=CARTESIAN_POINT('Ctrl Pts',(-4.05522060590922,5.72270047262923,
6.46977068579249));
#159781=CARTESIAN_POINT('Ctrl Pts',(-4.20968499214316,5.61005054602417,
6.47844292974947));
#159782=CARTESIAN_POINT('Ctrl Pts',(-4.3592931215613,5.49128309621789,6.48711517370645));
#159783=CARTESIAN_POINT('Ctrl Pts',(-4.50890064155567,5.37251613020689,
6.49578738233733));
#159784=CARTESIAN_POINT('Ctrl Pts',(-4.65365172183509,5.24763186748229,
6.50445959096822));
#159785=CARTESIAN_POINT('Ctrl Pts',(-4.7930633497115,5.1170470281357,6.5131317995991));
#159786=CARTESIAN_POINT('Ctrl Pts',(-4.93247442107403,4.98646271006755,
6.52180397361161));
#159787=CARTESIAN_POINT('Ctrl Pts',(-5.06654587536807,4.85017805510629,
6.53047614762413));
#159788=CARTESIAN_POINT('Ctrl Pts',(-5.19483033978703,4.70864782111894,
6.53914832163663));
#159789=CARTESIAN_POINT('Ctrl Pts',(-5.32311430257712,4.56711814055521,
6.54782046173846));
#159790=CARTESIAN_POINT('Ctrl Pts',(-5.44561113000693,4.42034313247674,
6.55649260184028));
#159791=CARTESIAN_POINT('Ctrl Pts',(-5.56191207495262,4.26881255538308,
6.56516474194211));
#159792=CARTESIAN_POINT('Ctrl Pts',(-5.67821257461712,4.11728255845425,
6.57383684884094));
#159793=CARTESIAN_POINT('Ctrl Pts',(-5.78831706632323,3.96099725427861,
6.58250895573975));
#159794=CARTESIAN_POINT('Ctrl Pts',(-5.89185815647412,3.80047813129998,
6.59118106263858));
#159795=CARTESIAN_POINT('Ctrl Pts',(-5.99539885864469,3.63995960980488,
6.59985313704202));
#159796=CARTESIAN_POINT('Ctrl Pts',(-6.09237605450686,3.47520753994929,
6.60852521144547));
#159797=CARTESIAN_POINT('Ctrl Pts',(-6.18246615568102,3.30677165772885,
6.61719728584892));
#159798=CARTESIAN_POINT('Ctrl Pts',(-6.27255592662724,3.13833639291513,
6.62586932846462));
#159799=CARTESIAN_POINT('Ctrl Pts',(-6.35575851943897,2.96621759322222,
6.63454137108032));
#159800=CARTESIAN_POINT('Ctrl Pts',(-6.43179631013701,2.79098957135421,
6.64321341369602));
#159801=CARTESIAN_POINT('Ctrl Pts',(-6.50783382831931,2.6157621774949,6.65188542523155));
#159802=CARTESIAN_POINT('Ctrl Pts',(-6.57670648270626,2.43742584432008,
6.66055743676707));
#159803=CARTESIAN_POINT('Ctrl Pts',(-6.63818446599492,2.25657562645787,
6.66922944830259));
#159804=CARTESIAN_POINT('Ctrl Pts',(-6.6996622339648,2.07572604200044,6.6779014294655));
#159805=CARTESIAN_POINT('Ctrl Pts',(-6.75374529124758,1.89236285939144,
6.68657341062841));
#159806=CARTESIAN_POINT('Ctrl Pts',(-6.80025318023397,1.70709790206002,
6.69524539179132));
#159807=CARTESIAN_POINT('Ctrl Pts',(-6.84676091012636,1.52183357848227,
6.70391734328915));
#159808=CARTESIAN_POINT('Ctrl Pts',(-6.88569345442288,1.3346677686782,6.71258929478698));
#159809=CARTESIAN_POINT('Ctrl Pts',(-6.91692090874678,1.14622497994137,
6.72126124628481));
#159810=CARTESIAN_POINT('Ctrl Pts',(-6.9481482587953,0.957782820456753,
6.72993316882507));
#159811=CARTESIAN_POINT('Ctrl Pts',(-6.97167052392502,0.768063970771554,
6.73860509136533));
#159812=CARTESIAN_POINT('Ctrl Pts',(-6.9874092190315,0.57770145256321,6.7472770139056));
#159813=CARTESIAN_POINT('Ctrl Pts',(-7.00314786286682,0.387339554489333,
6.75594890819577));
#159814=CARTESIAN_POINT('Ctrl Pts',(-7.01110296401743,0.196334275138324,
6.76462080248594));
#159815=CARTESIAN_POINT('Ctrl Pts',(-7.01124797942392,0.00532292437979963,
6.77329269677612));
#159816=CARTESIAN_POINT('Ctrl Pts',(-7.01139299436984,-0.185687819711539,
6.78196456352367));
#159817=CARTESIAN_POINT('Ctrl Pts',(-7.0037279729944,-0.376704351160677,
6.79063643027122));
#159818=CARTESIAN_POINT('Ctrl Pts',(-6.98827849031204,-0.567089326598627,
6.79930829701877));
#159819=CARTESIAN_POINT('Ctrl Pts',(-6.97282905543828,-0.757473712888125,
6.80798013693113));
#159820=CARTESIAN_POINT('Ctrl Pts',(-6.94959523043374,-0.947226264001047,
6.81665197684349));
#159821=CARTESIAN_POINT('Ctrl Pts',(-6.91865453650896,-1.13571385786388,
6.82532381675585));
#159822=CARTESIAN_POINT('Ctrl Pts',(-6.88771393580682,-1.3242008838237,
6.83399563054043));
#159823=CARTESIAN_POINT('Ctrl Pts',(-6.84906655865494,-1.51142267990842,
6.842667444325));
#159824=CARTESIAN_POINT('Ctrl Pts',(-6.80284135383486,-1.69675457183835,
6.85133925810957));
#159825=CARTESIAN_POINT('Ctrl Pts',(-6.75661628451852,-1.88208592048964,
6.86001104647374));
#159826=CARTESIAN_POINT('Ctrl Pts',(-6.70281350071451,-2.06552710051589,
6.86868283483791));
#159827=CARTESIAN_POINT('Ctrl Pts',(-6.64161251687612,-2.2464660554245,
6.87735462320208));
#159828=CARTESIAN_POINT('Ctrl Pts',(-6.58041170744941,-2.42740449468997,
6.88602638685323));
#159829=CARTESIAN_POINT('Ctrl Pts',(-6.51181283117298,-2.60584045408564,
6.89469815050438));
#159830=CARTESIAN_POINT('Ctrl Pts',(-6.43604476876237,-2.78117858056374,
6.90336991415553));
#159831=CARTESIAN_POINT('Ctrl Pts',(-6.35684774728261,-2.96445180845298,
6.91243412710089));
#159832=CARTESIAN_POINT('Ctrl Pts',(-6.26981768815679,-3.14433998862217,
6.92149834004625));
#159833=CARTESIAN_POINT('Ctrl Pts',(-6.17527181578122,-3.3201874290043,
6.93056255299162));
#159834=CARTESIAN_POINT('Ctrl Pts',(-6.08368050191737,-3.4905396368745,
6.93934350928244));
#159835=CARTESIAN_POINT('Ctrl Pts',(-5.98503618716623,-3.65709956718604,
6.94812446557326));
#159836=CARTESIAN_POINT('Ctrl Pts',(-5.87967633130112,-3.819297422516,6.95690542186409));
#159837=CARTESIAN_POINT('Ctrl Pts',(-5.77561495477707,-3.97949631379482,
6.96557815960957));
#159838=CARTESIAN_POINT('Ctrl Pts',(-5.66500279405234,-4.13543980257606,
6.97425089735506));
#159839=CARTESIAN_POINT('Ctrl Pts',(-5.54820899034585,-4.2866074653443,
6.98292363510055));
#159840=CARTESIAN_POINT('Ctrl Pts',(-5.4314163636836,-4.43777360464965,
6.99159628544246));
#159841=CARTESIAN_POINT('Ctrl Pts',(-5.30844239242685,-4.58416378940594,
7.00026893578438));
#159842=CARTESIAN_POINT('Ctrl Pts',(-5.17969746407092,-4.72528948776657,
7.00894158612629));
#159843=CARTESIAN_POINT('Ctrl Pts',(-5.05095379116799,-4.86641380994343,
7.01761415189707));
#159844=CARTESIAN_POINT('Ctrl Pts',(-4.91643946526928,-5.00227353854876,
7.02628671766785));
#159845=CARTESIAN_POINT('Ctrl Pts',(-4.77660337747906,-5.13241529270145,
7.03495928343862));
#159846=CARTESIAN_POINT('Ctrl Pts',(-4.63676860764499,-5.26255582026714,
7.0436317674704));
#159847=CARTESIAN_POINT('Ctrl Pts',(-4.49161238426941,-5.38697828766251,
7.05230425150218));
#159848=CARTESIAN_POINT('Ctrl Pts',(-4.34161910267562,-5.50526748939433,
7.06097673553396));
#159849=CARTESIAN_POINT('Ctrl Pts',(-4.19162718580484,-5.62355561486465,
7.06964914065862));
#159850=CARTESIAN_POINT('Ctrl Pts',(-4.03679852186307,-5.73571041041457,
7.07832154578328));
#159851=CARTESIAN_POINT('Ctrl Pts',(-3.87764977431538,-5.84135761533669,
7.08699395090793));
#159852=CARTESIAN_POINT('Ctrl Pts',(-3.7185024228424,-5.94700389350699,
7.09566627995706));
#159853=CARTESIAN_POINT('Ctrl Pts',(-3.55503530028438,-6.04614253816465,
7.10433860900618));
#159854=CARTESIAN_POINT('Ctrl Pts',(-3.38779388709407,-6.13844272931401,
7.1130109380553));
#159855=CARTESIAN_POINT('Ctrl Pts',(-3.22055388638018,-6.23074214092055,
7.12168319386025));
#159856=CARTESIAN_POINT('Ctrl Pts',(-3.04953990753581,-6.31620307732962,
7.1303554496652));
#159857=CARTESIAN_POINT('Ctrl Pts',(-2.87532260481251,-6.39454036508913,
7.13902770547014));
#159858=CARTESIAN_POINT('Ctrl Pts',(-2.70110671662093,-6.47287701680057,
7.14769989086198));
#159859=CARTESIAN_POINT('Ctrl Pts',(-2.52368781567603,-6.54409001910946,
7.15637207625383));
#159860=CARTESIAN_POINT('Ctrl Pts',(-2.34365791912392,-6.60794174615877,
7.16504426164567));
#159861=CARTESIAN_POINT('Ctrl Pts',(-2.16362942554292,-6.67179297561222,
7.17371637945526));
#159862=CARTESIAN_POINT('Ctrl Pts',(-1.98099024478671,-6.72828294965095,
7.18238849726485));
#159863=CARTESIAN_POINT('Ctrl Pts',(-1.79634980371134,-6.77722317363138,
7.19106061507444));
#159864=CARTESIAN_POINT('Ctrl Pts',(-1.61171074128092,-6.82616303219246,
7.19973266813239));
#159865=CARTESIAN_POINT('Ctrl Pts',(-1.42507072299576,-6.8675531807254,
7.20840472119034));
#159866=CARTESIAN_POINT('Ctrl Pts',(-1.2370525163378,-6.90125551145024,
7.21707677424829));
#159867=CARTESIAN_POINT('Ctrl Pts',(-1.04903565219027,-6.93495760152961,
7.225748765385));
#159868=CARTESIAN_POINT('Ctrl Pts',(-0.859640898939492,-6.96097193353415,
7.2344207565217));
#159869=CARTESIAN_POINT('Ctrl Pts',(-0.669500206860438,-6.97921170588154,
7.24309274765841));
#159870=CARTESIAN_POINT('Ctrl Pts',(-0.479360810402781,-6.99745135394286,
7.25176467970404));
#159871=CARTESIAN_POINT('Ctrl Pts',(-0.288475768013728,-7.00791652123622,
7.26043661174968));
#159872=CARTESIAN_POINT('Ctrl Pts',(-0.0974819939195787,-7.01057228929005,
7.26910854379531));
#159873=CARTESIAN_POINT('Ctrl Pts',(0.0935105410598241,-7.01322804011398,
7.27778041957985));
#159874=CARTESIAN_POINT('Ctrl Pts',(0.284611522346058,-7.00807448913595,
7.28645229536439));
#159875=CARTESIAN_POINT('Ctrl Pts',(0.475183323468245,-6.99512883166548,
7.29512417114893));
#159876=CARTESIAN_POINT('Ctrl Pts',(0.665753950392636,-6.98218325395897,
7.30379599350217));
#159877=CARTESIAN_POINT('Ctrl Pts',(0.855795120325422,-6.96144568508264,
7.31246781585542));
#159878=CARTESIAN_POINT('Ctrl Pts',(1.04467275076238,-6.93298531704161,
7.32113963820866));
#159879=CARTESIAN_POINT('Ctrl Pts',(1.23354927906265,-6.90452511507221,
7.32981140996019));
#159880=CARTESIAN_POINT('Ctrl Pts',(1.42126200062692,-6.86834224643129,
7.3384831817117));
#159881=CARTESIAN_POINT('Ctrl Pts',(1.60718460924519,-6.82455743578332,
7.34715495346322));
#159882=CARTESIAN_POINT('Ctrl Pts',(1.79763389405661,-6.77970659200761,
7.35603785770171));
#159883=CARTESIAN_POINT('Ctrl Pts',(1.98620448431676,-6.72687898190926,
7.3649207619402));
#159884=CARTESIAN_POINT('Ctrl Pts',(2.17223623427651,-6.66625954377687,
7.37380366617869));
#159885=CARTESIAN_POINT('Ctrl Pts',(2.35386532185837,-6.60707473666683,
7.38247634593503));
#159886=CARTESIAN_POINT('Ctrl Pts',(2.53307410227486,-6.54046283696597,
7.39114902569138));
#159887=CARTESIAN_POINT('Ctrl Pts',(2.70926451774061,-6.46664614273982,
7.39982170544772));
#159888=CARTESIAN_POINT('Ctrl Pts',(2.88545151535976,-6.39283088045386,
7.40849421696626));
#159889=CARTESIAN_POINT('Ctrl Pts',(3.05862000314199,-6.31181121311119,
7.4171667284848));
#159890=CARTESIAN_POINT('Ctrl Pts',(3.22819210344032,-6.22385751008051,
7.42583924000333));
#159891=CARTESIAN_POINT('Ctrl Pts',(3.39776113570901,-6.13590539837628,
7.43451159461208));
#159892=CARTESIAN_POINT('Ctrl Pts',(3.56373365851006,-6.04101963284017,
7.44318394922084));
#159893=CARTESIAN_POINT('Ctrl Pts',(3.7255558277518,-5.93951684371756,7.45185630382959));
#159894=CARTESIAN_POINT('Ctrl Pts',(3.88737528046406,-5.83801575853528,
7.46052851285441));
#159895=CARTESIAN_POINT('Ctrl Pts',(4.04504427838839,-5.72989802299715,
7.46920072187921));
#159896=CARTESIAN_POINT('Ctrl Pts',(4.19803670363139,-5.61552440983598,
7.47787293090403));
#159897=CARTESIAN_POINT('Ctrl Pts',(4.35102676029996,-5.5011525673665,7.48654500566879));
#159898=CARTESIAN_POINT('Ctrl Pts',(4.49934016166387,-5.38052521115996,
7.49521708043356));
#159899=CARTESIAN_POINT('Ctrl Pts',(4.64248202336615,-5.25404484423402,
7.50388915519832));
#159900=CARTESIAN_POINT('Ctrl Pts',(4.78562185584448,-5.12756627033347,
7.51256110702502));
#159901=CARTESIAN_POINT('Ctrl Pts',(4.92359008252393,-4.99523503982244,
7.52123305885172));
#159902=CARTESIAN_POINT('Ctrl Pts',(5.05592635132172,-4.85749269608413,
7.52990501067843));
#159903=CARTESIAN_POINT('Ctrl Pts',(5.18826091680305,-4.71975212524454,
7.53857685088737));
#159904=CARTESIAN_POINT('Ctrl Pts',(5.31496347269478,-4.57660078535332,
7.54724869109631));
#159905=CARTESIAN_POINT('Ctrl Pts',(5.43561126741903,-4.42851631045966,
7.55592053130525));
#159906=CARTESIAN_POINT('Ctrl Pts',(5.56176013705625,-4.27367975367592,
7.56498777403881));
#159907=CARTESIAN_POINT('Ctrl Pts',(5.68128895686563,-4.11344992041037,
7.57405501677237));
#159908=CARTESIAN_POINT('Ctrl Pts',(5.79376175354059,-3.9484112381704,7.58312225950592));
#159909=CARTESIAN_POINT('Ctrl Pts',(5.90133874236365,-3.79055649462729,
7.59179481588435));
#159910=CARTESIAN_POINT('Ctrl Pts',(6.00246078174245,-3.62830291661641,
7.60046737226278));
#159911=CARTESIAN_POINT('Ctrl Pts',(6.09679041553322,-3.46219196341887,
7.60913992864121));
#159912=CARTESIAN_POINT('Ctrl Pts',(6.1911166917875,-3.29608692271739,7.61781217633166));
#159913=CARTESIAN_POINT('Ctrl Pts',(6.27865090596307,-3.12612502860771,
7.6264844240221));
#159914=CARTESIAN_POINT('Ctrl Pts',(6.35910096686113,-2.95287342359368,
7.63515667171254));
#159915=CARTESIAN_POINT('Ctrl Pts',(6.43954858437068,-2.77962708048965,
7.64382865601387));
#159916=CARTESIAN_POINT('Ctrl Pts',(6.51291235952014,-2.60309148403811,
7.65250064031521));
#159917=CARTESIAN_POINT('Ctrl Pts',(6.57894750102532,-2.42385567665501,
7.66117262461654));
#159918=CARTESIAN_POINT('Ctrl Pts',(6.64498098171195,-2.24462437714676,
7.6698443908129));
#159919=CARTESIAN_POINT('Ctrl Pts',(6.70368609940955,-2.06269326909702,
7.67851615700926));
#159920=CARTESIAN_POINT('Ctrl Pts',(6.75486698389468,-1.8786693675018,7.68718792320563));
#159921=CARTESIAN_POINT('Ctrl Pts',(6.80605126222577,-1.69463326313241,
7.69586026443384));
#159922=CARTESIAN_POINT('Ctrl Pts',(6.84971023276689,-1.50850436117643,
7.70453260566205));
#159923=CARTESIAN_POINT('Ctrl Pts',(6.88569820761782,-1.32090376489309,
7.71320494689027));
#159924=CARTESIAN_POINT('Ctrl Pts',(6.92168406448288,-1.13331420939253,
7.72187677772865));
#159925=CARTESIAN_POINT('Ctrl Pts',(6.94999977553846,-0.944253411824701,
7.73054860856705));
#159926=CARTESIAN_POINT('Ctrl Pts',(6.97055086371898,-0.754352184862346,
7.73922043940544));
#159927=CARTESIAN_POINT('Ctrl Pts',(6.99110229108047,-0.564447823716458,
7.74789241336617));
#159928=CARTESIAN_POINT('Ctrl Pts',(7.00388880856509,-0.373703287790729,
7.7565643873269));
#159929=CARTESIAN_POINT('Ctrl Pts',(7.00886775178469,-0.182755028638574,
7.76523636128763));
#159930=CARTESIAN_POINT('Ctrl Pts',(7.01045582731897,-0.12185048618891,
7.7680023598286));
#159931=CARTESIAN_POINT('Ctrl Pts',(7.01125000000003,-0.0609252433271523,
7.77076835836956));
#159932=CARTESIAN_POINT('Ctrl Pts',(7.01125,3.55178232870534E-12,7.77353435691052));
#159933=CARTESIAN_POINT('Ctrl Pts',(7.01124860966183,0.00441542920857962,
7.77353435691052));
#159934=CARTESIAN_POINT('Ctrl Pts',(7.01111374519947,0.218566359853513,
7.7832434407798));
#159935=CARTESIAN_POINT('Ctrl Pts',(7.00116331493674,0.432422285858829,
7.79295252464907));
#159936=CARTESIAN_POINT('Ctrl Pts',(6.98150240916137,0.645174916882285,
7.80266160851835));
#159937=CARTESIAN_POINT('Ctrl Pts',(6.96175963902393,0.858813410368804,
7.81241111921059));
#159938=CARTESIAN_POINT('Ctrl Pts',(6.93222542281991,1.07133937000862,7.82216062990284));
#159939=CARTESIAN_POINT('Ctrl Pts',(6.89305680462996,1.28194947273466,7.83191014059508));
#159940=CARTESIAN_POINT('Ctrl Pts',(6.85375143361006,1.493294896973,7.84169369060858));
#159941=CARTESIAN_POINT('Ctrl Pts',(6.80474430104216,1.70271103413845,7.85147724062208));
#159942=CARTESIAN_POINT('Ctrl Pts',(6.74624425403649,1.90940174593501,7.86126079063558));
#159943=CARTESIAN_POINT('Ctrl Pts',(6.6950718161633,2.09020275635724,7.86981887102818));
#159944=CARTESIAN_POINT('Ctrl Pts',(6.63663641341989,2.26891856784468,7.87837695142078));
#159945=CARTESIAN_POINT('Ctrl Pts',(6.57110895151814,2.44502632087637,7.88693503181337));
#159946=CARTESIAN_POINT('',(7.01124941011649,0.0028760461125263,7.22646564306228));
#159947=CARTESIAN_POINT('Ctrl Pts',(6.57110895151815,2.44502632087633,7.33978485479521));
#159948=CARTESIAN_POINT('Ctrl Pts',(6.63540283922006,2.27223384931942,7.33140688128228));
#159949=CARTESIAN_POINT('Ctrl Pts',(6.69284696259494,2.09698487088329,7.32302890776936));
#159950=CARTESIAN_POINT('Ctrl Pts',(6.74327785184177,1.91985165451923,7.31465093425643));
#159951=CARTESIAN_POINT('Ctrl Pts',(6.77527636844613,1.80746021646097,7.30933509056286));
#159952=CARTESIAN_POINT('Ctrl Pts',(6.80445241352737,1.69431048651665,7.3040192468693));
#159953=CARTESIAN_POINT('Ctrl Pts',(6.83077487139492,1.58055092256459,7.29870340317573));
#159954=CARTESIAN_POINT('Ctrl Pts',(6.87364674711721,1.39526860916829,7.29004538988013));
#159955=CARTESIAN_POINT('Ctrl Pts',(6.90902110269817,1.20804545734485,7.28138737658453));
#159956=CARTESIAN_POINT('Ctrl Pts',(6.93673266435705,1.0194932592921,7.27272936328893));
#159957=CARTESIAN_POINT('Ctrl Pts',(6.9643773710318,0.83139594914365,7.26409223771336));
#159958=CARTESIAN_POINT('Ctrl Pts',(6.9843961214186,0.641976267544519,7.2554551121378));
#159959=CARTESIAN_POINT('Ctrl Pts',(6.99667434903633,0.451856853480315,
7.24681798656223));
#159960=CARTESIAN_POINT('Ctrl Pts',(7.00631840262508,0.302525706136942,
7.24003387207136));
#159961=CARTESIAN_POINT('Ctrl Pts',(7.01118792571456,0.152763206930641,
7.2332497575805));
#159962=CARTESIAN_POINT('Ctrl Pts',(7.01124941011624,0.00287604671680145,
7.22646564308963));
#159963=CARTESIAN_POINT('Ctrl Pts',(7.01124941011649,0.00287604611253946,
7.22646564306228));
#159964=CARTESIAN_POINT('Ctrl Pts',(7.01131757022025,-0.163285228295573,
7.21894493810047));
#159965=CARTESIAN_POINT('Ctrl Pts',(7.0054745942836,-0.329575821312576,
7.21142423313868));
#159966=CARTESIAN_POINT('Ctrl Pts',(6.99371928995505,-0.495496776791375,
7.20390352817687));
#159967=CARTESIAN_POINT('Ctrl Pts',(6.98196648505361,-0.661382453954761,
7.1963844222765));
#159968=CARTESIAN_POINT('Ctrl Pts',(6.96430388228091,-0.826898246025481,
7.18886531637613));
#159969=CARTESIAN_POINT('Ctrl Pts',(6.94078235372499,-0.991547719839916,
7.18134621047576));
#159970=CARTESIAN_POINT('Ctrl Pts',(6.91725260803397,-1.15625471317179,
7.17382447781119));
#159971=CARTESIAN_POINT('Ctrl Pts',(6.88785990483266,-1.32009438218466,
7.16630274514664));
#159972=CARTESIAN_POINT('Ctrl Pts',(6.85270668800832,-1.48257802851186,
7.15878101248207));
#159973=CARTESIAN_POINT('Ctrl Pts',(6.82350465433979,-1.61755437887948,
7.15253265428448));
#159974=CARTESIAN_POINT('Ctrl Pts',(6.79032839184365,-1.75159501383976,
7.14628429608688));
#159975=CARTESIAN_POINT('Ctrl Pts',(6.75326300162647,-1.8844270729755,7.14003593788929));
#159976=CARTESIAN_POINT('Ctrl Pts',(6.6959875362354,-2.08968642573767,7.13038063353122));
#159977=CARTESIAN_POINT('Ctrl Pts',(6.62943112543927,-2.29204274376962,
7.12072532917314));
#159978=CARTESIAN_POINT('Ctrl Pts',(6.55391163375439,-2.49075668411005,
7.11107002481508));
#159979=CARTESIAN_POINT('Ctrl Pts',(6.47797377825457,-2.69057146239716,
7.1013612318824));
#159980=CARTESIAN_POINT('Ctrl Pts',(6.39297332712872,-2.88670337037012,
7.09165243894973));
#159981=CARTESIAN_POINT('Ctrl Pts',(6.29927765817105,-3.07842939626152,
7.08194364601705));
#159982=CARTESIAN_POINT('Ctrl Pts',(6.20513111770013,-3.27107802406593,
7.07218813354855));
#159983=CARTESIAN_POINT('Ctrl Pts',(6.10220551435119,-3.45927823647201,
7.06243262108007));
#159984=CARTESIAN_POINT('Ctrl Pts',(5.99091723264469,-3.64232580559467,
7.05267710861158));
#159985=CARTESIAN_POINT('Ctrl Pts',(5.87951875841874,-3.82555461997077,
7.04291193668496));
#159986=CARTESIAN_POINT('Ctrl Pts',(5.75974107273603,-4.00362055912466,
7.03314676475832));
#159987=CARTESIAN_POINT('Ctrl Pts',(5.63204484367387,-4.17584691306405,
7.0233815928317));
#159988=CARTESIAN_POINT('Ctrl Pts',(5.50452272552154,-4.34783844027911,
7.01362973549534));
#159989=CARTESIAN_POINT('Ctrl Pts',(5.36910366545502,-4.51400626528277,
7.003877878159));
#159990=CARTESIAN_POINT('Ctrl Pts',(5.2262888972894,-4.67370633700595,6.99412602082265));
#159991=CARTESIAN_POINT('Ctrl Pts',(5.16401131506322,-4.743347134495,6.98987350474939));
#159992=CARTESIAN_POINT('Ctrl Pts',(5.10032791452013,-4.81175841621377,
6.98562098867613));
#159993=CARTESIAN_POINT('Ctrl Pts',(5.03528278304038,-4.87888858832799,
6.98136847260287));
#159994=CARTESIAN_POINT('Ctrl Pts',(4.912411875898,-5.00569815818591,6.97333542699789));
#159995=CARTESIAN_POINT('Ctrl Pts',(4.78461915748462,-5.12799552920953,
6.9653023813929));
#159996=CARTESIAN_POINT('Ctrl Pts',(4.65227703156344,-5.24537367439988,
6.95726933578793));
#159997=CARTESIAN_POINT('Ctrl Pts',(4.52001998025667,-5.36267636439883,
6.94924145413398));
#159998=CARTESIAN_POINT('Ctrl Pts',(4.38321961589875,-5.4750658809148,6.94121357248004));
#159999=CARTESIAN_POINT('Ctrl Pts',(4.24228557003584,-5.58217159399151,
6.93318569082609));
#160000=CARTESIAN_POINT('Ctrl Pts',(4.10141515728416,-5.68922894778277,
6.92516143383985));
#160001=CARTESIAN_POINT('Ctrl Pts',(3.95641507048716,-5.79100702697689,
6.91713717685362));
#160002=CARTESIAN_POINT('Ctrl Pts',(3.80772838996846,-5.88717513504806,
6.90911291986739));
#160003=CARTESIAN_POINT('Ctrl Pts',(3.65905968718424,-5.98333161541522,
6.90108963309558));
#160004=CARTESIAN_POINT('Ctrl Pts',(3.50670558196251,-6.0738792702854,6.89306634632377));
#160005=CARTESIAN_POINT('Ctrl Pts',(3.3511386818256,-6.15853035209475,6.88504305955196));
#160006=CARTESIAN_POINT('Ctrl Pts',(3.19558452900869,-6.24317449750292,
6.87702043021694));
#160007=CARTESIAN_POINT('Ctrl Pts',(3.03681842963845,-6.32192286056721,
6.86899780088192));
#160008=CARTESIAN_POINT('Ctrl Pts',(2.87533789368541,-6.39453349038355,
6.8609751715469));
#160009=CARTESIAN_POINT('Ctrl Pts',(2.71379665254778,-6.46717141662704,
6.85294952627444));
#160010=CARTESIAN_POINT('Ctrl Pts',(2.54953927212061,-6.5336668526107,6.84492388100198));
#160011=CARTESIAN_POINT('Ctrl Pts',(2.38308390614504,-6.5938257225053,6.83689823572952));
#160012=CARTESIAN_POINT('Ctrl Pts',(2.28493167991229,-6.62929905779368,
6.83216582625849));
#160013=CARTESIAN_POINT('Ctrl Pts',(2.18601556915375,-6.6625700913399,6.82743341678746));
#160014=CARTESIAN_POINT('Ctrl Pts',(2.08644434056026,-6.69360714235935,
6.82270100731643));
#160015=CARTESIAN_POINT('Ctrl Pts',(1.90276165401132,-6.75086232535084,
6.81397095850849));
#160016=CARTESIAN_POINT('Ctrl Pts',(1.71675704446272,-6.80054131086613,
6.80524090970055));
#160017=CARTESIAN_POINT('Ctrl Pts',(1.52905784929066,-6.84248556125788,
6.7965108608926));
#160018=CARTESIAN_POINT('Ctrl Pts',(1.3413043806691,-6.88444193988042,6.78777828778048));
#160019=CARTESIAN_POINT('Ctrl Pts',(1.15185561572288,-6.91865905944544,
6.77904571466835));
#160020=CARTESIAN_POINT('Ctrl Pts',(0.961349495982859,-6.94502942463698,
6.77031314155622));
#160021=CARTESIAN_POINT('Ctrl Pts',(0.768136931815597,-6.97177442308448,
6.76145650826237));
#160022=CARTESIAN_POINT('Ctrl Pts',(0.573837028153697,-6.99044797678349,
6.75259987496852));
#160023=CARTESIAN_POINT('Ctrl Pts',(0.379121580805413,-7.00099231462709,
6.74374324167466));
#160024=CARTESIAN_POINT('Ctrl Pts',(0.187011414285745,-7.01139556987243,
6.73500510959497));
#160025=CARTESIAN_POINT('Ctrl Pts',(-0.00550296647739609,-7.01388580322923,
6.72626697751529));
#160026=CARTESIAN_POINT('Ctrl Pts',(-0.197774497716119,-7.00846001704748,
6.7175288454356));
#160027=CARTESIAN_POINT('Ctrl Pts',(-0.393957232692518,-7.00292385906468,
6.70861296153466));
#160028=CARTESIAN_POINT('Ctrl Pts',(-0.589886835983756,-6.98914617974144,
6.69969707763373));
#160029=CARTESIAN_POINT('Ctrl Pts',(-0.78487840171196,-6.96717966303626,
6.6907811937328));
#160030=CARTESIAN_POINT('Ctrl Pts',(-0.979869967440173,-6.94521314633108,
6.68186530983186));
#160031=CARTESIAN_POINT('Ctrl Pts',(-1.17392319577496,-6.91505783214244,
6.67294942593093));
#160032=CARTESIAN_POINT('Ctrl Pts',(-1.36636015085385,-6.87682241305231,
6.66403354203));
#160033=CARTESIAN_POINT('Ctrl Pts',(-1.55501567164087,-6.83933832950921,
6.65529285747741));
#160034=CARTESIAN_POINT('Ctrl Pts',(-1.74213788700388,-6.79408476441464,
6.6465521729248));
#160035=CARTESIAN_POINT('Ctrl Pts',(-1.9270972911631,-6.74121076609327,
6.6378114883722));
#160036=CARTESIAN_POINT('Ctrl Pts',(-2.11202341805838,-6.688346280681,6.6290723764137));
#160037=CARTESIAN_POINT('Ctrl Pts',(-2.29478724770831,-6.62786417534572,
6.6203332644552));
#160038=CARTESIAN_POINT('Ctrl Pts',(-2.47477335420135,-6.55996367427709,
6.6115941524967));
#160039=CARTESIAN_POINT('Ctrl Pts',(-2.65709143798604,-6.49118342515641,
6.60274181285061));
#160040=CARTESIAN_POINT('Ctrl Pts',(-2.8365590434985,-6.41479128798384,
6.5938894732045));
#160041=CARTESIAN_POINT('Ctrl Pts',(-3.01255500787018,-6.33104563931238,
6.58503713355841));
#160042=CARTESIAN_POINT('Ctrl Pts',(-3.18621080598725,-6.2484135317479,
6.57630250085286));
#160043=CARTESIAN_POINT('Ctrl Pts',(-3.35648646466823,-6.15862238645124,
6.56756786814732));
#160044=CARTESIAN_POINT('Ctrl Pts',(-3.52280689854241,-6.06196817197864,
6.55883323544177));
#160045=CARTESIAN_POINT('Ctrl Pts',(-3.69248930596735,-5.9633602053118,
6.5499220423254));
#160046=CARTESIAN_POINT('Ctrl Pts',(-3.85805462311256,-5.85760888370049,
6.54101084920905));
#160047=CARTESIAN_POINT('Ctrl Pts',(-4.01891922818866,-5.74507744071352,
6.53209965609268));
#160048=CARTESIAN_POINT('Ctrl Pts',(-4.17978383326477,-5.63254599772656,
6.52318846297632));
#160049=CARTESIAN_POINT('Ctrl Pts',(-4.33594747016127,-5.51323459608025,
6.51427726985994));
#160050=CARTESIAN_POINT('Ctrl Pts',(-4.48685773942913,-5.38755363672836,
6.50536607674358));
#160051=CARTESIAN_POINT('Ctrl Pts',(-4.62277166467131,-5.2743619195802,
6.49734041195011));
#160052=CARTESIAN_POINT('Ctrl Pts',(-4.75448655588241,-5.15595124616252,
6.48931474715665));
#160053=CARTESIAN_POINT('Ctrl Pts',(-4.88157791519271,-5.03267559260507,
6.48128908236318));
#160054=CARTESIAN_POINT('Ctrl Pts',(-5.00862893882244,-4.90943906371678,
6.47326596471888));
#160055=CARTESIAN_POINT('Ctrl Pts',(-5.13105908918682,-4.78134088361919,
6.46524284707458));
#160056=CARTESIAN_POINT('Ctrl Pts',(-5.24847882072518,-4.64877366957128,
6.45721972943029));
#160057=CARTESIAN_POINT('Ctrl Pts',(-5.36588374460855,-4.51622317340838,
6.4491976235713));
#160058=CARTESIAN_POINT('Ctrl Pts',(-5.47827926571286,-4.37920504061177,
6.44117551771231));
#160059=CARTESIAN_POINT('Ctrl Pts',(-5.58531445971767,-4.23814687671024,
6.43315341185331));
#160060=CARTESIAN_POINT('Ctrl Pts',(-5.69238942836389,-4.09703629511619,
6.42512832495255));
#160061=CARTESIAN_POINT('Ctrl Pts',(-5.79409986651127,-3.95188297379347,
6.41710323805178));
#160062=CARTESIAN_POINT('Ctrl Pts',(-5.89013647044135,-3.80314592437323,
6.40907815115102));
#160063=CARTESIAN_POINT('Ctrl Pts',(-5.98619198830061,-3.65437958193445,
6.4010514837495));
#160064=CARTESIAN_POINT('Ctrl Pts',(-6.07657125439554,-3.50202841806052,
6.39302481634798));
#160065=CARTESIAN_POINT('Ctrl Pts',(-6.16100981452104,-3.34657804748005,
6.38499814894646));
#160066=CARTESIAN_POINT('Ctrl Pts',(-6.24551616162911,-3.19100288188241,
6.37696503776425));
#160067=CARTESIAN_POINT('Ctrl Pts',(-6.32407211075625,-3.03232386684494,
6.36893192658205));
#160068=CARTESIAN_POINT('Ctrl Pts',(-6.39646017371002,-2.87104925221453,
6.36089881539984));
#160069=CARTESIAN_POINT('Ctrl Pts',(-6.43911385352952,-2.77602038288491,
6.35616541408561));
#160070=CARTESIAN_POINT('Ctrl Pts',(-6.47962695838208,-2.68009070373161,
6.35143201277137));
#160071=CARTESIAN_POINT('Ctrl Pts',(-6.51796300787284,-2.58336694848045,
6.34669861145713));
#160072=CARTESIAN_POINT('Ctrl Pts',(-6.59693645836743,-2.38411301390853,
6.33694765799879));
#160073=CARTESIAN_POINT('Ctrl Pts',(-6.66671560835717,-2.18137117766495,
6.32719670454047));
#160074=CARTESIAN_POINT('Ctrl Pts',(-6.72706144207423,-1.97592280139134,
6.31744575108213));
#160075=CARTESIAN_POINT('Ctrl Pts',(-6.78749421530973,-1.77017843810756,
6.30768074954217));
#160076=CARTESIAN_POINT('Ctrl Pts',(-6.83846647645426,-1.56171977215431,
6.2979157480022));
#160077=CARTESIAN_POINT('Ctrl Pts',(-6.87978909168529,-1.35134326372988,
6.28815074646224));
#160078=CARTESIAN_POINT('Ctrl Pts',(-6.92104283065413,-1.14131740948047,
6.27840202116236));
#160079=CARTESIAN_POINT('Ctrl Pts',(-6.95267906171902,-0.92938013875767,
6.26865329586247));
#160080=CARTESIAN_POINT('Ctrl Pts',(-6.974560252916,-0.716335006086056,
6.25890457056258));
#160081=CARTESIAN_POINT('Ctrl Pts',(-6.99638138870826,-0.503874599883472,
6.24918260174219));
#160082=CARTESIAN_POINT('Ctrl Pts',(-7.00850093008893,-0.290312441622313,
6.2394606329218));
#160083=CARTESIAN_POINT('Ctrl Pts',(-7.0108331209835,-0.0764559495448779,
6.2297386641014));
#160084=CARTESIAN_POINT('Ctrl Pts',(-7.01314988037575,0.135985509585613,
6.22008102302742));
#160085=CARTESIAN_POINT('Ctrl Pts',(-7.00580835251575,0.348717373991946,
6.21042338195344));
#160086=CARTESIAN_POINT('Ctrl Pts',(-6.98877490237801,0.560938433690608,
6.20076574087945));
#160087=CARTESIAN_POINT('Ctrl Pts',(-6.98128811610057,0.654216877264134,
6.19652087597655));
#160088=CARTESIAN_POINT('Ctrl Pts',(-6.97192960369691,0.747396515675602,
6.19227601107363));
#160089=CARTESIAN_POINT('Ctrl Pts',(-6.96069965522493,0.840408753078836,
6.18803114617072));
#160090=CARTESIAN_POINT('Ctrl Pts',(-6.93992730107203,1.01245612628937,
6.18017929918189));
#160091=CARTESIAN_POINT('Ctrl Pts',(-6.91275659676435,1.18385961718861,
6.17232745219306));
#160092=CARTESIAN_POINT('Ctrl Pts',(-6.87924919440166,1.35408902359633,
6.16447560520423));
#160093=CARTESIAN_POINT('Ctrl Pts',(-6.84575129446697,1.52427015432279,
6.15662598493563));
#160094=CARTESIAN_POINT('Ctrl Pts',(-6.80592034468947,1.69327748896089,
6.14877636466701));
#160095=CARTESIAN_POINT('Ctrl Pts',(-6.75986945775669,1.86058901334718,
6.14092674439841));
#160096=CARTESIAN_POINT('Ctrl Pts',(-6.71382224739759,2.02788718005055,
6.13307775082147));
#160097=CARTESIAN_POINT('Ctrl Pts',(-6.66155619039472,2.19348943843572,
6.12522875724454));
#160098=CARTESIAN_POINT('Ctrl Pts',(-6.6032347459023,2.35688723807666,6.11737976366761));
#160099=CARTESIAN_POINT('Ctrl Pts',(-6.54488377496868,2.5203677612435,6.10952679637484));
#160100=CARTESIAN_POINT('Ctrl Pts',(-6.48047141959149,2.68164123600291,
6.10167382908207));
#160101=CARTESIAN_POINT('Ctrl Pts',(-6.41021006923064,2.84021714501446,
6.0938208617893));
#160102=CARTESIAN_POINT('Ctrl Pts',(-6.33993087484643,2.99883332698135,
6.08596590010658));
#160103=CARTESIAN_POINT('Ctrl Pts',(-6.26379989351225,3.15475023551417,
6.07811093842385));
#160104=CARTESIAN_POINT('Ctrl Pts',(-6.18207600021978,3.30750100378014,
6.07025597674112));
#160105=CARTESIAN_POINT('Ctrl Pts',(-6.10027098912941,3.46040338995675,
6.06239321835208));
#160106=CARTESIAN_POINT('Ctrl Pts',(-6.01286217068981,3.61013302988238,
6.05453045996305));
#160107=CARTESIAN_POINT('Ctrl Pts',(-5.9201526622887,3.75625065959342,6.04666770157402));
#160108=CARTESIAN_POINT('Ctrl Pts',(-5.85214229526773,3.86344045917565,
6.04089969467744));
#160109=CARTESIAN_POINT('Ctrl Pts',(-5.7812802946199,3.9686870491885,6.03513168778086));
#160110=CARTESIAN_POINT('Ctrl Pts',(-5.70770009220788,4.07182836326757,
6.02936368088429));
#160111=CARTESIAN_POINT('Ctrl Pts',(-5.60082438494124,4.22164177134821,
6.02098561455147));
#160112=CARTESIAN_POINT('Ctrl Pts',(-5.4879758233974,4.36734428812648,6.01260754821865));
#160113=CARTESIAN_POINT('Ctrl Pts',(-5.36949712189324,4.5084506452306,6.00422948188583));
#160114=CARTESIAN_POINT('Ctrl Pts',(-5.25109943473175,4.64946051546728,
5.99585714437624));
#160115=CARTESIAN_POINT('Ctrl Pts',(-5.12707949372502,4.78588024089517,
5.98748480686666));
#160116=CARTESIAN_POINT('Ctrl Pts',(-4.99782144854695,4.91725607742205,
5.97911246935706));
#160117=CARTESIAN_POINT('Ctrl Pts',(-4.86863283271904,5.0485613470535,5.97074462894436));
#160118=CARTESIAN_POINT('Ctrl Pts',(-4.73421195276814,5.17482789599584,
5.96237678853165));
#160119=CARTESIAN_POINT('Ctrl Pts',(-4.59498142208136,5.29563709984239,
5.95400894811894));
#160120=CARTESIAN_POINT('Ctrl Pts',(-4.45580528107472,5.41639911020401,
5.94564437655942));
#160121=CARTESIAN_POINT('Ctrl Pts',(-4.31182348396954,5.53170781163764,
5.93727980499988));
#160122=CARTESIAN_POINT('Ctrl Pts',(-4.16349382203681,5.64118301035885,
5.92891523344036));
#160123=CARTESIAN_POINT('Ctrl Pts',(-4.0152003924244,5.75063146769593,5.92055270508536));
#160124=CARTESIAN_POINT('Ctrl Pts',(-3.86256148044464,5.85424906933691,
5.91219017673037));
#160125=CARTESIAN_POINT('Ctrl Pts',(-3.7060664825293,5.95169705122605,5.90382764837537));
#160126=CARTESIAN_POINT('Ctrl Pts',(-3.54955899581676,6.04915280977324,
5.89546445266408));
#160127=CARTESIAN_POINT('Ctrl Pts',(-3.38919508417895,6.14043778605301,
5.88710125695277));
#160128=CARTESIAN_POINT('Ctrl Pts',(-3.22549219738419,6.2252571550992,5.87873806124149));
#160129=CARTESIAN_POINT('Ctrl Pts',(-3.06177814637302,6.31008230866031,
5.87037429517662));
#160130=CARTESIAN_POINT('Ctrl Pts',(-2.89472495800337,6.38844082427623,
5.86201052911176));
#160131=CARTESIAN_POINT('Ctrl Pts',(-2.72487385034697,6.46008429218964,
5.8536467630469));
#160132=CARTESIAN_POINT('Ctrl Pts',(-2.5549885140255,6.53174219780852,5.84528131150261));
#160133=CARTESIAN_POINT('Ctrl Pts',(-2.38230443704883,6.59668222958885,
5.83691585995833));
#160134=CARTESIAN_POINT('Ctrl Pts',(-2.20738233519328,6.65470433518851,
5.82855040841404));
#160135=CARTESIAN_POINT('Ctrl Pts',(-2.0324016522518,6.7127458722832,5.82018215529562));
#160136=CARTESIAN_POINT('Ctrl Pts',(-1.85518176182634,6.76386475996052,
5.8118139021772));
#160137=CARTESIAN_POINT('Ctrl Pts',(-1.67629844704744,6.80791084540084,
5.80344564905878));
#160138=CARTESIAN_POINT('Ctrl Pts',(-1.49724928186962,6.85199776785745,
5.79506963737372));
#160139=CARTESIAN_POINT('Ctrl Pts',(-1.31653393007678,6.88899870554986,
5.78669362568866));
#160140=CARTESIAN_POINT('Ctrl Pts',(-1.13473949834754,6.91881440952061,
5.7783176140036));
#160141=CARTESIAN_POINT('Ctrl Pts',(-0.95285591235669,6.94864473548526,
5.76993749461772));
#160142=CARTESIAN_POINT('Ctrl Pts',(-0.769892516413647,6.97128275400953,
5.76155737523184));
#160143=CARTESIAN_POINT('Ctrl Pts',(-0.586442106525143,6.98668105885723,
5.75317725584596));
#160144=CARTESIAN_POINT('Ctrl Pts',(-0.402782081242819,7.00209695822399,
5.74478756110929));
#160145=CARTESIAN_POINT('Ctrl Pts',(-0.218634258290256,7.01025659315712,
5.73639786637262));
#160146=CARTESIAN_POINT('Ctrl Pts',(-0.034593355991068,7.01116465804514,
5.72800817163596));
#160147=CARTESIAN_POINT('Ctrl Pts',(0.0822510668830052,7.01174117292009,
5.72268169786111));
#160148=CARTESIAN_POINT('Ctrl Pts',(0.199052410907578,7.00939580229304,
5.71735522408627));
#160149=CARTESIAN_POINT('Ctrl Pts',(0.31565942591468,7.00414061033409,5.71202875031143));
#160150=CARTESIAN_POINT('Ctrl Pts',(0.499142634924632,6.99587147245648,
5.70364744923058));
#160151=CARTESIAN_POINT('Ctrl Pts',(0.68251458485407,6.98037849663042,5.69526614814971));
#160152=CARTESIAN_POINT('Ctrl Pts',(0.865182576578385,6.95766380846942,
5.68688484706885));
#160153=CARTESIAN_POINT('Ctrl Pts',(1.04761906322664,6.93497790786754,5.67851416806646));
#160154=CARTESIAN_POINT('Ctrl Pts',(1.2293530471497,6.90508857495438,5.67014348906408));
#160155=CARTESIAN_POINT('Ctrl Pts',(1.40979338410086,6.86804988163638,5.6617728100617));
#160156=CARTESIAN_POINT('Ctrl Pts',(1.59002895208051,6.83105322091078,5.65341163035066));
#160157=CARTESIAN_POINT('Ctrl Pts',(1.76897348010267,6.78692343596839,5.64505045063961));
#160158=CARTESIAN_POINT('Ctrl Pts',(1.9460420495598,6.73576624474492,5.63668927092857));
#160159=CARTESIAN_POINT('Ctrl Pts',(2.12288085134853,6.68467543610186,5.62833894084925));
#160160=CARTESIAN_POINT('Ctrl Pts',(2.29784823671262,6.62657550030596,5.61998861076992));
#160161=CARTESIAN_POINT('Ctrl Pts',(2.47037064399661,6.56162292758276,5.6116382806906));
#160162=CARTESIAN_POINT('Ctrl Pts',(2.64276030541287,6.49672033205246,5.60329437570022));
#160163=CARTESIAN_POINT('Ctrl Pts',(2.81270843243529,6.42497572208527,5.59495047070984));
#160164=CARTESIAN_POINT('Ctrl Pts',(2.9796566649325,6.3465953645733,5.58660656571946));
#160165=CARTESIAN_POINT('Ctrl Pts',(3.14647080324813,6.26827796280358,5.5782693626216));
#160166=CARTESIAN_POINT('Ctrl Pts',(3.31028955679106,6.18333558203062,5.56993215952376));
#160167=CARTESIAN_POINT('Ctrl Pts',(3.470574455851,6.09202261230985,5.5615949564259));
#160168=CARTESIAN_POINT('Ctrl Pts',(3.52333928093263,6.0619629316833,5.55885039929227));
#160169=CARTESIAN_POINT('Ctrl Pts',(3.57572131606705,6.03121326287636,5.55610584215863));
#160170=CARTESIAN_POINT('Ctrl Pts',(3.62770187811974,5.999783799937,5.553361285025));
#160171=CARTESIAN_POINT('Ctrl Pts',(3.78562535409301,5.90429714416894,5.54502297575256));
#160172=CARTESIAN_POINT('Ctrl Pts',(3.93971164680453,5.80261084754989,5.53668466648012));
#160173=CARTESIAN_POINT('Ctrl Pts',(4.08947460581958,5.69507014977488,5.52834635720769));
#160174=CARTESIAN_POINT('Ctrl Pts',(4.23933179035228,5.58746179122458,5.52000280176816));
#160175=CARTESIAN_POINT('Ctrl Pts',(4.38485994949304,5.47399187566745,5.51165924632863));
#160176=CARTESIAN_POINT('Ctrl Pts',(4.52560533670533,5.3550464889564,5.5033156908891));
#160177=CARTESIAN_POINT('Ctrl Pts',(4.66645780219709,5.23601060928062,5.49496578772067));
#160178=CARTESIAN_POINT('Ctrl Pts',(4.80251998776095,5.11149116047744,5.48661588455225));
#160179=CARTESIAN_POINT('Ctrl Pts',(4.93337406187388,4.9819119751487,5.47826598138382));
#160180=CARTESIAN_POINT('Ctrl Pts',(5.0644244072465,4.85213843079747,5.46990355398927));
#160181=CARTESIAN_POINT('Ctrl Pts',(5.19025079776716,4.71729021501192,5.46154112659473));
#160182=CARTESIAN_POINT('Ctrl Pts',(5.31047385128612,4.5778263441623,5.45317869920018));
#160183=CARTESIAN_POINT('Ctrl Pts',(5.43079971181987,4.43824321278974,5.44480912079614));
#160184=CARTESIAN_POINT('Ctrl Pts',(5.54551247135562,4.29403680685261,5.43643954239211));
#160185=CARTESIAN_POINT('Ctrl Pts',(5.65427503038995,4.14569661736224,5.42806996398807));
#160186=CARTESIAN_POINT('Ctrl Pts',(5.76320534240702,3.997127631221,5.41968747653009));
#160187=CARTESIAN_POINT('Ctrl Pts',(5.86616693181532,3.84441239180857,5.41130498907212));
#160188=CARTESIAN_POINT('Ctrl Pts',(5.96286699486789,3.68806775480266,5.40292250161414));
#160189=CARTESIAN_POINT('Ctrl Pts',(5.99450891739559,3.63690910261986,5.40017960765562));
#160190=CARTESIAN_POINT('Ctrl Pts',(6.02548078590298,3.58536202772556,5.3974367136971));
#160191=CARTESIAN_POINT('Ctrl Pts',(6.05577344516303,3.5334451380145,5.39469381973858));
#160192=CARTESIAN_POINT('Ctrl Pts',(6.15138017468945,3.36959012648025,5.38603696599194));
#160193=CARTESIAN_POINT('Ctrl Pts',(6.24039807521569,3.20174082998824,5.3773801122453));
#160194=CARTESIAN_POINT('Ctrl Pts',(6.32250483875401,3.03043876797273,5.36872325849865));
#160195=CARTESIAN_POINT('Ctrl Pts',(6.40450656935418,2.85935583965718,5.36007747880662));
#160196=CARTESIAN_POINT('Ctrl Pts',(6.47961467772508,2.68482922005942,5.3514316991146));
#160197=CARTESIAN_POINT('Ctrl Pts',(6.5475526276583,2.50742520337994,5.34278591942257));
#160198=CARTESIAN_POINT('Ctrl Pts',(6.55550301070338,2.48666464337298,5.34177415412287));
#160199=CARTESIAN_POINT('Ctrl Pts',(6.56335525258107,2.4658647061558,5.34076238882317));
#160200=CARTESIAN_POINT('Ctrl Pts',(6.57110895151813,2.44502632087638,5.33975062352347));
#160201=CARTESIAN_POINT('Origin',(0.,0.,50.));
#160202=CARTESIAN_POINT('',(6.57110895151814,2.44502632087637,3.33981554959538));
#160203=CARTESIAN_POINT('',(6.57110895151814,2.44502632087637,3.88698101089639));
#160204=CARTESIAN_POINT('',(6.57110895151814,2.44502632087636,50.));
#160205=CARTESIAN_POINT('',(7.01124963752017,-0.002254522849646,5.77353435691053));
#160206=CARTESIAN_POINT('Ctrl Pts',(6.57110895151813,2.44502632087638,3.88698101089636));
#160207=CARTESIAN_POINT('Ctrl Pts',(6.50404475006846,2.62526412474361,3.8957147867161));
#160208=CARTESIAN_POINT('Ctrl Pts',(6.4295520875458,2.8027648898791,3.90444856253583));
#160209=CARTESIAN_POINT('Ctrl Pts',(6.34787495986428,2.9769296357872,3.91318233835557));
#160210=CARTESIAN_POINT('Ctrl Pts',(6.26622791776542,3.15103022851057,3.92191289710902));
#160211=CARTESIAN_POINT('Ctrl Pts',(6.17740181137757,3.32179700819347,3.93064345586247));
#160212=CARTESIAN_POINT('Ctrl Pts',(6.0816880179526,3.48865266468185,3.93937401461591));
#160213=CARTESIAN_POINT('Ctrl Pts',(6.01293388485033,3.608510164887,3.94564544088701));
#160214=CARTESIAN_POINT('Ctrl Pts',(5.9406267137465,3.72634995895831,3.9519168671581));
#160215=CARTESIAN_POINT('Ctrl Pts',(5.86488917672598,3.84196583889321,3.9581882934292));
#160216=CARTESIAN_POINT('Ctrl Pts',(5.76796621207628,3.98992198170838,3.9662139733059));
#160217=CARTESIAN_POINT('Ctrl Pts',(5.66537871576642,4.1343028176686,3.97423965318258));
#160218=CARTESIAN_POINT('Ctrl Pts',(5.55742985037872,4.27464618660066,3.98226533305928));
#160219=CARTESIAN_POINT('Ctrl Pts',(5.44951524390886,4.41494501581543,3.99028846588645));
#160220=CARTESIAN_POINT('Ctrl Pts',(5.33624287910824,4.55120863881733,3.99831159871363));
#160221=CARTESIAN_POINT('Ctrl Pts',(5.21795829982202,4.68300520433392,4.0063347315408));
#160222=CARTESIAN_POINT('Ctrl Pts',(5.09968863589183,4.81478515067062,4.01435685267326));
#160223=CARTESIAN_POINT('Ctrl Pts',(4.97640826161214,4.94209888918038,4.0223789738057));
#160224=CARTESIAN_POINT('Ctrl Pts',(4.84850189231907,5.06454893970612,4.03040109493816));
#160225=CARTESIAN_POINT('Ctrl Pts',(4.72054799115267,5.18704449445752,4.0384261972079));
#160226=CARTESIAN_POINT('Ctrl Pts',(4.58796492374278,5.30467249467776,4.04645129947765));
#160227=CARTESIAN_POINT('Ctrl Pts',(4.45117336088422,5.41707322027815,4.05447640174739));
#160228=CARTESIAN_POINT('Ctrl Pts',(4.31435485656344,5.52949608350048,4.06250308458238));
#160229=CARTESIAN_POINT('Ctrl Pts',(4.17332649434682,5.63668939520866,4.07052976741736));
#160230=CARTESIAN_POINT('Ctrl Pts',(4.02854049783307,5.73833495186704,4.07855645025234));
#160231=CARTESIAN_POINT('Ctrl Pts',(3.88363826722259,5.84006210950721,4.08658957690268));
#160232=CARTESIAN_POINT('Ctrl Pts',(3.73497268265571,5.93623241389945,4.09462270355302));
#160233=CARTESIAN_POINT('Ctrl Pts',(3.58302382035294,6.02657173401956,4.10265583020336));
#160234=CARTESIAN_POINT('Ctrl Pts',(3.49349193253668,6.07980181255923,4.10738913970745));
#160235=CARTESIAN_POINT('Ctrl Pts',(3.4028206236895,6.13100832511276,4.11212244921153));
#160236=CARTESIAN_POINT('Ctrl Pts',(3.31111175468872,6.18014283900156,4.11685575871562));
#160237=CARTESIAN_POINT('Ctrl Pts',(3.12218526897848,6.28136326770418,4.12660669709408));
#160238=CARTESIAN_POINT('Ctrl Pts',(2.92874330649919,6.37384810930519,4.13635763547254));
#160239=CARTESIAN_POINT('Ctrl Pts',(2.73153480289983,6.45727064502078,4.14610857385101));
#160240=CARTESIAN_POINT('Ctrl Pts',(2.53404219874635,6.54081336008051,4.15587355952939));
#160241=CARTESIAN_POINT('Ctrl Pts',(2.33277223522788,6.6152676398631,4.16563854520778));
#160242=CARTESIAN_POINT('Ctrl Pts',(2.12849454649652,6.68035459598026,4.17540353088616));
#160243=CARTESIAN_POINT('Ctrl Pts',(1.92455734720968,6.74533306535238,4.18515224031543));
#160244=CARTESIAN_POINT('Ctrl Pts',(1.71762247832009,6.80097540444875,4.1949009497447));
#160245=CARTESIAN_POINT('Ctrl Pts',(1.50847251728717,6.84705317834536,4.20464965917397));
#160246=CARTESIAN_POINT('Ctrl Pts',(1.29989658111883,6.89300448897231,4.21437161267375));
#160247=CARTESIAN_POINT('Ctrl Pts',(1.08911772845036,6.92944363070854,4.22409356617353));
#160248=CARTESIAN_POINT('Ctrl Pts',(0.876928290547881,6.95619316406156,
4.23381551967331));
#160249=CARTESIAN_POINT('Ctrl Pts',(0.666142826683952,6.98276570627524,
4.24347314683125));
#160250=CARTESIAN_POINT('Ctrl Pts',(0.453965425161636,6.99977640646201,
4.25313077398921));
#160251=CARTESIAN_POINT('Ctrl Pts',(0.241188204621614,7.00710031414218,
4.26278840114715));
#160252=CARTESIAN_POINT('Ctrl Pts',(0.147663498990188,7.01031948538674,
4.26703334209878));
#160253=CARTESIAN_POINT('Ctrl Pts',(0.0540231068225535,7.0116678307699,
4.27127828305041));
#160254=CARTESIAN_POINT('Ctrl Pts',(-0.0396647883018845,7.01113780117528,
4.27552322400204));
#160255=CARTESIAN_POINT('Ctrl Pts',(-0.212958871141432,7.01015740779197,
4.28337507239659));
#160256=CARTESIAN_POINT('Ctrl Pts',(-0.386344281526877,7.00274699430319,
4.29122692079114));
#160257=CARTESIAN_POINT('Ctrl Pts',(-0.559287245113946,6.98890723503702,
4.29907876918568));
#160258=CARTESIAN_POINT('Ctrl Pts',(-0.732181163610055,6.97507140060387,
4.30692839086565));
#160259=CARTESIAN_POINT('Ctrl Pts',(-0.904632505023892,6.95480987765904,
4.31477801254561));
#160260=CARTESIAN_POINT('Ctrl Pts',(-1.07610975018993,6.92817539963057,
4.32262763422557));
#160261=CARTESIAN_POINT('Ctrl Pts',(-1.24757330521086,6.90154304800591,
4.33047662921912));
#160262=CARTESIAN_POINT('Ctrl Pts',(-1.41806254197057,6.86853881345669,
4.33832562421267));
#160263=CARTESIAN_POINT('Ctrl Pts',(-1.58705356494276,6.82926698442099,
4.34617461920622));
#160264=CARTESIAN_POINT('Ctrl Pts',(-1.75613014321767,6.78997527318585,
4.35402758792056));
#160265=CARTESIAN_POINT('Ctrl Pts',(-1.92370662013163,6.74440971390524,
4.36188055663491));
#160266=CARTESIAN_POINT('Ctrl Pts',(-2.0892714250179,6.69272526517439,4.36973352534925));
#160267=CARTESIAN_POINT('Ctrl Pts',(-2.25487827788404,6.64102769030444,
4.3775884884577));
#160268=CARTESIAN_POINT('Ctrl Pts',(-2.41847208118997,6.58320825719328,
4.38544345156615));
#160269=CARTESIAN_POINT('Ctrl Pts',(-2.57955944907681,6.5194708076023,4.3932984146746));
#160270=CARTESIAN_POINT('Ctrl Pts',(-2.74080670963018,6.4556700932693,4.40116117448998));
#160271=CARTESIAN_POINT('Ctrl Pts',(-2.89954221680159,6.38593978368614,
4.40902393430535));
#160272=CARTESIAN_POINT('Ctrl Pts',(-3.05529495229387,6.3105308268788,4.41688669412072));
#160273=CARTESIAN_POINT('Ctrl Pts',(-3.16955273817767,6.25521198825049,
4.42265469250997));
#160274=CARTESIAN_POINT('Ctrl Pts',(-3.28220583408499,6.1968381901427,4.42842269089923));
#160275=CARTESIAN_POINT('Ctrl Pts',(-3.39307799138927,6.1355234745578,4.43419068928848));
#160276=CARTESIAN_POINT('Ctrl Pts',(-3.55412074152026,6.04646332941971,
4.44256875593696));
#160277=CARTESIAN_POINT('Ctrl Pts',(-3.71176189921157,5.95099977948684,
4.45094682258544));
#160278=CARTESIAN_POINT('Ctrl Pts',(-3.86548021925234,5.84941785454492,
4.45932488923393));
#160279=CARTESIAN_POINT('Ctrl Pts',(-4.01909342862745,5.74790539005344,
4.46769722706517));
#160280=CARTESIAN_POINT('Ctrl Pts',(-4.16878887486146,5.64028307220609,
4.4760695648964));
#160281=CARTESIAN_POINT('Ctrl Pts',(-4.31407189673789,5.52688069640338,
4.48444190272764));
#160282=CARTESIAN_POINT('Ctrl Pts',(-4.45927688174176,5.41353923320171,
4.49280974346726));
#160283=CARTESIAN_POINT('Ctrl Pts',(-4.60007390954522,5.29442410430156,
4.50117758420688));
#160284=CARTESIAN_POINT('Ctrl Pts',(-4.73599881429248,5.16990732929714,
4.5095454249465));
#160285=CARTESIAN_POINT('Ctrl Pts',(-4.87187062076033,5.04543919605208,
4.51790999683743));
#160286=CARTESIAN_POINT('Ctrl Pts',(-5.00287385753078,4.91557384630014,
4.52627456872838));
#160287=CARTESIAN_POINT('Ctrl Pts',(-5.12857851876306,4.78072263778,4.53463914061932));
#160288=CARTESIAN_POINT('Ctrl Pts',(-5.25425247431509,4.64590436915284,
4.54300166930941));
#160289=CARTESIAN_POINT('Ctrl Pts',(-5.37463021181935,4.50610291102831,
4.5513641979995));
#160290=CARTESIAN_POINT('Ctrl Pts',(-5.48931927309304,4.36176575259944,
4.55972672668959));
#160291=CARTESIAN_POINT('Ctrl Pts',(-5.60401748696586,4.21741707554675,
4.56808992273952));
#160292=CARTESIAN_POINT('Ctrl Pts',(-5.71302590842811,4.0685322286015,4.57645311878946));
#160293=CARTESIAN_POINT('Ctrl Pts',(-5.81599252567112,3.91559159053107,
4.58481631483939));
#160294=CARTESIAN_POINT('Ctrl Pts',(-5.91896616505678,3.76264052217747,
4.59318008124461));
#160295=CARTESIAN_POINT('Ctrl Pts',(-6.01589699478896,3.60563338380146,
4.60154384764983));
#160296=CARTESIAN_POINT('Ctrl Pts',(-6.10647639889291,3.44507946965871,
4.60990761405506));
#160297=CARTESIAN_POINT('Ctrl Pts',(-6.19707405671325,3.28449320041665,
4.61827306594079));
#160298=CARTESIAN_POINT('Ctrl Pts',(-6.28131757511131,3.12035901653803,
4.62663851782652));
#160299=CARTESIAN_POINT('Ctrl Pts',(-6.35894415133984,2.95321110702247,
4.63500396971225));
#160300=CARTESIAN_POINT('Ctrl Pts',(-6.43659672456651,2.78600721997828,
4.64337222317249));
#160301=CARTESIAN_POINT('Ctrl Pts',(-6.50762779842177,2.61578789281798,
4.65174047663273));
#160302=CARTESIAN_POINT('Ctrl Pts',(-6.57182242155123,2.44310798412525,
4.66010873009297));
#160303=CARTESIAN_POINT('Ctrl Pts',(-6.63607656225491,2.2702679765211,4.66848474211806));
#160304=CARTESIAN_POINT('Ctrl Pts',(-6.69348147160369,2.09496313714209,
4.67686075414315));
#160305=CARTESIAN_POINT('Ctrl Pts',(-6.74387147511934,1.91776538960629,
4.68523676616824));
#160306=CARTESIAN_POINT('Ctrl Pts',(-6.79428619051588,1.74048074210371,
4.69361688589321));
#160307=CARTESIAN_POINT('Ctrl Pts',(-6.83767905608054,1.56130165305553,
4.70199700561819));
#160308=CARTESIAN_POINT('Ctrl Pts',(-6.87393525061726,1.38081162104809,
4.71037712534316));
#160309=CARTESIAN_POINT('Ctrl Pts',(-6.91023287244005,1.20011535636002,
4.7187668204144));
#160310=CARTESIAN_POINT('Ctrl Pts',(-6.93937747039207,1.01810547924149,
4.72715651548564));
#160311=CARTESIAN_POINT('Ctrl Pts',(-6.96130576314523,0.835373350365624,
4.73554621055688));
#160312=CARTESIAN_POINT('Ctrl Pts',(-6.97522765034435,0.71935993726033,
4.74087268032504));
#160313=CARTESIAN_POINT('Ctrl Pts',(-6.98624186628859,0.603055503857434,
4.74619915009319));
#160314=CARTESIAN_POINT('Ctrl Pts',(-6.99434311623759,0.486611687939976,
4.75152561986134));
#160315=CARTESIAN_POINT('Ctrl Pts',(-7.00709058383346,0.303385176044988,
4.75990691919134));
#160316=CARTESIAN_POINT('Ctrl Pts',(-7.01264880468849,0.119443890517566,
4.76828821852136));
#160317=CARTESIAN_POINT('Ctrl Pts',(-7.01095217616347,-0.0646231076991999,
4.77666951785137));
#160318=CARTESIAN_POINT('Ctrl Pts',(-7.00925769786622,-0.248456827997147,
4.78504019511396));
#160319=CARTESIAN_POINT('Ctrl Pts',(-7.000326696783,-0.432415618489877,
4.79341087237654));
#160320=CARTESIAN_POINT('Ctrl Pts',(-6.98414535408082,-0.615906028198585,
4.80178154963913));
#160321=CARTESIAN_POINT('Ctrl Pts',(-6.96798237441494,-0.799188207903296,
4.8101427276251));
#160322=CARTESIAN_POINT('Ctrl Pts',(-6.94458548082489,-0.982002741824664,
4.81850390561106));
#160323=CARTESIAN_POINT('Ctrl Pts',(-6.91399287360902,-1.16375646343372,
4.82686508359703));
#160324=CARTESIAN_POINT('Ctrl Pts',(-6.88343996386488,-1.34527433841562,
4.83521541198052));
#160325=CARTESIAN_POINT('Ctrl Pts',(-6.84571001881127,-1.52573382513473,
4.84356574036403));
#160326=CARTESIAN_POINT('Ctrl Pts',(-6.80089297609878,-1.70454723904923,
4.85191606874752));
#160327=CARTESIAN_POINT('Ctrl Pts',(-6.75611041737426,-1.8832230669196,
4.86025997206131));
#160328=CARTESIAN_POINT('Ctrl Pts',(-6.70425170732621,-2.06025502952368,
4.8686038753751));
#160329=CARTESIAN_POINT('Ctrl Pts',(-6.64545797108466,-2.2350648574588,
4.87694777868888));
#160330=CARTESIAN_POINT('Ctrl Pts',(-6.58671145822536,-2.40973427738703,
4.88528498014358));
#160331=CARTESIAN_POINT('Ctrl Pts',(-6.52104113237506,-2.58218481257427,
4.89362218159826));
#160332=CARTESIAN_POINT('Ctrl Pts',(-6.44863819916045,-2.75185245586108,
4.90195938305295));
#160333=CARTESIAN_POINT('Ctrl Pts',(-6.42480349530858,-2.80770624315171,
4.90470395041789));
#160334=CARTESIAN_POINT('Ctrl Pts',(-6.40023958290911,-2.86325857395826,
4.90744851778282));
#160335=CARTESIAN_POINT('Ctrl Pts',(-6.37495445485824,-2.91848972261049,
4.91019308514775));
#160336=CARTESIAN_POINT('Ctrl Pts',(-6.29813533133291,-3.08628829662708,
4.91853139607132));
#160337=CARTESIAN_POINT('Ctrl Pts',(-6.21471876977992,-3.25098310266247,
4.92686970699488));
#160338=CARTESIAN_POINT('Ctrl Pts',(-6.12499220819046,-3.412051730573,4.93520801791844));
#160339=CARTESIAN_POINT('Ctrl Pts',(-6.03520919354579,-3.57322169766318,
4.94355157503799));
#160340=CARTESIAN_POINT('Ctrl Pts',(-5.93910841956194,-3.73076064971087,
4.95189513215755));
#160341=CARTESIAN_POINT('Ctrl Pts',(-5.83702160499504,-3.88417370174419,
4.9602386892771));
#160342=CARTESIAN_POINT('Ctrl Pts',(-5.73485712307548,-4.03770346998288,
4.96858859415072));
#160343=CARTESIAN_POINT('Ctrl Pts',(-5.62669769781581,-4.18710080451296,
4.97693849902432));
#160344=CARTESIAN_POINT('Ctrl Pts',(-5.51291665075828,-4.3319021877568,
4.98528840389795));
#160345=CARTESIAN_POINT('Ctrl Pts',(-5.39896494036342,-4.4769207625976,
4.99365083302468));
#160346=CARTESIAN_POINT('Ctrl Pts',(-5.27937496094569,-4.61732935272852,
5.00201326215141));
#160347=CARTESIAN_POINT('Ctrl Pts',(-5.15455938018053,-4.7526986185422,
5.01037569127813));
#160348=CARTESIAN_POINT('Ctrl Pts',(-5.02963706496323,-4.88818364365719,
5.01874527142949));
#160349=CARTESIAN_POINT('Ctrl Pts',(-4.89948046325721,-5.0186205148773,
5.02711485158085));
#160350=CARTESIAN_POINT('Ctrl Pts',(-4.76453734851883,-5.14361841674411,
5.0354844317322));
#160351=CARTESIAN_POINT('Ctrl Pts',(-4.62938610036217,-5.2688091127423,
5.04386692094771));
#160352=CARTESIAN_POINT('Ctrl Pts',(-4.48943383498774,-5.38854386317103,
5.05224941016321));
#160353=CARTESIAN_POINT('Ctrl Pts',(-4.34516057201549,-5.50247273195443,
5.06063189937873));
#160354=CARTESIAN_POINT('Ctrl Pts',(-4.297952067592,-5.53975206836868,5.06337478306388));
#160355=CARTESIAN_POINT('Ctrl Pts',(-4.25028113534252,-5.57641011894061,
5.06611766674903));
#160356=CARTESIAN_POINT('Ctrl Pts',(-4.20216521516231,-5.61243566261386,
5.06886055043419));
#160357=CARTESIAN_POINT('Ctrl Pts',(-4.05498959952626,-5.72262957657989,
5.07725040546489));
#160358=CARTESIAN_POINT('Ctrl Pts',(-3.90335144205631,-5.82712488836407,
5.08564026049558));
#160359=CARTESIAN_POINT('Ctrl Pts',(-3.74771901562778,-5.92555725163481,
5.09403011552628));
#160360=CARTESIAN_POINT('Ctrl Pts',(-3.59223020465912,-6.02389878287626,
5.10241222851429));
#160361=CARTESIAN_POINT('Ctrl Pts',(-3.43275474896385,-6.1161883439764,
5.1107943415023));
#160362=CARTESIAN_POINT('Ctrl Pts',(-3.26979150759739,-6.20210368015112,
5.11917645449031));
#160363=CARTESIAN_POINT('Ctrl Pts',(-3.10695469120247,-6.28795236421557,
5.12755206473336));
#160364=CARTESIAN_POINT('Ctrl Pts',(-2.94063577338977,-6.36743652951964,
5.13592767497642));
#160365=CARTESIAN_POINT('Ctrl Pts',(-2.77136032177016,-6.44027860650593,
5.14430328521948));
#160366=CARTESIAN_POINT('Ctrl Pts',(-2.60219134695455,-6.51307486473068,
5.15267362707777));
#160367=CARTESIAN_POINT('Ctrl Pts',(-2.43006984759372,-6.57923723553984,
5.16104396893607));
#160368=CARTESIAN_POINT('Ctrl Pts',(-2.25554400260356,-6.63853506542062,
5.16941431079436));
#160369=CARTESIAN_POINT('Ctrl Pts',(-2.08110235345898,-6.69780428847283,
5.17778061458018));
#160370=CARTESIAN_POINT('Ctrl Pts',(-1.90425898244624,-6.75021546896936,
5.18614691836599));
#160371=CARTESIAN_POINT('Ctrl Pts',(-1.72558039697261,-6.7955867190467,
5.19451322215181));
#160372=CARTESIAN_POINT('Ctrl Pts',(-1.54695178291753,-6.8409452800504,
5.20287718611573));
#160373=CARTESIAN_POINT('Ctrl Pts',(-1.36648929574014,-6.8792677543224,
5.21124115007965));
#160374=CARTESIAN_POINT('Ctrl Pts',(-1.1847734369315,-6.91042245203877,
5.21960511404357));
#160375=CARTESIAN_POINT('Ctrl Pts',(-1.00308554118659,-6.94157235556269,
5.22796779093183));
#160376=CARTESIAN_POINT('Ctrl Pts',(-0.820144982198395,-6.96555662617578,
5.23633046782008));
#160377=CARTESIAN_POINT('Ctrl Pts',(-0.636541676327658,-6.98229484172632,
5.24469314470834));
#160378=CARTESIAN_POINT('Ctrl Pts',(-0.452942150520935,-6.99903271266691,
5.25305564942403));
#160379=CARTESIAN_POINT('Ctrl Pts',(-0.268680232367219,-7.00852479657953,
5.26141815413972));
#160380=CARTESIAN_POINT('Ctrl Pts',(-0.0843506078705089,-7.01074258102891,
5.2697806588554));
#160381=CARTESIAN_POINT('Ctrl Pts',(0.0999997914405822,-7.01296061543302,
5.27814410606465));
#160382=CARTESIAN_POINT('Ctrl Pts',(0.28441758368971,-7.00790271241602,
5.28650755327388));
#160383=CARTESIAN_POINT('Ctrl Pts',(0.468307997633091,-6.99559248254591,
5.29487100048313));
#160384=CARTESIAN_POINT('Ctrl Pts',(0.652306691433842,-6.98327500406558,
5.30323937232575));
#160385=CARTESIAN_POINT('Ctrl Pts',(0.835777058075314,-6.96369668652385,
5.31160774416838));
#160386=CARTESIAN_POINT('Ctrl Pts',(1.018128319102,-6.93693313275705,5.319976116011));
#160387=CARTESIAN_POINT('Ctrl Pts',(1.20053421733961,-6.910161559929,5.32834699523687));
#160388=CARTESIAN_POINT('Ctrl Pts',(1.38182001688646,-6.87620051104627,
5.33671787446275));
#160389=CARTESIAN_POINT('Ctrl Pts',(1.56140433386273,-6.83517688642326,
5.34508875368862));
#160390=CARTESIAN_POINT('Ctrl Pts',(1.74114081072128,-6.7941185029193,5.35346672547146));
#160391=CARTESIAN_POINT('Ctrl Pts',(1.91917260488283,-6.74598566497967,
5.36184469725429));
#160392=CARTESIAN_POINT('Ctrl Pts',(2.09493158788415,-6.69095570188484,
5.37022266903713));
#160393=CARTESIAN_POINT('Ctrl Pts',(2.20662788146104,-6.65598370325123,
5.37554693969376));
#160394=CARTESIAN_POINT('Ctrl Pts',(2.31740656455883,-6.61822716054181,
5.38087121035041));
#160395=CARTESIAN_POINT('Ctrl Pts',(2.42712577899576,-6.5777417869231,5.38619548100704));
#160396=CARTESIAN_POINT('Ctrl Pts',(2.58915804863588,-6.51795338059578,
5.39405831217204));
#160397=CARTESIAN_POINT('Ctrl Pts',(2.74921560712769,-6.45208674590007,
5.40192114333703));
#160398=CARTESIAN_POINT('Ctrl Pts',(2.90678976092643,-6.38029778680222,
5.40978397450203));
#160399=CARTESIAN_POINT('Ctrl Pts',(3.06424283978368,-6.30856398804516,
5.41764076411896));
#160400=CARTESIAN_POINT('Ctrl Pts',(3.21921596389816,-6.23091707130824,
5.42549755373589));
#160401=CARTESIAN_POINT('Ctrl Pts',(3.3712172023382,-6.14756221092223,5.43335434335282));
#160402=CARTESIAN_POINT('Ctrl Pts',(3.52313271927187,-6.06425435873344,
5.44120670211217));
#160403=CARTESIAN_POINT('Ctrl Pts',(3.67207935122264,-5.97524514899978,
5.44905906087151));
#160404=CARTESIAN_POINT('Ctrl Pts',(3.81758694489274,-5.8807870630286,5.45691141963085));
#160405=CARTESIAN_POINT('Ctrl Pts',(3.96306018251841,-5.78635127971612,
5.46476192435646));
#160406=CARTESIAN_POINT('Ctrl Pts',(4.10509567386234,-5.68646938107938,
5.47261242908209));
#160407=CARTESIAN_POINT('Ctrl Pts',(4.24324966124329,-5.58143878178904,
5.4804629338077));
#160408=CARTESIAN_POINT('Ctrl Pts',(4.3813814239992,-5.47642507861391,5.48831217563438));
#160409=CARTESIAN_POINT('Ctrl Pts',(4.51563262390902,-5.36626455691305,
5.49616141746104));
#160410=CARTESIAN_POINT('Ctrl Pts',(4.64559057446229,-5.25129648534218,
5.50401065928772));
#160411=CARTESIAN_POINT('Ctrl Pts',(4.77559231039103,-5.13628967877926,
5.51186254567749));
#160412=CARTESIAN_POINT('Ctrl Pts',(4.90129762170006,-5.01647233999805,
5.51971443206726));
#160413=CARTESIAN_POINT('Ctrl Pts',(5.02232871478114,-4.89222248504551,
5.52756631845704));
#160414=CARTESIAN_POINT('Ctrl Pts',(5.11120034255486,-4.80098736042441,
5.53333186106919));
#160415=CARTESIAN_POINT('Ctrl Pts',(5.19755245283155,-4.70736313794122,
5.53909740368134));
#160416=CARTESIAN_POINT('Ctrl Pts',(5.28124885572657,-4.61151136682832,
5.54486294629348));
#160417=CARTESIAN_POINT('Ctrl Pts',(5.42141159660048,-4.45099255727263,
5.55451825078916));
#160418=CARTESIAN_POINT('Ctrl Pts',(5.55405446686134,-4.28430810827498,
5.56417355528482));
#160419=CARTESIAN_POINT('Ctrl Pts',(5.67873381976766,-4.11212946862413,
5.57382885978049));
#160420=CARTESIAN_POINT('Ctrl Pts',(5.80410387309668,-3.93899699133767,
5.58353765286702));
#160421=CARTESIAN_POINT('Ctrl Pts',(5.92142194851332,-3.76030935149879,
5.59324644595356));
#160422=CARTESIAN_POINT('Ctrl Pts',(6.03028522262628,-3.57677042823203,
5.60295523904009));
#160423=CARTESIAN_POINT('Ctrl Pts',(6.13967235620445,-3.39234829983506,
5.6127107516764));
#160424=CARTESIAN_POINT('Ctrl Pts',(6.24052312079776,-3.20302813553686,
5.62246626431272));
#160425=CARTESIAN_POINT('Ctrl Pts',(6.33247728879412,-3.00954447539935,
5.63222177694904));
#160426=CARTESIAN_POINT('Ctrl Pts',(6.42452250558758,-2.8158692366211,5.64198694904626));
#160427=CARTESIAN_POINT('Ctrl Pts',(6.50765349940626,-2.61802229548323,
5.65175212114348));
#160428=CARTESIAN_POINT('Ctrl Pts',(6.58155734801784,-2.41676011164792,
5.6615172932407));
#160429=CARTESIAN_POINT('Ctrl Pts',(6.65536043037557,-2.21577234432387,
5.67126915074296));
#160430=CARTESIAN_POINT('Ctrl Pts',(6.71996149939726,-2.01137867682215,
5.6810210082452));
#160431=CARTESIAN_POINT('Ctrl Pts',(6.77509719585795,-1.80435155919731,
5.69077286574746));
#160432=CARTESIAN_POINT('Ctrl Pts',(6.7991403477887,-1.71407276048134,5.69502538102494));
#160433=CARTESIAN_POINT('Ctrl Pts',(6.82138419463603,-1.62329342927667,
5.69927789630243));
#160434=CARTESIAN_POINT('Ctrl Pts',(6.84180979817911,-1.53207873428241,
5.70353041157991));
#160435=CARTESIAN_POINT('Ctrl Pts',(6.88098123745258,-1.35715068976807,
5.71168572232018));
#160436=CARTESIAN_POINT('Ctrl Pts',(6.91347900255069,-1.18054410539551,
5.71984103306045));
#160437=CARTESIAN_POINT('Ctrl Pts',(6.93916435907318,-1.00280833675662,
5.72799634380073));
#160438=CARTESIAN_POINT('Ctrl Pts',(6.96482790339024,-0.825223502720967,
5.73614472898741));
#160439=CARTESIAN_POINT('Ctrl Pts',(6.98369051605902,-0.646511743554583,
5.74429311417409));
#160440=CARTESIAN_POINT('Ctrl Pts',(6.995664336616,-0.467233401951416,5.75244149936078));
#160441=CARTESIAN_POINT('Ctrl Pts',(7.00599612160768,-0.312540480816032,
5.75947245187736));
#160442=CARTESIAN_POINT('Ctrl Pts',(7.01119974088769,-0.157426046806037,
5.76650340439395));
#160443=CARTESIAN_POINT('Ctrl Pts',(7.01124963752017,-0.002254522849646,
5.77353435691053));
#160444=CARTESIAN_POINT('Ctrl Pts',(7.01125,3.556613210152E-12,5.77353435691053));
#160445=CARTESIAN_POINT('Ctrl Pts',(7.0112499999999,0.191008754743661,5.78220613084263));
#160446=CARTESIAN_POINT('Ctrl Pts',(7.00344012880999,0.382017367486429,
5.79087790477474));
#160447=CARTESIAN_POINT('Ctrl Pts',(6.98784644419152,0.572388534913077,
5.79954967870684));
#160448=CARTESIAN_POINT('Ctrl Pts',(6.97225169663171,0.762772678963806,
5.8082220437492));
#160449=CARTESIAN_POINT('Ctrl Pts',(6.94887209704284,0.952519007630189,
5.81689440879155));
#160450=CARTESIAN_POINT('Ctrl Pts',(6.91778566246054,1.14099434299889,5.82556677383391));
#160451=CARTESIAN_POINT('Ctrl Pts',(6.88670108297145,1.32945843103985,5.83423862135003));
#160452=CARTESIAN_POINT('Ctrl Pts',(6.84791063501108,1.51665139731098,5.84291046886614));
#160453=CARTESIAN_POINT('Ctrl Pts',(6.80154374572927,1.70194865887049,5.85158231638226));
#160454=CARTESIAN_POINT('Ctrl Pts',(6.75517597619852,1.88724943819281,5.86025432852846));
#160455=CARTESIAN_POINT('Ctrl Pts',(6.70123154646085,2.07065416525472,5.86892634067466));
#160456=CARTESIAN_POINT('Ctrl Pts',(6.6398904528553,2.25155087363823,5.87759835282085));
#160457=CARTESIAN_POINT('Ctrl Pts',(6.61790934153639,2.31637382429788,5.88070590198798));
#160458=CARTESIAN_POINT('Ctrl Pts',(6.59497889661513,2.38087486019071,5.88381345115511));
#160459=CARTESIAN_POINT('Ctrl Pts',(6.57110895151814,2.44502632087637,5.88692100032223));
#160460=CARTESIAN_POINT('',(7.01124988024546,0.00129586190515713,5.22646564305715));
#160461=CARTESIAN_POINT('Ctrl Pts',(6.57110895151813,2.44502632087638,5.33975062352347));
#160462=CARTESIAN_POINT('Ctrl Pts',(6.63727736514693,2.26719598367653,5.33111643416571));
#160463=CARTESIAN_POINT('Ctrl Pts',(6.6962654193017,2.08656392115047,5.32248224480796));
#160464=CARTESIAN_POINT('Ctrl Pts',(6.74784989526467,1.90371960999422,5.3138480554502));
#160465=CARTESIAN_POINT('Ctrl Pts',(6.79935992125682,1.72113919128581,5.30522632749937));
#160466=CARTESIAN_POINT('Ctrl Pts',(6.84348761691352,1.53635317540665,5.29660459954852));
#160467=CARTESIAN_POINT('Ctrl Pts',(6.88005927097208,1.34996703308311,5.28798287159768));
#160468=CARTESIAN_POINT('Ctrl Pts',(6.91659744670839,1.1637515118456,5.27936903612517));
#160469=CARTESIAN_POINT('Ctrl Pts',(6.94559332009529,0.975939069717269,
5.27075520065265));
#160470=CARTESIAN_POINT('Ctrl Pts',(6.96692361721662,0.78714793677513,5.26214136518013));
#160471=CARTESIAN_POINT('Ctrl Pts',(6.98822860751318,0.598580790591932,
5.25353774938826));
#160472=CARTESIAN_POINT('Ctrl Pts',(7.00188613807103,0.409037558786854,
5.24493413359641));
#160473=CARTESIAN_POINT('Ctrl Pts',(7.00782436062502,0.219144457220791,
5.23633051780455));
#160474=CARTESIAN_POINT('Ctrl Pts',(7.0100939421181,0.146567542991075,5.23304222623291));
#160475=CARTESIAN_POINT('Ctrl Pts',(7.01123645377904,0.0739396047210392,
5.22975393466127));
#160476=CARTESIAN_POINT('Ctrl Pts',(7.01124988024532,0.00129586262259841,
5.22646564308963));
#160477=CARTESIAN_POINT('Ctrl Pts',(7.01124988024546,0.00129586190516873,
5.22646564305716));
#160478=CARTESIAN_POINT('Ctrl Pts',(7.01128652420434,-0.196965967775037,
5.21749112323366));
#160479=CARTESIAN_POINT('Ctrl Pts',(7.00290926625389,-0.395057195486619,
5.20851660341015));
#160480=CARTESIAN_POINT('Ctrl Pts',(6.98618743385599,-0.592293594033082,
5.19954208358664));
#160481=CARTESIAN_POINT('Ctrl Pts',(6.96943444002355,-0.789897546145331,
5.19055083958451));
#160482=CARTESIAN_POINT('Ctrl Pts',(6.94430580230218,-0.986643262615029,
5.18155959558237));
#160483=CARTESIAN_POINT('Ctrl Pts',(6.91092245162695,-1.18185338773412,
5.17256835158023));
#160484=CARTESIAN_POINT('Ctrl Pts',(6.87746142153865,-1.37751774550624,
5.16355618593474));
#160485=CARTESIAN_POINT('Ctrl Pts',(6.83570728321723,-1.57163914238257,
5.15454402028925));
#160486=CARTESIAN_POINT('Ctrl Pts',(6.78583228453984,-1.76354948005347,
5.14553185464376));
#160487=CARTESIAN_POINT('Ctrl Pts',(6.73590749769426,-1.95565139395338,
5.13651069252246));
#160488=CARTESIAN_POINT('Ctrl Pts',(6.6778457133722,-2.14553762481288,5.12748953040116));
#160489=CARTESIAN_POINT('Ctrl Pts',(6.61186906878772,-2.33255524687159,
5.11846836827986));
#160490=CARTESIAN_POINT('Ctrl Pts',(6.54581642848924,-2.51978828664077,
5.10943681506243));
#160491=CARTESIAN_POINT('Ctrl Pts',(6.47183077497929,-2.70414590213013,
5.100405261845));
#160492=CARTESIAN_POINT('Ctrl Pts',(6.39018315943529,-2.884993197803,5.09137370862757));
#160493=CARTESIAN_POINT('Ctrl Pts',(6.3479506085923,-2.97853717405308,5.08670210214029));
#160494=CARTESIAN_POINT('Ctrl Pts',(6.30366886474925,-3.07114230857741,
5.082030495653));
#160495=CARTESIAN_POINT('Ctrl Pts',(6.25738035770964,-3.16272313385943,
5.07735888916572));
#160496=CARTESIAN_POINT('Ctrl Pts',(6.17947165912919,-3.31686383462863,
5.06949605657549));
#160497=CARTESIAN_POINT('Ctrl Pts',(6.09575013385041,-3.4683483313541,5.06163322398526));
#160498=CARTESIAN_POINT('Ctrl Pts',(6.00642878203436,-3.61668907273617,
5.05377039139503));
#160499=CARTESIAN_POINT('Ctrl Pts',(5.91717606189674,-3.76491583382291,
5.04591360035463));
#160500=CARTESIAN_POINT('Ctrl Pts',(5.8223322672198,-3.9100033187394,5.03805680931422));
#160501=CARTESIAN_POINT('Ctrl Pts',(5.72215743083715,-4.05148625805583,
5.03020001827382));
#160502=CARTESIAN_POINT('Ctrl Pts',(5.62203908833992,-4.19288940766408,
5.0223476580932));
#160503=CARTESIAN_POINT('Ctrl Pts',(5.51659590430043,-4.3306917451642,5.01449529791258));
#160504=CARTESIAN_POINT('Ctrl Pts',(5.40613242074016,-4.46445504086693,
5.00664293773195));
#160505=CARTESIAN_POINT('Ctrl Pts',(5.29569501897807,-4.59818675339694,
4.99879243159093));
#160506=CARTESIAN_POINT('Ctrl Pts',(5.1802399129313,-4.72788102310245,4.99094192544991));
#160507=CARTESIAN_POINT('Ctrl Pts',(5.06011326814566,-4.85313097660019,
4.98309141930889));
#160508=CARTESIAN_POINT('Ctrl Pts',(4.9400059479837,-4.97836078129396,4.97524217606901));
#160509=CARTESIAN_POINT('Ctrl Pts',(4.81522885136987,-5.09914741976571,
4.96739293282913));
#160510=CARTESIAN_POINT('Ctrl Pts',(4.68616617399064,-5.21511966806572,
4.95954368958925));
#160511=CARTESIAN_POINT('Ctrl Pts',(4.55706001301264,-5.33113098955728,
4.95169180179441));
#160512=CARTESIAN_POINT('Ctrl Pts',(4.4236656712221,-5.44232442568857,4.94383991399956));
#160513=CARTESIAN_POINT('Ctrl Pts',(4.28640185157114,-5.54836784373094,
4.93598802620472));
#160514=CARTESIAN_POINT('Ctrl Pts',(4.18561090107159,-5.62623407917368,
4.93022249209624));
#160515=CARTESIAN_POINT('Ctrl Pts',(4.08273435008407,-5.7013243541646,4.92445695798776));
#160516=CARTESIAN_POINT('Ctrl Pts',(3.97794824856842,-5.77352182763791,
4.91869142387928));
#160517=CARTESIAN_POINT('Ctrl Pts',(3.802467499896,-5.894427811486,4.90903613346177));
#160518=CARTESIAN_POINT('Ctrl Pts',(3.62172062104522,-6.00715877938123,
4.89938084304426));
#160519=CARTESIAN_POINT('Ctrl Pts',(3.43642534724975,-6.11135070138177,
4.88972555262675));
#160520=CARTESIAN_POINT('Ctrl Pts',(3.25010359379651,-6.21611981505184,
4.88001677482664));
#160521=CARTESIAN_POINT('Ctrl Pts',(3.05918298030223,-6.31225503789554,
4.87030799702654));
#160522=CARTESIAN_POINT('Ctrl Pts',(2.8644087958511,-6.39943660119787,4.86059921922643));
#160523=CARTESIAN_POINT('Ctrl Pts',(2.66869735532569,-6.48703768339075,
4.85084372265302));
#160524=CARTESIAN_POINT('Ctrl Pts',(2.46909521703533,-6.5655987326719,4.84108822607961));
#160525=CARTESIAN_POINT('Ctrl Pts',(2.2663732636386,-6.63484580019492,4.83133272950621));
#160526=CARTESIAN_POINT('Ctrl Pts',(2.06345058237605,-6.70416143363221,
4.8215675733968));
#160527=CARTESIAN_POINT('Ctrl Pts',(1.85740194694757,-6.76414463665865,
4.81180241728738));
#160528=CARTESIAN_POINT('Ctrl Pts',(1.64901461157417,-6.81457096032574,
4.80203726117797));
#160529=CARTESIAN_POINT('Ctrl Pts',(1.44091138821088,-6.86492853353756,
4.79228541872856));
#160530=CARTESIAN_POINT('Ctrl Pts',(1.23047587455813,-6.90575526019108,
4.78253357627916));
#160531=CARTESIAN_POINT('Ctrl Pts',(1.01850554823742,-6.93687775665029,
4.77278173382975));
#160532=CARTESIAN_POINT('Ctrl Pts',(0.926069348134061,-6.95044968136426,
4.76852914208412));
#160533=CARTESIAN_POINT('Ctrl Pts',(0.833341447452034,-6.96217683157803,
4.76427655033848));
#160534=CARTESIAN_POINT('Ctrl Pts',(0.740388755513583,-6.97204783784571,
4.76002395859285));
#160535=CARTESIAN_POINT('Ctrl Pts',(0.56480297425954,-6.99069397182128,
4.75199089759764));
#160536=CARTESIAN_POINT('Ctrl Pts',(0.388329000813756,-7.00272228021521,
4.74395783660243));
#160537=CARTESIAN_POINT('Ctrl Pts',(0.211513544990063,-7.00805883128743,
4.73592477560721));
#160538=CARTESIAN_POINT('Ctrl Pts',(0.0348117535483582,-7.01339195180107,
4.72789687860011));
#160539=CARTESIAN_POINT('Ctrl Pts',(-0.142230718440287,-7.01204186670302,
4.71986898159302));
#160540=CARTESIAN_POINT('Ctrl Pts',(-0.319061895795209,-7.00398644124556,
4.71184108458592));
#160541=CARTESIAN_POINT('Ctrl Pts',(-0.495813231268391,-6.99593465293136,
4.70381681229259));
#160542=CARTESIAN_POINT('Ctrl Pts',(-0.672353096637324,-6.9811835691244,
4.69579253999928));
#160543=CARTESIAN_POINT('Ctrl Pts',(-0.848129418575118,-6.95976314624625,
4.68776826770595));
#160544=CARTESIAN_POINT('Ctrl Pts',(-1.02388448507122,-6.93834531359495,
4.67974496573359));
#160545=CARTESIAN_POINT('Ctrl Pts',(-1.19887582744569,-6.91025978490329,
4.67172166376123));
#160546=CARTESIAN_POINT('Ctrl Pts',(-1.3725562172269,-6.87558841067816,
4.66369836178887));
#160547=CARTESIAN_POINT('Ctrl Pts',(-1.54622237433824,-6.84091987768469,
4.65567571730588));
#160548=CARTESIAN_POINT('Ctrl Pts',(-1.71857743408248,-6.7996666498913,
4.64765307282289));
#160549=CARTESIAN_POINT('Ctrl Pts',(-1.88908438820088,-6.75196169544494,
4.6396304283399));
#160550=CARTESIAN_POINT('Ctrl Pts',(-2.05965543780748,-6.70423880816786,
4.63160476805431));
#160551=CARTESIAN_POINT('Ctrl Pts',(-2.22837664152133,-6.65005945106735,
4.62357910776871));
#160552=CARTESIAN_POINT('Ctrl Pts',(-2.39472581274701,-6.58960657735067,
4.61555344748312));
#160553=CARTESIAN_POINT('Ctrl Pts',(-2.49281334188007,-6.55396063473387,
4.61082112942422));
#160554=CARTESIAN_POINT('Ctrl Pts',(-2.59007646853187,-6.51613441841434,
4.60608881136533));
#160555=CARTESIAN_POINT('Ctrl Pts',(-2.6864113892892,-6.4761732844325,4.60135649330643));
#160556=CARTESIAN_POINT('Ctrl Pts',(-2.864126479334,-6.40245446608456,4.59262648840947));
#160557=CARTESIAN_POINT('Ctrl Pts',(-3.03877054673932,-6.32143101450485,
4.58389648351253));
#160558=CARTESIAN_POINT('Ctrl Pts',(-3.20976034755821,-6.23338311623335,
4.57516647861559));
#160559=CARTESIAN_POINT('Ctrl Pts',(-3.38079958204756,-6.1453097630472,
4.56643394984773));
#160560=CARTESIAN_POINT('Ctrl Pts',(-3.54818219764428,-6.05020803502009,
4.55770142107988));
#160561=CARTESIAN_POINT('Ctrl Pts',(-3.71134950974166,-5.94840410354243,
4.54896889231202));
#160562=CARTESIAN_POINT('Ctrl Pts',(-3.87683612734117,-5.84515310270155,
4.54011223695435));
#160563=CARTESIAN_POINT('Ctrl Pts',(-4.03798644674918,-5.73500806499387,
4.53125558159669));
#160564=CARTESIAN_POINT('Ctrl Pts',(-4.19424763424862,-5.61835503907504,
4.52239892623902));
#160565=CARTESIAN_POINT('Ctrl Pts',(-4.34841689211665,-5.50326369283764,
4.5136608383905));
#160566=CARTESIAN_POINT('Ctrl Pts',(-4.49782690134713,-5.38183771029516,
4.50492275054197));
#160567=CARTESIAN_POINT('Ctrl Pts',(-4.64197892218068,-5.2544893423177,
4.49618466269344));
#160568=CARTESIAN_POINT('Ctrl Pts',(-4.78906495094792,-5.12454898069474,
4.4872687235812));
#160569=CARTESIAN_POINT('Ctrl Pts',(-4.93067643526651,-4.98844275983394,
4.47835278446896));
#160570=CARTESIAN_POINT('Ctrl Pts',(-5.06632123745495,-4.84664994417928,
4.46943684535672));
#160571=CARTESIAN_POINT('Ctrl Pts',(-5.20196603964339,-4.70485712852462,
4.46052090624448));
#160572=CARTESIAN_POINT('Ctrl Pts',(-5.33164395503506,-4.55737794082467,
4.45160496713224));
#160573=CARTESIAN_POINT('Ctrl Pts',(-5.45490408292047,-4.40473018567967,
4.44268902802));
#160574=CARTESIAN_POINT('Ctrl Pts',(-5.57574224718921,-4.2550818376866,
4.43394828003006));
#160575=CARTESIAN_POINT('Ctrl Pts',(-5.69042532874889,-4.10045025632596,
4.4252075320401));
#160576=CARTESIAN_POINT('Ctrl Pts',(-5.79856547132975,-3.94135319873803,
4.41646678405016));
#160577=CARTESIAN_POINT('Ctrl Pts',(-5.90668616011713,-3.78228476180128,
4.40772760847081));
#160578=CARTESIAN_POINT('Ctrl Pts',(-6.00826610670791,-3.61875267926487,
4.39898843289146));
#160579=CARTESIAN_POINT('Ctrl Pts',(-6.10296041194863,-3.4513042132921,
4.39024925731211));
#160580=CARTESIAN_POINT('Ctrl Pts',(-6.19888057478418,-3.28168805652492,
4.38139694943056));
#160581=CARTESIAN_POINT('Ctrl Pts',(-6.28773541961175,-3.10805364858808,
4.37254464154902));
#160582=CARTESIAN_POINT('Ctrl Pts',(-6.36921354941784,-2.93099732589646,
4.36369233366747));
#160583=CARTESIAN_POINT('Ctrl Pts',(-6.44960915198586,-2.75629339264287,
4.35495763850513));
#160584=CARTESIAN_POINT('Ctrl Pts',(-6.52282273410569,-2.57825816930568,
4.34622294334278));
#160585=CARTESIAN_POINT('Ctrl Pts',(-6.58860235168398,-2.39748735426996,
4.33748824818043));
#160586=CARTESIAN_POINT('Ctrl Pts',(-6.65571055363997,-2.21306541918152,
4.32857713393929));
#160587=CARTESIAN_POINT('Ctrl Pts',(-6.71508118046617,-2.02579647754138,
4.31966601969815));
#160588=CARTESIAN_POINT('Ctrl Pts',(-6.76649883806085,-1.83633331315999,
4.31075490545701));
#160589=CARTESIAN_POINT('Ctrl Pts',(-6.81791649565554,-1.6468701487786,
4.30184379121587));
#160590=CARTESIAN_POINT('Ctrl Pts',(-6.86138109162614,-1.4552130506391,
4.29293267697472));
#160591=CARTESIAN_POINT('Ctrl Pts',(-6.89673142008012,-1.26203101458707,
4.28402156273358));
#160592=CARTESIAN_POINT('Ctrl Pts',(-6.92856904036456,-1.08804518252878,
4.27599593231008));
#160593=CARTESIAN_POINT('Ctrl Pts',(-6.95383899451739,-0.912742376751788,
4.26797030188659));
#160594=CARTESIAN_POINT('Ctrl Pts',(-6.97244213013839,-0.736666345349977,
4.2599446714631));
#160595=CARTESIAN_POINT('Ctrl Pts',(-6.99103936169988,-0.560646195031204,
4.25192158812632));
#160596=CARTESIAN_POINT('Ctrl Pts',(-7.00297394870145,-0.383853671762903,
4.24389850478953));
#160597=CARTESIAN_POINT('Ctrl Pts',(-7.0081983319312,-0.206839799885826,
4.23587542145275));
#160598=CARTESIAN_POINT('Ctrl Pts',(-7.01342205637091,-0.0298482492990209,
4.22785334981958));
#160599=CARTESIAN_POINT('Ctrl Pts',(-7.01193725225357,0.147364227971745,
4.21983127818641));
#160600=CARTESIAN_POINT('Ctrl Pts',(-7.00374843033031,0.324244486685203,
4.21180920655323));
#160601=CARTESIAN_POINT('Ctrl Pts',(-6.99555656518028,0.501190479730516,
4.203784153663));
#160602=CARTESIAN_POINT('Ctrl Pts',(-6.9806557191138,0.67780364091553,4.19575910077279));
#160603=CARTESIAN_POINT('Ctrl Pts',(-6.95910248079907,0.853533376170037,
4.18773404788256));
#160604=CARTESIAN_POINT('Ctrl Pts',(-6.93754499739822,1.02929772282963,
4.17970741439269));
#160605=CARTESIAN_POINT('Ctrl Pts',(-6.90933256489879,1.20417793415915,
4.1716807809028));
#160606=CARTESIAN_POINT('Ctrl Pts',(-6.87457325192067,1.37763172382061,
4.16365414741293));
#160607=CARTESIAN_POINT('Ctrl Pts',(-6.83978603290037,1.55122476850053,
4.15562106984942));
#160608=CARTESIAN_POINT('Ctrl Pts',(-6.7984415168326,1.72338874676363,4.14758799228592));
#160609=CARTESIAN_POINT('Ctrl Pts',(-6.75069833517884,1.89359408266756,
4.1395549147224));
#160610=CARTESIAN_POINT('Ctrl Pts',(-6.72256498307134,1.9938900093255,4.13482130896399));
#160611=CARTESIAN_POINT('Ctrl Pts',(-6.69221075140437,2.09350612363944,
4.13008770320556));
#160612=CARTESIAN_POINT('Ctrl Pts',(-6.65967601729574,2.19233708793971,
4.12535409744714));
#160613=CARTESIAN_POINT('Ctrl Pts',(-6.59265675514161,2.39592191771794,
4.11560320278182));
#160614=CARTESIAN_POINT('Ctrl Pts',(-6.51634348769467,2.59629432247953,
4.10585230811651));
#160615=CARTESIAN_POINT('Ctrl Pts',(-6.43105328435768,2.79270124006353,
4.09610141345119));
#160616=CARTESIAN_POINT('Ctrl Pts',(-6.34564023879427,2.98939103964446,
4.08633647471558));
#160617=CARTESIAN_POINT('Ctrl Pts',(-6.25122441024143,3.18210389205048,
4.07657153597996));
#160618=CARTESIAN_POINT('Ctrl Pts',(-6.14817084124316,3.37010710058113,
4.06680659724435));
#160619=CARTESIAN_POINT('Ctrl Pts',(-6.0452890566934,3.55779691843731,4.0570579361072));
#160620=CARTESIAN_POINT('Ctrl Pts',(-5.93379832692504,3.7407927495352,4.04730927497005));
#160621=CARTESIAN_POINT('Ctrl Pts',(-5.81410786029961,3.91838950990101,
4.03756061383289));
#160622=CARTESIAN_POINT('Ctrl Pts',(-5.6947458817172,4.0954988595824,4.02783870769728));
#160623=CARTESIAN_POINT('Ctrl Pts',(-5.56722911418537,4.26723868639639,
4.01811680156166));
#160624=CARTESIAN_POINT('Ctrl Pts',(-5.4320089959831,4.43293411072832,4.00839489542604));
#160625=CARTESIAN_POINT('Ctrl Pts',(-5.29768353520315,4.59753324374508,
3.99873731237784));
#160626=CARTESIAN_POINT('Ctrl Pts',(-5.15575632941792,4.75616763870949,
3.98907972932964));
#160627=CARTESIAN_POINT('Ctrl Pts',(-5.00671485939788,4.9082005744656,3.97942214628144));
#160628=CARTESIAN_POINT('Ctrl Pts',(-4.94120089189194,4.97502949672207,
3.97517697490786));
#160629=CARTESIAN_POINT('Ctrl Pts',(-4.87431288738266,5.04058320983856,
3.97093180353428));
#160630=CARTESIAN_POINT('Ctrl Pts',(-4.80609502587596,5.10480921923144,
3.9666866321607));
#160631=CARTESIAN_POINT('Ctrl Pts',(-4.67991776677176,5.22360306074756,
3.95883466969053));
#160632=CARTESIAN_POINT('Ctrl Pts',(-4.54924017819576,5.33780310879715,
3.95098270722035));
#160633=CARTESIAN_POINT('Ctrl Pts',(-4.41444929813602,5.44704176197378,
3.94313074475017));
#160634=CARTESIAN_POINT('Ctrl Pts',(-4.27969663339582,5.55624944428624,
3.93528100843398));
#160635=CARTESIAN_POINT('Ctrl Pts',(-4.14083329296949,5.66049828982512,
3.92743127211779));
#160636=CARTESIAN_POINT('Ctrl Pts',(-3.99828058058831,5.75945995397055,
3.9195815358016));
#160637=CARTESIAN_POINT('Ctrl Pts',(-3.85573923930518,5.85841372417438,
3.9117324256406));
#160638=CARTESIAN_POINT('Ctrl Pts',(-3.70950942570064,5.95208093565143,
3.9038833154796));
#160639=CARTESIAN_POINT('Ctrl Pts',(-3.56004247386272,6.04017583740684,
3.89603420531861));
#160640=CARTESIAN_POINT('Ctrl Pts',(-3.41049984156261,6.12831534476102,
3.88818112087248));
#160641=CARTESIAN_POINT('Ctrl Pts',(-3.25771712511903,6.21087671103691,
3.88032803642635));
#160642=CARTESIAN_POINT('Ctrl Pts',(-3.10217167427491,6.28761937984691,
3.87247495198022));
#160643=CARTESIAN_POINT('Ctrl Pts',(-2.94658671212205,6.3643815426586,3.86461987271108));
#160644=CARTESIAN_POINT('Ctrl Pts',(-2.78823796560874,6.43532190740176,
3.85676479344193));
#160645=CARTESIAN_POINT('Ctrl Pts',(-2.62762332414846,6.50024785903515,
3.84890971417279));
#160646=CARTESIAN_POINT('Ctrl Pts',(-2.46684925761971,6.56523825575394,
3.84104683800208));
#160647=CARTESIAN_POINT('Ctrl Pts',(-2.30380516265391,6.62420218634343,
3.83318396183138));
#160648=CARTESIAN_POINT('Ctrl Pts',(-2.13900521393938,6.6769965746015,3.82532108566067));
#160649=CARTESIAN_POINT('Ctrl Pts',(-2.01812682852617,6.71572049691636,
3.81955377939854));
#160650=CARTESIAN_POINT('Ctrl Pts',(-1.8963041239431,6.75112623947487,3.81378647313642));
#160651=CARTESIAN_POINT('Ctrl Pts',(-1.77374330284059,6.78317486566049,
3.80801916687429));
#160652=CARTESIAN_POINT('Ctrl Pts',(-1.5957060076044,6.82973012427246,3.79964132150356));
#160653=CARTESIAN_POINT('Ctrl Pts',(-1.41571643005527,6.86930273055416,
3.7912634761328));
#160654=CARTESIAN_POINT('Ctrl Pts',(-1.23434857655566,6.90173964693359,
3.78288563076206));
#160655=CARTESIAN_POINT('Ctrl Pts',(-1.05310478568828,6.93415437520664,
3.77451351616185));
#160656=CARTESIAN_POINT('Ctrl Pts',(-0.870484921105781,6.95944308732074,
3.76614140156164));
#160657=CARTESIAN_POINT('Ctrl Pts',(-0.687074608834716,6.97750349655195,
3.75776928696143));
#160658=CARTESIAN_POINT('Ctrl Pts',(-0.503762847088566,6.99555420151523,
3.74940167088847));
#160659=CARTESIAN_POINT('Ctrl Pts',(-0.319661810952985,7.00638431563537,
3.74103405481551));
#160660=CARTESIAN_POINT('Ctrl Pts',(-0.135364160697066,7.00994316000485,
3.73266643874256));
#160661=CARTESIAN_POINT('Ctrl Pts',(0.0488614725731419,7.01350061370416,
3.7243020924372));
#160662=CARTESIAN_POINT('Ctrl Pts',(0.233283238559968,7.00979245737618,
3.71593774613184));
#160663=CARTESIAN_POINT('Ctrl Pts',(0.417306087178902,6.99882005713131,
3.70757339982649));
#160664=CARTESIAN_POINT('Ctrl Pts',(0.601283974752137,6.98785033769804,
3.69921109712475));
#160665=CARTESIAN_POINT('Ctrl Pts',(0.784862811510427,6.9696199337488,3.69084879442301));
#160666=CARTESIAN_POINT('Ctrl Pts',(0.967449822494202,6.94418227032211,
3.68248649172126));
#160667=CARTESIAN_POINT('Ctrl Pts',(1.15005142104003,6.91874257458496,3.67412352092375));
#160668=CARTESIAN_POINT('Ctrl Pts',(1.33166070911257,6.88609450834275,3.66576055012623));
#160669=CARTESIAN_POINT('Ctrl Pts',(1.51169152188426,6.84634320679027,3.65739757932871));
#160670=CARTESIAN_POINT('Ctrl Pts',(1.69173462933279,6.80658919053913,3.64903403740661));
#160671=CARTESIAN_POINT('Ctrl Pts',(1.87019872536886,6.75973104238083,3.64067049548451));
#160672=CARTESIAN_POINT('Ctrl Pts',(2.04650913219775,6.70592476354539,3.63230695356241));
#160673=CARTESIAN_POINT('Ctrl Pts',(2.22285509621616,6.65210763339329,3.62394172493303));
#160674=CARTESIAN_POINT('Ctrl Pts',(2.39704619044741,6.59133967441651,3.61557649630364));
#160675=CARTESIAN_POINT('Ctrl Pts',(2.56852374778743,6.5238265090016,3.60721126767427));
#160676=CARTESIAN_POINT('Ctrl Pts',(2.7400587687183,6.45629071934959,3.59884323578549));
#160677=CARTESIAN_POINT('Ctrl Pts',(2.90887813370036,6.38200533641811,3.59047520389672));
#160678=CARTESIAN_POINT('Ctrl Pts',(3.07444357628501,6.30122394926096,3.58210717200794));
#160679=CARTESIAN_POINT('Ctrl Pts',(3.24016260788494,6.22036762416076,3.57373137740155));
#160680=CARTESIAN_POINT('Ctrl Pts',(3.4026213893167,6.13300339721256,3.56535558279515));
#160681=CARTESIAN_POINT('Ctrl Pts',(3.56130557270496,6.0394311967536,3.55697978818876));
#160682=CARTESIAN_POINT('Ctrl Pts',(3.72006762203486,5.94581308064417,3.54859988360038));
#160683=CARTESIAN_POINT('Ctrl Pts',(3.87505109997757,5.84598108878888,3.540219979012));
#160684=CARTESIAN_POINT('Ctrl Pts',(4.02577050542334,5.7402785995249,3.53184007442363));
#160685=CARTESIAN_POINT('Ctrl Pts',(4.17666223258766,5.63445525764376,3.52345058885558));
#160686=CARTESIAN_POINT('Ctrl Pts',(4.32327988002905,5.52274820075145,3.51506110328756));
#160687=CARTESIAN_POINT('Ctrl Pts',(4.46516985074383,5.4055420418778,3.50667161771951));
#160688=CARTESIAN_POINT('Ctrl Pts',(4.55530048957808,5.33109093077125,3.50134249058015));
#160689=CARTESIAN_POINT('Ctrl Pts',(4.64352420715157,5.25442173762314,3.49601336344078));
#160690=CARTESIAN_POINT('Ctrl Pts',(4.72973243973347,5.17564079231093,3.49068423630143));
#160691=CARTESIAN_POINT('Ctrl Pts',(4.86533391691881,5.05172208711947,3.48230177107087));
#160692=CARTESIAN_POINT('Ctrl Pts',(4.99622050371155,4.92232668016906,3.4739193058403));
#160693=CARTESIAN_POINT('Ctrl Pts',(5.12193835131295,4.78783605482159,3.46553684060975));
#160694=CARTESIAN_POINT('Ctrl Pts',(5.24749632646853,4.65351645805617,3.45716503516414));
#160695=CARTESIAN_POINT('Ctrl Pts',(5.36789843988125,4.51411479332084,3.44879322971853));
#160696=CARTESIAN_POINT('Ctrl Pts',(5.48272532811655,4.37005143435741,3.44042142427291));
#160697=CARTESIAN_POINT('Ctrl Pts',(5.59771704647468,4.2257812773041,3.43203760138312));
#160698=CARTESIAN_POINT('Ctrl Pts',(5.70711726478799,4.07683624319286,3.42365377849332));
#160699=CARTESIAN_POINT('Ctrl Pts',(5.81054159026457,3.92367595378437,3.41526995560352));
#160700=CARTESIAN_POINT('Ctrl Pts',(5.91356675244229,3.77110678224002,3.40691848984428));
#160701=CARTESIAN_POINT('Ctrl Pts',(6.01066186247285,3.61435509316714,3.39856702408504));
#160702=CARTESIAN_POINT('Ctrl Pts',(6.10148678868888,3.45390873214031,3.39021555832579));
#160703=CARTESIAN_POINT('Ctrl Pts',(6.19283955649819,3.29252991494346,3.38181555687072));
#160704=CARTESIAN_POINT('Ctrl Pts',(6.27784880476541,3.12741359563608,3.37341555541566));
#160705=CARTESIAN_POINT('Ctrl Pts',(6.35621222836559,2.95908645876996,3.36501555396059));
#160706=CARTESIAN_POINT('Ctrl Pts',(6.43457565196577,2.79075932190384,3.35661555250552));
#160707=CARTESIAN_POINT('Ctrl Pts',(6.50629307529157,2.61922165809476,3.34821555105044));
#160708=CARTESIAN_POINT('Ctrl Pts',(6.57110895151814,2.44502632087637,3.33981554959537));
#160709=CARTESIAN_POINT('Origin',(0.,0.,50.));
#160710=CARTESIAN_POINT('',(6.57110895151814,2.44502632087636,1.34015432832236));
#160711=CARTESIAN_POINT('',(6.57110895151814,2.44502632087635,1.88679067599786));
#160712=CARTESIAN_POINT('',(6.57110895151814,2.44502632087636,50.));
#160713=CARTESIAN_POINT('',(7.01124672537777,0.00677631016985116,1.22646564305006));
#160714=CARTESIAN_POINT('Ctrl Pts',(6.57110895151814,2.44502632087636,1.34015432832236));
#160715=CARTESIAN_POINT('Ctrl Pts',(6.63376189300869,2.27664395985542,1.33198913246426));
#160716=CARTESIAN_POINT('Ctrl Pts',(6.68988070270378,2.10600776687022,1.32382393660616));
#160717=CARTESIAN_POINT('Ctrl Pts',(6.73932882506234,1.93366841784827,1.31565874074806));
#160718=CARTESIAN_POINT('Ctrl Pts',(6.78885956678129,1.76104111923176,1.30747990224335));
#160719=CARTESIAN_POINT('Ctrl Pts',(6.8316972634231,1.58670532059054,1.29930106373863));
#160720=CARTESIAN_POINT('Ctrl Pts',(6.86775650424132,1.41122186808137,1.29112222523392));
#160721=CARTESIAN_POINT('Ctrl Pts',(6.8997684057998,1.25543492195056,1.28386139091976));
#160722=CARTESIAN_POINT('Ctrl Pts',(6.92643882991178,1.09874375883881,1.27660055660559));
#160723=CARTESIAN_POINT('Ctrl Pts',(6.94774241808982,0.94154227434327,1.26933972229143));
#160724=CARTESIAN_POINT('Ctrl Pts',(6.9896738586244,0.632125633165928,1.2550483625575));
#160725=CARTESIAN_POINT('Ctrl Pts',(7.01094414743398,0.319844675254871,
1.24075700282355));
#160726=CARTESIAN_POINT('Ctrl Pts',(7.01124672537693,0.00677631103669551,
1.22646564308963));
#160727=CARTESIAN_POINT('',(-5.31037376991255,4.57794244025903,0.));
#160728=CARTESIAN_POINT('Ctrl Pts',(7.01124672537777,0.00677631016984748,
1.22646564305006));
#160729=CARTESIAN_POINT('Ctrl Pts',(7.01141682993229,-0.169225816498521,
1.21843126464065));
#160730=CARTESIAN_POINT('Ctrl Pts',(7.00495567967284,-0.345511762794221,
1.21039688623124));
#160731=CARTESIAN_POINT('Ctrl Pts',(6.99182592907262,-0.52153306707037,
1.20236250782184));
#160732=CARTESIAN_POINT('Ctrl Pts',(6.97871089679715,-0.697357053149192,
1.19433713587373));
#160733=CARTESIAN_POINT('Ctrl Pts',(6.95894217120697,-0.87291662569608,
1.18631176392561));
#160734=CARTESIAN_POINT('Ctrl Pts',(6.93253436434061,-1.0476611330657,1.17828639197751));
#160735=CARTESIAN_POINT('Ctrl Pts',(6.90615057214422,-1.22224673168184,
1.17026831812347));
#160736=CARTESIAN_POINT('Ctrl Pts',(6.87313977264274,-1.39601838056077,
1.16225024426945));
#160737=CARTESIAN_POINT('Ctrl Pts',(6.8335685390142,-1.5684283806076,1.15423217041541));
#160738=CARTESIAN_POINT('Ctrl Pts',(6.7919833913311,-1.74961290928045,1.14580602963638));
#160739=CARTESIAN_POINT('Ctrl Pts',(6.74315260201287,-1.92929316192643,
1.13737988885733));
#160740=CARTESIAN_POINT('Ctrl Pts',(6.68721496429928,-2.1068418506741,1.1289537480783));
#160741=CARTESIAN_POINT('Ctrl Pts',(6.63404803922703,-2.27559616739471,
1.12094497234592));
#160742=CARTESIAN_POINT('Ctrl Pts',(6.57446140310177,-2.44242457829185,
1.11293619661355));
#160743=CARTESIAN_POINT('Ctrl Pts',(6.50862608358455,-2.60680130937954,
1.10492742088118));
#160744=CARTESIAN_POINT('Ctrl Pts',(6.44280441263479,-2.77114396290947,
1.09692030547819));
#160745=CARTESIAN_POINT('Ctrl Pts',(6.37073677303487,-2.93303560808939,
1.08891319007519));
#160746=CARTESIAN_POINT('Ctrl Pts',(6.29264303487681,-3.09196866059738,
1.0809060746722));
#160747=CARTESIAN_POINT('Ctrl Pts',(6.21455054475987,-3.25089917314522,
1.07289908723349));
#160748=CARTESIAN_POINT('Ctrl Pts',(6.1304323099791,-3.40687085824795,1.06489209979479));
#160749=CARTESIAN_POINT('Ctrl Pts',(6.04055500235253,-3.55939908215612,
1.05688511235608));
#160750=CARTESIAN_POINT('Ctrl Pts',(5.95066193371926,-3.71195405362074,
1.04887672080119));
#160751=CARTESIAN_POINT('Ctrl Pts',(5.8550079687018,-3.86106404641347,1.0408683292463));
#160752=CARTESIAN_POINT('Ctrl Pts',(5.75390406474699,-4.00627190492458,
1.03285993769141));
#160753=CARTESIAN_POINT('Ctrl Pts',(5.65272073837281,-4.1515938318246,1.02484525512491));
#160754=CARTESIAN_POINT('Ctrl Pts',(5.54607913401669,-4.29300720248875,
1.01683057255842));
#160755=CARTESIAN_POINT('Ctrl Pts',(5.43433198097541,-4.43008605819886,
1.00881588999193));
#160756=CARTESIAN_POINT('Ctrl Pts',(5.32253372883842,-4.56722759654004,
1.00079754251747));
#160757=CARTESIAN_POINT('Ctrl Pts',(5.20562551800962,-4.70003039580051,
0.992779195042993));
#160758=CARTESIAN_POINT('Ctrl Pts',(5.0839979594269,-4.82810431857506,0.984760847568531));
#160759=CARTESIAN_POINT('Ctrl Pts',(4.96223719035818,-4.95631851210481,
0.976733718137279));
#160760=CARTESIAN_POINT('Ctrl Pts',(4.83574701523879,-5.07979323295038,
0.96870658870603));
#160761=CARTESIAN_POINT('Ctrl Pts',(4.70495270924007,-5.19817723498483,
0.960679459274779));
#160762=CARTESIAN_POINT('Ctrl Pts',(4.6578376048721,-5.24082186365395,0.957787903422705));
#160763=CARTESIAN_POINT('Ctrl Pts',(4.61016428687613,-5.28280631233251,
0.954896347570646));
#160764=CARTESIAN_POINT('Ctrl Pts',(4.56195357994032,-5.32411552250416,
0.952004791718572));
#160765=CARTESIAN_POINT('Ctrl Pts',(4.42499058165173,-5.44147188671545,
0.943790098668195));
#160766=CARTESIAN_POINT('Ctrl Pts',(4.28336273305126,-5.55365432817702,
0.935575405617811));
#160767=CARTESIAN_POINT('Ctrl Pts',(4.13749531642573,-5.66027906282501,
0.927360712567442));
#160768=CARTESIAN_POINT('Ctrl Pts',(3.99174322317756,-5.76681949952082,
0.919152514087063));
#160769=CARTESIAN_POINT('Ctrl Pts',(3.84175851848875,-5.86781077799396,
0.910944315606697));
#160770=CARTESIAN_POINT('Ctrl Pts',(3.688000133595,-5.96290881844619,0.902736117126317));
#160771=CARTESIAN_POINT('Ctrl Pts',(3.53433743432414,-6.05794767828694,
0.894533026702872));
#160772=CARTESIAN_POINT('Ctrl Pts',(3.37690602898616,-6.14710042473106,
0.886329936279438));
#160773=CARTESIAN_POINT('Ctrl Pts',(3.21619461364133,-6.23006571150614,
0.878126845855995));
#160774=CARTESIAN_POINT('Ctrl Pts',(3.05555571771255,-6.31299356102677,
0.869927456994921));
#160775=CARTESIAN_POINT('Ctrl Pts',(2.89164007017492,-6.38973935584501,
0.861728068133851));
#160776=CARTESIAN_POINT('Ctrl Pts',(2.72496197649438,-6.46004711973217,
0.853528679272777));
#160777=CARTESIAN_POINT('Ctrl Pts',(2.55832821219312,-6.53033618470417,
0.845331471105103));
#160778=CARTESIAN_POINT('Ctrl Pts',(2.38893378670014,-6.59419049688694,
0.83713426293742));
#160779=CARTESIAN_POINT('Ctrl Pts',(2.21731424712931,-6.65140166370799,
0.828937054769746));
#160780=CARTESIAN_POINT('Ctrl Pts',(2.04569290397268,-6.70861343177321,
0.820739760455888));
#160781=CARTESIAN_POINT('Ctrl Pts',(1.87184672901308,-6.75918180167349,
0.81254246614204));
#160782=CARTESIAN_POINT('Ctrl Pts',(1.69632810358554,-6.80294770871318,
0.804345171828182));
#160783=CARTESIAN_POINT('Ctrl Pts',(1.61776226552343,-6.8225382516356,0.800675890029505));
#160784=CARTESIAN_POINT('Ctrl Pts',(1.53886152203894,-6.84076649049403,
0.797006608230821));
#160785=CARTESIAN_POINT('Ctrl Pts',(1.45967623572252,-6.85762144255331,
0.793337326432145));
#160786=CARTESIAN_POINT('Ctrl Pts',(1.2603658835866,-6.9000455668628,0.784101698433557));
#160787=CARTESIAN_POINT('Ctrl Pts',(1.05939543448741,-6.93373583637711,
0.774866070434961));
#160788=CARTESIAN_POINT('Ctrl Pts',(0.857490139534536,-6.95861604222428,
0.765630442436375));
#160789=CARTESIAN_POINT('Ctrl Pts',(0.655095352696672,-6.98355656674144,
0.756372423915742));
#160790=CARTESIAN_POINT('Ctrl Pts',(0.451761352159633,-6.99964427887868,
0.747114405395103));
#160791=CARTESIAN_POINT('Ctrl Pts',(0.248218246281154,-7.00685480545395,
0.737856386874469));
#160792=CARTESIAN_POINT('Ctrl Pts',(0.0441803191657221,-7.01408286110083,
0.728575861749368));
#160793=CARTESIAN_POINT('Ctrl Pts',(-0.160067563697973,-7.01239053413776,
0.719295336624267));
#160794=CARTESIAN_POINT('Ctrl Pts',(-0.363792928561735,-7.00180557196703,
0.710014811499164));
#160795=CARTESIAN_POINT('Ctrl Pts',(-0.567660667977806,-6.99121321243931,
0.70072780062983));
#160796=CARTESIAN_POINT('Ctrl Pts',(-0.771004994509795,-6.97171581173367,
0.691440789760502));
#160797=CARTESIAN_POINT('Ctrl Pts',(-0.973097359689014,-6.9433931251994,
0.68215377889117));
#160798=CARTESIAN_POINT('Ctrl Pts',(-1.17520208409502,-6.91506870655365,
0.672866200062363));
#160799=CARTESIAN_POINT('Ctrl Pts',(-1.37605453130155,-6.87791795119954,
0.663578621233559));
#160800=CARTESIAN_POINT('Ctrl Pts',(-1.57493393023453,-6.83207213646753,
0.654291042404751));
#160801=CARTESIAN_POINT('Ctrl Pts',(-1.71498653192544,-6.79978711517168,
0.647750648651738));
#160802=CARTESIAN_POINT('Ctrl Pts',(-1.85406084050494,-6.76319120099541,
0.641210254898729));
#160803=CARTESIAN_POINT('Ctrl Pts',(-1.9919081624325,-6.72234545638163,
0.634669861145717));
#160804=CARTESIAN_POINT('Ctrl Pts',(-2.16187146483775,-6.67198337791189,
0.62660567168053));
#160805=CARTESIAN_POINT('Ctrl Pts',(-2.33009322388277,-6.61512101676497,
0.618541482215349));
#160806=CARTESIAN_POINT('Ctrl Pts',(-2.49603703497435,-6.55190244757479,
0.610477292750161));
#160807=CARTESIAN_POINT('Ctrl Pts',(-2.66187495730633,-6.48872421815883,
0.602418249044939));
#160808=CARTESIAN_POINT('Ctrl Pts',(-2.82543748714466,-6.41919798424768,
0.594359205339728));
#160809=CARTESIAN_POINT('Ctrl Pts',(-2.98620339036206,-6.34351762619843,
0.586300161634504));
#160810=CARTESIAN_POINT('Ctrl Pts',(-3.14689695606165,-6.2678713209498,
0.578244744141095));
#160811=CARTESIAN_POINT('Ctrl Pts',(-3.30479607282164,-6.18607656046966,
0.570189326647669));
#160812=CARTESIAN_POINT('Ctrl Pts',(-3.45939951677418,-6.09837532018509,
0.562133909154262));
#160813=CARTESIAN_POINT('Ctrl Pts',(-3.61398280253898,-6.01068551495023,
0.554079541977809));
#160814=CARTESIAN_POINT('Ctrl Pts',(-3.76527095204614,-5.91709093718653,
0.546025174801362));
#160815=CARTESIAN_POINT('Ctrl Pts',(-3.9127872078451,-5.81787958182565,
0.537970807624909));
#160816=CARTESIAN_POINT('Ctrl Pts',(-4.0602908570555,-5.71867670496585,
0.529917128766447));
#160817=CARTESIAN_POINT('Ctrl Pts',(-4.20402295515093,-5.61385821280352,
0.521863449907972));
#160818=CARTESIAN_POINT('Ctrl Pts',(-4.34353582518329,-5.50375536319061,
0.513809771049509));
#160819=CARTESIAN_POINT('Ctrl Pts',(-4.48309818947319,-5.3936134529606,
0.505753235029154));
#160820=CARTESIAN_POINT('Ctrl Pts',(-4.61843805165705,-5.27818366768537,
0.497696699008806));
#160821=CARTESIAN_POINT('Ctrl Pts',(-4.74914061076898,-5.15783772734708,
0.489640162988451));
#160822=CARTESIAN_POINT('Ctrl Pts',(-4.82288988547179,-5.08993220297417,
0.485094240612061));
#160823=CARTESIAN_POINT('Ctrl Pts',(-4.89516335785953,-5.02046217445374,
0.480548318235672));
#160824=CARTESIAN_POINT('Ctrl Pts',(-4.96589168557297,-4.94949960396577,
0.476002395859283));
#160825=CARTESIAN_POINT('Ctrl Pts',(-5.10456501020033,-4.81036701180917,
0.467089444149383));
#160826=CARTESIAN_POINT('Ctrl Pts',(-5.23733419343256,-4.66545741061707,
0.458176492439488));
#160827=CARTESIAN_POINT('Ctrl Pts',(-5.36375573086079,-4.51527972800779,
0.449263540729589));
#160828=CARTESIAN_POINT('Ctrl Pts',(-5.49025725910387,-4.36500702333621,
0.440344949519613));
#160829=CARTESIAN_POINT('Ctrl Pts',(-5.61040296415482,-4.20945976339479,
0.431426358309636));
#160830=CARTESIAN_POINT('Ctrl Pts',(-5.72378996120478,-4.04917955177483,
0.42250776709966));
#160831=CARTESIAN_POINT('Ctrl Pts',(-5.83725514330947,-3.88878882027654,
0.413583026149766));
#160832=CARTESIAN_POINT('Ctrl Pts',(-5.94395216188509,-3.72365880956333,
0.40465828519986));
#160833=CARTESIAN_POINT('Ctrl Pts',(-6.04352085891127,-3.55436101014013,
0.395733544249964));
#160834=CARTESIAN_POINT('Ctrl Pts',(-6.14310049497154,-3.3850446109516,
0.386807822790647));
#160835=CARTESIAN_POINT('Ctrl Pts',(-6.23555012739648,-3.21155971820321,
0.377882101331347));
#160836=CARTESIAN_POINT('Ctrl Pts',(-6.32055488330501,-3.0345036710522,
0.368956379872031));
#160837=CARTESIAN_POINT('Ctrl Pts',(-6.40555790762161,-2.85745123062667,
0.360030840234392));
#160838=CARTESIAN_POINT('Ctrl Pts',(-6.48311625587417,-2.67682799855142,
0.35110530059676));
#160839=CARTESIAN_POINT('Ctrl Pts',(-6.55296211181921,-2.49325372225973,
0.34217976095912));
#160840=CARTESIAN_POINT('Ctrl Pts',(-6.61776896625368,-2.32292333915279,
0.333898150830369));
#160841=CARTESIAN_POINT('Ctrl Pts',(-6.67593642861803,-2.15005271925837,
0.325616540701606));
#160842=CARTESIAN_POINT('Ctrl Pts',(-6.72728788244206,-1.97515171803289,
0.317334930572855));
#160843=CARTESIAN_POINT('Ctrl Pts',(-6.77907180886242,-1.79877773241324,
0.308983574231145));
#160844=CARTESIAN_POINT('Ctrl Pts',(-6.82393755001756,-1.62029056482357,
0.300632217889427));
#160845=CARTESIAN_POINT('Ctrl Pts',(-6.86172539517146,-1.4402607971333,
0.292280861547717));
#160846=CARTESIAN_POINT('Ctrl Pts',(-6.89949937822051,-1.2602970716189,
0.283932568820159));
#160847=CARTESIAN_POINT('Ctrl Pts',(-6.93020057416922,-1.07879219770202,
0.275584276092606));
#160848=CARTESIAN_POINT('Ctrl Pts',(-6.95371995337483,-0.896328830584341,
0.267235983365048));
#160849=CARTESIAN_POINT('Ctrl Pts',(-6.97723395162932,-0.713907208890815,
0.258889600626471));
#160850=CARTESIAN_POINT('Ctrl Pts',(-6.99356936789201,-0.530527859304366,
0.250543217887913));
#160851=CARTESIAN_POINT('Ctrl Pts',(-7.00266874717422,-0.346780881608981,
0.242196835149336));
#160852=CARTESIAN_POINT('Ctrl Pts',(-7.01176860716355,-0.163024196824893,
0.233850011483357));
#160853=CARTESIAN_POINT('Ctrl Pts',(-7.01363164572049,0.0210998245950316,
0.225503187817363));
#160854=CARTESIAN_POINT('Ctrl Pts',(-7.00825244637512,0.20499807408169,
0.217156364151386));
#160855=CARTESIAN_POINT('Ctrl Pts',(-7.00287315096108,0.38889960785984,
0.208809391417094));
#160856=CARTESIAN_POINT('Ctrl Pts',(-6.99025137322777,0.572575031013105,
0.200462418682822));
#160857=CARTESIAN_POINT('Ctrl Pts',(-6.97043378629731,0.755433248768528,
0.192115445948531));
#160858=CARTESIAN_POINT('Ctrl Pts',(-6.95060935228489,0.938354645013201,
0.183765589290653));
#160859=CARTESIAN_POINT('Ctrl Pts',(-6.92358418101607,1.12045794309435,
0.175415732632769));
#160860=CARTESIAN_POINT('Ctrl Pts',(-6.88945667745427,1.30115842693376,
0.167065875974892));
#160861=CARTESIAN_POINT('Ctrl Pts',(-6.87801469298165,1.3617421765345,0.164266405745402));
#160862=CARTESIAN_POINT('Ctrl Pts',(-6.86577478234028,1.42216831972826,
0.16146693551591));
#160863=CARTESIAN_POINT('Ctrl Pts',(-6.85274193659805,1.48241509466492,
0.15866746528642));
#160864=CARTESIAN_POINT('Ctrl Pts',(-6.81252228002286,1.66833800403104,
0.150028236874645));
#160865=CARTESIAN_POINT('Ctrl Pts',(-6.76472908610749,1.85263628174639,
0.141389008462876));
#160866=CARTESIAN_POINT('Ctrl Pts',(-6.7095182968688,2.03469673083801,0.1327497800511));
#160867=CARTESIAN_POINT('Ctrl Pts',(-6.65431427480331,2.21673486482398,
0.12411161054748));
#160868=CARTESIAN_POINT('Ctrl Pts',(-6.59169455695899,2.39653544070573,
0.115473441043872));
#160869=CARTESIAN_POINT('Ctrl Pts',(-6.52186501817855,2.57350019373594,
0.106835271540255));
#160870=CARTESIAN_POINT('Ctrl Pts',(-6.44989512403592,2.75588911918205,
0.0979323322452363));
#160871=CARTESIAN_POINT('Ctrl Pts',(-6.37026650450594,2.93526531039644,
0.0890293929502093));
#160872=CARTESIAN_POINT('Ctrl Pts',(-6.28325856614943,3.11099475303475,
0.0801264536551898));
#160873=CARTESIAN_POINT('Ctrl Pts',(-6.19884731143077,3.28147968836712,
0.0714892155965488));
#160874=CARTESIAN_POINT('Ctrl Pts',(-6.1074910014181,3.44853214205245,0.0628519775378872));
#160875=CARTESIAN_POINT('Ctrl Pts',(-6.00949230903563,3.6115964268093,0.0542147394792423));
#160876=CARTESIAN_POINT('Ctrl Pts',(-5.90697162011571,3.78218505819899,
0.0451789495660293));
#160877=CARTESIAN_POINT('Ctrl Pts',(-5.79718119022459,3.94840845108158,
0.0361431596528352));
#160878=CARTESIAN_POINT('Ctrl Pts',(-5.68051992566802,4.10966177885585,
0.0271073697396247));
#160879=CARTESIAN_POINT('Ctrl Pts',(-5.56385866111145,4.27091510663012,
0.0180715798264141));
#160880=CARTESIAN_POINT('Ctrl Pts',(-5.44032677458003,4.42719807500911,
0.00903578991321001));
#160881=CARTESIAN_POINT('Ctrl Pts',(-5.31037376991255,4.57794244025903,
0.));
#160882=CARTESIAN_POINT('',(5.30919883249355,4.57930500398795,2.57697863048634E-7));
#160883=CARTESIAN_POINT('Origin',(0.,0.,0.));
#160884=CARTESIAN_POINT('',(7.01124999980813,-5.18702183968693E-5,1.77353435693496));
#160885=CARTESIAN_POINT('Ctrl Pts',(5.30919883249355,4.57930500398795,2.57697855943206E-7));
#160886=CARTESIAN_POINT('Ctrl Pts',(5.17711001830684,4.73244740822939,0.00920421453633651));
#160887=CARTESIAN_POINT('Ctrl Pts',(5.03841024185807,4.87985060242885,0.0184081713748201));
#160888=CARTESIAN_POINT('Ctrl Pts',(4.89359335575129,5.02099299253115,0.0276121282132991));
#160889=CARTESIAN_POINT('Ctrl Pts',(4.74881129473298,5.16210144117568,0.0368138717145086));
#160890=CARTESIAN_POINT('Ctrl Pts',(4.59791519661176,5.29695196575731,0.0460156152156967));
#160891=CARTESIAN_POINT('Ctrl Pts',(4.44143525766802,5.42506031435996,0.0552173587169094));
#160892=CARTESIAN_POINT('Ctrl Pts',(4.28516511765998,5.55299690295701,0.0644067650712253));
#160893=CARTESIAN_POINT('Ctrl Pts',(4.12332623735365,5.67420925882696,0.0735961714255482));
#160894=CARTESIAN_POINT('Ctrl Pts',(3.95648126927498,5.78825384104535,0.082785577779859));
#160895=CARTESIAN_POINT('Ctrl Pts',(3.78985279998986,5.90215043849234,0.0919630599184624));
#160896=CARTESIAN_POINT('Ctrl Pts',(3.61823136491426,6.00889772774248,0.101140542057079));
#160897=CARTESIAN_POINT('Ctrl Pts',(3.44220988242581,6.10809443998946,0.110318024195685));
#160898=CARTESIAN_POINT('Ctrl Pts',(3.26664748986962,6.20703243261163,0.119471570110178));
#160899=CARTESIAN_POINT('Ctrl Pts',(3.08670811918591,6.29845906723639,0.128625116024664));
#160900=CARTESIAN_POINT('Ctrl Pts',(2.90301021948285,6.38201835065351,0.137778661939159));
#160901=CARTESIAN_POINT('Ctrl Pts',(2.82012422289691,6.41972098357,0.141908816811068));
#160902=CARTESIAN_POINT('Ctrl Pts',(2.73647342649563,6.45582249259887,0.146038971682991));
#160903=CARTESIAN_POINT('Ctrl Pts',(2.65211653575299,6.49029309378903,0.1501691265549));
#160904=CARTESIAN_POINT('Ctrl Pts',(2.48468518033815,6.55871026076169,0.158366648087392));
#160905=CARTESIAN_POINT('Ctrl Pts',(2.31456968522649,6.62065883490012,0.166564169619877));
#160906=CARTESIAN_POINT('Ctrl Pts',(2.14230841566705,6.67593747833682,0.174761691152369));
#160907=CARTESIAN_POINT('Ctrl Pts',(1.97005289242181,6.73121427778122,0.182958939230855));
#160908=CARTESIAN_POINT('Ctrl Pts',(1.79565206881785,6.77982148391414,0.19115618730935));
#160909=CARTESIAN_POINT('Ctrl Pts',(1.6196603517921,6.82160735511307,0.199353435387835));
#160910=CARTESIAN_POINT('Ctrl Pts',(1.44364490628013,6.86339886018776,0.20755178867906));
#160911=CARTESIAN_POINT('Ctrl Pts',(1.26603847869501,6.89836711822185,0.215750141970292));
#160912=CARTESIAN_POINT('Ctrl Pts',(1.08740676178002,6.9264112711371,0.223948495261517));
#160913=CARTESIAN_POINT('Ctrl Pts',(0.90865370707236,6.95447447338845,0.232152417385136));
#160914=CARTESIAN_POINT('Ctrl Pts',(0.728874315852634,6.97560412070426,
0.240356339508754));
#160915=CARTESIAN_POINT('Ctrl Pts',(0.548641355408434,6.98975101313599,
0.248560261632377));
#160916=CARTESIAN_POINT('Ctrl Pts',(0.368339379111189,7.00390332277801,
0.256767325249556));
#160917=CARTESIAN_POINT('Ctrl Pts',(0.187583834733879,7.01106752899879,
0.264974388866734));
#160918=CARTESIAN_POINT('Ctrl Pts',(0.00694885283989022,7.01124655649366,
0.273181452483911));
#160919=CARTESIAN_POINT('Ctrl Pts',(-0.173861858901962,7.01142575815454,
0.281396500302297));
#160920=CARTESIAN_POINT('Ctrl Pts',(-0.354551426171415,7.00460621641048,
0.289611548120658));
#160921=CARTESIAN_POINT('Ctrl Pts',(-0.534548563057438,6.99084289597708,
0.297826595939043));
#160922=CARTESIAN_POINT('Ctrl Pts',(-0.614960663037309,6.98469425651597,
0.30149659457313));
#160923=CARTESIAN_POINT('Ctrl Pts',(-0.695234661285935,6.97716048410052,
0.305166593207232));
#160924=CARTESIAN_POINT('Ctrl Pts',(-0.775320191888788,6.96824979191687,
0.30883659184132));
#160925=CARTESIAN_POINT('Ctrl Pts',(-0.953332438724452,6.94844331346151,
0.31699417908361));
#160926=CARTESIAN_POINT('Ctrl Pts',(-1.13078883931233,6.92178858772017,
0.325151766325908));
#160927=CARTESIAN_POINT('Ctrl Pts',(-1.30712494444465,6.88832715121099,
0.333309353568197));
#160928=CARTESIAN_POINT('Ctrl Pts',(-1.48330105598897,6.85489607499181,
0.341459539253945));
#160929=CARTESIAN_POINT('Ctrl Pts',(-1.6583585512607,6.81467065416905,0.349609724939691));
#160930=CARTESIAN_POINT('Ctrl Pts',(-1.83173834330004,6.7677441739611,0.35775991062544));
#160931=CARTESIAN_POINT('Ctrl Pts',(-2.00499456597701,6.72085113868448,
0.365904287599363));
#160932=CARTESIAN_POINT('Ctrl Pts',(-2.17657512720709,6.66726664954513,
0.374048664573273));
#160933=CARTESIAN_POINT('Ctrl Pts',(-2.34593121972405,6.60713502774266,
0.382193041547197));
#160934=CARTESIAN_POINT('Ctrl Pts',(-2.51519956181275,6.54703456263192,
0.390333198581012));
#160935=CARTESIAN_POINT('Ctrl Pts',(-2.68224539890916,6.48039384135878,
0.398473355614832));
#160936=CARTESIAN_POINT('Ctrl Pts',(-2.8465350287286,6.4074070334825,0.406613512648647));
#160937=CARTESIAN_POINT('Ctrl Pts',(-3.01077149323455,6.3344438446656,0.41475103546872));
#160938=CARTESIAN_POINT('Ctrl Pts',(-3.17225320489948,6.25513880485553,
0.422888558288796));
#160939=CARTESIAN_POINT('Ctrl Pts',(-3.33046625360608,6.16973428083342,
0.431026081108868));
#160940=CARTESIAN_POINT('Ctrl Pts',(-3.48869526370463,6.08432114073891,
0.439164424886455));
#160941=CARTESIAN_POINT('Ctrl Pts',(-3.64365463637829,5.99280744701559,
0.447302768664046));
#160942=CARTESIAN_POINT('Ctrl Pts',(-3.79485442334125,5.89548186903729,
0.455441112441633));
#160943=CARTESIAN_POINT('Ctrl Pts',(-3.94606937134013,5.79814653207312,
0.463580272263508));
#160944=CARTESIAN_POINT('Ctrl Pts',(-4.09352368425078,5.69499834042374,
0.471719432085371));
#160945=CARTESIAN_POINT('Ctrl Pts',(-4.236755969054,5.58636961014802,0.479858591907245));
#160946=CARTESIAN_POINT('Ctrl Pts',(-4.38002786946516,5.47771083501756,
0.488000002881957));
#160947=CARTESIAN_POINT('Ctrl Pts',(-4.5190751328444,5.36356871457753,0.496141413856687));
#160948=CARTESIAN_POINT('Ctrl Pts',(-4.65346897011614,5.24431626684225,
0.5042828248314));
#160949=CARTESIAN_POINT('Ctrl Pts',(-4.78792367425065,5.12500980976756,
0.512427923044713));
#160950=CARTESIAN_POINT('Ctrl Pts',(-4.9177204885028,5.00058864848786,0.520573021258008));
#160951=CARTESIAN_POINT('Ctrl Pts',(-5.04246696641261,4.87146317394863,
0.528718119471321));
#160952=CARTESIAN_POINT('Ctrl Pts',(-5.16737490010896,4.74217057601317,
0.536873759651514));
#160953=CARTESIAN_POINT('Ctrl Pts',(-5.287219191426,4.60816175451188,0.545029399831718));
#160954=CARTESIAN_POINT('Ctrl Pts',(-5.40164643869375,4.46988168902121,
0.553185040011911));
#160955=CARTESIAN_POINT('Ctrl Pts',(-5.516149875366,4.33150955213938,0.561346110484132));
#160956=CARTESIAN_POINT('Ctrl Pts',(-5.62522886350364,4.18886078260095,
0.569507180956342));
#160957=CARTESIAN_POINT('Ctrl Pts',(-5.72857299043574,4.04240993168062,
0.577668251428562));
#160958=CARTESIAN_POINT('Ctrl Pts',(-5.83209280458033,3.89571011120075,
0.585843195894058));
#160959=CARTESIAN_POINT('Ctrl Pts',(-5.92985807979805,3.74519558773208,
0.594018140359565));
#160960=CARTESIAN_POINT('Ctrl Pts',(-6.02160329609183,3.59136747033718,
0.602193084825061));
#160961=CARTESIAN_POINT('Ctrl Pts',(-6.11130449436035,3.44096653375286,
0.610185897354768));
#160962=CARTESIAN_POINT('Ctrl Pts',(-6.19525095685086,3.28739838638717,
0.618178709884468));
#160963=CARTESIAN_POINT('Ctrl Pts',(-6.27323931727954,3.13114915496502,
0.626171522414175));
#160964=CARTESIAN_POINT('Ctrl Pts',(-6.35305293962011,2.97124302180383,
0.634351401016297));
#160965=CARTESIAN_POINT('Ctrl Pts',(-6.42687058601084,2.80803900398711,
0.642531279618431));
#160966=CARTESIAN_POINT('Ctrl Pts',(-6.4944077485214,2.64202470814435,0.650711158220552));
#160967=CARTESIAN_POINT('Ctrl Pts',(-6.56185810388352,2.4762237944913,0.658880523026866));
#160968=CARTESIAN_POINT('Ctrl Pts',(-6.62304391942665,2.30762011976076,
0.667049887833166));
#160969=CARTESIAN_POINT('Ctrl Pts',(-6.67772617467052,2.13672639769818,
0.675219252639479));
#160970=CARTESIAN_POINT('Ctrl Pts',(-6.73234876599132,1.96601913813318,
0.683379703834765));
#160971=CARTESIAN_POINT('Ctrl Pts',(-6.78048182329104,1.79302714164442,
0.691540155030056));
#160972=CARTESIAN_POINT('Ctrl Pts',(-6.8219340456616,1.61828379437696,0.699700606225342));
#160973=CARTESIAN_POINT('Ctrl Pts',(-6.8633490868576,1.44369718569983,0.707853737785077));
#160974=CARTESIAN_POINT('Ctrl Pts',(-6.89809514877191,1.26736269732015,
0.716006869344827));
#160975=CARTESIAN_POINT('Ctrl Pts',(-6.92603044060034,1.08982975660305,
0.724160000904561));
#160976=CARTESIAN_POINT('Ctrl Pts',(-6.9539460969969,0.912421601980324,
0.73230740171123));
#160977=CARTESIAN_POINT('Ctrl Pts',(-6.975060465986,0.733817021089351,0.74045480251789));
#160978=CARTESIAN_POINT('Ctrl Pts',(-6.98928259890422,0.554576699072976,
0.748602203324559));
#160979=CARTESIAN_POINT('Ctrl Pts',(-7.00349787038227,0.375422851198931,
0.756745673433665));
#160980=CARTESIAN_POINT('Ctrl Pts',(-7.01082750234475,0.195634224786323,
0.764889143542771));
#160981=CARTESIAN_POINT('Ctrl Pts',(-7.01123224688893,0.0157779176322022,
0.773032613651878));
#160982=CARTESIAN_POINT('Ctrl Pts',(-7.01163688829273,-0.164032557039414,
0.781174008574092));
#160983=CARTESIAN_POINT('Ctrl Pts',(-7.00512015578681,-0.343910325027825,
0.789315403496302));
#160984=CARTESIAN_POINT('Ctrl Pts',(-6.99169489609768,-0.523286768781423,
0.797456798418516));
#160985=CARTESIAN_POINT('Ctrl Pts',(-6.97827069719901,-0.702649039191136,
0.805597550052304));
#160986=CARTESIAN_POINT('Ctrl Pts',(-6.95793908487309,-0.881509711923539,
0.813738301686094));
#160987=CARTESIAN_POINT('Ctrl Pts',(-6.93076491788837,-1.05930364649039,
0.821879053319883));
#160988=CARTESIAN_POINT('Ctrl Pts',(-6.90358812056928,-1.23711479069232,
0.830020592940985));
#160989=CARTESIAN_POINT('Ctrl Pts',(-6.86956750309537,-1.41385864180084,
0.838162132562087));
#160990=CARTESIAN_POINT('Ctrl Pts',(-6.82881936249476,-1.588978501087,0.84630367218319));
#160991=CARTESIAN_POINT('Ctrl Pts',(-6.78804138159968,-1.76422660249885,
0.854451173939893));
#160992=CARTESIAN_POINT('Ctrl Pts',(-6.74052611273859,-1.93784799086778,
0.862598675696589));
#160993=CARTESIAN_POINT('Ctrl Pts',(-6.68644047313306,-2.1092985473252,
0.870746177453292));
#160994=CARTESIAN_POINT('Ctrl Pts',(-6.6323353760226,-2.28081078374184,
0.878896610303287));
#160995=CARTESIAN_POINT('Ctrl Pts',(-6.57165531205661,-2.45015029749233,
0.88704704315328));
#160996=CARTESIAN_POINT('Ctrl Pts',(-6.50461607235799,-2.61679122471055,
0.895197476003275));
#160997=CARTESIAN_POINT('Ctrl Pts',(-6.43749721470135,-2.78363006005553,
0.90335758856956));
#160998=CARTESIAN_POINT('Ctrl Pts',(-6.36400422904425,-2.94776357937369,
0.911517701135838));
#160999=CARTESIAN_POINT('Ctrl Pts',(-6.28440028099749,-3.10868777311243,
0.919677813702123));
#161000=CARTESIAN_POINT('Ctrl Pts',(-6.20691549353275,-3.2653279556126,
0.927620693463757));
#161001=CARTESIAN_POINT('Ctrl Pts',(-6.12364114321043,-3.41892726396892,
0.935563573225403));
#161002=CARTESIAN_POINT('Ctrl Pts',(-6.0348598328842,-3.56904656175019,
0.943506452987037));
#161003=CARTESIAN_POINT('Ctrl Pts',(-5.94312944520624,-3.72415242054883,
0.951713173941446));
#161004=CARTESIAN_POINT('Ctrl Pts',(-5.84532617622802,-3.87587088288704,
0.959919894895858));
#161005=CARTESIAN_POINT('Ctrl Pts',(-5.74172845038914,-4.02370239511969,
0.968126615850267));
#161006=CARTESIAN_POINT('Ctrl Pts',(-5.63821157389144,-4.17141853724869,
0.976326932146879));
#161007=CARTESIAN_POINT('Ctrl Pts',(-5.52890944776105,-4.31525348751679,
0.984527248443485));
#161008=CARTESIAN_POINT('Ctrl Pts',(-5.4141451452014,-4.45473443756102,
0.9927275647401));
#161009=CARTESIAN_POINT('Ctrl Pts',(-5.2994509438435,-4.59413018879342,
1.00092287205732));
#161010=CARTESIAN_POINT('Ctrl Pts',(-5.17930143457965,-4.72917697002963,
1.00911817937454));
#161011=CARTESIAN_POINT('Ctrl Pts',(-5.05406163145324,-4.85943284632808,
1.01731348669176));
#161012=CARTESIAN_POINT('Ctrl Pts',(-4.92887574014346,-4.98963265154735,
1.0255052661856));
#161013=CARTESIAN_POINT('Ctrl Pts',(-4.79860416296257,-5.11504541049285,
1.03369704567944));
#161014=CARTESIAN_POINT('Ctrl Pts',(-4.66365077157032,-5.23526389433537,
1.04188882517328));
#161015=CARTESIAN_POINT('Ctrl Pts',(-4.52873164262145,-5.35545185668486,
1.05007852490923));
#161016=CARTESIAN_POINT('Ctrl Pts',(-4.38913332933796,-5.47044794098969,
1.05826822464517));
#161017=CARTESIAN_POINT('Ctrl Pts',(-4.24529511770079,-5.57988314627877,
1.06645792438111));
#161018=CARTESIAN_POINT('Ctrl Pts',(-4.10145226326054,-5.6893218839123,
1.0746478884638));
#161019=CARTESIAN_POINT('Ctrl Pts',(-3.95336951282026,-5.79319917026139,
1.0828378525465));
#161020=CARTESIAN_POINT('Ctrl Pts',(-3.8015179559582,-5.89118729909578,
1.09102781662919));
#161021=CARTESIAN_POINT('Ctrl Pts',(-3.73263068243912,-5.93563949420083,
1.09474318384395));
#161022=CARTESIAN_POINT('Ctrl Pts',(-3.66296820625712,-5.97888029959006,
1.09845855105871));
#161023=CARTESIAN_POINT('Ctrl Pts',(-3.59257642105979,-6.02088209661551,
1.10217391827347));
#161024=CARTESIAN_POINT('Ctrl Pts',(-3.41746583716016,-6.12536814113538,
1.11141647577581));
#161025=CARTESIAN_POINT('Ctrl Pts',(-3.23796122535349,-6.22211184220953,
1.12065903327815));
#161026=CARTESIAN_POINT('Ctrl Pts',(-3.05472541606613,-6.3108065407632,
1.12990159078048));
#161027=CARTESIAN_POINT('Ctrl Pts',(-2.87104650153154,-6.39971572297312,
1.13916649885798));
#161028=CARTESIAN_POINT('Ctrl Pts',(-2.68361848851216,-6.48053689192567,
1.14843140693547));
#161029=CARTESIAN_POINT('Ctrl Pts',(-2.49312555262666,-6.5530108760279,
1.15769631501296));
#161030=CARTESIAN_POINT('Ctrl Pts',(-2.30217615922385,-6.62565852166094,
1.16698342358267));
#161031=CARTESIAN_POINT('Ctrl Pts',(-2.10814729959598,-6.68991889389765,
1.17627053215238));
#161032=CARTESIAN_POINT('Ctrl Pts',(-1.91174218981668,-6.74558139541544,
1.18555764072208));
#161033=CARTESIAN_POINT('Ctrl Pts',(-1.71520558877797,-6.80128116242207,
1.19485096691822));
#161034=CARTESIAN_POINT('Ctrl Pts',(-1.51628971763685,-6.84837151554262,
1.20414429311435));
#161035=CARTESIAN_POINT('Ctrl Pts',(-1.31571086991073,-6.88669234606126,
1.21343761931049));
#161036=CARTESIAN_POINT('Ctrl Pts',(-1.11513281857241,-6.92501302442905,
1.22273090860796));
#161037=CARTESIAN_POINT('Ctrl Pts',(-0.91289196553951,-6.9545642242027,
1.23202419790545));
#161038=CARTESIAN_POINT('Ctrl Pts',(-0.709713821382708,-6.97523711813716,
1.24131748720293));
#161039=CARTESIAN_POINT('Ctrl Pts',(-0.56743090082418,-6.98971406760236,
1.24782545265525));
#161040=CARTESIAN_POINT('Ctrl Pts',(-0.424688526390375,-6.99983815160022,
1.25433341810757));
#161041=CARTESIAN_POINT('Ctrl Pts',(-0.281737904202462,-7.00558707859917,
1.26084138355989));
#161042=CARTESIAN_POINT('Ctrl Pts',(-0.104003942047775,-7.01273485842708,
1.26893289423473));
#161043=CARTESIAN_POINT('Ctrl Pts',(0.0741727825111977,-7.01312142222494,
1.27702440490957));
#161044=CARTESIAN_POINT('Ctrl Pts',(0.252234662990571,-7.00671137105604,
1.2851159155844));
#161045=CARTESIAN_POINT('Ctrl Pts',(0.430183508079656,-7.00030538904913,
1.29320228969061));
#161046=CARTESIAN_POINT('Ctrl Pts',(0.608017295106995,-6.98711139578564,
1.30128866379682));
#161047=CARTESIAN_POINT('Ctrl Pts',(0.785176856287711,-6.96714603455749,
1.30937503790304));
#161048=CARTESIAN_POINT('Ctrl Pts',(0.962256743144636,-6.94718965239118,
1.31745777530806));
#161049=CARTESIAN_POINT('Ctrl Pts',(1.13866265029188,-6.92046800781922,
1.32554051271306));
#161050=CARTESIAN_POINT('Ctrl Pts',(1.3138389435012,-6.88704971617308,1.33362325011807));
#161051=CARTESIAN_POINT('Ctrl Pts',(1.48899055768737,-6.85363613253152,
1.34170484881842));
#161052=CARTESIAN_POINT('Ctrl Pts',(1.66291254770987,-6.81352784264098,
1.34978644751877));
#161053=CARTESIAN_POINT('Ctrl Pts',(1.83505767291986,-6.76684489991887,
1.35786804621912));
#161054=CARTESIAN_POINT('Ctrl Pts',(2.00718729145277,-6.72016616235398,
1.36594891693636));
#161055=CARTESIAN_POINT('Ctrl Pts',(2.17754001679949,-6.6669140498178,1.37402978765361));
#161056=CARTESIAN_POINT('Ctrl Pts',(2.34558220662477,-6.60725893805179,
1.38211065837086));
#161057=CARTESIAN_POINT('Ctrl Pts',(2.51368048924321,-6.54758391329936,
1.39019422649766));
#161058=CARTESIAN_POINT('Ctrl Pts',(2.67946635625044,-6.48150174261075,
1.39827779462447));
#161059=CARTESIAN_POINT('Ctrl Pts',(2.84242424131525,-6.40923170082682,
1.40636136275128));
#161060=CARTESIAN_POINT('Ctrl Pts',(2.93077163503861,-6.37005059686643,
1.4107438581163));
#161061=CARTESIAN_POINT('Ctrl Pts',(3.01828816610743,-6.32905155411584,
1.41512635348131));
#161062=CARTESIAN_POINT('Ctrl Pts',(3.10489448994163,-6.28627526988996,
1.41950884884632));
#161063=CARTESIAN_POINT('Ctrl Pts',(3.27771823665414,-6.20091478600073,
1.42825416022083));
#161064=CARTESIAN_POINT('Ctrl Pts',(3.44697940375194,-6.10844346605245,
1.43699947159534));
#161065=CARTESIAN_POINT('Ctrl Pts',(3.61211310649541,-6.00918176363339,
1.44574478296985));
#161066=CARTESIAN_POINT('Ctrl Pts',(3.77730538342889,-5.90988485232771,
1.45449319637334));
#161067=CARTESIAN_POINT('Ctrl Pts',(3.93836704090803,-5.80379289000895,
1.46324160977681));
#161068=CARTESIAN_POINT('Ctrl Pts',(4.09476082786269,-5.69127053698041,
1.47199002318029));
#161069=CARTESIAN_POINT('Ctrl Pts',(4.25295023698565,-5.57745626797834,
1.48083888075966));
#161070=CARTESIAN_POINT('Ctrl Pts',(4.40636368954346,-5.45706319406896,
1.48968773833904));
#161071=CARTESIAN_POINT('Ctrl Pts',(4.55447803406386,-5.33051183281022,
1.49853659591841));
#161072=CARTESIAN_POINT('Ctrl Pts',(4.70102050150528,-5.20530350949099,
1.50729154418434));
#161073=CARTESIAN_POINT('Ctrl Pts',(4.84237559824804,-5.07406717295695,
1.51604649245028));
#161074=CARTESIAN_POINT('Ctrl Pts',(4.97807157499556,-4.93724922975549,
1.52480144071622));
#161075=CARTESIAN_POINT('Ctrl Pts',(5.11595085122566,-4.79822993503458,
1.53369725295231));
#161076=CARTESIAN_POINT('Ctrl Pts',(5.24798713546572,-4.65344808564039,
1.54259306518839));
#161077=CARTESIAN_POINT('Ctrl Pts',(5.37372534685965,-4.50341009225432,
1.55148887742448));
#161078=CARTESIAN_POINT('Ctrl Pts',(5.49946355825359,-4.35337209886826,
1.56038468966057));
#161079=CARTESIAN_POINT('Ctrl Pts',(5.61890351354897,-4.19807819035687,
1.56928050189667));
#161080=CARTESIAN_POINT('Ctrl Pts',(5.73163312037252,-4.03806987754654,
1.57817631413276));
#161081=CARTESIAN_POINT('Ctrl Pts',(5.84190041495611,-3.88155656873942,
1.58687781834303));
#161082=CARTESIAN_POINT('Ctrl Pts',(5.94576623752495,-3.72050582006927,
1.5955793225533));
#161083=CARTESIAN_POINT('Ctrl Pts',(6.04287839307084,-3.55545317632754,
1.60428082676357));
#161084=CARTESIAN_POINT('Ctrl Pts',(6.13996557177791,-3.39044298343305,
1.61298009298348));
#161085=CARTESIAN_POINT('Ctrl Pts',(6.23030240926093,-3.22143319194772,
1.62167935920339));
#161086=CARTESIAN_POINT('Ctrl Pts',(6.31358137924273,-3.04898618071311,
1.6303786254233));
#161087=CARTESIAN_POINT('Ctrl Pts',(6.39851486807195,-2.87311313250504,
1.63925072158962));
#161088=CARTESIAN_POINT('Ctrl Pts',(6.47610696232078,-2.69366511636206,
1.64812281775594));
#161089=CARTESIAN_POINT('Ctrl Pts',(6.54608126140386,-2.51126396095617,
1.65699491392227));
#161090=CARTESIAN_POINT('Ctrl Pts',(6.61465203606897,-2.33252135560124,
1.66568905612877));
#161091=CARTESIAN_POINT('Ctrl Pts',(6.67590759491925,-2.1509432230381,1.67438319833527));
#161092=CARTESIAN_POINT('Ctrl Pts',(6.729636539265,-1.96713461966621,1.68307734054176));
#161093=CARTESIAN_POINT('Ctrl Pts',(6.78501509058346,-1.77768265297394,
1.692038413688));
#161094=CARTESIAN_POINT('Ctrl Pts',(6.83239738946693,-1.58586136081559,
1.70099948683424));
#161095=CARTESIAN_POINT('Ctrl Pts',(6.87160723836469,-1.39235071880399,
1.70996055998047));
#161096=CARTESIAN_POINT('Ctrl Pts',(6.91081708726246,-1.19884007679238,
1.71892163312671));
#161097=CARTESIAN_POINT('Ctrl Pts',(6.94185440853548,-1.00364040257306,
1.72788270627295));
#161098=CARTESIAN_POINT('Ctrl Pts',(6.9646004601257,-0.80744473081255,1.73684377941919));
#161099=CARTESIAN_POINT('Ctrl Pts',(6.98611826354928,-0.621843292217489,
1.74532096983004));
#161100=CARTESIAN_POINT('Ctrl Pts',(7.00022244399467,-0.435295819209708,
1.75379816024087));
#161101=CARTESIAN_POINT('Ctrl Pts',(7.00684800478492,-0.248410145408003,
1.76227535065171));
#161102=CARTESIAN_POINT('Ctrl Pts',(7.00978125769814,-0.165672553153999,
1.76602835273798));
#161103=CARTESIAN_POINT('Ctrl Pts',(7.01124938711065,-0.0828687677121652,
1.76978135482426));
#161104=CARTESIAN_POINT('Ctrl Pts',(7.01124999980813,-5.18707572911836E-5,
1.77353435691053));
#161105=CARTESIAN_POINT('Ctrl Pts',(7.01124999980813,-5.18702183956429E-5,
1.77353435693495));
#161106=CARTESIAN_POINT('Ctrl Pts',(7.01125130796046,0.176769884228194,
1.78154736439763));
#161107=CARTESIAN_POINT('Ctrl Pts',(7.00455917992508,0.353638611934562,
1.78956037186032));
#161108=CARTESIAN_POINT('Ctrl Pts',(6.99118901390433,0.530002579581904,
1.797573379323));
#161109=CARTESIAN_POINT('Ctrl Pts',(6.97781578052973,0.706407008259656,
1.80558822511209));
#161110=CARTESIAN_POINT('Ctrl Pts',(6.95776147010324,0.882306078325773,
1.8136030709012));
#161111=CARTESIAN_POINT('Ctrl Pts',(6.93109350035504,1.05715157467423,1.82161791669029));
#161112=CARTESIAN_POINT('Ctrl Pts',(6.90442269778751,1.23201564407883,1.82963361386064));
#161113=CARTESIAN_POINT('Ctrl Pts',(6.87113689907918,1.40582555445287,1.83764931103099));
#161114=CARTESIAN_POINT('Ctrl Pts',(6.83135485206238,1.57804228324331,1.84566500820135));
#161115=CARTESIAN_POINT('Ctrl Pts',(6.79154449996455,1.7503815449055,1.8536864085714));
#161116=CARTESIAN_POINT('Ctrl Pts',(6.74522875642327,1.92112500394349,1.86170780894145));
#161117=CARTESIAN_POINT('Ctrl Pts',(6.69257671255988,2.08974723567258,1.86972920931149));
#161118=CARTESIAN_POINT('Ctrl Pts',(6.65524652701859,2.20930003429072,1.87541636487362));
#161119=CARTESIAN_POINT('Ctrl Pts',(6.6147322762983,2.32778683862197,1.88110352043573));
#161120=CARTESIAN_POINT('Ctrl Pts',(6.57110895151814,2.44502632087635,1.88679067599786));
#161121=CARTESIAN_POINT('Origin',(0.,0.,50.));
#161122=CARTESIAN_POINT('',(7.01124998147128,0.000509724478514493,3.77353435695081));
#161123=CARTESIAN_POINT('Ctrl Pts',(6.57110895151814,2.44502632087635,1.88679067599786));
#161124=CARTESIAN_POINT('Ctrl Pts',(6.54881191176188,2.50495053366855,1.88969753223378));
#161125=CARTESIAN_POINT('Ctrl Pts',(6.52570281864319,2.5645489697426,1.89260438846969));
#161126=CARTESIAN_POINT('Ctrl Pts',(6.50179287697683,2.62379800049344,1.89551124470561));
#161127=CARTESIAN_POINT('Ctrl Pts',(6.42183274031803,2.82193987226578,1.90523241530129));
#161128=CARTESIAN_POINT('Ctrl Pts',(6.33286264442998,3.01629711353528,1.91495358589697));
#161129=CARTESIAN_POINT('Ctrl Pts',(6.23524423677873,3.20614345752302,1.92467475649266));
#161130=CARTESIAN_POINT('Ctrl Pts',(6.1375012290525,3.39623212126647,1.93440833518446));
#161131=CARTESIAN_POINT('Ctrl Pts',(6.03108785351913,3.58179832928602,1.94414191387626));
#161132=CARTESIAN_POINT('Ctrl Pts',(5.9164122242712,3.76213941195622,1.95387549256807));
#161133=CARTESIAN_POINT('Ctrl Pts',(5.80193074154801,3.94217517609713,1.96359259225305));
#161134=CARTESIAN_POINT('Ctrl Pts',(5.67921498599119,4.11700345412605,1.97330969193804));
#161135=CARTESIAN_POINT('Ctrl Pts',(5.54871539223631,4.285951943088,1.98302679162303));
#161136=CARTESIAN_POINT('Ctrl Pts',(5.41856219452529,4.45445197787085,1.99271809839332));
#161137=CARTESIAN_POINT('Ctrl Pts',(5.28066643653707,4.61710334255045,2.00240940516362));
#161138=CARTESIAN_POINT('Ctrl Pts',(5.13551887243857,4.77326643644865,2.01210071193392));
#161139=CARTESIAN_POINT('Ctrl Pts',(4.99129585024135,4.92843482316981,2.02173028829046));
#161140=CARTESIAN_POINT('Ctrl Pts',(4.83991312762028,5.07719727207463,2.03135986464701));
#161141=CARTESIAN_POINT('Ctrl Pts',(4.68189530183761,5.21895420032893,2.04098944100355));
#161142=CARTESIAN_POINT('Ctrl Pts',(4.60975160855841,5.28367391344689,2.04538586399972));
#161143=CARTESIAN_POINT('Ctrl Pts',(4.53622547746523,5.34693377424892,2.04978228699588));
#161144=CARTESIAN_POINT('Ctrl Pts',(4.46136984459352,5.40867873627669,2.05417870999204));
#161145=CARTESIAN_POINT('Ctrl Pts',(4.32760616633295,5.51901423032092,2.06203492185741));
#161146=CARTESIAN_POINT('Ctrl Pts',(4.18964934262517,5.62446438578487,2.06989113372279));
#161147=CARTESIAN_POINT('Ctrl Pts',(4.0479102567175,5.72468768720716,2.07774734558816));
#161148=CARTESIAN_POINT('Ctrl Pts',(3.9062107971707,5.82488296894325,2.08560136107217));
#161149=CARTESIAN_POINT('Ctrl Pts',(3.76073148972948,5.91985408365099,2.09345537655617));
#161150=CARTESIAN_POINT('Ctrl Pts',(3.6119148097489,6.00930095515415,2.10130939204018));
#161151=CARTESIAN_POINT('Ctrl Pts',(3.46310945214693,6.09874102129555,2.10916280996928));
#161152=CARTESIAN_POINT('Ctrl Pts',(3.31096755453269,6.1826574852981,2.11701622789838));
#161153=CARTESIAN_POINT('Ctrl Pts',(3.15595874177207,6.26079475647721,2.12486964582749));
#161154=CARTESIAN_POINT('Ctrl Pts',(3.0008708088336,6.33897191077445,2.13272707232754));
#161155=CARTESIAN_POINT('Ctrl Pts',(2.84291337771074,6.41136380665686,2.14058449882761));
#161156=CARTESIAN_POINT('Ctrl Pts',(2.68257905108324,6.47776166566735,2.14844192532766));
#161157=CARTESIAN_POINT('Ctrl Pts',(2.52220354053244,6.54417657981748,2.15630137010825));
#161158=CARTESIAN_POINT('Ctrl Pts',(2.35945027544116,6.60459425709277,2.16416081488881));
#161159=CARTESIAN_POINT('Ctrl Pts',(2.19482919393369,6.65885510969839,2.1720202596694));
#161160=CARTESIAN_POINT('Ctrl Pts',(2.03004440777395,6.71316992109183,2.17988752014201));
#161161=CARTESIAN_POINT('Ctrl Pts',(1.86338846141331,6.76131557379169,2.18775478061465));
#161162=CARTESIAN_POINT('Ctrl Pts',(1.69538428261545,6.80318298274863,2.19562204108727));
#161163=CARTESIAN_POINT('Ctrl Pts',(1.5727780068827,6.83373702684158,2.20136341915101));
#161164=CARTESIAN_POINT('Ctrl Pts',(1.44945394977381,6.86094846313475,2.20710479721472));
#161165=CARTESIAN_POINT('Ctrl Pts',(1.32561746232475,6.8847922921523,2.21284617527846));
#161166=CARTESIAN_POINT('Ctrl Pts',(1.14492041564138,6.91958421474189,2.22122375511282));
#161167=CARTESIAN_POINT('Ctrl Pts',(0.962732557221327,6.94728122495448,
2.22960133494719));
#161168=CARTESIAN_POINT('Ctrl Pts',(0.779636631868518,6.96776817099627,
2.23797891478154));
#161169=CARTESIAN_POINT('Ctrl Pts',(0.596666158168134,6.98824108001769,
2.24635075455788));
#161170=CARTESIAN_POINT('Ctrl Pts',(0.412789183680431,7.00151373752131,
2.25472259433422));
#161171=CARTESIAN_POINT('Ctrl Pts',(0.228596728856126,7.00752239368925,
2.26309443411056));
#161172=CARTESIAN_POINT('Ctrl Pts',(0.0445034355987655,7.01352781504629,
2.27146176683611));
#161173=CARTESIAN_POINT('Ctrl Pts',(-0.139904671468852,7.01227702179103,
2.27982909956166));
#161174=CARTESIAN_POINT('Ctrl Pts',(-0.324032928336835,7.00375822140181,
2.2881964322872));
#161175=CARTESIAN_POINT('Ctrl Pts',(-0.508089061088417,6.99524275787659,
2.29656048747952));
#161176=CARTESIAN_POINT('Ctrl Pts',(-0.691865234292956,6.97946497954218,
2.30492454267182));
#161177=CARTESIAN_POINT('Ctrl Pts',(-0.874767803901157,6.95646518368043,
2.31328859786414));
#161178=CARTESIAN_POINT('Ctrl Pts',(-1.05762553125399,6.9334710266827,2.32165060243957));
#161179=CARTESIAN_POINT('Ctrl Pts',(-1.23960975629789,6.9032584246089,2.33001260701502));
#161180=CARTESIAN_POINT('Ctrl Pts',(-1.42013251124371,6.86591947323945,
2.33837461159045));
#161181=CARTESIAN_POINT('Ctrl Pts',(-1.60066950234422,6.82857757729336,
2.34673727559959));
#161182=CARTESIAN_POINT('Ctrl Pts',(-1.77974446994,6.78410826993319,2.35509993960872));
#161183=CARTESIAN_POINT('Ctrl Pts',(-1.95677942634572,6.73265481360289,
2.36346260361786));
#161184=CARTESIAN_POINT('Ctrl Pts',(-2.13382636961676,6.68119787340892,
2.37182583385488));
#161185=CARTESIAN_POINT('Ctrl Pts',(-2.30883271038909,6.62275593287524,
2.38018906409187));
#161186=CARTESIAN_POINT('Ctrl Pts',(-2.4812352520754,6.55752225969217,2.38855229432889));
#161187=CARTESIAN_POINT('Ctrl Pts',(-2.65367247665255,6.49227546319697,
2.39691720702951));
#161188=CARTESIAN_POINT('Ctrl Pts',(-2.82350455007629,6.42023432597462,
2.40528211973014));
#161189=CARTESIAN_POINT('Ctrl Pts',(-2.99018749978493,6.34164058258034,
2.41364703243076));
#161190=CARTESIAN_POINT('Ctrl Pts',(-3.15692623686185,6.26302053452734,
2.42201474479665));
#161191=CARTESIAN_POINT('Ctrl Pts',(-3.32051345122711,6.17784364739914,
2.43038245716253));
#161192=CARTESIAN_POINT('Ctrl Pts',(-3.48042866702708,6.08639818416739,
2.43875016952842));
#161193=CARTESIAN_POINT('Ctrl Pts',(-3.64049217405539,5.99486792250042,
2.44712564137072));
#161194=CARTESIAN_POINT('Ctrl Pts',(-3.79687659237451,5.8970576321919,2.45550111321302));
#161195=CARTESIAN_POINT('Ctrl Pts',(-3.94908834715754,5.7933002501894,2.46387658505532));
#161196=CARTESIAN_POINT('Ctrl Pts',(-4.1013747601314,5.68949197633274,2.4722561649744));
#161197=CARTESIAN_POINT('Ctrl Pts',(-4.24948416030648,5.57973098428019,
2.48063574489348));
#161198=CARTESIAN_POINT('Ctrl Pts',(-4.39295460257362,5.46439167906431,
2.48901532481256));
#161199=CARTESIAN_POINT('Ctrl Pts',(-4.53658908447272,5.34892049848178,
2.49740448568214));
#161200=CARTESIAN_POINT('Ctrl Pts',(-4.67557375764741,5.22785847119752,
2.50579364655172));
#161201=CARTESIAN_POINT('Ctrl Pts',(-4.80948121262479,5.10161905946624,
2.51418280742131));
#161202=CARTESIAN_POINT('Ctrl Pts',(-4.89460261550951,5.02137202745653,
2.51951557356465));
#161203=CARTESIAN_POINT('Ctrl Pts',(-4.97767315107139,4.9390336635969,2.52484833970799));
#161204=CARTESIAN_POINT('Ctrl Pts',(-5.05859124150601,4.85471741853826,
2.53018110585133));
#161205=CARTESIAN_POINT('Ctrl Pts',(-5.1857527666769,4.72221574603521,2.53856146520638));
#161206=CARTESIAN_POINT('Ctrl Pts',(-5.30785359630183,4.58456025632525,
2.54694182456144));
#161207=CARTESIAN_POINT('Ctrl Pts',(-5.42446601166464,4.44216107888887,
2.55532218391649));
#161208=CARTESIAN_POINT('Ctrl Pts',(-5.54093063954313,4.29994236951103,
2.56369192251369));
#161209=CARTESIAN_POINT('Ctrl Pts',(-5.65192050908317,4.15299220491027,
2.57206166111089));
#161210=CARTESIAN_POINT('Ctrl Pts',(-5.75704484462818,4.00175726643186,
2.58043139970809));
#161211=CARTESIAN_POINT('Ctrl Pts',(-5.86204990942763,3.85069391433041,
2.58879164226465));
#161212=CARTESIAN_POINT('Ctrl Pts',(-5.96120251809666,3.69535574506099,
2.59715188482121));
#161213=CARTESIAN_POINT('Ctrl Pts',(-6.05415201487855,3.53622255284392,
2.60551212737776));
#161214=CARTESIAN_POINT('Ctrl Pts',(-6.14698098335738,3.37729570981951,
2.61386152914569));
#161215=CARTESIAN_POINT('Ctrl Pts',(-6.23362271923093,3.21458394103671,
2.62221093091362));
#161216=CARTESIAN_POINT('Ctrl Pts',(-6.31376980097288,3.04859598222245,
2.63056033268154));
#161217=CARTESIAN_POINT('Ctrl Pts',(-6.39385526816211,2.88273562972421,
2.63890331569229));
#161218=CARTESIAN_POINT('Ctrl Pts',(-6.46745588918847,2.7136044002636,2.64724629870304));
#161219=CARTESIAN_POINT('Ctrl Pts',(-6.53430957592106,2.54173659699946,
2.65558928171379));
#161220=CARTESIAN_POINT('Ctrl Pts',(-6.60110965729342,2.37000660267236,
2.66392557506191));
#161221=CARTESIAN_POINT('Ctrl Pts',(-6.66117347514114,2.19554471527738,
2.67226186841003));
#161222=CARTESIAN_POINT('Ctrl Pts',(-6.71428653058669,2.01890637417445,
2.68059816175815));
#161223=CARTESIAN_POINT('Ctrl Pts',(-6.73180848479055,1.9606335277436,2.68334829821801));
#161224=CARTESIAN_POINT('Ctrl Pts',(-6.74857435224345,1.9021239724077,2.68609843467789));
#161225=CARTESIAN_POINT('Ctrl Pts',(-6.7645775924045,1.84339810101858,2.68884857113775));
#161226=CARTESIAN_POINT('Ctrl Pts',(-6.81310307226829,1.66532784393962,
2.69718761311069));
#161227=CARTESIAN_POINT('Ctrl Pts',(-6.8545730863525,1.4854138533272,2.70552665508362));
#161228=CARTESIAN_POINT('Ctrl Pts',(-6.88887368500057,1.30424150930977,
2.71386569705655));
#161229=CARTESIAN_POINT('Ctrl Pts',(-6.92319593805141,1.12295478889478,
2.72221000357239));
#161230=CARTESIAN_POINT('Ctrl Pts',(-6.95033968674414,0.940408452339989,
2.73055431008823));
#161231=CARTESIAN_POINT('Ctrl Pts',(-6.97024261627548,0.757195108777878,
2.73889861660408));
#161232=CARTESIAN_POINT('Ctrl Pts',(-6.99016072631762,0.573842023368403,
2.7472492875516));
#161233=CARTESIAN_POINT('Ctrl Pts',(-7.00282696569165,0.389821241431179,
2.75559995849914));
#161234=CARTESIAN_POINT('Ctrl Pts',(-7.00823105916826,0.205727936385168,
2.76395062944666));
#161235=CARTESIAN_POINT('Ctrl Pts',(-7.01364327047901,0.021358093021924,
2.77231384447063));
#161236=CARTESIAN_POINT('Ctrl Pts',(-7.01177152674733,-0.163084163458303,
2.78067705949459));
#161237=CARTESIAN_POINT('Ctrl Pts',(-7.00265765997846,-0.347004696863131,
2.78904027451856));
#161238=CARTESIAN_POINT('Ctrl Pts',(-6.99353598803923,-0.531082740919804,
2.79741065185022));
#161239=CARTESIAN_POINT('Ctrl Pts',(-6.97715984707679,-0.714637844927594,
2.80578102918187));
#161240=CARTESIAN_POINT('Ctrl Pts',(-6.95362270461438,-0.897082964040355,
2.81415140651352));
#161241=CARTESIAN_POINT('Ctrl Pts',(-6.93004923143481,-1.07980969601372,
2.82253470392721));
#161242=CARTESIAN_POINT('Ctrl Pts',(-6.89929272341551,-1.26142269704876,
2.83091800134089));
#161243=CARTESIAN_POINT('Ctrl Pts',(-6.86149759690809,-1.4413456525499,
2.83930129875458));
#161244=CARTESIAN_POINT('Ctrl Pts',(-6.84915253210731,-1.50011409044292,
2.84203954464445));
#161245=CARTESIAN_POINT('Ctrl Pts',(-6.83605692651416,-1.5587023478056,
2.84477779053431));
#161246=CARTESIAN_POINT('Ctrl Pts',(-6.82221694956083,-1.61709073821631,
2.84751603642418));
#161247=CARTESIAN_POINT('Ctrl Pts',(-6.77981297178162,-1.79598554547567,
2.85590568318875));
#161248=CARTESIAN_POINT('Ctrl Pts',(-6.73033202143927,-1.9733641316168,
2.86429532995331));
#161249=CARTESIAN_POINT('Ctrl Pts',(-6.67390018366921,-2.14864676038666,
2.87268497671788));
#161250=CARTESIAN_POINT('Ctrl Pts',(-6.61752044903777,-2.32376755187697,
2.88106687737766));
#161251=CARTESIAN_POINT('Ctrl Pts',(-6.55420272092,-2.49679593235451,2.88944877803744));
#161252=CARTESIAN_POINT('Ctrl Pts',(-6.48412353651385,-2.66716488536557,
2.89783067869723));
#161253=CARTESIAN_POINT('Ctrl Pts',(-6.41409874967245,-2.83740159288559,
2.90620607307433));
#161254=CARTESIAN_POINT('Ctrl Pts',(-6.33732309494566,-3.00498268562944,
2.91458146745144));
#161255=CARTESIAN_POINT('Ctrl Pts',(-6.25402224617957,-3.16935834307057,
2.92295686182855));
#161256=CARTESIAN_POINT('Ctrl Pts',(-6.17077382624258,-3.33363054390376,
2.93132698480533));
#161257=CARTESIAN_POINT('Ctrl Pts',(-6.08100854927558,-3.4947010395989,
2.93969710778212));
#161258=CARTESIAN_POINT('Ctrl Pts',(-5.9849995091868,-3.65204154378531,
2.9480672307589));
#161259=CARTESIAN_POINT('Ctrl Pts',(-5.88903681621201,-3.80930609389201,
2.95643331316781));
#161260=CARTESIAN_POINT('Ctrl Pts',(-5.78683654163941,-3.96284396305371,
2.96479939557671));
#161261=CARTESIAN_POINT('Ctrl Pts',(-5.67871709607945,-4.11215256346296,
2.97316547798562));
#161262=CARTESIAN_POINT('Ctrl Pts',(-5.57062792117543,-4.26141936131535,
2.98152921810724));
#161263=CARTESIAN_POINT('Ctrl Pts',(-5.45662307118149,-4.40645898463984,
2.98989295822887));
#161264=CARTESIAN_POINT('Ctrl Pts',(-5.33706386300932,-4.5467984213796,
2.9982566983505));
#161265=CARTESIAN_POINT('Ctrl Pts',(-5.2175230703903,-4.68711624181399,
3.00661915021584));
#161266=CARTESIAN_POINT('Ctrl Pts',(-5.09242983843877,-4.82273506897357,
3.01498160208117));
#161267=CARTESIAN_POINT('Ctrl Pts',(-4.96218555970055,-4.95321522181294,
3.02334405394652));
#161268=CARTESIAN_POINT('Ctrl Pts',(-4.83194397380087,-5.08369267693699,
3.03170633291572));
#161269=CARTESIAN_POINT('Ctrl Pts',(-4.69655178595717,-5.2090314372549,
3.04006861188495));
#161270=CARTESIAN_POINT('Ctrl Pts',(-4.55644730890227,-5.3288286220986,
3.04843089085416));
#161271=CARTESIAN_POINT('Ctrl Pts',(-4.4163270454667,-5.44863930518307,
3.05679411204964));
#161272=CARTESIAN_POINT('Ctrl Pts',(-4.27149368438351,-5.56290695473472,
3.0651573332451));
#161273=CARTESIAN_POINT('Ctrl Pts',(-4.12241899829919,-5.6712686556856,
3.07352055444058));
#161274=CARTESIAN_POINT('Ctrl Pts',(-3.97325651111114,-5.77969417885334,
3.08188870135532));
#161275=CARTESIAN_POINT('Ctrl Pts',(-3.81984797284376,-5.88220660841301,
3.09025684827006));
#161276=CARTESIAN_POINT('Ctrl Pts',(-3.66269540106451,-5.97848550734389,
3.09862499518479));
#161277=CARTESIAN_POINT('Ctrl Pts',(-3.50549572969042,-6.07479326165448,
3.10699565008476));
#161278=CARTESIAN_POINT('Ctrl Pts',(-3.34455007043597,-6.16486359291279,
3.11536630498472));
#161279=CARTESIAN_POINT('Ctrl Pts',(-3.18038609269,-6.24842146977331,3.12373695988469));
#161280=CARTESIAN_POINT('Ctrl Pts',(-3.01608296101485,-6.33205017463787,
3.13211471018728));
#161281=CARTESIAN_POINT('Ctrl Pts',(-2.84855635538395,-6.40915525015496,
3.14049246048987));
#161282=CARTESIAN_POINT('Ctrl Pts',(-2.67835607621456,-6.4795088773382,
3.14887021079247));
#161283=CARTESIAN_POINT('Ctrl Pts',(-2.57013572790641,-6.52424261147582,
3.15419712952732));
#161284=CARTESIAN_POINT('Ctrl Pts',(-2.4608348332046,-6.5662477458062,3.15952404826219));
#161285=CARTESIAN_POINT('Ctrl Pts',(-2.35059822772696,-6.60547610201618,
3.16485096699704));
#161286=CARTESIAN_POINT('Ctrl Pts',(-2.18788037255686,-6.66338022521263,
3.17271391585551));
#161287=CARTESIAN_POINT('Ctrl Pts',(-2.0227845315506,-6.7153520709923,3.18057686471396));
#161288=CARTESIAN_POINT('Ctrl Pts',(-1.85580118382156,-6.76118543811856,
3.18843981357243));
#161289=CARTESIAN_POINT('Ctrl Pts',(-1.68894614423762,-6.80698358739587,
3.19629672062854));
#161290=CARTESIAN_POINT('Ctrl Pts',(-1.52020684742823,-6.84665253767507,
3.20415362768465));
#161291=CARTESIAN_POINT('Ctrl Pts',(-1.35009246772126,-6.88003465769631,
3.21201053474076));
#161292=CARTESIAN_POINT('Ctrl Pts',(-1.18007402925903,-6.91339795084263,
3.21986301065211));
#161293=CARTESIAN_POINT('Ctrl Pts',(-1.00868242354859,-6.94048139366133,
3.22771548656349));
#161294=CARTESIAN_POINT('Ctrl Pts',(-0.836440411758605,-6.96117763026322,
3.23556796247484));
#161295=CARTESIAN_POINT('Ctrl Pts',(-0.664239081800378,-6.98186897862208,
3.24341858371031));
#161296=CARTESIAN_POINT('Ctrl Pts',(-0.49118812271401,-6.99617606946939,
3.25126920494577));
#161297=CARTESIAN_POINT('Ctrl Pts',(-0.317818816115003,-7.00404295836507,
3.25911982618125));
#161298=CARTESIAN_POINT('Ctrl Pts',(-0.144477404799089,-7.01190858147098,
3.26696918424445));
#161299=CARTESIAN_POINT('Ctrl Pts',(0.0291818707969171,-7.0133360511738,
3.27481854230764));
#161300=CARTESIAN_POINT('Ctrl Pts',(0.202624771223616,-7.00832146555697,
3.28266790037083));
#161301=CARTESIAN_POINT('Ctrl Pts',(0.376126089262714,-7.00330519096862,
3.29051990219031));
#161302=CARTESIAN_POINT('Ctrl Pts',(0.549410504870092,-6.99184253813095,
3.29837190400979));
#161303=CARTESIAN_POINT('Ctrl Pts',(0.721945745408626,-6.97398171084399,
3.30622390582927));
#161304=CARTESIAN_POINT('Ctrl Pts',(0.848618974748946,-6.96086851342375,
3.31198874798067));
#161305=CARTESIAN_POINT('Ctrl Pts',(0.974888403198217,-6.9443075883769,
3.31775359013207));
#161306=CARTESIAN_POINT('Ctrl Pts',(1.10054604165771,-6.92433570623865,
3.32351843228348));
#161307=CARTESIAN_POINT('Ctrl Pts',(1.31100373558767,-6.89088579973248,
3.33317367807616));
#161308=CARTESIAN_POINT('Ctrl Pts',(1.51963775258519,-6.84788416589423,
3.34282892386885));
#161309=CARTESIAN_POINT('Ctrl Pts',(1.72567728556939,-6.79556211571713,
3.35248416966154));
#161310=CARTESIAN_POINT('Ctrl Pts',(1.93285815865867,-6.74295023157767,
3.36219289994376));
#161311=CARTESIAN_POINT('Ctrl Pts',(2.13741569195809,-6.68091445029618,
3.37190163022599));
#161312=CARTESIAN_POINT('Ctrl Pts',(2.33858964665929,-6.60973713751447,
3.38161036050822));
#161313=CARTESIAN_POINT('Ctrl Pts',(2.54073163563352,-6.53821732473898,
3.39136580848646));
#161314=CARTESIAN_POINT('Ctrl Pts',(2.73945737179978,-6.45746782909917,
3.40112125646469));
#161315=CARTESIAN_POINT('Ctrl Pts',(2.93401967882751,-6.36782184791259,
3.41087670444293));
#161316=CARTESIAN_POINT('Ctrl Pts',(3.12877465504619,-6.27808709301166,
3.42064181294739));
#161317=CARTESIAN_POINT('Ctrl Pts',(3.31935792518545,-6.17943825691252,
3.43040692145185));
#161318=CARTESIAN_POINT('Ctrl Pts',(3.50504459134553,-6.07225567439147,
3.44017202995631));
#161319=CARTESIAN_POINT('Ctrl Pts',(3.69047816886052,-5.96521918041382,
3.44992382873783));
#161320=CARTESIAN_POINT('Ctrl Pts',(3.87102844849001,-5.84967220600856,
3.45967562751936));
#161321=CARTESIAN_POINT('Ctrl Pts',(4.04599834227271,-5.72603911764725,
3.46942742630088));
#161322=CARTESIAN_POINT('Ctrl Pts',(4.12230386678096,-5.67212191252108,
3.47368025005722));
#161323=CARTESIAN_POINT('Ctrl Pts',(4.19754838569729,-5.6166674017912,3.47793307381355));
#161324=CARTESIAN_POINT('Ctrl Pts',(4.27167559387015,-5.55971349830493,
3.48218589756989));
#161325=CARTESIAN_POINT('Ctrl Pts',(4.41169191776097,-5.45213523663908,
3.4902189095124));
#161326=CARTESIAN_POINT('Ctrl Pts',(4.54778793700469,-5.33915192181211,
3.49825192145491));
#161327=CARTESIAN_POINT('Ctrl Pts',(4.67951674515051,-5.22108701271642,
3.50628493339742));
#161328=CARTESIAN_POINT('Ctrl Pts',(4.81116086930135,-5.10309800355718,
3.51431278118828));
#161329=CARTESIAN_POINT('Ctrl Pts',(4.9384430989766,-4.9800341463838,3.52234062897914));
#161330=CARTESIAN_POINT('Ctrl Pts',(5.06094843303202,-4.85226004256684,
3.53036847677));
#161331=CARTESIAN_POINT('Ctrl Pts',(5.18339845173464,-4.72454363313262,
3.53839269971271));
#161332=CARTESIAN_POINT('Ctrl Pts',(5.30107561634916,-4.59212147588672,
3.54641692265544));
#161333=CARTESIAN_POINT('Ctrl Pts',(5.41360077606581,-4.4553959644323,3.55444114559815));
#161334=CARTESIAN_POINT('Ctrl Pts',(5.5261123275988,-4.31868698782107,3.56246439813478));
#161335=CARTESIAN_POINT('Ctrl Pts',(5.63347287649328,-4.17767597157517,
3.5704876506714));
#161336=CARTESIAN_POINT('Ctrl Pts',(5.73534256614378,-4.03279955012387,
3.57851090320803));
#161337=CARTESIAN_POINT('Ctrl Pts',(5.83720390685092,-3.88793500232253,
3.58653349818222));
#161338=CARTESIAN_POINT('Ctrl Pts',(5.93357507709479,-3.7392059825822,3.59455609315643));
#161339=CARTESIAN_POINT('Ctrl Pts',(6.02415887192994,-3.58707909701583,
3.60257868813062));
#161340=CARTESIAN_POINT('Ctrl Pts',(6.11477671915454,-3.43489502369349,
3.61060429897017));
#161341=CARTESIAN_POINT('Ctrl Pts',(6.19960265975807,-3.27931084957656,
3.61862990980972));
#161342=CARTESIAN_POINT('Ctrl Pts',(6.27838469183871,-3.12081915909675,
3.62665552064927));
#161343=CARTESIAN_POINT('Ctrl Pts',(6.32484158600727,-3.02735835976525,
3.63138813471829));
#161344=CARTESIAN_POINT('Ctrl Pts',(6.36919768915796,-2.93288697902556,
3.63612074878732));
#161345=CARTESIAN_POINT('Ctrl Pts',(6.41140909568868,-2.83750946610236,
3.64085336285634));
#161346=CARTESIAN_POINT('Ctrl Pts',(6.48937692854863,-2.66133959645394,
3.64959487831509));
#161347=CARTESIAN_POINT('Ctrl Pts',(6.56006375811123,-2.48199048378617,
3.65833639377386));
#161348=CARTESIAN_POINT('Ctrl Pts',(6.62324011041767,-2.30006891250123,
3.66707790923261));
#161349=CARTESIAN_POINT('Ctrl Pts',(6.68735494721308,-2.11544489692144,
3.67594927987243));
#161350=CARTESIAN_POINT('Ctrl Pts',(6.74373430442291,-1.9281716611185,3.68482065051225));
#161351=CARTESIAN_POINT('Ctrl Pts',(6.79219060571534,-1.73890003684293,
3.69369202115208));
#161352=CARTESIAN_POINT('Ctrl Pts',(6.839973679427,-1.5522580577181,3.70244013741148));
#161353=CARTESIAN_POINT('Ctrl Pts',(6.88005238733607,-1.36367313327642,
3.71118825367088));
#161354=CARTESIAN_POINT('Ctrl Pts',(6.91229803400266,-1.17378126225587,
3.71993636993028));
#161355=CARTESIAN_POINT('Ctrl Pts',(6.94522515604355,-0.979876240709369,
3.72886936776033));
#161356=CARTESIAN_POINT('Ctrl Pts',(6.96998440141852,-0.78460870798043,
3.73780236559036));
#161357=CARTESIAN_POINT('Ctrl Pts',(6.98649418571502,-0.588664212832904,
3.74673536342041));
#161358=CARTESIAN_POINT('Ctrl Pts',(7.00300397001153,-0.392719717685374,
3.75566836125045));
#161359=CARTESIAN_POINT('Ctrl Pts',(7.01126427505398,-0.196098560856857,
3.76460135908049));
#161360=CARTESIAN_POINT('Ctrl Pts',(7.01124998147134,0.000509723592105507,
3.77353435691053));
#161361=CARTESIAN_POINT('Ctrl Pts',(7.01124998147128,0.000509724478513097,
3.77353435695083));
#161362=CARTESIAN_POINT('Ctrl Pts',(7.0112361212336,0.191157015833389,3.78219651401479));
#161363=CARTESIAN_POINT('Ctrl Pts',(7.00344264641733,0.381774601939896,
3.79085867107877));
#161364=CARTESIAN_POINT('Ctrl Pts',(6.9878983077323,0.571755020347058,3.79952082814276));
#161365=CARTESIAN_POINT('Ctrl Pts',(6.97221302745539,0.763458004322272,
3.80826152558279));
#161366=CARTESIAN_POINT('Ctrl Pts',(6.94863393904671,0.954525375757643,
3.81700222302283));
#161367=CARTESIAN_POINT('Ctrl Pts',(6.91723719363269,1.14431471611814,3.82574292046287));
#161368=CARTESIAN_POINT('Ctrl Pts',(6.88584628000161,1.3340688040911,3.8344819943636));
#161369=CARTESIAN_POINT('Ctrl Pts',(6.84664065413371,1.52254506505955,3.84322106826431));
#161370=CARTESIAN_POINT('Ctrl Pts',(6.79974792207753,1.70910934661956,3.85196014216504));
#161371=CARTESIAN_POINT('Ctrl Pts',(6.75286578113278,1.89563149109329,3.86069724227364));
#161372=CARTESIAN_POINT('Ctrl Pts',(6.69830006769018,2.08024225306533,3.86943434238223));
#161373=CARTESIAN_POINT('Ctrl Pts',(6.63622901049916,2.26231984535992,3.87817144249082));
#161374=CARTESIAN_POINT('Ctrl Pts',(6.61536704571558,2.32351577934635,3.88110796529267));
#161375=CARTESIAN_POINT('Ctrl Pts',(6.59365768196524,2.38442567898503,3.88404448809452));
#161376=CARTESIAN_POINT('Ctrl Pts',(6.57110895151813,2.44502632087638,3.88698101089636));
#161377=CARTESIAN_POINT('',(7.01124720379832,-0.00626176734468637,3.22646564312318));
#161378=CARTESIAN_POINT('Ctrl Pts',(6.57110895151814,2.44502632087637,3.33981554959537));
#161379=CARTESIAN_POINT('Ctrl Pts',(6.59116786340787,2.39111716891718,3.33721595673525));
#161380=CARTESIAN_POINT('Ctrl Pts',(6.61056612747059,2.33695364996059,3.33461636387513));
#161381=CARTESIAN_POINT('Ctrl Pts',(6.62929711484677,2.28255258988358,3.33201677101501));
#161382=CARTESIAN_POINT('Ctrl Pts',(6.68657087311147,2.11621041573025,3.32406799340565));
#161383=CARTESIAN_POINT('Ctrl Pts',(6.73757578283827,1.9477226746472,3.3161192157963));
#161384=CARTESIAN_POINT('Ctrl Pts',(6.78216126708799,1.77761500604361,3.30817043818693));
#161385=CARTESIAN_POINT('Ctrl Pts',(6.82677318622039,1.60740648003458,3.30021694772075));
#161386=CARTESIAN_POINT('Ctrl Pts',(6.86495798444076,1.43557646827349,3.29226345725457));
#161387=CARTESIAN_POINT('Ctrl Pts',(6.89661578464712,1.26266277424189,3.28430996678838));
#161388=CARTESIAN_POINT('Ctrl Pts',(6.92828431387039,1.0896904787302,3.27635378083694));
#161389=CARTESIAN_POINT('Ctrl Pts',(6.95342138408542,0.915634136736148,
3.26839759488551));
#161390=CARTESIAN_POINT('Ctrl Pts',(6.97197888062657,0.7410378199506,3.26044140893407));
#161391=CARTESIAN_POINT('Ctrl Pts',(6.99055419794468,0.566273838199409,
3.25247758265168));
#161392=CARTESIAN_POINT('Ctrl Pts',(7.00253730037618,0.390969216493217,
3.24451375636926));
#161393=CARTESIAN_POINT('Ctrl Pts',(7.00793215743723,0.215669745808578,
3.23654993008687));
#161394=CARTESIAN_POINT('Ctrl Pts',(7.01020925744765,0.141678086343953,
3.23318850109897));
#161395=CARTESIAN_POINT('Ctrl Pts',(7.01131324795972,0.0676873138780279,
3.22982707211106));
#161396=CARTESIAN_POINT('Ctrl Pts',(7.01124720379832,-0.00626176734468154,
3.22646564312316));
#161397=CARTESIAN_POINT('Ctrl Pts',(7.01124720379766,-0.00626176808276841,
3.22646564308963));
#161398=CARTESIAN_POINT('Ctrl Pts',(7.01104753157552,-0.229833016754554,
3.21630298976489));
#161399=CARTESIAN_POINT('Ctrl Pts',(7.00015032087287,-0.453038581422552,
3.20614033644017));
#161400=CARTESIAN_POINT('Ctrl Pts',(6.97868319966023,-0.674986934155092,
3.19597768311544));
#161401=CARTESIAN_POINT('Ctrl Pts',(6.96275015197123,-0.839718555761688,
3.18843489065315));
#161402=CARTESIAN_POINT('Ctrl Pts',(6.94099549368847,-1.00375802951733,
3.18089209819085));
#161403=CARTESIAN_POINT('Ctrl Pts',(6.91348882294048,-1.16674712666332,
3.17334930572856));
#161404=CARTESIAN_POINT('Ctrl Pts',(6.88289506747146,-1.34802855573501,
3.16495998263458));
#161405=CARTESIAN_POINT('Ctrl Pts',(6.8451407420748,-1.52826072867804,3.1565706595406));
#161406=CARTESIAN_POINT('Ctrl Pts',(6.80031366703914,-1.70685693377642,
3.14818133644661));
#161407=CARTESIAN_POINT('Ctrl Pts',(6.75552797832865,-1.88528825101159,
3.13979975874429));
#161408=CARTESIAN_POINT('Ctrl Pts',(6.70368263690095,-2.0620862940113,3.13141818104197));
#161409=CARTESIAN_POINT('Ctrl Pts',(6.64491664019896,-2.2366737373401,3.12303660333965));
#161410=CARTESIAN_POINT('Ctrl Pts',(6.58619625109565,-2.41112568540812,
3.11466153048118));
#161411=CARTESIAN_POINT('Ctrl Pts',(6.52056601942359,-2.58337014372758,
3.1062864576227));
#161412=CARTESIAN_POINT('Ctrl Pts',(6.44821510041239,-2.75284372627901,
3.09791138476423));
#161413=CARTESIAN_POINT('Ctrl Pts',(6.37590970147637,-2.9222106833677,3.08954158114009));
#161414=CARTESIAN_POINT('Ctrl Pts',(6.29689217492977,-3.08880993908589,
3.08117177751596));
#161415=CARTESIAN_POINT('Ctrl Pts',(6.2114004049943,-3.25209648862648,3.07280197389181));
#161416=CARTESIAN_POINT('Ctrl Pts',(6.12594987710188,-3.4153042671823,3.06443620794056));
#161417=CARTESIAN_POINT('Ctrl Pts',(6.03403148628287,-3.57520223562449,
3.0560704419893));
#161418=CARTESIAN_POINT('Ctrl Pts',(5.93593001954654,-3.73126806401606,
3.04770467603804));
#161419=CARTESIAN_POINT('Ctrl Pts',(5.83785594686929,-3.88729031225879,
3.0393412461608));
#161420=CARTESIAN_POINT('Ctrl Pts',(5.73360241458621,-4.03948227536512,
3.03097781628356));
#161421=CARTESIAN_POINT('Ctrl Pts',(5.62349896132917,-4.1873483249462,3.02261438640632));
#161422=CARTESIAN_POINT('Ctrl Pts',(5.5134124108012,-4.33519167460552,3.01425224045601));
#161423=CARTESIAN_POINT('Ctrl Pts',(5.39747792611674,-4.47871017123534,
3.0058900945057));
#161424=CARTESIAN_POINT('Ctrl Pts',(5.27606721836805,-4.61743882144226,
2.99752794855539));
#161425=CARTESIAN_POINT('Ctrl Pts',(5.15465894855081,-4.75616468597281,
2.98916597051727));
#161426=CARTESIAN_POINT('Ctrl Pts',(5.02777489172064,-4.89010064876383,
2.98080399247916));
#161427=CARTESIAN_POINT('Ctrl Pts',(4.89582600964123,-5.01881602031998,
2.97244201444104));
#161428=CARTESIAN_POINT('Ctrl Pts',(4.76386217056269,-5.14754598234231,
2.96407908853512));
#161429=CARTESIAN_POINT('Ctrl Pts',(4.62683259727144,-5.27105394415241,
2.95571616262919));
#161430=CARTESIAN_POINT('Ctrl Pts',(4.48518425625931,-5.38894690546341,
2.94735323672326));
#161431=CARTESIAN_POINT('Ctrl Pts',(4.34345230361911,-5.50690945616997,
2.93898537438218));
#161432=CARTESIAN_POINT('Ctrl Pts',(4.19709638768098,-5.61925017217225,
2.93061751204111));
#161433=CARTESIAN_POINT('Ctrl Pts',(4.04659643642701,-5.72561645966582,
2.92224964970003));
#161434=CARTESIAN_POINT('Ctrl Pts',(3.89605126911981,-5.8320147037393,2.91387927332684));
#161435=CARTESIAN_POINT('Ctrl Pts',(3.74135985549983,-5.93243475478525,
2.90550889695365));
#161436=CARTESIAN_POINT('Ctrl Pts',(3.58303069217646,-6.02656764845642,
2.89713852058046));
#161437=CARTESIAN_POINT('Ctrl Pts',(3.42456708812255,-6.1207804724116,2.88876103673894));
#161438=CARTESIAN_POINT('Ctrl Pts',(3.26245984774095,-6.20869530810382,
2.88038355289741));
#161439=CARTESIAN_POINT('Ctrl Pts',(3.09724264181671,-6.29004885356324,
2.87200606905589));
#161440=CARTESIAN_POINT('Ctrl Pts',(2.99211549249737,-6.3418138393789,2.8666755044225));
#161441=CARTESIAN_POINT('Ctrl Pts',(2.88572966766815,-6.39092327569232,
2.86134493978911));
#161442=CARTESIAN_POINT('Ctrl Pts',(2.77822683336806,-6.43731949066175,
2.85601437515572));
#161443=CARTESIAN_POINT('Ctrl Pts',(2.61956441318462,-6.50579522716049,
2.84814704504126));
#161444=CARTESIAN_POINT('Ctrl Pts',(2.4581382896286,-6.56850053935805,2.84027971492681));
#161445=CARTESIAN_POINT('Ctrl Pts',(2.29442486448226,-6.62519743885008,
2.83241238481235));
#161446=CARTESIAN_POINT('Ctrl Pts',(2.13083753904616,-6.68185066774764,
2.82455111448222));
#161447=CARTESIAN_POINT('Ctrl Pts',(1.96496677326853,-6.73250456367311,
2.81668984415209));
#161448=CARTESIAN_POINT('Ctrl Pts',(1.79731079744992,-6.77696838268189,
2.80882857382196));
#161449=CARTESIAN_POINT('Ctrl Pts',(1.6297497338721,-6.82140703014116,2.80097175385979));
#161450=CARTESIAN_POINT('Ctrl Pts',(1.46040583769453,-6.85966247432036,
2.79311493389762));
#161451=CARTESIAN_POINT('Ctrl Pts',(1.28979418668937,-6.89159324963991,
2.78525811393544));
#161452=CARTESIAN_POINT('Ctrl Pts',(1.1192236155632,-6.92351633666631,2.77740318573864));
#161453=CARTESIAN_POINT('Ctrl Pts',(0.947386269685783,-6.94911770765619,
2.76954825754183));
#161454=CARTESIAN_POINT('Ctrl Pts',(0.77480909498942,-6.96830663998232,
2.76169332934503));
#161455=CARTESIAN_POINT('Ctrl Pts',(0.602260058155004,-6.98749244364714,
2.75383968185574));
#161456=CARTESIAN_POINT('Ctrl Pts',(0.428971811777411,-7.00026785080396,
2.74598603436646));
#161457=CARTESIAN_POINT('Ctrl Pts',(0.2554776700235,-7.00659387453129,2.73813238687718));
#161458=CARTESIAN_POINT('Ctrl Pts',(0.0819260470773751,-7.01292199416446,
2.73027613735755));
#161459=CARTESIAN_POINT('Ctrl Pts',(-0.0918312262740901,-7.0127964482853,
2.72241988783793));
#161460=CARTESIAN_POINT('Ctrl Pts',(-0.265259376653958,-7.00623037200442,
2.7145636383183));
#161461=CARTESIAN_POINT('Ctrl Pts',(-0.391946857028583,-7.0014339208046,
2.7088247288353));
#161462=CARTESIAN_POINT('Ctrl Pts',(-0.518458670811295,-6.99320179469858,
2.70308581935229));
#161463=CARTESIAN_POINT('Ctrl Pts',(-0.644587821142319,-6.98155663898353,
2.69734690986928));
#161464=CARTESIAN_POINT('Ctrl Pts',(-0.856167445565318,-6.96202207725794,
2.68771998136127));
#161465=CARTESIAN_POINT('Ctrl Pts',(-1.06656328868496,-6.93289256428452,
2.67809305285326));
#161466=CARTESIAN_POINT('Ctrl Pts',(-1.27499597528205,-6.8943463668077,
2.66846612434526));
#161467=CARTESIAN_POINT('Ctrl Pts',(-1.48453805740377,-6.85559500487386,
2.65878795593061));
#161468=CARTESIAN_POINT('Ctrl Pts',(-1.6920959842416,-6.80732651379863,
2.64910978751596));
#161469=CARTESIAN_POINT('Ctrl Pts',(-1.8968979678959,-6.74977071180143,
2.63943161910131));
#161470=CARTESIAN_POINT('Ctrl Pts',(-2.10266028244323,-6.69194502660416,
2.62970806907487));
#161471=CARTESIAN_POINT('Ctrl Pts',(-2.30564070360076,-6.62474476636611,
2.61998451904842));
#161472=CARTESIAN_POINT('Ctrl Pts',(-2.50507743212523,-6.54845123838888,
2.61026096902198));
#161473=CARTESIAN_POINT('Ctrl Pts',(-2.70471732197539,-6.47207999205757,
2.60052751385254));
#161474=CARTESIAN_POINT('Ctrl Pts',(-2.90080625793617,-6.38659697746056,
2.59079405868311));
#161475=CARTESIAN_POINT('Ctrl Pts',(-3.09260159054713,-6.29233199733178,
2.58106060351368));
#161476=CARTESIAN_POINT('Ctrl Pts',(-3.28417339240915,-6.19817687973886,
2.57133849234566));
#161477=CARTESIAN_POINT('Ctrl Pts',(-3.47146155099836,-6.09526027644286,
2.56161638117764));
#161478=CARTESIAN_POINT('Ctrl Pts',(-3.65374801202568,-5.98395788981828,
2.55189427000961));
#161479=CARTESIAN_POINT('Ctrl Pts',(-3.73633925578969,-5.93352845861741,
2.54748932820069));
#161480=CARTESIAN_POINT('Ctrl Pts',(-3.81790402458919,-5.88137818228995,
2.54308438639177));
#161481=CARTESIAN_POINT('Ctrl Pts',(-3.89837706152768,-5.82754518203461,
2.53867944458285));
#161482=CARTESIAN_POINT('Ctrl Pts',(-4.04553163005916,-5.72910510537409,
2.53062448187785));
#161483=CARTESIAN_POINT('Ctrl Pts',(-4.18910593294209,-5.62498673949934,
2.52256951917284));
#161484=CARTESIAN_POINT('Ctrl Pts',(-4.32863101602867,-5.51548548085974,
2.51451455646784));
#161485=CARTESIAN_POINT('Ctrl Pts',(-4.46806543240845,-5.40605537873403,
2.50646482806857));
#161486=CARTESIAN_POINT('Ctrl Pts',(-4.60345558165775,-5.29124957136967,
2.49841509966931));
#161487=CARTESIAN_POINT('Ctrl Pts',(-4.73436169629557,-5.17140656796092,
2.49036537127004));
#161488=CARTESIAN_POINT('Ctrl Pts',(-4.86520750588745,-5.0516187731102,
2.4823193511715));
#161489=CARTESIAN_POINT('Ctrl Pts',(-4.99157312601222,-4.92679864862529,
2.47427333107296));
#161490=CARTESIAN_POINT('Ctrl Pts',(-5.11305210604816,-4.79732474649533,
2.46622731097442));
#161491=CARTESIAN_POINT('Ctrl Pts',(-5.23451372403499,-4.66786934906674,
2.45818244083118));
#161492=CARTESIAN_POINT('Ctrl Pts',(-5.35108983886226,-4.53376175975606,
2.45013757068795));
#161493=CARTESIAN_POINT('Ctrl Pts',(-5.46241097456368,-4.39541726204309,
2.44209270054471));
#161494=CARTESIAN_POINT('Ctrl Pts',(-5.57372174642829,-4.25708564400284,
2.43404857936724));
#161495=CARTESIAN_POINT('Ctrl Pts',(-5.67977828813721,-4.11451818964834,
2.42600445818977));
#161496=CARTESIAN_POINT('Ctrl Pts',(-5.7802516956113,-3.96816291221552,
2.41796033701231));
#161497=CARTESIAN_POINT('Ctrl Pts',(-5.88076006096164,-3.82175671315272,
2.40991341703067));
#161498=CARTESIAN_POINT('Ctrl Pts',(-5.97568120715722,-3.67156036033681,
2.40186649704902));
#161499=CARTESIAN_POINT('Ctrl Pts',(-6.06472960808963,-3.51805078747607,
2.39381957706738));
#161500=CARTESIAN_POINT('Ctrl Pts',(-6.1156619111748,-3.43024914242068,
2.38921704447706));
#161501=CARTESIAN_POINT('Ctrl Pts',(-6.16467382062123,-3.34136410659353,
2.38461451188674));
#161502=CARTESIAN_POINT('Ctrl Pts',(-6.21171869217826,-3.2514884978642,
2.38001197929643));
#161503=CARTESIAN_POINT('Ctrl Pts',(-6.30054239512107,-3.08179764512375,
2.37132210569158));
#161504=CARTESIAN_POINT('Ctrl Pts',(-6.38239382465608,-2.90849380649929,
2.36263223208672));
#161505=CARTESIAN_POINT('Ctrl Pts',(-6.45700612407809,-2.73216003852595,
2.35394235848187));
#161506=CARTESIAN_POINT('Ctrl Pts',(-6.53163751284605,-2.5557811560564,
2.34525026159742));
#161507=CARTESIAN_POINT('Ctrl Pts',(-6.59902596574914,-2.37637105548189,
2.33655816471299));
#161508=CARTESIAN_POINT('Ctrl Pts',(-6.65895292056474,-2.19453242496034,
2.32786606782853));
#161509=CARTESIAN_POINT('Ctrl Pts',(-6.7201532694509,-2.00882988654265,
2.31898927167699));
#161510=CARTESIAN_POINT('Ctrl Pts',(-6.77357138147548,-1.82059474689036,
2.31011247552542));
#161511=CARTESIAN_POINT('Ctrl Pts',(-6.81902811021397,-1.63048526353711,
2.30123567937387));
#161512=CARTESIAN_POINT('Ctrl Pts',(-6.863568952766,-1.44420620649368,2.29253773760101));
#161513=CARTESIAN_POINT('Ctrl Pts',(-6.9004661194254,-1.25612789758659,
2.28383979582816));
#161514=CARTESIAN_POINT('Ctrl Pts',(-6.9296025805661,-1.06688079836111,
2.2751418540553));
#161515=CARTESIAN_POINT('Ctrl Pts',(-6.95963773425792,-0.871796512609358,
2.26617563071442));
#161516=CARTESIAN_POINT('Ctrl Pts',(-6.98142572935617,-0.675470495382184,
2.25720940737353));
#161517=CARTESIAN_POINT('Ctrl Pts',(-6.99489582811723,-0.47860099904643,
2.24824318403265));
#161518=CARTESIAN_POINT('Ctrl Pts',(-7.00836592687828,-0.281731502710676,
2.23927696069177));
#161519=CARTESIAN_POINT('Ctrl Pts',(-7.01351811730095,-0.084318853007292,
2.23031073735089));
#161520=CARTESIAN_POINT('Ctrl Pts',(-7.01034036778413,0.112935779610404,
2.22134451401001));
#161521=CARTESIAN_POINT('Ctrl Pts',(-7.00723646838226,0.305606263221481,
2.21258666348793));
#161522=CARTESIAN_POINT('Ctrl Pts',(-6.99618509540164,0.498159174276181,
2.20382881296585));
#161523=CARTESIAN_POINT('Ctrl Pts',(-6.97722014547274,0.689946087828103,
2.19507096244377));
#161524=CARTESIAN_POINT('Ctrl Pts',(-6.95825895554909,0.881694977562244,
2.18631484825973));
#161525=CARTESIAN_POINT('Ctrl Pts',(-6.93138734864916,1.07267790347401,
2.17755873407569));
#161526=CARTESIAN_POINT('Ctrl Pts',(-6.89669110777299,1.26225129291475,
2.16880261989165));
#161527=CARTESIAN_POINT('Ctrl Pts',(-6.86164741998548,1.45372306347608,
2.15995882229431));
#161528=CARTESIAN_POINT('Ctrl Pts',(-6.81862155666545,1.64375663391736,
2.15111502469697));
#161529=CARTESIAN_POINT('Ctrl Pts',(-6.76775516826714,1.83169772203097,
2.14227122709963));
#161530=CARTESIAN_POINT('Ctrl Pts',(-6.71742360909971,2.01766272356223,
2.13352041667153));
#161531=CARTESIAN_POINT('Ctrl Pts',(-6.65941568650613,2.20157876791965,
2.12476960624344));
#161532=CARTESIAN_POINT('Ctrl Pts',(-6.59391944734918,2.38282456013242,
2.11601879581534));
#161533=CARTESIAN_POINT('Ctrl Pts',(-6.52737925176231,2.56695926188584,
2.10712850463338));
#161534=CARTESIAN_POINT('Ctrl Pts',(-6.45311007030879,2.74833759050299,
2.09823821345143));
#161535=CARTESIAN_POINT('Ctrl Pts',(-6.37136138372236,2.92632545703848,
2.08934792226946));
#161536=CARTESIAN_POINT('Ctrl Pts',(-6.28961269713594,3.10431332357397,
2.0804576310875));
#161537=CARTESIAN_POINT('Ctrl Pts',(-6.20038461379614,3.27891045438438,
2.07156733990554));
#161538=CARTESIAN_POINT('Ctrl Pts',(-6.10397786506047,3.44950442605193,
2.06267704872357));
#161539=CARTESIAN_POINT('Ctrl Pts',(-6.01631887157887,3.60461904247164,
2.05459344475404));
#161540=CARTESIAN_POINT('Ctrl Pts',(-5.92269477699021,3.75647621605263,
2.0465098407845));
#161541=CARTESIAN_POINT('Ctrl Pts',(-5.82338398339379,3.90459031710788,
2.03842623681497));
#161542=CARTESIAN_POINT('Ctrl Pts',(-5.72410160994942,4.05266203178077,
2.0303449461615));
#161543=CARTESIAN_POINT('Ctrl Pts',(-5.61913597921042,4.19699250786548,
2.02226365550803));
#161544=CARTESIAN_POINT('Ctrl Pts',(-5.50880960625082,4.33712384934749,
2.01418236485456));
#161545=CARTESIAN_POINT('Ctrl Pts',(-5.39849438982538,4.47724102032739,
2.00610189140547));
#161546=CARTESIAN_POINT('Ctrl Pts',(-5.28281973493344,4.61315961981969,
1.99802141795639));
#161547=CARTESIAN_POINT('Ctrl Pts',(-5.16214935538897,4.74445366666777,
1.9899409445073));
#161548=CARTESIAN_POINT('Ctrl Pts',(-5.04143258982531,4.87579818330139,
1.98185736490244));
#161549=CARTESIAN_POINT('Ctrl Pts',(-4.91571650574492,5.00251432843386,
1.97377378529757));
#161550=CARTESIAN_POINT('Ctrl Pts',(-4.7854030638399,5.1242115568243,1.9656902056927));
#161551=CARTESIAN_POINT('Ctrl Pts',(-4.65506242599418,5.24593418298307,
1.95760493907422));
#161552=CARTESIAN_POINT('Ctrl Pts',(-4.52012278784488,5.3626355651621,1.94951967245572));
#161553=CARTESIAN_POINT('Ctrl Pts',(-4.38102025938351,5.47396456413185,
1.94143440583724));
#161554=CARTESIAN_POINT('Ctrl Pts',(-4.24180835108692,5.58538110390836,
1.93334278156918));
#161555=CARTESIAN_POINT('Ctrl Pts',(-4.09842730155014,5.69141660436618,
1.92525115730112));
#161556=CARTESIAN_POINT('Ctrl Pts',(-3.95134388299007,5.79176208772917,
1.91715953303306));
#161557=CARTESIAN_POINT('Ctrl Pts',(-3.87166727433948,5.8461202736215,1.91277621650108));
#161558=CARTESIAN_POINT('Ctrl Pts',(-3.79090469083633,5.89880948512212,
1.90839289996912));
#161559=CARTESIAN_POINT('Ctrl Pts',(-3.70913347285415,5.94978616784275,
1.90400958343714));
#161560=CARTESIAN_POINT('Ctrl Pts',(-3.53577909345671,6.05785635946815,
1.8947169846982));
#161561=CARTESIAN_POINT('Ctrl Pts',(-3.35775526832687,6.15831162868173,
1.88542438595926));
#161562=CARTESIAN_POINT('Ctrl Pts',(-3.17570664580314,6.25080105764868,
1.87613178722032));
#161563=CARTESIAN_POINT('Ctrl Pts',(-2.99361604881069,6.34331181165829,
1.86683704591149));
#161564=CARTESIAN_POINT('Ctrl Pts',(-2.80749894707798,6.42785298311857,
1.85754230460267));
#161565=CARTESIAN_POINT('Ctrl Pts',(-2.61802323834685,6.50412030069985,
1.84824756329385));
#161566=CARTESIAN_POINT('Ctrl Pts',(-2.4287389281723,6.58031057698335,1.83896221105174));
#161567=CARTESIAN_POINT('Ctrl Pts',(-2.23610294376896,6.64824364362018,
1.82967685880963));
#161568=CARTESIAN_POINT('Ctrl Pts',(-2.04080166488643,6.70766390981963,
1.82039150656752));
#161569=CARTESIAN_POINT('Ctrl Pts',(-1.84574325221575,6.76701028415805,
1.81111770109223));
#161570=CARTESIAN_POINT('Ctrl Pts',(-1.64802632048138,6.81786495122889,
1.80184389561693));
#161571=CARTESIAN_POINT('Ctrl Pts',(-1.44835289833174,6.8600218982445,1.79257009014163));
#161572=CARTESIAN_POINT('Ctrl Pts',(-1.24927025242264,6.90205411497602,
1.78332372319007));
#161573=CARTESIAN_POINT('Ctrl Pts',(-1.04824283211687,6.93543994730127,
1.77407735623852));
#161574=CARTESIAN_POINT('Ctrl Pts',(-0.845982265906969,6.96002446606841,
1.76483098928696));
#161575=CARTESIAN_POINT('Ctrl Pts',(-0.703878521035723,6.97729699846627,
1.75833469890821));
#161576=CARTESIAN_POINT('Ctrl Pts',(-0.561166409073024,6.9902260899788,
1.75183840852947));
#161577=CARTESIAN_POINT('Ctrl Pts',(-0.418096783377079,6.99877286688386,
1.74534211815072));
#161578=CARTESIAN_POINT('Ctrl Pts',(-0.237722289166465,7.009548183824,1.7371519444111));
#161579=CARTESIAN_POINT('Ctrl Pts',(-0.056889423869269,7.01334864684188,
1.72896177067148));
#161580=CARTESIAN_POINT('Ctrl Pts',(0.123828300585204,7.01015642582063,
1.72077159693185));
#161581=CARTESIAN_POINT('Ctrl Pts',(0.304536860524118,7.00696436668254,
1.71258183853043));
#161582=CARTESIAN_POINT('Ctrl Pts',(0.485129942468523,6.99678033663585,
1.70439208012902));
#161583=CARTESIAN_POINT('Ctrl Pts',(0.665034749126982,6.97963862567065,
1.6962023217276));
#161584=CARTESIAN_POINT('Ctrl Pts',(0.84496092534677,6.96249487856838,1.68801159052535));
#161585=CARTESIAN_POINT('Ctrl Pts',(1.02419831620835,6.93839183785307,1.67982085932311));
#161586=CARTESIAN_POINT('Ctrl Pts',(1.20217976786569,6.90741560702948,1.67163012812087));
#161587=CARTESIAN_POINT('Ctrl Pts',(1.38027861073457,6.87641894521585,1.66343399455871));
#161588=CARTESIAN_POINT('Ctrl Pts',(1.55711951550437,6.83854009680515,1.65523786099655));
#161589=CARTESIAN_POINT('Ctrl Pts',(1.73214522940835,6.79391635706077,1.64704172743439));
#161590=CARTESIAN_POINT('Ctrl Pts',(1.90723594944459,6.74927604365608,1.63884254975414));
#161591=CARTESIAN_POINT('Ctrl Pts',(2.08050979909328,6.69788594002075,1.6306433720739));
#161592=CARTESIAN_POINT('Ctrl Pts',(2.25142498318926,6.63993314029375,1.62244419439365));
#161593=CARTESIAN_POINT('Ctrl Pts',(2.42250439563771,6.58192465509404,1.61423713831776));
#161594=CARTESIAN_POINT('Ctrl Pts',(2.59122028843721,6.51734099885884,1.60603008224185));
#161595=CARTESIAN_POINT('Ctrl Pts',(2.75705029625068,6.44641762736825,1.59782302616596));
#161596=CARTESIAN_POINT('Ctrl Pts',(2.83213750635506,6.41430378882573,1.59410690173206));
#161597=CARTESIAN_POINT('Ctrl Pts',(2.90663335369555,6.38089078951445,1.59039077729817));
#161598=CARTESIAN_POINT('Ctrl Pts',(2.98049102249514,6.34620357594412,1.58667465286428));
#161599=CARTESIAN_POINT('Ctrl Pts',(3.14270627245884,6.27001927292849,1.57851284565132));
#161600=CARTESIAN_POINT('Ctrl Pts',(3.30218226723319,6.18752525781849,1.57035103843836));
#161601=CARTESIAN_POINT('Ctrl Pts',(3.4583976801335,6.09894351904879,1.5621892312254));
#161602=CARTESIAN_POINT('Ctrl Pts',(3.61446761511558,6.01044427333602,1.55403502481636));
#161603=CARTESIAN_POINT('Ctrl Pts',(3.76728271123916,5.91586877054678,1.54588081840732));
#161604=CARTESIAN_POINT('Ctrl Pts',(3.91634350483618,5.81548623200395,1.53772661199827));
#161605=CARTESIAN_POINT('Ctrl Pts',(4.06682964618143,5.71414381647522,1.52949443351178));
#161606=CARTESIAN_POINT('Ctrl Pts',(4.21348897605338,5.60688287115958,1.52126225502529));
#161607=CARTESIAN_POINT('Ctrl Pts',(4.35583367523542,5.49402762608499,1.51303007653879));
#161608=CARTESIAN_POINT('Ctrl Pts',(4.49664671805326,5.38238672517176,1.50488647787748));
#161609=CARTESIAN_POINT('Ctrl Pts',(4.63323723830541,5.265271544388,1.49674287921618));
#161610=CARTESIAN_POINT('Ctrl Pts',(4.76516285886654,5.14303893539402,1.48859928055487));
#161611=CARTESIAN_POINT('Ctrl Pts',(4.89705026642743,5.02084173176481,1.48045804073286));
#161612=CARTESIAN_POINT('Ctrl Pts',(5.02427520692485,4.89353029247951,1.47231680091084));
#161613=CARTESIAN_POINT('Ctrl Pts',(5.14642961380638,4.7615006870352,1.46417556108882));
#161614=CARTESIAN_POINT('Ctrl Pts',(5.26857011421174,4.62948611229351,1.45603524809344));
#161615=CARTESIAN_POINT('Ctrl Pts',(5.38564099163647,4.49275470124292,1.44789493509806));
#161616=CARTESIAN_POINT('Ctrl Pts',(5.49727209523096,4.35173828182429,1.43975462210268));
#161617=CARTESIAN_POINT('Ctrl Pts',(5.61109338112971,4.20795514545604,1.43145459762098));
#161618=CARTESIAN_POINT('Ctrl Pts',(5.71925897298525,4.0597173999367,1.42315457313929));
#161619=CARTESIAN_POINT('Ctrl Pts',(5.82142064820782,3.90751688404793,1.4148545486576));
#161620=CARTESIAN_POINT('Ctrl Pts',(5.92167666008053,3.75815542639042,1.4067093479141));
#161621=CARTESIAN_POINT('Ctrl Pts',(6.01615060709697,3.60497805767956,1.39856414717059));
#161622=CARTESIAN_POINT('Ctrl Pts',(6.10455816450969,3.44847737104626,1.39041894642709));
#161623=CARTESIAN_POINT('Ctrl Pts',(6.19548639433195,3.28751454368182,1.3820415100763));
#161624=CARTESIAN_POINT('Ctrl Pts',(6.27999697204131,3.12303642653392,1.3736640737255));
#161625=CARTESIAN_POINT('Ctrl Pts',(6.35783226829758,2.95560406866246,1.36528663737471));
#161626=CARTESIAN_POINT('Ctrl Pts',(6.43566756455385,2.788171710791,1.35690920102392));
#161627=CARTESIAN_POINT('Ctrl Pts',(6.50682745250105,2.61778549733251,1.34853176467315));
#161628=CARTESIAN_POINT('Ctrl Pts',(6.57110895151814,2.44502632087636,1.34015432832236));
#161629=CARTESIAN_POINT('Origin',(0.,0.,-4.41670255678778));
#161630=CARTESIAN_POINT('',(2.10208451021623,-7.84862588447233,0.));
#161631=CARTESIAN_POINT('',(8.12525,4.45453136183049E-13,0.416702556787629));
#161632=CARTESIAN_POINT('Ctrl Pts',(2.10208451021623,-7.84862588447233,
1.77635683940025E-15));
#161633=CARTESIAN_POINT('Ctrl Pts',(2.30734049756823,-7.79365251231869,
0.00832438836227722));
#161634=CARTESIAN_POINT('Ctrl Pts',(2.5104411573911,-7.73062260289495,0.0166487767245511));
#161635=CARTESIAN_POINT('Ctrl Pts',(2.71075935410536,-7.65973049699728,
0.024973165086827));
#161636=CARTESIAN_POINT('Ctrl Pts',(2.91107282461945,-7.58884006368997,
0.0332973570479451));
#161637=CARTESIAN_POINT('Ctrl Pts',(3.10860370015948,-7.51008789831038,
0.0416215490090642));
#161638=CARTESIAN_POINT('Ctrl Pts',(3.30274228536127,-7.42371746222784,
0.0499457409701822));
#161639=CARTESIAN_POINT('Ctrl Pts',(3.49688087431976,-7.33734702447398,
0.0582699330923786));
#161640=CARTESIAN_POINT('Ctrl Pts',(3.68762691807514,-7.24335843006386,
0.0665941252145752));
#161641=CARTESIAN_POINT('Ctrl Pts',(3.87439200321211,-7.14204271675451,
0.0749183173367713));
#161642=CARTESIAN_POINT('Ctrl Pts',(4.06118273642806,-7.04071308995904,
0.0832436526037741));
#161643=CARTESIAN_POINT('Ctrl Pts',(4.24399117233817,-6.93205446539553,
0.0915689878707773));
#161644=CARTESIAN_POINT('Ctrl Pts',(4.42225369533016,-6.81640373046071,
0.0998943231377805));
#161645=CARTESIAN_POINT('Ctrl Pts',(4.60051640598431,-6.70075287377699,
0.108219667169107));
#161646=CARTESIAN_POINT('Ctrl Pts',(4.77423296131069,-6.57811004621418,
0.116545011200433));
#161647=CARTESIAN_POINT('Ctrl Pts',(4.94286836885875,-6.44885570086939,
0.124870355231759));
#161648=CARTESIAN_POINT('Ctrl Pts',(5.11152549662714,-6.31958470758037,
0.133196771566401));
#161649=CARTESIAN_POINT('Ctrl Pts',(5.27509994743933,-6.18370066507483,
0.141523187901042));
#161650=CARTESIAN_POINT('Ctrl Pts',(5.43308855487239,-6.04162530428813,
0.149849604235683));
#161651=CARTESIAN_POINT('Ctrl Pts',(5.48885971067159,-5.99147164314507,
0.152788891252597));
#161652=CARTESIAN_POINT('Ctrl Pts',(5.54393509745807,-5.9405468168862,0.155728178269512));
#161653=CARTESIAN_POINT('Ctrl Pts',(5.5982936114802,-5.88887053705207,0.158667465286427));
#161654=CARTESIAN_POINT('Ctrl Pts',(5.74712452149839,-5.74738345094562,
0.166715087069352));
#161655=CARTESIAN_POINT('Ctrl Pts',(5.89064187191427,-5.60020048953742,
0.174762708852277));
#161656=CARTESIAN_POINT('Ctrl Pts',(6.02840651757392,-5.44775205211951,
0.182810330635203));
#161657=CARTESIAN_POINT('Ctrl Pts',(6.16613103580062,-5.29534801915979,
0.190855608345004));
#161658=CARTESIAN_POINT('Ctrl Pts',(6.29810597726349,-5.13768180517975,
0.198900886054805));
#161659=CARTESIAN_POINT('Ctrl Pts',(6.42393006636541,-4.9752195996706,0.206946163764606));
#161660=CARTESIAN_POINT('Ctrl Pts',(6.54973363839208,-4.81278388550598,
0.214990129598681));
#161661=CARTESIAN_POINT('Ctrl Pts',(6.66938816373354,-4.64555399194908,
0.223034095432758));
#161662=CARTESIAN_POINT('Ctrl Pts',(6.78253321612534,-4.47402846824386,
0.231078061266833));
#161663=CARTESIAN_POINT('Ctrl Pts',(6.89569459095891,-4.30247820005963,
0.239123187533125));
#161664=CARTESIAN_POINT('Ctrl Pts',(7.00234443755863,-4.12663132763536,
0.247168313799416));
#161665=CARTESIAN_POINT('Ctrl Pts',(7.10216567530887,-3.94701536391291,
0.255213440065709));
#161666=CARTESIAN_POINT('Ctrl Pts',(7.20199262453546,-3.76738912309559,
0.263259026650361));
#161667=CARTESIAN_POINT('Ctrl Pts',(7.29499003409692,-3.58399364156959,
0.271304613235014));
#161668=CARTESIAN_POINT('Ctrl Pts',(7.38088672132661,-3.39738116340285,
0.279350199819667));
#161669=CARTESIAN_POINT('Ctrl Pts',(7.46682099106362,-3.21068703639666,
0.287399306601971));
#161670=CARTESIAN_POINT('Ctrl Pts',(7.54564819953609,-3.02077339122527,
0.295448413384275));
#161671=CARTESIAN_POINT('Ctrl Pts',(7.61714485605674,-2.82821353584703,
0.303497520166579));
#161672=CARTESIAN_POINT('Ctrl Pts',(7.65811538880073,-2.71786879745113,
0.308109990302005));
#161673=CARTESIAN_POINT('Ctrl Pts',(7.69667963643193,-2.60665545684858,
0.31272246043743));
#161674=CARTESIAN_POINT('Ctrl Pts',(7.73280286670624,-2.49468382508883,
0.317334930572856));
#161675=CARTESIAN_POINT('Ctrl Pts',(7.80025255645084,-2.2856091724334,0.325947385140962));
#161676=CARTESIAN_POINT('Ctrl Pts',(7.85920825178188,-2.07383061034273,
0.33455983970907));
#161677=CARTESIAN_POINT('Ctrl Pts',(7.90948727930528,-1.86002648932964,
0.343172294277177));
#161678=CARTESIAN_POINT('Ctrl Pts',(7.95976819968273,-1.64621431923495,
0.351785073078274));
#161679=CARTESIAN_POINT('Ctrl Pts',(8.001371750913,-1.4303766624732,0.360397851879371));
#161680=CARTESIAN_POINT('Ctrl Pts',(8.03416612107553,-1.21320332239168,
0.369010630680469));
#161681=CARTESIAN_POINT('Ctrl Pts',(8.0669557889288,-0.996061122295518,
0.377622174515039));
#161682=CARTESIAN_POINT('Ctrl Pts',(8.09093876693625,-0.777583848880212,
0.386233718349605));
#161683=CARTESIAN_POINT('Ctrl Pts',(8.1060347856621,-0.558468992994177,
0.394845262184174));
#161684=CARTESIAN_POINT('Ctrl Pts',(8.11880671657131,-0.373087678133646,
0.402131027051992));
#161685=CARTESIAN_POINT('Ctrl Pts',(8.12521827829703,-0.187250194103663,
0.40941679191981));
#161686=CARTESIAN_POINT('Ctrl Pts',(8.12524988254124,-0.0013815801172392,
0.416702556787628));
#161687=CARTESIAN_POINT('',(-2.1020845102162,-7.84862588447233,0.));
#161688=CARTESIAN_POINT('Origin',(0.,0.,0.));
#161689=CARTESIAN_POINT('',(8.13159794993462,0.00671758913419385,0.583297443212405));
#161690=CARTESIAN_POINT('Ctrl Pts',(-2.1020845102162,-7.84862588447233,
0.));
#161691=CARTESIAN_POINT('Ctrl Pts',(0.0676884603301917,-8.42975259623151,
0.0879975931412002));
#161692=CARTESIAN_POINT('Ctrl Pts',(2.47476766063835,-8.05858769184727,
0.175995186282401));
#161693=CARTESIAN_POINT('Ctrl Pts',(6.26263734649459,-5.64310942899612,
0.351990372564801));
#161694=CARTESIAN_POINT('Ctrl Pts',(7.61452387219173,-3.61722777291617,
0.439987965706001));
#161695=CARTESIAN_POINT('Ctrl Pts',(8.08425694621335,-0.941261955081332,
0.546422853635602));
#161696=CARTESIAN_POINT('Ctrl Pts',(8.12525000000002,-0.470634548223924,
0.564860148424005));
#161697=CARTESIAN_POINT('Ctrl Pts',(8.12525,4.45453585155269E-13,0.583297443212406));
#161698=CARTESIAN_POINT('',(8.13064101234911,-0.00726150239757081,2.58329744321241));
#161699=CARTESIAN_POINT('Ctrl Pts',(8.1326776545346,0.00786016460551604,
0.583297443212405));
#161700=CARTESIAN_POINT('Ctrl Pts',(8.13566645843386,0.371006238495569,
0.597588802946333));
#161701=CARTESIAN_POINT('Ctrl Pts',(7.9488919173957,3.41866176301992,0.717658472871213));
#161702=CARTESIAN_POINT('Ctrl Pts',(4.99171475646078,7.44423893657555,0.890617297891568));
#161703=CARTESIAN_POINT('Ctrl Pts',(-0.510988490918925,8.4371067902629,
1.10217391827347));
#161704=CARTESIAN_POINT('Ctrl Pts',(-4.47752894352082,7.19508636046628,
1.2608413835599));
#161705=CARTESIAN_POINT('Ctrl Pts',(-7.3764386431641,4.16414405786186,1.41950884884633));
#161706=CARTESIAN_POINT('Ctrl Pts',(-8.46487839372028,0.136812730728797,
1.57817631413276));
#161707=CARTESIAN_POINT('Ctrl Pts',(-7.50785040472005,-3.92613790885581,
1.73684377941919));
#161708=CARTESIAN_POINT('Ctrl Pts',(-4.70369331913998,-7.04503919375124,
1.89551124470561));
#161709=CARTESIAN_POINT('Ctrl Pts',(-0.787795848183251,-8.4201070003184,
2.05417870999205));
#161710=CARTESIAN_POINT('Ctrl Pts',(4.76217654495408,-7.59287955017986,
2.26573533037394));
#161711=CARTESIAN_POINT('Ctrl Pts',(7.88034319623104,-3.60392890592102,
2.44210824144741));
#161712=CARTESIAN_POINT('Ctrl Pts',(8.13264513995538,-0.45895858051545,
2.56559199742538));
#161713=CARTESIAN_POINT('Ctrl Pts',(8.13064101234911,-0.00726150239757081,
2.58329744321241));
#161714=CARTESIAN_POINT('',(8.1252498612179,0.00150175848002178,4.58329744319216));
#161715=CARTESIAN_POINT('Ctrl Pts',(8.12524675951605,-0.00725668477251276,
2.58329744321241));
#161716=CARTESIAN_POINT('Ctrl Pts',(8.12542154448592,0.188448524219183,
2.59097374895978));
#161717=CARTESIAN_POINT('Ctrl Pts',(8.11852158023305,0.384406059005546,
2.59865005470714));
#161718=CARTESIAN_POINT('Ctrl Pts',(8.10451899472242,0.580051227637208,
2.6063263604545));
#161719=CARTESIAN_POINT('Ctrl Pts',(8.0905296202666,0.775511810426265,2.61399542381825));
#161720=CARTESIAN_POINT('Ctrl Pts',(8.06945100009161,0.970660258994976,
2.621664487182));
#161721=CARTESIAN_POINT('Ctrl Pts',(8.04130730329936,1.16493107796317,2.62933355054574));
#161722=CARTESIAN_POINT('Ctrl Pts',(8.0131790158619,1.35909552895852,2.63699841491178));
#161723=CARTESIAN_POINT('Ctrl Pts',(7.97799340247663,1.55238295358604,2.64466327927782));
#161724=CARTESIAN_POINT('Ctrl Pts',(7.93582655914097,1.74423174656718,2.65232814364386));
#161725=CARTESIAN_POINT('Ctrl Pts',(7.89367489297021,1.93601148717118,2.65999024918563));
#161726=CARTESIAN_POINT('Ctrl Pts',(7.8445470758866,2.12635327763722,2.66765235472741));
#161727=CARTESIAN_POINT('Ctrl Pts',(7.78857053785034,2.31470441729168,2.67531446026918));
#161728=CARTESIAN_POINT('Ctrl Pts',(7.75561211810127,2.42560366434635,2.67982583055871));
#161729=CARTESIAN_POINT('Ctrl Pts',(7.72028039636842,2.53581298880038,2.68433720084825));
#161730=CARTESIAN_POINT('Ctrl Pts',(7.68260957495565,2.64522166959591,2.68884857113778));
#161731=CARTESIAN_POINT('Ctrl Pts',(7.61549722361775,2.84013841283621,2.69688579083545));
#161732=CARTESIAN_POINT('Ctrl Pts',(7.54098955720979,3.0324221846715,2.70492301053312));
#161733=CARTESIAN_POINT('Ctrl Pts',(7.45932971704242,3.22150395544501,2.7129602302308));
#161734=CARTESIAN_POINT('Ctrl Pts',(7.37762037695026,3.41070034233108,2.7210023218676));
#161735=CARTESIAN_POINT('Ctrl Pts',(7.28875033878966,3.5966905659627,2.7290444135044));
#161736=CARTESIAN_POINT('Ctrl Pts',(7.19300957783444,3.7789285221716,2.7370865051412));
#161737=CARTESIAN_POINT('Ctrl Pts',(7.09719909448777,3.96129919161561,2.74513445336255));
#161738=CARTESIAN_POINT('Ctrl Pts',(6.99450805242976,4.13991186269587,2.7531824015839));
#161739=CARTESIAN_POINT('Ctrl Pts',(6.88527107355487,4.31424730470665,2.76123034980525));
#161740=CARTESIAN_POINT('Ctrl Pts',(6.77587284440087,4.48884009216008,2.76929017801368));
#161741=CARTESIAN_POINT('Ctrl Pts',(6.6599095335933,4.65914276345852,2.7773500062221));
#161742=CARTESIAN_POINT('Ctrl Pts',(6.53775860245799,4.82466579345,2.78540983443052));
#161743=CARTESIAN_POINT('Ctrl Pts',(6.41550865653361,4.99032299538556,2.79347619588583));
#161744=CARTESIAN_POINT('Ctrl Pts',(6.28706127770004,5.1511925781628,2.80154255734113));
#161745=CARTESIAN_POINT('Ctrl Pts',(6.1528330915265,5.30681943449336,2.80960891879644));
#161746=CARTESIAN_POINT('Ctrl Pts',(6.01839397508925,5.46269084761026,2.81768795597804));
#161747=CARTESIAN_POINT('Ctrl Pts',(5.87815610848054,5.61330283573933,2.82576699315964));
#161748=CARTESIAN_POINT('Ctrl Pts',(5.73257296564144,5.75823712225338,2.83384603034124));
#161749=CARTESIAN_POINT('Ctrl Pts',(5.65046242022818,5.83998170533265,2.83840269903555));
#161750=CARTESIAN_POINT('Ctrl Pts',(5.56665210613339,5.91992088417901,2.84295936772987));
#161751=CARTESIAN_POINT('Ctrl Pts',(5.48122781329227,5.99798543023332,2.84751603642419));
#161752=CARTESIAN_POINT('Ctrl Pts',(5.32963895041481,6.13651412475151,2.85560202932981));
#161753=CARTESIAN_POINT('Ctrl Pts',(5.17267087758265,6.26940683553619,2.86368802223543));
#161754=CARTESIAN_POINT('Ctrl Pts',(5.0107695065041,6.39623924780716,2.87177401514105));
#161755=CARTESIAN_POINT('Ctrl Pts',(4.84901262311636,6.52295846942231,2.87985279176162));
#161756=CARTESIAN_POINT('Ctrl Pts',(4.68233146822159,6.64362798204878,2.8879315683822));
#161757=CARTESIAN_POINT('Ctrl Pts',(4.51120663100571,6.75786225776097,2.89601034500277));
#161758=CARTESIAN_POINT('Ctrl Pts',(4.34021113449181,6.87201019217021,2.90408301546917));
#161759=CARTESIAN_POINT('Ctrl Pts',(4.16477891564455,6.97973241345168,2.91215568593557));
#161760=CARTESIAN_POINT('Ctrl Pts',(3.98542178030168,7.08068505129249,2.92022835640197));
#161761=CARTESIAN_POINT('Ctrl Pts',(3.80617574113922,7.18157515773501,2.92829602654958));
#161762=CARTESIAN_POINT('Ctrl Pts',(3.62300990922674,7.27570388805911,2.93636369669719));
#161763=CARTESIAN_POINT('Ctrl Pts',(3.43646360804606,7.3627715863712,2.94443136684479));
#161764=CARTESIAN_POINT('Ctrl Pts',(3.25000744004199,7.44979721637006,2.9524951389535));
#161765=CARTESIAN_POINT('Ctrl Pts',(3.06017434701721,7.52976848513044,2.96055891106221));
#161766=CARTESIAN_POINT('Ctrl Pts',(2.8675272614942,7.60243217444836,2.96862268317092));
#161767=CARTESIAN_POINT('Ctrl Pts',(2.67219473769384,7.67610877217409,2.97679886166368));
#161768=CARTESIAN_POINT('Ctrl Pts',(2.47396947892957,7.74227239099172,2.98497504015643));
#161769=CARTESIAN_POINT('Ctrl Pts',(2.27345940018541,7.80070957786589,2.99315121864919));
#161770=CARTESIAN_POINT('Ctrl Pts',(2.07579972660383,7.85831603513186,3.00121116646899));
#161771=CARTESIAN_POINT('Ctrl Pts',(1.87592007785936,7.9084141940002,3.0092711142888));
#161772=CARTESIAN_POINT('Ctrl Pts',(1.67441853426039,7.9508496485989,3.0173310621086));
#161773=CARTESIAN_POINT('Ctrl Pts',(1.47292674455366,7.99328304906519,3.02539061977823));
#161774=CARTESIAN_POINT('Ctrl Pts',(1.26981352658252,8.02805441989696,3.03345017744786));
#161775=CARTESIAN_POINT('Ctrl Pts',(1.06568788024979,8.0550603290347,3.04150973511749));
#161776=CARTESIAN_POINT('Ctrl Pts',(0.861546829722573,8.08206827615388,
3.04956990099582));
#161777=CARTESIAN_POINT('Ctrl Pts',(0.656393512582881,8.10130955180625,
3.05763006687415));
#161778=CARTESIAN_POINT('Ctrl Pts',(0.45084339107128,8.11273244962678,3.06569023275248));
#161779=CARTESIAN_POINT('Ctrl Pts',(0.240110538496967,8.12444336385385,
3.07395362727286));
#161780=CARTESIAN_POINT('Ctrl Pts',(0.0289609577969593,8.12793642602925,
3.08221702179324));
#161781=CARTESIAN_POINT('Ctrl Pts',(-0.181940457436845,8.12321274080937,
3.09048041631362));
#161782=CARTESIAN_POINT('Ctrl Pts',(-0.387824207660257,8.11860143923576,
3.09854721212694));
#161783=CARTESIAN_POINT('Ctrl Pts',(-0.593471145601391,8.1061599576421,
3.10661400794026));
#161784=CARTESIAN_POINT('Ctrl Pts',(-0.798266002813213,8.08594205712931,
3.11468080375358));
#161785=CARTESIAN_POINT('Ctrl Pts',(-1.01054755085099,8.06498505031108,
3.12304249762749));
#161786=CARTESIAN_POINT('Ctrl Pts',(-1.22191317306984,8.0356723877964,3.1314041915014));
#161787=CARTESIAN_POINT('Ctrl Pts',(-1.4316867562105,7.99812231680608,3.13976588537531));
#161788=CARTESIAN_POINT('Ctrl Pts',(-1.64146033935117,7.96057224581576,
3.14812757924922));
#161789=CARTESIAN_POINT('Ctrl Pts',(-1.84964152006452,7.91478487093404,
3.15648927312313));
#161790=CARTESIAN_POINT('Ctrl Pts',(-2.05556894582339,7.86093657724488,
3.16485096699704));
#161791=CARTESIAN_POINT('Ctrl Pts',(-2.24220479106239,7.81213286996637,
3.17242932523678));
#161792=CARTESIAN_POINT('Ctrl Pts',(-2.42736339181452,7.75660979140615,
3.18000768347651));
#161793=CARTESIAN_POINT('Ctrl Pts',(-2.6105035175124,7.69447587217969,3.18758604171625));
#161794=CARTESIAN_POINT('Ctrl Pts',(-2.79350736016814,7.6323881896777,3.19515876054894));
#161795=CARTESIAN_POINT('Ctrl Pts',(-2.97449537018565,7.56369957030046,
3.20273147938162));
#161796=CARTESIAN_POINT('Ctrl Pts',(-3.15293799653857,7.48856925937681,
3.21030419821431));
#161797=CARTESIAN_POINT('Ctrl Pts',(-3.33128172004362,7.41348058985838,
3.21787271982421));
#161798=CARTESIAN_POINT('Ctrl Pts',(-3.50708252961938,7.33195747540202,
3.2254412414341));
#161799=CARTESIAN_POINT('Ctrl Pts',(-3.67982755711192,7.24420849454374,
3.233009763044));
#161800=CARTESIAN_POINT('Ctrl Pts',(-3.85253083465313,7.15648072133313,
3.24057645545271));
#161801=CARTESIAN_POINT('Ctrl Pts',(-4.02217946920668,7.06253023576544,
3.24814314786142));
#161802=CARTESIAN_POINT('Ctrl Pts',(-4.18828193421433,6.96261315901105,
3.25570984027014));
#161803=CARTESIAN_POINT('Ctrl Pts',(-4.35435492833486,6.86271381013861,
3.26327519015128));
#161804=CARTESIAN_POINT('Ctrl Pts',(-4.51688269178376,6.75685016943834,
3.27084054003243));
#161805=CARTESIAN_POINT('Ctrl Pts',(-4.67539985699655,6.64532344883954,
3.27840588991358));
#161806=CARTESIAN_POINT('Ctrl Pts',(-4.8339721285435,6.53375795749484,3.2859738697856));
#161807=CARTESIAN_POINT('Ctrl Pts',(-4.98853071348142,6.41652566237355,
3.29354184965763));
#161808=CARTESIAN_POINT('Ctrl Pts',(-5.13864032618363,6.29397038129505,
3.30110982952966));
#161809=CARTESIAN_POINT('Ctrl Pts',(-5.28679728649344,6.17300932098956,
3.30857936378094));
#161810=CARTESIAN_POINT('Ctrl Pts',(-5.4306200820621,6.04686317803796,3.31604889803221));
#161811=CARTESIAN_POINT('Ctrl Pts',(-5.56972346001078,5.9158996054282,3.32351843228349));
#161812=CARTESIAN_POINT('Ctrl Pts',(-5.74302290330132,5.75274099232116,
3.33282421727933));
#161813=CARTESIAN_POINT('Ctrl Pts',(-5.90891371658913,5.58218701785903,
3.34213000227518));
#161814=CARTESIAN_POINT('Ctrl Pts',(-6.06686896837867,5.40488561239032,
3.35143578727102));
#161815=CARTESIAN_POINT('Ctrl Pts',(-6.22567219020883,5.22663237861395,
3.36079152962372));
#161816=CARTESIAN_POINT('Ctrl Pts',(-6.37645442877942,5.04155914313817,
3.37014727197641));
#161817=CARTESIAN_POINT('Ctrl Pts',(-6.51872615786608,4.85035017717819,
3.37950301432911));
#161818=CARTESIAN_POINT('Ctrl Pts',(-6.66168851444334,4.65821302844297,
3.38890417211962));
#161819=CARTESIAN_POINT('Ctrl Pts',(-6.79605753013016,4.45988048359757,
3.39830532991012));
#161820=CARTESIAN_POINT('Ctrl Pts',(-6.92138273540747,4.25607196749578,
3.40770648770062));
#161821=CARTESIAN_POINT('Ctrl Pts',(-7.04684359176357,4.05204285055782,
3.41711782123505));
#161822=CARTESIAN_POINT('Ctrl Pts',(-7.16324104757251,3.84252594413645,
3.42652915476948));
#161823=CARTESIAN_POINT('Ctrl Pts',(-7.27016938693719,3.62826744435155,
3.4359404883039));
#161824=CARTESIAN_POINT('Ctrl Pts',(-7.37697234794513,3.41426017243366,
3.44534078662035));
#161825=CARTESIAN_POINT('Ctrl Pts',(-7.47432837298677,3.19552245461012,
3.4547410849368));
#161826=CARTESIAN_POINT('Ctrl Pts',(-7.56187933311759,2.97282164178563,
3.46414138325324));
#161827=CARTESIAN_POINT('Ctrl Pts',(-7.61789934795596,2.83032517092681,
3.47015622135879));
#161828=CARTESIAN_POINT('Ctrl Pts',(-7.66990594206708,2.68620662287665,
3.47617105946434));
#161829=CARTESIAN_POINT('Ctrl Pts',(-7.71781530533523,2.54067205188572,
3.48218589756989));
#161830=CARTESIAN_POINT('Ctrl Pts',(-7.77948397067406,2.35334076335584,
3.489928163651));
#161831=CARTESIAN_POINT('Ctrl Pts',(-7.8343900712243,2.16357430055282,3.49767042973211));
#161832=CARTESIAN_POINT('Ctrl Pts',(-7.88233822795875,1.97191065278325,
3.50541269581321));
#161833=CARTESIAN_POINT('Ctrl Pts',(-7.93025651605203,1.78036639923259,
3.51315013895673));
#161834=CARTESIAN_POINT('Ctrl Pts',(-7.97122540513269,1.58692765514176,
3.52088758210024));
#161835=CARTESIAN_POINT('Ctrl Pts',(-8.00509898102066,1.39214865102903,
3.52862502524376));
#161836=CARTESIAN_POINT('Ctrl Pts',(-8.03895747624439,1.19745636338144,
3.53635902364373));
#161837=CARTESIAN_POINT('Ctrl Pts',(-8.06572688911408,1.0014253514074,3.54409302204369));
#161838=CARTESIAN_POINT('Ctrl Pts',(-8.08531212440768,0.804621285702891,
3.55182702044366));
#161839=CARTESIAN_POINT('Ctrl Pts',(-8.10489485293535,0.607842409469903,
3.55956002894876));
#161840=CARTESIAN_POINT('Ctrl Pts',(-8.11729519281468,0.410291027156225,
3.56729303745387));
#161841=CARTESIAN_POINT('Ctrl Pts',(-8.12246972851236,0.212539577256358,
3.57502604595898));
#161842=CARTESIAN_POINT('Ctrl Pts',(-8.12764374719607,0.0148078857019956,
3.58275828182018));
#161843=CARTESIAN_POINT('Ctrl Pts',(-8.12559339413814,-0.183123480250224,
3.59049051768137));
#161844=CARTESIAN_POINT('Ctrl Pts',(-8.11632736431311,-0.380680545605153,
3.59822275354257));
#161845=CARTESIAN_POINT('Ctrl Pts',(-8.10705777033334,-0.578313600781254,
3.60595796358856));
#161846=CARTESIAN_POINT('Ctrl Pts',(-8.09056697090893,-0.775571714409861,
3.61369317363456));
#161847=CARTESIAN_POINT('Ctrl Pts',(-8.06691572793074,-0.971883841291524,
3.62142838368055));
#161848=CARTESIAN_POINT('Ctrl Pts',(-8.04711773496089,-1.13621288359535,
3.62790337673915));
#161849=CARTESIAN_POINT('Ctrl Pts',(-8.02230332607686,-1.29987903084078,
3.63437836979774));
#161850=CARTESIAN_POINT('Ctrl Pts',(-7.99253584895792,-1.46255197022961,
3.64085336285634));
#161851=CARTESIAN_POINT('Ctrl Pts',(-7.95385356750799,-1.67394242164687,
3.64926749559853));
#161852=CARTESIAN_POINT('Ctrl Pts',(-7.90678791254452,-1.88375739966851,
3.65768162834072));
#161853=CARTESIAN_POINT('Ctrl Pts',(-7.85149466753507,-2.09134383786319,
3.66609576108292));
#161854=CARTESIAN_POINT('Ctrl Pts',(-7.79618597220823,-2.29898828090738,
3.67451224494451));
#161855=CARTESIAN_POINT('Ctrl Pts',(-7.7326451652376,-2.50440268585466,
3.68292872880611));
#161856=CARTESIAN_POINT('Ctrl Pts',(-7.66107820026736,-2.70694816571879,
3.69134521266771));
#161857=CARTESIAN_POINT('Ctrl Pts',(-7.58949347906698,-2.90954389843566,
3.69976378471378));
#161858=CARTESIAN_POINT('Ctrl Pts',(-7.50987871227754,-3.10926903617535,
3.70818235675984));
#161859=CARTESIAN_POINT('Ctrl Pts',(-7.42248876835383,-3.30550269190046,
3.7166009288059));
#161860=CARTESIAN_POINT('Ctrl Pts',(-7.33506525103029,-3.50181173651689,
3.72502273509235));
#161861=CARTESIAN_POINT('Ctrl Pts',(-7.2398606936539,-3.69462637691134,
3.73344454137879));
#161862=CARTESIAN_POINT('Ctrl Pts',(-7.13717749240084,-3.88334713932026,
3.74186634766523));
#161863=CARTESIAN_POINT('Ctrl Pts',(-7.03448315831298,-4.0720883626911,
3.75028906703752));
#161864=CARTESIAN_POINT('Ctrl Pts',(-6.92430869024064,-4.25673459147822,
3.75871178640981));
#161865=CARTESIAN_POINT('Ctrl Pts',(-6.80700198349754,-4.43671179581913,
3.76713450578211));
#161866=CARTESIAN_POINT('Ctrl Pts',(-6.68967297221502,-4.61672322078355,
3.77555882663893));
#161867=CARTESIAN_POINT('Ctrl Pts',(-6.56520915723441,-4.79206362670022,
3.78398314749575));
#161868=CARTESIAN_POINT('Ctrl Pts',(-6.43400195451774,-4.96218766390005,
3.79240746835257));
#161869=CARTESIAN_POINT('Ctrl Pts',(-6.39707221043305,-5.01007098910143,
3.79477858828264));
#161870=CARTESIAN_POINT('Ctrl Pts',(-6.35960850789623,-5.05754125858306,
3.79714970821271));
#161871=CARTESIAN_POINT('Ctrl Pts',(-6.32162016755184,-5.10458676287335,
3.79952082814277));
#161872=CARTESIAN_POINT('Ctrl Pts',(-6.18665249013186,-5.27173337653293,
3.80794511167146));
#161873=CARTESIAN_POINT('Ctrl Pts',(-6.04504535410084,-5.43353292673586,
3.81636939520014));
#161874=CARTESIAN_POINT('Ctrl Pts',(-5.89723839174989,-5.58947823265921,
3.82479367872883));
#161875=CARTESIAN_POINT('Ctrl Pts',(-5.74945698348554,-5.74539657747201,
3.8332165057979));
#161876=CARTESIAN_POINT('Ctrl Pts',(-5.59547807123916,-5.89546250807257,
3.84163933286698));
#161877=CARTESIAN_POINT('Ctrl Pts',(-5.43577928233965,-6.03920451352552,
3.85006215993605));
#161878=CARTESIAN_POINT('Ctrl Pts',(-5.27611313587101,-6.18291713811398,
3.85848326537936));
#161879=CARTESIAN_POINT('Ctrl Pts',(-5.11072964350834,-6.32030824234214,
3.86690437082266));
#161880=CARTESIAN_POINT('Ctrl Pts',(-4.94014156378475,-6.45094480617114,
3.87532547626597));
#161881=CARTESIAN_POINT('Ctrl Pts',(-4.76960134775628,-6.58154471592282,
3.88374421891098));
#161882=CARTESIAN_POINT('Ctrl Pts',(-4.59385967038434,-6.70539371012401,
3.89216296155599));
#161883=CARTESIAN_POINT('Ctrl Pts',(-4.41346127678764,-6.82209990551267,
3.90058170420101));
#161884=CARTESIAN_POINT('Ctrl Pts',(-4.23311327418162,-6.93877350116091,
3.90899809522429));
#161885=CARTESIAN_POINT('Ctrl Pts',(-4.04811137390595,-7.04830813839393,
3.91741448624758));
#161886=CARTESIAN_POINT('Ctrl Pts',(-3.85902909530774,-7.15035537606826,
3.92583087727086));
#161887=CARTESIAN_POINT('Ctrl Pts',(-3.67001543178216,-7.25236558235776,
3.93424421411432));
#161888=CARTESIAN_POINT('Ctrl Pts',(-3.47692457894577,-7.34689368975686,
3.94265755095777));
#161889=CARTESIAN_POINT('Ctrl Pts',(-3.28035530375629,-7.43363683829241,
3.95107088780122));
#161890=CARTESIAN_POINT('Ctrl Pts',(-3.2249249280901,-7.4580974530307,3.95344335634387));
#161891=CARTESIAN_POINT('Ctrl Pts',(-3.16921810209201,-7.48193930733348,
3.95581582488653));
#161892=CARTESIAN_POINT('Ctrl Pts',(-3.11324858489207,-7.50515628159518,
3.95818829342918));
#161893=CARTESIAN_POINT('Ctrl Pts',(-2.93076550130723,-7.58085293339315,
3.96592349282039));
#161894=CARTESIAN_POINT('Ctrl Pts',(-2.74540735442137,-7.64993685540819,
3.97365869221159));
#161895=CARTESIAN_POINT('Ctrl Pts',(-2.5577036049958,-7.7121877461257,3.9813938916028));
#161896=CARTESIAN_POINT('Ctrl Pts',(-2.37005789584823,-7.7744193881121,
3.98912669917645));
#161897=CARTESIAN_POINT('Ctrl Pts',(-2.1800683634462,-7.82982209529938,
3.99685950675011));
#161898=CARTESIAN_POINT('Ctrl Pts',(-1.98828263028762,-7.87822440303629,
4.00459231432376));
#161899=CARTESIAN_POINT('Ctrl Pts',(-1.79652212509887,-7.92662034381389,
4.01232410470477));
#161900=CARTESIAN_POINT('Ctrl Pts',(-1.60296623243336,-7.96801763365407,
4.02005589508579));
#161901=CARTESIAN_POINT('Ctrl Pts',(-1.40817598455326,-8.0022951682019,
4.0277876854668));
#161902=CARTESIAN_POINT('Ctrl Pts',(-1.2133160332439,-8.0365849685676,4.03552224257926));
#161903=CARTESIAN_POINT('Ctrl Pts',(-1.0172211918205,-8.06374985805016,
4.04325679969172));
#161904=CARTESIAN_POINT('Ctrl Pts',(-0.820461557063465,-8.08372008396388,
4.05099135680417));
#161905=CARTESIAN_POINT('Ctrl Pts',(-0.623668690312049,-8.1036936827769,
4.0587272202555));
#161906=CARTESIAN_POINT('Ctrl Pts',(-0.426211158872913,-8.11647016867068,
4.06646308370682));
#161907=CARTESIAN_POINT('Ctrl Pts',(-0.22866254125838,-8.1220318273647,
4.07419894715815));
#161908=CARTESIAN_POINT('Ctrl Pts',(-0.0309522798858196,-8.12759803687474,
4.08194114046414));
#161909=CARTESIAN_POINT('Ctrl Pts',(0.166848862963725,-8.1259376218865,
4.08968333377014));
#161910=CARTESIAN_POINT('Ctrl Pts',(0.36416801257101,-8.11708501995144,
4.09742552707613));
#161911=CARTESIAN_POINT('Ctrl Pts',(0.529235654785898,-8.10967936200189,
4.10390227095596));
#161912=CARTESIAN_POINT('Ctrl Pts',(0.693965924963077,-8.09724141428031,
4.1103790148358));
#161913=CARTESIAN_POINT('Ctrl Pts',(0.858027275555607,-8.07981910421902,
4.11685575871563));
#161914=CARTESIAN_POINT('Ctrl Pts',(1.09608684901361,-8.05453863635218,
4.12625377281134));
#161915=CARTESIAN_POINT('Ctrl Pts',(1.33287327577442,-8.01874928881438,
4.13565178690704));
#161916=CARTESIAN_POINT('Ctrl Pts',(1.56755319678678,-7.97260713554503,
4.14504980100275));
#161917=CARTESIAN_POINT('Ctrl Pts',(1.80256702990828,-7.9263993293487,4.15446118697405));
#161918=CARTESIAN_POINT('Ctrl Pts',(2.0354683253152,-7.86980925921721,4.16387257294536));
#161919=CARTESIAN_POINT('Ctrl Pts',(2.26543342217421,-7.80304421185707,
4.17328395891666));
#161920=CARTESIAN_POINT('Ctrl Pts',(2.49505226591476,-7.7363796910819,4.18268117438215));
#161921=CARTESIAN_POINT('Ctrl Pts',(2.72174371303819,-7.65957082634099,
4.19207838984764));
#161922=CARTESIAN_POINT('Ctrl Pts',(2.94470151255391,-7.57287399634133,
4.20147560531313));
#161923=CARTESIAN_POINT('Ctrl Pts',(3.16709693949201,-7.48639584413569,
4.2108491179241));
#161924=CARTESIAN_POINT('Ctrl Pts',(3.38577748706466,-7.39007953936429,
4.22022263053508));
#161925=CARTESIAN_POINT('Ctrl Pts',(3.59995718815401,-7.28422925270466,
4.22959614314606));
#161926=CARTESIAN_POINT('Ctrl Pts',(3.81274604645226,-7.17906633794529,
4.23890878592495));
#161927=CARTESIAN_POINT('Ctrl Pts',(4.02109227437145,-7.0644928636502,4.24822142870384));
#161928=CARTESIAN_POINT('Ctrl Pts',(4.22423981990064,-6.94085625167859,
4.25753407148273));
#161929=CARTESIAN_POINT('Ctrl Pts',(4.35504594612473,-6.86124698921201,
4.26353045565584));
#161930=CARTESIAN_POINT('Ctrl Pts',(4.48369697723611,-6.77788110845369,
4.26952683982893));
#161931=CARTESIAN_POINT('Ctrl Pts',(4.60999450977774,-6.69086228989352,
4.27552322400203));
#161932=CARTESIAN_POINT('Ctrl Pts',(4.76938668679867,-6.58104130881041,
4.28309088354668));
#161933=CARTESIAN_POINT('Ctrl Pts',(4.9249653082953,-6.46544311001104,4.29065854309133));
#161934=CARTESIAN_POINT('Ctrl Pts',(5.07627240430222,-6.34437909017263,
4.29822620263598));
#161935=CARTESIAN_POINT('Ctrl Pts',(5.22753760620868,-6.22334859069344,
4.30579176683747));
#161936=CARTESIAN_POINT('Ctrl Pts',(5.37453334913977,-6.09685551090348,
4.31335733103895));
#161937=CARTESIAN_POINT('Ctrl Pts',(5.51683266023166,-5.96525313473798,
4.32092289524044));
#161938=CARTESIAN_POINT('Ctrl Pts',(5.65911950465485,-5.83366228809579,
4.32848779663209));
#161939=CARTESIAN_POINT('Ctrl Pts',(5.7967104668374,-5.69696328627307,4.33605269802375));
#161940=CARTESIAN_POINT('Ctrl Pts',(5.92921359509749,-5.55554801133166,
4.34361759941541));
#161941=CARTESIAN_POINT('Ctrl Pts',(6.06178175514736,-5.41406333056902,
4.3511862136181));
#161942=CARTESIAN_POINT('Ctrl Pts',(6.18925683847888,-5.26785801880553,
4.35875482782079));
#161943=CARTESIAN_POINT('Ctrl Pts',(6.31128517599999,-5.11735937664171,
4.36632344202348));
#161944=CARTESIAN_POINT('Ctrl Pts',(6.43334065053819,-4.96682726615152,
4.37389373935664));
#161945=CARTESIAN_POINT('Ctrl Pts',(6.54994674376694,-4.81200021614064,
4.3814640366898));
#161946=CARTESIAN_POINT('Ctrl Pts',(6.66079187115985,-4.65333635272488,
4.38903433402297));
#161947=CARTESIAN_POINT('Ctrl Pts',(6.77174931625615,-4.49451171759845,
4.39661230222476));
#161948=CARTESIAN_POINT('Ctrl Pts',(6.87693393149166,-4.33184280958211,
4.40419027042654));
#161949=CARTESIAN_POINT('Ctrl Pts',(6.97607856849142,-4.16581509055967,
4.41176823862833));
#161950=CARTESIAN_POINT('Ctrl Pts',(7.07386492635362,-4.00206194728666,
4.41924238884839));
#161951=CARTESIAN_POINT('Ctrl Pts',(7.16577564216525,-3.83504176562554,
4.42671653906844));
#161952=CARTESIAN_POINT('Ctrl Pts',(7.25159989324019,-3.66524031283883,
4.43419068928849));
#161953=CARTESIAN_POINT('Ctrl Pts',(7.35155880230678,-3.46747374026879,
4.44289578013214));
#161954=CARTESIAN_POINT('Ctrl Pts',(7.44343978347571,-3.26558398144789,
4.4516008709758));
#161955=CARTESIAN_POINT('Ctrl Pts',(7.52693546046989,-3.0602173348344,4.46030596181945));
#161956=CARTESIAN_POINT('Ctrl Pts',(7.61036495209151,-2.85501347830184,
4.46900415230968));
#161957=CARTESIAN_POINT('Ctrl Pts',(7.6854223337838,-2.64633843566982,4.47770234279992));
#161958=CARTESIAN_POINT('Ctrl Pts',(7.75184816053937,-2.4348588580126,4.48640053329015));
#161959=CARTESIAN_POINT('Ctrl Pts',(7.81816189742858,-2.22373614031112,
4.49508404607056));
#161960=CARTESIAN_POINT('Ctrl Pts',(7.87587310579198,-2.00981854287022,
4.50376755885097));
#161961=CARTESIAN_POINT('Ctrl Pts',(7.92477200248283,-1.79378824590983,
4.51245107163138));
#161962=CARTESIAN_POINT('Ctrl Pts',(7.97360943000941,-1.57802951339587,
4.52112366865889));
#161963=CARTESIAN_POINT('Ctrl Pts',(8.01365661180745,-1.36016359039827,
4.5297962656864));
#161964=CARTESIAN_POINT('Ctrl Pts',(8.04475399050408,-1.14088596922243,
4.53846886271391));
#161965=CARTESIAN_POINT('Ctrl Pts',(8.07577958197994,-0.922114542834185,
4.54712143935181));
#161966=CARTESIAN_POINT('Ctrl Pts',(8.09789658457935,-0.701938135039435,
4.5557740159897));
#161967=CARTESIAN_POINT('Ctrl Pts',(8.1109967727298,-0.481060199212926,
4.56442659262759));
#161968=CARTESIAN_POINT('Ctrl Pts',(8.1205203980151,-0.320485505899887,
4.57071687614912));
#161969=CARTESIAN_POINT('Ctrl Pts',(8.12527962600337,-0.159540328021134,
4.57700715967064));
#161970=CARTESIAN_POINT('Ctrl Pts',(8.1252498612179,0.00150175848001979,
4.58329744319216));
#161971=CARTESIAN_POINT('',(8.12524931639108,0.00333301459649942,6.58329744321241));
#161972=CARTESIAN_POINT('Ctrl Pts',(8.1252498612178,0.00150175899845503,
4.58329744321241));
#161973=CARTESIAN_POINT('Ctrl Pts',(8.12521061695668,0.213832384326663,
4.59159105057079));
#161974=CARTESIAN_POINT('Ctrl Pts',(8.11684406997655,0.426046074186561,
4.59988465792917));
#161975=CARTESIAN_POINT('Ctrl Pts',(8.10020335251704,0.637489772758512,
4.60817826528755));
#161976=CARTESIAN_POINT('Ctrl Pts',(8.08354769346874,0.849123325211606,
4.61647931942044));
#161977=CARTESIAN_POINT('Ctrl Pts',(8.05860305086515,1.05998522618361,4.62478037355333));
#161978=CARTESIAN_POINT('Ctrl Pts',(8.02547427528377,1.26942909185918,4.63308142768623));
#161979=CARTESIAN_POINT('Ctrl Pts',(7.99231477745251,1.47906718707278,4.64139017987179));
#161980=CARTESIAN_POINT('Ctrl Pts',(7.95095603491722,1.68728434421521,4.64969893205735));
#161981=CARTESIAN_POINT('Ctrl Pts',(7.90155388575722,1.89344494321196,4.65800768424292));
#161982=CARTESIAN_POINT('Ctrl Pts',(7.85207263488596,2.09993564234511,4.66632974023261));
#161983=CARTESIAN_POINT('Ctrl Pts',(7.79452229016653,2.3043629254726,4.67465179622231));
#161984=CARTESIAN_POINT('Ctrl Pts',(7.72910903618032,2.50610476024761,4.68297385221201));
#161985=CARTESIAN_POINT('Ctrl Pts',(7.66364328559863,2.70800850042935,4.69130258696451));
#161986=CARTESIAN_POINT('Ctrl Pts',(7.59030211941962,2.90722222466709,4.699631321717));
#161987=CARTESIAN_POINT('Ctrl Pts',(7.50934026374922,3.10314298183871,4.70796005646949));
#161988=CARTESIAN_POINT('Ctrl Pts',(7.42826014781913,3.29934991871097,4.71630095693047));
#161989=CARTESIAN_POINT('Ctrl Pts',(7.33953719817232,3.49225401381393,4.72464185739145));
#161990=CARTESIAN_POINT('Ctrl Pts',(7.24347352182253,3.68127408666564,4.73298275785243));
#161991=CARTESIAN_POINT('Ctrl Pts',(7.17228634393308,3.82134581889641,4.7391637118554));
#161992=CARTESIAN_POINT('Ctrl Pts',(7.0970690304504,3.95928515739477,4.74534466585837));
#161993=CARTESIAN_POINT('Ctrl Pts',(7.01796016192712,4.09486541025513,4.75152561986133));
#161994=CARTESIAN_POINT('Ctrl Pts',(6.91457202894797,4.27205653273904,4.75960356745843));
#161995=CARTESIAN_POINT('Ctrl Pts',(6.8043534006649,4.44552896342827,4.76768151505552));
#161996=CARTESIAN_POINT('Ctrl Pts',(6.68759103205316,4.61473875213994,4.77575946265262));
#161997=CARTESIAN_POINT('Ctrl Pts',(6.57097155683386,4.78374146248355,4.78382752448472));
#161998=CARTESIAN_POINT('Ctrl Pts',(6.44782448223716,4.9484916715378,4.79189558631683));
#161999=CARTESIAN_POINT('Ctrl Pts',(6.31848192230606,5.10847078488186,4.79996364814893));
#162000=CARTESIAN_POINT('Ctrl Pts',(6.18928172762075,5.26827381182556,4.80802282959699));
#162001=CARTESIAN_POINT('Ctrl Pts',(6.05389983934316,5.42331596799718,4.81608201104505));
#162002=CARTESIAN_POINT('Ctrl Pts',(5.91271140304813,5.57310787862254,4.8241411924931));
#162003=CARTESIAN_POINT('Ctrl Pts',(5.77170431816329,5.72270738698792,4.83219002221577));
#162004=CARTESIAN_POINT('Ctrl Pts',(5.62490577983017,5.86706987465934,4.84023885193844));
#162005=CARTESIAN_POINT('Ctrl Pts',(5.47273091592304,6.00573924545515,4.84828768166111));
#162006=CARTESIAN_POINT('Ctrl Pts',(5.32067115625161,6.14430372749645,4.85633042329295));
#162007=CARTESIAN_POINT('Ctrl Pts',(5.16324340916897,6.27718346434961,4.86437316492479));
#162008=CARTESIAN_POINT('Ctrl Pts',(5.00090029161773,6.40395845050526,4.87241590655662));
#162009=CARTESIAN_POINT('Ctrl Pts',(4.83868940833045,6.53063017390954,4.88045209708832));
#162010=CARTESIAN_POINT('Ctrl Pts',(4.67157138921698,6.65120687193072,4.88848828762003));
#162011=CARTESIAN_POINT('Ctrl Pts',(4.50003284081094,6.76530797481704,4.89652447815172));
#162012=CARTESIAN_POINT('Ctrl Pts',(4.40277726539928,6.82999878932741,4.90108068048374));
#162013=CARTESIAN_POINT('Ctrl Pts',(4.30410135635659,6.89260877847994,4.90563688281576));
#162014=CARTESIAN_POINT('Ctrl Pts',(4.20409836836367,6.95307446182061,4.91019308514777));
#162015=CARTESIAN_POINT('Ctrl Pts',(4.02770683320637,7.05972762211968,4.91822960025558));
#162016=CARTESIAN_POINT('Ctrl Pts',(3.84732439917407,7.15962256640634,4.9262661153634));
#162017=CARTESIAN_POINT('Ctrl Pts',(3.66350218994938,7.25247814658797,4.93430263047121));
#162018=CARTESIAN_POINT('Ctrl Pts',(3.47956893352285,7.34538982092926,4.94234400044677));
#162019=CARTESIAN_POINT('Ctrl Pts',(3.29219203813748,7.43125350482278,4.95038537042233));
#162020=CARTESIAN_POINT('Ctrl Pts',(3.10194390534103,7.50983565536674,4.9584267403979));
#162021=CARTESIAN_POINT('Ctrl Pts',(2.91155758205264,7.58847488560911,4.9664739513815));
#162022=CARTESIAN_POINT('Ctrl Pts',(2.71829615201036,7.6598219098172,4.97452116236509));
#162023=CARTESIAN_POINT('Ctrl Pts',(2.52274908496553,7.72369242116784,4.98256837334869));
#162024=CARTESIAN_POINT('Ctrl Pts',(2.32691379518903,7.78765707319537,4.99062744535975));
#162025=CARTESIAN_POINT('Ctrl Pts',(2.12878643574662,7.84412308924679,4.99868651737081));
#162026=CARTESIAN_POINT('Ctrl Pts',(1.92897034042226,7.89295641621511,5.00674558938187));
#162027=CARTESIAN_POINT('Ctrl Pts',(1.72899252394641,7.94182926643532,5.01481118400265));
#162028=CARTESIAN_POINT('Ctrl Pts',(1.52732355286919,7.98305703666817,5.02287677862344));
#162029=CARTESIAN_POINT('Ctrl Pts',(1.32457478472854,8.0165571913485,5.03094237324422));
#162030=CARTESIAN_POINT('Ctrl Pts',(1.12150765453683,8.0501099489524,5.03902063269778));
#162031=CARTESIAN_POINT('Ctrl Pts',(0.917357651253059,8.07591079719502,
5.04709889215135));
#162032=CARTESIAN_POINT('Ctrl Pts',(0.712740830625026,8.09392908733823,
5.05517715160492));
#162033=CARTESIAN_POINT('Ctrl Pts',(0.597210433682415,8.10410254329402,
5.05973828454801));
#162034=CARTESIAN_POINT('Ctrl Pts',(0.481531224403746,8.11179591523572,
5.06429941749109));
#162035=CARTESIAN_POINT('Ctrl Pts',(0.365813763653463,8.11701101716769,
5.06886055043418));
#162036=CARTESIAN_POINT('Ctrl Pts',(0.160664340009819,8.12625659815997,
5.07694674406796));
#162037=CARTESIAN_POINT('Ctrl Pts',(-0.0450043799496586,8.12772803245504,
5.08503293770174));
#162038=CARTESIAN_POINT('Ctrl Pts',(-0.250578138511302,8.1213852364606,
5.09311913133552));
#162039=CARTESIAN_POINT('Ctrl Pts',(-0.455968534985882,8.11504809794073,
5.10119811246635));
#162040=CARTESIAN_POINT('Ctrl Pts',(-0.661263823822632,8.10091063622865,
5.10927709359718));
#162041=CARTESIAN_POINT('Ctrl Pts',(-0.865847974163694,8.07898476593047,
5.117356074728));
#162042=CARTESIAN_POINT('Ctrl Pts',(-1.07027758216294,8.0570754583784,5.12542895301723));
#162043=CARTESIAN_POINT('Ctrl Pts',(-1.27399680900844,8.02738950775516,
5.13350183130646));
#162044=CARTESIAN_POINT('Ctrl Pts',(-1.47639234688607,7.98999081354642,
5.14157470959568));
#162045=CARTESIAN_POINT('Ctrl Pts',(-1.67866259284557,7.95261527080724,
5.14964259041107));
#162046=CARTESIAN_POINT('Ctrl Pts',(-1.87961047327186,7.90753656362804,
5.15771047122645));
#162047=CARTESIAN_POINT('Ctrl Pts',(-2.07862988130234,7.85487016945901,
5.16577835204184));
#162048=CARTESIAN_POINT('Ctrl Pts',(-2.27755319075201,7.80222920580345,
5.17384233719748));
#162049=CARTESIAN_POINT('Ctrl Pts',(-2.47454957933523,7.74200794346335,
5.18190632235312));
#162050=CARTESIAN_POINT('Ctrl Pts',(-2.66902456627974,7.6743726406199,5.18997030750876));
#162051=CARTESIAN_POINT('Ctrl Pts',(-2.86620213686945,7.60579742223165,
5.19814635640453));
#162052=CARTESIAN_POINT('Ctrl Pts',(-3.06078738364896,7.52960064206599,
5.20632240530029));
#162053=CARTESIAN_POINT('Ctrl Pts',(-3.25217684153511,7.44600788032639,
5.21449845419605));
#162054=CARTESIAN_POINT('Ctrl Pts',(-3.44085361458228,7.36359993210748,
5.22255861873681));
#162055=CARTESIAN_POINT('Ctrl Pts',(-3.626424296388,7.27400440932727,5.23061878327756));
#162056=CARTESIAN_POINT('Ctrl Pts',(-3.8083307277502,7.17748595474583,5.23867894781831));
#162057=CARTESIAN_POINT('Ctrl Pts',(-3.9902283702988,7.08097216345584,5.24673872293202));
#162058=CARTESIAN_POINT('Ctrl Pts',(-4.16846183575713,6.9775362560542,5.25479849804573));
#162059=CARTESIAN_POINT('Ctrl Pts',(-4.34249723919958,6.86748900909525,
5.26285827315944));
#162060=CARTESIAN_POINT('Ctrl Pts',(-4.51654578253325,6.75743345343113,
5.27091865679628));
#162061=CARTESIAN_POINT('Ctrl Pts',(-4.68639536425903,6.64076573241742,
5.27897904043312));
#162062=CARTESIAN_POINT('Ctrl Pts',(-4.85154027747262,6.51784047814618,
5.28703942406996));
#162063=CARTESIAN_POINT('Ctrl Pts',(-5.02083658679712,6.39182514127668,
5.29530242881472));
#162064=CARTESIAN_POINT('Ctrl Pts',(-5.18518831100657,6.25923374809879,
5.30356543355948));
#162065=CARTESIAN_POINT('Ctrl Pts',(-5.34408573461268,6.12049305396299,
5.31182843830423));
#162066=CARTESIAN_POINT('Ctrl Pts',(-5.49921422051319,5.98504319375995,
5.31989545025416));
#162067=CARTESIAN_POINT('Ctrl Pts',(-5.64914399369161,5.84373267320644,
5.32796246220408));
#162068=CARTESIAN_POINT('Ctrl Pts',(-5.79343706396068,5.69699697633996,
5.33602947415401));
#162069=CARTESIAN_POINT('Ctrl Pts',(-5.94298866160503,5.54491373452579,
5.34439047529618));
#162070=CARTESIAN_POINT('Ctrl Pts',(-6.08648473877691,5.38700273511236,
5.35275147643835));
#162071=CARTESIAN_POINT('Ctrl Pts',(-6.22348204251012,5.22378778560672,
5.36111247758053));
#162072=CARTESIAN_POINT('Ctrl Pts',(-6.36047934624334,5.06057283610108,
5.3694734787227));
#162073=CARTESIAN_POINT('Ctrl Pts',(-6.49097766467865,4.89205424938621,
5.37783447986487));
#162074=CARTESIAN_POINT('Ctrl Pts',(-6.61458230332845,4.71879100141065,
5.38619548100704));
#162075=CARTESIAN_POINT('Ctrl Pts',(-6.72661508444199,4.56174864646745,
5.39377372581309));
#162076=CARTESIAN_POINT('Ctrl Pts',(-6.83320887724693,4.40049359157615,
5.40135197061913));
#162077=CARTESIAN_POINT('Ctrl Pts',(-6.93401765419816,4.23545590624767,
5.40893021542518));
#162078=CARTESIAN_POINT('Ctrl Pts',(-7.03475141668576,4.07054102980367,
5.41650282105985));
#162079=CARTESIAN_POINT('Ctrl Pts',(-7.1297085367821,3.90184943399813,5.42407542669452));
#162080=CARTESIAN_POINT('Ctrl Pts',(-7.21858444593699,3.72984264539091,
5.43164803232919));
#162081=CARTESIAN_POINT('Ctrl Pts',(-7.30741109748623,3.55793118793294,
5.43921644100627));
#162082=CARTESIAN_POINT('Ctrl Pts',(-7.39016307655815,3.38270851918058,
5.44678484968334));
#162083=CARTESIAN_POINT('Ctrl Pts',(-7.46658023023578,3.20466335641549,
5.45435325836042));
#162084=CARTESIAN_POINT('Ctrl Pts',(-7.54297892091693,3.02666121078799,
5.46191983844933));
#162085=CARTESIAN_POINT('Ctrl Pts',(-7.61304568045102,2.84583826262366,
5.46948641853824));
#162086=CARTESIAN_POINT('Ctrl Pts',(-7.6765672014734,2.66270606033839,5.47705299862715));
#162087=CARTESIAN_POINT('Ctrl Pts',(-7.7400774540643,2.47960634488027,5.48461823643886));
#162088=CARTESIAN_POINT('Ctrl Pts',(-7.79704466169135,2.29419853912275,
5.49218347425057));
#162089=CARTESIAN_POINT('Ctrl Pts',(-7.84730449065638,2.10701205345965,
5.49974871206228));
#162090=CARTESIAN_POINT('Ctrl Pts',(-7.89758179737495,1.91976047407596,
5.50731658067009));
#162091=CARTESIAN_POINT('Ctrl Pts',(-7.94114696698577,1.73072933381126,
5.5148844492779));
#162092=CARTESIAN_POINT('Ctrl Pts',(-7.97788605957186,1.5404614837733,5.52245231788571));
#162093=CARTESIAN_POINT('Ctrl Pts',(-8.0141510545858,1.35264893459905,5.52992252735497));
#162094=CARTESIAN_POINT('Ctrl Pts',(-8.04376507047298,1.16363175200847,
5.53739273682422));
#162095=CARTESIAN_POINT('Ctrl Pts',(-8.06666783720681,0.9739392007067,5.54486294629347));
#162096=CARTESIAN_POINT('Ctrl Pts',(-8.09519843192592,0.737634069308306,
5.5541687878676));
#162097=CARTESIAN_POINT('Ctrl Pts',(-8.11330244404707,0.500397178607468,
5.56347462944173));
#162098=CARTESIAN_POINT('Ctrl Pts',(-8.12099040105428,0.263063620601914,
5.57278047101585));
#162099=CARTESIAN_POINT('Ctrl Pts',(-8.12871963316337,0.0244558662428032,
5.58213627379016));
#162100=CARTESIAN_POINT('Ctrl Pts',(-8.12592071876027,-0.214249548839692,
5.59149207656446));
#162101=CARTESIAN_POINT('Ctrl Pts',(-8.11265618823322,-0.452213593361826,
5.60084787933876));
#162102=CARTESIAN_POINT('Ctrl Pts',(-8.09932726561922,-0.691332823995937,
5.61024909945102));
#162103=CARTESIAN_POINT('Ctrl Pts',(-8.07543089672325,-0.92970342792701,
5.61965031956329));
#162104=CARTESIAN_POINT('Ctrl Pts',(-8.04108212224408,-1.16648440445067,
5.62905153967555));
#162105=CARTESIAN_POINT('Ctrl Pts',(-8.00669617218807,-1.40352164832363,
5.63846293470048));
#162106=CARTESIAN_POINT('Ctrl Pts',(-7.96183520505301,-1.63896578837552,
5.64787432972541));
#162107=CARTESIAN_POINT('Ctrl Pts',(-7.90666577561126,-1.8719839409775,
5.65728572475034));
#162108=CARTESIAN_POINT('Ctrl Pts',(-7.85156106085704,-2.10472875928746,
5.66668608004739));
#162109=CARTESIAN_POINT('Ctrl Pts',(-7.78617206616532,-2.33505324380799,
5.67608643534444));
#162110=CARTESIAN_POINT('Ctrl Pts',(-7.71071543733702,-2.56213875637376,
5.68548679064149));
#162111=CARTESIAN_POINT('Ctrl Pts',(-7.66243673705226,-2.70743272948673,
5.6915013309543));
#162112=CARTESIAN_POINT('Ctrl Pts',(-7.61003766399274,-2.85140099218548,
5.69751587126711));
#162113=CARTESIAN_POINT('Ctrl Pts',(-7.55358586981176,-2.99383167026474,
5.70353041157992));
#162114=CARTESIAN_POINT('Ctrl Pts',(-7.48091753331546,-3.17717748933431,
5.71127271004293));
#162115=CARTESIAN_POINT('Ctrl Pts',(-7.40149660188222,-3.35806044101228,
5.71901500850595));
#162116=CARTESIAN_POINT('Ctrl Pts',(-7.31551774020827,-3.53594227260543,
5.72675730696896));
#162117=CARTESIAN_POINT('Ctrl Pts',(-7.22959243558202,-3.71371329992003,
5.7344947826809));
#162118=CARTESIAN_POINT('Ctrl Pts',(-7.13711748749244,-3.88848661264783,
5.74223225839283));
#162119=CARTESIAN_POINT('Ctrl Pts',(-7.03833594562911,-4.05974317894189,
5.74996973410476));
#162120=CARTESIAN_POINT('Ctrl Pts',(-6.93959837940351,-4.2309235051148,
5.7577037652417));
#162121=CARTESIAN_POINT('Ctrl Pts',(-6.83455998714991,-4.39858989752977,
5.76543779637864));
#162122=CARTESIAN_POINT('Ctrl Pts',(-6.72351016729135,-4.56224709905435,
5.77317182751558));
#162123=CARTESIAN_POINT('Ctrl Pts',(-6.61247455831453,-4.72588335760812,
5.78090486893996));
#162124=CARTESIAN_POINT('Ctrl Pts',(-6.49542924588141,-4.88551115071757,
5.78863791036433));
#162125=CARTESIAN_POINT('Ctrl Pts',(-6.37270764469657,-5.04066313472006,
5.79637095178871));
#162126=CARTESIAN_POINT('Ctrl Pts',(-6.24999830330982,-5.19579961915296,
5.80410322068791));
#162127=CARTESIAN_POINT('Ctrl Pts',(-6.12161402475157,-5.34646091018045,
5.81183548958711));
#162128=CARTESIAN_POINT('Ctrl Pts',(-5.98792921918407,-5.49221187032525,
5.81956775848631));
#162129=CARTESIAN_POINT('Ctrl Pts',(-5.85419299115056,-5.63801889423708,
5.82730300163777));
#162130=CARTESIAN_POINT('Ctrl Pts',(-5.71515240164898,-5.77891155295762,
5.83503824478923));
#162131=CARTESIAN_POINT('Ctrl Pts',(-5.57121996140689,-5.91449031651261,
5.84277348794069));
#162132=CARTESIAN_POINT('Ctrl Pts',(-5.45074110708877,-6.02797671384943,
5.84924828424924));
#162133=CARTESIAN_POINT('Ctrl Pts',(-5.32683549395849,-6.13774047173051,
5.85572308055778));
#162134=CARTESIAN_POINT('Ctrl Pts',(-5.1997633585022,-6.24356857719029,
5.86219787686633));
#162135=CARTESIAN_POINT('Ctrl Pts',(-5.03463161213713,-6.38109345474372,
5.87061195142287));
#162136=CARTESIAN_POINT('Ctrl Pts',(-4.86407241924091,-6.51203776821705,
5.87902602597942));
#162137=CARTESIAN_POINT('Ctrl Pts',(-4.6886237841604,-6.63599989248835,
5.88744010053596));
#162138=CARTESIAN_POINT('Ctrl Pts',(-4.51312615108145,-6.75999663598578,
5.89585652491308));
#162139=CARTESIAN_POINT('Ctrl Pts',(-4.33273656549878,-6.87700714520411,
5.90427294929019));
#162140=CARTESIAN_POINT('Ctrl Pts',(-4.14802246900494,-6.98667282468058,
5.9126893736673));
#162141=CARTESIAN_POINT('Ctrl Pts',(-3.96326256468477,-7.0963657004918,
5.92110788525982));
#162142=CARTESIAN_POINT('Ctrl Pts',(-3.7741762353731,-7.19870997543418,
5.92952639685233));
#162143=CARTESIAN_POINT('Ctrl Pts',(-3.58135694828023,-7.29339221292156,
5.93794490844484));
#162144=CARTESIAN_POINT('Ctrl Pts',(-3.38846360009358,-7.38811081746629,
5.94636665355297));
#162145=CARTESIAN_POINT('Ctrl Pts',(-3.1918346653308,-7.4751613859921,5.9547883986611));
#162146=CARTESIAN_POINT('Ctrl Pts',(-2.9920863848915,-7.55427737297532,
5.96321014376923));
#162147=CARTESIAN_POINT('Ctrl Pts',(-2.79231645228214,-7.63340193591624,
5.97163280177162));
#162148=CARTESIAN_POINT('Ctrl Pts',(-2.58942674539637,-7.704590105673,5.980055459774));
#162149=CARTESIAN_POINT('Ctrl Pts',(-2.38405213892045,-7.76762402291774,
5.98847811777639));
#162150=CARTESIAN_POINT('Ctrl Pts',(-2.17863847611245,-7.83066992739716,
5.99690237752562));
#162151=CARTESIAN_POINT('Ctrl Pts',(-1.97073922199153,-7.88555840405078,
6.00532663727485));
#162152=CARTESIAN_POINT('Ctrl Pts',(-1.7610042924744,-7.93212149707673,
6.01375089702408));
#162153=CARTESIAN_POINT('Ctrl Pts',(-1.70196260050231,-7.94522929844312,
6.01612237873364));
#162154=CARTESIAN_POINT('Ctrl Pts',(-1.64277551537179,-7.95767765612669,
6.01849386044321));
#162155=CARTESIAN_POINT('Ctrl Pts',(-1.58345770236731,-7.96946354953165,
6.02086534215277));
#162156=CARTESIAN_POINT('Ctrl Pts',(-1.37274026585278,-8.0113311289237,
6.02928966734735));
#162157=CARTESIAN_POINT('Ctrl Pts',(-1.16035067532255,-8.04483934999749,
6.03771399254192));
#162158=CARTESIAN_POINT('Ctrl Pts',(-0.946951430774239,-8.06988045452066,
6.0461383177365));
#162159=CARTESIAN_POINT('Ctrl Pts',(-0.733589064234515,-8.09491723163364,
6.05456118710428));
#162160=CARTESIAN_POINT('Ctrl Pts',(-0.519217654164309,-8.11148978395286,
6.06298405647207));
#162161=CARTESIAN_POINT('Ctrl Pts',(-0.304506020712815,-8.11954208350752,
6.07140692583985));
#162162=CARTESIAN_POINT('Ctrl Pts',(-0.0898382639491243,-8.12759273756106,
6.07982807397994));
#162163=CARTESIAN_POINT('Ctrl Pts',(0.125169313769842,-8.1271266058822,
6.08824922212004));
#162164=CARTESIAN_POINT('Ctrl Pts',(0.339845578329916,-8.11813972196769,
6.09667037026013));
#162165=CARTESIAN_POINT('Ctrl Pts',(0.554461611973064,-8.10915535946959,
6.10508915571017));
#162166=CARTESIAN_POINT('Ctrl Pts',(0.76874625460702,-8.09165503050455,
6.11350794116021));
#162167=CARTESIAN_POINT('Ctrl Pts',(0.982030167741453,-8.06568684689318,
6.12192672661026));
#162168=CARTESIAN_POINT('Ctrl Pts',(1.19525450144443,-8.03972591731983,
6.13034316032902));
#162169=CARTESIAN_POINT('Ctrl Pts',(1.40747840200391,-8.00530188782437,
6.13875959404778));
#162170=CARTESIAN_POINT('Ctrl Pts',(1.61803826996039,-7.96251466054811,
6.14717602776654));
#162171=CARTESIAN_POINT('Ctrl Pts',(1.82852171693458,-7.91974296254611,
6.1555894068095));
#162172=CARTESIAN_POINT('Ctrl Pts',(2.03734207895128,-7.86861418081482,
6.16400278585247));
#162173=CARTESIAN_POINT('Ctrl Pts',(2.2438455737859,-7.80927939079538,6.17241616489543));
#162174=CARTESIAN_POINT('Ctrl Pts',(2.30207075494353,-7.79254950978005,
6.17478837907668));
#162175=CARTESIAN_POINT('Ctrl Pts',(2.3601118139356,-7.7751675618776,6.17716059325793));
#162176=CARTESIAN_POINT('Ctrl Pts',(2.41795427037059,-7.75713766210814,
6.17953280743918));
#162177=CARTESIAN_POINT('Ctrl Pts',(2.60656375600892,-7.69834676125057,
6.18726799235569));
#162178=CARTESIAN_POINT('Ctrl Pts',(2.79314417217995,-7.63263656410289,
6.19500317727219));
#162179=CARTESIAN_POINT('Ctrl Pts',(2.97714785180455,-7.56017712960454,
6.2027383621887));
#162180=CARTESIAN_POINT('Ctrl Pts',(3.1610946329462,-7.48774010135321,6.21047115519495));
#162181=CARTESIAN_POINT('Ctrl Pts',(3.34246593595063,-7.40855812119425,
6.21820394820121));
#162182=CARTESIAN_POINT('Ctrl Pts',(3.52073143724983,-7.32285038146081,
6.22593674120747));
#162183=CARTESIAN_POINT('Ctrl Pts',(3.69897348706952,-7.23715391689439,
6.23366851693649));
#162184=CARTESIAN_POINT('Ctrl Pts',(3.87411023102477,-7.14493355647251,
6.24140029266551));
#162185=CARTESIAN_POINT('Ctrl Pts',(4.04563331373399,-7.04645575117773,
6.24913206839453));
#162186=CARTESIAN_POINT('Ctrl Pts',(4.21721777208604,-6.94794270783505,
6.25686661076403));
#162187=CARTESIAN_POINT('Ctrl Pts',(4.38518567693939,-6.84316791854296,
6.26460115313354));
#162188=CARTESIAN_POINT('Ctrl Pts',(4.54905461260978,-6.73244307023785,
6.27233569550305));
#162189=CARTESIAN_POINT('Ctrl Pts',(4.71295122391648,-6.6216995217403,6.28007154415053));
#162190=CARTESIAN_POINT('Ctrl Pts',(4.87274719809861,-6.50500411610102,
6.28780739279802));
#162191=CARTESIAN_POINT('Ctrl Pts',(5.02799078569935,-6.38271072675414,
6.29554324144551));
#162192=CARTESIAN_POINT('Ctrl Pts',(5.18336140063324,-6.26031727141839,
6.30328541991465));
#162193=CARTESIAN_POINT('Ctrl Pts',(5.33417191366276,-6.13231690544928,
6.31102759838379));
#162194=CARTESIAN_POINT('Ctrl Pts',(5.4800045279485,-5.99910309431034,6.31876977685294));
#162195=CARTESIAN_POINT('Ctrl Pts',(5.60200292160804,-5.88766114388099,
6.3252466088105));
#162196=CARTESIAN_POINT('Ctrl Pts',(5.72051813165079,-5.77257137445318,
6.33172344076807));
#162197=CARTESIAN_POINT('Ctrl Pts',(5.8353262874522,-5.6540830097788,6.33820027272563));
#162198=CARTESIAN_POINT('Ctrl Pts',(6.00191549708611,-5.48215373450969,
6.34759830119504));
#162199=CARTESIAN_POINT('Ctrl Pts',(6.16079438656214,-5.3029712452053,6.35699632966446));
#162200=CARTESIAN_POINT('Ctrl Pts',(6.3114230822179,-5.11718929098261,6.36639435813387));
#162201=CARTESIAN_POINT('Ctrl Pts',(6.46226610989966,-4.93114298458938,
6.37580575921115));
#162202=CARTESIAN_POINT('Ctrl Pts',(6.60483543793473,-4.73847845832144,
6.38521716028845));
#162203=CARTESIAN_POINT('Ctrl Pts',(6.73863144967037,-4.53988256984841,
6.39462856136573));
#162204=CARTESIAN_POINT('Ctrl Pts',(6.87222600892987,-4.3415857010021,6.40402579199036));
#162205=CARTESIAN_POINT('Ctrl Pts',(6.9970736359882,-4.13737535138648,6.41342302261498));
#162206=CARTESIAN_POINT('Ctrl Pts',(7.1127195336528,-3.92796491813431,6.4228202532396));
#162207=CARTESIAN_POINT('Ctrl Pts',(7.22807372922396,-3.71908269611144,
6.43219378054313));
#162208=CARTESIAN_POINT('Ctrl Pts',(7.33427252055881,-3.5050266135619,6.44156730784666));
#162209=CARTESIAN_POINT('Ctrl Pts',(7.4309073037858,-3.28653376751903,6.45094083515019));
#162210=CARTESIAN_POINT('Ctrl Pts',(7.52691454640957,-3.06945980117793,
6.46025349131827));
#162211=CARTESIAN_POINT('Ctrl Pts',(7.61348155627842,-2.84800654052336,
6.46956614748636));
#162212=CARTESIAN_POINT('Ctrl Pts',(7.69025040874438,-2.62292512537186,
6.47887880365445));
#162213=CARTESIAN_POINT('Ctrl Pts',(7.73968098375228,-2.47799780892583,
6.48487511510698));
#162214=CARTESIAN_POINT('Ctrl Pts',(7.78505018096513,-2.33156685795491,
6.49087142655951));
#162215=CARTESIAN_POINT('Ctrl Pts',(7.82627209184742,-2.18383898373259,
6.49686773801204));
#162216=CARTESIAN_POINT('Ctrl Pts',(7.87610976657735,-2.00523460595254,
6.50411733448523));
#162217=CARTESIAN_POINT('Ctrl Pts',(7.91987916280345,-1.82474445529073,
6.51136693095843));
#162218=CARTESIAN_POINT('Ctrl Pts',(7.9574296753959,-1.64286351339015,6.51861652743162));
#162219=CARTESIAN_POINT('Ctrl Pts',(7.99496808093457,-1.46104121362771,
6.52586378648654));
#162220=CARTESIAN_POINT('Ctrl Pts',(8.02629151042615,-1.27782939594045,
6.53311104554146));
#162221=CARTESIAN_POINT('Ctrl Pts',(8.05129984720199,-1.0937359521133,6.54035830459638));
#162222=CARTESIAN_POINT('Ctrl Pts',(8.07631239206426,-0.909611531371167,
6.54760678312834));
#162223=CARTESIAN_POINT('Ctrl Pts',(8.09500765887235,-0.724605573874979,
6.5548552616603));
#162224=CARTESIAN_POINT('Ctrl Pts',(8.10733706991169,-0.539233898540962,
6.56210374019226));
#162225=CARTESIAN_POINT('Ctrl Pts',(8.11935365494763,-0.35856553629746,
6.56916830786564));
#162226=CARTESIAN_POINT('Ctrl Pts',(8.1253235154935,-0.177550143507737,
6.57623287553903));
#162227=CARTESIAN_POINT('Ctrl Pts',(8.12524931639108,0.00333301459649942,
6.58329744321241));
#162228=CARTESIAN_POINT('',(8.1252500832311,-0.00151305119605756,10.5836787518598));
#162229=CARTESIAN_POINT('Ctrl Pts',(8.1252493577062,0.00323072670080068,
6.5857174746832));
#162230=CARTESIAN_POINT('Ctrl Pts',(8.12506851487489,0.458048863603974,
6.60495129592261));
#162231=CARTESIAN_POINT('Ctrl Pts',(8.08669999959761,0.91206338244344,6.6243674061125));
#162232=CARTESIAN_POINT('Ctrl Pts',(8.00331728191846,1.40301841636916,6.64449536413657));
#162233=CARTESIAN_POINT('Ctrl Pts',(7.99575615035507,1.4454867178715,6.64622858465563));
#162234=CARTESIAN_POINT('Ctrl Pts',(7.98533186637207,1.50145020413107,6.64850049919071));
#162235=CARTESIAN_POINT('Ctrl Pts',(7.98277209453259,1.51500079901468,6.64904966738446));
#162236=CARTESIAN_POINT('Ctrl Pts',(7.97758522937364,1.54208021779063,6.65014516253916));
#162237=CARTESIAN_POINT('Ctrl Pts',(7.97495818822034,1.55560900901587,6.65069148943679));
#162238=CARTESIAN_POINT('Ctrl Pts',(7.97057719053874,1.57786757842396,6.65158866374817));
#162239=CARTESIAN_POINT('Ctrl Pts',(7.96884328695497,1.58660124609189,6.65194026390858));
#162240=CARTESIAN_POINT('Ctrl Pts',(7.96572449629611,1.60217649970945,6.65256650971597));
#162241=CARTESIAN_POINT('Ctrl Pts',(7.96434514416166,1.6090191770655,6.6528413684856));
#162242=CARTESIAN_POINT('Ctrl Pts',(7.96166200618667,1.62224167850085,6.65337196125073));
#162243=CARTESIAN_POINT('Ctrl Pts',(7.96035936555062,1.62862172889939,6.65362774010539));
#162244=CARTESIAN_POINT('Ctrl Pts',(7.95766572554249,1.64173415097857,6.65415291961192));
#162245=CARTESIAN_POINT('Ctrl Pts',(7.95627384865523,1.64846633799888,6.65442228483655));
#162246=CARTESIAN_POINT('Ctrl Pts',(7.95291096889975,1.66462833359493,6.65506828295408));
#162247=CARTESIAN_POINT('Ctrl Pts',(7.95093173341598,1.67405643269761,6.65544457922563));
#162248=CARTESIAN_POINT('Ctrl Pts',(7.94367465385001,1.70832237244617,6.65681016453348));
#162249=CARTESIAN_POINT('Ctrl Pts',(7.93829711754992,1.73313912534099,6.65779526868028));
#162250=CARTESIAN_POINT('Ctrl Pts',(7.85527509273323,2.10778272548637,6.6726033866534));
#162251=CARTESIAN_POINT('Ctrl Pts',(7.75468717983921,2.45212727384615,6.68527878474658));
#162252=CARTESIAN_POINT('Ctrl Pts',(7.60886089427707,2.85120154610489,6.69979572936306));
#162253=CARTESIAN_POINT('Ctrl Pts',(7.58525845803258,2.91341185007144,6.70205371008332));
#162254=CARTESIAN_POINT('Ctrl Pts',(7.52305042414752,3.07149484230334,6.70779144781689));
#162255=CARTESIAN_POINT('Ctrl Pts',(7.4833747926049,3.1669338838541,6.71125550356128));
#162256=CARTESIAN_POINT('Ctrl Pts',(7.38259362292187,3.39688374256376,6.71964568119447));
#162257=CARTESIAN_POINT('Ctrl Pts',(7.31961965685809,3.53053478886467,6.72455970264925));
#162258=CARTESIAN_POINT('Ctrl Pts',(7.10028125540747,3.96491440246287,6.74081570347696));
#162259=CARTESIAN_POINT('Ctrl Pts',(6.92875210910965,4.25757238634734,6.75224253116121));
#162260=CARTESIAN_POINT('Ctrl Pts',(6.61099920012536,4.72940411045619,6.77226320482249));
#162261=CARTESIAN_POINT('Ctrl Pts',(6.47450707693038,4.91460309634165,6.7805744202096));
#162262=CARTESIAN_POINT('Ctrl Pts',(6.25761448044106,5.18414984621858,6.79350908661515));
#162263=CARTESIAN_POINT('Ctrl Pts',(6.18295404121457,5.27297133140727,6.79791721325621));
#162264=CARTESIAN_POINT('Ctrl Pts',(6.09226463307138,5.37628678244633,6.80322894855996));
#162265=CARTESIAN_POINT('Ctrl Pts',(6.07804647112951,5.39235560890253,6.80406050199459));
#162266=CARTESIAN_POINT('Ctrl Pts',(6.05608061211405,5.41698333546571,6.80534337514342));
#162267=CARTESIAN_POINT('Ctrl Pts',(6.04837799741681,5.42558240525059,6.80579289271527));
#162268=CARTESIAN_POINT('Ctrl Pts',(6.03487703792565,5.44059016940609,6.80658021394662));
#162269=CARTESIAN_POINT('Ctrl Pts',(6.02908673732833,5.44700609211496,6.80691769456274));
#162270=CARTESIAN_POINT('Ctrl Pts',(6.01692205815316,5.4604419620549,6.80762631208383));
#162271=CARTESIAN_POINT('Ctrl Pts',(6.01054560751961,5.4674600111999,6.80799753225109));
#162272=CARTESIAN_POINT('Ctrl Pts',(5.99277641454043,5.48694848837617,6.80903140040465));
#162273=CARTESIAN_POINT('Ctrl Pts',(5.98135707903818,5.49939454464192,6.80969512200837));
#162274=CARTESIAN_POINT('Ctrl Pts',(5.93567853747192,5.5488694969207,6.81234737819525));
#162275=CARTESIAN_POINT('Ctrl Pts',(5.90111397066161,5.5856142175783,6.81434830590851));
#162276=CARTESIAN_POINT('Ctrl Pts',(5.25270631991151,6.26218343549144,6.85177831546235));
#162277=CARTESIAN_POINT('Ctrl Pts',(4.53861672800915,6.7975172662044,6.89209952473709));
#162278=CARTESIAN_POINT('Ctrl Pts',(3.52519598912004,7.3251848441121,6.94297758991279));
#162279=CARTESIAN_POINT('Ctrl Pts',(3.29244869271108,7.43270704362022,6.95422539958008));
#162280=CARTESIAN_POINT('Ctrl Pts',(2.96263572692282,7.56653241722902,6.96924913864206));
#162281=CARTESIAN_POINT('Ctrl Pts',(2.86958686411492,7.60230857997144,6.97338962316836));
#162282=CARTESIAN_POINT('Ctrl Pts',(2.72155291514907,7.65612050878128,6.97979943098742));
#162283=CARTESIAN_POINT('Ctrl Pts',(2.66699560334524,7.67529583024132,6.98212381510126));
#162284=CARTESIAN_POINT('Ctrl Pts',(2.59849408190045,7.69855354794333,6.98499969329111));
#162285=CARTESIAN_POINT('Ctrl Pts',(2.58473789961544,7.70318299264376,6.98557507933486));
#162286=CARTESIAN_POINT('Ctrl Pts',(2.56418191238656,7.71003955095519,6.98643178749436));
#162287=CARTESIAN_POINT('Ctrl Pts',(2.5573914955036,7.7122945675236,6.98671428690972));
#162288=CARTESIAN_POINT('Ctrl Pts',(2.54348585076419,7.71689208184667,6.9872917829858));
#162289=CARTESIAN_POINT('Ctrl Pts',(2.53637034312827,7.71923371578307,6.98758674361304));
#162290=CARTESIAN_POINT('Ctrl Pts',(2.52105188895716,7.72425138021242,6.98822059083882));
#162291=CARTESIAN_POINT('Ctrl Pts',(2.51284789275766,7.7269241927241,6.98855934604577));
#162292=CARTESIAN_POINT('Ctrl Pts',(2.49075974945243,7.73408147824269,6.9894695224137));
#162293=CARTESIAN_POINT('Ctrl Pts',(2.47686771996339,7.73854164185578,6.99003997287339));
#162294=CARTESIAN_POINT('Ctrl Pts',(2.41276687533607,7.75893151395074,6.9926632530704));
#162295=CARTESIAN_POINT('Ctrl Pts',(2.36241530647571,7.77441035037212,6.99469871348262));
#162296=CARTESIAN_POINT('Ctrl Pts',(1.92559200941377,7.9040607741543,7.0121643302506));
#162297=CARTESIAN_POINT('Ctrl Pts',(1.53125007587217,7.9898304307067,7.02665820915452));
#162298=CARTESIAN_POINT('Ctrl Pts',(0.659928805305274,8.11243461975554,
7.058258914541));
#162299=CARTESIAN_POINT('Ctrl Pts',(0.182783245919793,8.13717883820747,
7.07532819278513));
#162300=CARTESIAN_POINT('Ctrl Pts',(-0.466511668410448,8.1136879827477,
7.09956678266333));
#162301=CARTESIAN_POINT('Ctrl Pts',(-0.639004929851296,8.10192794173982,
7.10609483435487));
#162302=CARTESIAN_POINT('Ctrl Pts',(-0.892807870939498,8.07646849664879,
7.11585423782745));
#162303=CARTESIAN_POINT('Ctrl Pts',(-0.974496814572122,8.06701958598615,
7.11901886368915));
#162304=CARTESIAN_POINT('Ctrl Pts',(-1.08840127526852,8.05208893954448,
7.1234648236591));
#162305=CARTESIAN_POINT('Ctrl Pts',(-1.12074898971591,8.0476502977396,7.12473118787188));
#162306=CARTESIAN_POINT('Ctrl Pts',(-1.17560882179874,8.03978544162671,
7.12688522083534));
#162307=CARTESIAN_POINT('Ctrl Pts',(-1.1981349425908,8.03645933879725,7.12777151478346));
#162308=CARTESIAN_POINT('Ctrl Pts',(-1.24260074708423,8.02970261300227,
7.12952460616806));
#162309=CARTESIAN_POINT('Ctrl Pts',(-1.26454095244713,8.02627664898215,
7.13039132853214));
#162310=CARTESIAN_POINT('Ctrl Pts',(-1.31510141256166,8.01816917141084,
7.13239279191779));
#162311=CARTESIAN_POINT('Ctrl Pts',(-1.34371115593501,8.01342429342372,
7.13352838330375));
#162312=CARTESIAN_POINT('Ctrl Pts',(-1.42057873243792,8.00025270968165,
7.13658810675044));
#162313=CARTESIAN_POINT('Ctrl Pts',(-1.4687865936428,7.99154260746225,7.13851622905903));
#162314=CARTESIAN_POINT('Ctrl Pts',(-1.92540643512068,7.90477013406925,
7.15687310397061));
#162315=CARTESIAN_POINT('Ctrl Pts',(-2.32731471100886,7.79590624444567,
7.17379111161773));
#162316=CARTESIAN_POINT('Ctrl Pts',(-3.22132822465334,7.47842005584968,
7.21342263100111));
#162317=CARTESIAN_POINT('Ctrl Pts',(-3.7047640348543,7.2510978483851,7.23637391631977));
#162318=CARTESIAN_POINT('Ctrl Pts',(-4.31022689168872,6.88993764755602,
7.26572644660342));
#162319=CARTESIAN_POINT('Ctrl Pts',(-4.45517323706194,6.79711201938735,
7.27279269848444));
#162320=CARTESIAN_POINT('Ctrl Pts',(-4.62354053657463,6.68158598845901,
7.28096824325882));
#162321=CARTESIAN_POINT('Ctrl Pts',(-4.64990688479634,6.66326379565898,
7.28224752677352));
#162322=CARTESIAN_POINT('Ctrl Pts',(-4.68574312931519,6.63804459817739,
7.28398424347574));
#162323=CARTESIAN_POINT('Ctrl Pts',(-4.69530755491471,6.63128281162708,
7.28444756009791));
#162324=CARTESIAN_POINT('Ctrl Pts',(-4.71059955764046,6.62042211455746,
7.2851879708793));
#162325=CARTESIAN_POINT('Ctrl Pts',(-4.71633646639644,6.61633641099674,
7.28546566027693));
#162326=CARTESIAN_POINT('Ctrl Pts',(-4.72823132082869,6.60784181843816,
7.2860412393571));
#162327=CARTESIAN_POINT('Ctrl Pts',(-4.73438843127363,6.60343176712427,
7.28633907508634));
#162328=CARTESIAN_POINT('Ctrl Pts',(-4.74847081582593,6.59331539101312,
7.28702003277565));
#162329=CARTESIAN_POINT('Ctrl Pts',(-4.75639199526871,6.58760336712136,
7.28740288588776));
#162330=CARTESIAN_POINT('Ctrl Pts',(-4.7812657306256,6.56959847157609,7.28860450010607));
#162331=CARTESIAN_POINT('Ctrl Pts',(-4.79818115619207,6.55725427809367,
7.28942077550516));
#162332=CARTESIAN_POINT('Ctrl Pts',(-4.9836946525188,6.42077181501787,7.29836166164221));
#162333=CARTESIAN_POINT('Ctrl Pts',(-5.14747592292401,6.29023160081385,
7.30611111194316));
#162334=CARTESIAN_POINT('Ctrl Pts',(-5.83512534767394,5.69728655314435,
7.33859483463413));
#162335=CARTESIAN_POINT('Ctrl Pts',(-6.30319005430231,5.17471520366987,
7.36088202334357));
#162336=CARTESIAN_POINT('Ctrl Pts',(-6.92858383190715,4.2637394856707,7.39923867065006));
#162337=CARTESIAN_POINT('Ctrl Pts',(-7.13306093305325,3.91205172482726,
7.41390827205031));
#162338=CARTESIAN_POINT('Ctrl Pts',(-7.32446622966944,3.51751680673151,
7.43077356318846));
#162339=CARTESIAN_POINT('Ctrl Pts',(-7.33838586369557,3.48838399871033,
7.43202097217626));
#162340=CARTESIAN_POINT('Ctrl Pts',(-7.35793632868408,3.44683136587635,
7.43380328280909));
#162341=CARTESIAN_POINT('Ctrl Pts',(-7.36371017945046,3.4344789812522,7.43433350030101));
#162342=CARTESIAN_POINT('Ctrl Pts',(-7.37359982794669,3.41318181290075,
7.43524835003641));
#162343=CARTESIAN_POINT('Ctrl Pts',(-7.37773051756353,3.40424395717882,
7.43563249491743));
#162344=CARTESIAN_POINT('Ctrl Pts',(-7.38558937038807,3.38715773319133,
7.4363672534548));
#162345=CARTESIAN_POINT('Ctrl Pts',(-7.38932032210059,3.37901065909877,
7.43671777546324));
#162346=CARTESIAN_POINT('Ctrl Pts',(-7.39800051083408,3.35997308058562,
7.43753726377785));
#162347=CARTESIAN_POINT('Ctrl Pts',(-7.40293918386998,3.34907779829207,
7.43800657306172));
#162348=CARTESIAN_POINT('Ctrl Pts',(-7.41981616146235,3.31162550581032,
7.43962090391658));
#162349=CARTESIAN_POINT('Ctrl Pts',(-7.43163570069759,3.28501539591612,
7.44076977750974));
#162350=CARTESIAN_POINT('Ctrl Pts',(-7.55477318034031,3.00372186510362,
7.4529348925732));
#162351=CARTESIAN_POINT('Ctrl Pts',(-7.65308820831105,2.74356796448362,
7.46437073609428));
#162352=CARTESIAN_POINT('Ctrl Pts',(-7.83492931251577,2.17595230680987,
7.48970513956059));
#162353=CARTESIAN_POINT('Ctrl Pts',(-7.91410156959003,1.86758154772862,
7.50370154779696));
#162354=CARTESIAN_POINT('Ctrl Pts',(-8.04804951627489,1.18078267618282,
7.53501007428641));
#162355=CARTESIAN_POINT('Ctrl Pts',(-8.09462380115126,0.801506318363753,
7.55239154354304));
#162356=CARTESIAN_POINT('Ctrl Pts',(-8.13214650837807,0.077198212269558,
7.58465864371618));
#162357=CARTESIAN_POINT('Ctrl Pts',(-8.12813840593303,-0.266780047999812,
7.5995790610305));
#162358=CARTESIAN_POINT('Ctrl Pts',(-8.098824885156,-0.656461255678929,
7.61537839712574));
#162359=CARTESIAN_POINT('Ctrl Pts',(-8.09488351424861,-0.703396675891562,
7.61726282406029));
#162360=CARTESIAN_POINT('Ctrl Pts',(-8.08931697511869,-0.7634213810071,
7.61965197660907));
#162361=CARTESIAN_POINT('Ctrl Pts',(-8.08806778321992,-0.776544181494922,
7.62017302712088));
#162362=CARTESIAN_POINT('Ctrl Pts',(-8.08600943193197,-0.797623335483167,
7.62100802328078));
#162363=CARTESIAN_POINT('Ctrl Pts',(-8.08522045480616,-0.805581601330433,
7.62132281863089));
#162364=CARTESIAN_POINT('Ctrl Pts',(-8.08369928627636,-0.820697986996388,
7.62191992348114));
#162365=CARTESIAN_POINT('Ctrl Pts',(-8.08296933370346,-0.827856320658696,
7.62220232520776));
#162366=CARTESIAN_POINT('Ctrl Pts',(-8.0812888746549,-0.844121750168679,
7.62284321776499));
#162367=CARTESIAN_POINT('Ctrl Pts',(-8.08033247961804,-0.853228237017915,
7.62320146897822));
#162368=CARTESIAN_POINT('Ctrl Pts',(-8.07782203535444,-0.87674906026654,
7.6241253692235));
#162369=CARTESIAN_POINT('Ctrl Pts',(-8.07624479327208,-0.891160923783693,
7.62469009609325));
#162370=CARTESIAN_POINT('Ctrl Pts',(-8.06652146504213,-0.977860343993965,
7.62807952882937));
#162371=CARTESIAN_POINT('Ctrl Pts',(-8.05744332515673,-1.05004135050398,
7.63086846506619));
#162372=CARTESIAN_POINT('Ctrl Pts',(-8.00424884755594,-1.43154046959468,
7.64547641591087));
#162373=CARTESIAN_POINT('Ctrl Pts',(-7.94328554737833,-1.7382576791047,
7.65677186848395));
#162374=CARTESIAN_POINT('Ctrl Pts',(-7.72260550019974,-2.5887480965958,
7.68831684905884));
#162375=CARTESIAN_POINT('Ctrl Pts',(-7.5235178714004,-3.12040490831959,
7.7084419970786));
#162376=CARTESIAN_POINT('Ctrl Pts',(-7.09285591318382,-3.9837105863508,
7.74444849594742));
#162377=CARTESIAN_POINT('Ctrl Pts',(-6.88893313626673,-4.32679253032133,
7.75969780275065));
#162378=CARTESIAN_POINT('Ctrl Pts',(-6.60591985710963,-4.73187593007761,
7.77882716238859));
#162379=CARTESIAN_POINT('Ctrl Pts',(-6.54978895402285,-4.80927140458512,
7.78253981052386));
#162380=CARTESIAN_POINT('Ctrl Pts',(-6.46411244913894,-4.92312261383116,
7.78809415863395));
#162381=CARTESIAN_POINT('Ctrl Pts',(-6.43559546286425,-4.9603424317168,
7.78992515087991));
#162382=CARTESIAN_POINT('Ctrl Pts',(-6.38367713808798,-5.02690382729935,
7.79322779586642));
#162383=CARTESIAN_POINT('Ctrl Pts',(-6.36039160390264,-5.05633409936315,
7.79469817683162));
#162384=CARTESIAN_POINT('Ctrl Pts',(-6.3100251200391,-5.11909314556633,
7.79785589629071));
#162385=CARTESIAN_POINT('Ctrl Pts',(-6.2828821535919,-5.15237066532803,
7.79954387529148));
#162386=CARTESIAN_POINT('Ctrl Pts',(-6.20871267845345,-5.24184546388572,
7.80412017936905));
#162387=CARTESIAN_POINT('Ctrl Pts',(-6.16118783837029,-5.29762411961881,
7.8070139542251));
#162388=CARTESIAN_POINT('Ctrl Pts',(-5.85225311734252,-5.65043175104563,
7.82558857621375));
#162389=CARTESIAN_POINT('Ctrl Pts',(-5.57020058014652,-5.92866748899128,
7.84150606354376));
#162390=CARTESIAN_POINT('Ctrl Pts',(-4.96505118080151,-6.44417510396032,
7.87375733276426));
#162391=CARTESIAN_POINT('Ctrl Pts',(-4.64241597843746,-6.68035203775207,
7.89004798921172));
#162392=CARTESIAN_POINT('Ctrl Pts',(-4.23425855980627,-6.93523250203518,
7.90937004372964));
#162393=CARTESIAN_POINT('Ctrl Pts',(-4.16413716740915,-6.97756098145358,
7.91264608714295));
#162394=CARTESIAN_POINT('Ctrl Pts',(-4.04427514789393,-7.04746468475808,
7.91816819050737));
#162395=CARTESIAN_POINT('Ctrl Pts',(-3.99486335153644,-7.07559091785973,
7.92042267801759));
#162396=CARTESIAN_POINT('Ctrl Pts',(-3.92423133490674,-7.11482038596776,
7.92361292894792));
#162397=CARTESIAN_POINT('Ctrl Pts',(-3.90325119953369,-7.12635185592349,
7.92455651855231));
#162398=CARTESIAN_POINT('Ctrl Pts',(-3.86756672387046,-7.14576052281125,
7.92615449538628));
#162399=CARTESIAN_POINT('Ctrl Pts',(-3.85288856488585,-7.15368545028408,
7.92680981025561));
#162400=CARTESIAN_POINT('Ctrl Pts',(-3.82184520004718,-7.17032290431969,
7.92819172803375));
#162401=CARTESIAN_POINT('Ctrl Pts',(-3.80547436039207,-7.1790247374264,
7.92891813331191));
#162402=CARTESIAN_POINT('Ctrl Pts',(-3.75880206958781,-7.20362864170807,
7.93098265723723));
#162403=CARTESIAN_POINT('Ctrl Pts',(-3.72842967365028,-7.21939545879472,
7.93231850007248));
#162404=CARTESIAN_POINT('Ctrl Pts',(-3.55079425523386,-7.31018898023141,
7.94009018230389));
#162405=CARTESIAN_POINT('Ctrl Pts',(-3.40136773590529,-7.38090112204373,
7.94646480033873));
#162406=CARTESIAN_POINT('Ctrl Pts',(-3.11776657953699,-7.50466518170462,
7.95837279081931));
#162407=CARTESIAN_POINT('Ctrl Pts',(-2.9841345834056,-7.55879678061377,
7.96390724988982));
#162408=CARTESIAN_POINT('Ctrl Pts',(-2.73010354713418,-7.65391250092677,
7.97434329094935));
#162409=CARTESIAN_POINT('Ctrl Pts',(-2.61004491476187,-7.69568107732392,
7.97924072030386));
#162410=CARTESIAN_POINT('Ctrl Pts',(-2.40315601994212,-7.76225944872292,
7.98764799393247));
#162411=CARTESIAN_POINT('Ctrl Pts',(-2.31680143967154,-7.78846978246094,
7.99114765230988));
#162412=CARTESIAN_POINT('Ctrl Pts',(-2.1880979538327,-7.82520391507167,
7.99635556931798));
#162413=CARTESIAN_POINT('Ctrl Pts',(-2.14607174852429,-7.83683386323641,
7.99805486431949));
#162414=CARTESIAN_POINT('Ctrl Pts',(-2.07333671835877,-7.85633293644145,
8.00099425411069));
#162415=CARTESIAN_POINT('Ctrl Pts',(-2.04267165781704,-7.86436169355199,
8.00223301234753));
#162416=CARTESIAN_POINT('Ctrl Pts',(-1.97377900531381,-7.88196910985819,
8.00501518301959));
#162417=CARTESIAN_POINT('Ctrl Pts',(-1.93552715516518,-7.89144950107877,
8.00655937131698));
#162418=CARTESIAN_POINT('Ctrl Pts',(-1.83128521837362,-7.91648144142791,
8.01076639455341));
#162419=CARTESIAN_POINT('Ctrl Pts',(-1.76516722070955,-7.93148589959464,
8.01343361128471));
#162420=CARTESIAN_POINT('Ctrl Pts',(-1.39418490061335,-8.01080598686902,
8.02839540584334));
#162421=CARTESIAN_POINT('Ctrl Pts',(-1.08600913143585,-8.05837101056055,
8.0408249113099));
#162422=CARTESIAN_POINT('Ctrl Pts',(-0.62364412205684,-8.10272432042586,
8.05938033546882));
#162423=CARTESIAN_POINT('Ctrl Pts',(-0.471036062616764,-8.11302648903253,
8.06548696029151));
#162424=CARTESIAN_POINT('Ctrl Pts',(-0.235710951945573,-8.12225014445922,
8.07484021313481));
#162425=CARTESIAN_POINT('Ctrl Pts',(-0.153148991548546,-8.12422627825285,
8.07810958130518));
#162426=CARTESIAN_POINT('Ctrl Pts',(-0.0432080940608028,-8.12518119167401,
8.08244047333058));
#162427=CARTESIAN_POINT('Ctrl Pts',(-0.015844260820631,-8.12528062942543,
8.08351653896995));
#162428=CARTESIAN_POINT('Ctrl Pts',(0.0312397680984873,-8.12521387554218,
8.0853645286597));
#162429=CARTESIAN_POINT('Ctrl Pts',(0.050959761725058,-8.1251141254933,
8.08613744895639));
#162430=CARTESIAN_POINT('Ctrl Pts',(0.092861406918647,-8.12474962122101,
8.08777770398095));
#162431=CARTESIAN_POINT('Ctrl Pts',(0.115042742060254,-8.12446581752494,
8.08864476788495));
#162432=CARTESIAN_POINT('Ctrl Pts',(0.174884321978119,-8.1234550432774,
8.09098098206213));
#162433=CARTESIAN_POINT('Ctrl Pts',(0.212541205609717,-8.12255702475901,
8.09244792117921));
#162434=CARTESIAN_POINT('Ctrl Pts',(0.411886184091409,-8.11641593371033,
8.10019985312173));
#162435=CARTESIAN_POINT('Ctrl Pts',(0.573398458324473,-8.10660674880811,
8.10643363746578));
#162436=CARTESIAN_POINT('Ctrl Pts',(0.743539928098192,-8.09116296498737,
8.11299755615427));
#162437=CARTESIAN_POINT('Ctrl Pts',(0.752567202775413,-8.09032832189467,
8.1133458104373));
#162438=CARTESIAN_POINT('Ctrl Pts',(0.763852227499174,-8.08926588054208,
8.11378115986181));
#162439=CARTESIAN_POINT('Ctrl Pts',(0.766111302016934,-8.08905224265988,
8.11386830936705));
#162440=CARTESIAN_POINT('Ctrl Pts',(0.782018752425672,-8.0875411711376,
8.11448197868131));
#162441=CARTESIAN_POINT('Ctrl Pts',(0.795663919412676,-8.08621014144403,
8.11500837088762));
#162442=CARTESIAN_POINT('Ctrl Pts',(1.12918536632948,-8.05282412012167,
8.12787518608451));
#162443=CARTESIAN_POINT('Ctrl Pts',(1.44688185475672,-8.00184780213221,
8.14015402965942));
#162444=CARTESIAN_POINT('Ctrl Pts',(1.93827387127676,-7.89277266798919,
8.15955983397255));
#162445=CARTESIAN_POINT('Ctrl Pts',(2.1144522820973,-7.84741082013793,8.16660053198384));
#162446=CARTESIAN_POINT('Ctrl Pts',(2.35772781314247,-7.77598508202863,
8.17647147745223));
#162447=CARTESIAN_POINT('Ctrl Pts',(2.42622669512594,-7.75488545357596,
8.17926739528149));
#162448=CARTESIAN_POINT('Ctrl Pts',(2.54659238679437,-7.71605844868456,
8.18421098540876));
#162449=CARTESIAN_POINT('Ctrl Pts',(2.59857587805192,-7.69870730368207,
8.18635620305781));
#162450=CARTESIAN_POINT('Ctrl Pts',(2.71067135570806,-7.66002717155188,
8.19100455456611));
#162451=CARTESIAN_POINT('Ctrl Pts',(2.77071577958751,-7.6385135661183,8.19350858723749));
#162452=CARTESIAN_POINT('Ctrl Pts',(3.03093282318446,-7.54180716851412,
8.20442233573992));
#162453=CARTESIAN_POINT('Ctrl Pts',(3.22834592373732,-7.45943637626475,
8.21286489215665));
#162454=CARTESIAN_POINT('Ctrl Pts',(3.54045059601038,-7.31449747615005,
8.2264494520932));
#162455=CARTESIAN_POINT('Ctrl Pts',(3.65728570375875,-7.25678477187633,
8.23158986546695));
#162456=CARTESIAN_POINT('Ctrl Pts',(3.81195006038744,-7.17570136056437,
8.2384567579603));
#162457=CARTESIAN_POINT('Ctrl Pts',(3.85104839795112,-7.15479416422231,
8.24019807116571));
#162458=CARTESIAN_POINT('Ctrl Pts',(3.92888215815467,-7.11235098792857,
8.243674437032));
#162459=CARTESIAN_POINT('Ctrl Pts',(3.96761643292707,-7.09081599298028,
8.24540943304662));
#162460=CARTESIAN_POINT('Ctrl Pts',(4.10405026020627,-7.01349527370921,
8.2515414770699));
#162461=CARTESIAN_POINT('Ctrl Pts',(4.20076555097384,-6.95599837799962,
8.25592667111853));
#162462=CARTESIAN_POINT('Ctrl Pts',(4.42753395751192,-6.81473056543669,
8.26633276062376));
#162463=CARTESIAN_POINT('Ctrl Pts',(4.55645002556714,-6.72921784053184,
8.27234891134538));
#162464=CARTESIAN_POINT('Ctrl Pts',(4.74299424650599,-6.5976594491307,8.28124780044818));
#162465=CARTESIAN_POINT('Ctrl Pts',(4.80256263212642,-6.55442573802253,
8.28411960099532));
#162466=CARTESIAN_POINT('Ctrl Pts',(4.91349663191918,-6.47158743553914,
8.28952971157284));
#162467=CARTESIAN_POINT('Ctrl Pts',(4.96499146371565,-6.43216548429352,
8.29206687621601));
#162468=CARTESIAN_POINT('Ctrl Pts',(5.05903338116241,-6.35836927304515,
8.296751040562));
#162469=CARTESIAN_POINT('Ctrl Pts',(5.10171596297473,-6.32417368297417,
8.29889676889834));
#162470=CARTESIAN_POINT('Ctrl Pts',(5.19745840068094,-6.24586857462188,
8.3037565424415));
#162471=CARTESIAN_POINT('Ctrl Pts',(5.25030812133242,-6.20150890148645,
8.30647223130618));
#162472=CARTESIAN_POINT('Ctrl Pts',(5.42107177510248,-6.05442992635263,
8.31535998394037));
#162473=CARTESIAN_POINT('Ctrl Pts',(5.53658565480808,-5.94897970908474,
8.32155244944679));
#162474=CARTESIAN_POINT('Ctrl Pts',(5.70878421389509,-5.78242095659344,
8.33107799120264));
#162475=CARTESIAN_POINT('Ctrl Pts',(5.76769248563614,-5.723664266293,8.33439237140566));
#162476=CARTESIAN_POINT('Ctrl Pts',(6.0559574272559,-5.42717105058736,8.35089274022879));
#162477=CARTESIAN_POINT('Ctrl Pts',(6.2715688575507,-5.17650744042051,8.36415444487014));
#162478=CARTESIAN_POINT('Ctrl Pts',(6.52492715487124,-4.84281645342351,
8.38085641292913));
#162479=CARTESIAN_POINT('Ctrl Pts',(6.5773732338078,-4.77134227228956,8.38438142795461));
#162480=CARTESIAN_POINT('Ctrl Pts',(6.66361502264975,-4.64968600124284,
8.39028776082471));
#162481=CARTESIAN_POINT('Ctrl Pts',(6.69803878443076,-4.59995886886304,
8.39267637007353));
#162482=CARTESIAN_POINT('Ctrl Pts',(6.74680944483229,-4.5277984047061,8.39610391506119));
#162483=CARTESIAN_POINT('Ctrl Pts',(6.76160614123683,-4.50567181191829,
8.397149745348));
#162484=CARTESIAN_POINT('Ctrl Pts',(6.78729471156454,-4.46684626137138,
8.39897564398917));
#162485=CARTESIAN_POINT('Ctrl Pts',(6.79823433660271,-4.45017920227608,
8.39975651910052));
#162486=CARTESIAN_POINT('Ctrl Pts',(6.82102753639908,-4.41517244868763,
8.40139035447707));
#162487=CARTESIAN_POINT('Ctrl Pts',(6.83286870460551,-4.39682495375392,
8.40224305178656));
#162488=CARTESIAN_POINT('Ctrl Pts',(6.86781577781336,-4.34219349938828,
8.40477146175581));
#162489=CARTESIAN_POINT('Ctrl Pts',(6.89070769428885,-4.30577350163387,
8.40644334798275));
#162490=CARTESIAN_POINT('Ctrl Pts',(7.0112870914248,-4.11051258713604,8.41534049658046));
#162491=CARTESIAN_POINT('Ctrl Pts',(7.10377488535658,-3.9485243079388,8.42249021582988));
#162492=CARTESIAN_POINT('Ctrl Pts',(7.29946044159808,-3.57662010723258,
8.43857951931458));
#162493=CARTESIAN_POINT('Ctrl Pts',(7.3993338569666,-3.3651436925088,8.44750749987546));
#162494=CARTESIAN_POINT('Ctrl Pts',(7.51517549881037,-3.08966980570351,
8.45900823862386));
#162495=CARTESIAN_POINT('Ctrl Pts',(7.53967931607756,-3.02938245285457,
8.46151716705563));
#162496=CARTESIAN_POINT('Ctrl Pts',(7.59557544302184,-2.88697917594726,
8.46742875446918));
#162497=CARTESIAN_POINT('Ctrl Pts',(7.62636445055141,-2.80463548270725,
8.4708357836797));
#162498=CARTESIAN_POINT('Ctrl Pts',(7.67031490234861,-2.68101314961786,
8.47593878056291));
#162499=CARTESIAN_POINT('Ctrl Pts',(7.68449231014864,-2.64010229452998,
8.47762558520713));
#162500=CARTESIAN_POINT('Ctrl Pts',(7.70955205412459,-2.56587661997485,
8.48068298548938));
#162501=CARTESIAN_POINT('Ctrl Pts',(7.7205471384761,-2.53260095087661,8.48205254031005));
#162502=CARTESIAN_POINT('Ctrl Pts',(7.74389349668088,-2.46038010874637,
8.48502288731742));
#162503=CARTESIAN_POINT('Ctrl Pts',(7.75616699032932,-2.4214108220697,8.48662432381654));
#162504=CARTESIAN_POINT('Ctrl Pts',(7.7896006527893,-2.31239346806226,8.49110106700274));
#162505=CARTESIAN_POINT('Ctrl Pts',(7.81010919421641,-2.24214989816937,
8.49398182492996));
#162506=CARTESIAN_POINT('Ctrl Pts',(7.90802503056263,-1.88912242516791,
8.5084425888189));
#162507=CARTESIAN_POINT('Ctrl Pts',(7.97103478925703,-1.60257423112907,
8.52013667610983));
#162508=CARTESIAN_POINT('Ctrl Pts',(8.03709931868304,-1.19919940431071,
8.53643679629225));
#162509=CARTESIAN_POINT('Ctrl Pts',(8.05334343877357,-1.0847600246756,8.54104175269497));
#162510=CARTESIAN_POINT('Ctrl Pts',(8.0754214269259,-0.901147769265471,
8.54838203796153));
#162511=CARTESIAN_POINT('Ctrl Pts',(8.0828198330413,-0.832179165420568,
8.55112833007654));
#162512=CARTESIAN_POINT('Ctrl Pts',(8.0918512957371,-0.736443058255913,
8.55492142841022));
#162513=CARTESIAN_POINT('Ctrl Pts',(8.09423628599722,-0.709749761455962,
8.55597697178944));
#162514=CARTESIAN_POINT('Ctrl Pts',(8.09808970663029,-0.664073159925274,
8.55777935247312));
#162515=CARTESIAN_POINT('Ctrl Pts',(8.09962355278008,-0.645095624269162,
8.55852706959161));
#162516=CARTESIAN_POINT('Ctrl Pts',(8.10263537568373,-0.606126529499454,
8.56005999836525));
#162517=CARTESIAN_POINT('Ctrl Pts',(8.10410609618441,-0.586134613668799,
8.56084507042151));
#162518=CARTESIAN_POINT('Ctrl Pts',(8.10797637599208,-0.530723036553506,
8.5630173824105));
#162519=CARTESIAN_POINT('Ctrl Pts',(8.11021781218605,-0.495292754225757,
8.56440225631748));
#162520=CARTESIAN_POINT('Ctrl Pts',(8.1209324651045,-0.306274760923921,
8.5717709197774));
#162521=CARTESIAN_POINT('Ctrl Pts',(8.12527528680076,-0.152482634129329,
8.57769777076142));
#162522=CARTESIAN_POINT('Ctrl Pts',(8.125182719626,0.408164825321524,8.59918056248831));
#162523=CARTESIAN_POINT('Ctrl Pts',(8.09456184005172,0.814411360073113,
8.61452497607626));
#162524=CARTESIAN_POINT('Ctrl Pts',(8.01329831772904,1.35099982553224,8.6351925936212));
#162525=CARTESIAN_POINT('Ctrl Pts',(7.98958556626881,1.4848139978795,8.64037875206134));
#162526=CARTESIAN_POINT('Ctrl Pts',(7.91719876941115,1.84105174360256,8.65430843227127));
#162527=CARTESIAN_POINT('Ctrl Pts',(7.86251460153513,2.06212749641007,8.66308426533485));
#162528=CARTESIAN_POINT('Ctrl Pts',(7.77992147013455,2.34455711414634,8.6745246926588));
#162529=CARTESIAN_POINT('Ctrl Pts',(7.76043598271661,2.40826897182255,8.67712067203412));
#162530=CARTESIAN_POINT('Ctrl Pts',(7.72766479468173,2.51089108503831,8.68132786711606));
#162531=CARTESIAN_POINT('Ctrl Pts',(7.71486341604042,2.54995287755799,8.68293537427143));
#162532=CARTESIAN_POINT('Ctrl Pts',(7.68968758118228,2.62484847548354,8.68602953626025));
#162533=CARTESIAN_POINT('Ctrl Pts',(7.67735765786065,2.66069614914523,8.6875158289862));
#162534=CARTESIAN_POINT('Ctrl Pts',(7.64810768996246,2.74384027551099,8.69097567914695));
#162535=CARTESIAN_POINT('Ctrl Pts',(7.6309990348167,2.79106868453185,8.69295050739298));
#162536=CARTESIAN_POINT('Ctrl Pts',(7.57333148275497,2.94576505567647,8.69945091666786));
#162537=CARTESIAN_POINT('Ctrl Pts',(7.53093177068594,3.05253139720528,8.70398826968992));
#162538=CARTESIAN_POINT('Ctrl Pts',(7.24063133272663,3.74063206243468,8.73356875176072));
#162539=CARTESIAN_POINT('Ctrl Pts',(6.9279019071613,4.29222491871825,8.7589090755481));
#162540=CARTESIAN_POINT('Ctrl Pts',(6.30402989153378,5.14377470095022,8.80307618079208));
#162541=CARTESIAN_POINT('Ctrl Pts',(6.0272806678017,5.46544475055119,8.82116457929401));
#162542=CARTESIAN_POINT('Ctrl Pts',(5.54484101561906,5.94475867454676,8.84969961406211));
#162543=CARTESIAN_POINT('Ctrl Pts',(5.35450696844494,6.11675429558451,8.86031290433557));
#162544=CARTESIAN_POINT('Ctrl Pts',(5.14095158526736,6.29211423259743,8.87130511686792));
#162545=CARTESIAN_POINT('Ctrl Pts',(5.12550340556368,6.30470455818851,8.87209529929975));
#162546=CARTESIAN_POINT('Ctrl Pts',(5.10250147071666,6.32331080571663,8.87326430691714));
#162547=CARTESIAN_POINT('Ctrl Pts',(5.0949831202747,6.32937025378214,8.87364521461099));
#162548=CARTESIAN_POINT('Ctrl Pts',(5.08208854913336,6.33972482781171,8.87429643918843));
#162549=CARTESIAN_POINT('Ctrl Pts',(5.07671764987614,6.344026546085,8.87456707919515));
#162550=CARTESIAN_POINT('Ctrl Pts',(5.06568701150684,6.35283834495498,8.87512165091374));
#162551=CARTESIAN_POINT('Ctrl Pts',(5.06002669774812,6.35734769807042,8.87540554630125));
#162552=CARTESIAN_POINT('Ctrl Pts',(5.04694262300288,6.36774273001224,8.87606019979413));
#162553=CARTESIAN_POINT('Ctrl Pts',(5.03951456873107,6.37362300642583,8.87643068373376));
#162554=CARTESIAN_POINT('Ctrl Pts',(5.01621366716805,6.39200251754911,8.87758912836506));
#162555=CARTESIAN_POINT('Ctrl Pts',(5.00030439788749,6.40445561132186,8.87837469463885));
#162556=CARTESIAN_POINT('Ctrl Pts',(4.71661439390168,6.62481452093798,8.89228460660483));
#162557=CARTESIAN_POINT('Ctrl Pts',(4.43612901921814,6.81581818506839,8.90437727330124));
#162558=CARTESIAN_POINT('Ctrl Pts',(3.9577308585481,7.09952262867376,8.92349279391847));
#162559=CARTESIAN_POINT('Ctrl Pts',(3.76655789947534,7.20277030241508,8.93077367961808));
#162560=CARTESIAN_POINT('Ctrl Pts',(3.32598231856728,7.41837101108538,8.94714853350188));
#162561=CARTESIAN_POINT('Ctrl Pts',(3.07458504197616,7.52604224706054,8.95621727660027));
#162562=CARTESIAN_POINT('Ctrl Pts',(2.32875672476372,7.80185513908871,8.98317481311338));
#162563=CARTESIAN_POINT('Ctrl Pts',(1.82302384374018,7.93527320198415,9.00159640601862));
#162564=CARTESIAN_POINT('Ctrl Pts',(1.27586993043952,8.02451894916715,9.02290721311776));
#162565=CARTESIAN_POINT('Ctrl Pts',(1.2436925431829,8.02956893449013,9.0241650507121));
#162566=CARTESIAN_POINT('Ctrl Pts',(1.19896070351345,8.0363139088088,9.02592017373139));
#162567=CARTESIAN_POINT('Ctrl Pts',(1.18643116178892,8.03817324434369,9.02641249913906));
#162568=CARTESIAN_POINT('Ctrl Pts',(1.16485239355959,8.04132389716677,9.02726162938249));
#162569=CARTESIAN_POINT('Ctrl Pts',(1.15580522569965,8.04262925898584,9.02761801037268));
#162570=CARTESIAN_POINT('Ctrl Pts',(1.13713608099941,8.04529076648824,9.02835418797354));
#162571=CARTESIAN_POINT('Ctrl Pts',(1.12751383727057,8.04664492382057,9.02873404383304));
#162572=CARTESIAN_POINT('Ctrl Pts',(1.10512450230696,8.04975487069735,9.02961889481034));
#162573=CARTESIAN_POINT('Ctrl Pts',(1.09235563325358,8.05149755092593,9.0301242833098));
#162574=CARTESIAN_POINT('Ctrl Pts',(1.05170670195827,8.05694679218192,9.03173555755846));
#162575=CARTESIAN_POINT('Ctrl Pts',(1.02381165509941,8.06053895683023,9.032844875136));
#162576=CARTESIAN_POINT('Ctrl Pts',(0.48231095226244,8.12741405139886,9.05444963470158));
#162577=CARTESIAN_POINT('Ctrl Pts',(-0.0360949400586856,8.14162538617692,
9.07646773667047));
#162578=CARTESIAN_POINT('Ctrl Pts',(-1.32616395195673,8.05373575201676,
9.13370019919003));
#162579=CARTESIAN_POINT('Ctrl Pts',(-2.08855332663799,7.89046719957832,
9.16985986382854));
#162580=CARTESIAN_POINT('Ctrl Pts',(-2.85440477111827,7.60747762210895,
9.20281494154776));
#162581=CARTESIAN_POINT('Ctrl Pts',(-2.89245649901079,7.59309145573709,
9.20444316449478));
#162582=CARTESIAN_POINT('Ctrl Pts',(-2.94287120840034,7.57359725797457,
9.20658994141164));
#162583=CARTESIAN_POINT('Ctrl Pts',(-2.95533147876041,7.56874376820314,
9.20711967626199));
#162584=CARTESIAN_POINT('Ctrl Pts',(-2.97470799783421,7.56114113611318,
9.20794219173996));
#162585=CARTESIAN_POINT('Ctrl Pts',(-2.98163251263289,7.55841322717335,
9.20823588082018));
#162586=CARTESIAN_POINT('Ctrl Pts',(-2.99552710024956,7.55291739641583,
9.2088247046404));
#162587=CARTESIAN_POINT('Ctrl Pts',(-3.0024971079398,7.55014933115094,9.2091198328891));
#162588=CARTESIAN_POINT('Ctrl Pts',(-3.01810397376515,7.54392619916122,
9.20978013448992));
#162589=CARTESIAN_POINT('Ctrl Pts',(-3.0267387593589,7.54046593907381,9.2101450918043));
#162590=CARTESIAN_POINT('Ctrl Pts',(-3.05215445956522,7.530230290043,9.21121827508495));
#162591=CARTESIAN_POINT('Ctrl Pts',(-3.06891876179363,7.52341363384642,
9.21192482032293));
#162592=CARTESIAN_POINT('Ctrl Pts',(-3.19928010648258,7.46989821802504,
9.21740951179803));
#162593=CARTESIAN_POINT('Ctrl Pts',(-3.31183101789318,7.4206838984056,9.22208881726159));
#162594=CARTESIAN_POINT('Ctrl Pts',(-3.72771333181943,7.2274865252283,9.23929557784815));
#162595=CARTESIAN_POINT('Ctrl Pts',(-4.02315264457134,7.06729559820798,
9.25136337991569));
#162596=CARTESIAN_POINT('Ctrl Pts',(-4.84462103407879,6.55363455182756,
9.2861515482775));
#162597=CARTESIAN_POINT('Ctrl Pts',(-5.34030882697556,6.15642318869333,
9.30890778908585));
#162598=CARTESIAN_POINT('Ctrl Pts',(-5.84624108327607,5.64347368663516,
9.33644066665696));
#162599=CARTESIAN_POINT('Ctrl Pts',(-5.9066210350818,5.58024710267164,9.33980240538738));
#162600=CARTESIAN_POINT('Ctrl Pts',(-5.98906341417004,5.49108043051823,
9.34450029453073));
#162601=CARTESIAN_POINT('Ctrl Pts',(-6.01200119246856,5.46595705431438,
9.34581932250214));
#162602=CARTESIAN_POINT('Ctrl Pts',(-6.04866028798457,5.42529501067237,
9.34794671475477));
#162603=CARTESIAN_POINT('Ctrl Pts',(-6.06248114301694,5.40984654305795,
9.34875325234681));
#162604=CARTESIAN_POINT('Ctrl Pts',(-6.09077359222066,5.37797765523366,
9.35041355318815));
#162605=CARTESIAN_POINT('Ctrl Pts',(-6.10523826906305,5.36155129479687,
9.35126741735504));
#162606=CARTESIAN_POINT('Ctrl Pts',(-6.13757949360315,5.32452340645861,
9.35318802353218));
#162607=CARTESIAN_POINT('Ctrl Pts',(-6.1554190126457,5.30388992316072,9.35425541150572));
#162608=CARTESIAN_POINT('Ctrl Pts',(-6.20822369417321,5.24218991622258,
9.35743914425395));
#162609=CARTESIAN_POINT('Ctrl Pts',(-6.24288405600679,5.20086484658591,
9.35956099384458));
#162610=CARTESIAN_POINT('Ctrl Pts',(-6.65761041079696,4.69627259410928,
9.3853540921076));
#162611=CARTESIAN_POINT('Ctrl Pts',(-6.98568565628412,4.19271383247046,
9.41012990363884));
#162612=CARTESIAN_POINT('Ctrl Pts',(-7.33118660057727,3.50738292618752,
9.44263593248867));
#162613=CARTESIAN_POINT('Ctrl Pts',(-7.40228494005331,3.35472942106161,
9.44979119382671));
#162614=CARTESIAN_POINT('Ctrl Pts',(-7.61299214213051,2.86294930949839,
9.47246190222982));
#162615=CARTESIAN_POINT('Ctrl Pts',(-7.73442249284311,2.51651720664905,
9.48789027845702));
#162616=CARTESIAN_POINT('Ctrl Pts',(-7.83824832364922,2.14058273843573,
9.50344609326389));
#162617=CARTESIAN_POINT('Ctrl Pts',(-7.84435889627673,2.11808044292194,
9.50437270577527));
#162618=CARTESIAN_POINT('Ctrl Pts',(-7.85276810773991,2.08657779247594,
9.50566337810948));
#162619=CARTESIAN_POINT('Ctrl Pts',(-7.85514827453566,2.07759943778976,
9.50603047996719));
#162620=CARTESIAN_POINT('Ctrl Pts',(-7.85946989663317,2.06118402496943,
9.50670028345169));
#162621=CARTESIAN_POINT('Ctrl Pts',(-7.86141620305199,2.05374826202169,
9.50700317026875));
#162622=CARTESIAN_POINT('Ctrl Pts',(-7.86532383065232,2.03873242612407,
9.50761376504513));
#162623=CARTESIAN_POINT('Ctrl Pts',(-7.86728475257214,2.03115225643798,
9.5079214572226));
#162624=CARTESIAN_POINT('Ctrl Pts',(-7.87205877013605,2.01258710735715,
9.50867370150504));
#162625=CARTESIAN_POINT('Ctrl Pts',(-7.87485983766816,2.0015990317497,9.50911777541884));
#162626=CARTESIAN_POINT('Ctrl Pts',(-7.88485054513738,1.96206171915785,
9.51071141632596));
#162627=CARTESIAN_POINT('Ctrl Pts',(-7.89190806413483,1.93347910414778,
9.5118555859956));
#162628=CARTESIAN_POINT('Ctrl Pts',(-7.93008327903596,1.77517927702798,
9.5181464593863));
#162629=CARTESIAN_POINT('Ctrl Pts',(-7.95815733801256,1.64475346712227,
9.52314819155498));
#162630=CARTESIAN_POINT('Ctrl Pts',(-7.99856259789834,1.43166158392886,
9.53108050670572));
#162631=CARTESIAN_POINT('Ctrl Pts',(-8.01285176661908,1.34939453128148,
9.53408679184817));
#162632=CARTESIAN_POINT('Ctrl Pts',(-8.10241914036645,0.78199017682363,
9.55451076146514));
#162633=CARTESIAN_POINT('Ctrl Pts',(-8.13486373541702,0.291100010976691,
9.57066610291255));
#162634=CARTESIAN_POINT('Ctrl Pts',(-8.10837268012976,-0.786262068619116,
9.60708870836392));
#162635=CARTESIAN_POINT('Ctrl Pts',(-8.03047078835915,-1.36944161749787,
9.62751658244886));
#162636=CARTESIAN_POINT('Ctrl Pts',(-7.88168299525032,-1.97487099089194,
9.65144491329839));
#162637=CARTESIAN_POINT('Ctrl Pts',(-7.87265630206983,-2.01055340043818,
9.65286487400218));
#162638=CARTESIAN_POINT('Ctrl Pts',(-7.86002757618888,-2.05908525329603,
9.65480966336704));
#162639=CARTESIAN_POINT('Ctrl Pts',(-7.85663581582393,-2.07198919743552,
9.65532805910014));
#162640=CARTESIAN_POINT('Ctrl Pts',(-7.85081990499647,-2.09389620389514,
9.65621036854512));
#162641=CARTESIAN_POINT('Ctrl Pts',(-7.84841200861653,-2.10290357260312,
9.65657378365717));
#162642=CARTESIAN_POINT('Ctrl Pts',(-7.84373325546249,-2.12028570552623,
9.65727633463989));
#162643=CARTESIAN_POINT('Ctrl Pts',(-7.84146447564054,-2.12866101872184,
9.65761540639882));
#162644=CARTESIAN_POINT('Ctrl Pts',(-7.8360621465402,-2.14847814330986,
9.65841902335726));
#162645=CARTESIAN_POINT('Ctrl Pts',(-7.8329169505939,-2.15991674385787,
9.658883925919));
#162646=CARTESIAN_POINT('Ctrl Pts',(-7.82361092763713,-2.19347368165725,
9.66025088530729));
#162647=CARTESIAN_POINT('Ctrl Pts',(-7.81738140832054,-2.21557275790414,
9.66115505425801));
#162648=CARTESIAN_POINT('Ctrl Pts',(-7.76978174448922,-2.38173126239937,
9.6679833466699));
#162649=CARTESIAN_POINT('Ctrl Pts',(-7.72452776439988,-2.52464255814885,
9.67402720316051));
#162650=CARTESIAN_POINT('Ctrl Pts',(-7.55909379323849,-3.00088429411161,
9.69476095408454));
#162651=CARTESIAN_POINT('Ctrl Pts',(-7.42108433541074,-3.32756334259877,
9.70999610653406));
#162652=CARTESIAN_POINT('Ctrl Pts',(-7.0424348097251,-4.08214664848373,
9.74732285693284));
#162653=CARTESIAN_POINT('Ctrl Pts',(-6.78349995443966,-4.49932380980036,
9.76975394677767));
#162654=CARTESIAN_POINT('Ctrl Pts',(-6.26862024336325,-5.18243370737129,
9.80777817620634));
#162655=CARTESIAN_POINT('Ctrl Pts',(-6.02920071011497,-5.45912507791164,
9.82358536800317));
#162656=CARTESIAN_POINT('Ctrl Pts',(-5.75455485135851,-5.73632241861889,
9.83917321402805));
#162657=CARTESIAN_POINT('Ctrl Pts',(-5.73710781529798,-5.75377183790873,
9.84015380791609));
#162658=CARTESIAN_POINT('Ctrl Pts',(-5.71282150511364,-5.77784117065954,
9.8415059651135));
#162659=CARTESIAN_POINT('Ctrl Pts',(-5.70604979967101,-5.78452883365565,
9.84188161316139));
#162660=CARTESIAN_POINT('Ctrl Pts',(-5.69438876068727,-5.79600474782677,
9.84252616691749));
#162661=CARTESIAN_POINT('Ctrl Pts',(-5.68950510908996,-5.80079873885671,
9.84279540958758));
#162662=CARTESIAN_POINT('Ctrl Pts',(-5.6794335687255,-5.81066041825461,
9.84334924853374));
#162663=CARTESIAN_POINT('Ctrl Pts',(-5.67424493946721,-5.81572734274852,
9.8436338008379));
#162664=CARTESIAN_POINT('Ctrl Pts',(-5.6621888395409,-5.82746916111994,
9.84429320334781));
#162665=CARTESIAN_POINT('Ctrl Pts',(-5.65531632918775,-5.83413888215379,
9.84466776187203));
#162666=CARTESIAN_POINT('Ctrl Pts',(-5.63381755770509,-5.85492959969573,
9.84583537805118));
#162667=CARTESIAN_POINT('Ctrl Pts',(-5.6191500153604,-5.86900792340847,
9.84662609561483));
#162668=CARTESIAN_POINT('Ctrl Pts',(-5.47792635059363,-6.00354368998127,
9.8541847864595));
#162669=CARTESIAN_POINT('Ctrl Pts',(-5.34756372359454,-6.11994939718079,
9.8607446446613));
#162670=CARTESIAN_POINT('Ctrl Pts',(-5.06320898874539,-6.35783143124494,
9.87441729713133));
#162671=CARTESIAN_POINT('Ctrl Pts',(-4.90836798574893,-6.47811951448859,
9.88149629424793));
#162672=CARTESIAN_POINT('Ctrl Pts',(-4.503555850863,-6.7697431564852,9.8994161294254));
#162673=CARTESIAN_POINT('Ctrl Pts',(-4.24807861511865,-6.93291179475225,
9.91019819615098));
#162674=CARTESIAN_POINT('Ctrl Pts',(-3.43354064838567,-7.39117918649344,
9.94400062722491));
#162675=CARTESIAN_POINT('Ctrl Pts',(-2.84878029242084,-7.63564635039871,
9.96770957252968));
#162676=CARTESIAN_POINT('Ctrl Pts',(-2.12767790626376,-7.84262312616943,
9.99667905926199));
#162677=CARTESIAN_POINT('Ctrl Pts',(-2.01299010490966,-7.87284073630419,
10.0012752615384));
#162678=CARTESIAN_POINT('Ctrl Pts',(-1.85187288485123,-7.91154055837685,
10.0077272668261));
#162679=CARTESIAN_POINT('Ctrl Pts',(-1.8059682307994,-7.9221452847949,10.0095649703947));
#162680=CARTESIAN_POINT('Ctrl Pts',(-1.72237421614428,-7.9406925369856,
10.0129112107143));
#162681=CARTESIAN_POINT('Ctrl Pts',(-1.68471560644113,-7.94876746539863,
10.0144185674137));
#162682=CARTESIAN_POINT('Ctrl Pts',(-1.61263541033176,-7.96368797734493,
10.0173039002247));
#162683=CARTESIAN_POINT('Ctrl Pts',(-1.5782240700626,-7.97057889623961,
10.0186814493681));
#162684=CARTESIAN_POINT('Ctrl Pts',(-1.49382579057793,-7.9869117832368,
10.0220606065234));
#162685=CARTESIAN_POINT('Ctrl Pts',(-1.44379283484209,-7.99610764953757,
10.0240643017052));
#162686=CARTESIAN_POINT('Ctrl Pts',(-1.26794720997423,-8.02672315391913,
10.0311094126743));
#162687=CARTESIAN_POINT('Ctrl Pts',(-1.14172019073502,-8.04564784278232,
10.036172023216));
#162688=CARTESIAN_POINT('Ctrl Pts',(-0.831905031029516,-8.08465920321975,
10.0486211603613));
#162689=CARTESIAN_POINT('Ctrl Pts',(-0.647977991701629,-8.10147539601015,
10.0560321969358));
#162690=CARTESIAN_POINT('Ctrl Pts',(-0.179355597340776,-8.12825939199799,
10.0749737423686));
#162691=CARTESIAN_POINT('Ctrl Pts',(0.105584676168758,-8.12955219632266,
10.0865490769958));
#162692=CARTESIAN_POINT('Ctrl Pts',(0.495020917070936,-8.11083821153645,
10.1023925010561));
#162693=CARTESIAN_POINT('Ctrl Pts',(0.599933168815925,-8.1037536052002,
10.1066623410405));
#162694=CARTESIAN_POINT('Ctrl Pts',(0.865215571781854,-8.08065944319061,
10.1174530550649));
#162695=CARTESIAN_POINT('Ctrl Pts',(1.02530286659011,-8.06191106427882,
10.1239594023143));
#162696=CARTESIAN_POINT('Ctrl Pts',(1.28238060144516,-8.0240221059192,10.1343683114038));
#162697=CARTESIAN_POINT('Ctrl Pts',(1.37976393642195,-8.00785131075567,
10.138301999353));
#162698=CARTESIAN_POINT('Ctrl Pts',(1.5072753911121,-7.9842825032573,10.1434336478598));
#162699=CARTESIAN_POINT('Ctrl Pts',(1.53768918019316,-7.97848094536262,
10.1446562050728));
#162700=CARTESIAN_POINT('Ctrl Pts',(1.58505001863631,-7.96916579729514,
10.1465574892036));
#162701=CARTESIAN_POINT('Ctrl Pts',(1.6020201298794,-7.9657716871767,10.1472382321943));
#162702=CARTESIAN_POINT('Ctrl Pts',(1.63425463311115,-7.95921744504413,
10.1485303651622));
#162703=CARTESIAN_POINT('Ctrl Pts',(1.64952096862422,-7.9560675662774,10.1491419362434));
#162704=CARTESIAN_POINT('Ctrl Pts',(1.66482904541191,-7.95286312058463,
10.1497548497821));
#162705=CARTESIAN_POINT('Ctrl Pts',(1.66487991835834,-7.95285247082126,
10.1497568866586));
#162706=CARTESIAN_POINT('Ctrl Pts',(1.66498154272579,-7.95283119571714,
10.1497609555386));
#162707=CARTESIAN_POINT('Ctrl Pts',(1.6650323007612,-7.95282056899382,10.1497629878069));
#162708=CARTESIAN_POINT('Ctrl Pts',(1.66513370577417,-7.95279933778493,
10.1497670478897));
#162709=CARTESIAN_POINT('Ctrl Pts',(1.66518435252817,-7.95278873334837,
10.1497690756953));
#162710=CARTESIAN_POINT('Ctrl Pts',(1.66528553548582,-7.95276754661342,
10.149773126873));
#162711=CARTESIAN_POINT('Ctrl Pts',(1.66533607193129,-7.95275696426656,
10.1497751502548));
#162712=CARTESIAN_POINT('Ctrl Pts',(1.665437035628,-7.95273582143359,10.1497791926392));
#162713=CARTESIAN_POINT('Ctrl Pts',(1.66548746296985,-7.95272526093066,
10.1497812116456));
#162714=CARTESIAN_POINT('Ctrl Pts',(1.66558820962998,-7.95270416154685,
10.149785245326));
#162715=CARTESIAN_POINT('Ctrl Pts',(1.66563852899509,-7.95269362265831,
10.149787260002));
#162716=CARTESIAN_POINT('Ctrl Pts',(1.66573906108083,-7.95267256622083,
10.1497912850771));
#162717=CARTESIAN_POINT('Ctrl Pts',(1.6657892737062,-7.95266204869396,10.1497932954724));
#162718=CARTESIAN_POINT('Ctrl Pts',(1.66588959330177,-7.95264103477893,
10.1497973120257));
#162719=CARTESIAN_POINT('Ctrl Pts',(1.66593970029281,-7.95263053838849,
10.1497993181845));
#162720=CARTESIAN_POINT('Ctrl Pts',(1.66603980961057,-7.95260956654498,
10.1498033263047));
#162721=CARTESIAN_POINT('Ctrl Pts',(1.66608981196689,-7.95259909108778,
10.1498053282672));
#162722=CARTESIAN_POINT('Ctrl Pts',(1.66618971384362,-7.95257816073385,
10.1498093280679));
#162723=CARTESIAN_POINT('Ctrl Pts',(1.66623961300413,-7.95256770591455,
10.1498113258917));
#162724=CARTESIAN_POINT('Ctrl Pts',(1.66633930880072,-7.95254681677726,
10.1498153174276));
#162725=CARTESIAN_POINT('Ctrl Pts',(1.66638910563149,-7.95253638242047,
10.1498173111474));
#162726=CARTESIAN_POINT('Ctrl Pts',(1.6664885980956,-7.95251553393613,10.1498212945285));
#162727=CARTESIAN_POINT('Ctrl Pts',(1.66653829373343,-7.95250511980962,
10.1498232841899));
#162728=CARTESIAN_POINT('Ctrl Pts',(1.66663758511132,-7.95248431151939,
10.1498272595062));
#162729=CARTESIAN_POINT('Ctrl Pts',(1.6666871807584,-7.95247391737712,10.1498292451574));
#162730=CARTESIAN_POINT('Ctrl Pts',(1.66678627291365,-7.95245314890218,
10.1498332124837));
#162731=CARTESIAN_POINT('Ctrl Pts',(1.66683576954283,-7.95244277454608,
10.1498351941636));
#162732=CARTESIAN_POINT('Ctrl Pts',(1.66693466489529,-7.95242204539082,
10.1498391535969));
#162733=CARTESIAN_POINT('Ctrl Pts',(1.66698406360673,-7.95241169059605,
10.1498411313497));
#162734=CARTESIAN_POINT('Ctrl Pts',(1.66708276439456,-7.95239100030275,
10.1498450829795));
#162735=CARTESIAN_POINT('Ctrl Pts',(1.66713206638249,-7.95238066482464,
10.149847056853));
#162736=CARTESIAN_POINT('Ctrl Pts',(1.66723057429436,-7.95236001305058,
10.1498510007472));
#162737=CARTESIAN_POINT('Ctrl Pts',(1.66727978041752,-7.95234969671471,
10.1498529707758));
#162738=CARTESIAN_POINT('Ctrl Pts',(1.66737809812419,-7.9523290829111,10.1498569070413));
#162739=CARTESIAN_POINT('Ctrl Pts',(1.66742720957816,-7.95231878547235,
10.149858873273));
#162740=CARTESIAN_POINT('Ctrl Pts',(1.66752533900274,-7.95229820924695,
10.149862801987));
#162741=CARTESIAN_POINT('Ctrl Pts',(1.66757435693084,-7.95228793047102,
10.1498647644675));
#162742=CARTESIAN_POINT('Ctrl Pts',(1.66767229972826,-7.95226739148766,
10.1498686856962));
#162743=CARTESIAN_POINT('Ctrl Pts',(1.66772122492586,-7.95225713121317,
10.1498706444575));
#162744=CARTESIAN_POINT('Ctrl Pts',(1.66781898376004,-7.95223662892392,
10.1498745583077));
#162745=CARTESIAN_POINT('Ctrl Pts',(1.66786781735956,-7.95222638691869,
10.1498765133951));
#162746=CARTESIAN_POINT('Ctrl Pts',(1.66796539419119,-7.95220592092289,
10.1498804199454));
#162747=CARTESIAN_POINT('Ctrl Pts',(1.66801413731788,-7.95219569695616,
10.149882371404));
#162748=CARTESIAN_POINT('Ctrl Pts',(1.66811153371643,-7.95217526693505,
10.1498862707173));
#162749=CARTESIAN_POINT('Ctrl Pts',(1.66816018711285,-7.95216506085626,
10.1498882185769));
#162750=CARTESIAN_POINT('Ctrl Pts',(1.66825740605545,-7.95214466619563,
10.1498921107724));
#162751=CARTESIAN_POINT('Ctrl Pts',(1.66830597113018,-7.95213447771438,
10.1498940550894));
#162752=CARTESIAN_POINT('Ctrl Pts',(1.66840301361363,-7.95211411821526,
10.1498979402072));
#162753=CARTESIAN_POINT('Ctrl Pts',(1.66845149114522,-7.95210394717328,
10.1498998810129));
#162754=CARTESIAN_POINT('Ctrl Pts',(1.6685483596427,-7.95208362232682,10.149903759152));
#162755=CARTESIAN_POINT('Ctrl Pts',(1.66859675065309,-7.95207346851466,
10.1499056964872));
#162756=CARTESIAN_POINT('Ctrl Pts',(1.66869344705058,-7.95205317793503,
10.1499095677233));
#162757=CARTESIAN_POINT('Ctrl Pts',(1.66874175247925,-7.95204304116047,
10.1499115016258));
#162758=CARTESIAN_POINT('Ctrl Pts',(1.66883827893448,-7.95202278440465,
10.1499153660452));
#162759=CARTESIAN_POINT('Ctrl Pts',(1.66888649985005,-7.95201266444829,
10.1499172965577));
#162760=CARTESIAN_POINT('Ctrl Pts',(1.66898285814562,-7.9519924411518,10.149921154232));
#162761=CARTESIAN_POINT('Ctrl Pts',(1.66903099552138,-7.95198233781415,
10.1499230813935));
#162762=CARTESIAN_POINT('Ctrl Pts',(1.6691271875952,-7.95196214757977,10.1499269324003));
#162763=CARTESIAN_POINT('Ctrl Pts',(1.66917524238861,-7.95195206066459,
10.1499288562493));
#162764=CARTESIAN_POINT('Ctrl Pts',(1.66927127014065,-7.95193190310291,
10.1499327006647));
#162765=CARTESIAN_POINT('Ctrl Pts',(1.66931924326078,-7.95192183242404,
10.1499346212375));
#162766=CARTESIAN_POINT('Ctrl Pts',(1.66941510872256,-7.95190170711784,
10.1499384591429));
#162767=CARTESIAN_POINT('Ctrl Pts',(1.66946300113413,-7.95189165247735,
10.1499403764783));
#162768=CARTESIAN_POINT('Ctrl Pts',(1.66955870621739,-7.95187155903442,
10.1499442079503));
#162769=CARTESIAN_POINT('Ctrl Pts',(1.66960651889522,-7.95186152023219,
10.1499461220872));
#162770=CARTESIAN_POINT('Ctrl Pts',(1.66970206540729,-7.95184145828207,
10.1499499471983));
#162771=CARTESIAN_POINT('Ctrl Pts',(1.66974979926172,-7.95183143513143,
10.1499518581733));
#162772=CARTESIAN_POINT('Ctrl Pts',(1.66984518921076,-7.95181140426135,
10.1499556770039));
#162773=CARTESIAN_POINT('Ctrl Pts',(1.66989284524425,-7.95180139655621,
10.1499575848571));
#162774=CARTESIAN_POINT('Ctrl Pts',(1.66998808035551,-7.95178139641264,
10.1499613974764));
#162775=CARTESIAN_POINT('Ctrl Pts',(1.67003565949024,-7.95177140396368,
10.1499633022447));
#162776=CARTESIAN_POINT('Ctrl Pts',(1.67013074144333,-7.95175143420253,
10.14996710872));
#162777=CARTESIAN_POINT('Ctrl Pts',(1.67017824441422,-7.95174145685972,
10.1499690104329));
#162778=CARTESIAN_POINT('Ctrl Pts',(1.67027317558942,-7.95172151698958,
10.1499728108595));
#162779=CARTESIAN_POINT('Ctrl Pts',(1.67032060347758,-7.95171155453007,
10.1499747095604));
#162780=CARTESIAN_POINT('Ctrl Pts',(1.67041538549919,-7.95169164421816,
10.1499785040034));
#162781=CARTESIAN_POINT('Ctrl Pts',(1.67046273933832,-7.95168169642898,
10.1499803997337));
#162782=CARTESIAN_POINT('Ctrl Pts',(1.67055737356861,-7.95166181539744,
10.1499841882477));
#162783=CARTESIAN_POINT('Ctrl Pts',(1.67060465405356,-7.95165188213674,
10.1499860810352));
#162784=CARTESIAN_POINT('Ctrl Pts',(1.67069914295218,-7.951632029877,10.1499898637188));
#162785=CARTESIAN_POINT('Ctrl Pts',(1.67074635121749,-7.95162211091048,
10.1499917536089));
#162786=CARTESIAN_POINT('Ctrl Pts',(1.67084069584218,-7.95160228720838,
10.1499955305044));
#162787=CARTESIAN_POINT('Ctrl Pts',(1.67088783251507,-7.95159238240826,
10.1499974175224));
#162788=CARTESIAN_POINT('Ctrl Pts',(1.67098203531661,-7.9515725867568,10.150001188728));
#162789=CARTESIAN_POINT('Ctrl Pts',(1.67102910142358,-7.95156269591132,
10.1500030729149));
#162790=CARTESIAN_POINT('Ctrl Pts',(1.67112316386047,-7.95154292801185,
10.1500068384891));
#162791=CARTESIAN_POINT('Ctrl Pts',(1.67117016024723,-7.95153305094719,
10.1500087198788));
#162792=CARTESIAN_POINT('Ctrl Pts',(1.67126408417501,-7.95151331041747,
10.150012479896));
#162793=CARTESIAN_POINT('Ctrl Pts',(1.67131101174322,-7.95150344694796,
10.1500143585246));
#162794=CARTESIAN_POINT('Ctrl Pts',(1.6714047987701,-7.95148373345762,10.1500181130491));
#162795=CARTESIAN_POINT('Ctrl Pts',(1.67145165830128,-7.95147388342279,
10.1500199889479));
#162796=CARTESIAN_POINT('Ctrl Pts',(1.6715453104418,-7.95145419655589,10.1500237380606));
#162797=CARTESIAN_POINT('Ctrl Pts',(1.67159210289913,-7.95144435975701,
10.1500256112682));
#162798=CARTESIAN_POINT('Ctrl Pts',(1.67168562172243,-7.9514246991911,10.1500293550318));
#162799=CARTESIAN_POINT('Ctrl Pts',(1.6717323480043,-7.95141487544298,10.1500312255843));
#162800=CARTESIAN_POINT('Ctrl Pts',(1.67182573506276,-7.95139524085901,
10.150034964061));
#162801=CARTESIAN_POINT('Ctrl Pts',(1.67187239593607,-7.95138543000404,
10.1500368319891));
#162802=CARTESIAN_POINT('Ctrl Pts',(1.67196565308732,-7.95136582101864,
10.1500405652534));
#162803=CARTESIAN_POINT('Ctrl Pts',(1.67201224938012,-7.95135602288629,
10.1500424305902));
#162804=CARTESIAN_POINT('Ctrl Pts',(1.67210537853235,-7.95133643910533,
10.1500461587185));
#162805=CARTESIAN_POINT('Ctrl Pts',(1.67215191125789,-7.95132665348604,
10.1500480215047));
#162806=CARTESIAN_POINT('Ctrl Pts',(1.67224491351611,-7.95130709468415,
10.1500517445413));
#162807=CARTESIAN_POINT('Ctrl Pts',(1.67229138327103,-7.95129732145594,
10.1500536048007));
#162808=CARTESIAN_POINT('Ctrl Pts',(1.69057088484334,-7.94745272368089,
10.1507853616201));
#162809=CARTESIAN_POINT('Ctrl Pts',(1.70879070887859,-7.94355518819029,
10.1515142731423));
#162810=CARTESIAN_POINT('Ctrl Pts',(1.75281277139888,-7.93397964059079,
10.1532745713825));
#162811=CARTESIAN_POINT('Ctrl Pts',(1.77860106717169,-7.92823837934945,
10.1543050367159));
#162812=CARTESIAN_POINT('Ctrl Pts',(1.84850786305649,-7.91231674593432,
10.1570971787407));
#162813=CARTESIAN_POINT('Ctrl Pts',(1.89257010973498,-7.90189319194668,
10.1588557273213));
#162814=CARTESIAN_POINT('Ctrl Pts',(2.03849354505676,-7.86608234785184,
10.1646794663983));
#162815=CARTESIAN_POINT('Ctrl Pts',(2.13995013157618,-7.83908930294379,
10.1687284611599));
#162816=CARTESIAN_POINT('Ctrl Pts',(2.51647609251735,-7.73105787905047,
10.1838095159714));
#162817=CARTESIAN_POINT('Ctrl Pts',(2.78771618458517,-7.63744368176316,
10.1947921950815));
#162818=CARTESIAN_POINT('Ctrl Pts',(3.13505678288803,-7.49659012125501,
10.2092938959108));
#162819=CARTESIAN_POINT('Ctrl Pts',(3.21613064380215,-7.46216778335393,
10.2127101160946));
#162820=CARTESIAN_POINT('Ctrl Pts',(3.33613636829626,-7.40889668818547,
10.217819418823));
#162821=CARTESIAN_POINT('Ctrl Pts',(3.37550354160689,-7.39104402820663,
10.2195040381777));
#162822=CARTESIAN_POINT('Ctrl Pts',(3.44435470487714,-7.359155819407,10.2224659927665));
#162823=CARTESIAN_POINT('Ctrl Pts',(3.47390007818522,-7.34525506338436,
10.2237421270038));
#162824=CARTESIAN_POINT('Ctrl Pts',(3.5040818945928,-7.33083203171378,10.2250511143772));
#162825=CARTESIAN_POINT('Ctrl Pts',(3.50480293477164,-7.33048733643472,
10.2250823890818));
#162826=CARTESIAN_POINT('Ctrl Pts',(3.5061965566879,-7.32982085894873,10.2251428427155));
#162827=CARTESIAN_POINT('Ctrl Pts',(3.50686914502705,-7.32949909052912,
10.225172021523));
#162828=CARTESIAN_POINT('Ctrl Pts',(3.50816912171393,-7.32887695761007,
10.2252284235291));
#162829=CARTESIAN_POINT('Ctrl Pts',(3.5087965157786,-7.32857660512563,10.2252556466205));
#162830=CARTESIAN_POINT('Ctrl Pts',(3.51000915279073,-7.32799588775397,
10.2253082684474));
#162831=CARTESIAN_POINT('Ctrl Pts',(3.51059440075626,-7.3277155333018,10.2253336670913));
#162832=CARTESIAN_POINT('Ctrl Pts',(3.51172559532561,-7.32717348451479,
10.2253827627916));
#162833=CARTESIAN_POINT('Ctrl Pts',(3.51227154628423,-7.32691179926467,
10.2254064597676));
#162834=CARTESIAN_POINT('Ctrl Pts',(3.51332680799275,-7.32640584610242,
10.2254522668507));
#162835=CARTESIAN_POINT('Ctrl Pts',(3.51383612252943,-7.32616158609483,
10.2254743768878));
#162836=CARTESIAN_POINT('Ctrl Pts',(3.51482059463394,-7.32568932099896,
10.2255171172076));
#162837=CARTESIAN_POINT('Ctrl Pts',(3.5152957555056,-7.3254613227827,10.2255377474297));
#162838=CARTESIAN_POINT('Ctrl Pts',(3.51621423624747,-7.32502049479315,
10.2255776280752));
#162839=CARTESIAN_POINT('Ctrl Pts',(3.51665755898457,-7.32480767100172,
10.2255968784455));
#162840=CARTESIAN_POINT('Ctrl Pts',(3.51751452244458,-7.32439617698688,
10.2256340926169));
#162841=CARTESIAN_POINT('Ctrl Pts',(3.51792816566473,-7.32419751196616,
10.2256520563719));
#162842=CARTESIAN_POINT('Ctrl Pts',(3.51872778212257,-7.32381338792771,
10.2256867842389));
#162843=CARTESIAN_POINT('Ctrl Pts',(3.51911375752603,-7.32362793343991,
10.2257035483105));
#162844=CARTESIAN_POINT('Ctrl Pts',(3.51985991292835,-7.32326934610251,
10.2257359578351));
#162845=CARTESIAN_POINT('Ctrl Pts',(3.52022009482751,-7.32309621718691,
10.2257516032536));
#162846=CARTESIAN_POINT('Ctrl Pts',(3.52091640953461,-7.32276145580888,
10.2257818509848));
#162847=CARTESIAN_POINT('Ctrl Pts',(3.52125254398466,-7.32259982677545,
10.2257964532668));
#162848=CARTESIAN_POINT('Ctrl Pts',(3.52190239037642,-7.32228729539804,
10.2258246850882));
#162849=CARTESIAN_POINT('Ctrl Pts',(3.52221610375679,-7.32213639603381,
10.2258383146013));
#162850=CARTESIAN_POINT('Ctrl Pts',(3.52282262305852,-7.32184460600965,
10.2258646664471));
#162851=CARTESIAN_POINT('Ctrl Pts',(3.52311543022188,-7.3217037179483,10.2258773887566));
#162852=CARTESIAN_POINT('Ctrl Pts',(3.52368154816212,-7.32143128094813,
10.2259019872793));
#162853=CARTESIAN_POINT('Ctrl Pts',(3.52395486003317,-7.32129973426526,
10.2259138634728));
#162854=CARTESIAN_POINT('Ctrl Pts',(3.52448330174721,-7.32104535557484,
10.225936826679));
#162855=CARTESIAN_POINT('Ctrl Pts',(3.52473843252175,-7.32092252554165,
10.2259479136737));
#162856=CARTESIAN_POINT('Ctrl Pts',(3.5252317362463,-7.32068499787717,10.2259693515096));
#162857=CARTESIAN_POINT('Ctrl Pts',(3.52546991002964,-7.32057030195445,
10.2259797023362));
#162858=CARTESIAN_POINT('Ctrl Pts',(3.52593044019454,-7.3203484995131,10.2259997172483));
#162859=CARTESIAN_POINT('Ctrl Pts',(3.52615279729178,-7.32024139448731,
10.2260093813205));
#162860=CARTESIAN_POINT('Ctrl Pts',(3.52675068213241,-7.3199533715954,10.226035367371));
#162861=CARTESIAN_POINT('Ctrl Pts',(3.52712620082542,-7.31977243496631,
10.2260516895154));
#162862=CARTESIAN_POINT('Ctrl Pts',(3.52787186354028,-7.3194130806903,10.2260841019011));
#162863=CARTESIAN_POINT('Ctrl Pts',(3.52824201365148,-7.31923466111413,
10.2261001923827));
#162864=CARTESIAN_POINT('Ctrl Pts',(3.52897706204733,-7.31888028472595,
10.2261321467115));
#162865=CARTESIAN_POINT('Ctrl Pts',(3.52934195494318,-7.3187043314841,10.2261480103007));
#162866=CARTESIAN_POINT('Ctrl Pts',(3.53006658476145,-7.31835484444252,
10.2261795149417));
#162867=CARTESIAN_POINT('Ctrl Pts',(3.53042632206502,-7.31818131139801,
10.2261951559874));
#162868=CARTESIAN_POINT('Ctrl Pts',(3.53114074206643,-7.31783661865404,
10.2262262198812));
#162869=CARTESIAN_POINT('Ctrl Pts',(3.53149542509341,-7.31766545970364,
10.2262416427217));
#162870=CARTESIAN_POINT('Ctrl Pts',(3.56685255137686,-7.30060004562135,
10.2277791691853));
#162871=CARTESIAN_POINT('Ctrl Pts',(3.60173325761103,-7.28345492721995,
10.2293034803997));
#162872=CARTESIAN_POINT('Ctrl Pts',(3.71118441605843,-7.22867723777756,
10.2341107426513));
#162873=CARTESIAN_POINT('Ctrl Pts',(3.78529804408404,-7.19014485005422,
10.2374015663014));
#162874=CARTESIAN_POINT('Ctrl Pts',(3.95757713078065,-7.09717325481907,
10.2451371065078));
#162875=CARTESIAN_POINT('Ctrl Pts',(4.05523457613207,-7.04182911029313,
10.2495889123754));
#162876=CARTESIAN_POINT('Ctrl Pts',(4.30830254769003,-6.89140048273695,
10.2613001709367));
#162877=CARTESIAN_POINT('Ctrl Pts',(4.46171639275852,-6.79308161000347,
10.2685786282759));
#162878=CARTESIAN_POINT('Ctrl Pts',(4.63177606156879,-6.67584698457957,
10.2768294992151));
#162879=CARTESIAN_POINT('Ctrl Pts',(4.65179462951999,-6.66191332662261,
10.2778036733782));
#162880=CARTESIAN_POINT('Ctrl Pts',(4.82552668531783,-6.53982454489698,
10.2862829172916));
#162881=CARTESIAN_POINT('Ctrl Pts',(4.97550869415378,-6.42645526630782,
10.293774749702));
#162882=CARTESIAN_POINT('Ctrl Pts',(5.14773201326787,-6.28662794470906,
10.3025267626075));
#162883=CARTESIAN_POINT('Ctrl Pts',(5.17390509734162,-6.26510509525038,
10.3038609860312));
#162884=CARTESIAN_POINT('Ctrl Pts',(5.21405163519809,-6.23166833564856,
10.3059134209709));
#162885=CARTESIAN_POINT('Ctrl Pts',(5.22812050297963,-6.21986983043301,
10.3066337790557));
#162886=CARTESIAN_POINT('Ctrl Pts',(5.2563838979688,-6.19600379122663,10.3080832652032));
#162887=CARTESIAN_POINT('Ctrl Pts',(5.27057712280001,-6.18393494944108,
10.3088123683506));
#162888=CARTESIAN_POINT('Ctrl Pts',(5.30429008782234,-6.15506762167589,
10.3105472561971));
#162889=CARTESIAN_POINT('Ctrl Pts',(5.3237717419084,-6.13822492333912,10.3115522541191));
#162890=CARTESIAN_POINT('Ctrl Pts',(5.38847419393348,-6.0817472192066,10.3148989536424));
#162891=CARTESIAN_POINT('Ctrl Pts',(5.43333521065963,-6.04170273454323,
10.3172339862031));
#162892=CARTESIAN_POINT('Ctrl Pts',(5.54351828268168,-5.94112972933677,
10.3230117213443));
#162893=CARTESIAN_POINT('Ctrl Pts',(5.60829774390473,-5.88001819535284,
10.3264467278162));
#162894=CARTESIAN_POINT('Ctrl Pts',(5.91129756648928,-5.58461147961954,
10.3427326787712));
#162895=CARTESIAN_POINT('Ctrl Pts',(6.13592099468687,-5.33683417118405,
10.3554772539437));
#162896=CARTESIAN_POINT('Ctrl Pts',(6.48224024490431,-4.90395316903533,
10.3768056122942));
#162897=CARTESIAN_POINT('Ctrl Pts',(6.61277875294917,-4.72645224784754,
10.3853151448662));
#162898=CARTESIAN_POINT('Ctrl Pts',(6.77395761074221,-4.48751674341049,
10.3965297098054));
#162899=CARTESIAN_POINT('Ctrl Pts',(6.81126266711804,-4.43068945654746,
10.3991796890481));
#162900=CARTESIAN_POINT('Ctrl Pts',(6.87497336751892,-4.33093154833192,
10.403803019197));
#162901=CARTESIAN_POINT('Ctrl Pts',(6.90170085040494,-4.28821084265929,
10.4057739727337));
#162902=CARTESIAN_POINT('Ctrl Pts',(6.95545264356238,-4.20049057090326,
10.4098031666068));
#162903=CARTESIAN_POINT('Ctrl Pts',(6.98244179159792,-4.15547218959073,
10.4118615336058));
#162904=CARTESIAN_POINT('Ctrl Pts',(7.03894928240731,-4.05911166605496,
10.4162476134647));
#162905=CARTESIAN_POINT('Ctrl Pts',(7.06834634013845,-4.00770189850069,
10.4185758832597));
#162906=CARTESIAN_POINT('Ctrl Pts',(7.1107659305653,-3.93159945137952,10.42200514909));
#162907=CARTESIAN_POINT('Ctrl Pts',(7.12422746798997,-3.90715361195838,
10.4231041098016));
#162908=CARTESIAN_POINT('Ctrl Pts',(7.17337663564569,-3.81680133433638,
10.4271562674272));
#162909=CARTESIAN_POINT('Ctrl Pts',(7.20827778092115,-3.7504714616891,10.4301123142812));
#162910=CARTESIAN_POINT('Ctrl Pts',(7.33593554461111,-3.49949060674241,
10.4412249285254));
#162911=CARTESIAN_POINT('Ctrl Pts',(7.42255521428859,-3.3118060388286,10.4493910383001));
#162912=CARTESIAN_POINT('Ctrl Pts',(7.5148724022378,-3.08990554796304,10.4588440320815));
#162913=CARTESIAN_POINT('Ctrl Pts',(7.52762483364334,-3.05870689803732,
10.4601685037238));
#162914=CARTESIAN_POINT('Ctrl Pts',(7.55371688170796,-2.99372147230505,
10.4629173778105));
#162915=CARTESIAN_POINT('Ctrl Pts',(7.56702476633594,-2.95992283287973,
10.464341400777));
#162916=CARTESIAN_POINT('Ctrl Pts',(7.59471510713539,-2.88818902293506,
10.4673522393804));
#162917=CARTESIAN_POINT('Ctrl Pts',(7.60904097186529,-2.85023312918963,
10.4689386855553));
#162918=CARTESIAN_POINT('Ctrl Pts',(7.64556271482043,-2.75123196816582,
10.4730611587756));
#162919=CARTESIAN_POINT('Ctrl Pts',(7.66731193345125,-2.69002496553027,
10.4755946481013));
#162920=CARTESIAN_POINT('Ctrl Pts',(7.74695149019609,-2.4570860423642,10.4851890236454));
#162921=CARTESIAN_POINT('Ctrl Pts',(7.79982475366788,-2.28369504403652,
10.4922346519436));
#162922=CARTESIAN_POINT('Ctrl Pts',(7.87331385630181,-2.01022633545768,
10.503272909895));
#162923=CARTESIAN_POINT('Ctrl Pts',(7.89791625943527,-1.91128220100265,
10.5072515897117));
#162924=CARTESIAN_POINT('Ctrl Pts',(7.93237398500466,-1.76065173256889,
10.5132956950265));
#162925=CARTESIAN_POINT('Ctrl Pts',(7.9436000317772,-1.70928934836631,10.5153543432748));
#162926=CARTESIAN_POINT('Ctrl Pts',(7.96475263439291,-1.60779790912964,
10.5194191440834));
#162927=CARTESIAN_POINT('Ctrl Pts',(7.97470633569509,-1.55767695060615,
10.5214250577235));
#162928=CARTESIAN_POINT('Ctrl Pts',(7.99408052241681,-1.45506291582417,
10.525529997864));
#162929=CARTESIAN_POINT('Ctrl Pts',(8.00345830989705,-1.40256427466893,
10.5276291684506));
#162930=CARTESIAN_POINT('Ctrl Pts',(8.02429097204558,-1.27891928218496,
10.5325721218566));
#162931=CARTESIAN_POINT('Ctrl Pts',(8.03531752175575,-1.20770542584511,
10.5354182603425));
#162932=CARTESIAN_POINT('Ctrl Pts',(8.09849714336799,-0.760393423566754,
10.5532968006508));
#162933=CARTESIAN_POINT('Ctrl Pts',(8.12517915088166,-0.381183041305498,
10.5684829774549));
#162934=CARTESIAN_POINT('Ctrl Pts',(8.12524985909245,-0.00151321448057171,
10.5836791336291));
#162935=CARTESIAN_POINT('',(8.12631724021387,-0.0026888491199863,14.5832974432124));
#162936=CARTESIAN_POINT('Ctrl Pts',(8.12524985911998,-0.00151306667137495,
10.5836791395451));
#162937=CARTESIAN_POINT('Ctrl Pts',(8.12529265115791,0.228282491430003,
10.5928766288908));
#162938=CARTESIAN_POINT('Ctrl Pts',(8.11558692129937,0.457979970419391,
10.6020610450867));
#162939=CARTESIAN_POINT('Ctrl Pts',(8.09315866316021,0.722308052229391,
10.6125517107936));
#162940=CARTESIAN_POINT('Ctrl Pts',(8.0899278691087,0.757636559940404,10.6139521386737));
#162941=CARTESIAN_POINT('Ctrl Pts',(8.08419352636532,0.816115635688944,
10.6162669789118));
#162942=CARTESIAN_POINT('Ctrl Pts',(8.08182165012504,0.839278572863596,
10.6171830084473));
#162943=CARTESIAN_POINT('Ctrl Pts',(8.07734109287788,0.881252933032226,
10.6188412735829));
#162944=CARTESIAN_POINT('Ctrl Pts',(8.07526617865032,0.900067780436113,
10.6195839632212));
#162945=CARTESIAN_POINT('Ctrl Pts',(8.07108472871043,0.93680548842099,10.6210328256588));
#162946=CARTESIAN_POINT('Ctrl Pts',(8.06898419304009,0.954728922878413,
10.6217390820601));
#162947=CARTESIAN_POINT('Ctrl Pts',(8.06393028238987,0.996644521322071,
10.623389204976));
#162948=CARTESIAN_POINT('Ctrl Pts',(8.06092952216192,1.02063075704632,10.6243322776981));
#162949=CARTESIAN_POINT('Ctrl Pts',(8.05228363369517,1.08732308727048,10.6269515234829));
#162950=CARTESIAN_POINT('Ctrl Pts',(8.04640584367617,1.12999833755841,10.6286242518605));
#162951=CARTESIAN_POINT('Ctrl Pts',(8.02962009212361,1.2450910696279,10.6331297389549));
#162952=CARTESIAN_POINT('Ctrl Pts',(8.01807196723447,1.31741133804886,10.6359546758437));
#162953=CARTESIAN_POINT('Ctrl Pts',(7.96625029425089,1.61596563119189,10.6476130340297));
#162954=CARTESIAN_POINT('Ctrl Pts',(7.91736642247098,1.84059735638636,10.6563797654729));
#162955=CARTESIAN_POINT('Ctrl Pts',(7.80968269373701,2.25084876072845,10.6726264459083));
#162956=CARTESIAN_POINT('Ctrl Pts',(7.75360875783441,2.43700925418768,10.6800904127697));
#162957=CARTESIAN_POINT('Ctrl Pts',(7.66672913416935,2.69194599507781,10.6905122411309));
#162958=CARTESIAN_POINT('Ctrl Pts',(7.64156319577322,2.76257501026842,10.6934210417988));
#162959=CARTESIAN_POINT('Ctrl Pts',(7.61403276671079,2.83658394930537,10.6964937659909));
#162960=CARTESIAN_POINT('Ctrl Pts',(7.61263928763962,2.84032155754824,10.6966490117158));
#162961=CARTESIAN_POINT('Ctrl Pts',(7.60992488073863,2.84758582912157,10.696950871385));
#162962=CARTESIAN_POINT('Ctrl Pts',(7.60860425227359,2.85111260334811,10.6970974826651));
#162963=CARTESIAN_POINT('Ctrl Pts',(7.60601412460523,2.85801499387517,10.6973845386176));
#162964=CARTESIAN_POINT('Ctrl Pts',(7.60474482890162,2.86139068569684,10.6975249814674));
#162965=CARTESIAN_POINT('Ctrl Pts',(7.60223710546207,2.86804652121934,10.6978020006031));
#162966=CARTESIAN_POINT('Ctrl Pts',(7.60099880122183,2.87132671066121,10.6979385757707));
#162967=CARTESIAN_POINT('Ctrl Pts',(7.58815796127725,2.90527476393036,10.6993525901106));
#162968=CARTESIAN_POINT('Ctrl Pts',(7.57637203371379,2.93587286808058,10.7006316431492));
#162969=CARTESIAN_POINT('Ctrl Pts',(7.55209785131115,2.9977727244565,10.7032286783329));
#162970=CARTESIAN_POINT('Ctrl Pts',(7.53959941775076,3.02906980340426,10.7045467295308));
#162971=CARTESIAN_POINT('Ctrl Pts',(7.50984075115534,3.1022624880415,10.7076410795414));
#162972=CARTESIAN_POINT('Ctrl Pts',(7.49242407357638,3.1440932129875,10.709418748656));
#162973=CARTESIAN_POINT('Ctrl Pts',(7.43526071153168,3.27821331877689,10.715148624682));
#162974=CARTESIAN_POINT('Ctrl Pts',(7.39415185960124,3.36991134389192,10.7191126189783));
#162975=CARTESIAN_POINT('Ctrl Pts',(7.2178994729735,3.74430021180341,10.735490817272));
#162976=CARTESIAN_POINT('Ctrl Pts',(7.06816124149337,4.01981968477365,10.7480196970835));
#162977=CARTESIAN_POINT('Ctrl Pts',(6.862123225813,4.35165777445126,10.7635699358125));
#162978=CARTESIAN_POINT('Ctrl Pts',(6.8204211224188,4.41673141052762,10.766641694564));
#162979=CARTESIAN_POINT('Ctrl Pts',(6.75719266075966,4.51236419446143,10.7711841388713));
#162980=CARTESIAN_POINT('Ctrl Pts',(6.73637369886617,4.54338559694112,10.7726620863151));
#162981=CARTESIAN_POINT('Ctrl Pts',(6.69836453311552,4.5991857468792,10.7753278451495));
#162982=CARTESIAN_POINT('Ctrl Pts',(6.68124892407901,4.62401446548007,10.7765166325493));
#162983=CARTESIAN_POINT('Ctrl Pts',(6.65288023759654,4.66468107558776,10.7784676584035));
#162984=CARTESIAN_POINT('Ctrl Pts',(6.64170789764263,4.68057487901611,10.7792311762396));
#162985=CARTESIAN_POINT('Ctrl Pts',(6.61971775452888,4.71162084821153,10.7807243962234));
#162986=CARTESIAN_POINT('Ctrl Pts',(6.60890466668478,4.7267762034841,10.7814541679662));
#162987=CARTESIAN_POINT('Ctrl Pts',(6.58440445999246,4.76086665791639,10.7830975369568));
#162988=CARTESIAN_POINT('Ctrl Pts',(6.57068757961514,4.77978013759346,10.7840105872908));
#162989=CARTESIAN_POINT('Ctrl Pts',(6.51864108322602,4.85089685484496,10.7874491675334));
#162990=CARTESIAN_POINT('Ctrl Pts',(6.47976917033216,4.90270063014863,10.7899650087921));
#162991=CARTESIAN_POINT('Ctrl Pts',(6.17837103672735,5.29452046066359,10.8090991282585));
#162992=CARTESIAN_POINT('Ctrl Pts',(5.88986677228204,5.61370616202336,10.8253168143115));
#162993=CARTESIAN_POINT('Ctrl Pts',(5.30859019482285,6.16240905196027,10.8556902447381));
#162994=CARTESIAN_POINT('Ctrl Pts',(5.02269081090321,6.39757655641904,10.8697827030386));
#162995=CARTESIAN_POINT('Ctrl Pts',(4.63055603046021,6.67758956403809,10.8884167132347));
#162996=CARTESIAN_POINT('Ctrl Pts',(4.53799862327918,6.74083227399317,10.8927672121003));
#162997=CARTESIAN_POINT('Ctrl Pts',(4.41062536777149,6.8240513137138,10.8986958469211));
#162998=CARTESIAN_POINT('Ctrl Pts',(4.37692613319178,6.84571472371547,10.900258962277));
#162999=CARTESIAN_POINT('Ctrl Pts',(4.31356226024147,6.88578877191805,10.9031882058082));
#163000=CARTESIAN_POINT('Ctrl Pts',(4.28393647181853,6.90425916962392,10.90455379719));
#163001=CARTESIAN_POINT('Ctrl Pts',(4.22187352931657,6.94239947464928,10.9074064677361));
#163002=CARTESIAN_POINT('Ctrl Pts',(4.18941580722701,6.96203431093546,10.9088937939024));
#163003=CARTESIAN_POINT('Ctrl Pts',(4.11424812518309,7.00678992200614,10.9123279440105));
#163004=CARTESIAN_POINT('Ctrl Pts',(4.07144353127451,7.03174872955914,10.914275954168));
#163005=CARTESIAN_POINT('Ctrl Pts',(3.93338203666808,7.11056732350726,10.9205352733369));
#163006=CARTESIAN_POINT('Ctrl Pts',(3.83726479815657,7.16289470562214,10.9248570928374));
#163007=CARTESIAN_POINT('Ctrl Pts',(3.36121053052287,7.40973167124872,10.9460910605371));
#163008=CARTESIAN_POINT('Ctrl Pts',(2.96742000936151,7.57603226117489,10.9630780234009));
#163009=CARTESIAN_POINT('Ctrl Pts',(2.00833633791254,7.89475521907546,11.0044517423284));
#163010=CARTESIAN_POINT('Ctrl Pts',(1.43605565189704,8.01861883388864,11.0292861957511));
#163011=CARTESIAN_POINT('Ctrl Pts',(0.635130703420006,8.10341941460139,
11.0632324896176));
#163012=CARTESIAN_POINT('Ctrl Pts',(0.413886850961786,8.11772751179484,
11.0724984861625));
#163013=CARTESIAN_POINT('Ctrl Pts',(0.129590859632434,8.12445888940698,
11.0840878714626));
#163014=CARTESIAN_POINT('Ctrl Pts',(0.0668351667036395,8.12521749339648,
11.0866260193365));
#163015=CARTESIAN_POINT('Ctrl Pts',(-0.0220465098795425,8.12526208246541,
11.0901870086564));
#163016=CARTESIAN_POINT('Ctrl Pts',(-0.0481692811329664,8.12514921066762,
11.0912294606377));
#163017=CARTESIAN_POINT('Ctrl Pts',(-0.0935171110648323,8.12473456663143,
11.0930314186847));
#163018=CARTESIAN_POINT('Ctrl Pts',(-0.112742417193487,8.1244905306867,
11.093792963717));
#163019=CARTESIAN_POINT('Ctrl Pts',(-0.141589131703196,8.12402195310369,
11.0949318525471));
#163020=CARTESIAN_POINT('Ctrl Pts',(-0.151211231384496,8.12384855479316,
11.0953111094605));
#163021=CARTESIAN_POINT('Ctrl Pts',(-0.168091093588086,8.12351436552898,
11.0959753002843));
#163022=CARTESIAN_POINT('Ctrl Pts',(-0.175348981507235,8.12336094223565,
11.0962605172744));
#163023=CARTESIAN_POINT('Ctrl Pts',(-0.189434441725192,8.12304430597555,
11.0968133156299));
#163024=CARTESIAN_POINT('Ctrl Pts',(-0.196262030954958,8.12288221138896,
11.0970809406237));
#163025=CARTESIAN_POINT('Ctrl Pts',(-0.212551508866258,8.12247493105734,
11.0977186466833));
#163026=CARTESIAN_POINT('Ctrl Pts',(-0.222013202487022,8.12222181970473,
11.0980884105787));
#163027=CARTESIAN_POINT('Ctrl Pts',(-0.255822710572896,8.12125825363165,
11.09940732992));
#163028=CARTESIAN_POINT('Ctrl Pts',(-0.280167902308072,8.12045484227611,
11.1003526707005));
#163029=CARTESIAN_POINT('Ctrl Pts',(-0.719717783733941,8.10397028905207,
11.1173371884553));
#163030=CARTESIAN_POINT('Ctrl Pts',(-1.13312688033432,8.05657256933183,
11.131825676582));
#163031=CARTESIAN_POINT('Ctrl Pts',(-1.89297623454167,7.90978937642664,
11.1580067482654));
#163032=CARTESIAN_POINT('Ctrl Pts',(-2.23997418020351,7.81860901940375,
11.1697960761293));
#163033=CARTESIAN_POINT('Ctrl Pts',(-3.12792621930284,7.52129418690696,
11.2013369051586));
#163034=CARTESIAN_POINT('Ctrl Pts',(-3.6548209486279,7.2798338754045,11.2215530013828));
#163035=CARTESIAN_POINT('Ctrl Pts',(-4.17601726727558,6.97003392361174,
11.2449069805585));
#163036=CARTESIAN_POINT('Ctrl Pts',(-4.20033856836218,6.95540430202424,
11.2460045988469));
#163037=CARTESIAN_POINT('Ctrl Pts',(-4.23563207237819,6.93392211046934,
11.2476089261183));
#163038=CARTESIAN_POINT('Ctrl Pts',(-4.24666546278597,6.92717022541985,
11.2481121188675));
#163039=CARTESIAN_POINT('Ctrl Pts',(-4.26596529626576,6.91529624982362,
11.2489952220247));
#163040=CARTESIAN_POINT('Ctrl Pts',(-4.27423876756105,6.91018560451417,
11.2493747311537));
#163041=CARTESIAN_POINT('Ctrl Pts',(-4.29025952257052,6.90024956767657,
11.2501114415699));
#163042=CARTESIAN_POINT('Ctrl Pts',(-4.29800789232975,6.8954259494295,11.250468580315));
#163043=CARTESIAN_POINT('Ctrl Pts',(-4.31644599173505,6.88390446583105,
11.251320420033));
#163044=CARTESIAN_POINT('Ctrl Pts',(-4.3271282683962,6.87719475086799,11.2518155374269));
#163045=CARTESIAN_POINT('Ctrl Pts',(-4.36507270314597,6.85323781514009,
11.253579945961));
#163046=CARTESIAN_POINT('Ctrl Pts',(-4.39224755367537,6.83585324979259,
11.2548540774218));
#163047=CARTESIAN_POINT('Ctrl Pts',(-4.84284466526236,6.54379661686656,
11.2761577162981));
#163048=CARTESIAN_POINT('Ctrl Pts',(-5.23982019050381,6.2304570818495,11.297628900543));
#163049=CARTESIAN_POINT('Ctrl Pts',(-5.79100952472595,5.70524468651953,
11.3313031969452));
#163050=CARTESIAN_POINT('Ctrl Pts',(-5.96838379670385,5.51942010774735,
11.3428413712309));
#163051=CARTESIAN_POINT('Ctrl Pts',(-6.49110043748582,4.91708699120388,
11.3786662859981));
#163052=CARTESIAN_POINT('Ctrl Pts',(-6.80394575591562,4.47422117943838,
11.4028777576027));
#163053=CARTESIAN_POINT('Ctrl Pts',(-7.08429012982834,3.97910859437228,
11.4256860842845));
#163054=CARTESIAN_POINT('Ctrl Pts',(-7.09796286858158,3.95466749460866,
11.4268024466376));
#163055=CARTESIAN_POINT('Ctrl Pts',(-7.11694028075076,3.92032838958783,
11.4283581489933));
#163056=CARTESIAN_POINT('Ctrl Pts',(-7.12235111468058,3.91048951447941,
11.4288024306939));
#163057=CARTESIAN_POINT('Ctrl Pts',(-7.13151191494472,3.89374974193561,
11.4295558964342));
#163058=CARTESIAN_POINT('Ctrl Pts',(-7.13527229326003,3.88685458274594,
11.4298655520171));
#163059=CARTESIAN_POINT('Ctrl Pts',(-7.14268325889419,3.87321858289333,
11.4304765711139));
#163060=CARTESIAN_POINT('Ctrl Pts',(-7.14633431529943,3.86647800746843,
11.4307779553236));
#163061=CARTESIAN_POINT('Ctrl Pts',(-7.15435109770708,3.85162728813988,
11.4314405358723));
#163062=CARTESIAN_POINT('Ctrl Pts',(-7.15871258727613,3.84351486137858,
11.4318015473707));
#163063=CARTESIAN_POINT('Ctrl Pts',(-7.17384226158204,3.8152583796623,11.4330557989328));
#163064=CARTESIAN_POINT('Ctrl Pts',(-7.1845393447092,3.79507624620174,11.4339460105105));
#163065=CARTESIAN_POINT('Ctrl Pts',(-7.30939040062601,3.55710058317286,
11.4443793829554));
#163066=CARTESIAN_POINT('Ctrl Pts',(-7.4136915840685,3.33426762328105,11.4535284661577));
#163067=CARTESIAN_POINT('Ctrl Pts',(-7.82054910795897,2.35115279212803,
11.4924060625655));
#163068=CARTESIAN_POINT('Ctrl Pts',(-8.01742843781844,1.55236406007379,
11.5208665305891));
#163069=CARTESIAN_POINT('Ctrl Pts',(-8.09801399738059,0.668353344859133,
11.5546854401877));
#163070=CARTESIAN_POINT('Ctrl Pts',(-8.10343931057638,0.598997574237792,
11.557349112804));
#163071=CARTESIAN_POINT('Ctrl Pts',(-8.11154474092193,0.47490213009185,
11.5621344235867));
#163072=CARTESIAN_POINT('Ctrl Pts',(-8.11456292977148,0.420188659166743,
11.5642509465442));
#163073=CARTESIAN_POINT('Ctrl Pts',(-8.11825794597017,0.338118285954926,
11.5674357836876));
#163074=CARTESIAN_POINT('Ctrl Pts',(-8.11935040071199,0.310781458755766,
11.5684982883157));
#163075=CARTESIAN_POINT('Ctrl Pts',(-8.1210710357293,0.261486739850709,
11.5704172138061));
#163076=CARTESIAN_POINT('Ctrl Pts',(-8.12174827740896,0.239530782974643,
11.5712729687722));
#163077=CARTESIAN_POINT('Ctrl Pts',(-8.12288624877459,0.197048441890887,
11.572930810875));
#163078=CARTESIAN_POINT('Ctrl Pts',(-8.12335822854482,0.176522481287602,
11.573732757641));
#163079=CARTESIAN_POINT('Ctrl Pts',(-8.12438472758666,0.12306548295282,
11.5758239082714));
#163080=CARTESIAN_POINT('Ctrl Pts',(-8.12481682408881,0.0901325447555323,
11.5771147536032));
#163081=CARTESIAN_POINT('Ctrl Pts',(-8.12561658356266,-0.0234743099147386,
11.5815773309753));
#163082=CARTESIAN_POINT('Ctrl Pts',(-8.12498298390104,-0.104149851407131,
11.5847631281905));
#163083=CARTESIAN_POINT('Ctrl Pts',(-8.10433610808371,-1.01170351500131,
11.6208219477433));
#163084=CARTESIAN_POINT('Ctrl Pts',(-7.95936508962477,-1.83085476222711,
11.6561536426617));
#163085=CARTESIAN_POINT('Ctrl Pts',(-7.61448465331733,-2.84594486187559,
11.7012645010144));
#163086=CARTESIAN_POINT('Ctrl Pts',(-7.52515977387297,-3.07437113449255,
11.7114510975381));
#163087=CARTESIAN_POINT('Ctrl Pts',(-7.4096944074711,-3.3343154378054,11.7228700119843));
#163088=CARTESIAN_POINT('Ctrl Pts',(-7.39348766625363,-3.37009952968905,
11.7244379287296));
#163089=CARTESIAN_POINT('Ctrl Pts',(-7.37170466490312,-3.41728237323068,
11.7264987936629));
#163090=CARTESIAN_POINT('Ctrl Pts',(-7.36636044210507,-3.42878729642047,
11.7270007944998));
#163091=CARTESIAN_POINT('Ctrl Pts',(-7.35755157994219,-3.44763516511162,
11.7278223000871));
#163092=CARTESIAN_POINT('Ctrl Pts',(-7.35410284912168,-3.4549854946647,
11.7281424488936));
#163093=CARTESIAN_POINT('Ctrl Pts',(-7.34740518124786,-3.46920486623594,
11.7287613350122));
#163094=CARTESIAN_POINT('Ctrl Pts',(-7.34415761505196,-3.47607454279973,
11.7290601287303));
#163095=CARTESIAN_POINT('Ctrl Pts',(-7.33664634520981,-3.49190584885813,
11.7297482207586));
#163096=CARTESIAN_POINT('Ctrl Pts',(-7.33237584494681,-3.50086425351041,
11.7301372306741));
#163097=CARTESIAN_POINT('Ctrl Pts',(-7.32091098261479,-3.52480156492575,
11.7311756862282));
#163098=CARTESIAN_POINT('Ctrl Pts',(-7.31368704248173,-3.53976631112827,
11.7318238435214));
#163099=CARTESIAN_POINT('Ctrl Pts',(-7.25729415643373,-3.65567733766896,
11.7368355291189));
#163100=CARTESIAN_POINT('Ctrl Pts',(-7.20608706340845,-3.75560987903254,
11.7410983140621));
#163101=CARTESIAN_POINT('Ctrl Pts',(-6.82713873912917,-4.45883393915177,
11.7707338083873));
#163102=CARTESIAN_POINT('Ctrl Pts',(-6.42614615297047,-5.01954530813275,
11.7927778355634));
#163103=CARTESIAN_POINT('Ctrl Pts',(-5.61179172038431,-5.89821701954696,
11.8336009652055));
#163104=CARTESIAN_POINT('Ctrl Pts',(-5.22960669425561,-6.2395766536831,
11.8516698324195));
#163105=CARTESIAN_POINT('Ctrl Pts',(-4.78720361993821,-6.56535011823596,
11.8727520685766));
#163106=CARTESIAN_POINT('Ctrl Pts',(-4.7563498213442,-6.58773686514507,
11.8742226524467));
#163107=CARTESIAN_POINT('Ctrl Pts',(-4.71347846809473,-6.61838506657224,
11.8762667188977));
#163108=CARTESIAN_POINT('Ctrl Pts',(-4.70159429560587,-6.62683266994992,
11.8768334175325));
#163109=CARTESIAN_POINT('Ctrl Pts',(-4.6814943471707,-6.64103899254882,
11.8777920269946));
#163110=CARTESIAN_POINT('Ctrl Pts',(-4.67329050777977,-6.64681457934395,
11.8781833248629));
#163111=CARTESIAN_POINT('Ctrl Pts',(-4.65703564395792,-6.658213199561,11.8789587159831));
#163112=CARTESIAN_POINT('Ctrl Pts',(-4.64898508032753,-6.66383686189753,
11.879342785471));
#163113=CARTESIAN_POINT('Ctrl Pts',(-4.63121871570784,-6.6761995612146,
11.8801904643422));
#163114=CARTESIAN_POINT('Ctrl Pts',(-4.62149836737635,-6.68293200719578,
11.8806543102977));
#163115=CARTESIAN_POINT('Ctrl Pts',(-4.58749229554157,-6.70637540354939,
11.8822772857245));
#163116=CARTESIAN_POINT('Ctrl Pts',(-4.56313048606076,-6.72297529074886,
11.883440401352));
#163117=CARTESIAN_POINT('Ctrl Pts',(-4.30886999711988,-6.89420708232514,
11.8955847305446));
#163118=CARTESIAN_POINT('Ctrl Pts',(-4.07131186355975,-7.03710546185362,
11.9069827030973));
#163119=CARTESIAN_POINT('Ctrl Pts',(-3.70578840531833,-7.23226655614917,
11.924591624839));
#163120=CARTESIAN_POINT('Ctrl Pts',(-3.58302699048722,-7.2938647448299,
11.9305153698488));
#163121=CARTESIAN_POINT('Ctrl Pts',(-2.9154949321715,-7.60789314700132,
11.9627271364486));
#163122=CARTESIAN_POINT('Ctrl Pts',(-2.34561218264704,-7.80244741272736,
11.9903756857371));
#163123=CARTESIAN_POINT('Ctrl Pts',(-1.4305579981823,-8.0054192632853,12.0318452353692));
#163124=CARTESIAN_POINT('Ctrl Pts',(-1.09731261015582,-8.0578666042927,
12.0463258643458));
#163125=CARTESIAN_POINT('Ctrl Pts',(-0.738091934923298,-8.09169148247531,
12.0607265603345));
#163126=CARTESIAN_POINT('Ctrl Pts',(-0.714455018619491,-8.09381274774334,
12.061669047209));
#163127=CARTESIAN_POINT('Ctrl Pts',(-0.680727215952277,-8.09669070681349,
12.0630070578546));
#163128=CARTESIAN_POINT('Ctrl Pts',(-0.670643831490075,-8.09753214238101,
12.0634062034579));
#163129=CARTESIAN_POINT('Ctrl Pts',(-0.653239222353201,-8.09895178492797,
12.0640936920894));
#163130=CARTESIAN_POINT('Ctrl Pts',(-0.645918751949548,-8.09953890431957,
12.0643824066605));
#163131=CARTESIAN_POINT('Ctrl Pts',(-0.631905802522059,-8.10064365813612,
12.0649342295564));
#163132=CARTESIAN_POINT('Ctrl Pts',(-0.625213461827286,-8.10116292558314,
12.065197404548));
#163133=CARTESIAN_POINT('Ctrl Pts',(-0.609541213024148,-8.1023594198958,
12.0658128709066));
#163134=CARTESIAN_POINT('Ctrl Pts',(-0.600560796162926,-8.10303001293335,
12.0661648947441));
#163135=CARTESIAN_POINT('Ctrl Pts',(-0.569493237913271,-8.10529798381146,
12.0673805300424));
#163136=CARTESIAN_POINT('Ctrl Pts',(-0.547400581031609,-8.10682000356397,
12.068241172011));
#163137=CARTESIAN_POINT('Ctrl Pts',(-0.210674478157437,-8.12863516795831,
12.0813040481688));
#163138=CARTESIAN_POINT('Ctrl Pts',(0.104892474832877,-8.13068960530555,
12.0928329131821));
#163139=CARTESIAN_POINT('Ctrl Pts',(0.825502891211111,-8.09340922295008,
12.1188609473769));
#163140=CARTESIAN_POINT('Ctrl Pts',(1.22906490512882,-8.04202287321422,
12.1332444810864));
#163141=CARTESIAN_POINT('Ctrl Pts',(2.20786328258949,-7.84196480575918,
12.1695562714419));
#163142=CARTESIAN_POINT('Ctrl Pts',(2.77386969966544,-7.66006811214229,
12.1919170142696));
#163143=CARTESIAN_POINT('Ctrl Pts',(3.41806590246757,-7.37219469490929,
12.2191842372807));
#163144=CARTESIAN_POINT('Ctrl Pts',(3.52015105456113,-7.32399927498181,
12.2235620969215));
#163145=CARTESIAN_POINT('Ctrl Pts',(3.66587450289509,-7.25145105203742,
12.229903523818));
#163146=CARTESIAN_POINT('Ctrl Pts',(3.7103446981521,-7.22879799293918,12.231851331262));
#163147=CARTESIAN_POINT('Ctrl Pts',(3.78818133192683,-7.18824063046671,
12.2352837101963));
#163148=CARTESIAN_POINT('Ctrl Pts',(3.8216366418659,-7.17051006061672,12.2367665956087));
#163149=CARTESIAN_POINT('Ctrl Pts',(3.89127750408656,-7.13297612606508,
12.2398697126844));
#163150=CARTESIAN_POINT('Ctrl Pts',(3.92743864147188,-7.11312974216804,
12.2414903227027));
#163151=CARTESIAN_POINT('Ctrl Pts',(4.02219228751627,-7.0601830931749,12.2457620127695));
#163152=CARTESIAN_POINT('Ctrl Pts',(4.0805272593001,-7.02662887284802,12.2484174582775));
#163153=CARTESIAN_POINT('Ctrl Pts',(4.34092770662842,-6.87251035812182,
12.2603904851186));
#163154=CARTESIAN_POINT('Ctrl Pts',(4.5381126687349,-6.74392929621897,12.2697862865433));
#163155=CARTESIAN_POINT('Ctrl Pts',(5.090629043771,-6.34842435634939,12.2971340719851));
#163156=CARTESIAN_POINT('Ctrl Pts',(5.43000998420353,-6.0606914236517,12.315251763597));
#163157=CARTESIAN_POINT('Ctrl Pts',(5.85951213597909,-5.63137666391457,
12.3398516028791));
#163158=CARTESIAN_POINT('Ctrl Pts',(5.97136237091782,-5.51263258995273,
12.3464323664701));
#163159=CARTESIAN_POINT('Ctrl Pts',(6.12108115104263,-5.34377855151213,
12.3554625739321));
#163160=CARTESIAN_POINT('Ctrl Pts',(6.16205623417064,-5.29647682188468,
12.357958266947));
#163161=CARTESIAN_POINT('Ctrl Pts',(6.23241039838118,-5.21333816802961,
12.3622839555946));
#163162=CARTESIAN_POINT('Ctrl Pts',(6.2620368721053,-5.17771460055728,12.3641184790684));
#163163=CARTESIAN_POINT('Ctrl Pts',(6.30533136637005,-5.1247411204932,12.3668178522994));
#163164=CARTESIAN_POINT('Ctrl Pts',(6.31923584674851,-5.1075858791526,12.3676876564034));
#163165=CARTESIAN_POINT('Ctrl Pts',(6.34468522661543,-5.07592362634966,
12.3692848753012));
#163166=CARTESIAN_POINT('Ctrl Pts',(6.35625070560465,-5.06143341909078,
12.3700127568318));
#163167=CARTESIAN_POINT('Ctrl Pts',(6.382341256541,-5.02851451560522,12.3716596122835));
#163168=CARTESIAN_POINT('Ctrl Pts',(6.39683631066451,-5.01006221206307,
12.3725779796894));
#163169=CARTESIAN_POINT('Ctrl Pts',(6.43448041616303,-4.96171130944181,
12.374972516524));
#163170=CARTESIAN_POINT('Ctrl Pts',(6.45750109633736,-4.93171338940285,
12.3764463681937));
#163171=CARTESIAN_POINT('Ctrl Pts',(6.63112928979315,-4.70216080404274,
12.3876415538274));
#163172=CARTESIAN_POINT('Ctrl Pts',(6.77266538859039,-4.49590905071219,
12.3972309915625));
#163173=CARTESIAN_POINT('Ctrl Pts',(6.96773722830066,-4.18147452923651,
12.4114560571119));
#163174=CARTESIAN_POINT('Ctrl Pts',(7.02873944284768,-4.07810164525169,
12.4160720620689));
#163175=CARTESIAN_POINT('Ctrl Pts',(7.15011457969925,-3.86160336246185,
12.4256466546382));
#163176=CARTESIAN_POINT('Ctrl Pts',(7.21014471885082,-3.74832386558068,
12.4306058753737));
#163177=CARTESIAN_POINT('Ctrl Pts',(7.28947857508346,-3.5896534274096,12.4375012634681));
#163178=CARTESIAN_POINT('Ctrl Pts',(7.31108720016794,-3.54543559400808,
12.4394174298225));
#163179=CARTESIAN_POINT('Ctrl Pts',(7.34769540319897,-3.46876601457286,
12.4427314809984));
#163180=CARTESIAN_POINT('Ctrl Pts',(7.36288501303784,-3.43640650629159,
12.4441276655105));
#163181=CARTESIAN_POINT('Ctrl Pts',(7.39178592285411,-3.37376545243903,
12.4468257733171));
#163182=CARTESIAN_POINT('Ctrl Pts',(7.40552591923626,-3.34349791512338,
12.4481274148966));
#163183=CARTESIAN_POINT('Ctrl Pts',(7.44176488958444,-3.26234853847497,
12.4516120073448));
#163184=CARTESIAN_POINT('Ctrl Pts',(7.4639276068279,-3.21131862306415,12.4537978337567));
#163185=CARTESIAN_POINT('Ctrl Pts',(7.55328028810477,-2.9996599415525,12.4628432180989));
#163186=CARTESIAN_POINT('Ctrl Pts',(7.61582209448657,-2.8371210124757,12.4697415681784));
#163187=CARTESIAN_POINT('Ctrl Pts',(7.76489656313638,-2.40914095653798,
12.4877789786306));
#163188=CARTESIAN_POINT('Ctrl Pts',(7.84305907362351,-2.14102831124228,
12.4989609756006));
#163189=CARTESIAN_POINT('Ctrl Pts',(7.92042105107633,-1.81380396183036,
12.512346261099));
#163190=CARTESIAN_POINT('Ctrl Pts',(7.93298418642574,-1.75804333802678,
12.5146177882177));
#163191=CARTESIAN_POINT('Ctrl Pts',(7.95865504449285,-1.63822232793874,
12.5194757383592));
#163192=CARTESIAN_POINT('Ctrl Pts',(7.97158001161698,-1.57412665431497,
12.5220602645463));
#163193=CARTESIAN_POINT('Ctrl Pts',(7.98841825203901,-1.48509188440374,
12.5256274314229));
#163194=CARTESIAN_POINT('Ctrl Pts',(7.99299102021141,-1.46028032789587,
12.526619029474));
#163195=CARTESIAN_POINT('Ctrl Pts',(8.00058106963645,-1.41799315544178,
12.5283046120188));
#163196=CARTESIAN_POINT('Ctrl Pts',(8.00365682013918,-1.40052831047807,
12.528999502148));
#163197=CARTESIAN_POINT('Ctrl Pts',(8.01049901803404,-1.3609179431206,12.5305728006465));
#163198=CARTESIAN_POINT('Ctrl Pts',(8.01423085740361,-1.33876657204445,
12.5314507173465));
#163199=CARTESIAN_POINT('Ctrl Pts',(8.02418580735126,-1.27814261285496,
12.5338485135776));
#163200=CARTESIAN_POINT('Ctrl Pts',(8.03022407002165,-1.23964019581819,
12.5353659830407));
#163201=CARTESIAN_POINT('Ctrl Pts',(8.06845771197173,-0.983836286024178,
12.5454166505161));
#163202=CARTESIAN_POINT('Ctrl Pts',(8.09210663306075,-0.765346949249157,
12.5538541972457));
#163203=CARTESIAN_POINT('Ctrl Pts',(8.10736665149593,-0.538839006894385,
12.5625610443669));
#163204=CARTESIAN_POINT('Ctrl Pts',(8.10785037039943,-0.531510929684908,
12.5628426859488));
#163205=CARTESIAN_POINT('Ctrl Pts',(8.11963563174591,-0.349210351509505,
12.5698480294779));
#163206=CARTESIAN_POINT('Ctrl Pts',(8.12528048587414,-0.173918382653126,
12.576560895722));
#163207=CARTESIAN_POINT('Ctrl Pts',(8.12522641224824,0.135823389154046,
12.5884549462431));
#163208=CARTESIAN_POINT('Ctrl Pts',(8.12186803869165,0.270206438898749,
12.5936257863592));
#163209=CARTESIAN_POINT('Ctrl Pts',(8.10741118415194,0.560283777379415,
12.6048397644352));
#163210=CARTESIAN_POINT('Ctrl Pts',(8.09515708609359,0.715866712459239,
12.6108872219502));
#163211=CARTESIAN_POINT('Ctrl Pts',(8.07103413390869,0.939604708174832,
12.6196507742779));
#163212=CARTESIAN_POINT('Ctrl Pts',(8.06276361071442,1.0081130394713,12.622343154546));
#163213=CARTESIAN_POINT('Ctrl Pts',(8.0463755951845,1.13071587734183,12.627178718226));
#163214=CARTESIAN_POINT('Ctrl Pts',(8.03858258780985,1.18484959679853,12.6293198543425));
#163215=CARTESIAN_POINT('Ctrl Pts',(8.02035646582059,1.30298677889777,12.6340061135323));
#163216=CARTESIAN_POINT('Ctrl Pts',(8.00970246524742,1.36695236380762,12.636552271451));
#163217=CARTESIAN_POINT('Ctrl Pts',(7.9853252457818,1.50322450858034,12.6419954437753));
#163218=CARTESIAN_POINT('Ctrl Pts',(7.97138299263149,1.57548606664267,12.6448932154794));
#163219=CARTESIAN_POINT('Ctrl Pts',(7.92510995838367,1.79895122553601,12.653888771948));
#163220=CARTESIAN_POINT('Ctrl Pts',(7.88944369472393,1.94942848893371,12.659995758361));
#163221=CARTESIAN_POINT('Ctrl Pts',(7.820432934825,2.20752902130431,12.6705405833494));
#163222=CARTESIAN_POINT('Ctrl Pts',(7.78910373554606,2.31564651979451,12.6749792416968));
#163223=CARTESIAN_POINT('Ctrl Pts',(7.74231925136006,2.46538945028468,12.6811482070504));
#163224=CARTESIAN_POINT('Ctrl Pts',(7.72875389267594,2.507591636382,12.6828891870632));
#163225=CARTESIAN_POINT('Ctrl Pts',(7.70093454293506,2.5917676400348,12.6863655488141));
#163226=CARTESIAN_POINT('Ctrl Pts',(7.6866810535198,2.63374006556882,12.6881008722784));
#163227=CARTESIAN_POINT('Ctrl Pts',(7.62927067352579,2.79836045644615,12.6949181143822));
#163228=CARTESIAN_POINT('Ctrl Pts',(7.5835158515422,2.92008215772154,12.6999834793816));
#163229=CARTESIAN_POINT('Ctrl Pts',(7.45466117616743,3.23938912228191,12.7133915839555));
#163230=CARTESIAN_POINT('Ctrl Pts',(7.36663157493395,3.43487321047026,12.7217264267388));
#163231=CARTESIAN_POINT('Ctrl Pts',(7.24253407197357,3.68367326433715,12.7325923283225));
#163232=CARTESIAN_POINT('Ctrl Pts',(7.21342082468294,3.74036207792905,12.7350858325704));
#163233=CARTESIAN_POINT('Ctrl Pts',(7.15803331728252,3.84515936778576,12.7397311063965));
#163234=CARTESIAN_POINT('Ctrl Pts',(7.13193324719649,3.89335583621992,12.7418817495222));
#163235=CARTESIAN_POINT('Ctrl Pts',(7.07054271093535,4.00403069526038,12.7468551348575));
#163236=CARTESIAN_POINT('Ctrl Pts',(7.03490830119401,4.06631296981573,12.749679898323));
#163237=CARTESIAN_POINT('Ctrl Pts',(6.90569743345405,4.2853660497278,12.7597122306441));
#163238=CARTESIAN_POINT('Ctrl Pts',(6.8076682124996,4.43944498129916,12.7669491890796));
#163239=CARTESIAN_POINT('Ctrl Pts',(6.5213797708074,4.85761335604164,12.7871282773802));
#163240=CARTESIAN_POINT('Ctrl Pts',(6.32237899041786,5.11393424234623,12.8001312462778));
#163241=CARTESIAN_POINT('Ctrl Pts',(6.10601221395583,5.36062662406682,12.8132451629552));
#163242=CARTESIAN_POINT('Ctrl Pts',(6.10342270025719,5.363574768904,12.8134019727042));
#163243=CARTESIAN_POINT('Ctrl Pts',(5.98322556172651,5.50021868215928,12.8206741013764));
#163244=CARTESIAN_POINT('Ctrl Pts',(5.86125578380425,5.63001558501365,12.8277665808182));
#163245=CARTESIAN_POINT('Ctrl Pts',(5.70797719928455,5.78274605810582,12.8363063478163));
#163246=CARTESIAN_POINT('Ctrl Pts',(5.68064413497349,5.80959877378475,12.8378153842299));
#163247=CARTESIAN_POINT('Ctrl Pts',(5.63708802386881,5.85178814322042,12.8401978025678));
#163248=CARTESIAN_POINT('Ctrl Pts',(5.62099001452248,5.86725294521716,12.8410735806017));
#163249=CARTESIAN_POINT('Ctrl Pts',(5.59197786867657,5.89489492048746,12.8426432995449));
#163250=CARTESIAN_POINT('Ctrl Pts',(5.57908718359271,5.90709647861592,12.8433377316474));
#163251=CARTESIAN_POINT('Ctrl Pts',(5.54756603271848,5.93673731017992,12.8450283510913));
#163252=CARTESIAN_POINT('Ctrl Pts',(5.52889320415729,5.95413123113358,12.8460235201225));
#163253=CARTESIAN_POINT('Ctrl Pts',(5.46051063987603,6.01723118837448,12.8496457863755));
#163254=CARTESIAN_POINT('Ctrl Pts',(5.41031330004677,6.06240527570437,12.8522624192402));
#163255=CARTESIAN_POINT('Ctrl Pts',(5.27619003327776,6.18011405732958,12.8591547037826));
#163256=CARTESIAN_POINT('Ctrl Pts',(5.19133168771568,6.25156513372939,12.8634153933824));
#163257=CARTESIAN_POINT('Ctrl Pts',(4.81391014043049,6.55637016173753,12.8820118466904));
#163258=CARTESIAN_POINT('Ctrl Pts',(4.50689160434748,6.77108906724472,12.8962618687067));
#163259=CARTESIAN_POINT('Ctrl Pts',(4.1286791668259,6.99844236261406,12.9133565198978));
#163260=CARTESIAN_POINT('Ctrl Pts',(4.07076238092081,7.03228844221481,12.9159613342482));
#163261=CARTESIAN_POINT('Ctrl Pts',(3.97829228913194,7.0848020126076,12.9201018620056));
#163262=CARTESIAN_POINT('Ctrl Pts',(3.94401120632091,7.10394289712026,12.9216329242276));
#163263=CARTESIAN_POINT('Ctrl Pts',(3.88178116706388,7.13809982075457,12.9244055000265));
#163264=CARTESIAN_POINT('Ctrl Pts',(3.85388040109641,7.15320207504099,12.9256461548602));
#163265=CARTESIAN_POINT('Ctrl Pts',(3.78721485060061,7.18878385432034,12.9286049810804));
#163266=CARTESIAN_POINT('Ctrl Pts',(3.74837140701687,7.20911377380686,12.9303245258839));
#163267=CARTESIAN_POINT('Ctrl Pts',(3.62786248225703,7.2709485653715,12.9356460555939));
#163268=CARTESIAN_POINT('Ctrl Pts',(3.54565856797332,7.3113873087351,12.939257552339));
#163269=CARTESIAN_POINT('Ctrl Pts',(3.34521591942216,7.40581591237887,12.948019966004));
#163270=CARTESIAN_POINT('Ctrl Pts',(3.22633159949039,7.45837535378336,12.9531811865184));
#163271=CARTESIAN_POINT('Ctrl Pts',(2.97358353615235,7.56294241038155,12.9640708603669));
#163272=CARTESIAN_POINT('Ctrl Pts',(2.83949751547102,7.61429909300117,12.9698004062699));
#163273=CARTESIAN_POINT('Ctrl Pts',(2.55189027818813,7.71580225734242,12.9819613538924));
#163274=CARTESIAN_POINT('Ctrl Pts',(2.39809040965023,7.76497981508553,12.988388873169));
#163275=CARTESIAN_POINT('Ctrl Pts',(2.21029081637543,7.81891648814228,12.9961084248972));
#163276=CARTESIAN_POINT('Ctrl Pts',(2.17759608140437,7.82808506987927,12.9974476363544));
#163277=CARTESIAN_POINT('Ctrl Pts',(2.12701176194575,7.84192899495319,12.9995117913366));
#163278=CARTESIAN_POINT('Ctrl Pts',(2.10916214084377,7.84674865555616,13.0002386655092));
#163279=CARTESIAN_POINT('Ctrl Pts',(2.07516901176752,7.8558029298737,13.0016199651753));
#163280=CARTESIAN_POINT('Ctrl Pts',(2.05902860106362,7.86004881172323,13.0022745537269));
#163281=CARTESIAN_POINT('Ctrl Pts',(2.01957599720585,7.87029731570946,13.0038713705553));
#163282=CARTESIAN_POINT('Ctrl Pts',(1.99624996112023,7.87624613282752,13.0048127409227));
#163283=CARTESIAN_POINT('Ctrl Pts',(1.91697599265494,7.89608851115254,13.0080032020417));
#163284=CARTESIAN_POINT('Ctrl Pts',(1.86090652234849,7.90949035783482,13.0102449219928));
#163285=CARTESIAN_POINT('Ctrl Pts',(1.72335358951067,7.94082491959504,13.0157127795035));
#163286=CARTESIAN_POINT('Ctrl Pts',(1.6417271886123,7.9581015331882,13.0189304841876));
#163287=CARTESIAN_POINT('Ctrl Pts',(1.16626462801893,8.05110864238313,13.0375488955238));
#163288=CARTESIAN_POINT('Ctrl Pts',(0.767516496533518,8.09885474919749,
13.0526844958605));
#163289=CARTESIAN_POINT('Ctrl Pts',(-0.0243256322105377,8.13464477912087,
13.0828320313359));
#163290=CARTESIAN_POINT('Ctrl Pts',(-0.416285256848256,8.12402210800684,
13.0978017719164));
#163291=CARTESIAN_POINT('Ctrl Pts',(-0.878679891243662,8.07792996870312,
13.1158512736093));
#163292=CARTESIAN_POINT('Ctrl Pts',(-0.951316316782368,8.06969814280534,
13.1186975124839));
#163293=CARTESIAN_POINT('Ctrl Pts',(-1.06639269489724,8.05508130715052,
13.1232255901971));
#163294=CARTESIAN_POINT('Ctrl Pts',(-1.10891032474857,8.0493382411396,13.1249026847915));
#163295=CARTESIAN_POINT('Ctrl Pts',(-1.18853383091524,8.03794025607925,
13.1280513735352));
#163296=CARTESIAN_POINT('Ctrl Pts',(-1.22564991694263,8.03236444007877,
13.1295223727827));
#163297=CARTESIAN_POINT('Ctrl Pts',(-1.30910066704185,8.01923605120664,
13.1328372422107));
#163298=CARTESIAN_POINT('Ctrl Pts',(-1.35541116447638,8.01153867600735,
13.1346820409557));
#163299=CARTESIAN_POINT('Ctrl Pts',(-1.49612430276273,7.98689541309926,
13.1403037168932));
#163300=CARTESIAN_POINT('Ctrl Pts',(-1.59029561554957,7.96867906091219,
13.1440884340889));
#163301=CARTESIAN_POINT('Ctrl Pts',(-2.07638046892051,7.86569167020248,
13.1637430540058));
#163302=CARTESIAN_POINT('Ctrl Pts',(-2.46194117266534,7.7536634151502,13.1796706999063));
#163303=CARTESIAN_POINT('Ctrl Pts',(-3.37548708643007,7.41317937668523,
13.219369094247));
#163304=CARTESIAN_POINT('Ctrl Pts',(-3.89055131671592,7.15630364767962,
13.2436235605803));
#163305=CARTESIAN_POINT('Ctrl Pts',(-4.6817238195332,6.65088776830117,13.2833193094023));
#163306=CARTESIAN_POINT('Ctrl Pts',(-4.97567075385715,6.43393864775923,
13.2986554155622));
#163307=CARTESIAN_POINT('Ctrl Pts',(-5.271039703248,6.18355273141817,13.31405987864));
#163308=CARTESIAN_POINT('Ctrl Pts',(-5.28797527843433,6.16907621948654,
13.3149429953921));
#163309=CARTESIAN_POINT('Ctrl Pts',(-5.31157585719797,6.14873387727936,
13.3161732273468));
#163310=CARTESIAN_POINT('Ctrl Pts',(-5.31829103236338,6.14292657258945,
13.3165232208836));
#163311=CARTESIAN_POINT('Ctrl Pts',(-5.33054637658521,6.13229295416775,
13.3171618545407));
#163312=CARTESIAN_POINT('Ctrl Pts',(-5.3360895382101,6.12747011329402,13.3174506699977));
#163313=CARTESIAN_POINT('Ctrl Pts',(-5.34726691166493,6.11771854323587,
13.3180329461882));
#163314=CARTESIAN_POINT('Ctrl Pts',(-5.35290087026406,6.11278953281106,
13.3183263918714));
#163315=CARTESIAN_POINT('Ctrl Pts',(-5.36667910793966,6.1007016394232,13.3190438917053));
#163316=CARTESIAN_POINT('Ctrl Pts',(-5.37481589761371,6.09353421333666,
13.3194674920889));
#163317=CARTESIAN_POINT('Ctrl Pts',(-5.40403519183322,6.06769185358593,
13.3209881278449));
#163318=CARTESIAN_POINT('Ctrl Pts',(-5.42503507162761,6.04892348136956,
13.3220800358314));
#163319=CARTESIAN_POINT('Ctrl Pts',(-5.47489135842505,6.00389659496003,
13.3246691023441));
#163320=CARTESIAN_POINT('Ctrl Pts',(-5.50365661898026,5.97753909517631,
13.3261600399065));
#163321=CARTESIAN_POINT('Ctrl Pts',(-5.61319005240674,5.87571301501655,
13.3318254670337));
#163322=CARTESIAN_POINT('Ctrl Pts',(-5.69260618936603,5.7988052445606,13.3359105932849));
#163323=CARTESIAN_POINT('Ctrl Pts',(-5.84121769827905,5.64889132300337,
13.3435581474931));
#163324=CARTESIAN_POINT('Ctrl Pts',(-5.91067464328007,5.57617462807115,
13.3471337754295));
#163325=CARTESIAN_POINT('Ctrl Pts',(-6.34754353353314,5.10146574407053,
13.3697503737428));
#163326=CARTESIAN_POINT('Ctrl Pts',(-6.6751135739383,4.66467236324227,13.3873648446608));
#163327=CARTESIAN_POINT('Ctrl Pts',(-7.23816479058777,3.73172183817601,
13.4241844453894));
#163328=CARTESIAN_POINT('Ctrl Pts',(-7.47210109343363,3.23796257742278,
13.4433330854693));
#163329=CARTESIAN_POINT('Ctrl Pts',(-7.66589678109804,2.69347372518248,
13.4655461536033));
#163330=CARTESIAN_POINT('Ctrl Pts',(-7.67676087554533,2.66235170405505,
13.466819014893));
#163331=CARTESIAN_POINT('Ctrl Pts',(-7.69155799754245,2.61911916946679,
13.4685917905977));
#163332=CARTESIAN_POINT('Ctrl Pts',(-7.6956524539559,2.60706404976685,13.469086612322));
#163333=CARTESIAN_POINT('Ctrl Pts',(-7.70264339496538,2.58632097044656,
13.4699389058854));
#163334=CARTESIAN_POINT('Ctrl Pts',(-7.70555356083715,2.57763763018865,
13.4702959465569));
#163335=CARTESIAN_POINT('Ctrl Pts',(-7.71151842262826,2.55973932786888,
13.4710324245912));
#163336=CARTESIAN_POINT('Ctrl Pts',(-7.7145712958446,2.55052377556824,13.4714119185104));
#163337=CARTESIAN_POINT('Ctrl Pts',(-7.72162018532796,2.52911721060339,
13.4722941208803));
#163338=CARTESIAN_POINT('Ctrl Pts',(-7.72560385391594,2.51692217638347,
13.4727972154702));
#163339=CARTESIAN_POINT('Ctrl Pts',(-7.73813365574603,2.47825521040637,
13.4743940346073));
#163340=CARTESIAN_POINT('Ctrl Pts',(-7.74657269533374,2.45174893072979,
13.4754911045726));
#163341=CARTESIAN_POINT('Ctrl Pts',(-7.89106858409783,1.9897055463641,13.4946580149614));
#163342=CARTESIAN_POINT('Ctrl Pts',(-7.99032050392628,1.54356395549976,
13.5138974622575));
#163343=CARTESIAN_POINT('Ctrl Pts',(-8.13590801593221,0.469610143936951,
13.561464420844));
#163344=CARTESIAN_POINT('Ctrl Pts',(-8.14787814512287,-0.159913341030507,
13.5903960898329));
#163345=CARTESIAN_POINT('Ctrl Pts',(-8.06448285092655,-1.01960194796715,
13.6277739166654));
#163346=CARTESIAN_POINT('Ctrl Pts',(-8.03143646325101,-1.25360759790878,
13.6376928214678));
#163347=CARTESIAN_POINT('Ctrl Pts',(-7.9843266000613,-1.50687505773135,
13.6479782746439));
#163348=CARTESIAN_POINT('Ctrl Pts',(-7.98033816120067,-1.52785684564516,
13.6488274191142));
#163349=CARTESIAN_POINT('Ctrl Pts',(-7.97439042339924,-1.55848704097327,
13.6500630086645));
#163350=CARTESIAN_POINT('Ctrl Pts',(-7.97249626333242,-1.568147892881,13.6504521304163));
#163351=CARTESIAN_POINT('Ctrl Pts',(-7.96911149429858,-1.58524669946106,
13.6511398331978));
#163352=CARTESIAN_POINT('Ctrl Pts',(-7.96762802074529,-1.59268604258533,
13.6514387010863));
#163353=CARTESIAN_POINT('Ctrl Pts',(-7.96452861838806,-1.60811626267442,
13.652057911054));
#163354=CARTESIAN_POINT('Ctrl Pts',(-7.96291107627683,-1.61610680937648,
13.6523781888274));
#163355=CARTESIAN_POINT('Ctrl Pts',(-7.95897655298582,-1.63539376545993,
13.6531503567509));
#163356=CARTESIAN_POINT('Ctrl Pts',(-7.95664754097391,-1.64668772068941,
13.6536017782278));
#163357=CARTESIAN_POINT('Ctrl Pts',(-7.94724951612034,-1.69177560196719,
13.6554011076346));
#163358=CARTESIAN_POINT('Ctrl Pts',(-7.93998913030676,-1.72552954523484,
13.6567417524963));
#163359=CARTESIAN_POINT('Ctrl Pts',(-7.85045011729405,-2.12926688375388,
13.6727103171344));
#163360=CARTESIAN_POINT('Ctrl Pts',(-7.74259037580817,-2.49312490423682,
13.686446536905));
#163361=CARTESIAN_POINT('Ctrl Pts',(-7.51812037466152,-3.09286863595076,
13.7094869402501));
#163362=CARTESIAN_POINT('Ctrl Pts',(-7.41477146620844,-3.33303679540352,
13.7188240421466));
#163363=CARTESIAN_POINT('Ctrl Pts',(-7.22080962029552,-3.72989888120363,
13.734797834149));
#163364=CARTESIAN_POINT('Ctrl Pts',(-7.1362134658379,-3.88930494587637,
13.7413695874925));
#163365=CARTESIAN_POINT('Ctrl Pts',(-6.89634112509056,-4.30708354358129,
13.7591388010169));
#163366=CARTESIAN_POINT('Ctrl Pts',(-6.73188462752959,-4.55984736301125,
13.77047879151));
#163367=CARTESIAN_POINT('Ctrl Pts',(-6.52640603715794,-4.84023301346545,
13.7838664348178));
#163368=CARTESIAN_POINT('Ctrl Pts',(-6.49871836672879,-4.87734466039689,
13.7856553234286));
#163369=CARTESIAN_POINT('Ctrl Pts',(-6.45364850054224,-4.93668966660062,
13.788543322045));
#163370=CARTESIAN_POINT('Ctrl Pts',(-6.43646496279797,-4.95907275675567,
13.7896389474758));
#163371=CARTESIAN_POINT('Ctrl Pts',(-6.40562921220849,-4.99880880204938,
13.7915953392448));
#163372=CARTESIAN_POINT('Ctrl Pts',(-6.39202218135125,-5.01619651448734,
13.7924553334493));
#163373=CARTESIAN_POINT('Ctrl Pts',(-6.3640932228792,-5.05158729831142,
13.7942137650788));
#163374=CARTESIAN_POINT('Ctrl Pts',(-6.34976535078684,-5.06958546305727,
13.795112306174));
#163375=CARTESIAN_POINT('Ctrl Pts',(-6.31488382093588,-5.11302253745017,
13.7972914658354));
#163376=CARTESIAN_POINT('Ctrl Pts',(-6.2942526715158,-5.13839862539558,
13.7985734205575));
#163377=CARTESIAN_POINT('Ctrl Pts',(-6.24979673645968,-5.19240944362112,
13.8013215170356));
#163378=CARTESIAN_POINT('Ctrl Pts',(-6.22592713022495,-5.22100626552055,
13.802788463463));
#163379=CARTESIAN_POINT('Ctrl Pts',(-6.15891938904798,-5.30017145713959,
13.8068836613977));
#163380=CARTESIAN_POINT('Ctrl Pts',(-6.11535637965859,-5.35037584988356,
13.8095201028655));
#163381=CARTESIAN_POINT('Ctrl Pts',(-5.60167378669033,-5.92790138346935,
13.8403273616097));
#163382=CARTESIAN_POINT('Ctrl Pts',(-5.06535293188475,-6.39224516803299,
13.870189554341));
#163383=CARTESIAN_POINT('Ctrl Pts',(-4.1731431339223,-6.98112513724939,
13.9154807261136));
#163384=CARTESIAN_POINT('Ctrl Pts',(-3.85739039063744,-7.16043244712547,
13.9307341555609));
#163385=CARTESIAN_POINT('Ctrl Pts',(-3.50968662207309,-7.32818749529782,
13.9461324872889));
#163386=CARTESIAN_POINT('Ctrl Pts',(-3.48862483465983,-7.33823745373713,
13.9470598791207));
#163387=CARTESIAN_POINT('Ctrl Pts',(-3.4591168882185,-7.35216187597435,
13.9483514514342));
#163388=CARTESIAN_POINT('Ctrl Pts',(-3.4507070411492,-7.35611275157657,
13.9487186795228));
#163389=CARTESIAN_POINT('Ctrl Pts',(-3.43532726855884,-7.36330586161073,
13.9493886424841));
#163390=CARTESIAN_POINT('Ctrl Pts',(-3.42835948964244,-7.36655264448757,
13.9496915628579));
#163391=CARTESIAN_POINT('Ctrl Pts',(-3.41428626500377,-7.37308606704384,
13.9503021541476));
#163392=CARTESIAN_POINT('Ctrl Pts',(-3.40718065477388,-7.37637233589074,
13.9506098094754));
#163393=CARTESIAN_POINT('Ctrl Pts',(-3.39077061745227,-7.38393303225723,
13.9513188446949));
#163394=CARTESIAN_POINT('Ctrl Pts',(-3.38146282629712,-7.38820015704858,
13.9517199149312));
#163395=CARTESIAN_POINT('Ctrl Pts',(-3.34941098096333,-7.40282095767582,
13.9530971989544));
#163396=CARTESIAN_POINT('Ctrl Pts',(-3.32662710202135,-7.41308735905932,
13.9540696240554));
#163397=CARTESIAN_POINT('Ctrl Pts',(-3.04938497800849,-7.53647692759427,
13.9658194137989));
#163398=CARTESIAN_POINT('Ctrl Pts',(-2.78932587080811,-7.63654979001016,
13.9759205824542));
#163399=CARTESIAN_POINT('Ctrl Pts',(-2.24623522085326,-7.81408395708418,
13.9959170691738));
#163400=CARTESIAN_POINT('Ctrl Pts',(-1.96310325567743,-7.88997562693376,
14.0057762624287));
#163401=CARTESIAN_POINT('Ctrl Pts',(-1.05389143425787,-8.0816990929973,
14.0370185658688));
#163402=CARTESIAN_POINT('Ctrl Pts',(-0.418044759607934,-8.1393936853567,
14.0584267287375));
#163403=CARTESIAN_POINT('Ctrl Pts',(0.332034642464033,-8.11926481577325,
14.0864905474198));
#163404=CARTESIAN_POINT('Ctrl Pts',(0.446021357419688,-8.11380132263703,
14.0908253368615));
#163405=CARTESIAN_POINT('Ctrl Pts',(0.580351035453153,-8.10452357779809,
14.0960250643709));
#163406=CARTESIAN_POINT('Ctrl Pts',(0.600843807705472,-8.10303007885709,
14.0968208180633));
#163407=CARTESIAN_POINT('Ctrl Pts',(0.633771616807793,-8.10050472435891,
14.0981035155635));
#163408=CARTESIAN_POINT('Ctrl Pts',(0.64621037939032,-8.09952192388845,
14.098589001801));
#163409=CARTESIAN_POINT('Ctrl Pts',(0.668302200619706,-8.09772520987412,
14.0994529232982));
#163410=CARTESIAN_POINT('Ctrl Pts',(0.677956173038525,-8.09692267671162,
14.0998310195746));
#163411=CARTESIAN_POINT('Ctrl Pts',(0.698054440783082,-8.09521571432498,
14.1006193552372));
#163412=CARTESIAN_POINT('Ctrl Pts',(0.708498463867401,-8.09430833298691,
14.1010296817812));
#163413=CARTESIAN_POINT('Ctrl Pts',(0.735531870432197,-8.09190693655351,
14.1020935176946));
#163414=CARTESIAN_POINT('Ctrl Pts',(0.752118431179804,-8.09038212099813,
14.1027479425286));
#163415=CARTESIAN_POINT('Ctrl Pts',(0.822228055981327,-8.08371942252818,
14.1055213714936));
#163416=CARTESIAN_POINT('Ctrl Pts',(0.87570352049668,-8.07810137887934,
14.1076546511089));
#163417=CARTESIAN_POINT('Ctrl Pts',(1.24022518812339,-8.03614326948219,
14.1223208471738));
#163418=CARTESIAN_POINT('Ctrl Pts',(1.54897642954337,-7.98238078572129,
14.135376048327));
#163419=CARTESIAN_POINT('Ctrl Pts',(2.18728447981832,-7.83280074373423,
14.1636382699979));
#163420=CARTESIAN_POINT('Ctrl Pts',(2.51544151354283,-7.73366100248514,
14.1789059796341));
#163421=CARTESIAN_POINT('Ctrl Pts',(3.05109891142204,-7.53412241829739,
14.2046454737515));
#163422=CARTESIAN_POINT('Ctrl Pts',(3.26236994671229,-7.44507543081946,
14.2150168142248));
#163423=CARTESIAN_POINT('Ctrl Pts',(3.85611953556844,-7.16468759245913,
14.2444354636741));
#163424=CARTESIAN_POINT('Ctrl Pts',(4.22770209726597,-6.95191043031932,
14.2631858947543));
#163425=CARTESIAN_POINT('Ctrl Pts',(4.60406820829356,-6.69500059460983,
14.2814260489235));
#163426=CARTESIAN_POINT('Ctrl Pts',(4.62719245635694,-6.67903937922231,
14.2825440338913));
#163427=CARTESIAN_POINT('Ctrl Pts',(4.65847882429817,-6.65720389526688,
14.2840536065798));
#163428=CARTESIAN_POINT('Ctrl Pts',(4.6667133330728,-6.6514340805399,14.2844506366657));
#163429=CARTESIAN_POINT('Ctrl Pts',(4.68065410986139,-6.64162732497241,
14.2851223480283));
#163430=CARTESIAN_POINT('Ctrl Pts',(4.68636590397448,-6.63759828812231,
14.2853974325158));
#163431=CARTESIAN_POINT('Ctrl Pts',(4.6973584469272,-6.62982300698355,14.2859266092858));
#163432=CARTESIAN_POINT('Ctrl Pts',(4.70263992857332,-6.62607781310718,
14.2861807540156));
#163433=CARTESIAN_POINT('Ctrl Pts',(4.71509489543437,-6.61722337936885,
14.2867798553238));
#163434=CARTESIAN_POINT('Ctrl Pts',(4.72226456996205,-6.61210877538087,
14.287124545213));
#163435=CARTESIAN_POINT('Ctrl Pts',(4.74315948847447,-6.59715172512569,
14.2881286037214));
#163436=CARTESIAN_POINT('Ctrl Pts',(4.75686242450724,-6.58727809471519,
14.2887864526372));
#163437=CARTESIAN_POINT('Ctrl Pts',(4.85526228792436,-6.51590906199142,
14.2935067227391));
#163438=CARTESIAN_POINT('Ctrl Pts',(4.93879690337251,-6.45282333609843,
14.2974942624056));
#163439=CARTESIAN_POINT('Ctrl Pts',(5.31333347994523,-6.15843681109112,
14.3153886311979));
#163440=CARTESIAN_POINT('Ctrl Pts',(5.58948205134802,-5.90893994422799,
14.3286539555681));
#163441=CARTESIAN_POINT('Ctrl Pts',(6.06029308553835,-5.42092168292343,
14.3529351721314));
#163442=CARTESIAN_POINT('Ctrl Pts',(6.26035707750009,-5.18859035543701,
14.3639118186475));
#163443=CARTESIAN_POINT('Ctrl Pts',(6.72256391815325,-4.58607210050807,
14.391673525633));
#163444=CARTESIAN_POINT('Ctrl Pts',(6.96774721820448,-4.20421096007589,
14.4087209982007));
#163445=CARTESIAN_POINT('Ctrl Pts',(7.26203408503647,-3.64875137428103,
14.432884768104));
#163446=CARTESIAN_POINT('Ctrl Pts',(7.33919405593078,-3.49095336930485,
14.4396670969788));
#163447=CARTESIAN_POINT('Ctrl Pts',(7.4358103804484,-3.2759764516292,14.4488321095968));
#163448=CARTESIAN_POINT('Ctrl Pts',(7.45983210649493,-3.22090090167561,
14.451173687549));
#163449=CARTESIAN_POINT('Ctrl Pts',(7.49716967973637,-3.13263668391524,
14.4549174866989));
#163450=CARTESIAN_POINT('Ctrl Pts',(7.51088117621391,-3.09961767738581,
14.4563160642541));
#163451=CARTESIAN_POINT('Ctrl Pts',(7.53874294288063,-3.03125253053726,
14.4592081124436));
#163452=CARTESIAN_POINT('Ctrl Pts',(7.55286360259231,-2.99589526682532,
14.4607018158985));
#163453=CARTESIAN_POINT('Ctrl Pts',(7.58029613157925,-2.92577911101131,
14.4636603307241));
#163454=CARTESIAN_POINT('Ctrl Pts',(7.59361870678652,-2.89102538417816,
14.4651250048073));
#163455=CARTESIAN_POINT('Ctrl Pts',(7.62404083724737,-2.8100038923447,14.4685359180104));
#163456=CARTESIAN_POINT('Ctrl Pts',(7.64095877724817,-2.76366957094366,
14.4704837649845));
#163457=CARTESIAN_POINT('Ctrl Pts',(7.68407490465732,-2.64216152334515,
14.4755854009179));
#163458=CARTESIAN_POINT('Ctrl Pts',(7.70959198382766,-2.56675202821044,
14.478745170077));
#163459=CARTESIAN_POINT('Ctrl Pts',(7.78346298305599,-2.33739730368214,
14.4883392099087));
#163460=CARTESIAN_POINT('Ctrl Pts',(7.82834298630422,-2.18237652997822,
14.494802270924));
#163461=CARTESIAN_POINT('Ctrl Pts',(7.94553954914191,-1.72723645234392,
14.5137247948711));
#163462=CARTESIAN_POINT('Ctrl Pts',(8.00540878376709,-1.42420903210038,
14.5262623520816));
#163463=CARTESIAN_POINT('Ctrl Pts',(8.08845226859735,-0.826698105907153,
14.5507795449631));
#163464=CARTESIAN_POINT('Ctrl Pts',(8.11310822517487,-0.532887231041014,
14.5627392502568));
#163465=CARTESIAN_POINT('Ctrl Pts',(8.12405742833518,-0.159848937730708,
14.5776698109421));
#163466=CARTESIAN_POINT('Ctrl Pts',(8.12522331385657,-0.0812833074808247,
14.5807997949565));
#163467=CARTESIAN_POINT('Ctrl Pts',(8.12524954711001,-0.00271287458686051,
14.5839128245719));
#163468=CARTESIAN_POINT('',(8.1269655491554,-0.00168838483458986,16.5832974432124));
#163469=CARTESIAN_POINT('Ctrl Pts',(8.12631724021387,-0.0026888491199863,
14.5832974432124));
#163470=CARTESIAN_POINT('Ctrl Pts',(8.12636183407428,0.0449434531170251,
14.5851677846816));
#163471=CARTESIAN_POINT('Ctrl Pts',(8.11510270816418,1.43976685797085,14.6399272812462));
#163472=CARTESIAN_POINT('Ctrl Pts',(7.36660492052285,4.18569279410474,14.7475759329063));
#163473=CARTESIAN_POINT('Ctrl Pts',(4.46947152341234,7.18896984766691,14.9062433981928));
#163474=CARTESIAN_POINT('Ctrl Pts',(0.494311211965678,8.45828284271795,
15.0649108634792));
#163475=CARTESIAN_POINT('Ctrl Pts',(-3.62342745787823,7.65690432669853,
15.2235783287656));
#163476=CARTESIAN_POINT('Ctrl Pts',(-6.81611969460216,5.00581298154595,
15.382245794052));
#163477=CARTESIAN_POINT('Ctrl Pts',(-8.96101480030011,-0.17955105281227,
15.593802414434));
#163478=CARTESIAN_POINT('Ctrl Pts',(-6.78077229295221,-5.84776877811949,
15.8053590348158));
#163479=CARTESIAN_POINT('Ctrl Pts',(-1.74999298391495,-8.26945455504393,
16.0169156551978));
#163480=CARTESIAN_POINT('Ctrl Pts',(3.83053466397949,-8.09334768555441,
16.2284722755797));
#163481=CARTESIAN_POINT('Ctrl Pts',(7.65853128092144,-4.25683691476263,
16.4172662049179));
#163482=CARTESIAN_POINT('Ctrl Pts',(8.13065759321727,-0.773914348631322,
16.5531709791606));
#163483=CARTESIAN_POINT('Ctrl Pts',(8.1269655491554,-0.00168838483458986,
16.5832974432124));
#163484=CARTESIAN_POINT('',(8.12524999728007,-0.000210238467608934,18.5832974432342));
#163485=CARTESIAN_POINT('Ctrl Pts',(8.12524982465525,-0.00168802839118938,
16.5832974432124));
#163486=CARTESIAN_POINT('Ctrl Pts',(8.12528831832782,0.183599557962629,
16.5905275087158));
#163487=CARTESIAN_POINT('Ctrl Pts',(8.11898455471787,0.368960515185087,
16.5977575742192));
#163488=CARTESIAN_POINT('Ctrl Pts',(8.10634970717896,0.553879036811779,
16.6049876397226));
#163489=CARTESIAN_POINT('Ctrl Pts',(8.093715609276,0.738786587069809,16.6122172762602));
#163490=CARTESIAN_POINT('Ctrl Pts',(8.07475120840512,0.923251363949085,
16.6194469127978));
#163491=CARTESIAN_POINT('Ctrl Pts',(8.04951964886878,1.10676148513372,16.6266765493355));
#163492=CARTESIAN_POINT('Ctrl Pts',(8.02427989708313,1.29033118886856,16.6339085332105));
#163493=CARTESIAN_POINT('Ctrl Pts',(7.99276898989149,1.47294523245479,16.6411405170856));
#163494=CARTESIAN_POINT('Ctrl Pts',(7.95510137049552,1.65410088798726,16.6483725009607));
#163495=CARTESIAN_POINT('Ctrl Pts',(7.9495230652595,1.68092874591926,16.6494435060883));
#163496=CARTESIAN_POINT('Ctrl Pts',(7.94380982437166,1.70772464251782,16.6505145112159));
#163497=CARTESIAN_POINT('Ctrl Pts',(7.93796211318075,1.73448697089573,16.6515855163435));
#163498=CARTESIAN_POINT('Ctrl Pts',(7.88715201736832,1.96702179087069,16.6608913577867));
#163499=CARTESIAN_POINT('Ctrl Pts',(7.82618932688376,2.1970058040725,16.67019719923));
#163500=CARTESIAN_POINT('Ctrl Pts',(7.75535875541403,2.42365388150265,16.6795030406732));
#163501=CARTESIAN_POINT('Ctrl Pts',(7.68414790889602,2.65151878673472,16.6888588433017));
#163502=CARTESIAN_POINT('Ctrl Pts',(7.60296300456688,2.87601181259765,16.6982146459302));
#163503=CARTESIAN_POINT('Ctrl Pts',(7.51213915957558,3.09636122079952,16.7075704485587));
#163504=CARTESIAN_POINT('Ctrl Pts',(7.42087441429973,3.31778030532687,16.7169716685117));
#163505=CARTESIAN_POINT('Ctrl Pts',(7.31987695578548,3.53501541466431,16.7263728884648));
#163506=CARTESIAN_POINT('Ctrl Pts',(7.20953213564697,3.74731022836029,16.7357741084178));
#163507=CARTESIAN_POINT('Ctrl Pts',(7.0990678896688,3.9598348080421,16.7451855032805));
#163508=CARTESIAN_POINT('Ctrl Pts',(6.97923607346948,4.16740836932671,16.7545968981433));
#163509=CARTESIAN_POINT('Ctrl Pts',(6.85046801357916,4.36929920667248,16.7640082930061));
#163510=CARTESIAN_POINT('Ctrl Pts',(6.72185100078244,4.57095322268047,16.7734086481448));
#163511=CARTESIAN_POINT('Ctrl Pts',(6.58431871991006,4.76693781038664,16.7828090032836));
#163512=CARTESIAN_POINT('Ctrl Pts',(6.43834511216219,4.9565511980809,16.7922093584224));
#163513=CARTESIAN_POINT('Ctrl Pts',(6.34494818769979,5.07786975367987,16.7982238994916));
#163514=CARTESIAN_POINT('Ctrl Pts',(6.24809651951929,5.19658067909184,16.8042384405607));
#163515=CARTESIAN_POINT('Ctrl Pts',(6.14792370588667,5.31250615708789,16.8102529816299));
#163516=CARTESIAN_POINT('Ctrl Pts',(6.01897491033632,5.46173278075059,16.8179952801492));
#163517=CARTESIAN_POINT('Ctrl Pts',(5.88445987714346,5.60641184966154,16.8257375786684));
#163518=CARTESIAN_POINT('Ctrl Pts',(5.7447395344376,5.74609913280041,16.8334798771877));
#163519=CARTESIAN_POINT('Ctrl Pts',(5.60510622485313,5.88569940341101,16.8412173529561));
#163520=CARTESIAN_POINT('Ctrl Pts',(5.4602743105939,6.02031383074355,16.8489548287245));
#163521=CARTESIAN_POINT('Ctrl Pts',(5.31064408635514,6.14953225461589,16.8566923044929));
#163522=CARTESIAN_POINT('Ctrl Pts',(5.16108047460359,6.27869315294048,16.8644263356864));
#163523=CARTESIAN_POINT('Ctrl Pts',(5.00672307400017,6.40246260164256,16.8721603668799));
#163524=CARTESIAN_POINT('Ctrl Pts',(4.84800812455714,6.52046814168492,16.8798943980735));
#163525=CARTESIAN_POINT('Ctrl Pts',(4.68931348562947,6.63845858073431,16.8876274395546));
#163526=CARTESIAN_POINT('Ctrl Pts',(4.52626268731236,6.75068636347696,16.8953604810357));
#163527=CARTESIAN_POINT('Ctrl Pts',(4.35932435057244,6.85681987287155,16.9030935225168));
#163528=CARTESIAN_POINT('Ctrl Pts',(4.19240269084774,6.96294277960777,16.9108257914728));
#163529=CARTESIAN_POINT('Ctrl Pts',(4.02159456643663,7.06297243912803,16.9185580604289));
#163530=CARTESIAN_POINT('Ctrl Pts',(3.84739671419705,7.15662113612882,16.9262903293849));
#163531=CARTESIAN_POINT('Ctrl Pts',(3.67313185596631,7.25030585552416,16.9340255725931));
#163532=CARTESIAN_POINT('Ctrl Pts',(3.49547497637499,7.33760454106587,16.9417608158013));
#163533=CARTESIAN_POINT('Ctrl Pts',(3.31494707532762,7.41827563860206,16.9494960590096));
#163534=CARTESIAN_POINT('Ctrl Pts',(3.163835947401,7.48580149177516,16.9559708549785));
#163535=CARTESIAN_POINT('Ctrl Pts',(3.01071373698051,7.5486844727472,16.9624456509475));
#163536=CARTESIAN_POINT('Ctrl Pts',(2.85589627835534,7.6068090556932,16.9689204469164));
#163537=CARTESIAN_POINT('Ctrl Pts',(2.65470914632731,7.68234264374637,16.9773345214208));
#163538=CARTESIAN_POINT('Ctrl Pts',(2.4505619950606,7.74987627656709,16.9857485959252));
#163539=CARTESIAN_POINT('Ctrl Pts',(2.24409501977395,7.80920771299661,16.9941626704297));
#163540=CARTESIAN_POINT('Ctrl Pts',(2.03757038394225,7.86855571906376,17.0025790947536));
#163541=CARTESIAN_POINT('Ctrl Pts',(1.8287248845117,7.91969688292368,17.0109955190775));
#163542=CARTESIAN_POINT('Ctrl Pts',(1.61821235668358,7.96247928293547,17.0194119434014));
#163543=CARTESIAN_POINT('Ctrl Pts',(1.40764762321557,8.00527229268432,17.0278304549399));
#163544=CARTESIAN_POINT('Ctrl Pts',(1.195415294672,8.03970234764673,17.0362489664784));
#163545=CARTESIAN_POINT('Ctrl Pts',(0.982178923991239,8.06566873382284,
17.0446674780168));
#163546=CARTESIAN_POINT('Ctrl Pts',(0.768860650111411,8.0916450935794,17.0530892230704));
#163547=CARTESIAN_POINT('Ctrl Pts',(0.554537825397038,8.10915125503629,
17.061510968124));
#163548=CARTESIAN_POINT('Ctrl Pts',(0.339880079721553,8.11813827757993,
17.0699327131776));
#163549=CARTESIAN_POINT('Ctrl Pts',(0.125199065731904,8.12712627429231,
17.0783553711254));
#163550=CARTESIAN_POINT('Ctrl Pts',(-0.0898166778647321,8.12759328030146,
17.0867780290732));
#163551=CARTESIAN_POINT('Ctrl Pts',(-0.304495944304193,8.11954246139536,
17.095200687021));
#163552=CARTESIAN_POINT('Ctrl Pts',(-0.519216036560872,8.11149011145525,
17.1036249467159));
#163553=CARTESIAN_POINT('Ctrl Pts',(-0.733599260085607,8.09491671049226,
17.1120492064108));
#163554=CARTESIAN_POINT('Ctrl Pts',(-0.946976624282326,8.06987749817572,
17.1204734661057));
#163555=CARTESIAN_POINT('Ctrl Pts',(-1.00704369291895,8.06282880259132,
17.1228449481381));
#163556=CARTESIAN_POINT('Ctrl Pts',(-1.06703108059628,8.05510954281571,
17.1252164301704));
#163557=CARTESIAN_POINT('Ctrl Pts',(-1.12692394473314,8.04672169180015,
17.1275879122028));
#163558=CARTESIAN_POINT('Ctrl Pts',(-1.33968413391722,8.01692514099837,
17.1360122374229));
#163559=CARTESIAN_POINT('Ctrl Pts',(-1.55127286867005,7.97868449960255,
17.144436562643));
#163560=CARTESIAN_POINT('Ctrl Pts',(-1.76102908195827,7.93211599354152,
17.1528608878631));
#163561=CARTESIAN_POINT('Ctrl Pts',(-1.97074904680779,7.88555553508782,
17.1612837572568));
#163562=CARTESIAN_POINT('Ctrl Pts',(-2.17863686517976,7.83067014357823,
17.1697066266505));
#163563=CARTESIAN_POINT('Ctrl Pts',(-2.38404252274152,7.76762697432493,
17.1781294960442));
#163564=CARTESIAN_POINT('Ctrl Pts',(-2.58940620531185,7.70459668804924,
17.1865506442104));
#163565=CARTESIAN_POINT('Ctrl Pts',(-2.79228848781976,7.6334120304237,17.1949717923765));
#163566=CARTESIAN_POINT('Ctrl Pts',(-2.99205430072729,7.55429008074216,
17.2033929405427));
#163567=CARTESIAN_POINT('Ctrl Pts',(-3.19176406608829,7.47519033000993,
17.2118117260189));
#163568=CARTESIAN_POINT('Ctrl Pts',(-3.38835886300686,7.38815783212735,
17.220230511495));
#163569=CARTESIAN_POINT('Ctrl Pts',(-3.58122245304708,7.29345825409945,
17.2286492969712));
#163570=CARTESIAN_POINT('Ctrl Pts',(-3.77403216793572,7.19878512976414,
17.237065730716));
#163571=CARTESIAN_POINT('Ctrl Pts',(-3.96311252025934,7.09644931774732,
17.2454821644608));
#163572=CARTESIAN_POINT('Ctrl Pts',(-4.14786973175427,6.9867635032894,17.2538985982057));
#163573=CARTESIAN_POINT('Ctrl Pts',(-4.33255988712078,6.87711749840644,
17.2623119772743));
#163574=CARTESIAN_POINT('Ctrl Pts',(-4.51292980825997,6.76012695288952,
17.2707253563429));
#163575=CARTESIAN_POINT('Ctrl Pts',(-4.6884118251844,6.63614964568846,17.2791387354115));
#163576=CARTESIAN_POINT('Ctrl Pts',(-4.73789026879763,6.60119333329145,
17.2815109494374));
#163577=CARTESIAN_POINT('Ctrl Pts',(-4.78698029127896,6.56568184425487,
17.2838831634633));
#163578=CARTESIAN_POINT('Ctrl Pts',(-4.83566957250315,6.52962382898641,
17.2862553774892));
#163579=CARTESIAN_POINT('Ctrl Pts',(-4.99443290048469,6.41204783771085,
17.2939905623999));
#163580=CARTESIAN_POINT('Ctrl Pts',(-5.14900346709389,6.28860545606571,
17.3017257473106));
#163581=CARTESIAN_POINT('Ctrl Pts',(-5.29892005504036,6.15963747413686,
17.3094609322213));
#163582=CARTESIAN_POINT('Ctrl Pts',(-5.44879028507363,6.03070937229461,
17.3171937252217));
#163583=CARTESIAN_POINT('Ctrl Pts',(-5.59400913483348,5.89625930293477,
17.3249265182221));
#163584=CARTESIAN_POINT('Ctrl Pts',(-5.73414793131289,5.75666874714188,
17.3326593112225));
#163585=CARTESIAN_POINT('Ctrl Pts',(-5.87426829202127,5.61709655499695,
17.3403910869457));
#163586=CARTESIAN_POINT('Ctrl Pts',(-6.00930968090495,5.47238547321573,
17.3481228626689));
#163587=CARTESIAN_POINT('Ctrl Pts',(-6.13887971955536,5.32295438185712,
17.3558546383921));
#163588=CARTESIAN_POINT('Ctrl Pts',(-6.2684961219023,5.1734698199752,17.3635891807557));
#163589=CARTESIAN_POINT('Ctrl Pts',(-6.39263702761418,5.01926213857458,
17.3713237231193));
#163590=CARTESIAN_POINT('Ctrl Pts',(-6.51094943771995,4.86078439986328,
17.3790582654829));
#163591=CARTESIAN_POINT('Ctrl Pts',(-6.62928182947274,4.70227989602876,
17.3867941141244));
#163592=CARTESIAN_POINT('Ctrl Pts',(-6.74178355890835,4.53950418568419,
17.394529962766));
#163593=CARTESIAN_POINT('Ctrl Pts',(-6.84814446647343,4.37294007834653,
17.4022658114076));
#163594=CARTESIAN_POINT('Ctrl Pts',(-6.95459240334909,4.20623968071423,
17.4100079898708));
#163595=CARTESIAN_POINT('Ctrl Pts',(-7.05488929538259,4.03574499481885,
17.417750168334));
#163596=CARTESIAN_POINT('Ctrl Pts',(-7.14877007217295,3.86196504615259,
17.4254923467972));
#163597=CARTESIAN_POINT('Ctrl Pts',(-7.22730740136443,3.71658690270414,
17.43196917879));
#163598=CARTESIAN_POINT('Ctrl Pts',(-7.30135524443815,3.56891013651415,
17.4384460107828));
#163599=CARTESIAN_POINT('Ctrl Pts',(-7.37078419891133,3.41924375492288,
17.4449228427756));
#163600=CARTESIAN_POINT('Ctrl Pts',(-7.47152716887149,3.20207447880307,
17.4543208712471));
#163601=CARTESIAN_POINT('Ctrl Pts',(-7.56260259696826,2.98059280367584,
17.4637188997187));
#163602=CARTESIAN_POINT('Ctrl Pts',(-7.64371577516674,2.75559371297133,
17.4731169281902));
#163603=CARTESIAN_POINT('Ctrl Pts',(-7.72494437062792,2.53027446739513,
17.4825283292695));
#163604=CARTESIAN_POINT('Ctrl Pts',(-7.79618234821169,2.30142782976832,
17.4919397303489));
#163605=CARTESIAN_POINT('Ctrl Pts',(-7.85718390911585,2.06986680267859,
17.5013511314282));
#163606=CARTESIAN_POINT('Ctrl Pts',(-7.91809362187505,1.83865442979492,
17.5107483620549));
#163607=CARTESIAN_POINT('Ctrl Pts',(-7.96879771652282,1.6047358719949,17.5201455926816));
#163608=CARTESIAN_POINT('Ctrl Pts',(-8.00910145045261,1.36893444651592,
17.5295428233083));
#163609=CARTESIAN_POINT('Ctrl Pts',(-8.04930352333066,1.13372780019461,
17.5389163506139));
#163610=CARTESIAN_POINT('Ctrl Pts',(-8.07915760945394,0.896647806682439,
17.5482898779194));
#163611=CARTESIAN_POINT('Ctrl Pts',(-8.09852038546559,0.658524964369773,
17.557663405225));
#163612=CARTESIAN_POINT('Ctrl Pts',(-8.11775742074714,0.42194847780847,
17.5669760613947));
#163613=CARTESIAN_POINT('Ctrl Pts',(-8.12663893851337,0.184342685548523,
17.5762887175645));
#163614=CARTESIAN_POINT('Ctrl Pts',(-8.12507409327281,-0.0534653282699481,
17.5856013737343));
#163615=CARTESIAN_POINT('Ctrl Pts',(-8.12406650754745,-0.206587153923133,
17.5915976851769));
#163616=CARTESIAN_POINT('Ctrl Pts',(-8.11872894262562,-0.359792564339886,
17.5975939966195));
#163617=CARTESIAN_POINT('Ctrl Pts',(-8.10904828820628,-0.512858091521222,
17.6035903080621));
#163618=CARTESIAN_POINT('Ctrl Pts',(-8.09683079673091,-0.706034781082006,
17.6111579662761));
#163619=CARTESIAN_POINT('Ctrl Pts',(-8.07769740879767,-0.898911817353965,
17.6187256244901));
#163620=CARTESIAN_POINT('Ctrl Pts',(-8.0516796739349,-1.09093629091876,
17.6262932827041));
#163621=CARTESIAN_POINT('Ctrl Pts',(-8.02566914291522,-1.2829075963586,
17.6338588455696));
#163622=CARTESIAN_POINT('Ctrl Pts',(-7.99277810706042,-1.47402644483414,
17.641424408435));
#163623=CARTESIAN_POINT('Ctrl Pts',(-7.95308998041258,-1.66374497022859,
17.6489899713005));
#163624=CARTESIAN_POINT('Ctrl Pts',(-7.91340533082007,-1.8534468744856,
17.6565548713511));
#163625=CARTESIAN_POINT('Ctrl Pts',(-7.86692485180811,-2.04174834014855,
17.6641197714017));
#163626=CARTESIAN_POINT('Ctrl Pts',(-7.81378307047753,-2.22811168706119,
17.6716846714523));
#163627=CARTESIAN_POINT('Ctrl Pts',(-7.76061520748913,-2.41456649995265,
17.6792532843091));
#163628=CARTESIAN_POINT('Ctrl Pts',(-7.70077960856521,-2.59908093877052,
17.6868218971659));
#163629=CARTESIAN_POINT('Ctrl Pts',(-7.63446086414704,-2.78113194154957,
17.6943905100227));
#163630=CARTESIAN_POINT('Ctrl Pts',(-7.56812737160585,-2.96322342927155,
17.701960806006));
#163631=CARTESIAN_POINT('Ctrl Pts',(-7.49530799821113,-3.14285004816545,
17.7095311019892));
#163632=CARTESIAN_POINT('Ctrl Pts',(-7.41623541380621,-3.31950897716915,
17.7171013979725));
#163633=CARTESIAN_POINT('Ctrl Pts',(-7.33708270633128,-3.49634691202988,
17.7246793648237));
#163634=CARTESIAN_POINT('Ctrl Pts',(-7.25166428915407,-3.67021081810455,
17.7322573316749));
#163635=CARTESIAN_POINT('Ctrl Pts',(-7.16025912791398,-3.8406219266708,
17.7398352985261));
#163636=CARTESIAN_POINT('Ctrl Pts',(-7.07010610196467,-4.0086986182295,
17.7473094568003));
#163637=CARTESIAN_POINT('Ctrl Pts',(-6.97412953600833,-4.17341624939413,
17.7547836150744));
#163638=CARTESIAN_POINT('Ctrl Pts',(-6.87263762475836,-4.33434419967494,
17.7622577733485));
#163639=CARTESIAN_POINT('Ctrl Pts',(-6.76298914340258,-4.50820539845095,
17.7703326050674));
#163640=CARTESIAN_POINT('Ctrl Pts',(-6.64666942776123,-4.67801477267513,
17.7784074367863));
#163641=CARTESIAN_POINT('Ctrl Pts',(-6.52400396072606,-4.84324889747891,
17.7864822685052));
#163642=CARTESIAN_POINT('Ctrl Pts',(-6.40141964896652,-5.00837370365156,
17.7945517579284));
#163643=CARTESIAN_POINT('Ctrl Pts',(-6.27249814595655,-5.16892904292965,
17.8026212473516));
#163644=CARTESIAN_POINT('Ctrl Pts',(-6.13760819416067,-5.32442045836651,
17.8106907367748));
#163645=CARTESIAN_POINT('Ctrl Pts',(-6.00278910913358,-5.47983018369938,
17.8187559867522));
#163646=CARTESIAN_POINT('Ctrl Pts',(-5.86200803576692,-5.6301810520313,
17.8268212367296));
#163647=CARTESIAN_POINT('Ctrl Pts',(-5.71567433269601,-5.77501121081683,
17.834886486707));
#163648=CARTESIAN_POINT('Ctrl Pts',(-5.56939759429301,-5.91978499023296,
17.8429485970503));
#163649=CARTESIAN_POINT('Ctrl Pts',(-5.41757276213034,-6.0590421239127,
17.8510107073936));
#163650=CARTESIAN_POINT('Ctrl Pts',(-5.26064685945091,-6.1923567551175,
17.8590728177369));
#163651=CARTESIAN_POINT('Ctrl Pts',(-5.10376070590889,-6.3256376178908,
17.8671328859576));
#163652=CARTESIAN_POINT('Ctrl Pts',(-4.94177630046075,-6.45297877583114,
17.8751929541782));
#163653=CARTESIAN_POINT('Ctrl Pts',(-4.77517509400821,-6.57399348828881,
17.8832530223989));
#163654=CARTESIAN_POINT('Ctrl Pts',(-4.6060779530136,-6.69682118162071,
17.8914338424624));
#163655=CARTESIAN_POINT('Ctrl Pts',(-4.43222482790505,-6.81313114154238,
17.8996146625258));
#163656=CARTESIAN_POINT('Ctrl Pts',(-4.25415189119161,-6.92256305490754,
17.9077954825892));
#163657=CARTESIAN_POINT('Ctrl Pts',(-4.07869034262652,-7.03039018089239,
17.9158563332909));
#163658=CARTESIAN_POINT('Ctrl Pts',(-3.89913218443488,-7.13153945333932,
17.9239171839927));
#163659=CARTESIAN_POINT('Ctrl Pts',(-3.71601769607196,-7.225711040789,17.9319780346944));
#163660=CARTESIAN_POINT('Ctrl Pts',(-3.53287283983618,-7.31989824574017,
17.9400402222149));
#163661=CARTESIAN_POINT('Ctrl Pts',(-3.34617075889484,-7.40710531267174,
17.9481024097354));
#163662=CARTESIAN_POINT('Ctrl Pts',(-3.15647496882119,-7.48707909225655,
17.9561645972559));
#163663=CARTESIAN_POINT('Ctrl Pts',(-2.9667242194974,-7.56707604209178,
17.9642291205783));
#163664=CARTESIAN_POINT('Ctrl Pts',(-2.77397832304669,-7.63983540171236,
17.9722936439006));
#163665=CARTESIAN_POINT('Ctrl Pts',(-2.57881989454899,-7.70515253022147,
17.980358167223));
#163666=CARTESIAN_POINT('Ctrl Pts',(-2.37870002529172,-7.77213019200182,
17.9886277119479));
#163667=CARTESIAN_POINT('Ctrl Pts',(-2.17604367050982,-7.83128209833625,
17.9968972566727));
#163668=CARTESIAN_POINT('Ctrl Pts',(-1.97149434979881,-7.88244236206085,
18.0051668013976));
#163669=CARTESIAN_POINT('Ctrl Pts',(-1.77174675685978,-7.932401655485,18.0132422212902));
#163670=CARTESIAN_POINT('Ctrl Pts',(-1.57019439223873,-7.97474026313108,
18.0213176411829));
#163671=CARTESIAN_POINT('Ctrl Pts',(-1.36744602125939,-8.00935571325446,
18.0293930610755));
#163672=CARTESIAN_POINT('Ctrl Pts',(-1.15738685517106,-8.04521934338656,
18.0377596682165));
#163673=CARTESIAN_POINT('Ctrl Pts',(-0.946044203840001,-8.07279244431162,
18.0461262753574));
#163674=CARTESIAN_POINT('Ctrl Pts',(-0.734100270084997,-8.09201979458535,
18.0544928824984));
#163675=CARTESIAN_POINT('Ctrl Pts',(-0.522156336329993,-8.11124714485908,
18.0628594896394));
#163676=CARTESIAN_POINT('Ctrl Pts',(-0.309611496744794,-8.12212876252602,
18.0712260967804));
#163677=CARTESIAN_POINT('Ctrl Pts',(-0.0971476232154044,-8.12466921799304,
18.0795927039214));
#163678=CARTESIAN_POINT('Ctrl Pts',(0.107985978474591,-8.12712202453951,
18.0876706525545));
#163679=CARTESIAN_POINT('Ctrl Pts',(0.313442941770192,-8.12180438688238,
18.0957486011875));
#163680=CARTESIAN_POINT('Ctrl Pts',(0.518609289507992,-8.10868250502731,
18.1038265498206));
#163681=CARTESIAN_POINT('Ctrl Pts',(0.723524555302593,-8.09557668169076,
18.1118946126851));
#163682=CARTESIAN_POINT('Ctrl Pts',(0.928149601924156,-8.07468567214938,
18.1199626755495));
#163683=CARTESIAN_POINT('Ctrl Pts',(1.13186887190644,-8.04602761735934,
18.128030738414));
#163684=CARTESIAN_POINT('Ctrl Pts',(1.33536391130014,-8.01740110603838,
18.1360899208889));
#163685=CARTESIAN_POINT('Ctrl Pts',(1.53795485079752,-7.98102463602732,
18.1441491033638));
#163686=CARTESIAN_POINT('Ctrl Pts',(1.7390290633868,-7.9369682800926,18.1522082858387));
#163687=CARTESIAN_POINT('Ctrl Pts',(1.93984500317893,-7.892968513007,18.1602571165754));
#163688=CARTESIAN_POINT('Ctrl Pts',(2.1391477956511,-7.84130860665253,18.1683059473121));
#163689=CARTESIAN_POINT('Ctrl Pts',(2.33633279343447,-7.78211003782539,
18.1763547780488));
#163690=CARTESIAN_POINT('Ctrl Pts',(2.53336864137543,-7.72295624652854,
18.1843975206863));
#163691=CARTESIAN_POINT('Ctrl Pts',(2.72828958651205,-7.65627524909058,
18.1924402633237));
#163692=CARTESIAN_POINT('Ctrl Pts',(2.92050265501969,-7.58223923419216,
18.2004830059612));
#163693=CARTESIAN_POINT('Ctrl Pts',(3.11255915874804,-7.50826352441463,
18.208519197482));
#163694=CARTESIAN_POINT('Ctrl Pts',(3.30191189189283,-7.42694486085441,
18.2165553890029));
#163695=CARTESIAN_POINT('Ctrl Pts',(3.48798422267296,-7.33850486304155,
18.2245915805238));
#163696=CARTESIAN_POINT('Ctrl Pts',(3.59347972379901,-7.28836295397996,
18.2291477767518));
#163697=CARTESIAN_POINT('Ctrl Pts',(3.69792105796595,-7.23593284044076,
18.2337039729798));
#163698=CARTESIAN_POINT('Ctrl Pts',(3.80120582549461,-7.18126185532361,
18.2382601692078));
#163699=CARTESIAN_POINT('Ctrl Pts',(3.98338619948005,-7.08482962477197,
18.2462966837165));
#163700=CARTESIAN_POINT('Ctrl Pts',(4.16182284614464,-6.98149918834426,
18.2543331982252));
#163701=CARTESIAN_POINT('Ctrl Pts',(4.33599122287397,-6.87159862605929,
18.2623697127338));
#163702=CARTESIAN_POINT('Ctrl Pts',(4.51026481463818,-6.76163167289607,
18.2704110820972));
#163703=CARTESIAN_POINT('Ctrl Pts',(4.68026472520352,-6.64508684402324,
18.2784524514605));
#163704=CARTESIAN_POINT('Ctrl Pts',(4.84549629750284,-6.52233494949365,
18.2864938208239));
#163705=CARTESIAN_POINT('Ctrl Pts',(5.01084788878781,-6.39949389187214,
18.2945410311834));
#163706=CARTESIAN_POINT('Ctrl Pts',(5.17142397839643,-6.27043696160652,
18.302588241543));
#163707=CARTESIAN_POINT('Ctrl Pts',(5.3267633583719,-6.13557492712839,18.3106354519026));
#163708=CARTESIAN_POINT('Ctrl Pts',(5.48233169749899,-6.0005141156434,18.3186945232755));
#163709=CARTESIAN_POINT('Ctrl Pts',(5.63264766150448,-5.85963130608115,
18.3267535946485));
#163710=CARTESIAN_POINT('Ctrl Pts',(5.77728601207804,-5.7133750005708,18.3348126660214));
#163711=CARTESIAN_POINT('Ctrl Pts',(5.9220414255642,-5.56700032265755,18.3428782599961));
#163712=CARTESIAN_POINT('Ctrl Pts',(6.06110984260431,-5.41524370229707,
18.3509438539708));
#163713=CARTESIAN_POINT('Ctrl Pts',(6.19410608185046,-5.25858701642211,
18.3590094479456));
#163714=CARTESIAN_POINT('Ctrl Pts',(6.32731115557887,-5.1016843437578,18.3670877067457));
#163715=CARTESIAN_POINT('Ctrl Pts',(6.45442479817904,-4.93986647417383,
18.3751659655457));
#163716=CARTESIAN_POINT('Ctrl Pts',(6.57510391216856,-4.77364599721069,
18.3832442243458));
#163717=CARTESIAN_POINT('Ctrl Pts',(6.64324160759418,-4.67979479248775,
18.3878053610619));
#163718=CARTESIAN_POINT('Ctrl Pts',(6.70932882071092,-4.5845405536798,18.3923664977781));
#163719=CARTESIAN_POINT('Ctrl Pts',(6.77331025023357,-4.4879790347751,18.3969276344942));
#163720=CARTESIAN_POINT('Ctrl Pts',(6.88817556936919,-4.31462295680121,
18.4051162046533));
#163721=CARTESIAN_POINT('Ctrl Pts',(6.99647176939325,-4.1367191744666,18.4133047748123));
#163722=CARTESIAN_POINT('Ctrl Pts',(7.0978411999887,-3.95478670249648,18.4214933449713));
#163723=CARTESIAN_POINT('Ctrl Pts',(7.1991119185707,-3.77303139360711,18.429673941225));
#163724=CARTESIAN_POINT('Ctrl Pts',(7.2934691728929,-3.58725548170466,18.4378545374786));
#163725=CARTESIAN_POINT('Ctrl Pts',(7.380598997499,-3.39800618019107,18.4460351337322));
#163726=CARTESIAN_POINT('Ctrl Pts',(7.4676520891475,-3.20892354558741,18.4542085255487));
#163727=CARTESIAN_POINT('Ctrl Pts',(7.5474903194604,-3.01637389587714,18.4623819173652));
#163728=CARTESIAN_POINT('Ctrl Pts',(7.61984564791169,-2.82092890100074,
18.4705553091817));
#163729=CARTESIAN_POINT('Ctrl Pts',(7.6921439731308,-2.62563788229526,18.4787222618076));
#163730=CARTESIAN_POINT('Ctrl Pts',(7.75697105008127,-2.42745635098308,
18.4868892144335));
#163731=CARTESIAN_POINT('Ctrl Pts',(7.81410667775081,-2.22697651339886,
18.4950561670594));
#163732=CARTESIAN_POINT('Ctrl Pts',(7.87119180948338,-2.02667385803275,
18.5032159018084));
#163733=CARTESIAN_POINT('Ctrl Pts',(7.92059897554161,-1.82407724048578,
18.5113756365574));
#163734=CARTESIAN_POINT('Ctrl Pts',(7.96215748145354,-1.61979498796403,
18.5195353713064));
#163735=CARTESIAN_POINT('Ctrl Pts',(8.00369332716982,-1.41562412240651,
18.5276906568776));
#163736=CARTESIAN_POINT('Ctrl Pts',(8.03738898762161,-1.20976975079092,
18.5358459424487));
#163737=CARTESIAN_POINT('Ctrl Pts',(8.06312434927614,-1.00285257670819,
18.5440012280198));
#163738=CARTESIAN_POINT('Ctrl Pts',(8.08884554679798,-0.796049284930593,
18.5521520251152));
#163739=CARTESIAN_POINT('Ctrl Pts',(8.10661515075115,-0.588184657728283,
18.5603028222105));
#163740=CARTESIAN_POINT('Ctrl Pts',(8.1163645301893,-0.379887319589674,
18.5684536193059));
#163741=CARTESIAN_POINT('Ctrl Pts',(8.12228289088803,-0.253440422378366,
18.5734015606081));
#163742=CARTESIAN_POINT('Ctrl Pts',(8.12524672091287,-0.12683422128016,
18.5783495019102));
#163743=CARTESIAN_POINT('Ctrl Pts',(8.12524999728006,-0.000210239024478989,
18.5832974432124));
#163744=CARTESIAN_POINT('',(8.13282513948647,0.00629553435497102,20.5832974432124));
#163745=CARTESIAN_POINT('Ctrl Pts',(8.12524999728007,-0.000210238467663868,
18.5832974432342));
#163746=CARTESIAN_POINT('Ctrl Pts',(8.12525592540781,0.22889873702772,18.5922500740262));
#163747=CARTESIAN_POINT('Ctrl Pts',(8.11556726318553,0.457755304909344,
18.6012027048182));
#163748=CARTESIAN_POINT('Ctrl Pts',(8.09627343309599,0.685597592647516,
18.6101553356103));
#163749=CARTESIAN_POINT('Ctrl Pts',(8.07688960545325,0.914502668246784,
18.6191497266367));
#163750=CARTESIAN_POINT('Ctrl Pts',(8.04781084098892,1.14238383675527,18.6281441176631));
#163751=CARTESIAN_POINT('Ctrl Pts',(8.00917884981307,1.36848153593939,18.6371385086895));
#163752=CARTESIAN_POINT('Ctrl Pts',(7.97047456489684,1.5950023416698,18.6461497313145));
#163753=CARTESIAN_POINT('Ctrl Pts',(7.9221813288671,1.81973286353389,18.6551609539395));
#163754=CARTESIAN_POINT('Ctrl Pts',(7.86449187315936,2.04192437164316,18.6641721765645));
#163755=CARTESIAN_POINT('Ctrl Pts',(7.80669877566234,2.2645150571269,18.6731995882699));
#163756=CARTESIAN_POINT('Ctrl Pts',(7.73947572271128,2.48455746566079,18.6822269999754));
#163757=CARTESIAN_POINT('Ctrl Pts',(7.66306594241722,2.70131596165003,18.6912544116808));
#163758=CARTESIAN_POINT('Ctrl Pts',(7.59815077062031,2.88546666790035,18.6989237961429));
#163759=CARTESIAN_POINT('Ctrl Pts',(7.52660580849166,3.06724741300914,18.7065931806049));
#163760=CARTESIAN_POINT('Ctrl Pts',(7.44860772744946,3.24621787393887,18.714262565067));
#163761=CARTESIAN_POINT('Ctrl Pts',(7.37153654171261,3.42306152767263,18.7218408098965));
#163762=CARTESIAN_POINT('Ctrl Pts',(7.28805534919494,3.59740693234696,18.7294190547259));
#163763=CARTESIAN_POINT('Ctrl Pts',(7.19835504487957,3.76873615557747,18.7369972995554));
#163764=CARTESIAN_POINT('Ctrl Pts',(7.10872148891895,3.93993788822854,18.7445699052136));
#163765=CARTESIAN_POINT('Ctrl Pts',(7.0128781968328,4.10812758098797,18.7521425108718));
#163766=CARTESIAN_POINT('Ctrl Pts',(6.91106436292493,4.27280668109488,18.7597151165301));
#163767=CARTESIAN_POINT('Ctrl Pts',(6.80930695719371,4.43739451127317,18.7672835252308));
#163768=CARTESIAN_POINT('Ctrl Pts',(6.70158578678349,4.59847530888974,18.7748519339316));
#163769=CARTESIAN_POINT('Ctrl Pts',(6.58818620684434,4.75557463052006,18.7824203426324));
#163770=CARTESIAN_POINT('Ctrl Pts',(6.4748140251489,4.91263599570024,18.7899869227452));
#163771=CARTESIAN_POINT('Ctrl Pts',(6.35576637298534,5.06571749724551,18.797553502858));
#163772=CARTESIAN_POINT('Ctrl Pts',(6.2313722770221,5.21437312700774,18.8051200829708));
#163773=CARTESIAN_POINT('Ctrl Pts',(6.10700024800852,5.363002385934,18.8126853208065));
#163774=CARTESIAN_POINT('Ctrl Pts',(5.97728390138052,5.50720705583517,18.8202505586423));
#163775=CARTESIAN_POINT('Ctrl Pts',(5.84259276800369,5.64657394441718,18.827815796478));
#163776=CARTESIAN_POINT('Ctrl Pts',(5.70785479605658,5.78598929755392,18.83538366511));
#163777=CARTESIAN_POINT('Ctrl Pts',(5.56813883473249,5.92056324141084,18.8429515337419));
#163778=CARTESIAN_POINT('Ctrl Pts',(5.42385185756968,6.04991889116193,18.8505194023739));
#163779=CARTESIAN_POINT('Ctrl Pts',(5.28142682683539,6.17760527529528,18.8579896117004));
#163780=CARTESIAN_POINT('Ctrl Pts',(5.13454833590424,6.30020704009739,18.865459821027));
#163781=CARTESIAN_POINT('Ctrl Pts',(4.98363930632379,6.4174003168701,18.8729300303535));
#163782=CARTESIAN_POINT('Ctrl Pts',(4.79564785384241,6.56339114580067,18.8822358717968));
#163783=CARTESIAN_POINT('Ctrl Pts',(4.60149533023253,6.70091893766865,18.8915417132401));
#163784=CARTESIAN_POINT('Ctrl Pts',(4.40190335348933,6.82956326781145,18.9008475546834));
#163785=CARTESIAN_POINT('Ctrl Pts',(4.20123980769149,6.95889826340827,18.9102033573119));
#163786=CARTESIAN_POINT('Ctrl Pts',(3.99507831279999,7.07925417467187,18.9195591599404));
#163787=CARTESIAN_POINT('Ctrl Pts',(3.78417060822886,7.19025315064197,18.9289149625689));
#163788=CARTESIAN_POINT('Ctrl Pts',(3.5722390616589,7.30179096616588,18.9383161825219));
#163789=CARTESIAN_POINT('Ctrl Pts',(3.35551516149101,7.40388078177639,18.9477174024749));
#163790=CARTESIAN_POINT('Ctrl Pts',(3.1347793400703,7.49618876840548,18.9571186224279));
#163791=CARTESIAN_POINT('Ctrl Pts',(2.91380461698811,7.58859665966822,18.9665300172908));
#163792=CARTESIAN_POINT('Ctrl Pts',(2.6888093259892,7.67120154176815,18.9759414121536));
#163793=CARTESIAN_POINT('Ctrl Pts',(2.46059342949554,7.74371794019019,18.9853528070164));
#163794=CARTESIAN_POINT('Ctrl Pts',(2.23264523407621,7.8161492756606,18.9947531621551));
#163795=CARTESIAN_POINT('Ctrl Pts',(2.00148402037825,7.87851577453662,19.0041535172939));
#163796=CARTESIAN_POINT('Ctrl Pts',(1.76792329316785,7.93058224797994,19.0135538724327));
#163797=CARTESIAN_POINT('Ctrl Pts',(1.61848632347989,7.96389545138806,19.0195684135018));
#163798=CARTESIAN_POINT('Ctrl Pts',(1.46806739129636,7.99299311936093,19.0255829545708));
#163799=CARTESIAN_POINT('Ctrl Pts',(1.31688299790545,8.01782431413457,19.0315974956399));
#163800=CARTESIAN_POINT('Ctrl Pts',(1.12226886331984,8.0497886020694,19.0393397941592));
#163801=CARTESIAN_POINT('Ctrl Pts',(0.926294388794416,8.07469507653537,
19.0470820926784));
#163802=CARTESIAN_POINT('Ctrl Pts',(0.729521306748375,8.09243388761998,
19.0548243911977));
#163803=CARTESIAN_POINT('Ctrl Pts',(0.532870796514254,8.11016164903156,
19.0625618669661));
#163804=CARTESIAN_POINT('Ctrl Pts',(0.335423019633146,8.12073060539961,
19.0702993427345));
#163805=CARTESIAN_POINT('Ctrl Pts',(0.137748106460787,8.12408228796745,
19.0780368185028));
#163806=CARTESIAN_POINT('Ctrl Pts',(-0.0598388056572187,8.12743247843093,
19.0857708496964));
#163807=CARTESIAN_POINT('Ctrl Pts',(-0.257652300201885,8.12357178815811,
19.09350488089));
#163808=CARTESIAN_POINT('Ctrl Pts',(-0.455118801602479,8.11249372504706,
19.1012389120836));
#163809=CARTESIAN_POINT('Ctrl Pts',(-0.652560033508927,8.10141707957925,
19.1089719535647));
#163810=CARTESIAN_POINT('Ctrl Pts',(-0.849654007780657,8.08312491303037,
19.1167049950458));
#163811=CARTESIAN_POINT('Ctrl Pts',(-1.04582845265743,8.05766283795197,
19.1244380365269));
#163812=CARTESIAN_POINT('Ctrl Pts',(-1.24198329985284,8.03220330651596,
19.1321703054829));
#163813=CARTESIAN_POINT('Ctrl Pts',(-1.4372184506385,7.9995753423428,19.1399025744389));
#163814=CARTESIAN_POINT('Ctrl Pts',(-1.63096817213315,7.95987627943982,
19.1476348433949));
#163815=CARTESIAN_POINT('Ctrl Pts',(-1.8247924203341,7.92016194611281,19.1553700866032));
#163816=CARTESIAN_POINT('Ctrl Pts',(-2.01712975118378,7.87337115081103,
19.1631053298114));
#163817=CARTESIAN_POINT('Ctrl Pts',(-2.20742537649299,7.8196522153939,19.1708405730196));
#163818=CARTESIAN_POINT('Ctrl Pts',(-2.36671259145059,7.77468670660105,
19.1773153689885));
#163819=CARTESIAN_POINT('Ctrl Pts',(-2.52456938131791,7.72486788974736,
19.1837901649575));
#163820=CARTESIAN_POINT('Ctrl Pts',(-2.68067922985854,7.67030940895509,
19.1902649609264));
#163821=CARTESIAN_POINT('Ctrl Pts',(-2.88354583797946,7.59941001313845,
19.1986790354308));
#163822=CARTESIAN_POINT('Ctrl Pts',(-3.08355983584028,7.52047173603659,
19.2070931099352));
#163823=CARTESIAN_POINT('Ctrl Pts',(-3.28010010219494,7.4337494497784,19.2155071844396));
#163824=CARTESIAN_POINT('Ctrl Pts',(-3.47669525683877,7.34700294437157,
19.2239236087635));
#163825=CARTESIAN_POINT('Ctrl Pts',(-3.66981450173128,7.25246819665597,
19.2323400330874));
#163826=CARTESIAN_POINT('Ctrl Pts',(-3.85885848100777,7.15044745355523,
19.2407564574114));
#163827=CARTESIAN_POINT('Ctrl Pts',(-4.04794934187362,7.0484014100212,19.2491749689499));
#163828=CARTESIAN_POINT('Ctrl Pts',(-4.23296268720622,6.9388657901859,19.2575934804884));
#163829=CARTESIAN_POINT('Ctrl Pts',(-4.41332450707338,6.82218838480479,
19.2660119920269));
#163830=CARTESIAN_POINT('Ctrl Pts',(-4.59375560316165,6.70546616412,19.2744337370805));
#163831=CARTESIAN_POINT('Ctrl Pts',(-4.76953138108732,6.58159681852937,
19.282855482134));
#163832=CARTESIAN_POINT('Ctrl Pts',(-4.94010633476706,6.45097178444413,
19.2912772271876));
#163833=CARTESIAN_POINT('Ctrl Pts',(-5.11069977830508,6.3203325909626,19.2996998851353));
#163834=CARTESIAN_POINT('Ctrl Pts',(-5.27609106428128,6.1829364097518,19.3081225430831));
#163835=CARTESIAN_POINT('Ctrl Pts',(-5.43576685901174,6.03921569551624,
19.3165452010308));
#163836=CARTESIAN_POINT('Ctrl Pts',(-5.59547301948438,5.89546764973576,
19.3249694607257));
#163837=CARTESIAN_POINT('Ctrl Pts',(-5.74946132117493,5.74539284475124,
19.3333937204206));
#163838=CARTESIAN_POINT('Ctrl Pts',(-5.8972534943276,5.58946229848103,19.3418179801156));
#163839=CARTESIAN_POINT('Ctrl Pts',(-5.93885791962491,5.54556687001903,
19.344189462148));
#163840=CARTESIAN_POINT('Ctrl Pts',(-5.97997155248067,5.50120762244448,
19.3465609441804));
#163841=CARTESIAN_POINT('Ctrl Pts',(-6.02058426057031,5.45639557985608,
19.3489324262128));
#163842=CARTESIAN_POINT('Ctrl Pts',(-6.16485466040496,5.29720769001222,
19.3573567514329));
#163843=CARTESIAN_POINT('Ctrl Pts',(-6.30281570137254,5.13228682867604,
19.365781076653));
#163844=CARTESIAN_POINT('Ctrl Pts',(-6.43403426978162,4.96214576345513,
19.3742054018731));
#163845=CARTESIAN_POINT('Ctrl Pts',(-6.56523016201678,4.79203410069175,
19.3826282712668));
#163846=CARTESIAN_POINT('Ctrl Pts',(-6.68968574781638,4.6167042447302,19.3910511406605));
#163847=CARTESIAN_POINT('Ctrl Pts',(-6.80700902898126,4.43670098630363,
19.3994740100541));
#163848=CARTESIAN_POINT('Ctrl Pts',(-6.92430833493756,4.25673451184374,
19.4078951582203));
#163849=CARTESIAN_POINT('Ctrl Pts',(-7.03447810275593,4.072096763005,19.4163163063866));
#163850=CARTESIAN_POINT('Ctrl Pts',(-7.13716979400008,3.88336128812564,
19.4247374545528));
#163851=CARTESIAN_POINT('Ctrl Pts',(-7.23983267342025,3.69467876605302,
19.4331562400289));
#163852=CARTESIAN_POINT('Ctrl Pts',(-7.33502154067406,3.50190104583061,
19.4415750255051));
#163853=CARTESIAN_POINT('Ctrl Pts',(-7.42243344493677,3.30562691754288,
19.4499938109812));
#163854=CARTESIAN_POINT('Ctrl Pts',(-7.50982093126933,3.10940761711866,
19.458410244726));
#163855=CARTESIAN_POINT('Ctrl Pts',(-7.58943568483281,2.90969409962262,
19.4668266784708));
#163856=CARTESIAN_POINT('Ctrl Pts',(-7.66102212334421,2.7071068667732,19.4752431122157));
#163857=CARTESIAN_POINT('Ctrl Pts',(-7.73258258014016,2.50459316131174,
19.4836564912843));
#163858=CARTESIAN_POINT('Ctrl Pts',(-7.79612045284465,2.29920807196793,
19.492069870353));
#163859=CARTESIAN_POINT('Ctrl Pts',(-7.85142909578997,2.09158999717502,
19.5004832494216));
#163860=CARTESIAN_POINT('Ctrl Pts',(-7.86702377391825,2.03305055600291,
19.5028554634475));
#163861=CARTESIAN_POINT('Ctrl Pts',(-7.88196453026747,1.97433369334482,
19.5052276774733));
#163862=CARTESIAN_POINT('Ctrl Pts',(-7.89624744735517,1.91545394427456,
19.5075998914992));
#163863=CARTESIAN_POINT('Ctrl Pts',(-7.94282039715334,1.72346209969962,
19.5153350764099));
#163864=CARTESIAN_POINT('Ctrl Pts',(-7.98241564907852,1.52965214723825,
19.5230702613206));
#163865=CARTESIAN_POINT('Ctrl Pts',(-8.01489740902469,1.3345812396813,19.5308054462313));
#163866=CARTESIAN_POINT('Ctrl Pts',(-8.04736912480807,1.13957065286909,
19.5385382392317));
#163867=CARTESIAN_POINT('Ctrl Pts',(-8.07273167110675,0.943300235532242,
19.5462710322321));
#163868=CARTESIAN_POINT('Ctrl Pts',(-8.09090031138873,0.746337533338505,
19.5540038252324));
#163869=CARTESIAN_POINT('Ctrl Pts',(-8.1090665615195,0.549400742309951,
19.5617356009556));
#163870=CARTESIAN_POINT('Ctrl Pts',(-8.12004075901487,0.351772199607964,
19.5694673766787));
#163871=CARTESIAN_POINT('Ctrl Pts',(-8.1237899953504,0.154024913389804,
19.5771991524018));
#163872=CARTESIAN_POINT('Ctrl Pts',(-8.12754057326508,-0.0437931322072041,
19.5849336947655));
#163873=CARTESIAN_POINT('Ctrl Pts',(-8.12406101389956,-0.241729652689559,
19.5926682371291));
#163874=CARTESIAN_POINT('Ctrl Pts',(-8.1133705443868,-0.439210623706513,
19.6004027794927));
#163875=CARTESIAN_POINT('Ctrl Pts',(-8.10267826937293,-0.636724947057523,
19.6081386281343));
#163876=CARTESIAN_POINT('Ctrl Pts',(-8.08477268431997,-0.833783215161422,
19.6158744767758));
#163877=CARTESIAN_POINT('Ctrl Pts',(-8.05972496735744,-1.02981600932158,
19.6236103254174));
#163878=CARTESIAN_POINT('Ctrl Pts',(-8.03465675521876,-1.22600920639016,
19.6313525038806));
#163879=CARTESIAN_POINT('Ctrl Pts',(-8.00243478745337,-1.42117490333365,
19.6390946823438));
#163880=CARTESIAN_POINT('Ctrl Pts',(-7.96318165813537,-1.6147524398608,
19.646836860807));
#163881=CARTESIAN_POINT('Ctrl Pts',(-7.93034388192087,-1.77669254336533,
19.6533136927999));
#163882=CARTESIAN_POINT('Ctrl Pts',(-7.89258635038262,-1.93752126949681,
19.6597905247928));
#163883=CARTESIAN_POINT('Ctrl Pts',(-7.85000767911045,-2.09691845344709,
19.6662673567857));
#163884=CARTESIAN_POINT('Ctrl Pts',(-7.7882250722227,-2.32820734200977,
19.6756653852572));
#163885=CARTESIAN_POINT('Ctrl Pts',(-7.71625675473131,-2.55661361884394,
19.6850634137287));
#163886=CARTESIAN_POINT('Ctrl Pts',(-7.63438577001621,-2.78133807313565,
19.6944614422002));
#163887=CARTESIAN_POINT('Ctrl Pts',(-7.55239828974155,-3.00638229151891,
19.7038728432797));
#163888=CARTESIAN_POINT('Ctrl Pts',(-7.46047996925675,-3.22773417284017,
19.7132842443592));
#163889=CARTESIAN_POINT('Ctrl Pts',(-7.3589629495185,-3.44461200574374,
19.7226956454386));
#163890=CARTESIAN_POINT('Ctrl Pts',(-7.25759878078772,-3.66116329246478,
19.7320928760653));
#163891=CARTESIAN_POINT('Ctrl Pts',(-7.1466648168046,-3.87325396301017,
19.741490106692));
#163892=CARTESIAN_POINT('Ctrl Pts',(-7.02653900850146,-4.08012709661198,
19.7508873373187));
#163893=CARTESIAN_POINT('Ctrl Pts',(-6.90671620229702,-4.2864784190016,
19.7602608646244));
#163894=CARTESIAN_POINT('Ctrl Pts',(-6.77774786475057,-4.48763844906163,
19.76963439193));
#163895=CARTESIAN_POINT('Ctrl Pts',(-6.64005602798172,-4.68287769515323,
19.7790079192357));
#163896=CARTESIAN_POINT('Ctrl Pts',(-6.50325835391401,-4.87684906904738,
19.7883205754055));
#163897=CARTESIAN_POINT('Ctrl Pts',(-6.35785012077209,-5.06497625902391,
19.7976332315753));
#163898=CARTESIAN_POINT('Ctrl Pts',(-6.20429146649526,-5.24656601609797,
19.8069458877452));
#163899=CARTESIAN_POINT('Ctrl Pts',(-6.10541682762634,-5.36348955738288,
19.8129421991875));
#163900=CARTESIAN_POINT('Ctrl Pts',(-6.0031640198267,-5.47770317598873,
19.8189385106297));
#163901=CARTESIAN_POINT('Ctrl Pts',(-5.89766614670997,-5.58902689065379,
19.824934822072));
#163902=CARTESIAN_POINT('Ctrl Pts',(-5.76452232092045,-5.72952323274787,
19.832502480286));
#163903=CARTESIAN_POINT('Ctrl Pts',(-5.62626035307251,-5.86535866958873,
19.8400701385));
#163904=CARTESIAN_POINT('Ctrl Pts',(-5.48325870140168,-5.9961288825377,
19.8476377967141));
#163905=CARTESIAN_POINT('Ctrl Pts',(-5.3402966443179,-6.12686288756515,
19.8552033595795));
#163906=CARTESIAN_POINT('Ctrl Pts',(-5.19259778567835,-6.25253421141723,
19.862768922445));
#163907=CARTESIAN_POINT('Ctrl Pts',(-5.04057717490936,-6.3727756359598,
19.8703344853105));
#163908=CARTESIAN_POINT('Ctrl Pts',(-4.88856988258483,-6.49300652621542,
19.877899385361));
#163909=CARTESIAN_POINT('Ctrl Pts',(-4.73224188063717,-6.60780823659695,
19.8854642854116));
#163910=CARTESIAN_POINT('Ctrl Pts',(-4.57204093794369,-6.71685411664322,
19.8930291854621));
#163911=CARTESIAN_POINT('Ctrl Pts',(-4.41176136961659,-6.82595351573418,
19.9005977983189));
#163912=CARTESIAN_POINT('Ctrl Pts',(-4.24760536564726,-6.92929123097728,
19.9081664111757));
#163913=CARTESIAN_POINT('Ctrl Pts',(-4.08004976876579,-7.02658391018667,
19.9157350240325));
#163914=CARTESIAN_POINT('Ctrl Pts',(-3.91245691046559,-7.12389822557729,
19.9233053200157));
#163915=CARTESIAN_POINT('Ctrl Pts',(-3.74146327695546,-7.21516465234817,
19.9308756159989));
#163916=CARTESIAN_POINT('Ctrl Pts',(-3.56756965920367,-7.30014618273014,
19.9384459119822));
#163917=CARTESIAN_POINT('Ctrl Pts',(-3.39349983764244,-7.38521382362943,
19.9460238788334));
#163918=CARTESIAN_POINT('Ctrl Pts',(-3.21652449632797,-7.46398369347404,
19.9536018456846));
#163919=CARTESIAN_POINT('Ctrl Pts',(-3.03716456310491,-7.53626691267764,
19.9611798125359));
#163920=CARTESIAN_POINT('Ctrl Pts',(-2.86026163448587,-7.60755994305152,
19.9686539708101));
#163921=CARTESIAN_POINT('Ctrl Pts',(-2.68103936948266,-7.67254285586047,
19.9761281290843));
#163922=CARTESIAN_POINT('Ctrl Pts',(-2.50001029116415,-7.73108246667783,
19.9836022873585));
#163923=CARTESIAN_POINT('Ctrl Pts',(-2.30443250300125,-7.79432671290568,
19.9916771190774));
#163924=CARTESIAN_POINT('Ctrl Pts',(-2.10632834216557,-7.85018583285089,
19.9997519507963));
#163925=CARTESIAN_POINT('Ctrl Pts',(-1.90628306307884,-7.89846646165689,
20.0078267825152));
#163926=CARTESIAN_POINT('Ctrl Pts',(-1.70637013362725,-7.94671514807647,
20.0158962719384));
#163927=CARTESIAN_POINT('Ctrl Pts',(-1.50451895381468,-7.98739526751259,
20.0239657613616));
#163928=CARTESIAN_POINT('Ctrl Pts',(-1.30132943440447,-8.02036341231821,
20.0320352507848));
#163929=CARTESIAN_POINT('Ctrl Pts',(-1.09824666412182,-8.05331423673887,
20.0401005007622));
#163930=CARTESIAN_POINT('Ctrl Pts',(-0.893827268475251,-8.07856111595242,
20.0481657507397));
#163931=CARTESIAN_POINT('Ctrl Pts',(-0.688681455135274,-8.09601169810498,
20.0562310007171));
#163932=CARTESIAN_POINT('Ctrl Pts',(-0.483615500793642,-8.11345548710887,
20.0642931110604));
#163933=CARTESIAN_POINT('Ctrl Pts',(-0.277824007947301,-8.12310900535834,
20.0723552214037));
#163934=CARTESIAN_POINT('Ctrl Pts',(-0.0719230421407833,-8.12493166977478,
20.0804173317471));
#163935=CARTESIAN_POINT('Ctrl Pts',(0.13392576920437,-8.12675387251257,
20.0884773999678));
#163936=CARTESIAN_POINT('Ctrl Pts',(0.33988368171443,-8.12074917529332,
20.0965374681885));
#163937=CARTESIAN_POINT('Ctrl Pts',(0.545333256425216,-8.10692908578437,
20.1045975364092));
#163938=CARTESIAN_POINT('Ctrl Pts',(0.753860772172276,-8.09290195072333,
20.1127783564726));
#163939=CARTESIAN_POINT('Ctrl Pts',(0.961864263866713,-8.07082337898981,
20.120959176536));
#163940=CARTESIAN_POINT('Ctrl Pts',(1.16870120791535,-8.0407602283066,20.1291399965995));
#163941=CARTESIAN_POINT('Ctrl Pts',(1.37250494796214,-8.01113794503893,
20.1372008473012));
#163942=CARTESIAN_POINT('Ctrl Pts',(1.57517580240228,-7.9737637259802,20.1452616980029));
#163943=CARTESIAN_POINT('Ctrl Pts',(1.7761068432484,-7.92875349874532,20.1533225487046));
#163944=CARTESIAN_POINT('Ctrl Pts',(1.97707120668057,-7.88373580697354,
20.1613847362251));
#163945=CARTESIAN_POINT('Ctrl Pts',(2.17629487176969,-7.831079650457,20.1694469237456));
#163946=CARTESIAN_POINT('Ctrl Pts',(2.37318297748875,-7.77095168675354,
20.1775091112661));
#163947=CARTESIAN_POINT('Ctrl Pts',(2.57012812623594,-7.71080630259132,
20.1855736345884));
#163948=CARTESIAN_POINT('Ctrl Pts',(2.76473606299467,-7.64318488615618,
20.1936381579107));
#163949=CARTESIAN_POINT('Ctrl Pts',(2.95642833990572,-7.5683035769915,20.201702681233));
#163950=CARTESIAN_POINT('Ctrl Pts',(3.15299393888453,-7.49151858791704,
20.2099722259579));
#163951=CARTESIAN_POINT('Ctrl Pts',(3.34649333758662,-7.40709981714679,
20.2182417706827));
#163952=CARTESIAN_POINT('Ctrl Pts',(3.53632615328153,-7.31533217975213,
20.2265113154076));
#163953=CARTESIAN_POINT('Ctrl Pts',(3.72170270630046,-7.22571875734863,
20.2345867353002));
#163954=CARTESIAN_POINT('Ctrl Pts',(3.90358262151928,-7.12909779781385,
20.2426621551928));
#163955=CARTESIAN_POINT('Ctrl Pts',(4.08143282956132,-7.02578064134364,
20.2507375750854));
#163956=CARTESIAN_POINT('Ctrl Pts',(4.26569604316778,-6.91873802676664,
20.2591041822264));
#163957=CARTESIAN_POINT('Ctrl Pts',(4.44563321745642,-6.80450753401025,
20.2674707893673));
#163958=CARTESIAN_POINT('Ctrl Pts',(4.62068516870312,-6.68348383212132,
20.2758373965083));
#163959=CARTESIAN_POINT('Ctrl Pts',(4.79573711994984,-6.56246013023236,
20.2842040036493));
#163960=CARTESIAN_POINT('Ctrl Pts',(4.96590357056133,-6.43464347433915,
20.2925706107903));
#163961=CARTESIAN_POINT('Ctrl Pts',(5.13066389792557,-6.3004742304864,20.3009372179313));
#163962=CARTESIAN_POINT('Ctrl Pts',(5.28973978601087,-6.17093399491485,
20.3090151665644));
#163963=CARTESIAN_POINT('Ctrl Pts',(5.44408564280906,-6.03522033485833,
20.3170931151974));
#163964=CARTESIAN_POINT('Ctrl Pts',(5.59320839334807,-5.893700656725,20.3251710638305));
#163965=CARTESIAN_POINT('Ctrl Pts',(5.74214864792508,-5.75235416993711,
20.3332391266949));
#163966=CARTESIAN_POINT('Ctrl Pts',(5.88587831053196,-5.60521604411245,
20.3413071895594));
#163967=CARTESIAN_POINT('Ctrl Pts',(6.02393636997626,-5.45269457910281,
20.3493752524238));
#163968=CARTESIAN_POINT('Ctrl Pts',(6.16184247109141,-5.30034099206478,
20.3574344348987));
#163969=CARTESIAN_POINT('Ctrl Pts',(6.29408920336521,-5.14261611089609,
20.3654936173736));
#163970=CARTESIAN_POINT('Ctrl Pts',(6.42025107695133,-4.97996623195432,
20.3735527998484));
#163971=CARTESIAN_POINT('Ctrl Pts',(6.54625090002091,-4.8175252710965,20.3816016305851));
#163972=CARTESIAN_POINT('Ctrl Pts',(6.66618126400666,-4.65017218087765,
20.3896504613218));
#163973=CARTESIAN_POINT('Ctrl Pts',(6.77965573911101,-4.47838761404583,
20.3976992920585));
#163974=CARTESIAN_POINT('Ctrl Pts',(6.89304438263525,-4.30673298428397,
20.405742034696));
#163975=CARTESIAN_POINT('Ctrl Pts',(6.99998669746815,-4.13065382148837,
20.4137847773335));
#163976=CARTESIAN_POINT('Ctrl Pts',(7.10013770665113,-3.95066223677636,
20.421827519971));
#163977=CARTESIAN_POINT('Ctrl Pts',(7.20020713906716,-3.7708172619855,20.4298637114919));
#163978=CARTESIAN_POINT('Ctrl Pts',(7.29349614738342,-3.58706649730646,
20.4378999030128));
#163979=CARTESIAN_POINT('Ctrl Pts',(7.37970397129483,-3.39994953764837,
20.4459360945336));
#163980=CARTESIAN_POINT('Ctrl Pts',(7.4285803278516,-3.29386177411235,20.4504922907617));
#163981=CARTESIAN_POINT('Ctrl Pts',(7.47518128976442,-3.18669247143071,
20.4550484869897));
#163982=CARTESIAN_POINT('Ctrl Pts',(7.51945855803589,-3.07854357716125,
20.4596046832177));
#163983=CARTESIAN_POINT('Ctrl Pts',(7.59483891164273,-2.89442422629621,
20.4673614328136));
#163984=CARTESIAN_POINT('Ctrl Pts',(7.66344208910574,-2.70756079826281,
20.4751181824095));
#163985=CARTESIAN_POINT('Ctrl Pts',(7.72507857473524,-2.5185012560383,20.4828749320054));
#163986=CARTESIAN_POINT('Ctrl Pts',(7.78673278871381,-2.32938733508789,
20.4906339126559));
#163987=CARTESIAN_POINT('Ctrl Pts',(7.84141621163983,-2.13807637330443,
20.4983928933064));
#163988=CARTESIAN_POINT('Ctrl Pts',(7.88898940919516,-1.94513075758588,
20.5061518739568));
#163989=CARTESIAN_POINT('Ctrl Pts',(7.936605053796,-1.75201298670952,20.513917777535));
#163990=CARTESIAN_POINT('Ctrl Pts',(7.97709772009937,-1.5572579879613,20.5216836811131));
#163991=CARTESIAN_POINT('Ctrl Pts',(8.01037906330588,-1.36143851298943,
20.5294495846912));
#163992=CARTESIAN_POINT('Ctrl Pts',(8.04367786171188,-1.16551633579244,
20.537219561284));
#163993=CARTESIAN_POINT('Ctrl Pts',(8.06975775261683,-0.968528914529841,
20.5449895378767));
#163994=CARTESIAN_POINT('Ctrl Pts',(8.08858232180068,-0.771053555827045,
20.5527595144694));
#163995=CARTESIAN_POINT('Ctrl Pts',(8.10742814851175,-0.573355199308356,
20.5605382652597));
#163996=CARTESIAN_POINT('Ctrl Pts',(8.1190022729157,-0.3751681520917,20.5683170160499));
#163997=CARTESIAN_POINT('Ctrl Pts',(8.1233203645512,-0.177070091680339,
20.5760957668402));
#163998=CARTESIAN_POINT('Ctrl Pts',(8.12465294777881,-0.115936105881015,
20.5784963256309));
#163999=CARTESIAN_POINT('Ctrl Pts',(8.12529486266356,-0.0548105630326315,
20.5808968844217));
#164000=CARTESIAN_POINT('Ctrl Pts',(8.12524756561721,0.0062896686347757,
20.5832974432124));
#164001=CARTESIAN_POINT('',(8.12952934429449,-0.00742862902943328,22.5832974432124));
#164002=CARTESIAN_POINT('Ctrl Pts',(8.13282513948647,0.00629553435497102,
20.5832974432124));
#164003=CARTESIAN_POINT('Ctrl Pts',(8.13377449793336,0.303304450376019,
20.5949556783097));
#164004=CARTESIAN_POINT('Ctrl Pts',(7.97387079026596,3.29181374846737,20.7123922235979));
#164005=CARTESIAN_POINT('Ctrl Pts',(5.18705264259532,7.30934400029911,20.8827179239816));
#164006=CARTESIAN_POINT('Ctrl Pts',(-0.307003826939621,8.45123659280713,
21.0942745443635));
#164007=CARTESIAN_POINT('Ctrl Pts',(-4.29449854831533,7.30169108010176,
21.2529420096499));
#164008=CARTESIAN_POINT('Ctrl Pts',(-7.27250765093382,4.34712832670042,
21.4116094749364));
#164009=CARTESIAN_POINT('Ctrl Pts',(-8.45799212067998,0.346168247782319,
21.5702769402227));
#164010=CARTESIAN_POINT('Ctrl Pts',(-7.60342709026192,-3.73828686763913,
21.7289444055092));
#164011=CARTESIAN_POINT('Ctrl Pts',(-4.87682214009204,-6.92632775896643,
21.8876118707956));
#164012=CARTESIAN_POINT('Ctrl Pts',(-0.996603673995455,-8.39788261494148,
22.0462793360821));
#164013=CARTESIAN_POINT('Ctrl Pts',(4.57239175033109,-7.70877801686285,
22.257835956464));
#164014=CARTESIAN_POINT('Ctrl Pts',(7.83647938259924,-3.73996568278254,
22.4368419921741));
#164015=CARTESIAN_POINT('Ctrl Pts',(8.13195251875851,-0.526615112399208,
22.5629588727887));
#164016=CARTESIAN_POINT('Ctrl Pts',(8.12952934429449,-0.00742862902943328,
22.5832974432124));
#164017=CARTESIAN_POINT('',(8.12524972840108,0.00210085977608716,24.5832973448731));
#164018=CARTESIAN_POINT('Ctrl Pts',(8.12524660770977,-0.00742471553580177,
22.5832974432124));
#164019=CARTESIAN_POINT('Ctrl Pts',(8.12542479040845,0.187569740615188,
22.590940205944));
#164020=CARTESIAN_POINT('Ctrl Pts',(8.11857947866919,0.382805355671729,
22.5985829686756));
#164021=CARTESIAN_POINT('Ctrl Pts',(8.10468543979817,0.577720939921199,
22.6062257314072));
#164022=CARTESIAN_POINT('Ctrl Pts',(8.09080312872884,0.77247199812196,22.6138620429689));
#164023=CARTESIAN_POINT('Ctrl Pts',(8.06988396792512,0.966903205231081,
22.6214983545305));
#164024=CARTESIAN_POINT('Ctrl Pts',(8.04195478485132,1.16045284303454,22.6291346660922));
#164025=CARTESIAN_POINT('Ctrl Pts',(8.01403914810007,1.35390860462911,22.6367672738599));
#164026=CARTESIAN_POINT('Ctrl Pts',(7.9791203079503,1.54648329159617,22.6443998816277));
#164027=CARTESIAN_POINT('Ctrl Pts',(7.93727699992421,1.73761946034627,22.6520324893954));
#164028=CARTESIAN_POINT('Ctrl Pts',(7.89544627498311,1.92869815078578,22.6596628018916));
#164029=CARTESIAN_POINT('Ctrl Pts',(7.84669530549005,2.11833883197029,22.6672931143878));
#164030=CARTESIAN_POINT('Ctrl Pts',(7.79115408820036,2.30599339470408,22.674923426884));
#164031=CARTESIAN_POINT('Ctrl Pts',(7.77653351531357,2.35539125355325,22.6769320169986));
#164032=CARTESIAN_POINT('Ctrl Pts',(7.76144268937172,2.40465154912763,22.6789406071132));
#164033=CARTESIAN_POINT('Ctrl Pts',(7.74588456348442,2.45376443279989,22.6809491972278));
#164034=CARTESIAN_POINT('Ctrl Pts',(7.68363537510436,2.65026863708177,22.6889857117365));
#164035=CARTESIAN_POINT('Ctrl Pts',(7.61392907563297,2.84432493762119,22.6970222262451));
#164036=CARTESIAN_POINT('Ctrl Pts',(7.53699450845214,3.03535851952652,22.7050587407538));
#164037=CARTESIAN_POINT('Ctrl Pts',(7.46001346513546,3.22650750472886,22.7131001101171));
#164038=CARTESIAN_POINT('Ctrl Pts',(7.37579556050196,3.41462983532245,22.7211414794804));
#164039=CARTESIAN_POINT('Ctrl Pts',(7.28461702904298,3.59917244692125,22.7291828488437));
#164040=CARTESIAN_POINT('Ctrl Pts',(7.19337226838382,3.78384910443377,22.7372300592033));
#164041=CARTESIAN_POINT('Ctrl Pts',(7.09515693347681,3.96494057246139,22.7452772695628));
#164042=CARTESIAN_POINT('Ctrl Pts',(6.99029256122135,4.14191953942051,22.7533244799224));
#164043=CARTESIAN_POINT('Ctrl Pts',(6.88527362637015,4.31915936073787,22.7613835512953));
#164044=CARTESIAN_POINT('Ctrl Pts',(6.77358622807121,4.49227429402328,22.7694426226682));
#164045=CARTESIAN_POINT('Ctrl Pts',(6.65559546828131,4.66076565867598,22.7775016940412));
#164046=CARTESIAN_POINT('Ctrl Pts',(6.53750921278107,4.829393391656,22.7855672880159));
#164047=CARTESIAN_POINT('Ctrl Pts',(6.41310960554954,4.99338983723397,22.7936328819907));
#164048=CARTESIAN_POINT('Ctrl Pts',(6.28280175711014,5.15228974761259,22.8016984759655));
#164049=CARTESIAN_POINT('Ctrl Pts',(6.1522892955766,5.31143916715515,22.8097767347655));
#164050=CARTESIAN_POINT('Ctrl Pts',(6.01585025820671,5.46547581907097,22.8178549935656));
#164051=CARTESIAN_POINT('Ctrl Pts',(5.87392750789945,5.6139703592415,22.8259332523657));
#164052=CARTESIAN_POINT('Ctrl Pts',(5.79379525622176,5.69781316696575,22.8304943890819));
#164053=CARTESIAN_POINT('Ctrl Pts',(5.71191545704096,5.77988988860286,22.8350555257981));
#164054=CARTESIAN_POINT('Ctrl Pts',(5.62837241333386,5.86012896951273,22.8396166625142));
#164055=CARTESIAN_POINT('Ctrl Pts',(5.48026344874251,6.00238051633197,22.8477028562464));
#164056=CARTESIAN_POINT('Ctrl Pts',(5.32663687057979,6.13913088424393,22.8557890499786));
#164057=CARTESIAN_POINT('Ctrl Pts',(5.16792796774153,6.26994482294181,22.8638752437108));
#164058=CARTESIAN_POINT('Ctrl Pts',(5.00936062571359,6.40064208181373,22.8719542249418));
#164059=CARTESIAN_POINT('Ctrl Pts',(4.8457202410562,6.52541326870424,22.8800332061729));
#164060=CARTESIAN_POINT('Ctrl Pts',(4.67747772977852,6.64386104986596,22.888112187404));
#164061=CARTESIAN_POINT('Ctrl Pts',(4.50936230842683,6.76221935590258,22.8961850657951));
#164062=CARTESIAN_POINT('Ctrl Pts',(4.33665195086314,6.87426359959673,22.9042579441861));
#164063=CARTESIAN_POINT('Ctrl Pts',(4.15984981173212,6.97963731911138,22.9123308225772));
#164064=CARTESIAN_POINT('Ctrl Pts',(3.98315712102488,7.08494580758546,22.9203987034959));
#164065=CARTESIAN_POINT('Ctrl Pts',(3.80237797166621,7.18359184517078,22.9284665844145));
#164066=CARTESIAN_POINT('Ctrl Pts',(3.61804412261134,7.2752624893771,22.9365344653332));
#164067=CARTESIAN_POINT('Ctrl Pts',(3.43379928103538,7.36688886947799,22.9445984505932));
#164068=CARTESIAN_POINT('Ctrl Pts',(3.24600344630447,7.45154643311539,22.9526624358533));
#164069=CARTESIAN_POINT('Ctrl Pts',(3.05521312959896,7.52896807638511,22.9607264211134));
#164070=CARTESIAN_POINT('Ctrl Pts',(2.86177143845073,7.60746563257234,22.9689024699456));
#164071=CARTESIAN_POINT('Ctrl Pts',(2.66525171009062,7.67852450396723,22.9770785187779));
#164072=CARTESIAN_POINT('Ctrl Pts',(2.46625633353229,7.74191625244111,22.9852545676101));
#164073=CARTESIAN_POINT('Ctrl Pts',(2.27008144123943,7.80440951054691,22.9933147322571));
#164074=CARTESIAN_POINT('Ctrl Pts',(2.07150092702902,7.85945145889397,23.001374896904));
#164075=CARTESIAN_POINT('Ctrl Pts',(1.87110888729118,7.90687290238056,23.009435061551));
#164076=CARTESIAN_POINT('Ctrl Pts',(1.67072652949127,7.95429205470093,23.0174948367712));
#164077=CARTESIAN_POINT('Ctrl Pts',(1.46853312899585,7.99409136367617,23.0255546119915));
#164078=CARTESIAN_POINT('Ctrl Pts',(1.26513496224844,8.02615232161692,23.0336143872117));
#164079=CARTESIAN_POINT('Ctrl Pts',(1.06172143868044,8.05821570020081,23.0416747709553));
#164080=CARTESIAN_POINT('Ctrl Pts',(0.857103280432245,8.0825395137122,23.0497351546988));
#164081=CARTESIAN_POINT('Ctrl Pts',(0.651894507060131,8.09905680398433,
23.0577955384424));
#164082=CARTESIAN_POINT('Ctrl Pts',(0.441527223964406,8.11598930361166,
23.0660585429961));
#164083=CARTESIAN_POINT('Ctrl Pts',(0.230539591331538,8.12471762147112,
23.0743215475498));
#164084=CARTESIAN_POINT('Ctrl Pts',(0.0195962091400046,8.12522636922119,
23.0825845521035));
#164085=CARTESIAN_POINT('Ctrl Pts',(-0.186343748433672,8.1257230498422,
23.0906515641593));
#164086=CARTESIAN_POINT('Ctrl Pts',(-0.392241209201706,8.11838569250262,
23.0987185762151));
#164087=CARTESIAN_POINT('Ctrl Pts',(-0.59747973076114,8.10325277489414,
23.1067855882709));
#164088=CARTESIAN_POINT('Ctrl Pts',(-0.81019782658627,8.08756836344206,
23.1151465890736));
#164089=CARTESIAN_POINT('Ctrl Pts',(-1.02220768026863,8.06350955838493,
23.1235075898763));
#164090=CARTESIAN_POINT('Ctrl Pts',(-1.23283064176945,8.03117775741605,
23.131868590679));
#164091=CARTESIAN_POINT('Ctrl Pts',(-1.44345360327031,7.99884595644717,
23.1402295914817));
#164092=CARTESIAN_POINT('Ctrl Pts',(-1.65268930698428,7.95824125502719,
23.1485905922844));
#164093=CARTESIAN_POINT('Ctrl Pts',(-1.85987240871919,7.90952351193073,
23.1569515930871));
#164094=CARTESIAN_POINT('Ctrl Pts',(-2.0476590513144,7.86536671857118,23.1645298379165));
#164095=CARTESIAN_POINT('Ctrl Pts',(-2.23413571045512,7.81445615747484,
23.172108082746));
#164096=CARTESIAN_POINT('Ctrl Pts',(-2.41875864124654,7.75688688830095,
23.1796863275755));
#164097=CARTESIAN_POINT('Ctrl Pts',(-2.60324418926097,7.69936045793389,
23.1872589332337));
#164098=CARTESIAN_POINT('Ctrl Pts',(-2.78587840456789,7.63518528525991,
23.1948315388919));
#164099=CARTESIAN_POINT('Ctrl Pts',(-2.96612795935251,7.56450741894324,
23.2024041445502));
#164100=CARTESIAN_POINT('Ctrl Pts',(-3.14627761461197,7.49386872434765,
23.209972553251));
#164101=CARTESIAN_POINT('Ctrl Pts',(-3.32404489826436,7.41673464122926,
23.2175409619518));
#164102=CARTESIAN_POINT('Ctrl Pts',(-3.49891193578316,7.33330095033159,
23.2251093706526));
#164103=CARTESIAN_POINT('Ctrl Pts',(-3.67373672402911,7.24988741767998,
23.2326759507654));
#164104=CARTESIAN_POINT('Ctrl Pts',(-3.84566232611258,7.16017745753476,
23.2402425308782));
#164105=CARTESIAN_POINT('Ctrl Pts',(-4.01419102258741,7.06441490830477,
23.247809110991));
#164106=CARTESIAN_POINT('Ctrl Pts',(-4.1826898228336,6.96866934691796,23.2553743488267));
#164107=CARTESIAN_POINT('Ctrl Pts',(-4.34779259874365,6.86687351797403,
23.2629395866624));
#164108=CARTESIAN_POINT('Ctrl Pts',(-4.50902666291086,6.75931698588393,
23.2705048244982));
#164109=CARTESIAN_POINT('Ctrl Pts',(-4.67031679589973,6.65172305122602,
23.2780726931301));
#164110=CARTESIAN_POINT('Ctrl Pts',(-4.82773522134604,6.53836461288113,
23.2856405617621));
#164111=CARTESIAN_POINT('Ctrl Pts',(-4.98083826730238,6.41957457449293,
23.293208430394));
#164112=CARTESIAN_POINT('Ctrl Pts',(-5.13196560016682,6.30231745814797,
23.3006786397205));
#164113=CARTESIAN_POINT('Ctrl Pts',(-5.2788880160263,6.1797683351468,23.308148849047));
#164114=CARTESIAN_POINT('Ctrl Pts',(-5.42121114614919,6.05228529328945,
23.3156190583735));
#164115=CARTESIAN_POINT('Ctrl Pts',(-5.59850691186894,5.89347622618373,
23.3249248998167));
#164116=CARTESIAN_POINT('Ctrl Pts',(-5.76857974752031,5.72709014944377,
23.33423074126));
#164117=CARTESIAN_POINT('Ctrl Pts',(-5.93088679969662,5.55376172802582,
23.3435365827032));
#164118=CARTESIAN_POINT('Ctrl Pts',(-6.09406524569156,5.37950274128128,
23.3528923853317));
#164119=CARTESIAN_POINT('Ctrl Pts',(-6.2493943065823,5.19822673571199,23.3622481879602));
#164120=CARTESIAN_POINT('Ctrl Pts',(-6.39636762042764,5.01060563473567,
23.3716039905888));
#164121=CARTESIAN_POINT('Ctrl Pts',(-6.54405440963679,4.822073735535,23.3810052105418));
#164122=CARTESIAN_POINT('Ctrl Pts',(-6.68330412251971,4.62713503538254,
23.3904064304948));
#164123=CARTESIAN_POINT('Ctrl Pts',(-6.81364856918951,4.4264975700978,23.3998076504478));
#164124=CARTESIAN_POINT('Ctrl Pts',(-6.94413408722986,4.22564295553717,
23.4092190453106));
#164125=CARTESIAN_POINT('Ctrl Pts',(-7.06569504966478,4.01907727607903,
23.4186304401733));
#164126=CARTESIAN_POINT('Ctrl Pts',(-7.17790734213764,3.80753644108451,
23.4280418350361));
#164127=CARTESIAN_POINT('Ctrl Pts',(-7.28998800770875,3.59624374703865,
23.4374421901748));
#164128=CARTESIAN_POINT('Ctrl Pts',(-7.39274190945744,3.379987596664,23.4468425453135));
#164129=CARTESIAN_POINT('Ctrl Pts',(-7.48579198072721,3.1595262277405,23.4562429004522));
#164130=CARTESIAN_POINT('Ctrl Pts',(-7.5453273351781,3.01847049761071,23.4622574415214));
#164131=CARTESIAN_POINT('Ctrl Pts',(-7.60089114414173,2.87569377480425,
23.4682719825907));
#164132=CARTESIAN_POINT('Ctrl Pts',(-7.65239452295604,2.73139993913971,
23.4742865236599));
#164133=CARTESIAN_POINT('Ctrl Pts',(-7.71869293690673,2.54565576724932,
23.4820288221792));
#164134=CARTESIAN_POINT('Ctrl Pts',(-7.77829123086381,2.35730935636452,
23.4897711206984));
#164135=CARTESIAN_POINT('Ctrl Pts',(-7.83098073752968,2.16689368704123,
23.4975134192177));
#164136=CARTESIAN_POINT('Ctrl Pts',(-7.88363742340425,1.97659662943663,
23.5052508949861));
#164137=CARTESIAN_POINT('Ctrl Pts',(-7.92939379701267,1.78423321891253,
23.5129883707545));
#164138=CARTESIAN_POINT('Ctrl Pts',(-7.968090237771,1.59035389936909,23.5207258465229));
#164139=CARTESIAN_POINT('Ctrl Pts',(-8.00676945162113,1.39656089115494,
23.5284598777165));
#164140=CARTESIAN_POINT('Ctrl Pts',(-8.03839492315798,1.20125366368059,
23.5361939089101));
#164141=CARTESIAN_POINT('Ctrl Pts',(-8.06285755130023,1.00499535816884,
23.5439279401037));
#164142=CARTESIAN_POINT('Ctrl Pts',(-8.08731704899631,0.808762167540782,
23.5516609815848));
#164143=CARTESIAN_POINT('Ctrl Pts',(-8.10461547775754,0.611578490696759,
23.5593940230659));
#164144=CARTESIAN_POINT('Ctrl Pts',(-8.11469523237386,0.414015516845526,
23.5671270645471));
#164145=CARTESIAN_POINT('Ctrl Pts',(-8.1247739800302,0.216472279388297,
23.5748593335031));
#164146=CARTESIAN_POINT('Ctrl Pts',(-8.12763547556959,0.0185501735186514,
23.5825916024591));
#164147=CARTESIAN_POINT('Ctrl Pts',(-8.12327417012775,-0.179176782634739,
23.5903238714152));
#164148=CARTESIAN_POINT('Ctrl Pts',(-8.11891118709006,-0.37697979535549,
23.5980591146234));
#164149=CARTESIAN_POINT('Ctrl Pts',(-8.10731986004562,-0.574587154785271,
23.6057943578316));
#164150=CARTESIAN_POINT('Ctrl Pts',(-8.0885467637086,-0.771426479840539,
23.6135296010399));
#164151=CARTESIAN_POINT('Ctrl Pts',(-8.07283271759351,-0.936191107670352,
23.6200043970087));
#164152=CARTESIAN_POINT('Ctrl Pts',(-8.05208766086729,-1.10041754659114,
23.6264791929775));
#164153=CARTESIAN_POINT('Ctrl Pts',(-8.02636671998218,-1.26377404580982,
23.6329539889464));
#164154=CARTESIAN_POINT('Ctrl Pts',(-7.9929420508541,-1.47605776282834,
23.6413680634508));
#164155=CARTESIAN_POINT('Ctrl Pts',(-7.95109761222765,-1.68697455658355,
23.6497821379552));
#164156=CARTESIAN_POINT('Ctrl Pts',(-7.90097292802332,-1.89586770454655,
23.6581962124596));
#164157=CARTESIAN_POINT('Ctrl Pts',(-7.85083424537385,-2.10481919061817,
23.6666126367834));
#164158=CARTESIAN_POINT('Ctrl Pts',(-7.79241076234982,-2.3117456459217,
23.6750290611073));
#164159=CARTESIAN_POINT('Ctrl Pts',(-7.72589250952882,-2.51600327776148,
23.6834454854312));
#164160=CARTESIAN_POINT('Ctrl Pts',(-7.65935776064481,-2.7203115640701,
23.6918639969697));
#164161=CARTESIAN_POINT('Ctrl Pts',(-7.58472431602536,-2.92194945462536,
23.7002825085081));
#164162=CARTESIAN_POINT('Ctrl Pts',(-7.50223155273221,-3.12028993711951,
23.7087010200466));
#164163=CARTESIAN_POINT('Ctrl Pts',(-7.41970710431301,-3.31870660136509,
23.7171227651002));
#164164=CARTESIAN_POINT('Ctrl Pts',(-7.32931740498692,-3.51382308231481,
23.7255445101538));
#164165=CARTESIAN_POINT('Ctrl Pts',(-7.23134987631622,-3.70503259483656,
23.7339662552074));
#164166=CARTESIAN_POINT('Ctrl Pts',(-7.13337172823285,-3.8962628339475,
23.7423889131551));
#164167=CARTESIAN_POINT('Ctrl Pts',(-7.02781423380644,-4.08358502552981,
23.7508115711029));
#164168=CARTESIAN_POINT('Ctrl Pts',(-6.91501093115956,-4.26641669137506,
23.7592342290507));
#164169=CARTESIAN_POINT('Ctrl Pts',(-6.80218617657099,-4.44928312654128,
23.7676584887456));
#164170=CARTESIAN_POINT('Ctrl Pts',(-6.68211299959844,-4.62765710536148,
23.7760827484405));
#164171=CARTESIAN_POINT('Ctrl Pts',(-6.55516915733622,-4.80098374098559,
23.7845070081354));
#164172=CARTESIAN_POINT('Ctrl Pts',(-6.51943366817024,-4.84977627789909,
23.7868784901679));
#164173=CARTESIAN_POINT('Ctrl Pts',(-6.48315396805183,-4.89816901507628,
23.7892499722003));
#164174=CARTESIAN_POINT('Ctrl Pts',(-6.44633908841521,-4.9461500098228,
23.7916214542328));
#164175=CARTESIAN_POINT('Ctrl Pts',(-6.31555989011196,-5.11659511486402,
23.8000457794529));
#164176=CARTESIAN_POINT('Ctrl Pts',(-6.17801053486217,-5.2818594915429,
23.808470104673));
#164177=CARTESIAN_POINT('Ctrl Pts',(-6.03411794096312,-5.44142520274303,
23.8168944298932));
#164178=CARTESIAN_POINT('Ctrl Pts',(-5.89025021346363,-5.60096333903729,
23.8253172992869));
#164179=CARTESIAN_POINT('Ctrl Pts',(-5.74004161340068,-5.75480458089382,
23.8337401686806));
#164180=CARTESIAN_POINT('Ctrl Pts',(-5.5839579273677,-5.90246570747238,
23.8421630380743));
#164181=CARTESIAN_POINT('Ctrl Pts',(-5.42790613729704,-6.05009665925273,
23.8505841862406));
#164182=CARTESIAN_POINT('Ctrl Pts',(-5.26598185035697,-6.1915498364416,
23.8590053344068));
#164183=CARTESIAN_POINT('Ctrl Pts',(-5.09868692850712,-6.32637962562876,
23.8674264825731));
#164184=CARTESIAN_POINT('Ctrl Pts',(-4.93143894396884,-6.46117158612539,
23.8758452680492));
#164185=CARTESIAN_POINT('Ctrl Pts',(-4.75882353938873,-6.58934370464174,
23.8842640535254));
#164186=CARTESIAN_POINT('Ctrl Pts',(-4.58137557411481,-6.71049069825778,
23.8926828390016));
#164187=CARTESIAN_POINT('Ctrl Pts',(-4.40397717774242,-6.83160385027193,
23.9010992727464));
#164188=CARTESIAN_POINT('Ctrl Pts',(-4.22174913378615,-6.94569564687138,
23.9095157064911));
#164189=CARTESIAN_POINT('Ctrl Pts',(-4.03525614485675,-7.05240351992821,
23.9179321402359));
#164190=CARTESIAN_POINT('Ctrl Pts',(-3.84883084204029,-7.15907266423074,
23.9263455193046));
#164191=CARTESIAN_POINT('Ctrl Pts',(-3.65814391431436,-7.25836310579939,
23.9347588983732));
#164192=CARTESIAN_POINT('Ctrl Pts',(-3.46378643510607,-7.34995721718672,
23.9431722774418));
#164193=CARTESIAN_POINT('Ctrl Pts',(-3.40898591626193,-7.37578284966323,
23.9455444914676));
#164194=CARTESIAN_POINT('Ctrl Pts',(-3.35389374188062,-7.40099690293442,
23.9479167054934));
#164195=CARTESIAN_POINT('Ctrl Pts',(-3.2985235105494,-7.42559291995278,
23.9502889195192));
#164196=CARTESIAN_POINT('Ctrl Pts',(-3.11797530822053,-7.5057942582956,
23.9580241044299));
#164197=CARTESIAN_POINT('Ctrl Pts',(-2.93438884552525,-7.57945627267954,
23.9657592893406));
#164198=CARTESIAN_POINT('Ctrl Pts',(-2.74828795142395,-7.64634559110154,
23.9734944742513));
#164199=CARTESIAN_POINT('Ctrl Pts',(-2.56224460431735,-7.71321422569356,
23.9812272672516));
#164200=CARTESIAN_POINT('Ctrl Pts',(-2.37368870625444,-7.77331421556117,
23.988960060252));
#164201=CARTESIAN_POINT('Ctrl Pts',(-2.18316345428642,-7.82646055981682,
23.9966928532524));
#164202=CARTESIAN_POINT('Ctrl Pts',(-1.99266326661282,-7.87959991247631,
24.0044246289756));
#164203=CARTESIAN_POINT('Ctrl Pts',(-1.80019458149582,-7.9257873474648,
24.0121564046987));
#164204=CARTESIAN_POINT('Ctrl Pts',(-1.60631525135556,-7.96488787590651,
24.0198881804219));
#164205=CARTESIAN_POINT('Ctrl Pts',(-1.41236654589798,-8.00400239558476,
24.0276227227855));
#164206=CARTESIAN_POINT('Ctrl Pts',(-1.21700653278392,-8.0360248681617,
24.0353572651491));
#164207=CARTESIAN_POINT('Ctrl Pts',(-1.02080340047309,-8.06087141567725,
24.0430918075127));
#164208=CARTESIAN_POINT('Ctrl Pts',(-0.824567131640385,-8.0857221594977,
24.0508276561542));
#164209=CARTESIAN_POINT('Ctrl Pts',(-0.627487811452396,-8.10339452658514,
24.0585635047958));
#164210=CARTESIAN_POINT('Ctrl Pts',(-0.43013840036865,-8.11385657496041,
24.0662993534374));
#164211=CARTESIAN_POINT('Ctrl Pts',(-0.232627509060942,-8.12432718385738,
24.0740415319006));
#164212=CARTESIAN_POINT('Ctrl Pts',(-0.0348464387509563,-8.12757567537919,
24.0817837103638));
#164213=CARTESIAN_POINT('Ctrl Pts',(0.162631259539863,-8.12362226078493,
24.089525888827));
#164214=CARTESIAN_POINT('Ctrl Pts',(0.327834100089828,-8.12031497430906,
24.0960027208199));
#164215=CARTESIAN_POINT('Ctrl Pts',(0.492824541233774,-8.11196843802761,
24.1024795528128));
#164216=CARTESIAN_POINT('Ctrl Pts',(0.657269933842987,-8.09862233942082,
24.1089563848056));
#164217=CARTESIAN_POINT('Ctrl Pts',(0.89588388638438,-8.07925685104171,
24.1183544132772));
#164218=CARTESIAN_POINT('Ctrl Pts',(1.13348584590962,-8.04935409446737,
24.1277524417488));
#164219=CARTESIAN_POINT('Ctrl Pts',(1.36923883430365,-8.00904941782324,
24.1371504702204));
#164220=CARTESIAN_POINT('Ctrl Pts',(1.60532727946876,-7.96868739099755,
24.1465618713));
#164221=CARTESIAN_POINT('Ctrl Pts',(1.83956145406953,-7.91789384362429,
24.1559732723795));
#164222=CARTESIAN_POINT('Ctrl Pts',(2.07111280434926,-7.85685556149281,
24.165384673459));
#164223=CARTESIAN_POINT('Ctrl Pts',(2.30231551498804,-7.79590918279761,
24.1747819040857));
#164224=CARTESIAN_POINT('Ctrl Pts',(2.53084344038941,-7.72474891151579,
24.1841791347124));
#164225=CARTESIAN_POINT('Ctrl Pts',(2.75588421315682,-7.64361104231325,
24.1935763653391));
#164226=CARTESIAN_POINT('Ctrl Pts',(2.98035734914987,-7.56267783308314,
24.2029498926447));
#164227=CARTESIAN_POINT('Ctrl Pts',(3.20136085931515,-7.4718172900622,24.2123234199504));
#164228=CARTESIAN_POINT('Ctrl Pts',(3.41810146809121,-7.37131398845095,
24.2216969472561));
#164229=CARTESIAN_POINT('Ctrl Pts',(3.63343457608372,-7.27146334937751,
24.2310096034259));
#164230=CARTESIAN_POINT('Ctrl Pts',(3.84455991957934,-7.16209478347236,
24.2403222595958));
#164231=CARTESIAN_POINT('Ctrl Pts',(4.05071305595546,-7.04353684598952,
24.2496349157657));
#164232=CARTESIAN_POINT('Ctrl Pts',(4.18345267265937,-6.96719876326461,
24.2556312272078));
#164233=CARTESIAN_POINT('Ctrl Pts',(4.31413112295855,-6.8870518356622,24.2616275386499));
#164234=CARTESIAN_POINT('Ctrl Pts',(4.44254749922859,-6.80319478477559,
24.2676238500921));
#164235=CARTESIAN_POINT('Ctrl Pts',(4.60461567298398,-6.69736280688885,
24.2751915083061));
#164236=CARTESIAN_POINT('Ctrl Pts',(4.76301482345829,-6.58566076221604,
24.2827591665201));
#164237=CARTESIAN_POINT('Ctrl Pts',(4.91727939477646,-6.4683885872918,24.2903268247341));
#164238=CARTESIAN_POINT('Ctrl Pts',(5.0715012530076,-6.35114888292493,24.2978923875996));
#164239=CARTESIAN_POINT('Ctrl Pts',(5.22159051755009,-6.22834233932318,
24.3054579504651));
#164240=CARTESIAN_POINT('Ctrl Pts',(5.36711158068566,-6.10031153655039,
24.3130235133306));
#164241=CARTESIAN_POINT('Ctrl Pts',(5.51261989480059,-5.97229195048613,
24.3205884133812));
#164242=CARTESIAN_POINT('Ctrl Pts',(5.65356052862592,-5.83904925973904,
24.3281533134319));
#164243=CARTESIAN_POINT('Ctrl Pts',(5.78953192706015,-5.70096549963698,
24.3357182134826));
#164244=CARTESIAN_POINT('Ctrl Pts',(5.92557005941518,-5.56281396888009,
24.3432868263393));
#164245=CARTESIAN_POINT('Ctrl Pts',(6.05663382334175,-5.41981688213972,
24.3508554391961));
#164246=CARTESIAN_POINT('Ctrl Pts',(6.18235905565871,-5.27239263232688,
24.3584240520529));
#164247=CARTESIAN_POINT('Ctrl Pts',(6.30811224705745,-5.12493559795217,
24.3659943480362));
#164248=CARTESIAN_POINT('Ctrl Pts',(6.42852431209391,-4.97304972648763,
24.3735646440194));
#164249=CARTESIAN_POINT('Ctrl Pts',(6.54327239428554,-4.81718527115999,
24.3811349400027));
#164250=CARTESIAN_POINT('Ctrl Pts',(6.65813674899674,-4.66116288070536,
24.3887129068539));
#164251=CARTESIAN_POINT('Ctrl Pts',(6.76732544559469,-4.50115415480637,
24.3962908737051));
#164252=CARTESIAN_POINT('Ctrl Pts',(6.87055937175272,-4.33763777668455,
24.4038688405563));
#164253=CARTESIAN_POINT('Ctrl Pts',(6.97237912347573,-4.17636136647107,
24.4113429988304));
#164254=CARTESIAN_POINT('Ctrl Pts',(7.06840609847094,-4.01167311764415,
24.4188171571044));
#164255=CARTESIAN_POINT('Ctrl Pts',(7.15841748436539,-3.84405341820739,
24.4262913153785));
#164256=CARTESIAN_POINT('Ctrl Pts',(7.26188771774732,-3.65137057872229,
24.4348830384507));
#164257=CARTESIAN_POINT('Ctrl Pts',(7.3575986811752,-3.45446294962123,24.4434747615229));
#164258=CARTESIAN_POINT('Ctrl Pts',(7.44523300044756,-3.25395038861175,
24.4520664845951));
#164259=CARTESIAN_POINT('Ctrl Pts',(7.5328002175112,-3.053591361467,24.460651628925));
#164260=CARTESIAN_POINT('Ctrl Pts',(7.61230304488907,-2.84963312958498,
24.469236773255));
#164261=CARTESIAN_POINT('Ctrl Pts',(7.68347137690855,-2.64271738230312,
24.477821917585));
#164262=CARTESIAN_POINT('Ctrl Pts',(7.75633467562903,-2.43087366647677,
24.4866115283307));
#164263=CARTESIAN_POINT('Ctrl Pts',(7.82046144178498,-2.21593003026772,
24.4954011390765));
#164264=CARTESIAN_POINT('Ctrl Pts',(7.87561412889134,-1.99859692166958,
24.5041907498222));
#164265=CARTESIAN_POINT('Ctrl Pts',(7.92934991502028,-1.78684721272346,
24.5127545509346));
#164266=CARTESIAN_POINT('Ctrl Pts',(7.97456692045833,-1.57282952820372,
24.5213183520469));
#164267=CARTESIAN_POINT('Ctrl Pts',(8.01109526635494,-1.35721781445919,
24.5298821531592));
#164268=CARTESIAN_POINT('Ctrl Pts',(8.04906837707402,-1.13307825167902,
24.5387846687216));
#164269=CARTESIAN_POINT('Ctrl Pts',(8.07765147264861,-0.907216233308902,
24.5476871842841));
#164270=CARTESIAN_POINT('Ctrl Pts',(8.09671154652852,-0.680404067309817,
24.5565896998465));
#164271=CARTESIAN_POINT('Ctrl Pts',(8.11577162040843,-0.453591901310732,
24.5654922154089));
#164272=CARTESIAN_POINT('Ctrl Pts',(8.12530859140817,-0.225829868379238,
24.5743947309714));
#164273=CARTESIAN_POINT('Ctrl Pts',(8.12524972905207,0.00209834202667678,
24.5832972465338));
#164274=CARTESIAN_POINT('',(8.12524906564331,0.00389663476247341,26.5832974432124));
#164275=CARTESIAN_POINT('Ctrl Pts',(8.1252497277501,0.00210337752549754,
24.5832974432124));
#164276=CARTESIAN_POINT('Ctrl Pts',(8.12519425373155,0.216396935667924,
24.5916674107232));
#164277=CARTESIAN_POINT('Ctrl Pts',(8.11665690499827,0.430542956075556,
24.600037378234));
#164278=CARTESIAN_POINT('Ctrl Pts',(8.09969814556991,0.643876939446739,
24.6084073457449));
#164279=CARTESIAN_POINT('Ctrl Pts',(8.0827194136445,0.857462168339349,24.6167871706484));
#164280=CARTESIAN_POINT('Ctrl Pts',(8.05729948082891,1.0702331833302,24.6251669955519));
#164281=CARTESIAN_POINT('Ctrl Pts',(8.02355045062957,1.28153257028528,24.6335468204554));
#164282=CARTESIAN_POINT('Ctrl Pts',(7.9897621507523,1.4930778208644,24.641936395951));
#164283=CARTESIAN_POINT('Ctrl Pts',(7.94762543634056,1.70314775912192,24.6503259714466));
#164284=CARTESIAN_POINT('Ctrl Pts',(7.89730330546843,1.9110960373402,24.6587155469422));
#164285=CARTESIAN_POINT('Ctrl Pts',(7.84689148431164,2.11941494653026,24.66712007537));
#164286=CARTESIAN_POINT('Ctrl Pts',(7.78826513417819,2.32560437296713,24.6755246037978));
#164287=CARTESIAN_POINT('Ctrl Pts',(7.72163751836189,2.52903175099207,24.6839291322256));
#164288=CARTESIAN_POINT('Ctrl Pts',(7.65494828323145,2.73264726505277,24.6923414334256));
#164289=CARTESIAN_POINT('Ctrl Pts',(7.58024309317629,2.93349537735955,24.7007537346256));
#164290=CARTESIAN_POINT('Ctrl Pts',(7.49778366339738,3.13096274321355,24.7091660358256));
#164291=CARTESIAN_POINT('Ctrl Pts',(7.41520770443899,3.32870916399406,24.717590225036));
#164292=CARTESIAN_POINT('Ctrl Pts',(7.32485570562134,3.52306504198502,24.7260144142463));
#164293=CARTESIAN_POINT('Ctrl Pts',(7.22703660311154,3.71343903946006,24.7344386034567));
#164294=CARTESIAN_POINT('Ctrl Pts',(7.19147524044649,3.7826480036859,24.7375011509549));
#164295=CARTESIAN_POINT('Ctrl Pts',(7.15492743429019,3.85133096343416,24.7405636984531));
#164296=CARTESIAN_POINT('Ctrl Pts',(7.11740948051402,3.91946040280918,24.7436262459513));
#164297=CARTESIAN_POINT('Ctrl Pts',(7.01845000197587,4.09916246848877,24.7517041945844));
#164298=CARTESIAN_POINT('Ctrl Pts',(6.91256985386025,4.2753164785814,24.7597821432174));
#164299=CARTESIAN_POINT('Ctrl Pts',(6.80004220534934,4.4473715347346,24.7678600918505));
#164300=CARTESIAN_POINT('Ctrl Pts',(6.68765226782676,4.61921603044206,24.775928154715));
#164301=CARTESIAN_POINT('Ctrl Pts',(6.56863121752924,4.78697130925881,24.7839962175795));
#164302=CARTESIAN_POINT('Ctrl Pts',(6.4432981979165,4.95011069524975,24.792064280444));
#164303=CARTESIAN_POINT('Ctrl Pts',(6.31810313038334,5.11307051628942,24.8001234629189));
#164304=CARTESIAN_POINT('Ctrl Pts',(6.18661013476264,5.27142432407205,24.8081826453937));
#164305=CARTESIAN_POINT('Ctrl Pts',(6.04918209785142,5.4246735855288,24.8162418278685));
#164306=CARTESIAN_POINT('Ctrl Pts',(5.91193058244908,5.57772600366686,24.8242906586052));
#164307=CARTESIAN_POINT('Ctrl Pts',(5.76875944385984,5.72568672171993,24.832339489342));
#164308=CARTESIAN_POINT('Ctrl Pts',(5.62007236464318,5.86808948284483,24.8403883200787));
#164309=CARTESIAN_POINT('Ctrl Pts',(5.4714977516622,6.01038453116388,24.8484310627161));
#164310=CARTESIAN_POINT('Ctrl Pts',(5.31741574139684,6.14712978477373,24.8564738053536));
#164311=CARTESIAN_POINT('Ctrl Pts',(5.15826838948651,6.27789413613548,24.8645165479911));
#164312=CARTESIAN_POINT('Ctrl Pts',(4.99925066908542,6.40855197501042,24.8725527395119));
#164313=CARTESIAN_POINT('Ctrl Pts',(4.83517608049207,6.53323842964819,24.8805889310327));
#164314=CARTESIAN_POINT('Ctrl Pts',(4.66652163703117,6.65156097270557,24.8886251225535));
#164315=CARTESIAN_POINT('Ctrl Pts',(4.57090137497581,6.71864507877495,24.8931813187816));
#164316=CARTESIAN_POINT('Ctrl Pts',(4.47380958691757,6.78368424989858,24.8977375150097));
#164317=CARTESIAN_POINT('Ctrl Pts',(4.37533792323006,6.84661271141029,24.9022937112378));
#164318=CARTESIAN_POINT('Ctrl Pts',(4.2016472140727,6.95761001456172,24.9103302257465));
#164319=CARTESIAN_POINT('Ctrl Pts',(4.02379913650775,7.0619502142526,24.9183667402552));
#164320=CARTESIAN_POINT('Ctrl Pts',(3.84233766798678,7.15933857333692,24.9264032547638));
#164321=CARTESIAN_POINT('Ctrl Pts',(3.6607665786784,7.25678576468295,24.9344446241271));
#164322=CARTESIAN_POINT('Ctrl Pts',(3.47557802179457,7.34727258763503,24.9424859934904));
#164323=CARTESIAN_POINT('Ctrl Pts',(3.28733842738293,7.43055136758717,24.9505273628537));
#164324=CARTESIAN_POINT('Ctrl Pts',(3.09896210168703,7.51389063860958,24.9585745732132));
#164325=CARTESIAN_POINT('Ctrl Pts',(2.9075306054883,7.59001129326978,24.9666217835727));
#164326=CARTESIAN_POINT('Ctrl Pts',(2.71362865353334,7.65871445434695,24.9746689939322));
#164327=CARTESIAN_POINT('Ctrl Pts',(2.51944090394765,7.72751887897748,24.9827280653051));
#164328=CARTESIAN_POINT('Ctrl Pts',(2.32277571896713,7.78888385336661,24.9907871366781));
#164329=CARTESIAN_POINT('Ctrl Pts',(2.12423292010315,7.84266039451219,24.998846208051));
#164330=CARTESIAN_POINT('Ctrl Pts',(1.92552943081086,7.89648045965097,25.0069118020258));
#164331=CARTESIAN_POINT('Ctrl Pts',(1.72494560219532,7.94269976449133,25.0149773960006));
#164332=CARTESIAN_POINT('Ctrl Pts',(1.52309055541323,7.98122062860757,25.0230429899754));
#164333=CARTESIAN_POINT('Ctrl Pts',(1.32091855008999,8.01980197928131,25.0311212487755));
#164334=CARTESIAN_POINT('Ctrl Pts',(1.1174716486926,8.0506606792476,25.0391995075756));
#164335=CARTESIAN_POINT('Ctrl Pts',(0.913364956665286,8.07375080234929,
25.0472777663756));
#164336=CARTESIAN_POINT('Ctrl Pts',(0.798122483000528,8.08678791973644,
25.0518389030918));
#164337=CARTESIAN_POINT('Ctrl Pts',(0.682669701434189,8.0973494052993,25.056400039808));
#164338=CARTESIAN_POINT('Ctrl Pts',(0.567117184085187,8.10543432901749,
25.0609611765242));
#164339=CARTESIAN_POINT('Ctrl Pts',(0.362260346926869,8.11976765502001,
25.0690473702564));
#164340=CARTESIAN_POINT('Ctrl Pts',(0.156691465199783,8.12634211374536,
25.0771335639886));
#164341=CARTESIAN_POINT('Ctrl Pts',(-0.0489763871425417,8.12510239172421,
25.0852197577207));
#164342=CARTESIAN_POINT('Ctrl Pts',(-0.254460793520063,8.12386377547628,
25.0932987389518));
#164343=CARTESIAN_POINT('Ctrl Pts',(-0.460043679226377,8.11482487766477,
25.1013777201829));
#164344=CARTESIAN_POINT('Ctrl Pts',(-0.665108907424412,8.0979823230089,
25.109456701414));
#164345=CARTESIAN_POINT('Ctrl Pts',(-0.870019229918433,8.08115249117206,
25.1175295798051));
#164346=CARTESIAN_POINT('Ctrl Pts',(-1.07441236006256,8.05653078317278,
25.1256024581962));
#164347=CARTESIAN_POINT('Ctrl Pts',(-1.27767359326996,8.02416586017267,
25.1336753365873));
#164348=CARTESIAN_POINT('Ctrl Pts',(-1.48080899869202,7.99182097250601,
25.1417432175059));
#164349=CARTESIAN_POINT('Ctrl Pts',(-1.68281359250667,7.95174247887163,
25.1498110984246));
#164350=CARTESIAN_POINT('Ctrl Pts',(-1.88307858900344,7.90403078119872,
25.1578789793432));
#164351=CARTESIAN_POINT('Ctrl Pts',(-2.08324688550376,7.85634212160574,
25.1659429646033));
#164352=CARTESIAN_POINT('Ctrl Pts',(-2.2816769524035,7.8010276825022,25.1740069498633));
#164353=CARTESIAN_POINT('Ctrl Pts',(-2.47777036642716,7.73823891940249,
25.1820709351234));
#164354=CARTESIAN_POINT('Ctrl Pts',(-2.67658885096461,7.67457759356133,
25.1902469839556));
#164355=CARTESIAN_POINT('Ctrl Pts',(-2.87300493183574,7.60323272679547,
25.1984230327879));
#164356=CARTESIAN_POINT('Ctrl Pts',(-3.06640973223818,7.52441485542464,
25.2065990816201));
#164357=CARTESIAN_POINT('Ctrl Pts',(-3.25707328706062,7.44671411838073,
25.2146592462671));
#164358=CARTESIAN_POINT('Ctrl Pts',(-3.4448100598985,7.36175094502759,25.222719410914));
#164359=CARTESIAN_POINT('Ctrl Pts',(-3.62905549654197,7.26977604644864,
25.230779575561));
#164360=CARTESIAN_POINT('Ctrl Pts',(-3.81329203137077,7.17780559163513,
25.2388393507812));
#164361=CARTESIAN_POINT('Ctrl Pts',(-3.99403728309498,7.0788242288538,25.2468991260015));
#164362=CARTESIAN_POINT('Ctrl Pts',(-4.17074981954013,6.97312939112032,
25.2549589012217));
#164363=CARTESIAN_POINT('Ctrl Pts',(-4.34747569800599,6.86742657329247,
25.2630192849653));
#164364=CARTESIAN_POINT('Ctrl Pts',(-4.52016798236891,6.7550094326517,25.2710796687088));
#164365=CARTESIAN_POINT('Ctrl Pts',(-4.68831232156532,6.63621994345868,
25.2791400524523));
#164366=CARTESIAN_POINT('Ctrl Pts',(-4.86068344987307,6.51444434053824,
25.287403057006));
#164367=CARTESIAN_POINT('Ctrl Pts',(-5.02827469447822,6.38597201126693,
25.2956660615597));
#164368=CARTESIAN_POINT('Ctrl Pts',(-5.19056590735157,6.25121693144139,
25.3039290661135));
#164369=CARTESIAN_POINT('Ctrl Pts',(-5.34900768991199,6.11965814474792,
25.3119960781692));
#164370=CARTESIAN_POINT('Ctrl Pts',(-5.50239778719732,5.98211150095628,
25.320063090225));
#164371=CARTESIAN_POINT('Ctrl Pts',(-5.6502875377432,5.83900148170249,25.3281301022808));
#164372=CARTESIAN_POINT('Ctrl Pts',(-5.80356688262015,5.69067605742136,
25.3364911030835));
#164373=CARTESIAN_POINT('Ctrl Pts',(-5.95093718245841,5.53637440841922,
25.3448521038862));
#164374=CARTESIAN_POINT('Ctrl Pts',(-6.09194232304138,5.37660918193216,
25.3532131046889));
#164375=CARTESIAN_POINT('Ctrl Pts',(-6.23294746362432,5.21684395544513,
25.3615741054916));
#164376=CARTESIAN_POINT('Ctrl Pts',(-6.36758722539411,5.05161545900265,
25.3699351062943));
#164377=CARTESIAN_POINT('Ctrl Pts',(-6.4954531649779,4.88147270237974,25.378296107097));
#164378=CARTESIAN_POINT('Ctrl Pts',(-6.61134830939662,4.72725869187157,
25.3858743519265));
#164379=CARTESIAN_POINT('Ctrl Pts',(-6.72191067443861,4.56869831513259,
25.3934525967559));
#164380=CARTESIAN_POINT('Ctrl Pts',(-6.82678366733251,4.40621292290126,
25.4010308415854));
#164381=CARTESIAN_POINT('Ctrl Pts',(-6.9315786214752,4.24384844032217,25.4086034472436));
#164382=CARTESIAN_POINT('Ctrl Pts',(-7.03069242767589,4.07756505928574,
25.4161760529018));
#164383=CARTESIAN_POINT('Ctrl Pts',(-7.12380915881508,3.90781660665932,
25.4237486585601));
#164384=CARTESIAN_POINT('Ctrl Pts',(-7.21687428196408,3.73816223354332,
25.4313170672609));
#164385=CARTESIAN_POINT('Ctrl Pts',(-7.30394876770481,3.5650469313644,25.4388854759616));
#164386=CARTESIAN_POINT('Ctrl Pts',(-7.38476041616239,3.38895281147158,
25.4464538846624));
#164387=CARTESIAN_POINT('Ctrl Pts',(-7.46555253988048,3.2129012373241,25.4540204647752));
#164388=CARTESIAN_POINT('Ctrl Pts',(-7.54008467769878,3.03387260823567,
25.4615870448881));
#164389=CARTESIAN_POINT('Ctrl Pts',(-7.60813089433697,2.85237302208797,
25.4691536250009));
#164390=CARTESIAN_POINT('Ctrl Pts',(-7.67616503988421,2.67090563314568,
25.4767188628366));
#164391=CARTESIAN_POINT('Ctrl Pts',(-7.73771542824444,2.48696850503807,
25.4842841006724));
#164392=CARTESIAN_POINT('Ctrl Pts',(-7.79260463949582,2.30108680736043,
25.4918493385081));
#164393=CARTESIAN_POINT('Ctrl Pts',(-7.84751293835988,2.11514046969674,
25.4994172071401));
#164394=CARTESIAN_POINT('Ctrl Pts',(-7.89575532499491,1.9272485636824,25.506985075772));
#164395=CARTESIAN_POINT('Ctrl Pts',(-7.93720442422442,1.73795094596259,
25.514552944404));
#164396=CARTESIAN_POINT('Ctrl Pts',(-7.97811864495121,1.55109611296469,
25.5220231537305));
#164397=CARTESIAN_POINT('Ctrl Pts',(-8.01241382660653,1.36287197969354,
25.529493363057));
#164398=CARTESIAN_POINT('Ctrl Pts',(-8.04001658451674,1.17380615230786,
25.5369635723835));
#164399=CARTESIAN_POINT('Ctrl Pts',(-8.0744020852813,0.938281746620939,
25.5462694138267));
#164400=CARTESIAN_POINT('Ctrl Pts',(-8.0983873350054,0.701567142603875,
25.5555752552699));
#164401=CARTESIAN_POINT('Ctrl Pts',(-8.11196213589248,0.46449743631869,
25.5648810967131));
#164402=CARTESIAN_POINT('Ctrl Pts',(-8.12560981714687,0.226154950608267,
25.5742368993416));
#164403=CARTESIAN_POINT('Ctrl Pts',(-8.12873501736658,-0.012546411925814,
25.5835927019701));
#164404=CARTESIAN_POINT('Ctrl Pts',(-8.12137942789707,-0.250766326747155,
25.5929485045987));
#164405=CARTESIAN_POINT('Ctrl Pts',(-8.11398813104817,-0.490142669467328,
25.6023497245517));
#164406=CARTESIAN_POINT('Ctrl Pts',(-8.09601406568459,-0.729032837388664,
25.6117509445047));
#164407=CARTESIAN_POINT('Ctrl Pts',(-8.06755136842397,-0.966593234168639,
25.6211521644577));
#164408=CARTESIAN_POINT('Ctrl Pts',(-8.03905786607876,-1.20441074179269,
25.6305635593205));
#164409=CARTESIAN_POINT('Ctrl Pts',(-8.00005304104605,-1.44089556401629,
25.6399749541832));
#164410=CARTESIAN_POINT('Ctrl Pts',(-7.9506827295727,-1.67521094079952,
25.649386349046));
#164411=CARTESIAN_POINT('Ctrl Pts',(-7.90137033030281,-1.90925146171552,
25.6587867041847));
#164412=CARTESIAN_POINT('Ctrl Pts',(-7.84171675979681,-2.1411275890458,
25.6681870593234));
#164413=CARTESIAN_POINT('Ctrl Pts',(-7.77191828339444,-2.37001556086435,
25.6775874144622));
#164414=CARTESIAN_POINT('Ctrl Pts',(-7.72725977882757,-2.51646280529752,
25.6836019555314));
#164415=CARTESIAN_POINT('Ctrl Pts',(-7.67844927289484,-2.66168699044815,
25.6896164966007));
#164416=CARTESIAN_POINT('Ctrl Pts',(-7.62554913898239,-2.80547462855483,
25.6956310376699));
#164417=CARTESIAN_POINT('Ctrl Pts',(-7.55745273333087,-2.99056719086086,
25.7033733361892));
#164418=CARTESIAN_POINT('Ctrl Pts',(-7.48254469812438,-3.1733652034248,
25.7111156347085));
#164419=CARTESIAN_POINT('Ctrl Pts',(-7.40100628188632,-3.35332574886175,
25.7188579332277));
#164420=CARTESIAN_POINT('Ctrl Pts',(-7.31951865669797,-3.53317419517499,
25.7265954089961));
#164421=CARTESIAN_POINT('Ctrl Pts',(-7.23140901920778,-3.7101883731819,
25.7343328847645));
#164422=CARTESIAN_POINT('Ctrl Pts',(-7.13690746498119,-3.88384337979735,
25.7420703605329));
#164423=CARTESIAN_POINT('Ctrl Pts',(-7.0424479810221,-4.05742107855643,
25.7498043917264));
#164424=CARTESIAN_POINT('Ctrl Pts',(-6.94160241609006,-4.22764227461244,
25.75753842292));
#164425=CARTESIAN_POINT('Ctrl Pts',(-6.83464779015968,-4.39400468217382,
25.7652724541136));
#164426=CARTESIAN_POINT('Ctrl Pts',(-6.72770685105335,-4.56034580058589,
25.7730054955947));
#164427=CARTESIAN_POINT('Ctrl Pts',(-6.61465859256753,-4.72282881294278,
25.7807385370758));
#164428=CARTESIAN_POINT('Ctrl Pts',(-6.4958247300516,-4.88097824610498,
25.7884715785569));
#164429=CARTESIAN_POINT('Ctrl Pts',(-6.37700273894996,-5.03911188025669,
25.7962038475129));
#164430=CARTESIAN_POINT('Ctrl Pts',(-6.25239651026016,-5.19291251718738,
25.8039361164689));
#164431=CARTESIAN_POINT('Ctrl Pts',(-6.12236954133246,-5.34193586276217,
25.811668385425));
#164432=CARTESIAN_POINT('Ctrl Pts',(-5.99229255694347,-5.49101653084038,
25.8194036286332));
#164433=CARTESIAN_POINT('Ctrl Pts',(-5.85679089893089,-5.63531596964487,
25.8271388718414));
#164434=CARTESIAN_POINT('Ctrl Pts',(-5.71626703704535,-5.77442453614979,
25.8348741150497));
#164435=CARTESIAN_POINT('Ctrl Pts',(-5.59864134513404,-5.89086555311572,
25.8413489110186));
#164436=CARTESIAN_POINT('Ctrl Pts',(-5.47749757611778,-6.00367010908838,
25.8478237069875));
#164437=CARTESIAN_POINT('Ctrl Pts',(-5.35309060059063,-6.11261879920286,
25.8542985029564));
#164438=CARTESIAN_POINT('Ctrl Pts',(-5.19142225366823,-6.2541989200565,
25.8627125774608));
#164439=CARTESIAN_POINT('Ctrl Pts',(-5.02416484090899,-6.38933518021291,
25.8711266519651));
#164440=CARTESIAN_POINT('Ctrl Pts',(-4.85184623503741,-6.51761272814312,
25.8795407264695));
#164441=CARTESIAN_POINT('Ctrl Pts',(-4.67947950532052,-6.64592610046295,
25.8879571507934));
#164442=CARTESIAN_POINT('Ctrl Pts',(-4.50204897257131,-6.76737677901806,
25.8963735751173));
#164443=CARTESIAN_POINT('Ctrl Pts',(-4.32011300543683,-6.88159219823113,
25.9047899994412));
#164444=CARTESIAN_POINT('Ctrl Pts',(-4.1381319194507,-6.99583594207202,
25.9132085109796));
#164445=CARTESIAN_POINT('Ctrl Pts',(-3.95164339201225,-7.10284070410267,
25.9216270225181));
#164446=CARTESIAN_POINT('Ctrl Pts',(-3.76123292994817,-7.20227841791564,
25.9300455340565));
#164447=CARTESIAN_POINT('Ctrl Pts',(-3.57074933202065,-7.30175432533931,
25.9384672791101));
#164448=CARTESIAN_POINT('Ctrl Pts',(-3.37634102263371,-7.39365725306045,
25.9468890241637));
#164449=CARTESIAN_POINT('Ctrl Pts',(-3.17861743884908,-7.47770544618766,
25.9553107692173));
#164450=CARTESIAN_POINT('Ctrl Pts',(-2.98087242236817,-7.56176274990937,
25.9637334271651));
#164451=CARTESIAN_POINT('Ctrl Pts',(-2.77981165806754,-7.63796351858892,
25.9721560851128));
#164452=CARTESIAN_POINT('Ctrl Pts',(-2.57606441916061,-7.70607420615937,
25.9805787430605));
#164453=CARTESIAN_POINT('Ctrl Pts',(-2.37227843339153,-7.77419784642274,
25.9890030027555));
#164454=CARTESIAN_POINT('Ctrl Pts',(-2.1658052027137,-7.83422824840479,
25.9974272624504));
#164455=CARTESIAN_POINT('Ctrl Pts',(-1.95729027524906,-7.88598138096429,
26.0058515221453));
#164456=CARTESIAN_POINT('Ctrl Pts',(-1.89859201309983,-7.90055021293694,
26.0082230041778));
#164457=CARTESIAN_POINT('Ctrl Pts',(-1.83973203903542,-7.91446341189762,
26.0105944862103));
#164458=CARTESIAN_POINT('Ctrl Pts',(-1.78072493887738,-7.92771759427391,
26.0129659682427));
#164459=CARTESIAN_POINT('Ctrl Pts',(-1.57111129002023,-7.97480103886061,
26.0213902934629));
#164460=CARTESIAN_POINT('Ctrl Pts',(-1.3596185723426,-8.01356919200245,
26.029814618683));
#164461=CARTESIAN_POINT('Ctrl Pts',(-1.14690640793186,-8.04389788932858,
26.0382389439031));
#164462=CARTESIAN_POINT('Ctrl Pts',(-0.934231002784703,-8.07422134548488,
26.0466618132968));
#164463=CARTESIAN_POINT('Ctrl Pts',(-0.720336832960184,-8.09610822154253,
26.0550846826904));
#164464=CARTESIAN_POINT('Ctrl Pts',(-0.505891122389207,-8.10948591063501,
26.0635075520841));
#164465=CARTESIAN_POINT('Ctrl Pts',(-0.291489234159958,-8.12286086597422,
26.0719287002503));
#164466=CARTESIAN_POINT('Ctrl Pts',(-0.0765362935174903,-8.12773009032672,
26.0803498484164));
#164467=CARTESIAN_POINT('Ctrl Pts',(0.138296870498141,-8.12407296484408,
26.0887709965826));
#164468=CARTESIAN_POINT('Ctrl Pts',(0.353069759577974,-8.12041686542743,
26.0971897820588));
#164469=CARTESIAN_POINT('Ctrl Pts',(0.567722675450266,-8.10823919853883,
26.1056085675349));
#164470=CARTESIAN_POINT('Ctrl Pts',(0.781585291870921,-8.08757145217469,
26.1140273530111));
#164471=CARTESIAN_POINT('Ctrl Pts',(0.995388167201144,-8.06690947920716,
26.1224437867559));
#164472=CARTESIAN_POINT('Ctrl Pts',(1.20840092136047,-8.03776218737824,
26.1308602205007));
#164473=CARTESIAN_POINT('Ctrl Pts',(1.41995768024003,-8.00021298146664,
26.1392766542455));
#164474=CARTESIAN_POINT('Ctrl Pts',(1.63143765631525,-7.96267740373382,
26.1476900333141));
#164475=CARTESIAN_POINT('Ctrl Pts',(1.84146243275004,-7.91674604760285,
26.1561034123828));
#164476=CARTESIAN_POINT('Ctrl Pts',(2.04937467982987,-7.86255371900073,
26.1645167914514));
#164477=CARTESIAN_POINT('Ctrl Pts',(2.10799706504014,-7.84727379390072,
26.1668890054773));
#164478=CARTESIAN_POINT('Ctrl Pts',(2.16645156523244,-7.83133743396191,
26.1692612195033));
#164479=CARTESIAN_POINT('Ctrl Pts',(2.2247236023665,-7.81474839361917,26.1716334335292));
#164480=CARTESIAN_POINT('Ctrl Pts',(2.41473385330918,-7.76065576405877,
26.1793686184399));
#164481=CARTESIAN_POINT('Ctrl Pts',(2.60288735546081,-7.69959561931575,
26.1871038033505));
#164482=CARTESIAN_POINT('Ctrl Pts',(2.78863239052449,-7.63172437611695,
26.1948389882612));
#164483=CARTESIAN_POINT('Ctrl Pts',(2.97431998863419,-7.56387412038341,
26.2025717812616));
#164484=CARTESIAN_POINT('Ctrl Pts',(3.15760027133842,-7.48921708154389,
26.210304574262));
#164485=CARTESIAN_POINT('Ctrl Pts',(3.33793763931164,-7.40795922495302,
26.2180373672624));
#164486=CARTESIAN_POINT('Ctrl Pts',(3.51825128324374,-7.32671205813075,
26.2257691429855));
#164487=CARTESIAN_POINT('Ctrl Pts',(3.69562246188648,-7.23886594900611,
26.2335009187087));
#164488=CARTESIAN_POINT('Ctrl Pts',(3.86953636465702,-7.14467465215155,
26.2412326944318));
#164489=CARTESIAN_POINT('Ctrl Pts',(4.04351249857005,-7.05044965107944,
26.2489672367954));
#164490=CARTESIAN_POINT('Ctrl Pts',(4.21402857197604,-6.94987509075678,
26.256701779159));
#164491=CARTESIAN_POINT('Ctrl Pts',(4.38059458351416,-6.84325059145041,
26.2644363215226));
#164492=CARTESIAN_POINT('Ctrl Pts',(4.54718872619452,-6.7366080844549,26.2721721701642));
#164493=CARTESIAN_POINT('Ctrl Pts',(4.70983118419788,-6.62391379951222,
26.2799080188058));
#164494=CARTESIAN_POINT('Ctrl Pts',(4.86806156612962,-6.50551029135084,
26.2876438674473));
#164495=CARTESIAN_POINT('Ctrl Pts',(5.02642141932461,-6.3870099000777,26.2953860459106));
#164496=CARTESIAN_POINT('Ctrl Pts',(5.18036170501404,-6.26279116996034,
26.3031282243738));
#164497=CARTESIAN_POINT('Ctrl Pts',(5.32945499152679,-6.13323707806817,
26.310870402837));
#164498=CARTESIAN_POINT('Ctrl Pts',(5.45418114871876,-6.02485671830715,
26.3173472348298));
#164499=CARTESIAN_POINT('Ctrl Pts',(5.57551571201498,-5.91274323077475,
26.3238240668227));
#164500=CARTESIAN_POINT('Ctrl Pts',(5.69322869546535,-5.7971402073462,26.3303008988156));
#164501=CARTESIAN_POINT('Ctrl Pts',(5.86403287429022,-5.62939762783106,
26.3396989272871));
#164502=CARTESIAN_POINT('Ctrl Pts',(6.02730908883279,-5.45421274325348,
26.3490969557586));
#164503=CARTESIAN_POINT('Ctrl Pts',(6.18250140949143,-5.27222570496906,
26.3584949842301));
#164504=CARTESIAN_POINT('Ctrl Pts',(6.3379145558335,-5.08997971436063,26.3679063853096));
#164505=CARTESIAN_POINT('Ctrl Pts',(6.48522077508968,-4.90091223758863,
26.377317786389));
#164506=CARTESIAN_POINT('Ctrl Pts',(6.62390356071435,-4.7056975233068,26.3867291874685));
#164507=CARTESIAN_POINT('Ctrl Pts',(6.76237753599913,-4.51077673772461,
26.3961264180952));
#164508=CARTESIAN_POINT('Ctrl Pts',(6.89225400991554,-4.30972724525927,
26.4055236487219));
#164509=CARTESIAN_POINT('Ctrl Pts',(7.0130606230254,-4.10325093800885,26.4149208793486));
#164510=CARTESIAN_POINT('Ctrl Pts',(7.1335625167913,-3.89729544102925,26.4242944066541));
#164511=CARTESIAN_POINT('Ctrl Pts',(7.24504020994197,-3.68594049381563,
26.4336679339596));
#164512=CARTESIAN_POINT('Ctrl Pts',(7.34706693404567,-3.4699128273132,26.4430414612652));
#164513=CARTESIAN_POINT('Ctrl Pts',(7.44843110259639,-3.25528803178695,
26.452354117435));
#164514=CARTESIAN_POINT('Ctrl Pts',(7.54046661329701,-3.03605103982633,
26.4616667736048));
#164515=CARTESIAN_POINT('Ctrl Pts',(7.62279701287586,-2.8129438783934,26.4709794297747));
#164516=CARTESIAN_POINT('Ctrl Pts',(7.67580860355992,-2.66928776132039,
26.4769757412171));
#164517=CARTESIAN_POINT('Ctrl Pts',(7.72479737831623,-2.52402769341761,
26.4829720526596));
#164518=CARTESIAN_POINT('Ctrl Pts',(7.76967232571477,-2.37736819056747,
26.4889683641021));
#164519=CARTESIAN_POINT('Ctrl Pts',(7.82403259858036,-2.1997089161741,26.4962321303034));
#164520=CARTESIAN_POINT('Ctrl Pts',(7.87234909752469,-2.02000793831355,
26.5034958965047));
#164521=CARTESIAN_POINT('Ctrl Pts',(7.91445874219333,-1.83875783631765,
26.510759662706));
#164522=CARTESIAN_POINT('Ctrl Pts',(7.9565588222911,-1.65754890254958,26.5180217790523));
#164523=CARTESIAN_POINT('Ctrl Pts',(7.99245475556078,-1.47479192120609,
26.5252838953987));
#164524=CARTESIAN_POINT('Ctrl Pts',(8.02203357363806,-1.2909937668028,26.532546011745));
#164525=CARTESIAN_POINT('Ctrl Pts',(8.05160832091196,-1.10722090773581,
26.539807128638));
#164526=CARTESIAN_POINT('Ctrl Pts',(8.07486762491511,-0.922407545912508,
26.547068245531));
#164527=CARTESIAN_POINT('Ctrl Pts',(8.0917498982538,-0.73706929566335,26.554329362424));
#164528=CARTESIAN_POINT('Ctrl Pts',(8.10863655287446,-0.551682946493031,
26.5615923637197));
#164529=CARTESIAN_POINT('Ctrl Pts',(8.11914284310628,-0.365771825371201,
26.5688553650154));
#164530=CARTESIAN_POINT('Ctrl Pts',(8.12325917997313,-0.179855101351589,
26.576118366311));
#164531=CARTESIAN_POINT('Ctrl Pts',(8.12461543742631,-0.118598952795572,
26.5785113919448));
#164532=CARTESIAN_POINT('Ctrl Pts',(8.12527843401783,-0.0573421962115691,
26.5809044175786));
#164533=CARTESIAN_POINT('Ctrl Pts',(8.12524906564331,0.00389663476247341,
26.5832974432124));
#164534=CARTESIAN_POINT('',(8.12524985409108,-0.00153983533529523,30.5838443095726));
#164535=CARTESIAN_POINT('Ctrl Pts',(8.12524912703364,0.00376644912446197,
26.5863743722194));
#164536=CARTESIAN_POINT('Ctrl Pts',(8.12504495498968,0.444220751611364,
26.6050223615419));
#164537=CARTESIAN_POINT('Ctrl Pts',(8.08902685666685,0.883951628366578,
26.623712746037));
#164538=CARTESIAN_POINT('Ctrl Pts',(8.01504120179438,1.333806306405,26.641849757576));
#164539=CARTESIAN_POINT('Ctrl Pts',(8.01249876033298,1.34899531095105,26.6424608883332));
#164540=CARTESIAN_POINT('Ctrl Pts',(8.00830498727768,1.37361950306895,26.643449516136));
#164541=CARTESIAN_POINT('Ctrl Pts',(8.00668013404125,1.38305912403317,26.6438279961786));
#164542=CARTESIAN_POINT('Ctrl Pts',(8.00380323325127,1.39959755855871,26.6444901860161));
#164543=CARTESIAN_POINT('Ctrl Pts',(8.00255842566831,1.40669761025795,26.6447741721005));
#164544=CARTESIAN_POINT('Ctrl Pts',(8.00003461415254,1.42098098880658,26.6453448665394));
#164545=CARTESIAN_POINT('Ctrl Pts',(7.99875537924197,1.42816426985755,26.6456315656395));
#164546=CARTESIAN_POINT('Ctrl Pts',(7.99627076304714,1.4420080657223,26.6461834889836));
#164547=CARTESIAN_POINT('Ctrl Pts',(7.99506673173401,1.44866881412612,26.6464487666777));
#164548=CARTESIAN_POINT('Ctrl Pts',(7.99220071902629,1.46441130463962,26.6470750862407));
#164549=CARTESIAN_POINT('Ctrl Pts',(7.99053157671914,1.47349174572936,26.6474358372344));
#164550=CARTESIAN_POINT('Ctrl Pts',(7.9855296119797,1.50044490706627,26.6485050664808));
#164551=CARTESIAN_POINT('Ctrl Pts',(7.98215226176878,1.5183093822101,26.6492116902806));
#164552=CARTESIAN_POINT('Ctrl Pts',(7.93918514452742,1.74147743152986,26.658011987617));
#164553=CARTESIAN_POINT('Ctrl Pts',(7.89174631816007,1.94518467158631,26.6657214896003));
#164554=CARTESIAN_POINT('Ctrl Pts',(7.80616977090938,2.25756079995807,26.6772609747527));
#164555=CARTESIAN_POINT('Ctrl Pts',(7.77349293372523,2.36763086703,26.6812736618258));
#164556=CARTESIAN_POINT('Ctrl Pts',(7.72019045351377,2.53415703804759,26.6873037899847));
#164557=CARTESIAN_POINT('Ctrl Pts',(7.70125348714104,2.59113630800775,26.6893597126843));
#164558=CARTESIAN_POINT('Ctrl Pts',(7.65311018921146,2.73080230995007,26.6943901908952));
#164559=CARTESIAN_POINT('Ctrl Pts',(7.62319343136999,2.81323638634756,26.6973515368996));
#164560=CARTESIAN_POINT('Ctrl Pts',(7.54814595963977,3.01003187040682,26.7044297225124));
#164561=CARTESIAN_POINT('Ctrl Pts',(7.5017426782117,3.12388481781467,26.7085318363778));
#164562=CARTESIAN_POINT('Ctrl Pts',(7.35398857354184,3.46410722027513,26.7209008103668));
#164563=CARTESIAN_POINT('Ctrl Pts',(7.24484205175407,3.68692939580951,26.7291556799172));
#164564=CARTESIAN_POINT('Ctrl Pts',(6.94753257749294,4.22952929722464,26.7501718443442));
#164565=CARTESIAN_POINT('Ctrl Pts',(6.74735537569329,4.54205858420145,26.7631315789055));
#164566=CARTESIAN_POINT('Ctrl Pts',(6.43537459756574,4.96276860101953,26.7824965863518));
#164567=CARTESIAN_POINT('Ctrl Pts',(6.34074438564564,5.08311677585026,26.7882757335438));
#164568=CARTESIAN_POINT('Ctrl Pts',(6.22800172430092,5.21844945864787,26.7950763289506));
#164569=CARTESIAN_POINT('Ctrl Pts',(6.21315378715827,5.23611881425771,26.7959703171741));
#164570=CARTESIAN_POINT('Ctrl Pts',(6.19054413108309,5.26279319837987,26.79732923558));
#164571=CARTESIAN_POINT('Ctrl Pts',(6.18283754712518,5.27184490972763,26.7977920096806));
#164572=CARTESIAN_POINT('Ctrl Pts',(6.16893258434562,5.28810445288811,26.7986262500124));
#164573=CARTESIAN_POINT('Ctrl Pts',(6.16274136140793,5.29531838952981,26.7989974350539));
#164574=CARTESIAN_POINT('Ctrl Pts',(6.15033126136748,5.30972724150064,26.7997409435223));
#164575=CARTESIAN_POINT('Ctrl Pts',(6.14411238403888,5.31692213740844,26.8001132667633));
#164576=CARTESIAN_POINT('Ctrl Pts',(6.12672227105973,5.33697028082346,26.8011536942763));
#164577=CARTESIAN_POINT('Ctrl Pts',(6.11552326700168,5.34979931694466,26.8018228950645));
#164578=CARTESIAN_POINT('Ctrl Pts',(6.07030912612532,5.40126694818107,26.8045214427148));
#164579=CARTESIAN_POINT('Ctrl Pts',(6.03596783001374,5.43961669316477,26.806563732999));
#164580=CARTESIAN_POINT('Ctrl Pts',(5.40032426472651,6.13602379163725,26.8442376855673));
#164581=CARTESIAN_POINT('Ctrl Pts',(4.69519226122991,6.69095422004784,26.8848189525063));
#164582=CARTESIAN_POINT('Ctrl Pts',(3.74917403078295,7.21102661120727,26.9328587902915));
#164583=CARTESIAN_POINT('Ctrl Pts',(3.58089608289444,7.29605362875179,26.941155126988));
#164584=CARTESIAN_POINT('Ctrl Pts',(3.27939021903004,7.43545103384776,26.955429180201));
#164585=CARTESIAN_POINT('Ctrl Pts',(3.14738980245291,7.49228090305327,26.9614865221012));
#164586=CARTESIAN_POINT('Ctrl Pts',(2.96970110594588,7.56325544356129,26.9693294310407));
#164587=CARTESIAN_POINT('Ctrl Pts',(2.92530227422235,7.58053852182867,26.9712631953241));
#164588=CARTESIAN_POINT('Ctrl Pts',(2.84986377623592,7.60914287210126,26.9745059910686));
#164589=CARTESIAN_POINT('Ctrl Pts',(2.81890445132915,7.62066640986863,26.9758248792002));
#164590=CARTESIAN_POINT('Ctrl Pts',(2.77666046922116,7.63609761321342,26.9776092625627));
#164591=CARTESIAN_POINT('Ctrl Pts',(2.7654364849857,7.6401695772657,26.9780819040022));
#164592=CARTESIAN_POINT('Ctrl Pts',(2.74762675482655,7.64658640490091,26.9788296120083));
#164593=CARTESIAN_POINT('Ctrl Pts',(2.74104691425429,7.64894752535956,26.9791053662295));
#164594=CARTESIAN_POINT('Ctrl Pts',(2.72735757256258,7.65383989810297,26.9796780716101));
#164595=CARTESIAN_POINT('Ctrl Pts',(2.72024757350879,7.6563697437958,26.9799749640592));
#164596=CARTESIAN_POINT('Ctrl Pts',(2.70395242127774,7.6621422426963,26.9806541369966));
#164597=CARTESIAN_POINT('Ctrl Pts',(2.69476493125208,7.66537829530659,26.9810361475208));
#164598=CARTESIAN_POINT('Ctrl Pts',(2.66644527566709,7.67529594453423,26.982210888139));
#164599=CARTESIAN_POINT('Ctrl Pts',(2.64729383639985,7.68192251958345,26.9830014222104));
#164600=CARTESIAN_POINT('Ctrl Pts',(2.4953607260324,7.73385713237851,26.9892433610403));
#164601=CARTESIAN_POINT('Ctrl Pts',(2.36144647314292,7.77579219058717,26.994566741772));
#164602=CARTESIAN_POINT('Ctrl Pts',(1.82242295399138,7.92937606807615,27.0154901887677));
#164603=CARTESIAN_POINT('Ctrl Pts',(1.40999927824042,8.01299935331532,27.0304116026265));
#164604=CARTESIAN_POINT('Ctrl Pts',(0.660769176253835,8.10525058116122,
27.0575458576452));
#164605=CARTESIAN_POINT('Ctrl Pts',(0.326390255874048,8.12558699641569,
27.0696587962195));
#164606=CARTESIAN_POINT('Ctrl Pts',(-0.177155189189466,8.12507360333953,
27.0883697443591));
#164607=CARTESIAN_POINT('Ctrl Pts',(-0.345976441303749,8.11963689778604,
27.0947187339356));
#164608=CARTESIAN_POINT('Ctrl Pts',(-0.621380310231354,8.10216285005407,
27.1052282514291));
#164609=CARTESIAN_POINT('Ctrl Pts',(-0.728111953039665,8.09326935241919,
27.109338386292));
#164610=CARTESIAN_POINT('Ctrl Pts',(-0.870298382844737,8.07858611981485,
27.1148651873212));
#164611=CARTESIAN_POINT('Ctrl Pts',(-0.905936419142222,8.07466730935062,
27.1162547399789));
#164612=CARTESIAN_POINT('Ctrl Pts',(-0.964819738644798,8.0677976806562,
27.1185577271724));
#164613=CARTESIAN_POINT('Ctrl Pts',(-0.98808034573605,8.06498194477458,
27.119469304014));
#164614=CARTESIAN_POINT('Ctrl Pts',(-1.03308061725437,8.05933698299409,
27.1212363744053));
#164615=CARTESIAN_POINT('Ctrl Pts',(-1.05482167936488,8.05652030276375,
27.1220916838275));
#164616=CARTESIAN_POINT('Ctrl Pts',(-1.10387839432974,8.04996274411877,
27.1240253214184));
#164617=CARTESIAN_POINT('Ctrl Pts',(-1.13118691179693,8.04617075716757,
27.1251043311196));
#164618=CARTESIAN_POINT('Ctrl Pts',(-1.20115898269141,8.03609135975492,
27.1278760987031));
#164619=CARTESIAN_POINT('Ctrl Pts',(-1.24379261550845,8.02960317452887,
27.1295716503858));
#164620=CARTESIAN_POINT('Ctrl Pts',(-1.51488467816214,7.98613625647129,
27.1403989672989));
#164621=CARTESIAN_POINT('Ctrl Pts',(-1.74172001424296,7.93975148413848,
27.149670942605));
#164622=CARTESIAN_POINT('Ctrl Pts',(-2.00682782838697,7.87363179869951,
27.1608092369255));
#164623=CARTESIAN_POINT('Ctrl Pts',(-2.047316191557,7.86320113009674,27.1625186137577));
#164624=CARTESIAN_POINT('Ctrl Pts',(-2.3051200284098,7.7946591879031,27.1734561977457));
#164625=CARTESIAN_POINT('Ctrl Pts',(-2.52001834698053,7.72785824960592,
27.1828200523401));
#164626=CARTESIAN_POINT('Ctrl Pts',(-2.98688157013249,7.56118701341906,
27.2036689058034));
#164627=CARTESIAN_POINT('Ctrl Pts',(-3.2371873230016,7.45745438236957,27.2151868003348));
#164628=CARTESIAN_POINT('Ctrl Pts',(-3.79231845979541,7.19417028891366,
27.2412291812873));
#164629=CARTESIAN_POINT('Ctrl Pts',(-4.09315255536006,7.02736681955361,
27.2557088550449));
#164630=CARTESIAN_POINT('Ctrl Pts',(-4.40889166699642,6.82512578680511,
27.2708038404595));
#164631=CARTESIAN_POINT('Ctrl Pts',(-4.43515729151717,6.80808692409041,
27.2720586049615));
#164632=CARTESIAN_POINT('Ctrl Pts',(-4.47467627013302,6.78212467223915,
27.2739443986552));
#164633=CARTESIAN_POINT('Ctrl Pts',(-4.48800272424986,6.77331339475466,
27.2745799538916));
#164634=CARTESIAN_POINT('Ctrl Pts',(-4.51238662521907,6.75708751945513,
27.2757420712478));
#164635=CARTESIAN_POINT('Ctrl Pts',(-4.52345198869404,6.74968494890674,
27.2762691411422));
#164636=CARTESIAN_POINT('Ctrl Pts',(-4.54131252194983,6.73767285940162,
27.2771193444464));
#164637=CARTESIAN_POINT('Ctrl Pts',(-4.54811896228853,6.73308019318088,
27.2774432204508));
#164638=CARTESIAN_POINT('Ctrl Pts',(-4.5611486217632,6.72425961841571,27.2780629619965));
#164639=CARTESIAN_POINT('Ctrl Pts',(-4.56737295138885,6.72003336963871,
27.2783589020312));
#164640=CARTESIAN_POINT('Ctrl Pts',(-4.58148511281325,6.71042270895644,
27.2790296022601));
#164641=CARTESIAN_POINT('Ctrl Pts',(-4.58936934785459,6.70503301720098,
27.2794041181184));
#164642=CARTESIAN_POINT('Ctrl Pts',(-4.61316302846303,6.68870594140596,
27.280533737152));
#164643=CARTESIAN_POINT('Ctrl Pts',(-4.62904308012671,6.67772569580436,
27.2812868055664));
#164644=CARTESIAN_POINT('Ctrl Pts',(-4.7576487820478,6.58812221079325,27.2873777982892));
#164645=CARTESIAN_POINT('Ctrl Pts',(-4.86839034530911,6.50671594090737,
27.2925608167521));
#164646=CARTESIAN_POINT('Ctrl Pts',(-4.99147147059543,6.41133636953067,
27.2982785279222));
#164647=CARTESIAN_POINT('Ctrl Pts',(-5.0058778935764,6.40009437471773,27.2989472119939));
#164648=CARTESIAN_POINT('Ctrl Pts',(-5.61092787975708,5.92465326648763,
27.3270120174434));
#164649=CARTESIAN_POINT('Ctrl Pts',(-6.13442693929759,5.38080109036826,
27.3507781349952));
#164650=CARTESIAN_POINT('Ctrl Pts',(-6.79573746522483,4.46966211418129,
27.3898300812517));
#164651=CARTESIAN_POINT('Ctrl Pts',(-6.99447624571964,4.15177038423666,
27.4032933162527));
#164652=CARTESIAN_POINT('Ctrl Pts',(-7.19870656872638,3.76853931490387,
27.4198284025264));
#164653=CARTESIAN_POINT('Ctrl Pts',(-7.2262514353202,3.71544813539016,27.4221248696142));
#164654=CARTESIAN_POINT('Ctrl Pts',(-7.26101351622446,3.64659708039299,
27.4251116067529));
#164655=CARTESIAN_POINT('Ctrl Pts',(-7.26877023200484,3.63111096765797,
27.425783942505));
#164656=CARTESIAN_POINT('Ctrl Pts',(-7.28120825261779,3.60607916948017,
27.426871629301));
#164657=CARTESIAN_POINT('Ctrl Pts',(-7.28592045787562,3.59654885620008,
27.4272859571489));
#164658=CARTESIAN_POINT('Ctrl Pts',(-7.29487211906814,3.57835456129404,
27.4280773661577));
#164659=CARTESIAN_POINT('Ctrl Pts',(-7.29911488066169,3.56969222175066,
27.4284543372659));
#164660=CARTESIAN_POINT('Ctrl Pts',(-7.30876951807077,3.5498914135657,27.4293164532751));
#164661=CARTESIAN_POINT('Ctrl Pts',(-7.31417136874242,3.53874809832885,
27.4298019273731));
#164662=CARTESIAN_POINT('Ctrl Pts',(-7.32813960755549,3.50976482143206,
27.4310654187901));
#164663=CARTESIAN_POINT('Ctrl Pts',(-7.3366663075571,3.49190588281732,27.4318447381637));
#164664=CARTESIAN_POINT('Ctrl Pts',(-7.38873996604644,3.38180631413665,
27.4366541301956));
#164665=CARTESIAN_POINT('Ctrl Pts',(-7.43061099778543,3.28878571923863,
27.4407388400703));
#164666=CARTESIAN_POINT('Ctrl Pts',(-7.75767053821409,2.52403855201772,
27.4745072055012));
#164667=CARTESIAN_POINT('Ctrl Pts',(-7.9528870064651,1.81755562707462,27.507247877958));
#164668=CARTESIAN_POINT('Ctrl Pts',(-8.12210712489587,0.572953983549243,
27.5638672130948));
#164669=CARTESIAN_POINT('Ctrl Pts',(-8.14217491902688,0.0454953328315635,
27.5874015854159));
#164670=CARTESIAN_POINT('Ctrl Pts',(-8.10938784797166,-0.508233392943172,
27.6095964057986));
#164671=CARTESIAN_POINT('Ctrl Pts',(-8.10758724064435,-0.536191770245362,
27.6107107550455));
#164672=CARTESIAN_POINT('Ctrl Pts',(-8.10489077804785,-0.574934884158393,
27.6122469003449));
#164673=CARTESIAN_POINT('Ctrl Pts',(-8.1041179426227,-0.585727768445667,
27.6126739656274));
#164674=CARTESIAN_POINT('Ctrl Pts',(-8.10277432282676,-0.603979968090866,
27.6133947691628));
#164675=CARTESIAN_POINT('Ctrl Pts',(-8.10221479345928,-0.611440078558552,
27.613688977288));
#164676=CARTESIAN_POINT('Ctrl Pts',(-8.10108498479843,-0.626229733087682,
27.6142714660751));
#164677=CARTESIAN_POINT('Ctrl Pts',(-8.10051505942049,-0.633559296434201,
27.6145597609602));
#164678=CARTESIAN_POINT('Ctrl Pts',(-8.09923369186252,-0.64975400234305,
27.6151959309906));
#164679=CARTESIAN_POINT('Ctrl Pts',(-8.0985176399946,-0.658618777795756,
27.6155436199414));
#164680=CARTESIAN_POINT('Ctrl Pts',(-8.09594888310631,-0.689782516011133,
27.6167640511219));
#164681=CARTESIAN_POINT('Ctrl Pts',(-8.09401861259611,-0.712075100314758,
27.6176337322592));
#164682=CARTESIAN_POINT('Ctrl Pts',(-8.06056871702522,-1.08066352035856,
27.631961831488));
#164683=CARTESIAN_POINT('Ctrl Pts',(-8.00694071291827,-1.42461627342084,
27.64460283728));
#164684=CARTESIAN_POINT('Ctrl Pts',(-7.80410019677652,-2.33659714835224,
27.6782068451738));
#164685=CARTESIAN_POINT('Ctrl Pts',(-7.61515768913519,-2.89362100891587,
27.6989790456875));
#164686=CARTESIAN_POINT('Ctrl Pts',(-7.19726980372854,-3.79246742956814,
27.7359392296924));
#164687=CARTESIAN_POINT('Ctrl Pts',(-6.99945863165327,-4.14621004875965,
27.7514187267339));
#164688=CARTESIAN_POINT('Ctrl Pts',(-6.72293651233366,-4.56411039903529,
27.7708154654909));
#164689=CARTESIAN_POINT('Ctrl Pts',(-6.66831862798011,-4.64354450432267,
27.7745586408029));
#164690=CARTESIAN_POINT('Ctrl Pts',(-6.58496682574687,-4.7602638243464,
27.7801493908441));
#164691=CARTESIAN_POINT('Ctrl Pts',(-6.55730118086169,-4.79830188425201,
27.7819860466356));
#164692=CARTESIAN_POINT('Ctrl Pts',(-6.50696372714352,-4.86626343498263,
27.7852947973815));
#164693=CARTESIAN_POINT('Ctrl Pts',(-6.48441181170715,-4.89627411490688,
27.7867656005553));
#164694=CARTESIAN_POINT('Ctrl Pts',(-6.43567861521451,-4.9601979584752,
27.7899197615014));
#164695=CARTESIAN_POINT('Ctrl Pts',(-6.40943545064592,-4.99406249561231,
27.7916037449566));
#164696=CARTESIAN_POINT('Ctrl Pts',(-6.3378632442213,-5.08492679980873,
27.7961581829827));
#164697=CARTESIAN_POINT('Ctrl Pts',(-6.29203384723242,-5.14152711074746,
27.799033998337));
#164698=CARTESIAN_POINT('Ctrl Pts',(-5.99821214250416,-5.49459061357686,
27.8172264317339));
#164699=CARTESIAN_POINT('Ctrl Pts',(-5.73009656858327,-5.77365189297787,
27.832768219621));
#164700=CARTESIAN_POINT('Ctrl Pts',(-5.14353717392916,-6.30290102227069,
27.8648101494429));
#164701=CARTESIAN_POINT('Ctrl Pts',(-4.82420207667574,-6.55054297964778,
27.8812774526664));
#164702=CARTESIAN_POINT('Ctrl Pts',(-4.41674766685772,-6.82050516829263,
27.9009137496598));
#164703=CARTESIAN_POINT('Ctrl Pts',(-4.34496580950138,-6.86645636620171,
27.9043242744606));
#164704=CARTESIAN_POINT('Ctrl Pts',(-4.22265342038315,-6.94206858780283,
27.9100486955717));
#164705=CARTESIAN_POINT('Ctrl Pts',(-4.17250108294612,-6.97232765909977,
27.9123718045247));
#164706=CARTESIAN_POINT('Ctrl Pts',(-4.10114935210433,-7.01433164383792,
27.9156414667269));
#164707=CARTESIAN_POINT('Ctrl Pts',(-4.08021813137192,-7.02652790681888,
27.9165963708055));
#164708=CARTESIAN_POINT('Ctrl Pts',(-4.04323572380125,-7.04785594740855,
27.9182759147257));
#164709=CARTESIAN_POINT('Ctrl Pts',(-4.02720739490974,-7.05702693593348,
27.9190013218911));
#164710=CARTESIAN_POINT('Ctrl Pts',(-3.99220086276577,-7.07689865010142,
27.9205803813758));
#164711=CARTESIAN_POINT('Ctrl Pts',(-3.97321058477317,-7.08757785749688,
27.9214336347637));
#164712=CARTESIAN_POINT('Ctrl Pts',(-3.92014615948622,-7.11713841266393,
27.9238089858409));
#164713=CARTESIAN_POINT('Ctrl Pts',(-3.88597875257644,-7.13585133350465,
27.9253282706055));
#164714=CARTESIAN_POINT('Ctrl Pts',(-3.64082767774847,-7.26783358683459,
27.9361628959527));
#164715=CARTESIAN_POINT('Ctrl Pts',(-3.42505979414316,-7.37197390206753,
27.9453547448434));
#164716=CARTESIAN_POINT('Ctrl Pts',(-2.9794540121391,-7.56325254263238,
27.9639950109622));
#164717=CARTESIAN_POINT('Ctrl Pts',(-2.74963268203394,-7.64980090504412,
27.9734350185419));
#164718=CARTESIAN_POINT('Ctrl Pts',(-2.46205071714114,-7.74346451913729,
27.9851771251564));
#164719=CARTESIAN_POINT('Ctrl Pts',(-2.40766934727779,-7.76054539113466,
27.9873942076133));
#164720=CARTESIAN_POINT('Ctrl Pts',(-2.31751997807577,-7.78782200307736,
27.9910654727267));
#164721=CARTESIAN_POINT('Ctrl Pts',(-2.28185359621469,-7.79834691163931,
27.9925169155283));
#164722=CARTESIAN_POINT('Ctrl Pts',(-2.21181835834764,-7.8184922326294,
27.9953653380202));
#164723=CARTESIAN_POINT('Ctrl Pts',(-2.17745586629732,-7.82813178107578,
27.9967621253935));
#164724=CARTESIAN_POINT('Ctrl Pts',(-2.10163323537106,-7.84886407170304,
27.999842802647));
#164725=CARTESIAN_POINT('Ctrl Pts',(-2.06014648992588,-7.85985533543133,
28.0015274908302));
#164726=CARTESIAN_POINT('Ctrl Pts',(-1.91599931605334,-7.89682518466611,
28.0073784373591));
#164727=CARTESIAN_POINT('Ctrl Pts',(-1.81292006381937,-7.92112504377917,
28.0115581179478));
#164728=CARTESIAN_POINT('Ctrl Pts',(-1.53134671696038,-7.98171876310866,
28.0229662656647));
#164729=CARTESIAN_POINT('Ctrl Pts',(-1.35206085761498,-8.01403691720267,
28.0302214412698));
#164730=CARTESIAN_POINT('Ctrl Pts',(-0.972042837407182,-8.06942302788869,
28.0455550208727));
#164731=CARTESIAN_POINT('Ctrl Pts',(-0.771227236737414,-8.0910854753154,
28.0536323662989));
#164732=CARTESIAN_POINT('Ctrl Pts',(-0.50454617565077,-8.10983363424549,
28.0642625999318));
#164733=CARTESIAN_POINT('Ctrl Pts',(-0.439225678494732,-8.11363354456344,
28.0668584888699));
#164734=CARTESIAN_POINT('Ctrl Pts',(-0.327234461611584,-8.11879204678575,
28.0712917005822));
#164735=CARTESIAN_POINT('Ctrl Pts',(-0.280584910102654,-8.12053808789684,
28.0731331638217));
#164736=CARTESIAN_POINT('Ctrl Pts',(-0.211503752198051,-8.12252773170449,
28.0758510581416));
#164737=CARTESIAN_POINT('Ctrl Pts',(-0.189082199637715,-8.12308060513052,
28.0767317654798));
#164738=CARTESIAN_POINT('Ctrl Pts',(-0.146857455740234,-8.1239468669636,
28.0783875900045));
#164739=CARTESIAN_POINT('Ctrl Pts',(-0.127054935295905,-8.12428069776725,
28.079163028899));
#164740=CARTESIAN_POINT('Ctrl Pts',(-0.0815579675385686,-8.12488129916687,
28.0809422912167));
#164741=CARTESIAN_POINT('Ctrl Pts',(-0.0558630553067464,-8.12509859343093,
28.0819454385214));
#164742=CARTESIAN_POINT('Ctrl Pts',(0.0123321803156192,-8.12535179092587,
28.0846038109864));
#164743=CARTESIAN_POINT('Ctrl Pts',(0.0548325785432046,-8.12517613483883,
28.0862564136738));
#164744=CARTESIAN_POINT('Ctrl Pts',(0.466865940851603,-8.12024016437,28.102246367865));
#164745=CARTESIAN_POINT('Ctrl Pts',(0.835673724279217,-8.09060689178403,
28.1163289610305));
#164746=CARTESIAN_POINT('Ctrl Pts',(1.36171559170572,-8.01197630593596,
28.1367427278862));
#164747=CARTESIAN_POINT('Ctrl Pts',(1.52149108235116,-7.98317593955166,
28.1429844969318));
#164748=CARTESIAN_POINT('Ctrl Pts',(1.8294569047133,-7.91808171486078,28.1551434116098));
#164749=CARTESIAN_POINT('Ctrl Pts',(1.97770007846394,-7.88236210945986,
28.1610547662165));
#164750=CARTESIAN_POINT('Ctrl Pts',(2.19036474760366,-7.82474262670952,
28.169637768838));
#164751=CARTESIAN_POINT('Ctrl Pts',(2.25565481629169,-7.80617167365945,
28.1722869295281));
#164752=CARTESIAN_POINT('Ctrl Pts',(2.37253447944986,-7.77133789514597,
28.1770558060398));
#164753=CARTESIAN_POINT('Ctrl Pts',(2.42420899652686,-7.75537383063506,
28.1791735847055));
#164754=CARTESIAN_POINT('Ctrl Pts',(2.53919588065115,-7.71858881878494,
28.1839074247384));
#164755=CARTESIAN_POINT('Ctrl Pts',(2.60241921002566,-7.69750240586071,
28.1865247984051));
#164756=CARTESIAN_POINT('Ctrl Pts',(2.8201751190918,-7.62188639411661,28.1955902793935));
#164757=CARTESIAN_POINT('Ctrl Pts',(2.97331235408543,-7.56346172097323,
28.2020551993836));
#164758=CARTESIAN_POINT('Ctrl Pts',(3.23082771049877,-7.45618455648439,
28.2130687196345));
#164759=CARTESIAN_POINT('Ctrl Pts',(3.33612557796847,-7.40966949471904,
28.2176136158665));
#164760=CARTESIAN_POINT('Ctrl Pts',(3.47248339557143,-7.34593771105184,
28.2235467158364));
#164761=CARTESIAN_POINT('Ctrl Pts',(3.50446870106782,-7.33073263158408,
28.2249418982325));
#164762=CARTESIAN_POINT('Ctrl Pts',(3.5842138529842,-7.2921824249444,28.2284285133474));
#164763=CARTESIAN_POINT('Ctrl Pts',(3.63184600546289,-7.26857675760056,
28.2305184755822));
#164764=CARTESIAN_POINT('Ctrl Pts',(3.71493708460978,-7.22637756351334,
28.2341759286306));
#164765=CARTESIAN_POINT('Ctrl Pts',(3.75049648094866,-7.20798629212294,
28.2357447932639));
#164766=CARTESIAN_POINT('Ctrl Pts',(3.83724572913597,-7.16230394572566,
28.2395821513508));
#164767=CARTESIAN_POINT('Ctrl Pts',(3.88828200788044,-7.1347260391798,28.24184851559));
#164768=CARTESIAN_POINT('Ctrl Pts',(4.10309923676867,-7.01565804426127,
28.2514335021144));
#164769=CARTESIAN_POINT('Ctrl Pts',(4.26398113862629,-6.91905674564863,
28.258726457263));
#164770=CARTESIAN_POINT('Ctrl Pts',(4.4726074431752,-6.78374521170415,28.2684128602265));
#164771=CARTESIAN_POINT('Ctrl Pts',(4.5234634679115,-6.74994034615889,28.2707926744326));
#164772=CARTESIAN_POINT('Ctrl Pts',(4.64547231913918,-6.66684080992021,
28.2765511623152));
#164773=CARTESIAN_POINT('Ctrl Pts',(4.71622778047766,-6.61697626587097,
28.2799317551831));
#164774=CARTESIAN_POINT('Ctrl Pts',(4.83167103075533,-6.53282577637391,
28.2855223450995));
#164775=CARTESIAN_POINT('Ctrl Pts',(4.87682315933426,-6.49918867405571,
28.2877283381414));
#164776=CARTESIAN_POINT('Ctrl Pts',(4.96265729005221,-6.43384643404949,
28.2919610396371));
#164777=CARTESIAN_POINT('Ctrl Pts',(5.00339420700395,-6.40221787375495,
28.2939871429361));
#164778=CARTESIAN_POINT('Ctrl Pts',(5.11385160527922,-6.31475944197586,
28.2995299029359));
#164779=CARTESIAN_POINT('Ctrl Pts',(5.1829568059752,-6.25816456147672,28.3030518812139));
#164780=CARTESIAN_POINT('Ctrl Pts',(5.60382535447295,-5.9017336896606,28.3248545362757));
#164781=CARTESIAN_POINT('Ctrl Pts',(5.93040213901739,-5.57347630803897,
28.3433769084533));
#164782=CARTESIAN_POINT('Ctrl Pts',(6.30944676719428,-5.12122325539886,
28.3669641391104));
#164783=CARTESIAN_POINT('Ctrl Pts',(6.3892781368325,-5.02127188926251,28.3720659022832));
#164784=CARTESIAN_POINT('Ctrl Pts',(6.49914872931917,-4.87684556159425,
28.3792682256689));
#164785=CARTESIAN_POINT('Ctrl Pts',(6.5311580874893,-4.83389397054078,28.3813895356861));
#164786=CARTESIAN_POINT('Ctrl Pts',(6.58728506909712,-4.75700493840835,
28.3851489230498));
#164787=CARTESIAN_POINT('Ctrl Pts',(6.61157096589775,-4.72319277124167,
28.3867892883353));
#164788=CARTESIAN_POINT('Ctrl Pts',(6.6488853105583,-4.67038991291695,28.3893304012743));
#164789=CARTESIAN_POINT('Ctrl Pts',(6.66209462314542,-4.65152803375784,
28.3902340900905));
#164790=CARTESIAN_POINT('Ctrl Pts',(6.68642112081441,-4.61647548153039,
28.3919058846795));
#164791=CARTESIAN_POINT('Ctrl Pts',(6.69756012531071,-4.60030016929301,
28.3926743730259));
#164792=CARTESIAN_POINT('Ctrl Pts',(6.722772751041,-4.56340241229061,28.3944205045569));
#164793=CARTESIAN_POINT('Ctrl Pts',(6.73680939544143,-4.54265497380317,
28.3953974031079));
#164794=CARTESIAN_POINT('Ctrl Pts',(6.78317025027726,-4.473441924763,28.39864063697));
#164795=CARTESIAN_POINT('Ctrl Pts',(6.81506931242188,-4.42469339469146,
28.4008995542559));
#164796=CARTESIAN_POINT('Ctrl Pts',(6.98445764197613,-4.15965414156242,
28.4130601179966));
#164797=CARTESIAN_POINT('Ctrl Pts',(7.11218039061369,-3.93729142326717,
28.4228380667149));
#164798=CARTESIAN_POINT('Ctrl Pts',(7.30652765221472,-3.55851765458915,
28.4391348646639));
#164799=CARTESIAN_POINT('Ctrl Pts',(7.37913997443588,-3.405390860543,28.4456296473036));
#164800=CARTESIAN_POINT('Ctrl Pts',(7.49144533363264,-3.14806760404676,
28.4564546324736));
#164801=CARTESIAN_POINT('Ctrl Pts',(7.53387679643335,-3.04512445606553,
28.4607619721768));
#164802=CARTESIAN_POINT('Ctrl Pts',(7.59125404797554,-2.89737369857054,
28.4669215266301));
#164803=CARTESIAN_POINT('Ctrl Pts',(7.6079455888539,-2.85325713217651,28.4687578283302));
#164804=CARTESIAN_POINT('Ctrl Pts',(7.63650475067113,-2.77574114322045,
28.4719800059662));
#164805=CARTESIAN_POINT('Ctrl Pts',(7.64853974281833,-2.74240469168815,
28.4733643369791));
#164806=CARTESIAN_POINT('Ctrl Pts',(7.67162880007682,-2.67711454237781,
28.4760731019836));
#164807=CARTESIAN_POINT('Ctrl Pts',(7.68270229199834,-2.64516846389922,
28.4773973333898));
#164808=CARTESIAN_POINT('Ctrl Pts',(7.71249874957965,-2.55744256295543,
28.481030830821));
#164809=CARTESIAN_POINT('Ctrl Pts',(7.73081568842897,-2.50152716734897,
28.4833435660064));
#164810=CARTESIAN_POINT('Ctrl Pts',(7.84458081642091,-2.14105227149758,
28.4982342846135));
#164811=CARTESIAN_POINT('Ctrl Pts',(7.92262000226991,-1.83129465904164,
28.5109599042098));
#164812=CARTESIAN_POINT('Ctrl Pts',(8.00407540433138,-1.4029016608351,28.5283499277034));
#164813=CARTESIAN_POINT('Ctrl Pts',(8.02343271857365,-1.28758834492242,
28.5330085806917));
#164814=CARTESIAN_POINT('Ctrl Pts',(8.05037215295286,-1.10275899651597,
28.5404225416406));
#164815=CARTESIAN_POINT('Ctrl Pts',(8.05955711371782,-1.0334933140502,28.5431890497934));
#164816=CARTESIAN_POINT('Ctrl Pts',(8.07103589264158,-0.937437553376661,
28.5470050190817));
#164817=CARTESIAN_POINT('Ctrl Pts',(8.07409182211956,-0.910741896416319,
28.5480633507946));
#164818=CARTESIAN_POINT('Ctrl Pts',(8.07908818026832,-0.865092323177715,
28.5498690303063));
#164819=CARTESIAN_POINT('Ctrl Pts',(8.08109446338499,-0.846145867366758,
28.5506172656255));
#164820=CARTESIAN_POINT('Ctrl Pts',(8.0848174206114,-0.809766438884356,
28.5520515383226));
#164821=CARTESIAN_POINT('Ctrl Pts',(8.08654438942083,-0.792334683167217,
28.5527377083982));
#164822=CARTESIAN_POINT('Ctrl Pts',(8.09129691783765,-0.742728797868847,
28.5546872951811));
#164823=CARTESIAN_POINT('Ctrl Pts',(8.09418692505041,-0.710541987581968,
28.555948666698));
#164824=CARTESIAN_POINT('Ctrl Pts',(8.106246228188,-0.566597980644516,28.5615750224486));
#164825=CARTESIAN_POINT('Ctrl Pts',(8.11329358806528,-0.4546743959761,28.5659103248057));
#164826=CARTESIAN_POINT('Ctrl Pts',(8.12284980933912,-0.228262882292652,
28.5746280449117));
#164827=CARTESIAN_POINT('Ctrl Pts',(8.12525961307267,-0.113795904479086,
28.5790085855748));
#164828=CARTESIAN_POINT('Ctrl Pts',(8.12521102066998,0.463152093692499,
28.601021137259));
#164829=CARTESIAN_POINT('Ctrl Pts',(8.08568865389865,0.924772151804552,
28.6184464143668));
#164830=CARTESIAN_POINT('Ctrl Pts',(8.00536840890349,1.39063642197348,28.6365482129313));
#164831=CARTESIAN_POINT('Ctrl Pts',(8.00360443074266,1.40075306046991,28.6369415453282));
#164832=CARTESIAN_POINT('Ctrl Pts',(7.96184204248208,1.63761119612558,28.6461561966252));
#164833=CARTESIAN_POINT('Ctrl Pts',(7.91224357422852,1.86255160589202,28.6550310951516));
#164834=CARTESIAN_POINT('Ctrl Pts',(7.83600451298075,2.14969542757179,28.6665813468389));
#164835=CARTESIAN_POINT('Ctrl Pts',(7.81805157199845,2.21409726869623,28.6691863202413));
#164836=CARTESIAN_POINT('Ctrl Pts',(7.78776634404721,2.31777407639103,28.6734044642257));
#164837=CARTESIAN_POINT('Ctrl Pts',(7.77592678247158,2.35718984349811,28.6750138895457));
#164838=CARTESIAN_POINT('Ctrl Pts',(7.7526120905646,2.43272052754385,28.6781093266258));
#164839=CARTESIAN_POINT('Ctrl Pts',(7.74118276003807,2.46884848805137,28.6795949694409));
#164840=CARTESIAN_POINT('Ctrl Pts',(7.71405078779952,2.55257119964036,28.6830496825253));
#164841=CARTESIAN_POINT('Ctrl Pts',(7.69815968689519,2.60010320902206,28.6850200116938));
#164842=CARTESIAN_POINT('Ctrl Pts',(7.64463098638386,2.75541980784102,28.6914882772974));
#164843=CARTESIAN_POINT('Ctrl Pts',(7.60516155718549,2.86255806637339,28.6959978278142));
#164844=CARTESIAN_POINT('Ctrl Pts',(7.33791660138649,3.54339675670948,28.7249662376889));
#164845=CARTESIAN_POINT('Ctrl Pts',(7.04766185027582,4.0903663112696,28.7496957152889));
#164846=CARTESIAN_POINT('Ctrl Pts',(6.45944286310693,4.94705511114485,28.7931144107963));
#164847=CARTESIAN_POINT('Ctrl Pts',(6.19385696125358,5.275782263275,28.8111156805866));
#164848=CARTESIAN_POINT('Ctrl Pts',(5.71598457986253,5.78118122759725,28.8403510712852));
#164849=CARTESIAN_POINT('Ctrl Pts',(5.51809146173939,5.97036135413446,28.8517051509626));
#164850=CARTESIAN_POINT('Ctrl Pts',(5.29418462694404,6.16374820111944,28.8634750693944));
#164851=CARTESIAN_POINT('Ctrl Pts',(5.277283863633,6.17822448485748,28.8643571240423));
#164852=CARTESIAN_POINT('Ctrl Pts',(5.25356075648793,6.19837605194243,28.8655861292096));
#164853=CARTESIAN_POINT('Ctrl Pts',(5.24678834445119,6.20410979695755,28.8659359505329));
#164854=CARTESIAN_POINT('Ctrl Pts',(5.23439196275649,6.21457016310033,28.8665743666754));
#164855=CARTESIAN_POINT('Ctrl Pts',(5.22877095432844,6.21930026928137,28.8668631364096));
#164856=CARTESIAN_POINT('Ctrl Pts',(5.21740837017732,6.22883564699329,28.8674454176526));
#164857=CARTESIAN_POINT('Ctrl Pts',(5.21166655141813,6.23364061971493,28.8677389138479));
#164858=CARTESIAN_POINT('Ctrl Pts',(5.19758784069716,6.24538917260404,28.8684567120695));
#164859=CARTESIAN_POINT('Ctrl Pts',(5.18924365225288,6.25232401576301,28.8688805594446));
#164860=CARTESIAN_POINT('Ctrl Pts',(5.15915754422196,6.27722682018807,28.8704030486156));
#164861=CARTESIAN_POINT('Ctrl Pts',(5.13733582630375,6.29509839107362,28.8714965461627));
#164862=CARTESIAN_POINT('Ctrl Pts',(5.01894054955742,6.39103622174745,28.877369303994));
#164863=CARTESIAN_POINT('Ctrl Pts',(4.92068219428892,6.46699271945491,28.8820202432015));
#164864=CARTESIAN_POINT('Ctrl Pts',(4.71942037264646,6.61533029714115,28.8911644107891));
#164865=CARTESIAN_POINT('Ctrl Pts',(4.61639694108509,6.68763071607416,28.8956554097436));
#164866=CARTESIAN_POINT('Ctrl Pts',(4.26847342695982,6.91992602048347,28.9103214262475));
#164867=CARTESIAN_POINT('Ctrl Pts',(4.0166133158609,7.06909255233249,28.9201411925925));
#164868=CARTESIAN_POINT('Ctrl Pts',(3.51428889040444,7.33106731651561,28.9390562081445));
#164869=CARTESIAN_POINT('Ctrl Pts',(3.26507238246662,7.44540630423332,28.9481470197449));
#164870=CARTESIAN_POINT('Ctrl Pts',(2.52446722262292,7.74084220411182,28.9751721474256));
#164871=CARTESIAN_POINT('Ctrl Pts',(2.02083344357673,7.88731448636748,28.9936397925508));
#164872=CARTESIAN_POINT('Ctrl Pts',(1.47462488986316,7.99038362122887,29.0150067851694));
#164873=CARTESIAN_POINT('Ctrl Pts',(1.44257465548439,7.99623206981226,29.0162649372631));
#164874=CARTESIAN_POINT('Ctrl Pts',(1.39801453120897,8.00408666961414,29.0180204303382));
#164875=CARTESIAN_POINT('Ctrl Pts',(1.3855336388237,8.00625658957524,29.0185128085441));
#164876=CARTESIAN_POINT('Ctrl Pts',(1.36403799224707,8.00994203975643,29.019362005657));
#164877=CARTESIAN_POINT('Ctrl Pts',(1.35502564545496,8.01147156420298,29.019718400564));
#164878=CARTESIAN_POINT('Ctrl Pts',(1.33642812901512,8.0145955503846,29.0204545843139));
#164879=CARTESIAN_POINT('Ctrl Pts',(1.32684264353852,8.01618803289866,29.0208344323483));
#164880=CARTESIAN_POINT('Ctrl Pts',(1.30453879500382,8.01985237670853,29.0217192265081));
#164881=CARTESIAN_POINT('Ctrl Pts',(1.29181833020364,8.02191118199211,29.0222245658597));
#164882=CARTESIAN_POINT('Ctrl Pts',(1.25132490918671,8.02836622222461,29.0238355295637));
#164883=CARTESIAN_POINT('Ctrl Pts',(1.22353414386686,8.03264852996908,29.0249445838759));
#164884=CARTESIAN_POINT('Ctrl Pts',(0.685409459483516,8.11271130881777,
29.0464872510533));
#164885=CARTESIAN_POINT('Ctrl Pts',(0.16909180260856,8.13985034632006,29.0684338652075));
#164886=CARTESIAN_POINT('Ctrl Pts',(-1.12268337179519,8.08475129161273,
29.1256504133413));
#164887=CARTESIAN_POINT('Ctrl Pts',(-1.89037985788163,7.94041817319647,
29.1618853402616));
#164888=CARTESIAN_POINT('Ctrl Pts',(-2.66449371428447,7.67605521460815,
29.1949045500488));
#164889=CARTESIAN_POINT('Ctrl Pts',(-2.70298428075024,7.66258614799331,
29.1965367723628));
#164890=CARTESIAN_POINT('Ctrl Pts',(-2.75397260883419,7.64431171487656,
29.1986880105995));
#164891=CARTESIAN_POINT('Ctrl Pts',(-2.76656178358605,7.63976456606172,
29.1992182662749));
#164892=CARTESIAN_POINT('Ctrl Pts',(-2.78613575088601,7.6326398165577,29.2000414050681));
#164893=CARTESIAN_POINT('Ctrl Pts',(-2.79312829941951,7.63008370171299,
29.2003351989473));
#164894=CARTESIAN_POINT('Ctrl Pts',(-2.80715708602389,7.62493363208737,
29.2009241124625));
#164895=CARTESIAN_POINT('Ctrl Pts',(-2.81419326540717,7.62233954011127,
29.201219225934));
#164896=CARTESIAN_POINT('Ctrl Pts',(-2.82994463512915,7.61650755678943,
29.2018793149002));
#164897=CARTESIAN_POINT('Ctrl Pts',(-2.83865788809669,7.61326443753016,
29.2022440749804));
#164898=CARTESIAN_POINT('Ctrl Pts',(-2.86429221991598,7.60367307708203,
29.2033161105881));
#164899=CARTESIAN_POINT('Ctrl Pts',(-2.88119776670928,7.59728330520904,
29.2040217108194));
#164900=CARTESIAN_POINT('Ctrl Pts',(-3.01217327747922,7.54727857530014,
29.2094783821334));
#164901=CARTESIAN_POINT('Ctrl Pts',(-3.12527129844734,7.50115208856428,
29.2141317423543));
#164902=CARTESIAN_POINT('Ctrl Pts',(-3.53580528194383,7.32282017330772,
29.2309299066784));
#164903=CARTESIAN_POINT('Ctrl Pts',(-3.82627153629619,7.17532405638642,
29.2426446485696));
#164904=CARTESIAN_POINT('Ctrl Pts',(-4.31543381568048,6.8887596004457,29.2630060607293));
#164905=CARTESIAN_POINT('Ctrl Pts',(-4.51820929001019,6.75749670778909,
29.2716508204654));
#164906=CARTESIAN_POINT('Ctrl Pts',(-5.08240585990947,6.35551184511476,
29.296756307632));
#164907=CARTESIAN_POINT('Ctrl Pts',(-5.42749549566616,6.0634678165698,29.3134814424705));
#164908=CARTESIAN_POINT('Ctrl Pts',(-5.7848942471704,5.70592928095342,29.332935832273));
#164909=CARTESIAN_POINT('Ctrl Pts',(-5.82286047651229,5.66717974098427,
29.335031290318));
#164910=CARTESIAN_POINT('Ctrl Pts',(-5.87963071255195,5.60806546012648,
29.3382086166792));
#164911=CARTESIAN_POINT('Ctrl Pts',(-5.89872337734747,5.58797978077181,
29.3392848790092));
#164912=CARTESIAN_POINT('Ctrl Pts',(-5.9327476148363,5.55181724244866,29.3412166510521));
#164913=CARTESIAN_POINT('Ctrl Pts',(-5.94771756131865,5.53577679831917,
29.3420714440379));
#164914=CARTESIAN_POINT('Ctrl Pts',(-5.97849766343348,5.50252663583306,
29.3438390733126));
#164915=CARTESIAN_POINT('Ctrl Pts',(-5.99429893409404,5.4853089223439,29.3447520714455));
#164916=CARTESIAN_POINT('Ctrl Pts',(-6.03396036557016,5.44171616360803,
29.3470580380991));
#164917=CARTESIAN_POINT('Ctrl Pts',(-6.05772198679256,5.41525223891945,
29.3484527918219));
#164918=CARTESIAN_POINT('Ctrl Pts',(-6.15203517129034,5.3088156730309,29.354043148718));
#164919=CARTESIAN_POINT('Ctrl Pts',(-6.22118216425379,5.22761442220968,
29.3582651676087));
#164920=CARTESIAN_POINT('Ctrl Pts',(-6.80567378490065,4.51320361615728,
29.3950979085542));
#164921=CARTESIAN_POINT('Ctrl Pts',(-7.22443059655724,3.80703759476793,
29.4301046632004));
#164922=CARTESIAN_POINT('Ctrl Pts',(-7.62326116974548,2.82243334289596,
29.4747026127156));
#164923=CARTESIAN_POINT('Ctrl Pts',(-7.70524212450984,2.59026915961201,
29.4848865695197));
#164924=CARTESIAN_POINT('Ctrl Pts',(-7.78318193915348,2.3328712572935,29.4956110856699));
#164925=CARTESIAN_POINT('Ctrl Pts',(-7.78970998080644,2.31097984159077,
29.4965187558656));
#164926=CARTESIAN_POINT('Ctrl Pts',(-7.79874055977998,2.28022325313414,
29.4977875307137));
#164927=CARTESIAN_POINT('Ctrl Pts',(-7.80132044440041,2.27138101768604,
29.4981515434644));
#164928=CARTESIAN_POINT('Ctrl Pts',(-7.80601993237078,2.25517164417241,
29.4988174510952));
#164929=CARTESIAN_POINT('Ctrl Pts',(-7.80814415421196,2.24780586278804,
29.4991195235741));
#164930=CARTESIAN_POINT('Ctrl Pts',(-7.81242352858224,2.23288778356903,
29.4997302396844));
#164931=CARTESIAN_POINT('Ctrl Pts',(-7.81457816211327,2.22533534387853,
29.5000388627305));
#164932=CARTESIAN_POINT('Ctrl Pts',(-7.81984873202484,2.2067588470496,29.500796582186));
#164933=CARTESIAN_POINT('Ctrl Pts',(-7.82295231613081,2.19573128183345,
29.501245184032));
#164934=CARTESIAN_POINT('Ctrl Pts',(-7.8341537878458,2.15560531637361,29.5028730542717));
#164935=CARTESIAN_POINT('Ctrl Pts',(-7.84211279282706,2.12646815838037,
29.5040466078946));
#164936=CARTESIAN_POINT('Ctrl Pts',(-7.8858527837557,1.96275429835592,29.5105904225291));
#164937=CARTESIAN_POINT('Ctrl Pts',(-7.91833107552188,1.82732355530139,
29.51580195099));
#164938=CARTESIAN_POINT('Ctrl Pts',(-7.96649898867044,1.60096170895218,
29.5242446944981));
#164939=CARTESIAN_POINT('Ctrl Pts',(-7.98414908105906,1.51047960836138,
29.5275507328029));
#164940=CARTESIAN_POINT('Ctrl Pts',(-8.08425921209319,0.946347628245944,
29.5478272988772));
#164941=CARTESIAN_POINT('Ctrl Pts',(-8.12608706747604,0.46644102575913,
29.5636522508804));
#164942=CARTESIAN_POINT('Ctrl Pts',(-8.1242080640507,-0.596718045028775,
29.5996011020268));
#164943=CARTESIAN_POINT('Ctrl Pts',(-8.06057789846687,-1.17721256102332,
29.6199016716797));
#164944=CARTESIAN_POINT('Ctrl Pts',(-7.92771808430967,-1.78108723528828,
29.643640451902));
#164945=CARTESIAN_POINT('Ctrl Pts',(-7.91974216599924,-1.8162240359905,
29.6450307567085));
#164946=CARTESIAN_POINT('Ctrl Pts',(-7.90852037216439,-1.86418022113962,
29.6469409461985));
#164947=CARTESIAN_POINT('Ctrl Pts',(-7.90547646707857,-1.87704666972729,
29.6474546893532));
#164948=CARTESIAN_POINT('Ctrl Pts',(-7.90024023726166,-1.89894130233668,
29.6483310565548));
#164949=CARTESIAN_POINT('Ctrl Pts',(-7.89806380357127,-1.90797327816207,
29.6486931961492));
#164950=CARTESIAN_POINT('Ctrl Pts',(-7.89382236300144,-1.92544320276013,
29.6493948640573));
#164951=CARTESIAN_POINT('Ctrl Pts',(-7.89175930487326,-1.93388161454557,
29.6497343325644));
#164952=CARTESIAN_POINT('Ctrl Pts',(-7.88682861868789,-1.95391004238932,
29.6505413555836));
#164953=CARTESIAN_POINT('Ctrl Pts',(-7.88394897285358,-1.96549706341457,
29.6510092764643));
#164954=CARTESIAN_POINT('Ctrl Pts',(-7.87536771534645,-1.99970374506789,
29.6523937249784));
#164955=CARTESIAN_POINT('Ctrl Pts',(-7.86959424304695,-2.02230515966519,
29.6533124476196));
#164956=CARTESIAN_POINT('Ctrl Pts',(-7.82346080321223,-2.19971429328974,
29.6605554698521));
#164957=CARTESIAN_POINT('Ctrl Pts',(-7.77863555744,-2.35331833991026,29.6670165185949));
#164958=CARTESIAN_POINT('Ctrl Pts',(-7.6699044722138,-2.68874755660881,
29.6815573981063));
#164959=CARTESIAN_POINT('Ctrl Pts',(-7.6040063183904,-2.86982230903358,
29.6896942914052));
#164960=CARTESIAN_POINT('Ctrl Pts',(-7.29689184978755,-3.62862131807226,
29.724967207713));
#164961=CARTESIAN_POINT('Ctrl Pts',(-6.99578470658754,-4.17976217141215,
29.7537197560156));
#164962=CARTESIAN_POINT('Ctrl Pts',(-6.41412666281492,-5.00243139653624,
29.798598682341));
#164963=CARTESIAN_POINT('Ctrl Pts',(-6.17207808033691,-5.29819710814815,
29.8151578857698));
#164964=CARTESIAN_POINT('Ctrl Pts',(-5.89360885157717,-5.59335667277126,
29.8313613095273));
#164965=CARTESIAN_POINT('Ctrl Pts',(-5.87705296038322,-5.61074974338915,
29.8323153297048));
#164966=CARTESIAN_POINT('Ctrl Pts',(-5.85390392428884,-5.63485447075486,
29.8336367782613));
#164967=CARTESIAN_POINT('Ctrl Pts',(-5.84737596831092,-5.64162834185619,
29.8340080509093));
#164968=CARTESIAN_POINT('Ctrl Pts',(-5.83609920906597,-5.6532893096456,
29.8346470782887));
#164969=CARTESIAN_POINT('Ctrl Pts',(-5.83135600410458,-5.65818178838506,
29.8349151568689));
#164970=CARTESIAN_POINT('Ctrl Pts',(-5.82154113256962,-5.66828009421042,
29.8354684317371));
#164971=CARTESIAN_POINT('Ctrl Pts',(-5.81646862395893,-5.67348509573713,
29.8357535793346));
#164972=CARTESIAN_POINT('Ctrl Pts',(-5.80462609726033,-5.68560437186763,
29.8364174667649));
#164973=CARTESIAN_POINT('Ctrl Pts',(-5.79785068874845,-5.69251338113643,
29.8367959023975));
#164974=CARTESIAN_POINT('Ctrl Pts',(-5.77643563556829,-5.71427281139948,
29.837987705191));
#164975=CARTESIAN_POINT('Ctrl Pts',(-5.76175108914249,-5.72907905441195,
29.8387985913185));
#164976=CARTESIAN_POINT('Ctrl Pts',(-5.62588767952376,-5.86501770531323,
29.8462445242745));
#164977=CARTESIAN_POINT('Ctrl Pts',(-5.50095792987442,-5.98234995085719,
29.8526800935489));
#164978=CARTESIAN_POINT('Ctrl Pts',(-5.22708443820016,-6.22372874318939,
29.8661508812412));
#164979=CARTESIAN_POINT('Ctrl Pts',(-5.07722417345722,-6.34657457128917,
29.8731510625904));
#164980=CARTESIAN_POINT('Ctrl Pts',(-4.68360836149387,-6.64636278576619,
29.8909279154655));
#164981=CARTESIAN_POINT('Ctrl Pts',(-4.43415021129654,-6.81532375125243,
29.9016428294598));
#164982=CARTESIAN_POINT('Ctrl Pts',(-3.88156966596984,-7.14638533138326,
29.9249268245644));
#164983=CARTESIAN_POINT('Ctrl Pts',(-3.57638540903953,-7.30389360585907,
29.9375295617889));
#164984=CARTESIAN_POINT('Ctrl Pts',(-2.96121525483293,-7.57356376023444,
29.9628036825153));
#164985=CARTESIAN_POINT('Ctrl Pts',(-2.65254288386724,-7.68711057698692,
29.9754032641058));
#164986=CARTESIAN_POINT('Ctrl Pts',(-2.24388601139363,-7.80988417039206,
29.9919170204162));
#164987=CARTESIAN_POINT('Ctrl Pts',(-2.1494116744319,-7.83641145136924,
29.9957267675228));
#164988=CARTESIAN_POINT('Ctrl Pts',(-2.00866857717258,-7.87319377382159,
30.0013968059592));
#164989=CARTESIAN_POINT('Ctrl Pts',(-1.96275286158611,-7.88476574365364,
30.0032457109251));
#164990=CARTESIAN_POINT('Ctrl Pts',(-1.88023255502938,-7.90479755192614,
30.0065677436987));
#164991=CARTESIAN_POINT('Ctrl Pts',(-1.84366542265012,-7.91340613101175,
30.0080395364648));
#164992=CARTESIAN_POINT('Ctrl Pts',(-1.77285824905165,-7.92955801918312,
30.0108892392314));
#164993=CARTESIAN_POINT('Ctrl Pts',(-1.73862647281402,-7.93713391144263,
30.0122668310761));
#164994=CARTESIAN_POINT('Ctrl Pts',(-1.65580289318513,-7.95490221873269,
30.0155999909796));
#164995=CARTESIAN_POINT('Ctrl Pts',(-1.60716469468192,-7.96487125722936,
30.0175574637148));
#164996=CARTESIAN_POINT('Ctrl Pts',(-1.40798594837367,-8.00379682326964,
30.0255751825452));
#164997=CARTESIAN_POINT('Ctrl Pts',(-1.25673306531207,-8.02893574162506,
30.0316679447973));
#164998=CARTESIAN_POINT('Ctrl Pts',(-0.862835566601014,-8.08299958215693,
30.0475622327331));
#164999=CARTESIAN_POINT('Ctrl Pts',(-0.619437856786041,-8.10528601980463,
30.0574120715731));
#165000=CARTESIAN_POINT('Ctrl Pts',(-0.146004772702246,-8.12718335888819,
30.0766207129285));
#165001=CARTESIAN_POINT('Ctrl Pts',(0.0837464571762289,-8.12806328904075,
30.0859645841273));
#165002=CARTESIAN_POINT('Ctrl Pts',(0.507325104650065,-8.11172236668132,
30.1031780208249));
#165003=CARTESIAN_POINT('Ctrl Pts',(0.701096048755897,-8.09727633919893,
30.1110467758922));
#165004=CARTESIAN_POINT('Ctrl Pts',(1.01819889995054,-8.06216669375217,
30.1238639838073));
#165005=CARTESIAN_POINT('Ctrl Pts',(1.14190232473057,-8.0455777037495,30.1288487005528));
#165006=CARTESIAN_POINT('Ctrl Pts',(1.29804400351407,-8.0209648104311,30.135108095079));
#165007=CARTESIAN_POINT('Ctrl Pts',(1.33088020515995,-8.01558186421176,
30.1364225950309));
#165008=CARTESIAN_POINT('Ctrl Pts',(1.38110367565676,-8.00703144069184,
30.138430009667));
#165009=CARTESIAN_POINT('Ctrl Pts',(1.39851509495466,-8.00400870737513,
30.1391253485611));
#165010=CARTESIAN_POINT('Ctrl Pts',(1.43239125474688,-7.99801367653606,
30.1404770928145));
#165011=CARTESIAN_POINT('Ctrl Pts',(1.4488568926458,-7.99504729088915,30.1411336091373));
#165012=CARTESIAN_POINT('Ctrl Pts',(1.46536600291902,-7.99202039805092,
30.1417914243835));
#165013=CARTESIAN_POINT('Ctrl Pts',(1.46541872333055,-7.99201073139202,
30.141793525055));
#165014=CARTESIAN_POINT('Ctrl Pts',(1.46552404096696,-7.9919914195842,30.1417977214806));
#165015=CARTESIAN_POINT('Ctrl Pts',(1.46557663824738,-7.9919817744276,30.141799817237));
#165016=CARTESIAN_POINT('Ctrl Pts',(1.46568171045387,-7.99196250547932,
30.1418040038657));
#165017=CARTESIAN_POINT('Ctrl Pts',(1.46573418568748,-7.99195288163371,
30.1418060947503));
#165018=CARTESIAN_POINT('Ctrl Pts',(1.46583901572518,-7.9919336549618,30.1418102717121));
#165019=CARTESIAN_POINT('Ctrl Pts',(1.46589137041116,-7.99192405215961,
30.1418123577847));
#165020=CARTESIAN_POINT('Ctrl Pts',(1.46599596040802,-7.99190486738848,
30.1418165251646));
#165021=CARTESIAN_POINT('Ctrl Pts',(1.46604819577357,-7.99189528541193,
30.1418186064742));
#165022=CARTESIAN_POINT('Ctrl Pts',(1.46615254837484,-7.99187614207087,
30.1418227643776));
#165023=CARTESIAN_POINT('Ctrl Pts',(1.46620466565408,-7.99186658070077,
30.1418248409734));
#165024=CARTESIAN_POINT('Ctrl Pts',(1.4663087836147,-7.99184747829871,30.1418289895103));
#165025=CARTESIAN_POINT('Ctrl Pts',(1.46636078419824,-7.99183793728705,
30.1418310614477));
#165026=CARTESIAN_POINT('Ctrl Pts',(1.4664646697254,-7.99181887543317,30.1418352007062));
#165027=CARTESIAN_POINT('Ctrl Pts',(1.46651655480009,-7.99180935456921,
30.1418372680326));
#165028=CARTESIAN_POINT('Ctrl Pts',(1.46662021037785,-7.99179033282166,
30.1418413981118));
#165029=CARTESIAN_POINT('Ctrl Pts',(1.46667198103232,-7.99178083191257,
30.1418434608707));
#165030=CARTESIAN_POINT('Ctrl Pts',(1.4667754097956,-7.99176184970982,30.1418475818955));
#165031=CARTESIAN_POINT('Ctrl Pts',(1.46682706760386,-7.99175236847358,
30.1418496401496));
#165032=CARTESIAN_POINT('Ctrl Pts',(1.4669302710439,-7.99173342555553,30.1418537521797));
#165033=CARTESIAN_POINT('Ctrl Pts',(1.46698181693616,-7.99172396382815,
30.1418558059661));
#165034=CARTESIAN_POINT('Ctrl Pts',(1.46708479830107,-7.99170505961204,
30.1418599091309));
#165035=CARTESIAN_POINT('Ctrl Pts',(1.46713623370998,-7.9916956171372,30.1418619585068));
#165036=CARTESIAN_POINT('Ctrl Pts',(1.46723899465904,-7.99167675133167,
30.1418660528727));
#165037=CARTESIAN_POINT('Ctrl Pts',(1.46729032046092,-7.99166732795509,
30.141868097873));
#165038=CARTESIAN_POINT('Ctrl Pts',(1.46739286448532,-7.99164849993224,
30.1418721835791));
#165039=CARTESIAN_POINT('Ctrl Pts',(1.46744408230829,-7.99163909536148,
30.1418742242688));
#165040=CARTESIAN_POINT('Ctrl Pts',(1.46754641061946,-7.99162030491178,
30.1418783013634));
#165041=CARTESIAN_POINT('Ctrl Pts',(1.46759752133859,-7.99161091899257,
30.1418803377775));
#165042=CARTESIAN_POINT('Ctrl Pts',(1.46769963697649,-7.99159216557053,
30.141884406382));
#165043=CARTESIAN_POINT('Ctrl Pts',(1.46775064182439,-7.99158279808283,
30.1418864385695));
#165044=CARTESIAN_POINT('Ctrl Pts',(1.46785254719436,-7.99156408125927,
30.1418904987797));
#165045=CARTESIAN_POINT('Ctrl Pts',(1.46790344750882,-7.99155473196361,
30.1418925267941));
#165046=CARTESIAN_POINT('Ctrl Pts',(1.46800514443233,-7.99153605141637,
30.1418965786828));
#165047=CARTESIAN_POINT('Ctrl Pts',(1.46805594120636,-7.99152672013653,
30.1418986025636));
#165048=CARTESIAN_POINT('Ctrl Pts',(1.46815743237814,-7.99150807538286,
30.1419026462382));
#165049=CARTESIAN_POINT('Ctrl Pts',(1.46820812681643,-7.9914987619036,30.1419046660335));
#165050=CARTESIAN_POINT('Ctrl Pts',(1.46830941436799,-7.991480152564,30.1419087015791));
#165051=CARTESIAN_POINT('Ctrl Pts',(1.46836000756202,-7.99147085669081,
30.1419107173325));
#165052=CARTESIAN_POINT('Ctrl Pts',(1.46846109392803,-7.99145228232987,
30.1419147448461));
#165053=CARTESIAN_POINT('Ctrl Pts',(1.46851158707424,-7.99144300384882,
30.1419167566053));
#165054=CARTESIAN_POINT('Ctrl Pts',(1.46861247432569,-7.99142446409777,
30.1419207761695));
#165055=CARTESIAN_POINT('Ctrl Pts',(1.46866286849074,-7.9914152028187,30.141922783977));
#165056=CARTESIAN_POINT('Ctrl Pts',(1.46876355896914,-7.99139669725884,
30.1419267956854));
#165057=CARTESIAN_POINT('Ctrl Pts',(1.46881385525859,-7.99138745298434,
30.1419287995853));
#165058=CARTESIAN_POINT('Ctrl Pts',(1.46891435139421,-7.99136898118046,
30.1419328035347));
#165059=CARTESIAN_POINT('Ctrl Pts',(1.46896455110614,-7.99135975367763,
30.1419348035788));
#165060=CARTESIAN_POINT('Ctrl Pts',(1.4690648544144,-7.9913413153625,30.1419387998296));
#165061=CARTESIAN_POINT('Ctrl Pts',(1.4691149583401,-7.9913321044915,30.1419407960495));
#165062=CARTESIAN_POINT('Ctrl Pts',(1.46921507178171,-7.99131369913201,
30.1419447847199));
#165063=CARTESIAN_POINT('Ctrl Pts',(1.46926508117365,-7.99130450466814,
30.1419467771654));
#165064=CARTESIAN_POINT('Ctrl Pts',(1.46936500660038,-7.99128613193484,
30.1419507583292));
#165065=CARTESIAN_POINT('Ctrl Pts',(1.46941492254477,-7.99127695368385,
30.1419527470439));
#165066=CARTESIAN_POINT('Ctrl Pts',(1.46951466213173,-7.99125861318767,
30.1419567207878));
#165067=CARTESIAN_POINT('Ctrl Pts',(1.46956448573254,-7.99124945095196,
30.1419587058155));
#165068=CARTESIAN_POINT('Ctrl Pts',(1.46966404133941,-7.99123114236166,
30.1419626722138));
#165069=CARTESIAN_POINT('Ctrl Pts',(1.46971377344337,-7.99122199599084,
30.1419646535884));
#165070=CARTESIAN_POINT('Ctrl Pts',(1.46981314797316,-7.99120371878311,
30.1419686127568));
#165071=CARTESIAN_POINT('Ctrl Pts',(1.46986278998158,-7.9911945880247,30.1419705905341));
#165072=CARTESIAN_POINT('Ctrl Pts',(1.46996198475956,-7.9911763419662,30.1419745425255));
#165073=CARTESIAN_POINT('Ctrl Pts',(1.47001153762577,-7.99116722665004,
30.1419765167435));
#165074=CARTESIAN_POINT('Ctrl Pts',(1.47011055472865,-7.99114901136908,
30.1419804616408));
#165075=CARTESIAN_POINT('Ctrl Pts',(1.47016001928639,-7.9911399113469,30.1419824323328));
#165076=CARTESIAN_POINT('Ctrl Pts',(1.4702588613271,-7.99112172637295,30.1419863702401));
#165077=CARTESIAN_POINT('Ctrl Pts',(1.47030823873138,-7.99111264143732,
30.1419883374522));
#165078=CARTESIAN_POINT('Ctrl Pts',(1.47040690751414,-7.99109448644844,
30.1419922684415));
#165079=CARTESIAN_POINT('Ctrl Pts',(1.47045619877328,-7.9910854164188,30.1419942322139));
#165080=CARTESIAN_POINT('Ctrl Pts',(1.47055469649628,-7.99106729102039,
30.1419981563728));
#165081=CARTESIAN_POINT('Ctrl Pts',(1.47060390274324,-7.99105823569317,
30.1420001167507));
#165082=CARTESIAN_POINT('Ctrl Pts',(1.47070223114057,-7.99104013957588,
30.1420040341485));
#165083=CARTESIAN_POINT('Ctrl Pts',(1.47075135331427,-7.99103109878312,
30.1420059911693));
#165084=CARTESIAN_POINT('Ctrl Pts',(1.47084951467059,-7.99101303153609,
30.142009901897));
#165085=CARTESIAN_POINT('Ctrl Pts',(1.47089855389559,-7.99100400507559,
30.1420118556055));
#165086=CARTESIAN_POINT('Ctrl Pts',(1.47099654964575,-7.99098596644421,
30.1420157597204));
#165087=CARTESIAN_POINT('Ctrl Pts',(1.47104550658709,-7.99097695419828,
30.1420177101433));
#165088=CARTESIAN_POINT('Ctrl Pts',(1.47114333973886,-7.99095894363823,
30.1420216077652));
#165089=CARTESIAN_POINT('Ctrl Pts',(1.47119221574097,-7.990949945364,30.142023554956));
#165090=CARTESIAN_POINT('Ctrl Pts',(1.47128988731677,-7.99093196269629,
30.1420274461259));
#165091=CARTESIAN_POINT('Ctrl Pts',(1.47133868311205,-7.99092297826351,
30.1420293901138));
#165092=CARTESIAN_POINT('Ctrl Pts',(1.47143619576111,-7.99090502300946,
30.1420332749372));
#165093=CARTESIAN_POINT('Ctrl Pts',(1.47148491251084,-7.99089605220883,
30.1420352157686));
#165094=CARTESIAN_POINT('Ctrl Pts',(1.47158226764469,-7.9908781241175,30.1420390943018));
#165095=CARTESIAN_POINT('Ctrl Pts',(1.47163090614589,-7.99086916680671,
30.1420410320084));
#165096=CARTESIAN_POINT('Ctrl Pts',(1.47172810619937,-7.99085126543856,
30.1420449043486));
#165097=CARTESIAN_POINT('Ctrl Pts',(1.47177666756755,-7.99084232141656,
30.1420468389749));
#165098=CARTESIAN_POINT('Ctrl Pts',(1.47187371411487,-7.99082444649038,
30.1420507051848));
#165099=CARTESIAN_POINT('Ctrl Pts',(1.4719221992592,-7.99081551559405,30.142052636767));
#165100=CARTESIAN_POINT('Ctrl Pts',(1.47201909434683,-7.9907976667415,30.1420564969283));
#165101=CARTESIAN_POINT('Ctrl Pts',(1.47206750425578,-7.99078874879302,
30.1420584255059));
#165102=CARTESIAN_POINT('Ctrl Pts',(1.47216424963049,-7.99077092570082,
30.1420622796881));
#165103=CARTESIAN_POINT('Ctrl Pts',(1.47221258517073,-7.99076202054476,
30.1420642052957));
#165104=CARTESIAN_POINT('Ctrl Pts',(1.47230918291279,-7.99074422283801,
30.1420680535818));
#165105=CARTESIAN_POINT('Ctrl Pts',(1.47235744506002,-7.99073533029875,
30.1420699762582));
#165106=CARTESIAN_POINT('Ctrl Pts',(1.47245389703113,-7.99071755764268,
30.1420738187226));
#165107=CARTESIAN_POINT('Ctrl Pts',(1.47250208677945,-7.99070867754114,
30.1420757385075));
#165108=CARTESIAN_POINT('Ctrl Pts',(1.47259839466091,-7.99069092963406,
30.1420795752171));
#165109=CARTESIAN_POINT('Ctrl Pts',(1.47264651287776,-7.99068206181443,
30.1420814921451));
#165110=CARTESIAN_POINT('Ctrl Pts',(1.47274267855942,-7.99066433831609,
30.1420853231752));
#165111=CARTESIAN_POINT('Ctrl Pts',(1.47279072608794,-7.99065548262696,
30.1420872372799));
#165112=CARTESIAN_POINT('Ctrl Pts',(1.47288675182275,-7.99063778313003,
30.1420910627205));
#165113=CARTESIAN_POINT('Ctrl Pts',(1.47293472983619,-7.99062893935906,
30.1420929740487));
#165114=CARTESIAN_POINT('Ctrl Pts',(1.47303061661909,-7.99061126368791,
30.1420967939394));
#165115=CARTESIAN_POINT('Ctrl Pts',(1.47307852571092,-7.99060243172958,
30.1420987025147));
#165116=CARTESIAN_POINT('Ctrl Pts',(1.4731742761607,-7.99058477940914,30.1421025169599));
#165117=CARTESIAN_POINT('Ctrl Pts',(1.47322211740726,-7.99057595906882,
30.1421044228254));
#165118=CARTESIAN_POINT('Ctrl Pts',(1.47331773299548,-7.99055832983534,
30.1421082318838));
#165119=CARTESIAN_POINT('Ctrl Pts',(1.47336550730776,-7.99054952094884,
30.1421101350756));
#165120=CARTESIAN_POINT('Ctrl Pts',(1.47346098966733,-7.9905319145087,30.1421139388123));
#165121=CARTESIAN_POINT('Ctrl Pts',(1.4735086978039,-7.99052311693982,30.1421158393608));
#165122=CARTESIAN_POINT('Ctrl Pts',(1.47360404914403,-7.99050553289298,
30.1421196378639));
#165123=CARTESIAN_POINT('Ctrl Pts',(1.4736516921524,-7.99049674645221,30.1421215358108));
#165124=CARTESIAN_POINT('Ctrl Pts',(1.47374691378359,-7.99047918456422,
30.1421253291326));
#165125=CARTESIAN_POINT('Ctrl Pts',(1.47379449240464,-7.99047040911851,
30.1421272245075));
#165126=CARTESIAN_POINT('Ctrl Pts',(1.47388958661129,-7.99045286897516,
30.142131012739));
#165127=CARTESIAN_POINT('Ctrl Pts',(1.47393710196607,-7.99044410432126,
30.1421329055865));
#165128=CARTESIAN_POINT('Ctrl Pts',(1.47403206985605,-7.99042658572521,
30.142136688772));
#165129=CARTESIAN_POINT('Ctrl Pts',(1.47407952266179,-7.9904178317343,30.1421385791207));
#165130=CARTESIAN_POINT('Ctrl Pts',(1.47417436605759,-7.99040033435628,
30.1421423573328));
#165131=CARTESIAN_POINT('Ctrl Pts',(1.47422175695718,-7.99039159091321,
30.1421442452084));
#165132=CARTESIAN_POINT('Ctrl Pts',(1.4743164783842,-7.9903741142941,30.1421480185477));
#165133=CARTESIAN_POINT('Ctrl Pts',(1.47436380858966,-7.9903653811786,30.1421499039986));
#165134=CARTESIAN_POINT('Ctrl Pts',(1.4744584089388,-7.99034792516072,30.1421536725007));
#165135=CARTESIAN_POINT('Ctrl Pts',(1.47450567917972,-7.9903392022415,30.1421555555559));
#165136=CARTESIAN_POINT('Ctrl Pts',(1.49288206123529,-7.98694798476592,
30.1428875949228));
#165137=CARTESIAN_POINT('Ctrl Pts',(1.51119951711735,-7.98350242577363,
30.1436167655524));
#165138=CARTESIAN_POINT('Ctrl Pts',(1.55546136568063,-7.97501887059435,
30.1453776877116));
#165139=CARTESIAN_POINT('Ctrl Pts',(1.58139338011566,-7.96991725370093,
30.146408517276));
#165140=CARTESIAN_POINT('Ctrl Pts',(1.65170744605864,-7.95572764719713,
30.1492019954247));
#165141=CARTESIAN_POINT('Ctrl Pts',(1.69603922700832,-7.94639483373781,
30.1509615122151));
#165142=CARTESIAN_POINT('Ctrl Pts',(1.84292345629172,-7.91418729947237,
30.156789895026));
#165143=CARTESIAN_POINT('Ctrl Pts',(1.94511051148342,-7.88969408812483,
30.1608425384323));
#165144=CARTESIAN_POINT('Ctrl Pts',(2.36154630305787,-7.78129603544755,
30.177409404943));
#165145=CARTESIAN_POINT('Ctrl Pts',(2.67109336479942,-7.68054219511478,
30.1898607436242));
#165146=CARTESIAN_POINT('Ctrl Pts',(3.03429369939984,-7.53770385451671,
30.2049968631895));
#165147=CARTESIAN_POINT('Ctrl Pts',(3.09453211940317,-7.51317433296674,
30.2075245217721));
#165148=CARTESIAN_POINT('Ctrl Pts',(3.19023650905459,-7.47285654267423,
30.2115702360824));
#165149=CARTESIAN_POINT('Ctrl Pts',(3.22589517901687,-7.45753271343991,
30.2130843246569));
#165150=CARTESIAN_POINT('Ctrl Pts',(3.2925127203717,-7.42833751989845,30.2159259474213));
#165151=CARTESIAN_POINT('Ctrl Pts',(3.32349718996094,-7.41452660273821,
30.2172529300907));
#165152=CARTESIAN_POINT('Ctrl Pts',(3.35472447711157,-7.40037238094552,
30.2185958257017));
#165153=CARTESIAN_POINT('Ctrl Pts',(3.35505474268786,-7.40022265662057,
30.2186100290394));
#165154=CARTESIAN_POINT('Ctrl Pts',(3.35571072501243,-7.39992521721995,
30.2186382413304));
#165155=CARTESIAN_POINT('Ctrl Pts',(3.35603644202967,-7.39977750274831,
30.2186522502782));
#165156=CARTESIAN_POINT('Ctrl Pts',(3.35668341227773,-7.39948404665378,
30.2186800773963));
#165157=CARTESIAN_POINT('Ctrl Pts',(3.35700466573514,-7.3993383056309,30.2186938955598));
#165158=CARTESIAN_POINT('Ctrl Pts',(3.3576427919385,-7.39904876084293,30.2187213446339));
#165159=CARTESIAN_POINT('Ctrl Pts',(3.35795966496274,-7.39890495763199,
30.2187349755404));
#165160=CARTESIAN_POINT('Ctrl Pts',(3.35858911172659,-7.3986192535452,30.2187620535557));
#165161=CARTESIAN_POINT('Ctrl Pts',(3.35890168570724,-7.39847735321878,
30.2187755006594));
#165162=CARTESIAN_POINT('Ctrl Pts',(3.35952261400977,-7.39819542071905,
30.2188022144486));
#165163=CARTESIAN_POINT('Ctrl Pts',(3.35983096857272,-7.39805538907429,
30.2188154811296));
#165164=CARTESIAN_POINT('Ctrl Pts',(3.36044353600026,-7.39777716043799,
30.2188418373831));
#165165=CARTESIAN_POINT('Ctrl Pts',(3.36074774908447,-7.39763896396462,
30.2188549269507));
#165166=CARTESIAN_POINT('Ctrl Pts',(3.36135210975156,-7.39736437290071,
30.2188809322128));
#165167=CARTESIAN_POINT('Ctrl Pts',(3.36165225758187,-7.3972279787963,30.218893847904));
#165168=CARTESIAN_POINT('Ctrl Pts',(3.36224856240444,-7.3969569603278,30.2189195085847));
#165169=CARTESIAN_POINT('Ctrl Pts',(3.36254471960628,-7.3968223364483,30.2189322535695));
#165170=CARTESIAN_POINT('Ctrl Pts',(3.36313311611353,-7.3965548270031,30.2189575759359));
#165171=CARTESIAN_POINT('Ctrl Pts',(3.36342535565635,-7.39642194189125,
30.2189701533146));
#165172=CARTESIAN_POINT('Ctrl Pts',(3.40605668117479,-7.377033875977,30.2208049880218));
#165173=CARTESIAN_POINT('Ctrl Pts',(3.44822954070459,-7.35741557437806,
30.2226304058214));
#165174=CARTESIAN_POINT('Ctrl Pts',(3.59006003122931,-7.28995042345373,
30.22880518051));
#165175=CARTESIAN_POINT('Ctrl Pts',(3.68890840245935,-7.24043249454735,
30.2331689395441));
#165176=CARTESIAN_POINT('Ctrl Pts',(3.93610279181215,-7.11022440194357,
30.244237974039));
#165177=CARTESIAN_POINT('Ctrl Pts',(4.08300046540657,-7.02689851247347,
30.250962508483));
#165178=CARTESIAN_POINT('Ctrl Pts',(4.44541152655336,-6.80612184090205,
30.2679030383154));
#165179=CARTESIAN_POINT('Ctrl Pts',(4.6572371040205,-6.66296642533312,30.278133541243));
#165180=CARTESIAN_POINT('Ctrl Pts',(4.9096079167721,-6.4744863549968,30.2906149367545));
#165181=CARTESIAN_POINT('Ctrl Pts',(4.95685906150458,-6.43838269849963,
30.2929647836191));
#165182=CARTESIAN_POINT('Ctrl Pts',(5.02360174453563,-6.38621566313445,
30.2962999157217));
#165183=CARTESIAN_POINT('Ctrl Pts',(5.04342113744842,-6.37057518787796,
30.2972923184733));
#165184=CARTESIAN_POINT('Ctrl Pts',(5.0776894357839,-6.34327220903865,30.29901150349));
#165185=CARTESIAN_POINT('Ctrl Pts',(5.09217179928574,-6.33165212985064,
30.2997391089253));
#165186=CARTESIAN_POINT('Ctrl Pts',(5.12295458306643,-6.30677930749208,
30.301288063531));
#165187=CARTESIAN_POINT('Ctrl Pts',(5.13924370107714,-6.29351277730319,
30.3021091606912));
#165188=CARTESIAN_POINT('Ctrl Pts',(5.15558720053953,-6.28009619344603,
30.3029345695073));
#165189=CARTESIAN_POINT('Ctrl Pts',(5.15569318195253,-6.28000918748293,
30.302939922038));
#165190=CARTESIAN_POINT('Ctrl Pts',(5.15590548975005,-6.27983488335417,
30.3029506446556));
#165191=CARTESIAN_POINT('Ctrl Pts',(5.15601181693012,-6.27974758450557,
30.3029560147831));
#165192=CARTESIAN_POINT('Ctrl Pts',(5.15622482441792,-6.27957268781964,
30.3029667730077));
#165193=CARTESIAN_POINT('Ctrl Pts',(5.15633150472092,-6.27948508995576,
30.302972161105));
#165194=CARTESIAN_POINT('Ctrl Pts',(5.15654522576583,-6.27930958914404,
30.3029829556398));
#165195=CARTESIAN_POINT('Ctrl Pts',(5.15665226642527,-6.27922168623276,
30.3029883620736));
#165196=CARTESIAN_POINT('Ctrl Pts',(5.15686671522975,-6.27904556944555,
30.3029991936389));
#165197=CARTESIAN_POINT('Ctrl Pts',(5.15697412341429,-6.27895735550526,
30.3030046187728));
#165198=CARTESIAN_POINT('Ctrl Pts',(5.15718931459771,-6.27878061054486,
30.3030154881099));
#165199=CARTESIAN_POINT('Ctrl Pts',(5.15729709759758,-6.27869207949128,
30.3030209323136));
#165200=CARTESIAN_POINT('Ctrl Pts',(5.15751304573589,-6.27851469418993,
30.3030318401618));
#165201=CARTESIAN_POINT('Ctrl Pts',(5.15762121086413,-6.27842583991714,
30.3030373038062));
#165202=CARTESIAN_POINT('Ctrl Pts',(5.15783793080416,-6.27824780187878,
30.3030482509185));
#165203=CARTESIAN_POINT('Ctrl Pts',(5.15794648551746,-6.27815861815994,
30.3030537343819));
#165204=CARTESIAN_POINT('Ctrl Pts',(5.15816399201908,-6.27797991505405,
30.3030647215071));
#165205=CARTESIAN_POINT('Ctrl Pts',(5.15827294378432,-6.27789039565098,
30.3030702251683));
#165206=CARTESIAN_POINT('Ctrl Pts',(5.15849125179416,-6.27771101498763,
30.3030812530647));
#165207=CARTESIAN_POINT('Ctrl Pts',(5.15860060810347,-6.2776211536384,30.3030867773037));
#165208=CARTESIAN_POINT('Ctrl Pts',(5.15881973276674,-6.27744108275843,
30.3030978467396));
#165209=CARTESIAN_POINT('Ctrl Pts',(5.15892950116818,-6.27735087315211,
30.3031033919395));
#165210=CARTESIAN_POINT('Ctrl Pts',(5.18800642511015,-6.25345366695034,
30.3045722977923));
#165211=CARTESIAN_POINT('Ctrl Pts',(5.2168085396806,-6.22944637267108,30.3060323351036));
#165212=CARTESIAN_POINT('Ctrl Pts',(5.28210544772624,-6.17424927852298,
30.3093552393287));
#165213=CARTESIAN_POINT('Ctrl Pts',(5.31849211309834,-6.14293364675795,
30.3112162348533));
#165214=CARTESIAN_POINT('Ctrl Pts',(5.43553092929178,-6.0403865237015,30.3172365382661));
#165215=CARTESIAN_POINT('Ctrl Pts',(5.51504646368256,-5.96787471198371,
30.3213804556262));
#165216=CARTESIAN_POINT('Ctrl Pts',(5.7493593032263,-5.74551667747788,30.3337940624134));
#165217=CARTESIAN_POINT('Ctrl Pts',(5.8996610551997,-5.59107271111529,30.3420339954998));
#165218=CARTESIAN_POINT('Ctrl Pts',(6.14589558491515,-5.31705339146994,
30.3561685992208));
#165219=CARTESIAN_POINT('Ctrl Pts',(6.2449092090683,-5.20040362897507,30.3620473470211));
#165220=CARTESIAN_POINT('Ctrl Pts',(6.42515938471843,-4.97547105453828,
30.3731689837913));
#165221=CARTESIAN_POINT('Ctrl Pts',(6.50709872949034,-4.8678178953817,30.3784048732876));
#165222=CARTESIAN_POINT('Ctrl Pts',(6.63578606519205,-4.68968745430107,
30.3869457646013));
#165223=CARTESIAN_POINT('Ctrl Pts',(6.68418889519141,-4.62043762344156,
30.3902370743582));
#165224=CARTESIAN_POINT('Ctrl Pts',(6.75996815779295,-4.50833688935472,
30.3955212442209));
#165225=CARTESIAN_POINT('Ctrl Pts',(6.78803769180149,-4.46596185334051,
30.3975089066777));
#165226=CARTESIAN_POINT('Ctrl Pts',(6.84439285965936,-4.37912667004756,
30.401562557886));
#165227=CARTESIAN_POINT('Ctrl Pts',(6.87264731107048,-4.33464911213736,
30.4036286498146));
#165228=CARTESIAN_POINT('Ctrl Pts',(6.93128826621763,-4.2403229079573,30.4079891084106));
#165229=CARTESIAN_POINT('Ctrl Pts',(6.96157421715762,-4.19041522841973,
30.4102839305323));
#165230=CARTESIAN_POINT('Ctrl Pts',(7.00721703626377,-4.11334053468719,
30.4138091290514));
#165231=CARTESIAN_POINT('Ctrl Pts',(7.0229596478429,-4.08640413189459,30.4150376509937));
#165232=CARTESIAN_POINT('Ctrl Pts',(7.07691093637252,-3.9928581039347,30.4192920208487));
#165233=CARTESIAN_POINT('Ctrl Pts',(7.1143301842911,-3.92579803804068,30.4223207665638));
#165234=CARTESIAN_POINT('Ctrl Pts',(7.24808014725884,-3.67790681400281,
30.4334372111958));
#165235=CARTESIAN_POINT('Ctrl Pts',(7.33851251863353,-3.49398035093157,
30.4415338862254));
#165236=CARTESIAN_POINT('Ctrl Pts',(7.43578454744889,-3.27566180058298,
30.4509346847701));
#165237=CARTESIAN_POINT('Ctrl Pts',(7.44947627069259,-3.24440369982931,
30.4522757002718));
#165238=CARTESIAN_POINT('Ctrl Pts',(7.4773038111099,-3.17976870895714,30.4550380018823));
#165239=CARTESIAN_POINT('Ctrl Pts',(7.49141399502494,-3.14638168207501,
30.4564589521642));
#165240=CARTESIAN_POINT('Ctrl Pts',(7.52085929775964,-3.07538815393943,
30.4594683959595));
#165241=CARTESIAN_POINT('Ctrl Pts',(7.53613679786254,-3.03775888600757,
30.4610565073474));
#165242=CARTESIAN_POINT('Ctrl Pts',(7.57516587432124,-2.93952153255506,
30.4651861205042));
#165243=CARTESIAN_POINT('Ctrl Pts',(7.59847238430118,-2.87873971037574,
30.4677250730214));
#165244=CARTESIAN_POINT('Ctrl Pts',(7.68426292898823,-2.64670034033938,
30.477366695346));
#165245=CARTESIAN_POINT('Ctrl Pts',(7.74170767784476,-2.47363734453655,
30.4844539699317));
#165246=CARTESIAN_POINT('Ctrl Pts',(7.82188357613527,-2.20182751976962,
30.4955010572092));
#165247=CARTESIAN_POINT('Ctrl Pts',(7.84867225671503,-2.10434094374101,
30.4994464644676));
#165248=CARTESIAN_POINT('Ctrl Pts',(7.88659327813456,-1.95552753551339,
30.5054534458347));
#165249=CARTESIAN_POINT('Ctrl Pts',(7.89905870405772,-1.90455061542485,
30.5075083797333));
#165250=CARTESIAN_POINT('Ctrl Pts',(7.92267390389353,-1.80375487054386,
30.5115674944845));
#165251=CARTESIAN_POINT('Ctrl Pts',(7.93384974390912,-1.75394459459873,
30.5135714413131));
#165252=CARTESIAN_POINT('Ctrl Pts',(7.95575518627726,-1.6518168418978,30.5176773882836));
#165253=CARTESIAN_POINT('Ctrl Pts',(7.96643985811064,-1.59949223977298,
30.5197795461509));
#165254=CARTESIAN_POINT('Ctrl Pts',(7.9903707577024,-1.47610553600316,30.5247343769686));
#165255=CARTESIAN_POINT('Ctrl Pts',(8.00318604566494,-1.40496457375376,
30.5275894309627));
#165256=CARTESIAN_POINT('Ctrl Pts',(8.08830978631117,-0.893387501392534,
30.5481147225231));
#165257=CARTESIAN_POINT('Ctrl Pts',(8.12516527517489,-0.447837443061713,
30.5660079510785));
#165258=CARTESIAN_POINT('Ctrl Pts',(8.12524985409108,-0.00153983533529523,
30.5838443095726));
#165259=CARTESIAN_POINT('',(8.12524976787349,-0.00315471203393718,34.5839446402054));
#165260=CARTESIAN_POINT('Ctrl Pts',(8.12524985424774,-0.0015390084936643,
30.5838443426175));
#165261=CARTESIAN_POINT('Ctrl Pts',(8.12528247079636,0.170661215270594,
30.5907263532811));
#165262=CARTESIAN_POINT('Ctrl Pts',(8.11984086030867,0.342822053948763,
30.597587868216));
#165263=CARTESIAN_POINT('Ctrl Pts',(8.1069234245787,0.546339019308158,30.6056444485861));
#165264=CARTESIAN_POINT('Ctrl Pts',(8.10472878616853,0.577983606759902,
30.606895558429));
#165265=CARTESIAN_POINT('Ctrl Pts',(8.10071272379043,0.631360835254744,
30.6090028482588));
#165266=CARTESIAN_POINT('Ctrl Pts',(8.09898900937166,0.653100426989475,
30.6098602553929));
#165267=CARTESIAN_POINT('Ctrl Pts',(8.095624524121,0.69347017906358,30.6114507150424));
#165268=CARTESIAN_POINT('Ctrl Pts',(8.09400691274582,0.712102116221887,
30.6121840824149));
#165269=CARTESIAN_POINT('Ctrl Pts',(8.09054299384729,0.750462688824823,
30.6136924866601));
#165270=CARTESIAN_POINT('Ctrl Pts',(8.08868881693465,0.770190501797474,
30.6144674020753));
#165271=CARTESIAN_POINT('Ctrl Pts',(8.08444274227309,0.813659931638667,
30.6161729724052));
#165272=CARTESIAN_POINT('Ctrl Pts',(8.08201838515726,0.837398211912516,
30.6171031059458));
#165273=CARTESIAN_POINT('Ctrl Pts',(8.07217385705014,0.929764259374635,
30.6207181314146));
#165274=CARTESIAN_POINT('Ctrl Pts',(8.06398380363852,0.998307410475564,
30.6233918974572));
#165275=CARTESIAN_POINT('Ctrl Pts',(8.05031374394521,1.10152978492683,30.6274120270276));
#165276=CARTESIAN_POINT('Ctrl Pts',(8.04548081838411,1.13629118411745,30.6287647472822));
#165277=CARTESIAN_POINT('Ctrl Pts',(8.00109498567051,1.44105180738447,30.640619645082));
#165278=CARTESIAN_POINT('Ctrl Pts',(7.94818878491817,1.7089318053496,30.6510154559394));
#165279=CARTESIAN_POINT('Ctrl Pts',(7.84740436597334,2.11142273227072,30.6669273971922));
#165280=CARTESIAN_POINT('Ctrl Pts',(7.80929739861739,2.24827376586878,30.6723887332309));
#165281=CARTESIAN_POINT('Ctrl Pts',(7.74271476470716,2.46521039637097,30.6811598054927));
#165282=CARTESIAN_POINT('Ctrl Pts',(7.71653611354067,2.54597024712916,30.6844505340548));
#165283=CARTESIAN_POINT('Ctrl Pts',(7.67783370094684,2.6592802546164,30.6891077639006));
#165284=CARTESIAN_POINT('Ctrl Pts',(7.66635849801055,2.69218297705172,30.6904649335769));
#165285=CARTESIAN_POINT('Ctrl Pts',(7.64346574112435,2.75648971149616,30.6931271949241));
#165286=CARTESIAN_POINT('Ctrl Pts',(7.63206541271041,2.78789913598944,30.6944321093348));
#165287=CARTESIAN_POINT('Ctrl Pts',(7.60895125113949,2.85037731580584,30.6970371524867));
#165288=CARTESIAN_POINT('Ctrl Pts',(7.59724007399523,2.88144637880839,30.6983372346837));
#165289=CARTESIAN_POINT('Ctrl Pts',(7.56546515317382,2.96420286987429,30.7018128285314));
#165290=CARTESIAN_POINT('Ctrl Pts',(7.54506228544194,3.01575806496623,30.7039912945516));
#165291=CARTESIAN_POINT('Ctrl Pts',(7.45840977052033,3.22833184312651,30.7130296304252));
#165292=CARTESIAN_POINT('Ctrl Pts',(7.38752126880635,3.387407750811,30.7199286936997));
#165293=CARTESIAN_POINT('Ctrl Pts',(7.30899732817388,3.54940567143891,30.7270908298909));
#165294=CARTESIAN_POINT('Ctrl Pts',(7.30641098760531,3.55472657793394,30.7273262268182));
#165295=CARTESIAN_POINT('Ctrl Pts',(7.21536591222871,3.74151545316565,30.7355951172384));
#165296=CARTESIAN_POINT('Ctrl Pts',(7.12018050810158,3.91962656204717,30.7436600314797));
#165297=CARTESIAN_POINT('Ctrl Pts',(6.97729756854017,4.16457446076842,30.754952879232));
#165298=CARTESIAN_POINT('Ctrl Pts',(6.93507192500324,4.23451759860916,30.7582010978384));
#165299=CARTESIAN_POINT('Ctrl Pts',(6.87129514370992,4.33664489925658,30.7629729818043));
#165300=CARTESIAN_POINT('Ctrl Pts',(6.85055730123445,4.36933068253685,30.7645046678036));
#165301=CARTESIAN_POINT('Ctrl Pts',(6.81266698332157,4.42811828379468,30.7672666635422));
#165302=CARTESIAN_POINT('Ctrl Pts',(6.79559607843407,4.45427175982513,30.7684980110969));
#165303=CARTESIAN_POINT('Ctrl Pts',(6.7683005737375,4.49556767237572,30.7704459535256));
#165304=CARTESIAN_POINT('Ctrl Pts',(6.75817498752247,4.51077512117577,30.7711640880348));
#165305=CARTESIAN_POINT('Ctrl Pts',(6.73785024976349,4.54107844852082,30.7725965576603));
#165306=CARTESIAN_POINT('Ctrl Pts',(6.72765143860333,4.55617444668117,30.7733108909738));
#165307=CARTESIAN_POINT('Ctrl Pts',(6.70503356722658,4.58941126270888,30.7748851384559));
#165308=CARTESIAN_POINT('Ctrl Pts',(6.6925914864767,4.6075362261853,30.7757446343125));
#165309=CARTESIAN_POINT('Ctrl Pts',(6.64937187947682,4.66995182676276,30.7787082946067));
#165310=CARTESIAN_POINT('Ctrl Pts',(6.61822689426013,4.71398656045055,30.7808059613261));
#165311=CARTESIAN_POINT('Ctrl Pts',(6.37813174307391,5.04637804579907,30.7967035595993));
#165312=CARTESIAN_POINT('Ctrl Pts',(6.15086256520502,5.32103317362352,30.8102144036779));
#165313=CARTESIAN_POINT('Ctrl Pts',(5.81142103534428,5.68033132425206,30.8289850994278));
#165314=CARTESIAN_POINT('Ctrl Pts',(5.71398878704995,5.77833111347079,30.8342299777271));
#165315=CARTESIAN_POINT('Ctrl Pts',(5.35427408959011,6.12214204831554,30.8531589818201));
#165316=CARTESIAN_POINT('Ctrl Pts',(5.07825482086978,6.35296745365093,30.866898061753));
#165317=CARTESIAN_POINT('Ctrl Pts',(4.71927078629036,6.61478488161998,30.8841269456628));
#165318=CARTESIAN_POINT('Ctrl Pts',(4.64989562896481,6.66373516122892,30.8874283553265));
#165319=CARTESIAN_POINT('Ctrl Pts',(4.54874467994175,6.73275722426316,30.8922041238203));
#165320=CARTESIAN_POINT('Ctrl Pts',(4.51757660767819,6.75371006093393,30.8936706247982));
#165321=CARTESIAN_POINT('Ctrl Pts',(4.45437064610633,6.79556716008406,30.8966345757298));
#165322=CARTESIAN_POINT('Ctrl Pts',(4.42232814298473,6.8164627677941,30.8981320576086));
#165323=CARTESIAN_POINT('Ctrl Pts',(4.36029442563252,6.85629477507591,30.9010215507255));
#165324=CARTESIAN_POINT('Ctrl Pts',(4.33032440687999,6.8752626163293,30.9024132707204));
#165325=CARTESIAN_POINT('Ctrl Pts',(4.25871598755421,6.91992917558295,30.9057285954105));
#165326=CARTESIAN_POINT('Ctrl Pts',(4.21696779556318,6.94544917535118,30.9076535200677));
#165327=CARTESIAN_POINT('Ctrl Pts',(4.06075400472072,7.03901245233356,30.9148272997049));
#165328=CARTESIAN_POINT('Ctrl Pts',(3.94485213724083,7.10461544637965,30.920092790392));
#165329=CARTESIAN_POINT('Ctrl Pts',(3.46826454477096,7.35911531849033,30.9415180185751));
#165330=CARTESIAN_POINT('Ctrl Pts',(3.09524408805171,7.52362202755177,30.9577615474354));
#165331=CARTESIAN_POINT('Ctrl Pts',(2.21333738502024,7.83581909018226,30.9961228071158));
#165332=CARTESIAN_POINT('Ctrl Pts',(1.69920155889772,7.96313926510935,31.018527855726));
#165333=CARTESIAN_POINT('Ctrl Pts',(0.926181120888742,8.07625039229386,
31.0515363904339));
#165334=CARTESIAN_POINT('Ctrl Pts',(0.674393805133385,8.10116233462654,
31.0621575254606));
#165335=CARTESIAN_POINT('Ctrl Pts',(0.353219044933369,8.11785974538554,
31.0752934584494));
#165336=CARTESIAN_POINT('Ctrl Pts',(0.28454423565166,8.12055696352107,31.0780778939256));
#165337=CARTESIAN_POINT('Ctrl Pts',(0.187960759556835,8.12312355301155,
31.0819527615336));
#165338=CARTESIAN_POINT('Ctrl Pts',(0.16007515997635,8.12372091282373,31.0830666924367));
#165339=CARTESIAN_POINT('Ctrl Pts',(0.111400383025119,8.12451289055111,
31.0850020547166));
#165340=CARTESIAN_POINT('Ctrl Pts',(0.0906125788835788,8.12477132749947,
31.0858257286801));
#165341=CARTESIAN_POINT('Ctrl Pts',(0.0601811948849875,8.12503284761978,
31.08702708921));
#165342=CARTESIAN_POINT('Ctrl Pts',(0.050538324573565,8.12509854893207,
31.087407117667));
#165343=CARTESIAN_POINT('Ctrl Pts',(0.0336328899902811,8.12518363704173,
31.0880722006534));
#165344=CARTESIAN_POINT('Ctrl Pts',(0.0263703837190008,8.12521045329035,
31.0883575405795));
#165345=CARTESIAN_POINT('Ctrl Pts',(0.0122839970648353,8.12524357979321,
31.0889102432341));
#165346=CARTESIAN_POINT('Ctrl Pts',(0.00546012760196375,8.12525103088518,
31.0891776504658));
#165347=CARTESIAN_POINT('Ctrl Pts',(-0.0108075042916905,8.1252483004969,
31.0898143107965));
#165348=CARTESIAN_POINT('Ctrl Pts',(-0.0202512684566991,8.12523025113662,
31.0901832491593));
#165349=CARTESIAN_POINT('Ctrl Pts',(-0.0539249154189347,8.12510718466993,
31.091496372948));
#165350=CARTESIAN_POINT('Ctrl Pts',(-0.0781544889130888,8.12491024885604,
31.0924367883519));
#165351=CARTESIAN_POINT('Ctrl Pts',(-0.511659506401743,8.11944739357702,
31.1091785798839));
#165352=CARTESIAN_POINT('Ctrl Pts',(-0.919967366466715,8.08337124097557,
31.1234753381119));
#165353=CARTESIAN_POINT('Ctrl Pts',(-1.67958053316098,7.95793408467524,
31.1495473342186));
#165354=CARTESIAN_POINT('Ctrl Pts',(-2.03103940878968,7.87556915019174,
31.1614069321283));
#165355=CARTESIAN_POINT('Ctrl Pts',(-2.93260403420878,7.59989847859046,
31.1931467735776));
#165356=CARTESIAN_POINT('Ctrl Pts',(-3.46936823476809,7.37034701138322,
31.213491066032));
#165357=CARTESIAN_POINT('Ctrl Pts',(-4.00173808893761,7.07153350401814,
31.2370058994623));
#165358=CARTESIAN_POINT('Ctrl Pts',(-4.02642598227002,7.05750576484256,
31.2381040028691));
#165359=CARTESIAN_POINT('Ctrl Pts',(-4.06225473612356,7.03689856446319,
31.239708909996));
#165360=CARTESIAN_POINT('Ctrl Pts',(-4.07345432698614,7.03042138081406,
31.2402121938627));
#165361=CARTESIAN_POINT('Ctrl Pts',(-4.09304524164,7.01902862146628,31.2410954026919));
#165362=CARTESIAN_POINT('Ctrl Pts',(-4.10144331246228,7.0141246704718,31.2414749260792));
#165363=CARTESIAN_POINT('Ctrl Pts',(-4.11770544667906,7.00458940334058,
31.2422116242612));
#165364=CARTESIAN_POINT('Ctrl Pts',(-4.12557055360719,6.99995988999779,
31.2425687364064));
#165365=CARTESIAN_POINT('Ctrl Pts',(-4.14428612261227,6.98890114138488,
31.2434204492749));
#165366=CARTESIAN_POINT('Ctrl Pts',(-4.15512943294846,6.98245988343932,
31.2439154661339));
#165367=CARTESIAN_POINT('Ctrl Pts',(-4.19364151223203,6.9594610526682,31.2456791752966));
#165368=CARTESIAN_POINT('Ctrl Pts',(-4.22122649595426,6.94276415539712,
31.2469527029078));
#165369=CARTESIAN_POINT('Ctrl Pts',(-4.67676331132769,6.66331407014106,
31.2681551685278));
#165370=CARTESIAN_POINT('Ctrl Pts',(-5.07949684904348,6.36164092646036,
31.2895106101507));
#165371=CARTESIAN_POINT('Ctrl Pts',(-5.6418802566825,5.85274349116283,31.3230458893457));
#165372=CARTESIAN_POINT('Ctrl Pts',(-5.82373212839376,5.67182144027073,
31.3345652369883));
#165373=CARTESIAN_POINT('Ctrl Pts',(-6.36387846540575,5.0810247336261,31.3705250870506));
#165374=CARTESIAN_POINT('Ctrl Pts',(-6.68983264678388,4.64350167313261,
31.3948988468288));
#165375=CARTESIAN_POINT('Ctrl Pts',(-6.97935005797233,4.16037476210969,
31.4174732962628));
#165376=CARTESIAN_POINT('Ctrl Pts',(-6.98901697266284,4.14411476158781,
31.418228607833));
#165377=CARTESIAN_POINT('Ctrl Pts',(-7.00628258876623,4.11484130068387,
31.419580685251));
#165378=CARTESIAN_POINT('Ctrl Pts',(-7.01390201641288,4.10184021528339,
31.4201784498773));
#165379=CARTESIAN_POINT('Ctrl Pts',(-7.02600549775053,4.08105562254526,
31.4211298457988));
#165380=CARTESIAN_POINT('Ctrl Pts',(-7.03051286671243,4.07328578430004,
31.4214845609186));
#165381=CARTESIAN_POINT('Ctrl Pts',(-7.0383863138654,4.0596614716043,31.4221049250644));
#165382=CARTESIAN_POINT('Ctrl Pts',(-7.04175798972041,4.05381025478175,
31.4223708285228));
#165383=CARTESIAN_POINT('Ctrl Pts',(-7.04936917548767,4.04056363089996,
31.4229716396852));
#165384=CARTESIAN_POINT('Ctrl Pts',(-7.05360435403549,4.03316573488961,
31.4233063535936));
#165385=CARTESIAN_POINT('Ctrl Pts',(-7.06501260536965,4.01316517572387,
31.4242090781151));
#165386=CARTESIAN_POINT('Ctrl Pts',(-7.07216361362104,4.00054992059042,
31.4247761228645));
#165387=CARTESIAN_POINT('Ctrl Pts',(-7.10393441427424,3.94415092767576,
31.4273010205447));
#165388=CARTESIAN_POINT('Ctrl Pts',(-7.12818193667875,3.90015808719331,
31.429243174669));
#165389=CARTESIAN_POINT('Ctrl Pts',(-7.15513296747459,3.85016919144534,
31.4314219938937));
#165390=CARTESIAN_POINT('Ctrl Pts',(-7.15823871129711,3.84439190735535,
31.4316733820945));
#165391=CARTESIAN_POINT('Ctrl Pts',(-7.19074644531438,3.78374526672226,
31.4343079551018));
#165392=CARTESIAN_POINT('Ctrl Pts',(-7.2195243255123,3.72854279771346,31.4366686522266));
#165393=CARTESIAN_POINT('Ctrl Pts',(-7.3044836113224,3.56089943932909,31.4437389541875));
#165394=CARTESIAN_POINT('Ctrl Pts',(-7.35869388862764,3.44747894563927,
31.4483899265534));
#165395=CARTESIAN_POINT('Ctrl Pts',(-7.55990471390446,3.00010648016679,
31.466356801721));
#165396=CARTESIAN_POINT('Ctrl Pts',(-7.68697894014235,2.6576611880201,31.4793224560771));
#165397=CARTESIAN_POINT('Ctrl Pts',(-7.92752084641353,1.84565706251403,
31.5098198431401));
#165398=CARTESIAN_POINT('Ctrl Pts',(-8.02302685373317,1.37224135173242,
31.5274604729183));
#165399=CARTESIAN_POINT('Ctrl Pts',(-8.0828506232712,0.831315728240489,
31.548240037948));
#165400=CARTESIAN_POINT('Ctrl Pts',(-8.08898033149878,0.76938750580692,
31.5506267195295));
#165401=CARTESIAN_POINT('Ctrl Pts',(-8.09875036287201,0.657593557474825,
31.5549495661381));
#165402=CARTESIAN_POINT('Ctrl Pts',(-8.10264297018093,0.607752889225413,
31.556881934779));
#165403=CARTESIAN_POINT('Ctrl Pts',(-8.10786522399183,0.531872764438596,
31.5598316777369));
#165404=CARTESIAN_POINT('Ctrl Pts',(-8.10952991247481,0.505857410521775,
31.5608443827085));
#165405=CARTESIAN_POINT('Ctrl Pts',(-8.11236055637585,0.458008524910283,
31.5627095403002));
#165406=CARTESIAN_POINT('Ctrl Pts',(-8.11356363662832,0.436177389571904,
31.5635614857001));
#165407=CARTESIAN_POINT('Ctrl Pts',(-8.11573929959759,0.393568104531198,
31.5652261752182));
#165408=CARTESIAN_POINT('Ctrl Pts',(-8.11672024080398,0.37279050551324,
31.5660388173605));
#165409=CARTESIAN_POINT('Ctrl Pts',(-8.11911203612603,0.317633773093442,
31.5681985975125));
#165410=CARTESIAN_POINT('Ctrl Pts',(-8.12038431228878,0.283249136489211,
31.5695476006472));
#165411=CARTESIAN_POINT('Ctrl Pts',(-8.124187705308,0.159125845537355,31.5744276026128));
#165412=CARTESIAN_POINT('Ctrl Pts',(-8.12544991894614,0.0693556532507427,
31.577976507428));
#165413=CARTESIAN_POINT('Ctrl Pts',(-8.12364523290431,-0.648873365100727,
31.6065565417131));
#165414=CARTESIAN_POINT('Ctrl Pts',(-8.04915849450093,-1.27498306389039,
31.6328523778494));
#165415=CARTESIAN_POINT('Ctrl Pts',(-7.80688437413114,-2.29013351656759,
31.6771420373107));
#165416=CARTESIAN_POINT('Ctrl Pts',(-7.67964846878573,-2.68610772424907,
31.6947971988147));
#165417=CARTESIAN_POINT('Ctrl Pts',(-7.50307559111217,-3.11869197162453,
31.7136373202818));
#165418=CARTESIAN_POINT('Ctrl Pts',(-7.48299505776451,-3.16657039096945,
31.7157155461714));
#165419=CARTESIAN_POINT('Ctrl Pts',(-7.45690258107033,-3.22714867802599,
31.7183335330937));
#165420=CARTESIAN_POINT('Ctrl Pts',(-7.45131495196176,-3.2400293491326,
31.7188895269094));
#165421=CARTESIAN_POINT('Ctrl Pts',(-7.44232244740854,-3.2606126836703,
31.719776875421));
#165422=CARTESIAN_POINT('Ctrl Pts',(-7.43893894768588,-3.26832461933621,
31.7201090827914));
#165423=CARTESIAN_POINT('Ctrl Pts',(-7.43251301203704,-3.28290943841109,
31.7207368546782));
#165424=CARTESIAN_POINT('Ctrl Pts',(-7.42947301878973,-3.28978338473071,
31.7210325186244));
#165425=CARTESIAN_POINT('Ctrl Pts',(-7.42257632345727,-3.30531968120215,
31.7217002797579));
#165426=CARTESIAN_POINT('Ctrl Pts',(-7.41871398326682,-3.31397952738481,
31.7220721410722));
#165427=CARTESIAN_POINT('Ctrl Pts',(-7.40733106373546,-3.33938182032185,
31.7231618858423));
#165428=CARTESIAN_POINT('Ctrl Pts',(-7.39976887469859,-3.35610563567921,
31.723877985281));
#165429=CARTESIAN_POINT('Ctrl Pts',(-7.34425757278031,-3.47776936141311,
31.7290770291821));
#165430=CARTESIAN_POINT('Ctrl Pts',(-7.29413866459474,-3.58169529646949,
31.7334535791792));
#165431=CARTESIAN_POINT('Ctrl Pts',(-6.92624761706545,-4.30477253661834,
31.763512276686));
#165432=CARTESIAN_POINT('Ctrl Pts',(-6.53227769766478,-4.88195569984678,
31.7858074583021));
#165433=CARTESIAN_POINT('Ctrl Pts',(-5.72851080681119,-5.78506499444763,
31.8270755685524));
#165434=CARTESIAN_POINT('Ctrl Pts',(-5.35200188795915,-6.13504839106379,
31.8452679142687));
#165435=CARTESIAN_POINT('Ctrl Pts',(-4.92273492580914,-6.46429875253288,
31.8661105862301));
#165436=CARTESIAN_POINT('Ctrl Pts',(-4.90034498314662,-6.48128818517181,
31.8671976901516));
#165437=CARTESIAN_POINT('Ctrl Pts',(-4.86756380394301,-6.50589549292822,
31.8687894175402));
#165438=CARTESIAN_POINT('Ctrl Pts',(-4.85724178199454,-6.51360543936992,
31.8692906285841));
#165439=CARTESIAN_POINT('Ctrl Pts',(-4.83910306685712,-6.52708690622081,
31.870171435037));
#165440=CARTESIAN_POINT('Ctrl Pts',(-4.83129426504732,-6.53286902491861,
31.8705506382207));
#165441=CARTESIAN_POINT('Ctrl Pts',(-4.81611834147574,-6.54406412393385,
31.87128762502));
#165442=CARTESIAN_POINT('Ctrl Pts',(-4.80875241663528,-6.54947870689944,
31.8716453488043));
#165443=CARTESIAN_POINT('Ctrl Pts',(-4.7911554999995,-6.56236825282006,
31.872499974418));
#165444=CARTESIAN_POINT('Ctrl Pts',(-4.7809161446393,-6.56983172744738,
31.872997296715));
#165445=CARTESIAN_POINT('Ctrl Pts',(-4.74427406698634,-6.5964091433548,
31.8747771183247));
#165446=CARTESIAN_POINT('Ctrl Pts',(-4.7177740023966,-6.61538800385599,
31.8760645471377));
#165447=CARTESIAN_POINT('Ctrl Pts',(-4.26146320762387,-6.93805314176026,
31.8982386239194));
#165448=CARTESIAN_POINT('Ctrl Pts',(-3.803319967873,-7.19939473096263,31.9206954705144));
#165449=CARTESIAN_POINT('Ctrl Pts',(-3.07124336563301,-7.52750796880281,
31.9563398205341));
#165450=CARTESIAN_POINT('Ctrl Pts',(-2.81371577029783,-7.62751008427983,
31.9688146292455));
#165451=CARTESIAN_POINT('Ctrl Pts',(-2.23350151034259,-7.81942572771731,
31.9963713431774));
#165452=CARTESIAN_POINT('Ctrl Pts',(-1.90918187769633,-7.90487129567162,
32.0114163764458));
#165453=CARTESIAN_POINT('Ctrl Pts',(-1.50483039132854,-7.98505632957965,
32.0291588720601));
#165454=CARTESIAN_POINT('Ctrl Pts',(-1.42894629344759,-7.99898444079158,
32.032444915965));
#165455=CARTESIAN_POINT('Ctrl Pts',(-1.26057295362894,-8.02741588302058,
32.0396251693525));
#165456=CARTESIAN_POINT('Ctrl Pts',(-1.168006801833,-8.04140604061696,32.0434990583466));
#165457=CARTESIAN_POINT('Ctrl Pts',(-1.02180671999395,-8.06092439326722,
32.0494830105657));
#165458=CARTESIAN_POINT('Ctrl Pts',(-0.968327469031864,-8.06752334727937,
32.0516429925421));
#165459=CARTESIAN_POINT('Ctrl Pts',(-0.901075451385636,-8.07514340355942,
32.0543267051102));
#165460=CARTESIAN_POINT('Ctrl Pts',(-0.887360830051181,-8.07666197867091,
32.0548723040733));
#165461=CARTESIAN_POINT('Ctrl Pts',(-0.865554461149743,-8.079020312903,
32.0557372208834));
#165462=CARTESIAN_POINT('Ctrl Pts',(-0.85746524469735,-8.07988286402116,
32.0560575012112));
#165463=CARTESIAN_POINT('Ctrl Pts',(-0.842241128964453,-8.08148308750492,
32.0566592336269));
#165464=CARTESIAN_POINT('Ctrl Pts',(-0.83510652622942,-8.08222346283701,
32.0569407973939));
#165465=CARTESIAN_POINT('Ctrl Pts',(-0.819083944226715,-8.08386472314833,
32.0575721711827));
#165466=CARTESIAN_POINT('Ctrl Pts',(-0.810195432698298,-8.08476040037743,
32.0579217690558));
#165467=CARTESIAN_POINT('Ctrl Pts',(-0.78759852629135,-8.08699980515402,
32.0588089090743));
#165468=CARTESIAN_POINT('Ctrl Pts',(-0.773888128070361,-8.08832334018192,
32.0593456475872));
#165469=CARTESIAN_POINT('Ctrl Pts',(-0.697694270364975,-8.09548321612502,
32.0623203557184));
#165470=CARTESIAN_POINT('Ctrl Pts',(-0.635147221693498,-8.10063047244903,
32.0647318494417));
#165471=CARTESIAN_POINT('Ctrl Pts',(0.168378852009121,-8.15739204748286,
32.0953873818867));
#165472=CARTESIAN_POINT('Ctrl Pts',(0.913042336203379,-8.10789647728921,
32.1207537490992));
#165473=CARTESIAN_POINT('Ctrl Pts',(1.93143525043313,-7.89793545087173,
32.1588528104005));
#165474=CARTESIAN_POINT('Ctrl Pts',(2.21868846704255,-7.82209940438737,
32.1699286086786));
#165475=CARTESIAN_POINT('Ctrl Pts',(2.76815283081297,-7.64432964278293,
32.1918659482263));
#165476=CARTESIAN_POINT('Ctrl Pts',(3.03050839562459,-7.54416725885528,
32.2026621821433));
#165477=CARTESIAN_POINT('Ctrl Pts',(3.35722349958563,-7.39963577039196,
32.2165222905908));
#165478=CARTESIAN_POINT('Ctrl Pts',(3.42685685089504,-7.3676462444179,32.2195030852754));
#165479=CARTESIAN_POINT('Ctrl Pts',(3.53498910794463,-7.31610569219422,
32.2241769749749));
#165480=CARTESIAN_POINT('Ctrl Pts',(3.57380252766926,-7.29722453859515,
32.2258638434513));
#165481=CARTESIAN_POINT('Ctrl Pts',(3.64605904908973,-7.26135990646171,
32.2290220055994));
#165482=CARTESIAN_POINT('Ctrl Pts',(3.67953859679297,-7.2444523590404,32.2304925471651));
#165483=CARTESIAN_POINT('Ctrl Pts',(3.7543243160916,-7.20603256772677,32.2337940616937));
#165484=CARTESIAN_POINT('Ctrl Pts',(3.79556497946751,-7.1843957922038,32.2356261845027));
#165485=CARTESIAN_POINT('Ctrl Pts',(3.91606353848306,-7.11984948404659,
32.2410141334521));
#165486=CARTESIAN_POINT('Ctrl Pts',(3.99479582906798,-7.0759745911311,32.2445791751044));
#165487=CARTESIAN_POINT('Ctrl Pts',(4.61584434419199,-6.71621536902354,
32.2730727282953));
#165488=CARTESIAN_POINT('Ctrl Pts',(5.12062435961599,-6.33977408395982,
32.2986405974118));
#165489=CARTESIAN_POINT('Ctrl Pts',(5.70083760110399,-5.79216076006512,
32.330974333908));
#165490=CARTESIAN_POINT('Ctrl Pts',(5.82095447564454,-5.67143418830815,
32.3378484183871));
#165491=CARTESIAN_POINT('Ctrl Pts',(5.98111482216503,-5.50000842473647,
32.3472392679594));
#165492=CARTESIAN_POINT('Ctrl Pts',(6.02447930698563,-5.45247433443074,
32.349805954986));
#165493=CARTESIAN_POINT('Ctrl Pts',(6.09875713207264,-5.36908644935416,
32.3542421932685));
#165494=CARTESIAN_POINT('Ctrl Pts',(6.12993011458357,-5.3334683550301,32.3561165797468));
#165495=CARTESIAN_POINT('Ctrl Pts',(6.17530749837897,-5.28069698435748,
32.3588628671799));
#165496=CARTESIAN_POINT('Ctrl Pts',(6.18975533905747,-5.26375457166278,
32.3597399703606));
#165497=CARTESIAN_POINT('Ctrl Pts',(6.21609387553395,-5.2326100148138,32.3613438143193));
#165498=CARTESIAN_POINT('Ctrl Pts',(6.22800596580027,-5.21842623111169,
32.3620710485733));
#165499=CARTESIAN_POINT('Ctrl Pts',(6.25477770944952,-5.18632674838755,
32.3637099141099));
#165500=CARTESIAN_POINT('Ctrl Pts',(6.2696091020324,-5.16838766433379,32.3646209617581));
#165501=CARTESIAN_POINT('Ctrl Pts',(6.30791479292844,-5.1216480762636,32.3669826121085));
#165502=CARTESIAN_POINT('Ctrl Pts',(6.3312690393567,-5.09274978989321,32.3684309980676));
#165503=CARTESIAN_POINT('Ctrl Pts',(6.49067129282625,-4.89271599841485,
32.378381180507));
#165504=CARTESIAN_POINT('Ctrl Pts',(6.61996362776574,-4.71630864668829,
32.3867815391193));
#165505=CARTESIAN_POINT('Ctrl Pts',(6.84009164366276,-4.38904683079814,
32.4019423483583));
#165506=CARTESIAN_POINT('Ctrl Pts',(6.93343889365346,-4.24004841101013,
32.408696778887));
#165507=CARTESIAN_POINT('Ctrl Pts',(7.07767457411369,-3.99230603235469,
32.4197679513116));
#165508=CARTESIAN_POINT('Ctrl Pts',(7.1315012617118,-3.89534007995964,32.4240626430327));
#165509=CARTESIAN_POINT('Ctrl Pts',(7.20524250773771,-3.75584439742551,
32.4301982667575));
#165510=CARTESIAN_POINT('Ctrl Pts',(7.22679945378193,-3.7141965975612,32.43202476766));
#165511=CARTESIAN_POINT('Ctrl Pts',(7.26399454421795,-3.64078618164708,
32.4352356884437));
#165512=CARTESIAN_POINT('Ctrl Pts',(7.27978791650323,-3.60910357839188,
32.436618695001));
#165513=CARTESIAN_POINT('Ctrl Pts',(7.31241338036254,-3.54256912571246,
32.4395176036191));
#165514=CARTESIAN_POINT('Ctrl Pts',(7.32920451766121,-3.50769818836835,
32.441033831366));
#165515=CARTESIAN_POINT('Ctrl Pts',(7.37324690373862,-3.41453627857709,
32.4450768217813));
#165516=CARTESIAN_POINT('Ctrl Pts',(7.40005587643885,-3.35603946132916,
32.4476073888213));
#165517=CARTESIAN_POINT('Ctrl Pts',(7.5653304115969,-2.98380091827299,32.4636627246735));
#165518=CARTESIAN_POINT('Ctrl Pts',(7.68450946151777,-2.66187903421615,
32.4773568973211));
#165519=CARTESIAN_POINT('Ctrl Pts',(7.83512182652158,-2.15951533750572,
32.4983029906778));
#165520=CARTESIAN_POINT('Ctrl Pts',(7.88141179818942,-1.98393284992453,
32.5055431625944));
#165521=CARTESIAN_POINT('Ctrl Pts',(7.93145751493271,-1.76452886687975,
32.5144374058751));
#165522=CARTESIAN_POINT('Ctrl Pts',(7.94079210973867,-1.72203401057349,
32.5161529534149));
#165523=CARTESIAN_POINT('Ctrl Pts',(7.95431498375473,-1.65802322609323,
32.5187252856981));
#165524=CARTESIAN_POINT('Ctrl Pts',(7.95875820721713,-1.63656215372334,
32.5195856981216));
#165525=CARTESIAN_POINT('Ctrl Pts',(7.96707320446151,-1.59556533455696,
32.5212254835987));
#165526=CARTESIAN_POINT('Ctrl Pts',(7.97096007348666,-1.57603289691244,
32.5220051002901));
#165527=CARTESIAN_POINT('Ctrl Pts',(7.97976232866371,-1.53093387861084,
32.5238016156476));
#165528=CARTESIAN_POINT('Ctrl Pts',(7.9846267308726,-1.50535754483411,32.5248178085377));
#165529=CARTESIAN_POINT('Ctrl Pts',(7.99750618907957,-1.43582001361855,
32.5275740537169));
#165530=CARTESIAN_POINT('Ctrl Pts',(8.00528167191042,-1.39181526713075,
32.5293111077043));
#165531=CARTESIAN_POINT('Ctrl Pts',(8.05157034809311,-1.11661778338643,
32.5401359972281));
#165532=CARTESIAN_POINT('Ctrl Pts',(8.08042845627572,-0.883910872356917,
32.5491235740261));
#165533=CARTESIAN_POINT('Ctrl Pts',(8.11659211714103,-0.433495816826945,
32.5664456895671));
#165534=CARTESIAN_POINT('Ctrl Pts',(8.12528685465813,-0.216100174705383,
32.5747735029619));
#165535=CARTESIAN_POINT('Ctrl Pts',(8.1252148313152,0.207564060050729,32.5910810763637));
#165536=CARTESIAN_POINT('Ctrl Pts',(8.11733180208154,0.413668928979134,
32.5990503936479));
#165537=CARTESIAN_POINT('Ctrl Pts',(8.09637390907078,0.687860569421236,
32.6097490170675));
#165538=CARTESIAN_POINT('Ctrl Pts',(8.09025818525974,0.756402722435157,
32.6124313259992));
#165539=CARTESIAN_POINT('Ctrl Pts',(8.07813975817032,0.875158272765247,
32.6170935771905));
#165540=CARTESIAN_POINT('Ctrl Pts',(8.07253755769331,0.925408727783274,
32.6190710091661));
#165541=CARTESIAN_POINT('Ctrl Pts',(8.05956375811885,1.03267845500922,32.6233025143087));
#165542=CARTESIAN_POINT('Ctrl Pts',(8.0520552479269,1.08967840149722,32.6255572385031));
#165543=CARTESIAN_POINT('Ctrl Pts',(8.03043517581979,1.24135428422705,32.6315738916608));
#165544=CARTESIAN_POINT('Ctrl Pts',(8.01525451054449,1.33586848182048,32.6353407045382));
#165545=CARTESIAN_POINT('Ctrl Pts',(7.973354691458,1.57021131428595,32.6447229341092));
#165546=CARTESIAN_POINT('Ctrl Pts',(7.94462414572993,1.70964782061066,32.6503437383102));
#165547=CARTESIAN_POINT('Ctrl Pts',(7.88309418467115,1.97305281031318,32.6610220856643));
#165548=CARTESIAN_POINT('Ctrl Pts',(7.85099411561768,2.09714160038705,32.6660783754364));
#165549=CARTESIAN_POINT('Ctrl Pts',(7.80352648557912,2.26422971382283,32.6729098821461));
#165550=CARTESIAN_POINT('Ctrl Pts',(7.79071236860552,2.30793470785181,32.6746989234244));
#165551=CARTESIAN_POINT('Ctrl Pts',(7.76501602029368,2.39292370613741,32.6781810876642));
#165552=CARTESIAN_POINT('Ctrl Pts',(7.75217030621685,2.43421716674739,32.67987437888));
#165553=CARTESIAN_POINT('Ctrl Pts',(7.70549457704128,2.58014201066397,32.6858662049425));
#165554=CARTESIAN_POINT('Ctrl Pts',(7.66987079878365,2.68418731722489,32.6901531768509));
#165555=CARTESIAN_POINT('Ctrl Pts',(7.54792257124269,3.0180829679344,32.7039996722679));
#165556=CARTESIAN_POINT('Ctrl Pts',(7.45329089396366,3.24475181393152,32.7135410718613));
#165557=CARTESIAN_POINT('Ctrl Pts',(7.32233868847677,3.52233096797071,32.7255396766941));
#165558=CARTESIAN_POINT('Ctrl Pts',(7.29550617516009,3.57757584597496,32.7279435012674));
#165559=CARTESIAN_POINT('Ctrl Pts',(7.24334663466436,3.68193840358759,32.7325170129718));
#165560=CARTESIAN_POINT('Ctrl Pts',(7.21813976619774,3.73111232306919,32.7346858883515));
#165561=CARTESIAN_POINT('Ctrl Pts',(7.15713918955166,3.84718101541651,32.7398401442193));
#165562=CARTESIAN_POINT('Ctrl Pts',(7.12090634880916,3.91383901596761,32.7428281175572));
#165563=CARTESIAN_POINT('Ctrl Pts',(6.97427729022818,4.1748159634934,32.7546431837811));
#165564=CARTESIAN_POINT('Ctrl Pts',(6.85681840337655,4.36505116611303,32.7635168717157));
#165565=CARTESIAN_POINT('Ctrl Pts',(6.61715442447659,4.71961543042617,32.7805929966325));
#165566=CARTESIAN_POINT('Ctrl Pts',(6.49628584743972,4.88464657636596,32.7887818613617));
#165567=CARTESIAN_POINT('Ctrl Pts',(6.22636072498286,5.2254314730179,32.8061822103099));
#165568=CARTESIAN_POINT('Ctrl Pts',(6.0757915542451,5.39976487694747,32.8153852092055));
#165569=CARTESIAN_POINT('Ctrl Pts',(5.88393646439128,5.60370000057754,32.826458874718));
#165570=CARTESIAN_POINT('Ctrl Pts',(5.84951953762156,5.63961729505303,32.8284213410047));
#165571=CARTESIAN_POINT('Ctrl Pts',(5.79732235758433,5.69309804814422,32.8313606706472));
#165572=CARTESIAN_POINT('Ctrl Pts',(5.77978746277707,5.71089912315492,32.8323419441815));
#165573=CARTESIAN_POINT('Ctrl Pts',(5.748265107292,5.74260610010903,32.8340948228185));
#165574=CARTESIAN_POINT('Ctrl Pts',(5.73430861107618,5.75654247973182,32.8348670439069));
#165575=CARTESIAN_POINT('Ctrl Pts',(5.70396513175934,5.78662237184294,32.8365375063944));
#165576=CARTESIAN_POINT('Ctrl Pts',(5.68756014066338,5.80274731035957,32.8374352974443));
#165577=CARTESIAN_POINT('Ctrl Pts',(5.63507108063098,5.853903887184,32.840291272097));
#165578=CARTESIAN_POINT('Ctrl Pts',(5.59873007104388,5.88867034602701,32.8422439569608));
#165579=CARTESIAN_POINT('Ctrl Pts',(5.50923195387236,5.97271331004832,32.8469976905782));
#165580=CARTESIAN_POINT('Ctrl Pts',(5.45573363886717,6.0216203443547,32.8497927398034));
#165581=CARTESIAN_POINT('Ctrl Pts',(5.21434179889784,6.23643765490802,32.8622222596676));
#165582=CARTESIAN_POINT('Ctrl Pts',(5.01948474468476,6.39431693517205,32.871778192934));
#165583=CARTESIAN_POINT('Ctrl Pts',(4.65316637916709,6.66404145962618,32.8892158365611));
#165584=CARTESIAN_POINT('Ctrl Pts',(4.48418521203038,6.77890017180955,32.8970725600345));
#165585=CARTESIAN_POINT('Ctrl Pts',(4.26225348471805,6.91781741855808,32.9072289483574));
#165586=CARTESIAN_POINT('Ctrl Pts',(4.21312639666072,6.94784632284871,32.9094671584578));
#165587=CARTESIAN_POINT('Ctrl Pts',(4.13484063120782,6.99456279898814,32.9130192694158));
#165588=CARTESIAN_POINT('Ctrl Pts',(4.10589040136404,7.01159609485373,32.9143297340322));
#165589=CARTESIAN_POINT('Ctrl Pts',(4.04609244235053,7.04628175971614,32.9170304132808));
#165590=CARTESIAN_POINT('Ctrl Pts',(4.01523283882967,7.06391222542537,32.9184208089124));
#165591=CARTESIAN_POINT('Ctrl Pts',(3.94252577172092,7.10482027033506,32.9216891320663));
#165592=CARTESIAN_POINT('Ctrl Pts',(3.90058628947827,7.12793147460847,32.9235685934922));
#165593=CARTESIAN_POINT('Ctrl Pts',(3.75465751071743,7.20667348580747,32.9300888076946));
#165594=CARTESIAN_POINT('Ctrl Pts',(3.64966368146107,7.26040979659319,32.9347464889797));
#165595=CARTESIAN_POINT('Ctrl Pts',(3.33667353415491,7.41209423074448,32.9485329851351));
#165596=CARTESIAN_POINT('Ctrl Pts',(3.12564873000594,7.50352249827698,32.9577063713795));
#165597=CARTESIAN_POINT('Ctrl Pts',(2.75496299822714,7.64577082206427,32.9735391667336));
#165598=CARTESIAN_POINT('Ctrl Pts',(2.5970800979167,7.70083166089534,32.9801968469499));
#165599=CARTESIAN_POINT('Ctrl Pts',(2.40494039904607,7.76125776786437,32.9881549154239));
#165600=CARTESIAN_POINT('Ctrl Pts',(2.37220556374065,7.7713255780076,32.9895057097309));
#165601=CARTESIAN_POINT('Ctrl Pts',(2.32164826973755,7.78652559171573,32.9915836394985));
#165602=CARTESIAN_POINT('Ctrl Pts',(2.30387031532559,7.79180422312438,32.9923127453324));
#165603=CARTESIAN_POINT('Ctrl Pts',(2.2700682077112,7.8017149472182,32.9936959194609));
#165604=CARTESIAN_POINT('Ctrl Pts',(2.25404755821642,7.80635865129979,32.9943501568963));
#165605=CARTESIAN_POINT('Ctrl Pts',(2.21501133281587,7.81754340275779,32.995940950572));
#165606=CARTESIAN_POINT('Ctrl Pts',(2.19198091453339,7.82403219156989,32.9968766664075));
#165607=CARTESIAN_POINT('Ctrl Pts',(2.11420729352716,7.8455744516473,33.0000275551866));
#165608=CARTESIAN_POINT('Ctrl Pts',(2.05933483172817,7.8601559194015,33.002235600231));
#165609=CARTESIAN_POINT('Ctrl Pts',(1.92509061931744,7.89432686384117,33.007605324992));
#165610=CARTESIAN_POINT('Ctrl Pts',(1.84556714299306,7.91329593870069,33.0107589549172));
#165611=CARTESIAN_POINT('Ctrl Pts',(1.37617050839793,8.01780234030301,33.0292443542907));
#165612=CARTESIAN_POINT('Ctrl Pts',(0.980704518829582,8.07571821241874,
33.0443100834936));
#165613=CARTESIAN_POINT('Ctrl Pts',(0.187528273138893,8.13273611939767,
33.0745516796444));
#165614=CARTESIAN_POINT('Ctrl Pts',(-0.209069287422505,8.13221031865402,
33.0896887638983));
#165615=CARTESIAN_POINT('Ctrl Pts',(-0.67712071932834,8.09731843804846,
33.1079189984643));
#165616=CARTESIAN_POINT('Ctrl Pts',(-0.75012628911817,8.09088183237677,
33.1107724829534));
#165617=CARTESIAN_POINT('Ctrl Pts',(-0.86575850440745,8.07910849276919,
33.1153094545543));
#165618=CARTESIAN_POINT('Ctrl Pts',(-0.908447256264389,8.07441981770192,
33.1169881647341));
#165619=CARTESIAN_POINT('Ctrl Pts',(-0.988366222594918,8.06500019117109,
33.1201382782823));
#165620=CARTESIAN_POINT('Ctrl Pts',(-1.02560476084279,8.06034929377814,
33.1216090816124));
#165621=CARTESIAN_POINT('Ctrl Pts',(-1.10929159725117,8.04930791397624,
33.1249213741454));
#165622=CARTESIAN_POINT('Ctrl Pts',(-1.15571946767966,8.04277304381749,
33.1267637856276));
#165623=CARTESIAN_POINT('Ctrl Pts',(-1.29662017735922,8.0216955794533,33.1323702017767));
#165624=CARTESIAN_POINT('Ctrl Pts',(-1.39089500128511,8.00588750870998,
33.1361419851181));
#165625=CARTESIAN_POINT('Ctrl Pts',(-1.87661071241143,7.9156038243077,33.1556837957243));
#165626=CARTESIAN_POINT('Ctrl Pts',(-2.26245830105097,7.81407215881483,
33.1715106457957));
#165627=CARTESIAN_POINT('Ctrl Pts',(-3.17441249612268,7.50086161851529,
33.2107606324346));
#165628=CARTESIAN_POINT('Ctrl Pts',(-3.68885167627541,7.26168892426218,
33.2346432486699));
#165629=CARTESIAN_POINT('Ctrl Pts',(-4.44555375225147,6.80857926200083,
33.271950159523));
#165630=CARTESIAN_POINT('Ctrl Pts',(-4.70716935697516,6.63040479873872,
33.2852665966486));
#165631=CARTESIAN_POINT('Ctrl Pts',(-5.01309809244351,6.39479612948546,
33.3009020541447));
#165632=CARTESIAN_POINT('Ctrl Pts',(-5.06790667848614,6.35144804333882,
33.3037050848216));
#165633=CARTESIAN_POINT('Ctrl Pts',(-5.13325094679323,6.29838286980679,
33.3070426977266));
#165634=CARTESIAN_POINT('Ctrl Pts',(-5.14432798413,6.2893387293319,33.3076083333918));
#165635=CARTESIAN_POINT('Ctrl Pts',(-5.16241166554682,6.27449409067359,
33.3085314295035));
#165636=CARTESIAN_POINT('Ctrl Pts',(-5.16943252351469,6.26871100658931,
33.3088897341949));
#165637=CARTESIAN_POINT('Ctrl Pts',(-5.18198469426588,6.2583363498778,33.3095301584647));
#165638=CARTESIAN_POINT('Ctrl Pts',(-5.187519646386,6.25374920816197,33.3098124988295));
#165639=CARTESIAN_POINT('Ctrl Pts',(-5.19922620390779,6.24402105709245,
33.3104095184286));
#165640=CARTESIAN_POINT('Ctrl Pts',(-5.20539629162219,6.238878226779,33.3107241041577));
#165641=CARTESIAN_POINT('Ctrl Pts',(-5.22179231492686,6.22517072094772,
33.3115598264899));
#165642=CARTESIAN_POINT('Ctrl Pts',(-5.23200483001681,6.21658997736299,
33.3120801209566));
#165643=CARTESIAN_POINT('Ctrl Pts',(-5.27941937711179,6.17655180146707,
33.314494392046));
#165644=CARTESIAN_POINT('Ctrl Pts',(-5.31635998682655,6.14478460519842,
33.3163714649488));
#165645=CARTESIAN_POINT('Ctrl Pts',(-5.63828225135742,5.86287020820128,
33.3326776606034));
#165646=CARTESIAN_POINT('Ctrl Pts',(-5.9057365426996,5.59337054007154,33.345885074585));
#165647=CARTESIAN_POINT('Ctrl Pts',(-6.47473094779781,4.93352346552174,
33.3753885300817));
#165648=CARTESIAN_POINT('Ctrl Pts',(-6.76154366202761,4.53247494956825,
33.3914161624046));
#165649=CARTESIAN_POINT('Ctrl Pts',(-7.23483215105991,3.72479549759572,
33.4235711503161));
#165650=CARTESIAN_POINT('Ctrl Pts',(-7.42754090550808,3.32392553683809,
33.4394835533475));
#165651=CARTESIAN_POINT('Ctrl Pts',(-7.59795117892184,2.87955605455806,
33.4577833649623));
#165652=CARTESIAN_POINT('Ctrl Pts',(-7.60919785367271,2.84970405217055,
33.4590155157355));
#165653=CARTESIAN_POINT('Ctrl Pts',(-7.62462518739809,2.80801280673342,
33.4607403887706));
#165654=CARTESIAN_POINT('Ctrl Pts',(-7.62895470053215,2.79622877222548,
33.4612283736669));
#165655=CARTESIAN_POINT('Ctrl Pts',(-7.63637918944062,2.77587525870261,
33.4620720121724));
#165656=CARTESIAN_POINT('Ctrl Pts',(-7.63948709919662,2.76731050612988,
33.4624272545863));
#165657=CARTESIAN_POINT('Ctrl Pts',(-7.64588545697751,2.7495850390564,33.4631629581514));
#165658=CARTESIAN_POINT('Ctrl Pts',(-7.64917386217789,2.74042360477825,
33.4635434833142));
#165659=CARTESIAN_POINT('Ctrl Pts',(-7.65681295154492,2.71902037095412,
33.4644331275457));
#165660=CARTESIAN_POINT('Ctrl Pts',(-7.66115074698399,2.70677401766435,
33.464942653103));
#165661=CARTESIAN_POINT('Ctrl Pts',(-7.67497213568423,2.66745443768777,
33.4665802010536));
#165662=CARTESIAN_POINT('Ctrl Pts',(-7.68434168568798,2.64034151158299,
33.46771181527));
#165663=CARTESIAN_POINT('Ctrl Pts',(-7.82199843728846,2.23506073598694,
33.4846641574656));
#165664=CARTESIAN_POINT('Ctrl Pts',(-7.92236684617675,1.84802748926903,
33.5013711828175));
#165665=CARTESIAN_POINT('Ctrl Pts',(-8.11431059827551,0.793631006419028,
33.5479877968932));
#165666=CARTESIAN_POINT('Ctrl Pts',(-8.15214524576274,0.119707986867872,
33.5790717026292));
#165667=CARTESIAN_POINT('Ctrl Pts',(-8.08979768496112,-0.797344986955767,
33.6189498864962));
#165668=CARTESIAN_POINT('Ctrl Pts',(-8.06184921967412,-1.04269300039899,
33.6293382421936));
#165669=CARTESIAN_POINT('Ctrl Pts',(-8.01935850934616,-1.30768503771266,
33.640054614647));
#165670=CARTESIAN_POINT('Ctrl Pts',(-8.01586544542677,-1.32892897937696,
33.6409106423736));
#165671=CARTESIAN_POINT('Ctrl Pts',(-8.01064672141316,-1.35989860736942,
33.6421543496556));
#165672=CARTESIAN_POINT('Ctrl Pts',(-8.00898771469601,-1.36963531809947,
33.6425447565389));
#165673=CARTESIAN_POINT('Ctrl Pts',(-8.00602229080303,-1.38684976259633,
33.6432339491426));
#165674=CARTESIAN_POINT('Ctrl Pts',(-8.00472314284669,-1.39432872441258,
33.6435330258265));
#165675=CARTESIAN_POINT('Ctrl Pts',(-8.00200936854663,-1.40982263719879,
33.6441519072817));
#165676=CARTESIAN_POINT('Ctrl Pts',(-8.00059317627839,-1.41783730764706,
33.6444716499121));
#165677=CARTESIAN_POINT('Ctrl Pts',(-7.99770100236625,-1.43406270198511,
33.645118184647));
#165678=CARTESIAN_POINT('Ctrl Pts',(-7.99622441285837,-1.44227330847059,
33.6454449527693));
#165679=CARTESIAN_POINT('Ctrl Pts',(-7.99036609639732,-1.47456305777359,
33.6467284970901));
#165680=CARTESIAN_POINT('Ctrl Pts',(-7.98588820377531,-1.49862476222004,
33.6476816158453));
#165681=CARTESIAN_POINT('Ctrl Pts',(-7.97484755090284,-1.55649614028407,
33.6499665775846));
#165682=CARTESIAN_POINT('Ctrl Pts',(-7.96817838746579,-1.59028516925733,
33.6512945876178));
#165683=CARTESIAN_POINT('Ctrl Pts',(-7.87812716199637,-2.03173259818602,
33.6685749822379));
#165684=CARTESIAN_POINT('Ctrl Pts',(-7.76375964116079,-2.43246798265785,
33.6835144469549));
#165685=CARTESIAN_POINT('Ctrl Pts',(-7.40130286211927,-3.41083372520171,
33.7209762249408));
#165686=CARTESIAN_POINT('Ctrl Pts',(-7.1160617334785,-3.97173797477331,
33.7435258618707));
#165687=CARTESIAN_POINT('Ctrl Pts',(-6.71934526035408,-4.56926660170042,
33.7709207418354));
#165688=CARTESIAN_POINT('Ctrl Pts',(-6.66828894152333,-4.64345994866827,
33.7743827768551));
#165689=CARTESIAN_POINT('Ctrl Pts',(-6.59601827954355,-4.74483049751722,
33.7791982912188));
#165690=CARTESIAN_POINT('Ctrl Pts',(-6.57584819510753,-4.77274492226766,
33.7805334602269));
#165691=CARTESIAN_POINT('Ctrl Pts',(-6.54320851785536,-4.81731696733,33.7826800456467));
#165692=CARTESIAN_POINT('Ctrl Pts',(-6.53085130460895,-4.83405644417927,
33.7834895701032));
#165693=CARTESIAN_POINT('Ctrl Pts',(-6.50537813431219,-4.86828726139497,
33.7851518572876));
#165694=CARTESIAN_POINT('Ctrl Pts',(-6.49225559268988,-4.88577351561603,
33.7860047104204));
#165695=CARTESIAN_POINT('Ctrl Pts',(-6.46424224172423,-4.92279016060579,
33.7878181159801));
#165696=CARTESIAN_POINT('Ctrl Pts',(-6.44933313984825,-4.94230642215768,
33.7887789728178));
#165697=CARTESIAN_POINT('Ctrl Pts',(-6.40603611082097,-4.99845341838384,
33.7915574136489));
#165698=CARTESIAN_POINT('Ctrl Pts',(-6.37742309055053,-5.03490912647706,
33.7933789086692));
#165699=CARTESIAN_POINT('Ctrl Pts',(-6.31253952978128,-5.11613643932448,
33.7974782060486));
#165700=CARTESIAN_POINT('Ctrl Pts',(-6.27610156364835,-5.16077091717461,
33.79975909037));
#165701=CARTESIAN_POINT('Ctrl Pts',(-5.97297074854373,-5.52413045624327,
33.8185697154205));
#165702=CARTESIAN_POINT('Ctrl Pts',(-5.68267465692152,-5.82233396317462,
33.8356029037756));
#165703=CARTESIAN_POINT('Ctrl Pts',(-4.95011341237386,-6.46764740613027,
33.8765686475052));
#165704=CARTESIAN_POINT('Ctrl Pts',(-4.49214409700214,-6.79372582829143,
33.900783458123));
#165705=CARTESIAN_POINT('Ctrl Pts',(-3.93214788560305,-7.11089089617738,
33.927214717837));
#165706=CARTESIAN_POINT('Ctrl Pts',(-3.85941100478618,-7.15062958733917,
33.9305880209453));
#165707=CARTESIAN_POINT('Ctrl Pts',(-3.74723530029025,-7.20970473276271,
33.9356877646213));
#165708=CARTESIAN_POINT('Ctrl Pts',(-3.70822729570702,-7.22984544342074,
33.9374424741675));
#165709=CARTESIAN_POINT('Ctrl Pts',(-3.65677885777473,-7.25588349766887,
33.9397307565242));
#165710=CARTESIAN_POINT('Ctrl Pts',(-3.64448432787603,-7.26206657453796,
33.9402756423671));
#165711=CARTESIAN_POINT('Ctrl Pts',(-3.62544209724839,-7.27158262002453,
33.9411165244803));
#165712=CARTESIAN_POINT('Ctrl Pts',(-3.618705404597,-7.27493748396271,33.9414134183786));
#165713=CARTESIAN_POINT('Ctrl Pts',(-3.60525495409538,-7.28161248460411,
33.9420050055379));
#165714=CARTESIAN_POINT('Ctrl Pts',(-3.59854124752889,-7.28493270732433,
33.9422997022343));
#165715=CARTESIAN_POINT('Ctrl Pts',(-3.58360488734655,-7.29229370728755,
33.9429540050611));
#165716=CARTESIAN_POINT('Ctrl Pts',(-3.57537996334899,-7.29632987333364,
33.9433134149623));
#165717=CARTESIAN_POINT('Ctrl Pts',(-3.55341736040113,-7.30706139126438,
33.9442707216236));
#165718=CARTESIAN_POINT('Ctrl Pts',(-3.5396675495396,-7.31373193080876,
33.9448675401887));
#165719=CARTESIAN_POINT('Ctrl Pts',(-3.45276213509059,-7.35559046718009,
33.9486235631744));
#165720=CARTESIAN_POINT('Ctrl Pts',(-3.37910137013628,-7.38971937890137,
33.9517334707855));
#165721=CARTESIAN_POINT('Ctrl Pts',(-3.15744706403265,-7.48840976585039,
33.9608647035056));
#165722=CARTESIAN_POINT('Ctrl Pts',(-3.00802815570864,-7.54967042149677,
33.9667327855221));
#165723=CARTESIAN_POINT('Ctrl Pts',(-2.54822416056238,-7.72236667659126,
33.9841656014499));
#165724=CARTESIAN_POINT('Ctrl Pts',(-2.23278909703562,-7.81940290782685,
33.9952850637137));
#165725=CARTESIAN_POINT('Ctrl Pts',(-1.66537994019427,-7.95680548702152,
34.014919921732));
#165726=CARTESIAN_POINT('Ctrl Pts',(-1.41577032388048,-8.00498822318895,
34.0234356572105));
#165727=CARTESIAN_POINT('Ctrl Pts',(-0.675254841694477,-8.11220772453912,
34.0490198485259));
#165728=CARTESIAN_POINT('Ctrl Pts',(-0.180803789254281,-8.13825099129294,
34.0665743506315));
#165729=CARTESIAN_POINT('Ctrl Pts',(0.345096415947835,-8.11798204425424,
34.0868109876204));
#165730=CARTESIAN_POINT('Ctrl Pts',(0.377258515518901,-8.11655099112909,
34.0880544864004));
#165731=CARTESIAN_POINT('Ctrl Pts',(0.421998725643097,-8.11429377648015,
34.0897926938534));
#165732=CARTESIAN_POINT('Ctrl Pts',(0.434584875729363,-8.11362942212407,
34.0902826047125));
#165733=CARTESIAN_POINT('Ctrl Pts',(0.456279798934822,-8.11243363973997,
34.091128677513));
#165734=CARTESIAN_POINT('Ctrl Pts',(0.465389332093407,-8.11191614743428,
34.0914844255091));
#165735=CARTESIAN_POINT('Ctrl Pts',(0.484207668082196,-8.11081531646407,
34.0922203388239));
#165736=CARTESIAN_POINT('Ctrl Pts',(0.493916332083764,-8.11022988698553,
34.0926005656683));
#165737=CARTESIAN_POINT('Ctrl Pts',(0.516544678422956,-8.10882462185563,
34.0934880823108));
#165738=CARTESIAN_POINT('Ctrl Pts',(0.529463482458952,-8.10799134013463,
34.0939957705801));
#165739=CARTESIAN_POINT('Ctrl Pts',(0.570754115866871,-8.10522892853629,
34.0956216247193));
#165740=CARTESIAN_POINT('Ctrl Pts',(0.599117688160791,-8.10318173439424,
34.0967432944178));
#165741=CARTESIAN_POINT('Ctrl Pts',(1.22279740266531,-8.05487401314389,
34.1215150127503));
#165742=CARTESIAN_POINT('Ctrl Pts',(1.81114176485396,-7.94328741004424,
34.1472219782726));
#165743=CARTESIAN_POINT('Ctrl Pts',(2.67870071124136,-7.67728061249906,
34.1878190799151));
#165744=CARTESIAN_POINT('Ctrl Pts',(2.97006393104812,-7.56933237039539,
34.2019094294658));
#165745=CARTESIAN_POINT('Ctrl Pts',(3.65366591513917,-7.27049966854171,
34.2353702913956));
#165746=CARTESIAN_POINT('Ctrl Pts',(4.0381867641873,-7.06417741010834,34.2545264991492));
#165747=CARTESIAN_POINT('Ctrl Pts',(4.43007032808527,-6.81139492856672,
34.2732198434407));
#165748=CARTESIAN_POINT('Ctrl Pts',(4.45569197321239,-6.79466210065862,
34.274438504391));
#165749=CARTESIAN_POINT('Ctrl Pts',(4.49088419683294,-6.7713943137474,34.2761083698036));
#165750=CARTESIAN_POINT('Ctrl Pts',(4.50053601990347,-6.76498317493022,
34.2765659288214));
#165751=CARTESIAN_POINT('Ctrl Pts',(4.51589424193868,-6.75473419527171,
34.2772933942727));
#165752=CARTESIAN_POINT('Ctrl Pts',(4.52160951732829,-6.75090973324119,
34.2775639710552));
#165753=CARTESIAN_POINT('Ctrl Pts',(4.53272636786691,-6.74345027611619,
34.2780900220962));
#165754=CARTESIAN_POINT('Ctrl Pts',(4.53812844082812,-6.73981603660379,
34.2783455332897));
#165755=CARTESIAN_POINT('Ctrl Pts',(4.55105260527848,-6.7310987339041,34.2789565668001));
#165756=CARTESIAN_POINT('Ctrl Pts',(4.5585705673934,-6.72600954240551,34.2793117900612));
#165757=CARTESIAN_POINT('Ctrl Pts',(4.57419979502485,-6.71539128867663,
34.2800498580517));
#165758=CARTESIAN_POINT('Ctrl Pts',(4.58230960524889,-6.70986010342584,
34.2804326005274));
#165759=CARTESIAN_POINT('Ctrl Pts',(4.62268420443701,-6.68221582344231,
34.282337023455));
#165760=CARTESIAN_POINT('Ctrl Pts',(4.65479935830878,-6.65988442553224,
34.2838484920453));
#165761=CARTESIAN_POINT('Ctrl Pts',(4.76582298799821,-6.5814883085693,34.2890663176853));
#165762=CARTESIAN_POINT('Ctrl Pts',(4.8438913464674,-6.52424512882819,34.2927223269575));
#165763=CARTESIAN_POINT('Ctrl Pts',(5.15829651597877,-6.2849544377533,34.3074663557614));
#165764=CARTESIAN_POINT('Ctrl Pts',(5.3855523049217,-6.09134742262948,34.3181820223332));
#165765=CARTESIAN_POINT('Ctrl Pts',(5.85317095283381,-5.6462946223562,34.3413139571226));
#165766=CARTESIAN_POINT('Ctrl Pts',(6.08908327940377,-5.39104025281047,
34.353706048313));
#165767=CARTESIAN_POINT('Ctrl Pts',(6.3156060260362,-5.11204028791617,34.3668330060366));
#165768=CARTESIAN_POINT('Ctrl Pts',(6.32324826142825,-5.10258432612098,
34.3672774078631));
#165769=CARTESIAN_POINT('Ctrl Pts',(6.37582500265867,-5.03723007467763,
34.3703454820283));
#165770=CARTESIAN_POINT('Ctrl Pts',(6.42003863745138,-4.98075647501979,
34.3729796857612));
#165771=CARTESIAN_POINT('Ctrl Pts',(6.74175157660048,-4.55843405440522,
34.3925682400157));
#165772=CARTESIAN_POINT('Ctrl Pts',(6.98852941388315,-4.17024653751808,
34.4100350729619));
#165773=CARTESIAN_POINT('Ctrl Pts',(7.25367663233563,-3.66288218579916,
34.4321517180385));
#165774=CARTESIAN_POINT('Ctrl Pts',(7.304058251123,-3.56135695340024,34.4365456890109));
#165775=CARTESIAN_POINT('Ctrl Pts',(7.37199521170549,-3.41694525725551,
34.4427610488648));
#165776=CARTESIAN_POINT('Ctrl Pts',(7.39133288143138,-3.37491133293512,
34.4445660701108));
#165777=CARTESIAN_POINT('Ctrl Pts',(7.42602012554167,-3.297784043843,34.447871342758));
#165778=CARTESIAN_POINT('Ctrl Pts',(7.44148260983002,-3.26274287353098,
34.4493705108081));
#165779=CARTESIAN_POINT('Ctrl Pts',(7.47061059140215,-3.19544861651566,
34.4522451476228));
#165780=CARTESIAN_POINT('Ctrl Pts',(7.4843164217422,-3.1632138969406,34.4536202078877));
#165781=CARTESIAN_POINT('Ctrl Pts',(7.51264123705642,-3.09538204469376,
34.4565100247779));
#165782=CARTESIAN_POINT('Ctrl Pts',(7.52721663338313,-3.05976765445253,
34.4580251494618));
#165783=CARTESIAN_POINT('Ctrl Pts',(7.5611756689012,-2.97507881858999,34.4616233450183));
#165784=CARTESIAN_POINT('Ctrl Pts',(7.5803353415005,-2.92591653101328,34.4637084196999));
#165785=CARTESIAN_POINT('Ctrl Pts',(7.72816897301282,-2.53538564026938,
34.4802453549446));
#165786=CARTESIAN_POINT('Ctrl Pts',(7.83419583355483,-2.1858960060258,34.4949002505393));
#165787=CARTESIAN_POINT('Ctrl Pts',(7.94489085578469,-1.70716576582002,
34.5148131290753));
#165788=CARTESIAN_POINT('Ctrl Pts',(7.97051813427188,-1.58320756061054,
34.5199534865266));
#165789=CARTESIAN_POINT('Ctrl Pts',(8.0247580622937,-1.28598935142951,34.5322320223368));
#165790=CARTESIAN_POINT('Ctrl Pts',(8.05067070629606,-1.11230033672865,
34.5393702383502));
#165791=CARTESIAN_POINT('Ctrl Pts',(8.0985327887415,-0.700435079277564,
34.5561678856575));
#165792=CARTESIAN_POINT('Ctrl Pts',(8.11563527375969,-0.461855511904104,
34.5657978978396));
#165793=CARTESIAN_POINT('Ctrl Pts',(8.1232414279722,-0.184654997437717,
34.5767943916186));
#165794=CARTESIAN_POINT('Ctrl Pts',(8.12402025543175,-0.146436607375029,
34.578306231622));
#165795=CARTESIAN_POINT('Ctrl Pts',(8.12479443884352,-0.0883121798156752,
34.5805985308869));
#165796=CARTESIAN_POINT('Ctrl Pts',(8.1249863921664,-0.0684094129417031,
34.5813822011467));
#165797=CARTESIAN_POINT('Ctrl Pts',(8.1251678565596,-0.0380128451970877,
34.5825771148768));
#165798=CARTESIAN_POINT('Ctrl Pts',(8.12521017267968,-0.0275195204497364,
34.5829892674196));
#165799=CARTESIAN_POINT('Ctrl Pts',(8.12524185021272,-0.0124023265984525,
34.5835825578118));
#165800=CARTESIAN_POINT('Ctrl Pts',(8.12524759234424,-0.00777851420400875,
34.5837639600232));
#165801=CARTESIAN_POINT('Ctrl Pts',(8.12524938758068,-0.00315469804944397,
34.5839452996515));
#165802=CARTESIAN_POINT('',(8.12524999535401,0.000274771867430455,38.5832974955445));
#165803=CARTESIAN_POINT('Ctrl Pts',(8.12524938756529,-0.00315473768782347,
34.5839452980969));
#165804=CARTESIAN_POINT('Ctrl Pts',(8.12525212190974,0.00388775925662743,
34.584221495017));
#165805=CARTESIAN_POINT('Ctrl Pts',(8.12524570021172,0.0109302651159309,
34.5844975467655));
#165806=CARTESIAN_POINT('Ctrl Pts',(8.1251952209293,0.0337512308952398,
34.5853916272751));
#165807=CARTESIAN_POINT('Ctrl Pts',(8.12511435888944,0.0495295917114283,
34.5860090885223));
#165808=CARTESIAN_POINT('Ctrl Pts',(8.12469453002567,0.101760909957368,
34.5880509431436));
#165809=CARTESIAN_POINT('Ctrl Pts',(8.12415620062433,0.138211921603296,
34.5894724639253));
#165810=CARTESIAN_POINT('Ctrl Pts',(8.11865004461308,0.394303865798785,
34.5994403309321));
#165811=CARTESIAN_POINT('Ctrl Pts',(8.10502098785227,0.613670069212227,
34.6078825785361));
#165812=CARTESIAN_POINT('Ctrl Pts',(8.05651078099494,1.08480344278174,34.6260885981769));
#165813=CARTESIAN_POINT('Ctrl Pts',(8.01867720209948,1.33603107781036,34.6358452139881));
#165814=CARTESIAN_POINT('Ctrl Pts',(7.96013183450352,1.63037486290319,34.6474878045885));
#165815=CARTESIAN_POINT('Ctrl Pts',(7.95073512257806,1.67559899932941,34.6492823782081));
#165816=CARTESIAN_POINT('Ctrl Pts',(7.93358549751132,1.75474188970223,34.6524338953235));
#165817=CARTESIAN_POINT('Ctrl Pts',(7.92599936934352,1.78869559559917,34.6537895123514));
#165818=CARTESIAN_POINT('Ctrl Pts',(7.91063343276423,1.85545216549814,34.6564621699032));
#165819=CARTESIAN_POINT('Ctrl Pts',(7.90286707186119,1.88825741937345,34.657779077092));
#165820=CARTESIAN_POINT('Ctrl Pts',(7.8869890112249,1.95351238051163,34.6604059132159));
#165821=CARTESIAN_POINT('Ctrl Pts',(7.87888064952394,1.98596223174793,34.6617157906311));
#165822=CARTESIAN_POINT('Ctrl Pts',(7.85646476118541,2.07337269222533,34.6652542648441));
#165823=CARTESIAN_POINT('Ctrl Pts',(7.84178102714466,2.12823474854227,34.6674859057408));
#165824=CARTESIAN_POINT('Ctrl Pts',(7.77536165569618,2.36636919079482,34.6772211395378));
#165825=CARTESIAN_POINT('Ctrl Pts',(7.71776763344515,2.547942978051,34.684771890944));
#165826=CARTESIAN_POINT('Ctrl Pts',(7.58580755604703,2.91827028414676,34.7004316959874));
#165827=CARTESIAN_POINT('Ctrl Pts',(7.51064521760747,3.10660356839709,34.7085401809579));
#165828=CARTESIAN_POINT('Ctrl Pts',(7.38332260460776,3.3939180336083,34.7210816270863));
#165829=CARTESIAN_POINT('Ctrl Pts',(7.33603007462666,3.4949671364998,34.7255259358814));
#165830=CARTESIAN_POINT('Ctrl Pts',(7.2660361428698,3.63683675352567,34.7317991828828));
#165831=CARTESIAN_POINT('Ctrl Pts',(7.24504073060462,3.67848442223049,34.7336449231816));
#165832=CARTESIAN_POINT('Ctrl Pts',(7.21161330937314,3.7433963997994,34.7365268329542));
#165833=CARTESIAN_POINT('Ctrl Pts',(7.19942466904675,3.76678477904054,34.7375662649226));
#165834=CARTESIAN_POINT('Ctrl Pts',(7.17838778414793,3.80667663643544,34.7393406626569));
#165835=CARTESIAN_POINT('Ctrl Pts',(7.16959597268729,3.82320961842986,34.7400764988261));
#165836=CARTESIAN_POINT('Ctrl Pts',(7.15175952202237,3.85647313089009,34.741557745098));
#165837=CARTESIAN_POINT('Ctrl Pts',(7.14271314518782,3.87320257649082,34.7423031317843));
#165838=CARTESIAN_POINT('Ctrl Pts',(7.1229826065227,3.90938600675234,34.7439163723241));
#165839=CARTESIAN_POINT('Ctrl Pts',(7.11227729782873,3.92882829933022,34.744783884676));
#165840=CARTESIAN_POINT('Ctrl Pts',(7.08316312212893,3.98119462059008,34.7471226379167));
#165841=CARTESIAN_POINT('Ctrl Pts',(7.06460438922882,4.01403478607073,34.7485916595854));
#165842=CARTESIAN_POINT('Ctrl Pts',(6.96495715168983,4.18753134282294,34.7563682696062));
#165843=CARTESIAN_POINT('Ctrl Pts',(6.87989440218827,4.32586417139037,34.7626242877761));
#165844=CARTESIAN_POINT('Ctrl Pts',(6.60405022690194,4.74571475518898,34.7819250060177));
#165845=CARTESIAN_POINT('Ctrl Pts',(6.39970527204536,5.01787408418438,34.7949003377759));
#165846=CARTESIAN_POINT('Ctrl Pts',(6.06993991454218,5.40404266739938,34.814472740586));
#165847=CARTESIAN_POINT('Ctrl Pts',(5.95704000488348,5.52824758463407,34.8209647054593));
#165848=CARTESIAN_POINT('Ctrl Pts',(5.8338976671695,5.65556472922741,34.8278527360451));
#165849=CARTESIAN_POINT('Ctrl Pts',(5.82740768923605,5.66225167409398,34.8282152080505));
#165850=CARTESIAN_POINT('Ctrl Pts',(5.81727192675331,5.67265916714917,34.8287804510937));
#165851=CARTESIAN_POINT('Ctrl Pts',(5.81363404175725,5.6763874008854,34.8289831557022));
#165852=CARTESIAN_POINT('Ctrl Pts',(5.80802481337773,5.68212488889154,34.8292954433741));
#165853=CARTESIAN_POINT('Ctrl Pts',(5.80605600631053,5.68413662198172,34.8294050051147));
#165854=CARTESIAN_POINT('Ctrl Pts',(5.80304106807818,5.68721409434241,34.8295727072432));
#165855=CARTESIAN_POINT('Ctrl Pts',(5.80199568765323,5.68828056912998,34.8296308413213));
#165856=CARTESIAN_POINT('Ctrl Pts',(5.796363663638,5.69402307194969,34.8299439659951));
#165857=CARTESIAN_POINT('Ctrl Pts',(5.79177166233974,5.69869383949588,34.8301990015068));
#165858=CARTESIAN_POINT('Ctrl Pts',(5.78354494819218,5.70704145113668,34.8306554299977));
#165859=CARTESIAN_POINT('Ctrl Pts',(5.77991236381637,5.71072038882402,34.8308568049596));
#165860=CARTESIAN_POINT('Ctrl Pts',(5.77344282400862,5.71725998639819,34.8312151551819));
#165861=CARTESIAN_POINT('Ctrl Pts',(5.77060724731175,5.72012200843901,34.8313721187841));
#165862=CARTESIAN_POINT('Ctrl Pts',(5.76558130167161,5.72518728674974,34.8316501536577));
#165863=CARTESIAN_POINT('Ctrl Pts',(5.76339179533751,5.72739139818271,34.8317712176427));
#165864=CARTESIAN_POINT('Ctrl Pts',(5.75952578721011,5.73127873278362,34.8319848756536));
#165865=CARTESIAN_POINT('Ctrl Pts',(5.75784981021638,5.7329624775839,34.8320774652504));
#165866=CARTESIAN_POINT('Ctrl Pts',(5.75489941426114,5.73592394919647,34.8322403995011));
#165867=CARTESIAN_POINT('Ctrl Pts',(5.75362530754072,5.73720198700158,34.8323107415223));
#165868=CARTESIAN_POINT('Ctrl Pts',(5.75138758764029,5.73944511596621,34.8324342485982));
#165869=CARTESIAN_POINT('Ctrl Pts',(5.75042415702783,5.74041038922492,34.8324874121141));
#165870=CARTESIAN_POINT('Ctrl Pts',(5.74873510732527,5.74210181746458,34.8325805964454));
#165871=CARTESIAN_POINT('Ctrl Pts',(5.74800959353507,5.74282807760712,34.8326206163738));
#165872=CARTESIAN_POINT('Ctrl Pts',(5.74510652671018,5.74573302962187,34.8327807261616));
#165873=CARTESIAN_POINT('Ctrl Pts',(5.7429278727156,5.74791062036725,34.8329008252742));
#165874=CARTESIAN_POINT('Ctrl Pts',(5.70452897669493,5.78624715090123,34.8350165605289));
#165875=CARTESIAN_POINT('Ctrl Pts',(5.66796920996702,5.82206423440826,34.8370150224519));
#165876=CARTESIAN_POINT('Ctrl Pts',(5.59210909301375,5.89499150056361,34.8411297617647));
#165877=CARTESIAN_POINT('Ctrl Pts',(5.55277190915635,5.93205976030752,34.8432462605495));
#165878=CARTESIAN_POINT('Ctrl Pts',(5.46398479265107,6.01406869368731,34.8479856115783));
#165879=CARTESIAN_POINT('Ctrl Pts',(5.414344451711,6.05879742059624,34.850609800139));
#165880=CARTESIAN_POINT('Ctrl Pts',(5.25207208880888,6.20142688986855,34.8591065291));
#165881=CARTESIAN_POINT('Ctrl Pts',(5.13729352249396,6.29683822921074,34.8649923382592));
#165882=CARTESIAN_POINT('Ctrl Pts',(4.92210510023832,6.46591476967828,34.8757956607437));
#165883=CARTESIAN_POINT('Ctrl Pts',(4.82250374100534,6.54053745106074,34.8807100605435));
#165884=CARTESIAN_POINT('Ctrl Pts',(4.65930643014928,6.65705188715999,34.8886154910679));
#165885=CARTESIAN_POINT('Ctrl Pts',(4.5967669250635,6.70038880480338,34.8916113962469));
#165886=CARTESIAN_POINT('Ctrl Pts',(4.50236519510259,6.76386090929375,34.8960807802276));
#165887=CARTESIAN_POINT('Ctrl Pts',(4.4709566407817,6.78466310754317,34.8975591725953));
#165888=CARTESIAN_POINT('Ctrl Pts',(4.40468152525041,6.82789769957922,34.9006602946229));
#165889=CARTESIAN_POINT('Ctrl Pts',(4.36978567694507,6.85028316828618,34.9022826918794));
#165890=CARTESIAN_POINT('Ctrl Pts',(4.31827577954882,6.88277268586828,34.9046633429927));
#165891=CARTESIAN_POINT('Ctrl Pts',(4.30179440232076,6.89308570052938,34.9054229561689));
#165892=CARTESIAN_POINT('Ctrl Pts',(4.19818723961457,6.95740026974355,34.9101853649551));
#165893=CARTESIAN_POINT('Ctrl Pts',(4.11008291273003,7.00980835385641,34.9141788531029));
#165894=CARTESIAN_POINT('Ctrl Pts',(3.848984644853,7.15850513001163,34.9258795982784));
#165895=CARTESIAN_POINT('Ctrl Pts',(3.67343620960111,7.25015480069218,34.9335791681863));
#165896=CARTESIAN_POINT('Ctrl Pts',(3.44347555253292,7.35971366841279,34.943527121756));
#165897=CARTESIAN_POINT('Ctrl Pts',(3.39198032275537,7.38358846561801,34.9457459744189));
#165898=CARTESIAN_POINT('Ctrl Pts',(3.29157894963733,7.42886565662324,34.9500571029993));
#165899=CARTESIAN_POINT('Ctrl Pts',(3.24270366710774,7.45032951158792,34.952148942539));
#165900=CARTESIAN_POINT('Ctrl Pts',(3.13897147623036,7.49466996164132,34.9565758312534));
#165901=CARTESIAN_POINT('Ctrl Pts',(3.08406789967719,7.51742940899239,34.9589114295993));
#165902=CARTESIAN_POINT('Ctrl Pts',(2.9353718012212,7.57716593019159,34.965219145366));
#165903=CARTESIAN_POINT('Ctrl Pts',(2.84113297527614,7.6130029810279,34.9691979268653));
#165904=CARTESIAN_POINT('Ctrl Pts',(2.29066579744459,7.81068919112221,34.9923468109638));
#165905=CARTESIAN_POINT('Ctrl Pts',(1.82137143975115,7.93325972300021,35.011781675766));
#165906=CARTESIAN_POINT('Ctrl Pts',(1.24493358579442,8.02993857246595,35.0351051038665));
#165907=CARTESIAN_POINT('Ctrl Pts',(1.14559010426156,8.04471234011166,35.0391028100846));
#165908=CARTESIAN_POINT('Ctrl Pts',(1.00046783942304,8.06355130087438,35.0449030369057));
#165909=CARTESIAN_POINT('Ctrl Pts',(0.954888367142722,8.0690757658899,35.0467190574877));
#165910=CARTESIAN_POINT('Ctrl Pts',(0.882052499240776,8.07727805808648,
35.0496110110271));
#165911=CARTESIAN_POINT('Ctrl Pts',(0.85482524299561,8.08020490151107,35.0506898347288));
#165912=CARTESIAN_POINT('Ctrl Pts',(0.807510189156024,8.08504929017713,
35.0525604766157));
#165913=CARTESIAN_POINT('Ctrl Pts',(0.787429105458315,8.08702974752103,
35.0533531125639));
#165914=CARTESIAN_POINT('Ctrl Pts',(0.748503174202609,8.09072237879436,
35.0548869848895));
#165915=CARTESIAN_POINT('Ctrl Pts',(0.729659311744389,8.09244356817922,
35.0556283444389));
#165916=CARTESIAN_POINT('Ctrl Pts',(0.692475101540281,8.09570902030665,
35.0570888304099));
#165917=CARTESIAN_POINT('Ctrl Pts',(0.674135181562731,8.09725682370546,
35.0578079980902));
#165918=CARTESIAN_POINT('Ctrl Pts',(0.621677422069094,8.10150455462117,
35.059861640936));
#165919=CARTESIAN_POINT('Ctrl Pts',(0.587547533193598,8.10405125714766,
35.0611937413131));
#165920=CARTESIAN_POINT('Ctrl Pts',(0.342648571307864,8.12076989723983,
35.0707275147846));
#165921=CARTESIAN_POINT('Ctrl Pts',(0.131411071492284,8.12693331272511,
35.0788222704203));
#165922=CARTESIAN_POINT('Ctrl Pts',(-0.259227200681319,8.12309521647083,
35.0937759633845));
#165923=CARTESIAN_POINT('Ctrl Pts',(-0.438518066267162,8.11539132358751,
35.1006326683191));
#165924=CARTESIAN_POINT('Ctrl Pts',(-0.731067458314353,8.09309717001299,
35.1118981749349));
#165925=CARTESIAN_POINT('Ctrl Pts',(-0.844533070922323,8.08204460959697,
35.1162862962646));
#165926=CARTESIAN_POINT('Ctrl Pts',(-1.04139663533081,8.05867729114972,
35.1239494405474));
#165927=CARTESIAN_POINT('Ctrl Pts',(-1.12490531834648,8.04744521742355,
35.1272157068452));
#165928=CARTESIAN_POINT('Ctrl Pts',(-1.24261299023128,8.02974531823331,
35.1318456219096));
#165929=CARTESIAN_POINT('Ctrl Pts',(-1.27696854548493,8.02435344704153,
35.1332000978312));
#165930=CARTESIAN_POINT('Ctrl Pts',(-1.34431242333893,8.0133408403655,35.1358615916867));
#165931=CARTESIAN_POINT('Ctrl Pts',(-1.3773027463569,8.00773653732853,35.137168444919));
#165932=CARTESIAN_POINT('Ctrl Pts',(-1.44303308442542,7.99615224273553,
35.1397785260649));
#165933=CARTESIAN_POINT('Ctrl Pts',(-1.47577286123667,7.99017456786248,
35.1410817102892));
#165934=CARTESIAN_POINT('Ctrl Pts',(-1.56338967279644,7.97362048088784,
35.1445778271022));
#165935=CARTESIAN_POINT('Ctrl Pts',(-1.61819572774218,7.96267878216658,
35.1467737794527));
#165936=CARTESIAN_POINT('Ctrl Pts',(-1.86061339478575,7.9116753963471,35.1565281319363));
#165937=CARTESIAN_POINT('Ctrl Pts',(-2.04688286352506,7.86554251038108,
35.1641351280624));
#165938=CARTESIAN_POINT('Ctrl Pts',(-2.44366439053522,7.75222222016196,
35.1805634253704));
#165939=CARTESIAN_POINT('Ctrl Pts',(-2.65342534770506,7.68295378145173,
35.189388727527));
#165940=CARTESIAN_POINT('Ctrl Pts',(-2.91965137689471,7.58283395539435,
35.2006991382305));
#165941=CARTESIAN_POINT('Ctrl Pts',(-2.97893399856467,7.55974121557897,
35.2032245785618));
#165942=CARTESIAN_POINT('Ctrl Pts',(-3.08066115270987,7.51873235129915,
35.2075664676156));
#165943=CARTESIAN_POINT('Ctrl Pts',(-3.12323576093065,7.50114709367621,
35.2093861572494));
#165944=CARTESIAN_POINT('Ctrl Pts',(-3.18298432258327,7.47587133799463,
35.2119422126967));
#165945=CARTESIAN_POINT('Ctrl Pts',(-3.20028449363887,7.46848181509135,
35.2126825935082));
#165946=CARTESIAN_POINT('Ctrl Pts',(-3.23406452424598,7.45391422800095,
35.21412866372));
#165947=CARTESIAN_POINT('Ctrl Pts',(-3.25054653852426,7.44674142619944,
35.2148344268593));
#165948=CARTESIAN_POINT('Ctrl Pts',(-3.28529311071579,7.43148273953059,
35.2163225694715));
#165949=CARTESIAN_POINT('Ctrl Pts',(-3.30355185747248,7.42338411092282,
35.2171047081253));
#165950=CARTESIAN_POINT('Ctrl Pts',(-3.35364376234865,7.40094453927139,
35.2192509636639));
#165951=CARTESIAN_POINT('Ctrl Pts',(-3.38541466303249,7.38646560506674,
35.2206128242698));
#165952=CARTESIAN_POINT('Ctrl Pts',(-3.56283426038929,7.30422511698172,
35.2282236052211));
#165953=CARTESIAN_POINT('Ctrl Pts',(-3.70654347269636,7.23235986783352,
35.2344100843979));
#165954=CARTESIAN_POINT('Ctrl Pts',(-4.16341040741607,6.98669632923451,
35.2542758829501));
#165955=CARTESIAN_POINT('Ctrl Pts',(-4.4672382165251,6.7964474479209,35.2678054737171));
#165956=CARTESIAN_POINT('Ctrl Pts',(-4.96904173892923,6.43400275186682,
35.2913490098663));
#165957=CARTESIAN_POINT('Ctrl Pts',(-5.17307479709484,6.27112924474943,
35.3013049557861));
#165958=CARTESIAN_POINT('Ctrl Pts',(-5.45074493110372,6.0266867036711,35.3155509933524));
#165959=CARTESIAN_POINT('Ctrl Pts',(-5.53111559373208,5.95301041182328,
35.3197633498159));
#165960=CARTESIAN_POINT('Ctrl Pts',(-5.67071636512488,5.81976916067414,
35.3272484262055));
#165961=CARTESIAN_POINT('Ctrl Pts',(-5.73055130712703,5.76086094021573,
35.3305141097278));
#165962=CARTESIAN_POINT('Ctrl Pts',(-5.81546198121001,5.67463325786226,
35.3352347097355));
#165963=CARTESIAN_POINT('Ctrl Pts',(-5.84128073350422,5.64805276606012,
35.3366819435522));
#165964=CARTESIAN_POINT('Ctrl Pts',(-5.8931978231614,5.59386718218471,35.339616446664));
#165965=CARTESIAN_POINT('Ctrl Pts',(-5.91928620629358,5.56625380592011,
35.3411037708838));
#165966=CARTESIAN_POINT('Ctrl Pts',(-5.96965688710703,5.5121841115854,35.3440005876965));
#165967=CARTESIAN_POINT('Ctrl Pts',(-5.99395934970122,5.48574774620612,
35.345409854201));
#165968=CARTESIAN_POINT('Ctrl Pts',(-6.05902495780542,5.41402040377905,
35.3492146848566));
#165969=CARTESIAN_POINT('Ctrl Pts',(-6.09945511412735,5.36843064978203,
35.3516130813039));
#165970=CARTESIAN_POINT('Ctrl Pts',(-6.25689812573659,5.18682040243138,
35.3610902014444));
#165971=CARTESIAN_POINT('Ctrl Pts',(-6.36990444139595,5.04739501328758,
35.3681977333362));
#165972=CARTESIAN_POINT('Ctrl Pts',(-6.90784827420129,4.336819335229,35.4036217736309));
#165973=CARTESIAN_POINT('Ctrl Pts',(-7.26103288330256,3.71532824108283,
35.432735717903));
#165974=CARTESIAN_POINT('Ctrl Pts',(-7.67635558963884,2.69209288273319,
35.4794316237433));
#165975=CARTESIAN_POINT('Ctrl Pts',(-7.79744362954527,2.318119578179,35.4961603448697));
#165976=CARTESIAN_POINT('Ctrl Pts',(-7.9194696069256,1.82096898233787,35.5171791218376));
#165977=CARTESIAN_POINT('Ctrl Pts',(-7.94535898206296,1.70446442989422,
35.5220164216116));
#165978=CARTESIAN_POINT('Ctrl Pts',(-7.97281025926088,1.56666285180608,
35.5276040582959));
#165979=CARTESIAN_POINT('Ctrl Pts',(-7.97686594816583,1.54588019473454,
35.5284431881772));
#165980=CARTESIAN_POINT('Ctrl Pts',(-7.98268411838763,1.51543337700562,
35.5296670655407));
#165981=CARTESIAN_POINT('Ctrl Pts',(-7.98451037152187,1.50578158515982,
35.530054239054));
#165982=CARTESIAN_POINT('Ctrl Pts',(-7.98766180079866,1.48895926415792,
35.5307276284014));
#165983=CARTESIAN_POINT('Ctrl Pts',(-7.98899483361551,1.48179022914358,
35.5310141512046));
#165984=CARTESIAN_POINT('Ctrl Pts',(-7.99154781872775,1.46795671825823,
35.531566150358));
#165985=CARTESIAN_POINT('Ctrl Pts',(-7.99276908912684,1.46129249430836,
35.531831679063));
#165986=CARTESIAN_POINT('Ctrl Pts',(-7.99563939702669,1.4455185578327,35.5324592293984));
#165987=CARTESIAN_POINT('Ctrl Pts',(-7.99728120582328,1.43640752721332,
35.5328209573329));
#165988=CARTESIAN_POINT('Ctrl Pts',(-8.00211839470062,1.40929872228121,
35.5338949797603));
#165989=CARTESIAN_POINT('Ctrl Pts',(-8.00526862993003,1.39129287406691,
35.5346053958517));
#165990=CARTESIAN_POINT('Ctrl Pts',(-8.04467637079795,1.16148386495849,
35.5436334077829));
#165991=CARTESIAN_POINT('Ctrl Pts',(-8.07257791224346,0.948339309571144,
35.5515446086187));
#165992=CARTESIAN_POINT('Ctrl Pts',(-8.10178077860499,0.62653955769214,
35.5630344761891));
#165993=CARTESIAN_POINT('Ctrl Pts',(-8.10940843079419,0.518555089387819,
35.5668155815941));
#165994=CARTESIAN_POINT('Ctrl Pts',(-8.1471196490731,-0.227023988679579,
35.5925653863522));
#165995=CARTESIAN_POINT('Ctrl Pts',(-8.10413803092976,-0.866079136845537,
35.6129862188969));
#165996=CARTESIAN_POINT('Ctrl Pts',(-7.91392581108344,-1.88326007959288,
35.6489069896832));
#165997=CARTESIAN_POINT('Ctrl Pts',(-7.81262480900694,-2.26710020180854,
35.6632585365121));
#165998=CARTESIAN_POINT('Ctrl Pts',(-7.67434427473708,-2.66926186990742,
35.6796358574786));
#165999=CARTESIAN_POINT('Ctrl Pts',(-7.66482354556395,-2.69647899535085,
35.6807508148663));
#166000=CARTESIAN_POINT('Ctrl Pts',(-7.65079400609647,-2.7359108434309,
35.6823758535913));
#166001=CARTESIAN_POINT('Ctrl Pts',(-7.64640034701529,-2.74816644295808,
35.6828822881947));
#166002=CARTESIAN_POINT('Ctrl Pts',(-7.63866887894711,-2.76957039139912,
35.6837691576179));
#166003=CARTESIAN_POINT('Ctrl Pts',(-7.6353440387107,-2.77872341279585,
35.684149180601));
#166004=CARTESIAN_POINT('Ctrl Pts',(-7.6288791277273,-2.79642158778652,
35.6848854824854));
#166005=CARTESIAN_POINT('Ctrl Pts',(-7.62574113347528,-2.8049674876381,
35.6852416950567));
#166006=CARTESIAN_POINT('Ctrl Pts',(-7.61825147280863,-2.8252590957727,
35.6860891056933));
#166007=CARTESIAN_POINT('Ctrl Pts',(-7.61388700095014,-2.83700003458964,
35.6865807102438));
#166008=CARTESIAN_POINT('Ctrl Pts',(-7.59836983315337,-2.87844930631459,
35.6883207894881));
#166009=CARTESIAN_POINT('Ctrl Pts',(-7.58707033537717,-2.90810216953385,
35.6895739317359));
#166010=CARTESIAN_POINT('Ctrl Pts',(-7.41613012697682,-3.34891626200274,
35.7083277013317));
#166011=CARTESIAN_POINT('Ctrl Pts',(-7.22346226096286,-3.74643122317459,
35.726915754654));
#166012=CARTESIAN_POINT('Ctrl Pts',(-6.73867952448173,-4.56877307563761,
35.7687588665495));
#166013=CARTESIAN_POINT('Ctrl Pts',(-6.43648092504908,-4.98549581195371,
35.7921975420767));
#166014=CARTESIAN_POINT('Ctrl Pts',(-5.98219779545448,-5.50119615750303,
35.8226319921396));
#166015=CARTESIAN_POINT('Ctrl Pts',(-5.86324575088658,-5.62780623019203,
35.8302275616457));
#166016=CARTESIAN_POINT('Ctrl Pts',(-5.63344940755418,-5.85719550351363,
35.8440914417724));
#166017=CARTESIAN_POINT('Ctrl Pts',(-5.52361418973488,-5.96088786656312,
35.850400467349));
#166018=CARTESIAN_POINT('Ctrl Pts',(-5.37596919377233,-6.09268749216142,
35.8584105855136));
#166019=CARTESIAN_POINT('Ctrl Pts',(-5.34072363013724,-6.12360652624086,
35.8602896121216));
#166020=CARTESIAN_POINT('Ctrl Pts',(-5.29495134522953,-6.1630642807339,
35.862690076382));
#166021=CARTESIAN_POINT('Ctrl Pts',(-5.2846686365472,-6.17188370610218,
35.8632267822232));
#166022=CARTESIAN_POINT('Ctrl Pts',(-5.26804176133746,-6.18607247283605,
35.8640905835701));
#166023=CARTESIAN_POINT('Ctrl Pts',(-5.26171135487337,-6.19145784585777,
35.8644185215657));
#166024=CARTESIAN_POINT('Ctrl Pts',(-5.24962331142428,-6.20170939985228,
35.8650429569472));
#166025=CARTESIAN_POINT('Ctrl Pts',(-5.24386714617091,-6.20657729717903,
35.8653395425626));
#166026=CARTESIAN_POINT('Ctrl Pts',(-5.23070627584658,-6.21767585747659,
35.866015934899));
#166027=CARTESIAN_POINT('Ctrl Pts',(-5.22329718981457,-6.22390132318167,
35.8663954794687));
#166028=CARTESIAN_POINT('Ctrl Pts',(-5.20399979876033,-6.24005717923453,
35.8673808519901));
#166029=CARTESIAN_POINT('Ctrl Pts',(-5.19209415770805,-6.24996686127758,
35.8679856620792));
#166030=CARTESIAN_POINT('Ctrl Pts',(-5.11655979007391,-6.31247324647411,
35.8718035711892));
#166031=CARTESIAN_POINT('Ctrl Pts',(-5.05215970817499,-6.36413272795087,
35.8749725129444));
#166032=CARTESIAN_POINT('Ctrl Pts',(-4.88750382144314,-6.49213915936372,
35.8828862778145));
#166033=CARTESIAN_POINT('Ctrl Pts',(-4.78623752821311,-6.56715281767075,
35.8875818171872));
#166034=CARTESIAN_POINT('Ctrl Pts',(-4.47754523141419,-6.78488405822624,
35.9014952066341));
#166035=CARTESIAN_POINT('Ctrl Pts',(-4.26518816792894,-6.92034954297207,
35.9105465344359));
#166036=CARTESIAN_POINT('Ctrl Pts',(-3.65242796048224,-7.27230239167732,
35.9359197842129));
#166037=CARTESIAN_POINT('Ctrl Pts',(-3.23965726544051,-7.46533464582141,
35.9522163590045));
#166038=CARTESIAN_POINT('Ctrl Pts',(-2.58638533019122,-7.70639983955096,
35.9781460471032));
#166039=CARTESIAN_POINT('Ctrl Pts',(-2.35625562275052,-7.77984840295317,
35.987292088998));
#166040=CARTESIAN_POINT('Ctrl Pts',(-2.07876945527919,-7.85496811652075,
35.9983777145646));
#166041=CARTESIAN_POINT('Ctrl Pts',(-2.03423507736334,-7.86661897962906,
36.0001584172041));
#166042=CARTESIAN_POINT('Ctrl Pts',(-1.96474679361952,-7.88416862499366,
36.0029392848707));
#166043=CARTESIAN_POINT('Ctrl Pts',(-1.93985977139226,-7.89032882275543,
36.0039357171235));
#166044=CARTESIAN_POINT('Ctrl Pts',(-1.89380678936169,-7.90149710292535,
36.0057804455528));
#166045=CARTESIAN_POINT('Ctrl Pts',(-1.87264902883714,-7.90653819529095,
36.006628275466));
#166046=CARTESIAN_POINT('Ctrl Pts',(-1.82752784230803,-7.91709758922762,
36.0084370928113));
#166047=CARTESIAN_POINT('Ctrl Pts',(-1.80355907149269,-7.92259218448324,
36.0093984051002));
#166048=CARTESIAN_POINT('Ctrl Pts',(-1.73937356810138,-7.93699968252074,
36.0119741616048));
#166049=CARTESIAN_POINT('Ctrl Pts',(-1.69911350196255,-7.94571567881999,
36.0135913438358));
#166050=CARTESIAN_POINT('Ctrl Pts',(-1.51783624683178,-7.98352005384629,
36.0208818460534));
#166051=CARTESIAN_POINT('Ctrl Pts',(-1.37612954105435,-8.00916259505948,
36.026605645455));
#166052=CARTESIAN_POINT('Ctrl Pts',(-1.06649678523281,-8.05673193915344,
36.0391945575339));
#166053=CARTESIAN_POINT('Ctrl Pts',(-0.898416280861058,-8.07720191991345,
36.0460807236975));
#166054=CARTESIAN_POINT('Ctrl Pts',(-0.191505968885995,-8.140955380252,
36.0752914460687));
#166055=CARTESIAN_POINT('Ctrl Pts',(0.350298812512999,-8.13566648358123,
36.0984028383942));
#166056=CARTESIAN_POINT('Ctrl Pts',(1.10364705433365,-8.05288308602651,
36.1303954368781));
#166057=CARTESIAN_POINT('Ctrl Pts',(1.31874068321201,-8.02046699754834,
36.1394950996924));
#166058=CARTESIAN_POINT('Ctrl Pts',(1.62541922591264,-7.96157615004829,
36.1522445953865));
#166059=CARTESIAN_POINT('Ctrl Pts',(1.71824071320448,-7.94206094609121,
36.1560730096295));
#166060=CARTESIAN_POINT('Ctrl Pts',(1.8272195016843,-7.91714870215879,36.1605176585653));
#166061=CARTESIAN_POINT('Ctrl Pts',(1.84372614491277,-7.91332095817349,
36.1611895076565));
#166062=CARTESIAN_POINT('Ctrl Pts',(1.86903940233612,-7.90736753572726,
36.1622175919455));
#166063=CARTESIAN_POINT('Ctrl Pts',(1.87785458652531,-7.90527872913061,
36.1625752040756));
#166064=CARTESIAN_POINT('Ctrl Pts',(1.89323778996243,-7.9016064112902,36.1631985272878));
#166065=CARTESIAN_POINT('Ctrl Pts',(1.89980735279523,-7.90002944493805,
36.1634644887706));
#166066=CARTESIAN_POINT('Ctrl Pts',(1.91355705725721,-7.89671080505675,
36.1640206276264));
#166067=CARTESIAN_POINT('Ctrl Pts',(1.92073680764272,-7.89496752787937,
36.1643107421241));
#166068=CARTESIAN_POINT('Ctrl Pts',(1.94064265913624,-7.89010553234284,
36.1651142704634));
#166069=CARTESIAN_POINT('Ctrl Pts',(1.95336364227486,-7.88696581237407,
36.1656268480819));
#166070=CARTESIAN_POINT('Ctrl Pts',(2.00360632379976,-7.87443618957103,
36.1676475340369));
#166071=CARTESIAN_POINT('Ctrl Pts',(2.04106876044858,-7.86480908787035,
36.1691458661266));
#166072=CARTESIAN_POINT('Ctrl Pts',(2.08149656914881,-7.85411162717253,
36.1707527829844));
#166073=CARTESIAN_POINT('Ctrl Pts',(2.08453123079472,-7.85330675367765,
36.1708733429704));
#166074=CARTESIAN_POINT('Ctrl Pts',(2.87584152954999,-7.64293910041931,
36.2022941622812));
#166075=CARTESIAN_POINT('Ctrl Pts',(3.62812932137937,-7.31586438032348,
36.2279383522161));
#166076=CARTESIAN_POINT('Ctrl Pts',(4.60642238122568,-6.70191151903222,
36.26757646638));
#166077=CARTESIAN_POINT('Ctrl Pts',(4.88214351938511,-6.50379882585563,
36.279539521296));
#166078=CARTESIAN_POINT('Ctrl Pts',(5.25764080508549,-6.19662851666698,
36.2975259157453));
#166079=CARTESIAN_POINT('Ctrl Pts',(5.36810105644125,-6.10118680156614,
36.3030447017041));
#166080=CARTESIAN_POINT('Ctrl Pts',(5.4927775842711,-5.98745372789434,36.3095616672778));
#166081=CARTESIAN_POINT('Ctrl Pts',(5.50956240914706,-5.97201220558443,
36.310445240007));
#166082=CARTESIAN_POINT('Ctrl Pts',(5.53495512813061,-5.94845351895876,
36.3117914821505));
#166083=CARTESIAN_POINT('Ctrl Pts',(5.54361073082386,-5.94038783256665,
36.312252071842));
#166084=CARTESIAN_POINT('Ctrl Pts',(5.55858098871185,-5.92637664832765,
36.313051639171));
#166085=CARTESIAN_POINT('Ctrl Pts',(5.56490380768753,-5.92043988201485,
36.3133902620669));
#166086=CARTESIAN_POINT('Ctrl Pts',(5.57898374680872,-5.90717713956545,
36.3141463794268));
#166087=CARTESIAN_POINT('Ctrl Pts',(5.58673596026024,-5.89984599075726,
36.3145640845531));
#166088=CARTESIAN_POINT('Ctrl Pts',(5.60715767521192,-5.88045714822414,
36.3156681539073));
#166089=CARTESIAN_POINT('Ctrl Pts',(5.61980269233511,-5.86837380893584,
36.3163555676741));
#166090=CARTESIAN_POINT('Ctrl Pts',(5.67204451425932,-5.81812880651341,
36.3192113352447));
#166091=CARTESIAN_POINT('Ctrl Pts',(5.71129195134477,-5.77960689692655,
36.3213945349094));
#166092=CARTESIAN_POINT('Ctrl Pts',(6.48430616026728,-5.0053195401276,36.3651606142523));
#166093=CARTESIAN_POINT('Ctrl Pts',(7.07052454473827,-4.13596002392158,
36.4137675947646));
#166094=CARTESIAN_POINT('Ctrl Pts',(7.57766521280065,-2.94359778476221,
36.4704911374173));
#166095=CARTESIAN_POINT('Ctrl Pts',(7.66700988559747,-2.70236214952331,
36.4814399135141));
#166096=CARTESIAN_POINT('Ctrl Pts',(7.75725705945687,-2.41792368580554,
36.4934676328857));
#166097=CARTESIAN_POINT('Ctrl Pts',(7.76944281194368,-2.37847651303313,
36.495116693381));
#166098=CARTESIAN_POINT('Ctrl Pts',(7.78494528881399,-2.32690188028682,
36.4972500385471));
#166099=CARTESIAN_POINT('Ctrl Pts',(7.7885351250395,-2.31485768867119,36.4977466286107));
#166100=CARTESIAN_POINT('Ctrl Pts',(7.79432461538074,-2.2952675509555,36.4985518002413));
#166101=CARTESIAN_POINT('Ctrl Pts',(7.79654128142491,-2.28772668560349,
36.4988611248705));
#166102=CARTESIAN_POINT('Ctrl Pts',(7.80077593196587,-2.27324321034897,
36.4994540805397));
#166103=CARTESIAN_POINT('Ctrl Pts',(7.80279559807271,-2.26630110296022,
36.4997377834086));
#166104=CARTESIAN_POINT('Ctrl Pts',(7.8073833280754,-2.25045307459042,36.5003843038641));
#166105=CARTESIAN_POINT('Ctrl Pts',(7.80994542686963,-2.24154542730656,
36.5007468704185));
#166106=CARTESIAN_POINT('Ctrl Pts',(7.81789537591416,-2.21372674655005,
36.5018766615201));
#166107=CARTESIAN_POINT('Ctrl Pts',(7.82322984629559,-2.19480044595643,
36.5026416946868));
#166108=CARTESIAN_POINT('Ctrl Pts',(7.86655399876549,-2.03892472935387,
36.5089140739986));
#166109=CARTESIAN_POINT('Ctrl Pts',(7.90101451164937,-1.90101500980129,
36.5142839923224));
#166110=CARTESIAN_POINT('Ctrl Pts',(8.06032380919927,-1.18397564052055,
36.5415801273203));
#166111=CARTESIAN_POINT('Ctrl Pts',(8.12518544520021,-0.593344303531527,
36.5621749605033));
#166112=CARTESIAN_POINT('Ctrl Pts',(8.12531225746491,0.571359736454304,
36.6045462755366));
#166113=CARTESIAN_POINT('Ctrl Pts',(8.06492182062517,1.14198041596768,36.6261305132673));
#166114=CARTESIAN_POINT('Ctrl Pts',(7.92025865124707,1.8174889000819,36.6528063994685));
#166115=CARTESIAN_POINT('Ctrl Pts',(7.89287697407166,1.93293965918776,36.6574045826282));
#166116=CARTESIAN_POINT('Ctrl Pts',(7.85110161518185,2.09334933695066,36.6638589267518));
#166117=CARTESIAN_POINT('Ctrl Pts',(7.83882943854375,2.1388457231402,36.6656969709959));
#166118=CARTESIAN_POINT('Ctrl Pts',(7.81580821771251,2.22133135432998,36.6690436398938));
#166119=CARTESIAN_POINT('Ctrl Pts',(7.80519056784129,2.25835587710605,36.6705510834822));
#166120=CARTESIAN_POINT('Ctrl Pts',(7.78322840666032,2.33293420659731,36.6735985615533));
#166121=CARTESIAN_POINT('Ctrl Pts',(7.77187437421485,2.37048415710379,36.6751386431613));
#166122=CARTESIAN_POINT('Ctrl Pts',(7.74317078963537,2.46298895615645,36.6789472006798));
#166123=CARTESIAN_POINT('Ctrl Pts',(7.72550770376431,2.51784414665875,36.6812184158831));
#166124=CARTESIAN_POINT('Ctrl Pts',(7.65531858192967,2.72813165306475,36.6899763545899));
#166125=CARTESIAN_POINT('Ctrl Pts',(7.59867342392271,2.88214608070219,36.6964994918006));
#166126=CARTESIAN_POINT('Ctrl Pts',(7.38594796939817,3.41056373907316,36.7192880564137));
#166127=CARTESIAN_POINT('Ctrl Pts',(7.20653660629888,3.77491625561562,36.7357458514446));
#166128=CARTESIAN_POINT('Ctrl Pts',(6.92217154077558,4.25759907073516,36.7585140857127));
#166129=CARTESIAN_POINT('Ctrl Pts',(6.83987535277774,4.38858908808458,36.7647962019272));
#166130=CARTESIAN_POINT('Ctrl Pts',(6.74099578967446,4.53643045926457,36.7719920884833));
#166131=CARTESIAN_POINT('Ctrl Pts',(6.72801852177775,4.55565498267227,36.7729298999151));
#166132=CARTESIAN_POINT('Ctrl Pts',(6.6069725036783,4.73332719802691,36.7816160983808));
#166133=CARTESIAN_POINT('Ctrl Pts',(6.49340597611092,4.88796000930419,36.7893171041997));
#166134=CARTESIAN_POINT('Ctrl Pts',(6.35117826922837,5.06790226201678,36.7984093801731));
#166135=CARTESIAN_POINT('Ctrl Pts',(6.32767973886511,5.09721177620872,36.7998946432409));
#166136=CARTESIAN_POINT('Ctrl Pts',(6.29108704159569,5.1422105084732,36.8021811512811));
#166137=CARTESIAN_POINT('Ctrl Pts',(6.27813561271742,5.15801495856683,36.8029853984066));
#166138=CARTESIAN_POINT('Ctrl Pts',(6.25310310061931,5.1883278239817,36.8045302105095));
#166139=CARTESIAN_POINT('Ctrl Pts',(6.24103084355399,5.20284326200802,36.8052709832846));
#166140=CARTESIAN_POINT('Ctrl Pts',(6.21227881432031,5.23717005555784,36.8070254988119));
#166141=CARTESIAN_POINT('Ctrl Pts',(6.19555467901422,5.25694402522529,36.8080383379982));
#166142=CARTESIAN_POINT('Ctrl Pts',(6.13772406271013,5.32466141307292,36.8115151893253));
#166143=CARTESIAN_POINT('Ctrl Pts',(6.09615315390873,5.37220556601296,36.8139707233928));
#166144=CARTESIAN_POINT('Ctrl Pts',(6.01819376327414,5.45929653478943,36.8185023654904));
#166145=CARTESIAN_POINT('Ctrl Pts',(5.98195914882804,5.4989762325039,36.8205803174095));
#166146=CARTESIAN_POINT('Ctrl Pts',(5.769923233633,5.72659583849324,36.8325897514008));
#166147=CARTESIAN_POINT('Ctrl Pts',(5.58566569856093,5.90645864221255,36.8424434608015));
#166148=CARTESIAN_POINT('Ctrl Pts',(5.36427886832688,6.10292497201267,36.8538484782136));
#166149=CARTESIAN_POINT('Ctrl Pts',(5.33519184989719,6.12836918832851,36.8553386316102));
#166150=CARTESIAN_POINT('Ctrl Pts',(5.21695299834538,6.23032022758931,36.8613645598991));
#166151=CARTESIAN_POINT('Ctrl Pts',(5.12632875123194,6.30509650775852,36.8659116862093));
#166152=CARTESIAN_POINT('Ctrl Pts',(4.99956641569756,6.40515109198602,36.8721891698899));
#166153=CARTESIAN_POINT('Ctrl Pts',(4.96479633468429,6.43213978337149,36.8739026862686));
#166154=CARTESIAN_POINT('Ctrl Pts',(4.90123654671812,6.48065273283447,36.8770206081783));
#166155=CARTESIAN_POINT('Ctrl Pts',(4.87251999146576,6.50227102270908,36.8784240460397));
#166156=CARTESIAN_POINT('Ctrl Pts',(4.81408304603306,6.54565879951769,36.8812697481869));
#166157=CARTESIAN_POINT('Ctrl Pts',(4.78435615145248,6.56741813031245,36.8827120756956));
#166158=CARTESIAN_POINT('Ctrl Pts',(4.70975343137167,6.62125007601148,36.8863189907494));
#166159=CARTESIAN_POINT('Ctrl Pts',(4.66469714847353,6.65306924869126,36.8884860001418));
#166160=CARTESIAN_POINT('Ctrl Pts',(4.46890306496718,6.78837413212094,36.8978555449286));
#166161=CARTESIAN_POINT('Ctrl Pts',(4.3150213719998,6.88721331881913,36.9051015130549));
#166162=CARTESIAN_POINT('Ctrl Pts',(3.93092016645313,7.11599432806845,36.9229013176412));
#166163=CARTESIAN_POINT('Ctrl Pts',(3.69744233740538,7.24005718718887,36.9334850347367));
#166164=CARTESIAN_POINT('Ctrl Pts',(3.35299403627075,7.40207204874327,36.9486439654369));
#166165=CARTESIAN_POINT('Ctrl Pts',(3.24659832048503,7.44935160758738,36.9532652616882));
#166166=CARTESIAN_POINT('Ctrl Pts',(3.1101921085545,7.50648941035271,36.959096746244));
#166167=CARTESIAN_POINT('Ctrl Pts',(3.08109088575267,7.51848104246908,36.9603355100902));
#166168=CARTESIAN_POINT('Ctrl Pts',(3.0351720827525,7.53709125463276,36.9622813049226));
#166169=CARTESIAN_POINT('Ctrl Pts',(3.01840092689088,7.54382330109867,36.9629901133941));
#166170=CARTESIAN_POINT('Ctrl Pts',(2.98243881361758,7.55811959349055,36.9645061446395));
#166171=CARTESIAN_POINT('Ctrl Pts',(2.96324120935344,7.5656668314918,36.9653131068324));
#166172=CARTESIAN_POINT('Ctrl Pts',(2.91570218016145,7.58414735609598,36.9673058684282));
#166173=CARTESIAN_POINT('Ctrl Pts',(2.88732774747386,7.59499498427004,36.9684904473159));
#166174=CARTESIAN_POINT('Ctrl Pts',(2.77830382789714,7.63597588208995,36.9730247383472));
#166175=CARTESIAN_POINT('Ctrl Pts',(2.6972376993684,7.66498589719664,36.9763602419914));
#166176=CARTESIAN_POINT('Ctrl Pts',(2.53946354156291,7.71863334916932,36.9827961774222));
#166177=CARTESIAN_POINT('Ctrl Pts',(2.46281999595053,7.74342906068706,36.9858975488375));
#166178=CARTESIAN_POINT('Ctrl Pts',(1.94896226853173,7.90127112892282,37.0065595550243));
#166179=CARTESIAN_POINT('Ctrl Pts',(1.50156382844315,7.99836511061295,37.0239653412887));
#166180=CARTESIAN_POINT('Ctrl Pts',(0.936820774476916,8.07184681462946,
37.0460353699289));
#166181=CARTESIAN_POINT('Ctrl Pts',(0.824970751193029,8.08404398672223,
37.0504084235212));
#166182=CARTESIAN_POINT('Ctrl Pts',(0.651625994246511,8.09931202436136,
37.0571951293637));
#166183=CARTESIAN_POINT('Ctrl Pts',(0.590288697053064,8.10401326008582,
37.0595983417141));
#166184=CARTESIAN_POINT('Ctrl Pts',(0.479455008772099,8.1112431892095,37.0639446893855));
#166185=CARTESIAN_POINT('Ctrl Pts',(0.429977542506816,8.11401642061859,
37.0658863299871));
#166186=CARTESIAN_POINT('Ctrl Pts',(0.307841494888655,8.11974191824522,
37.0706829402597));
#166187=CARTESIAN_POINT('Ctrl Pts',(0.235162830702437,8.12217172909592,
37.0735404148275));
#166188=CARTESIAN_POINT('Ctrl Pts',(0.074311987732583,8.12538852871123,
37.0798714590032));
#166189=CARTESIAN_POINT('Ctrl Pts',(-0.0138602377930529,8.12571651275672,
37.0833465282569));
#166190=CARTESIAN_POINT('Ctrl Pts',(-0.331099602795912,8.1217329617424,
37.0958631325346));
#166191=CARTESIAN_POINT('Ctrl Pts',(-0.559955207509258,8.10916911467058,
37.1049205555704));
#166192=CARTESIAN_POINT('Ctrl Pts',(-0.832912518291242,8.08257279461785,
37.1157060478797));
#166193=CARTESIAN_POINT('Ctrl Pts',(-0.877814268914422,8.07781953068325,
37.1174795902134));
#166194=CARTESIAN_POINT('Ctrl Pts',(-0.965958097893199,8.0677450684702,
37.1209588086008));
#166195=CARTESIAN_POINT('Ctrl Pts',(-1.00920163269568,8.06244985194533,
37.1226645815448));
#166196=CARTESIAN_POINT('Ctrl Pts',(-1.16631669276499,8.04192708463447,
37.1288610723782));
#166197=CARTESIAN_POINT('Ctrl Pts',(-1.27990480261986,8.02463268486345,
37.1333390870921));
#166198=CARTESIAN_POINT('Ctrl Pts',(-1.62786416739518,7.96407778132853,
37.1470954496238));
#166199=CARTESIAN_POINT('Ctrl Pts',(-1.86072828706355,7.91291137565185,
37.1563587235238));
#166200=CARTESIAN_POINT('Ctrl Pts',(-2.15069763973565,7.83568778525316,
37.1680892408126));
#166201=CARTESIAN_POINT('Ctrl Pts',(-2.2102062441972,7.81911067398425,37.17050694979));
#166202=CARTESIAN_POINT('Ctrl Pts',(-2.32248887998552,7.78644823374001,
37.1750906684271));
#166203=CARTESIAN_POINT('Ctrl Pts',(-2.37529945309148,7.77050083178002,
37.1772558155614));
#166204=CARTESIAN_POINT('Ctrl Pts',(-2.4996355222113,7.73156863143087,37.1823770365599));
#166205=CARTESIAN_POINT('Ctrl Pts',(-2.57101261945997,7.70812722304184,
37.1853355988369));
#166206=CARTESIAN_POINT('Ctrl Pts',(-2.84548604213709,7.61374903360236,
37.1967903236632));
#166207=CARTESIAN_POINT('Ctrl Pts',(-3.04605780890262,7.53574783376042,
37.2053292329106));
#166208=CARTESIAN_POINT('Ctrl Pts',(-3.43914479004118,7.36461792670848,
37.2224290542481));
#166209=CARTESIAN_POINT('Ctrl Pts',(-3.63155482000086,7.2716657698307,37.2309826625957));
#166210=CARTESIAN_POINT('Ctrl Pts',(-4.02498365326236,7.06208856917623,
37.2488248246091));
#166211=CARTESIAN_POINT('Ctrl Pts',(-4.22511930649394,6.94420312453342,
37.2581047900152));
#166212=CARTESIAN_POINT('Ctrl Pts',(-4.45765602806329,6.79345356826654,
37.2690639667071));
#166213=CARTESIAN_POINT('Ctrl Pts',(-4.49517561882424,6.76868560620335,
37.2708378177359));
#166214=CARTESIAN_POINT('Ctrl Pts',(-4.55415734680582,6.72904303092446,
37.2736343195132));
#166215=CARTESIAN_POINT('Ctrl Pts',(-4.57575656662218,6.71437421518159,
37.2746601115597));
#166216=CARTESIAN_POINT('Ctrl Pts',(-4.61371543992115,6.68832673317683,
37.2764656628244));
#166217=CARTESIAN_POINT('Ctrl Pts',(-4.63010462158914,6.6769915266387,37.2772461600805));
#166218=CARTESIAN_POINT('Ctrl Pts',(-4.66439429131561,6.6530888927767,37.2788809638243));
#166219=CARTESIAN_POINT('Ctrl Pts',(-4.68228600789291,6.64050929256558,
37.2797350014692));
#166220=CARTESIAN_POINT('Ctrl Pts',(-4.7353904189701,6.60285044641319,37.282273078244));
#166221=CARTESIAN_POINT('Ctrl Pts',(-4.77045403140547,6.577562223487,37.2839532452505));
#166222=CARTESIAN_POINT('Ctrl Pts',(-4.83100169349847,6.53315581991052,
37.2868641500685));
#166223=CARTESIAN_POINT('Ctrl Pts',(-4.85657814364462,6.51416541661162,
37.2880967879791));
#166224=CARTESIAN_POINT('Ctrl Pts',(-4.92771580974685,6.46069416844313,
37.2915349384889));
#166225=CARTESIAN_POINT('Ctrl Pts',(-4.97302607511141,6.42588234740215,
37.2937360834726));
#166226=CARTESIAN_POINT('Ctrl Pts',(-5.23730694547424,6.21836611197104,
37.3066559117297));
#166227=CARTESIAN_POINT('Ctrl Pts',(-5.44763640421366,6.03495815963397,
37.3172784499985));
#166228=CARTESIAN_POINT('Ctrl Pts',(-5.77344463889071,5.71991405206738,
37.3346744063742));
#166229=CARTESIAN_POINT('Ctrl Pts',(-5.89483619001525,5.59472833245317,
37.341391299524));
#166230=CARTESIAN_POINT('Ctrl Pts',(-6.04953844358453,5.42456161279612,
37.350315043653));
#166231=CARTESIAN_POINT('Ctrl Pts',(-6.08654678626711,5.38300401726181,
37.352478749762));
#166232=CARTESIAN_POINT('Ctrl Pts',(-6.14497671301229,5.31601860457312,
37.3559427166102));
#166233=CARTESIAN_POINT('Ctrl Pts',(-6.16667424127562,5.29083371509603,
37.3572398454762));
#166234=CARTESIAN_POINT('Ctrl Pts',(-6.21138111746079,5.23829265191314,
37.3599353522033));
#166235=CARTESIAN_POINT('Ctrl Pts',(-6.23436571971809,5.21091636425199,
37.3613339696851));
#166236=CARTESIAN_POINT('Ctrl Pts',(-6.28855855415036,5.14549706166993,
37.3646625506542));
#166237=CARTESIAN_POINT('Ctrl Pts',(-6.31960328727504,5.10732052683797,
37.3665942183325));
#166238=CARTESIAN_POINT('Ctrl Pts',(-6.43021904730197,4.96874053892814,
37.3735682163607));
#166239=CARTESIAN_POINT('Ctrl Pts',(-6.50775912934821,4.86674123106792,
37.3786308862793));
#166240=CARTESIAN_POINT('Ctrl Pts',(-6.65313256662602,4.66582125550979,
37.3884685363232));
#166241=CARTESIAN_POINT('Ctrl Pts',(-6.72125181436785,4.56714733262331,
37.3932398884131));
#166242=CARTESIAN_POINT('Ctrl Pts',(-6.92436992050757,4.25852975226594,
37.4079663257018));
#166243=CARTESIAN_POINT('Ctrl Pts',(-7.05189979707022,4.04384526566632,
37.4179427814488));
#166244=CARTESIAN_POINT('Ctrl Pts',(-7.18731112831798,3.78994771072142,
37.4293273762951));
#166245=CARTESIAN_POINT('Ctrl Pts',(-7.20503828235505,3.75613741401394,
37.4308350727097));
#166246=CARTESIAN_POINT('Ctrl Pts',(-7.23332315298065,3.7012537308262,37.4332682411994));
#166247=CARTESIAN_POINT('Ctrl Pts',(-7.24402857630317,3.68025719292538,
37.4341957381148));
#166248=CARTESIAN_POINT('Ctrl Pts',(-7.26299657439394,3.64265184023095,
37.4358507160412));
#166249=CARTESIAN_POINT('Ctrl Pts',(-7.27129390453646,3.6260607586376,37.4365787323128));
#166250=CARTESIAN_POINT('Ctrl Pts',(-7.2893011607907,3.58974365940494,37.4381675119752));
#166251=CARTESIAN_POINT('Ctrl Pts',(-7.29898795445569,3.57000641399389,
37.4390278538829));
#166252=CARTESIAN_POINT('Ctrl Pts',(-7.32861120175805,3.50902323739837,
37.4416768092871));
#166253=CARTESIAN_POINT('Ctrl Pts',(-7.34827908632698,3.4676477235463,37.4434610245958));
#166254=CARTESIAN_POINT('Ctrl Pts',(-7.3818123117158,3.39553695917885,37.4465497289992));
#166255=CARTESIAN_POINT('Ctrl Pts',(-7.39583816218207,3.36487773013587,
37.4478564563702));
#166256=CARTESIAN_POINT('Ctrl Pts',(-7.4538689188653,3.23591195432174,37.4533275106493));
#166257=CARTESIAN_POINT('Ctrl Pts',(-7.49610802228035,3.13682210138511,
37.4574690966713));
#166258=CARTESIAN_POINT('Ctrl Pts',(-7.69790516422688,2.63604621061694,
37.4781500982383));
#166259=CARTESIAN_POINT('Ctrl Pts',(-7.82720384377732,2.22291883598962,
37.4944365599125));
#166260=CARTESIAN_POINT('Ctrl Pts',(-7.94457133691743,1.70672625379305,
37.5146186533732));
#166261=CARTESIAN_POINT('Ctrl Pts',(-7.96441236199904,1.611602877583,37.5183299258014));
#166262=CARTESIAN_POINT('Ctrl Pts',(-8.02642445376506,1.28510802657773,
37.5310584673055));
#166263=CARTESIAN_POINT('Ctrl Pts',(-8.06025468096189,1.05227573223682,
37.5401209007361));
#166264=CARTESIAN_POINT('Ctrl Pts',(-8.09071468911015,0.751365732986816,
37.5518786850018));
#166265=CARTESIAN_POINT('Ctrl Pts',(-8.09665915119347,0.684342876344953,
37.5545002457673));
#166266=CARTESIAN_POINT('Ctrl Pts',(-8.10490386671329,0.576126850744388,
37.5587385843922));
#166267=CARTESIAN_POINT('Ctrl Pts',(-8.10772404064693,0.534976357811187,
37.5603515488994));
#166268=CARTESIAN_POINT('Ctrl Pts',(-8.11253189252067,0.456012620539981,
37.5634493811644));
#166269=CARTESIAN_POINT('Ctrl Pts',(-8.11456881803018,0.418203424295577,
37.564933867445));
#166270=CARTESIAN_POINT('Ctrl Pts',(-8.11867798966098,0.330524489802689,
37.5683793165677));
#166271=CARTESIAN_POINT('Ctrl Pts',(-8.12055514569915,0.280647181741935,
37.5703415168093));
#166272=CARTESIAN_POINT('Ctrl Pts',(-8.12517923581325,0.117891912762824,
37.5767520528683));
#166273=CARTESIAN_POINT('Ctrl Pts',(-8.1260329277843,0.00497391683127357,
37.58121172188));
#166274=CARTESIAN_POINT('Ctrl Pts',(-8.11665230415639,-0.701196864132818,
37.6091807082722));
#166275=CARTESIAN_POINT('Ctrl Pts',(-8.04381465928052,-1.29179221580849,
37.6329213363231));
#166276=CARTESIAN_POINT('Ctrl Pts',(-7.81238451289496,-2.27083316461565,
37.6748536593953));
#166277=CARTESIAN_POINT('Ctrl Pts',(-7.6869719600454,-2.66467296174595,
37.6924274748187));
#166278=CARTESIAN_POINT('Ctrl Pts',(-7.41659325181163,-3.33299204629362,
37.7228173492243));
#166279=CARTESIAN_POINT('Ctrl Pts',(-7.28482673799094,-3.61192553044677,
37.7356724099883));
#166280=CARTESIAN_POINT('Ctrl Pts',(-7.12694563527753,-3.90215629721046,
37.7488173307995));
#166281=CARTESIAN_POINT('Ctrl Pts',(-7.11628512855021,-3.92156395290631,
37.7496951091407));
#166282=CARTESIAN_POINT('Ctrl Pts',(-7.10117773045857,-3.9488027923744,
37.7509251099551));
#166283=CARTESIAN_POINT('Ctrl Pts',(-7.09679700226935,-3.95667043889293,
37.7512801503172));
#166284=CARTESIAN_POINT('Ctrl Pts',(-7.08912805737579,-3.97038990581443,
37.7518988366926));
#166285=CARTESIAN_POINT('Ctrl Pts',(-7.08584565599744,-3.97624495696774,
37.752162737189));
#166286=CARTESIAN_POINT('Ctrl Pts',(-7.07895676186823,-3.98849754432416,
37.752714693498));
#166287=CARTESIAN_POINT('Ctrl Pts',(-7.07534884220114,-3.99489427382888,
37.7530026851226));
#166288=CARTESIAN_POINT('Ctrl Pts',(-7.06674921007585,-4.01009296096322,
37.7536865373082));
#166289=CARTESIAN_POINT('Ctrl Pts',(-7.06174971083145,-4.01889051560899,
37.7540820415204));
#166290=CARTESIAN_POINT('Ctrl Pts',(-7.04496872040151,-4.04829181342596,
37.7554026316139));
#166291=CARTESIAN_POINT('Ctrl Pts',(-7.03311331796509,-4.06885339510998,
37.7563242358379));
#166292=CARTESIAN_POINT('Ctrl Pts',(-6.85147081991003,-4.38072165329726,
37.7702695720496));
#166293=CARTESIAN_POINT('Ctrl Pts',(-6.66380210607934,-4.66123576650295,
37.7822764784878));
#166294=CARTESIAN_POINT('Ctrl Pts',(-6.36942033038937,-5.04698887739755,
37.7989411004005));
#166295=CARTESIAN_POINT('Ctrl Pts',(-6.27639023583888,-5.16222228308908,
37.8039421614306));
#166296=CARTESIAN_POINT('Ctrl Pts',(-5.69224879535813,-5.84662977798414,
37.8341213880324));
#166297=CARTESIAN_POINT('Ctrl Pts',(-5.12729278828457,-6.34788275721227,
37.8586461976948));
#166298=CARTESIAN_POINT('Ctrl Pts',(-4.397775925233,-6.83335756294451,37.8912973635573));
#166299=CARTESIAN_POINT('Ctrl Pts',(-4.29248813739423,-6.89998207903976,
37.896020176308));
#166300=CARTESIAN_POINT('Ctrl Pts',(-4.16758827443107,-6.97505144784735,
37.9016452888115));
#166301=CARTESIAN_POINT('Ctrl Pts',(-4.1494214556568,-6.98587405416044,
37.9024640060834));
#166302=CARTESIAN_POINT('Ctrl Pts',(-4.12031503642813,-7.00306016864682,
37.9037766448004));
#166303=CARTESIAN_POINT('Ctrl Pts',(-4.1094024076463,-7.00946927915374,
37.9042689850591));
#166304=CARTESIAN_POINT('Ctrl Pts',(-4.09008618469824,-7.02075330351876,
37.905140836942));
#166305=CARTESIAN_POINT('Ctrl Pts',(-4.08168872559977,-7.02563869649252,
37.9055199857134));
#166306=CARTESIAN_POINT('Ctrl Pts',(-4.06446027107756,-7.03562038671822,
37.9062981155256));
#166307=CARTESIAN_POINT('Ctrl Pts',(-4.05562840624721,-7.04071514483439,
37.9066971485883));
#166308=CARTESIAN_POINT('Ctrl Pts',(-4.03312209054852,-7.05364176109653,
37.9077143674218));
#166309=CARTESIAN_POINT('Ctrl Pts',(-4.01943443013445,-7.06145047066264,
37.9083333461994));
#166310=CARTESIAN_POINT('Ctrl Pts',(-3.98974274318605,-7.07827505959329,
37.909676803749));
#166311=CARTESIAN_POINT('Ctrl Pts',(-3.97373070204795,-7.08727657695736,
37.9104017692501));
#166312=CARTESIAN_POINT('Ctrl Pts',(-3.92777101827637,-7.11290909821862,
37.9124840352482));
#166313=CARTESIAN_POINT('Ctrl Pts',(-3.89774870999761,-7.12940502217578,
37.9138459138456));
#166314=CARTESIAN_POINT('Ctrl Pts',(-3.60835263734616,-7.28604094650006,
37.9269902949133));
#166315=CARTESIAN_POINT('Ctrl Pts',(-3.34165616195927,-7.41214636706515,
37.9392431162941));
#166316=CARTESIAN_POINT('Ctrl Pts',(-2.3253892448422,-7.82666643400389,
37.9863302161116));
#166317=CARTESIAN_POINT('Ctrl Pts',(-1.5413366552053,-8.0179935602057,38.023851977727));
#166318=CARTESIAN_POINT('Ctrl Pts',(-0.550792223272148,-8.10883456324062,
38.0663988107547));
#166319=CARTESIAN_POINT('Ctrl Pts',(-0.358968438655843,-8.1195892367817,
38.0743831353632));
#166320=CARTESIAN_POINT('Ctrl Pts',(-0.146292963925848,-8.12395909474444,
38.0828725226761));
#166321=CARTESIAN_POINT('Ctrl Pts',(-0.125669405570101,-8.12430429117005,
38.0836923663129));
#166322=CARTESIAN_POINT('Ctrl Pts',(-0.095339674949844,-8.12469643191405,
38.0848933261827));
#166323=CARTESIAN_POINT('Ctrl Pts',(-0.0856344763786124,-8.12480452084219,
38.0852769085455));
#166324=CARTESIAN_POINT('Ctrl Pts',(-0.0683648892897313,-8.12496590924495,
38.0859582253492));
#166325=CARTESIAN_POINT('Ctrl Pts',(-0.0608005870605701,-8.12502603525592,
38.0862562290318));
#166326=CARTESIAN_POINT('Ctrl Pts',(-0.0450206665026735,-8.1251294266556,
38.0868770330987));
#166327=CARTESIAN_POINT('Ctrl Pts',(-0.0368050415279358,-8.12517079511895,
38.087199759495));
#166328=CARTESIAN_POINT('Ctrl Pts',(-0.0154694692249841,-8.12524586652023,
38.0880366251711));
#166329=CARTESIAN_POINT('Ctrl Pts',(-0.00234944978153691,-8.12526025296515,
38.0885500278008));
#166330=CARTESIAN_POINT('Ctrl Pts',(0.0537593022354977,-8.12518587678321,
38.0907406157975));
#166331=CARTESIAN_POINT('Ctrl Pts',(0.096747353920764,-8.12478772793749,
38.0924063553373));
#166332=CARTESIAN_POINT('Ctrl Pts',(0.428863352570705,-8.1190754538842,
38.1051898146597));
#166333=CARTESIAN_POINT('Ctrl Pts',(0.717539034679774,-8.09867045626168,
38.1158064118681));
#166334=CARTESIAN_POINT('Ctrl Pts',(1.47688289625519,-8.00406721871315,
38.1435128653537));
#166335=CARTESIAN_POINT('Ctrl Pts',(1.94315502220824,-7.90382372627553,
38.1603511095473));
#166336=CARTESIAN_POINT('Ctrl Pts',(2.72693599327359,-7.66172636292324,
38.190433974542));
#166337=CARTESIAN_POINT('Ctrl Pts',(3.04909583246139,-7.53931227673395,
38.2033358106881));
#166338=CARTESIAN_POINT('Ctrl Pts',(3.40986830431454,-7.37530961912341,
38.2185931745888));
#166339=CARTESIAN_POINT('Ctrl Pts',(3.45701835618854,-7.35332699250995,
38.2206031942479));
#166340=CARTESIAN_POINT('Ctrl Pts',(3.5281829894454,-7.31931236692451,38.2236613493931));
#166341=CARTESIAN_POINT('Ctrl Pts',(3.55235454295654,-7.30761150617925,
38.2247043762492));
#166342=CARTESIAN_POINT('Ctrl Pts',(3.59616437697616,-7.28613550037504,
38.2266026283042));
#166343=CARTESIAN_POINT('Ctrl Pts',(3.61582196510093,-7.27640022730247,
38.2274572517716));
#166344=CARTESIAN_POINT('Ctrl Pts',(3.65635295502987,-7.25612275663772,
38.2292253037126));
#166345=CARTESIAN_POINT('Ctrl Pts',(3.67722078418132,-7.2455697975122,38.2301388962755));
#166346=CARTESIAN_POINT('Ctrl Pts',(3.72977441057085,-7.21870766642493,
38.2324482368461));
#166347=CARTESIAN_POINT('Ctrl Pts',(3.76139893641345,-7.20227988555951,
38.2338457810541));
#166348=CARTESIAN_POINT('Ctrl Pts',(3.88773803660394,-7.13559228865542,
38.2394617742274));
#166349=CARTESIAN_POINT('Ctrl Pts',(3.98156055472042,-7.08366849594916,
38.2437069544241));
#166350=CARTESIAN_POINT('Ctrl Pts',(4.21363294470644,-6.94916611545733,
38.2544114808591));
#166351=CARTESIAN_POINT('Ctrl Pts',(4.35050530885193,-6.86430724083353,
38.2609113765764));
#166352=CARTESIAN_POINT('Ctrl Pts',(4.55559190907852,-6.72855738594327,
38.270956421412));
#166353=CARTESIAN_POINT('Ctrl Pts',(4.62567988378337,-6.68056790062044,
38.2744458740129));
#166354=CARTESIAN_POINT('Ctrl Pts',(5.02295929208667,-6.39929960150985,
38.2945532403175));
#166355=CARTESIAN_POINT('Ctrl Pts',(5.33323121619031,-6.14310832854294,
38.3115915519528));
#166356=CARTESIAN_POINT('Ctrl Pts',(5.92115130602959,-5.57942307948749,
38.3461481302878));
#166357=CARTESIAN_POINT('Ctrl Pts',(6.19685755177092,-5.27152512183989,
38.3636140891569));
#166358=CARTESIAN_POINT('Ctrl Pts',(6.46190407002446,-4.9258508646601,38.3809845082919));
#166359=CARTESIAN_POINT('Ctrl Pts',(6.47574789880091,-4.90763691755449,
38.3818935354847));
#166360=CARTESIAN_POINT('Ctrl Pts',(6.4950607049772,-4.88200357891946,38.3831638804721));
#166361=CARTESIAN_POINT('Ctrl Pts',(6.50059419916956,-4.87463306972731,
38.3835281158643));
#166362=CARTESIAN_POINT('Ctrl Pts',(6.51070814152812,-4.86111364271003,
38.38419430383));
#166363=CARTESIAN_POINT('Ctrl Pts',(6.5152924458337,-4.85496763091724,38.3844964345482));
#166364=CARTESIAN_POINT('Ctrl Pts',(6.52455378603278,-4.8425145440255,38.3851071395459));
#166365=CARTESIAN_POINT('Ctrl Pts',(6.52923039364126,-4.83620715884043,
38.3854156935906));
#166366=CARTESIAN_POINT('Ctrl Pts',(6.54070250292334,-4.82068764516996,
38.386173008969));
#166367=CARTESIAN_POINT('Ctrl Pts',(6.54748770574271,-4.81146789960011,
38.386621276952));
#166368=CARTESIAN_POINT('Ctrl Pts',(6.57207127214443,-4.77791540498625,
38.3882466038051));
#166369=CARTESIAN_POINT('Ctrl Pts',(6.58975379945234,-4.7534977982744,38.3894179718311));
#166370=CARTESIAN_POINT('Ctrl Pts',(6.68809068872795,-4.61610219657266,
38.395942851039));
#166371=CARTESIAN_POINT('Ctrl Pts',(6.76597309302061,-4.50117367956736,
38.4011386815693));
#166372=CARTESIAN_POINT('Ctrl Pts',(7.31415715154847,-3.64583640047183,
38.4382074511942));
#166373=CARTESIAN_POINT('Ctrl Pts',(7.66478285444663,-2.835564676331,38.4653766302818));
#166374=CARTESIAN_POINT('Ctrl Pts',(7.89231785045313,-1.93234034343207,
38.4985622363037));
#166375=CARTESIAN_POINT('Ctrl Pts',(7.90502134343568,-1.87969617621614,
38.5005040552427));
#166376=CARTESIAN_POINT('Ctrl Pts',(7.97060789577559,-1.59546970793206,
38.511036158012));
#166377=CARTESIAN_POINT('Ctrl Pts',(8.01383973962798,-1.36179164402329,
38.5198712366129));
#166378=CARTESIAN_POINT('Ctrl Pts',(8.05030829622664,-1.1013057759995,38.5300037371131));
#166379=CARTESIAN_POINT('Ctrl Pts',(8.05372561466883,-1.07603056937347,
38.5309897882464));
#166380=CARTESIAN_POINT('Ctrl Pts',(8.05865928522981,-1.03819941419508,
38.5324700867801));
#166381=CARTESIAN_POINT('Ctrl Pts',(8.0602654320464,-1.02565523559198,38.5329616528943));
#166382=CARTESIAN_POINT('Ctrl Pts',(8.06298135965207,-1.00404313387082,
38.5338098204781));
#166383=CARTESIAN_POINT('Ctrl Pts',(8.06410514757251,-0.994976979126865,
38.5341660032078));
#166384=CARTESIAN_POINT('Ctrl Pts',(8.06633167306494,-0.97676292044406,
38.5348823509958));
#166385=CARTESIAN_POINT('Ctrl Pts',(8.06743414469654,-0.967614997290918,
38.5352425234403));
#166386=CARTESIAN_POINT('Ctrl Pts',(8.06963369640123,-0.949098802267439,
38.5359723384472));
#166387=CARTESIAN_POINT('Ctrl Pts',(8.07073002877807,-0.939730457322439,
38.5363420027014));
#166388=CARTESIAN_POINT('Ctrl Pts',(8.07321103188665,-0.918205262162394,
38.5371923130173));
#166389=CARTESIAN_POINT('Ctrl Pts',(8.07458455919379,-0.906047164163022,
38.5376732908264));
#166390=CARTESIAN_POINT('Ctrl Pts',(8.07803815099798,-0.874845236316933,
38.5389094468736));
#166391=CARTESIAN_POINT('Ctrl Pts',(8.08007833162871,-0.855797116816095,
38.539665812593));
#166392=CARTESIAN_POINT('Ctrl Pts',(8.11085524541885,-0.558524386217931,
38.5514970428282));
#166393=CARTESIAN_POINT('Ctrl Pts',(8.12527172054597,-0.279029717205217,
38.5629994860888));
#166394=CARTESIAN_POINT('Ctrl Pts',(8.12524997543795,0.000631779634971061,
38.5748840163789));
#166395=CARTESIAN_POINT('',(8.13321556035817,0.00564624965145891,40.5832974432124));
#166396=CARTESIAN_POINT('Ctrl Pts',(8.12524999535401,0.000274771867430455,
38.5832974955445));
#166397=CARTESIAN_POINT('Ctrl Pts',(8.12524210757769,0.233523376081798,
38.5924146984481));
#166398=CARTESIAN_POINT('Ctrl Pts',(8.11518633213374,0.466490767603277,
38.6015319013518));
#166399=CARTESIAN_POINT('Ctrl Pts',(8.09518039536984,0.698385229597441,
38.6106491042555));
#166400=CARTESIAN_POINT('Ctrl Pts',(8.07505952886503,0.931611874670458,
38.6198186835003));
#166401=CARTESIAN_POINT('Ctrl Pts',(8.04487389372223,1.16375312819179,38.628988262745));
#166402=CARTESIAN_POINT('Ctrl Pts',(8.00477373273416,1.39401759322803,38.6381578419898));
#166403=CARTESIAN_POINT('Ctrl Pts',(7.96458288338273,1.62480281197092,38.6473481586609));
#166404=CARTESIAN_POINT('Ctrl Pts',(7.91443266829132,1.85370265519256,38.6565384753319));
#166405=CARTESIAN_POINT('Ctrl Pts',(7.85452446651707,2.07993580847695,38.665728792003));
#166406=CARTESIAN_POINT('Ctrl Pts',(7.79451478749117,2.30655217337424,38.6749346759595));
#166407=CARTESIAN_POINT('Ctrl Pts',(7.72471407706188,2.53049271850867,38.6841405599161));
#166408=CARTESIAN_POINT('Ctrl Pts',(7.64537423766149,2.7509889728245,38.6933464438726));
#166409=CARTESIAN_POINT('Ctrl Pts',(7.60797979718048,2.85491323232152,38.697685359634));
#166410=CARTESIAN_POINT('Ctrl Pts',(7.56846701995292,2.95807261897161,38.7020242753955));
#166411=CARTESIAN_POINT('Ctrl Pts',(7.52686604962479,3.06038805276484,38.706363191157));
#166412=CARTESIAN_POINT('Ctrl Pts',(7.4542068057907,3.23908970307095,38.7139414359864));
#166413=CARTESIAN_POINT('Ctrl Pts',(7.3750775372003,3.41545293191262,38.7215196808159));
#166414=CARTESIAN_POINT('Ctrl Pts',(7.28965622804766,3.58895522950425,38.7290979256453));
#166415=CARTESIAN_POINT('Ctrl Pts',(7.20429848313715,3.76232841947436,38.7366705313035));
#166416=CARTESIAN_POINT('Ctrl Pts',(7.11265817321843,3.93284458582282,38.7442431369617));
#166417=CARTESIAN_POINT('Ctrl Pts',(7.01496204782145,4.09999939391761,38.7518157426199));
#166418=CARTESIAN_POINT('Ctrl Pts',(6.91732006844743,4.26706155997525,38.7593841513207));
#166419=CARTESIAN_POINT('Ctrl Pts',(6.81362913699136,4.43076575860533,38.7669525600214));
#166420=CARTESIAN_POINT('Ctrl Pts',(6.70416274786647,4.59063061165015,38.7745209687222));
#166421=CARTESIAN_POINT('Ctrl Pts',(6.59472280669528,4.75045684006997,38.782087548835));
#166422=CARTESIAN_POINT('Ctrl Pts',(6.47951038602011,4.90644526182936,38.7896541289478));
#166423=CARTESIAN_POINT('Ctrl Pts',(6.35884334392026,5.05814184162336,38.7972207090606));
#166424=CARTESIAN_POINT('Ctrl Pts',(6.23819770760759,5.20981151113062,38.8047859468963));
#166425=CARTESIAN_POINT('Ctrl Pts',(6.11209960723124,5.35719056827615,38.812351184732));
#166426=CARTESIAN_POINT('Ctrl Pts',(5.98090820689058,5.49985677843059,38.8199164225677));
#166427=CARTESIAN_POINT('Ctrl Pts',(5.84967118500481,5.64257260047213,38.8274842911997));
#166428=CARTESIAN_POINT('Ctrl Pts',(5.71333757148827,5.78057202814926,38.8350521598316));
#166429=CARTESIAN_POINT('Ctrl Pts',(5.57230486251974,5.913468194016,38.8426200284635));
#166430=CARTESIAN_POINT('Ctrl Pts',(5.43309210538238,6.04464940579732,38.8500902377902));
#166431=CARTESIAN_POINT('Ctrl Pts',(5.28930108925228,6.17085807234827,38.8575604471169));
#166432=CARTESIAN_POINT('Ctrl Pts',(5.14134656895274,6.2917599302912,38.8650306564436));
#166433=CARTESIAN_POINT('Ctrl Pts',(4.95703562845422,6.44237063890872,38.8743364978869));
#166434=CARTESIAN_POINT('Ctrl Pts',(4.76635551154618,6.58467379760845,38.8836423393301));
#166435=CARTESIAN_POINT('Ctrl Pts',(4.57001718157966,6.71823120490555,38.8929481807734));
#166436=CARTESIAN_POINT('Ctrl Pts',(4.37262475073004,6.85250565497774,38.9023039834019));
#166437=CARTESIAN_POINT('Ctrl Pts',(4.16951325608752,6.97794021200562,38.9116597860305));
#166438=CARTESIAN_POINT('Ctrl Pts',(3.96142482957386,7.09413848766259,38.9210155886591));
#166439=CARTESIAN_POINT('Ctrl Pts',(3.75232624712042,7.21090084264062,38.9304168086122));
#166440=CARTESIAN_POINT('Ctrl Pts',(3.53820234340236,7.31833702468645,38.9398180285652));
#166441=CARTESIAN_POINT('Ctrl Pts',(3.31982502679976,7.41609394182234,38.9492192485183));
#166442=CARTESIAN_POINT('Ctrl Pts',(3.101211361138,7.51395666095154,38.9586306433812));
#166443=CARTESIAN_POINT('Ctrl Pts',(2.87833511302379,7.60211915607006,38.968042038244));
#166444=CARTESIAN_POINT('Ctrl Pts',(2.65198891477359,7.68027619024329,38.9774534331069));
#166445=CARTESIAN_POINT('Ctrl Pts',(2.42590822441072,7.75834154490441,38.9868537882457));
#166446=CARTESIAN_POINT('Ctrl Pts',(2.19636575557207,7.82642489015275,38.9962541433845));
#166447=CARTESIAN_POINT('Ctrl Pts',(1.96416892654065,7.88427092320604,39.0056544985233));
#166448=CARTESIAN_POINT('Ctrl Pts',(1.81560460703967,7.9212820080354,39.0116690395921));
#166449=CARTESIAN_POINT('Ctrl Pts',(1.66595402282328,7.95410322194627,39.017683580661));
#166450=CARTESIAN_POINT('Ctrl Pts',(1.51543234454219,7.98267827058158,39.0236981217298));
#166451=CARTESIAN_POINT('Ctrl Pts',(1.32167129884812,8.0194618845272,39.0314404202491));
#166452=CARTESIAN_POINT('Ctrl Pts',(1.12637519902295,8.04922361378799,39.0391827187683));
#166453=CARTESIAN_POINT('Ctrl Pts',(0.930102878696077,8.0718397034097,39.0469250172875));
#166454=CARTESIAN_POINT('Ctrl Pts',(0.733952818251539,8.09444170525555,
39.0546624930559));
#166455=CARTESIAN_POINT('Ctrl Pts',(0.536828097577449,8.10990688979997,
39.0623999688243));
#166456=CARTESIAN_POINT('Ctrl Pts',(0.339297220629357,8.11816265903641,
39.0701374445926));
#166457=CARTESIAN_POINT('Ctrl Pts',(0.141854280614204,8.12641475296378,
39.0778714757861));
#166458=CARTESIAN_POINT('Ctrl Pts',(-0.0559941033429836,8.12746380893499,
39.0856055069797));
#166459=CARTESIAN_POINT('Ctrl Pts',(-0.253674693380241,8.12128910410401,
39.0933395381732));
#166460=CARTESIAN_POINT('Ctrl Pts',(-0.451329986527172,8.11511518944079,
39.1010725796543));
#166461=CARTESIAN_POINT('Ctrl Pts',(-0.648817175395356,8.10171935859924,
39.1088056211354));
#166462=CARTESIAN_POINT('Ctrl Pts',(-0.845563032603451,8.08113300969576,
39.1165386626164));
#166463=CARTESIAN_POINT('Ctrl Pts',(-1.04228923504712,8.06054871735318,
39.1242709315724));
#166464=CARTESIAN_POINT('Ctrl Pts',(-1.23827390224691,8.03277537814228,
39.1320032005285));
#166465=CARTESIAN_POINT('Ctrl Pts',(-1.43294906026735,7.99789625796552,
39.1397354694845));
#166466=CARTESIAN_POINT('Ctrl Pts',(-1.62769910096705,7.96300372137758,
39.1474707126927));
#166467=CARTESIAN_POINT('Ctrl Pts',(-1.82113827796923,7.92100000530547,
39.1552059559009));
#166468=CARTESIAN_POINT('Ctrl Pts',(-2.01270829344443,7.87201961938612,
39.1629411991091));
#166469=CARTESIAN_POINT('Ctrl Pts',(-2.17306223844902,7.83102051996792,
39.1694159950782));
#166470=CARTESIAN_POINT('Ctrl Pts',(-2.33210662913009,7.7851341122364,39.1758907910473));
#166471=CARTESIAN_POINT('Ctrl Pts',(-2.48952222673874,7.73446615126563,
39.1823655870165));
#166472=CARTESIAN_POINT('Ctrl Pts',(-2.69408567132472,7.66862253231183,
39.1907796615209));
#166473=CARTESIAN_POINT('Ctrl Pts',(-2.8959968613616,7.59467172251155,39.1991937360253));
#166474=CARTESIAN_POINT('Ctrl Pts',(-3.09462854244247,7.51285310296963,
39.2076078105297));
#166475=CARTESIAN_POINT('Ctrl Pts',(-3.29331569588629,7.43101163373861,
39.2160242348536));
#166476=CARTESIAN_POINT('Ctrl Pts',(-3.48872126784141,7.34129806886591,
39.2244406591775));
#166477=CARTESIAN_POINT('Ctrl Pts',(-3.68023858701895,7.24399968975129,
39.2328570835014));
#166478=CARTESIAN_POINT('Ctrl Pts',(-3.87180340115735,7.14667718131652,
39.2412755950399));
#166479=CARTESIAN_POINT('Ctrl Pts',(-4.05947780215079,7.0417662229967,39.2496941065784));
#166480=CARTESIAN_POINT('Ctrl Pts',(-4.2426793267108,6.9296002549354,39.2581126181169));
#166481=CARTESIAN_POINT('Ctrl Pts',(-4.42595121821116,6.81739120439429,
39.2665343631705));
#166482=CARTESIAN_POINT('Ctrl Pts',(-4.60474657423996,6.69792171228346,
39.2749561082241));
#166483=CARTESIAN_POINT('Ctrl Pts',(-4.77851034355444,6.57156955825952,
39.2833778532777));
#166484=CARTESIAN_POINT('Ctrl Pts',(-4.95229294838677,6.44520370800729,
39.2918005112255));
#166485=CARTESIAN_POINT('Ctrl Pts',(-5.1210426658387,6.31195386392228,39.3002231691733));
#166486=CARTESIAN_POINT('Ctrl Pts',(-5.28423558932979,6.17223960965227,
39.3086458271211));
#166487=CARTESIAN_POINT('Ctrl Pts',(-5.44745954741912,6.03249878575132,
39.317070086816));
#166488=CARTESIAN_POINT('Ctrl Pts',(-5.60512439998086,5.88629126742338,
39.325494346511));
#166489=CARTESIAN_POINT('Ctrl Pts',(-5.75674033665574,5.73407605973454,
39.3339186062059));
#166490=CARTESIAN_POINT('Ctrl Pts',(-5.79942117540584,5.69122652242889,
39.3362900882382));
#166491=CARTESIAN_POINT('Ctrl Pts',(-5.84162288207641,5.64790113027133,
39.3386615702704));
#166492=CARTESIAN_POINT('Ctrl Pts',(-5.88333505391007,5.60411065254184,
39.3410330523027));
#166493=CARTESIAN_POINT('Ctrl Pts',(-6.03151112962291,5.44855171474736,
39.3494573775228));
#166494=CARTESIAN_POINT('Ctrl Pts',(-6.17352204756723,5.28710500987745,
39.3578817027429));
#166495=CARTESIAN_POINT('Ctrl Pts',(-6.30892210356419,5.12027240033762,
39.366306027963));
#166496=CARTESIAN_POINT('Ctrl Pts',(-6.44429876077515,4.95346862151356,
39.3747288973567));
#166497=CARTESIAN_POINT('Ctrl Pts',(-6.57306667160138,4.78128100183735,
39.3831517667504));
#166498=CARTESIAN_POINT('Ctrl Pts',(-6.69482044007219,4.6042444372222,39.391574636144));
#166499=CARTESIAN_POINT('Ctrl Pts',(-6.81654932795624,4.42724405032592,
39.3999957843102));
#166500=CARTESIAN_POINT('Ctrl Pts',(-6.93126678632341,4.2453969145697,39.4084169324764));
#166501=CARTESIAN_POINT('Ctrl Pts',(-7.03861015199073,4.05926775303046,
39.4168380806426));
#166502=CARTESIAN_POINT('Ctrl Pts',(-7.14592340073171,3.87319081305343,
39.4252568661188));
#166503=CARTESIAN_POINT('Ctrl Pts',(-7.24586655720186,3.68283447526028,
39.4336756515949));
#166504=CARTESIAN_POINT('Ctrl Pts',(-7.33812190544222,3.48878982791584,
39.4420944370711));
#166505=CARTESIAN_POINT('Ctrl Pts',(-7.43035148276851,3.2947993856449,39.4505108708158));
#166506=CARTESIAN_POINT('Ctrl Pts',(-7.51489742641705,3.09712292911058,
39.4589273045606));
#166507=CARTESIAN_POINT('Ctrl Pts',(-7.59148883563105,2.89637442693258,
39.4673437383054));
#166508=CARTESIAN_POINT('Ctrl Pts',(-7.66805244661633,2.69569878478992,
39.475757117374));
#166509=CARTESIAN_POINT('Ctrl Pts',(-7.73666719450974,2.49195356996512,
39.4841704964427));
#166510=CARTESIAN_POINT('Ctrl Pts',(-7.79711065601113,2.28577185659849,
39.4925838755113));
#166511=CARTESIAN_POINT('Ctrl Pts',(-7.8141531339479,2.2276374080786,39.4949560895373));
#166512=CARTESIAN_POINT('Ctrl Pts',(-7.83054629400759,2.16930936624431,
39.4973283035632));
#166513=CARTESIAN_POINT('Ctrl Pts',(-7.84628585923969,2.11080216448517,
39.4997005175892));
#166514=CARTESIAN_POINT('Ctrl Pts',(-7.89760856712009,1.92002510168161,
39.5074357024999));
#166515=CARTESIAN_POINT('Ctrl Pts',(-7.94200084032748,1.72725734574842,
39.5151708874106));
#166516=CARTESIAN_POINT('Ctrl Pts',(-7.97931310134191,1.53305250831581,
39.5229060723212));
#166517=CARTESIAN_POINT('Ctrl Pts',(-8.01661382448334,1.33890772381724,
39.5306388653216));
#166518=CARTESIAN_POINT('Ctrl Pts',(-8.04683882868994,1.14332708930259,
39.538371658322));
#166519=CARTESIAN_POINT('Ctrl Pts',(-8.06988932040479,0.94687587302495,
39.5461044513224));
#166520=CARTESIAN_POINT('Ctrl Pts',(-8.09293677974301,0.750450500624451,
39.5538362270456));
#166521=CARTESIAN_POINT('Ctrl Pts',(-8.10881156616961,0.553155125470171,
39.5615680027687));
#166522=CARTESIAN_POINT('Ctrl Pts',(-8.11746656262995,0.355561762686395,
39.5692997784919));
#166523=CARTESIAN_POINT('Ctrl Pts',(-8.12612465608434,0.157897695602473,
39.5770343208555));
#166524=CARTESIAN_POINT('Ctrl Pts',(-8.12755777838015,-0.0400642190034208,
39.584768863219));
#166525=CARTESIAN_POINT('Ctrl Pts',(-8.1217709068508,-0.237749656428669,
39.5925034055826));
#166526=CARTESIAN_POINT('Ctrl Pts',(-8.11598305798337,-0.435468480720032,
39.6002392542242));
#166527=CARTESIAN_POINT('Ctrl Pts',(-8.10297280358738,-0.632910381755871,
39.6079751028658));
#166528=CARTESIAN_POINT('Ctrl Pts',(-8.0827971702813,-0.829504349953945,
39.6157109515074));
#166529=CARTESIAN_POINT('Ctrl Pts',(-8.06260502835847,-1.02625918023887,
39.6234531299706));
#166530=CARTESIAN_POINT('Ctrl Pts',(-8.0352358371097,-1.22216434056028,
39.6311953084338));
#166531=CARTESIAN_POINT('Ctrl Pts',(-8.00079824059787,-1.41665630120576,
39.638937486897));
#166532=CARTESIAN_POINT('Ctrl Pts',(-7.97198896838768,-1.57936137950603,
39.6454143188899));
#166533=CARTESIAN_POINT('Ctrl Pts',(-7.93823387793344,-1.74107750178691,
39.6518911508828));
#166534=CARTESIAN_POINT('Ctrl Pts',(-7.89962360986838,-1.90148215477032,
39.6583679828757));
#166535=CARTESIAN_POINT('Ctrl Pts',(-7.84359924502978,-2.1342329034937,
39.6677660113473));
#166536=CARTESIAN_POINT('Ctrl Pts',(-7.77732077661169,-2.36435467700588,
39.6771640398188));
#166537=CARTESIAN_POINT('Ctrl Pts',(-7.70105132916896,-2.59104148712539,
39.6865620682903));
#166538=CARTESIAN_POINT('Ctrl Pts',(-7.62467335668622,-2.8180508536022,
39.6959734693698));
#166539=CARTESIAN_POINT('Ctrl Pts',(-7.53827597995956,-3.04161544449088,
39.7053848704492));
#166540=CARTESIAN_POINT('Ctrl Pts',(-7.4421718402354,-3.26094554736923,
39.7147962715287));
#166541=CARTESIAN_POINT('Ctrl Pts',(-7.34621240151355,-3.4799454117603,
39.7241935021554));
#166542=CARTESIAN_POINT('Ctrl Pts',(-7.24057542820372,-3.69472349902118,
39.7335907327821));
#166543=CARTESIAN_POINT('Ctrl Pts',(-7.12561997257765,-3.90451374295218,
39.7429879634088));
#166544=CARTESIAN_POINT('Ctrl Pts',(-7.01095447749335,-4.11377481762839,
39.7523614907143));
#166545=CARTESIAN_POINT('Ctrl Pts',(-6.88701745004613,-4.31807313629427,
39.7617350180199));
#166546=CARTESIAN_POINT('Ctrl Pts',(-6.75421269074996,-4.51666895959979,
39.7711085453255));
#166547=CARTESIAN_POINT('Ctrl Pts',(-6.62227035775963,-4.71397511329438,
39.7804212014953));
#166548=CARTESIAN_POINT('Ctrl Pts',(-6.48157509905111,-4.90565254558841,
39.7897338576651));
#166549=CARTESIAN_POINT('Ctrl Pts',(-6.33256970855235,-5.0909968030657,
39.799046513835));
#166550=CARTESIAN_POINT('Ctrl Pts',(-6.23662686349042,-5.21033782367401,
39.8050428252773));
#166551=CARTESIAN_POINT('Ctrl Pts',(-6.13723964548609,-5.32705358214587,
39.8110391367196));
#166552=CARTESIAN_POINT('Ctrl Pts',(-6.03453665110094,-5.44096084979661,
39.817035448162));
#166553=CARTESIAN_POINT('Ctrl Pts',(-5.90492010824206,-5.58471777069049,
39.824603106376));
#166554=CARTESIAN_POINT('Ctrl Pts',(-5.77007134326542,-5.72394222342455,
39.83217076459));
#166555=CARTESIAN_POINT('Ctrl Pts',(-5.63035866508292,-5.85822062276812,
39.839738422804));
#166556=CARTESIAN_POINT('Ctrl Pts',(-5.49068467082975,-5.99246184283649,
39.8473039856694));
#166557=CARTESIAN_POINT('Ctrl Pts',(-5.34614970784548,-6.12175947992718,
39.8548695485349));
#166558=CARTESIAN_POINT('Ctrl Pts',(-5.19715958558022,-6.24573612991388,
39.8624351114004));
#166559=CARTESIAN_POINT('Ctrl Pts',(-5.04818251625903,-6.3697019183733,
39.870000011451));
#166560=CARTESIAN_POINT('Ctrl Pts',(-4.89475134769421,-6.48834741307377,
39.8775649115016));
#166561=CARTESIAN_POINT('Ctrl Pts',(-4.73730560536102,-6.60133495316781,
39.8851298115521));
#166562=CARTESIAN_POINT('Ctrl Pts',(-4.57978258963036,-6.71437794684837,
39.8926984244089));
#166563=CARTESIAN_POINT('Ctrl Pts',(-4.41824136106163,-6.82175722093497,
39.9002670372657));
#166564=CARTESIAN_POINT('Ctrl Pts',(-4.25315158443686,-6.92317767808268,
39.9078356501225));
#166565=CARTESIAN_POINT('Ctrl Pts',(-4.08802509474823,-7.02462068935697,
39.9154059461058));
#166566=CARTESIAN_POINT('Ctrl Pts',(-3.91934880428558,-7.12010206132231,
39.922976242089));
#166567=CARTESIAN_POINT('Ctrl Pts',(-3.74761746868852,-7.20937243252703,
39.9305465380722));
#166568=CARTESIAN_POINT('Ctrl Pts',(-3.57571212029093,-7.29873326006718,
39.9381245049234));
#166569=CARTESIAN_POINT('Ctrl Pts',(-3.40074587347904,-7.38187035350387,
39.9457024717746));
#166570=CARTESIAN_POINT('Ctrl Pts',(-3.22323480882442,-7.45858196507101,
39.9532804386259));
#166571=CARTESIAN_POINT('Ctrl Pts',(-3.04815542160801,-7.53424272442532,
39.9607545969001));
#166572=CARTESIAN_POINT('Ctrl Pts',(-2.87060083248374,-7.60365286137363,
39.9682287551743));
#166573=CARTESIAN_POINT('Ctrl Pts',(-2.69108010185882,-7.66666651471678,
39.9757029134486));
#166574=CARTESIAN_POINT('Ctrl Pts',(-2.49713188231875,-7.73474436750891,
39.9837777451675));
#166575=CARTESIAN_POINT('Ctrl Pts',(-2.30047481299285,-7.79550205760272,
39.9918525768864));
#166576=CARTESIAN_POINT('Ctrl Pts',(-2.10168916992473,-7.84873175713893,
39.9999274086052));
#166577=CARTESIAN_POINT('Ctrl Pts',(-1.90303504311832,-7.90192623999154,
40.0079968980285));
#166578=CARTESIAN_POINT('Ctrl Pts',(-1.70225545583536,-7.94760258222244,
40.0160663874517));
#166579=CARTESIAN_POINT('Ctrl Pts',(-1.49994657558979,-7.98560253411579,
40.0241358768749));
#166580=CARTESIAN_POINT('Ctrl Pts',(-1.29774398181256,-8.02358252207735,
40.0322011268523));
#166581=CARTESIAN_POINT('Ctrl Pts',(-1.09401400802125,-8.05389410411521,
40.0402663768297));
#166582=CARTESIAN_POINT('Ctrl Pts',(-0.889364382368222,-8.07642981507762,
40.0483316268072));
#166583=CARTESIAN_POINT('Ctrl Pts',(-0.684794422560027,-8.09895675335625,
40.0563937371504));
#166584=CARTESIAN_POINT('Ctrl Pts',(-0.479305839345301,-8.11371382319431,
40.0644558474937));
#166585=CARTESIAN_POINT('Ctrl Pts',(-0.273513501540643,-8.12064516691716,
40.072517957837));
#166586=CARTESIAN_POINT('Ctrl Pts',(-0.0677732906805856,-8.12757475493921,
40.0805780260577));
#166587=CARTESIAN_POINT('Ctrl Pts',(0.138270204976888,-8.12668256027873,
40.0886380942784));
#166588=CARTESIAN_POINT('Ctrl Pts',(0.343999451035131,-8.11796476588729,
40.0966981624991));
#166589=CARTESIAN_POINT('Ctrl Pts',(0.552810828024079,-8.10911636593415,
40.1048789825625));
#166590=CARTESIAN_POINT('Ctrl Pts',(0.761298131211823,-8.09220600530942,
40.1130598026259));
#166591=CARTESIAN_POINT('Ctrl Pts',(0.968817375836679,-8.06728457752526,
40.1212406226894));
#166592=CARTESIAN_POINT('Ctrl Pts',(1.17329341071894,-8.04272861527645,
40.1293014733911));
#166593=CARTESIAN_POINT('Ctrl Pts',(1.37682926588926,-8.01039499268433,
40.1373623240928));
#166594=CARTESIAN_POINT('Ctrl Pts',(1.5788153236076,-7.97038454131555,40.1454231747945));
#166595=CARTESIAN_POINT('Ctrl Pts',(1.78083487887691,-7.93036745457723,
40.1534853623151));
#166596=CARTESIAN_POINT('Ctrl Pts',(1.98130381317512,-7.88267106129582,
40.1615475498356));
#166597=CARTESIAN_POINT('Ctrl Pts',(2.17962331319072,-7.8274472067907,40.1696097373561));
#166598=CARTESIAN_POINT('Ctrl Pts',(2.37800027094315,-7.77220735266023,
40.1776742606784));
#166599=CARTESIAN_POINT('Ctrl Pts',(2.57422624714499,-7.70943577251278,
40.1857387840007));
#166600=CARTESIAN_POINT('Ctrl Pts',(2.76771760874932,-7.63933418569439,
40.1938033073231));
#166601=CARTESIAN_POINT('Ctrl Pts',(2.96612802988728,-7.56745043208517,
40.2020728520479));
#166602=CARTESIAN_POINT('Ctrl Pts',(3.16166262005876,-7.48785916244496,
40.2103423967728));
#166603=CARTESIAN_POINT('Ctrl Pts',(3.35371411149903,-7.40083030617729,
40.2186119414977));
#166604=CARTESIAN_POINT('Ctrl Pts',(3.54125725758373,-7.31584442357785,
40.2266873613903));
#166605=CARTESIAN_POINT('Ctrl Pts',(3.72547872804214,-7.22376639577497,
40.234762781283));
#166606=CARTESIAN_POINT('Ctrl Pts',(3.90583789202167,-7.12489423947806,
40.2428382011756));
#166607=CARTESIAN_POINT('Ctrl Pts',(4.09270053066488,-7.02245690495992,
40.2512048083166));
#166608=CARTESIAN_POINT('Ctrl Pts',(4.27541682254546,-6.91272655889478,
40.2595714154575));
#166609=CARTESIAN_POINT('Ctrl Pts',(4.45341796277665,-6.79608387318155,
40.2679380225985));
#166610=CARTESIAN_POINT('Ctrl Pts',(4.63141910300777,-6.67944118746835,
40.2763046297395));
#166611=CARTESIAN_POINT('Ctrl Pts',(4.80470480775092,-6.55588641026857,
40.2846712368804));
#166612=CARTESIAN_POINT('Ctrl Pts',(4.97274368742939,-6.4258468532662,40.2930378440214));
#166613=CARTESIAN_POINT('Ctrl Pts',(5.13498501363584,-6.30029382513525,
40.3011157926545));
#166614=CARTESIAN_POINT('Ctrl Pts',(5.29265095278334,-6.16845190210063,
40.3091937412875));
#166615=CARTESIAN_POINT('Ctrl Pts',(5.44523946487812,-6.03067614224424,
40.3172716899206));
#166616=CARTESIAN_POINT('Ctrl Pts',(5.59764123962346,-5.89306899193688,
40.3253397527851));
#166617=CARTESIAN_POINT('Ctrl Pts',(5.74497774094924,-5.7495426899506,40.3334078156496));
#166618=CARTESIAN_POINT('Ctrl Pts',(5.88677796803571,-5.60049397085198,
40.3414758785141));
#166619=CARTESIAN_POINT('Ctrl Pts',(6.02842211784675,-5.45160930732971,
40.3495350609889));
#166620=CARTESIAN_POINT('Ctrl Pts',(6.16454192508588,-5.29721457162391,
40.3575942434637));
#166621=CARTESIAN_POINT('Ctrl Pts',(6.29470095649393,-5.13774536453631,
40.3656534259386));
#166622=CARTESIAN_POINT('Ctrl Pts',(6.4246928031767,-4.97848099006993,40.3737022566753));
#166623=CARTESIAN_POINT('Ctrl Pts',(6.54873894957274,-4.81415539079815,
40.381751087412));
#166624=CARTESIAN_POINT('Ctrl Pts',(6.66644115792267,-4.64523948257295,
40.3897999181487));
#166625=CARTESIAN_POINT('Ctrl Pts',(6.78405433685325,-4.47645134157862,
40.3978426607861));
#166626=CARTESIAN_POINT('Ctrl Pts',(6.89533296268568,-4.30308007029934,
40.4058854034236));
#166627=CARTESIAN_POINT('Ctrl Pts',(6.99991945712543,-4.12562906188338,
40.413928146061));
#166628=CARTESIAN_POINT('Ctrl Pts',(7.10442076192845,-3.94832259399369,
40.4219643375818));
#166629=CARTESIAN_POINT('Ctrl Pts',(7.20224064897075,-3.76694328896893,
40.4300005291027));
#166630=CARTESIAN_POINT('Ctrl Pts',(7.2930650610116,-3.58202311248154,40.4380367206235));
#166631=CARTESIAN_POINT('Ctrl Pts',(7.34455883669927,-3.47718083633352,
40.4425929168516));
#166632=CARTESIAN_POINT('Ctrl Pts',(7.39380475576001,-3.37120089226644,
40.4471491130796));
#166633=CARTESIAN_POINT('Ctrl Pts',(7.44075200433485,-3.26418399795216,
40.4517053093077));
#166634=CARTESIAN_POINT('Ctrl Pts',(7.52120398147608,-3.08079261727573,
40.4595131150027));
#166635=CARTESIAN_POINT('Ctrl Pts',(7.59485701558088,-2.89445919022869,
40.4673209206978));
#166636=CARTESIAN_POINT('Ctrl Pts',(7.66150718331788,-2.70573377154303,
40.4751287263929));
#166637=CARTESIAN_POINT('Ctrl Pts',(7.72817956003812,-2.51694546629906,
40.4829391337833));
#166638=CARTESIAN_POINT('Ctrl Pts',(7.78784430650326,-2.32576390492744,
40.4907495411736));
#166639=CARTESIAN_POINT('Ctrl Pts',(7.84034725305165,-2.13275467742199,
40.498559948564));
#166640=CARTESIAN_POINT('Ctrl Pts',(7.89290272100167,-1.93955237284525,
40.5063781691071));
#166641=CARTESIAN_POINT('Ctrl Pts',(7.93828198712675,-1.74451908146978,
40.5141963896502));
#166642=CARTESIAN_POINT('Ctrl Pts',(7.97638169558376,-1.548232091405,40.5220146101934));
#166643=CARTESIAN_POINT('Ctrl Pts',(8.01450240419812,-1.35183691002216,
40.5298371400572));
#166644=CARTESIAN_POINT('Ctrl Pts',(8.04533550241622,-1.15418699087737,
40.537659669921));
#166645=CARTESIAN_POINT('Ctrl Pts',(8.06882945521055,-0.955865463978399,
40.5454821997848));
#166646=CARTESIAN_POINT('Ctrl Pts',(8.09235375840566,-0.75728773762769,
40.5533148350965));
#166647=CARTESIAN_POINT('Ctrl Pts',(8.10851994674541,-0.5580370118204,40.5611474704083));
#166648=CARTESIAN_POINT('Ctrl Pts',(8.11732856393124,-0.358698407699219,
40.56898010572));
#166649=CARTESIAN_POINT('Ctrl Pts',(8.12269567815148,-0.237240858318737,
40.5737525515508));
#166650=CARTESIAN_POINT('Ctrl Pts',(8.12533231449817,-0.115750656374641,
40.5785249973816));
#166651=CARTESIAN_POINT('Ctrl Pts',(8.12524804204743,0.00564071843232957,
40.5832974432124));
#166652=CARTESIAN_POINT('',(8.12839272208226,-0.00745291321414085,42.5832974432124));
#166653=CARTESIAN_POINT('Ctrl Pts',(8.1335321614197,0.00564646944258829,
40.5832974432124));
#166654=CARTESIAN_POINT('Ctrl Pts',(8.13406518936364,0.235442656146337,
40.592322553673));
#166655=CARTESIAN_POINT('Ctrl Pts',(8.01157082498974,3.15609430641961,40.7071259743246));
#166656=CARTESIAN_POINT('Ctrl Pts',(5.36683002199982,7.17838145731516,40.8748185500716));
#166657=CARTESIAN_POINT('Ctrl Pts',(-0.0971997372527671,8.45625233235374,
41.0863751704535));
#166658=CARTESIAN_POINT('Ctrl Pts',(-4.11199154399871,7.40600674809268,
41.2450426357399));
#166659=CARTESIAN_POINT('Ctrl Pts',(-7.16239838942506,4.52625027289421,
41.4037101010264));
#166660=CARTESIAN_POINT('Ctrl Pts',(-8.44679792391067,0.555938847209571,
41.5623775663127));
#166661=CARTESIAN_POINT('Ctrl Pts',(-7.69384797441526,-3.5484638321857,
41.7210450315993));
#166662=CARTESIAN_POINT('Ctrl Pts',(-5.04719085354645,-6.80318123369981,
41.8797124968856));
#166663=CARTESIAN_POINT('Ctrl Pts',(-1.20468243235761,-8.37056697807599,
42.0383799621721));
#166664=CARTESIAN_POINT('Ctrl Pts',(4.37969769530886,-7.8198639968973,42.249936582554));
#166665=CARTESIAN_POINT('Ctrl Pts',(7.7907102434175,-3.87609838062196,42.4315757429007));
#166666=CARTESIAN_POINT('Ctrl Pts',(8.13117600443575,-0.594204244146628,
42.560325748152));
#166667=CARTESIAN_POINT('Ctrl Pts',(8.12839272208226,-0.00745291321414085,
42.5832974432124));
#166668=CARTESIAN_POINT('',(8.12524955251516,0.00269662821826551,44.583297171399));
#166669=CARTESIAN_POINT('Ctrl Pts',(8.12524658453976,-0.00745002852452582,
42.5832974432124));
#166670=CARTESIAN_POINT('Ctrl Pts',(8.125424793707,0.186910761202144,42.5909097800438));
#166671=CARTESIAN_POINT('Ctrl Pts',(8.1186250423802,0.38149919825017,42.5985221168752));
#166672=CARTESIAN_POINT('Ctrl Pts',(8.10482517209636,0.575757320624921,
42.6061344537066));
#166673=CARTESIAN_POINT('Ctrl Pts',(8.0910334440581,0.769900826173182,42.6137422990816));
#166674=CARTESIAN_POINT('Ctrl Pts',(8.07024984038095,0.963714043864039,
42.6213501444566));
#166675=CARTESIAN_POINT('Ctrl Pts',(8.04250426345775,1.15663854974833,42.6289579898316));
#166676=CARTESIAN_POINT('Ctrl Pts',(8.01476867647924,1.34949359212325,42.6365630959608));
#166677=CARTESIAN_POINT('Ctrl Pts',(7.98007615324187,1.54146019994278,42.6441682020901));
#166678=CARTESIAN_POINT('Ctrl Pts',(7.93850849296427,1.73198454659221,42.6517733082193));
#166679=CARTESIAN_POINT('Ctrl Pts',(7.89974440751617,1.90965877709106,42.6588654799188));
#166680=CARTESIAN_POINT('Ctrl Pts',(7.85500184496421,2.08607854171707,42.6659576516182));
#166681=CARTESIAN_POINT('Ctrl Pts',(7.80438735580326,2.26080197343293,42.6730498233177));
#166682=CARTESIAN_POINT('Ctrl Pts',(7.74703340365876,2.45879032631913,42.6810863378217));
#166683=CARTESIAN_POINT('Ctrl Pts',(7.68216389414845,2.65451657047691,42.6891228523257));
#166684=CARTESIAN_POINT('Ctrl Pts',(7.60999333669341,2.84740038947492,42.6971593668296));
#166685=CARTESIAN_POINT('Ctrl Pts',(7.53777918103935,3.04040072949511,42.7052007361881));
#166686=CARTESIAN_POINT('Ctrl Pts',(7.45825528881192,3.23055492283526,42.7132421055467));
#166687=CARTESIAN_POINT('Ctrl Pts',(7.37168408566763,3.417303220906,42.7212834749052));
#166688=CARTESIAN_POINT('Ctrl Pts',(7.28504999994233,3.60418716702778,42.7293306852598));
#166689=CARTESIAN_POINT('Ctrl Pts',(7.19135852319594,3.78765999591063,42.7373778956144));
#166690=CARTESIAN_POINT('Ctrl Pts',(7.09091800857552,3.96718657970096,42.745425105969));
#166691=CARTESIAN_POINT('Ctrl Pts',(6.99032945180891,4.14697777285597,42.7534841773371));
#166692=CARTESIAN_POINT('Ctrl Pts',(6.88297212967956,4.32281081980967,42.7615432487051));
#166693=CARTESIAN_POINT('Ctrl Pts',(6.76919865742865,4.49417813384897,42.7696023200731));
#166694=CARTESIAN_POINT('Ctrl Pts',(6.65533310272477,4.66568414386302,42.777667914043));
#166695=CARTESIAN_POINT('Ctrl Pts',(6.53504121920107,4.83271695246856,42.7857335080129));
#166696=CARTESIAN_POINT('Ctrl Pts',(6.40871644794992,4.99480140268621,42.7937991019827));
#166697=CARTESIAN_POINT('Ctrl Pts',(6.28219331794693,5.15714036252158,42.8018773607779));
#166698=CARTESIAN_POINT('Ctrl Pts',(6.14961856844111,5.31451519149669,42.809955619573));
#166699=CARTESIAN_POINT('Ctrl Pts',(6.01142427219216,5.46648568846558,42.8180338783681));
#166700=CARTESIAN_POINT('Ctrl Pts',(5.93339717518889,5.55229108731696,42.8225950151135));
#166701=CARTESIAN_POINT('Ctrl Pts',(5.85357924497781,5.63637430762845,42.8271561518589));
#166702=CARTESIAN_POINT('Ctrl Pts',(5.77205298301743,5.71866172489155,42.8317172886043));
#166703=CARTESIAN_POINT('Ctrl Pts',(5.62751946306841,5.86454465609143,42.8398034823403));
#166704=CARTESIAN_POINT('Ctrl Pts',(5.47733352188085,6.00506501671852,42.8478896760762));
#166705=CARTESIAN_POINT('Ctrl Pts',(5.32191951398793,6.13977688919837,42.8559758698122));
#166706=CARTESIAN_POINT('Ctrl Pts',(5.16664412801486,6.27436860508074,42.8640548510471));
#166707=CARTESIAN_POINT('Ctrl Pts',(5.00615021152948,6.40316195653402,42.872133832282));
#166708=CARTESIAN_POINT('Ctrl Pts',(4.84089867607219,6.52574804681444,42.8802128135169));
#166709=CARTESIAN_POINT('Ctrl Pts',(4.6757719711654,6.64824153590304,42.8882856919118));
#166710=CARTESIAN_POINT('Ctrl Pts',(4.50589506732835,6.7645369259048,42.8963585703067));
#166711=CARTESIAN_POINT('Ctrl Pts',(4.33176211900848,6.87426537942951,42.9044314487016));
#166712=CARTESIAN_POINT('Ctrl Pts',(4.15773696676393,6.98392590613879,42.9124993296241));
#166713=CARTESIAN_POINT('Ctrl Pts',(3.97946129164463,7.08702743509267,42.9205672105466));
#166714=CARTESIAN_POINT('Ctrl Pts',(3.79745892349286,7.18324392505812,42.9286350914691));
#166715=CARTESIAN_POINT('Ctrl Pts',(3.61554443704029,7.27941395591035,42.936699076733));
#166716=CARTESIAN_POINT('Ctrl Pts',(3.42990712615521,7.36870543069015,42.944763061997));
#166717=CARTESIAN_POINT('Ctrl Pts',(3.24109670272519,7.45083751843267,42.9528270472609));
#166718=CARTESIAN_POINT('Ctrl Pts',(3.04966241917648,7.5341109791226,42.9610030960907));
#166719=CARTESIAN_POINT('Ctrl Pts',(2.85496646216837,7.61002442414159,42.9691791449206));
#166720=CARTESIAN_POINT('Ctrl Pts',(2.65760536674899,7.67833453797938,42.9773551937504));
#166721=CARTESIAN_POINT('Ctrl Pts',(2.46304159177226,7.74567645047297,42.9854153584012));
#166722=CARTESIAN_POINT('Ctrl Pts',(2.26588803830114,7.80562904084697,42.9934755230519));
#166723=CARTESIAN_POINT('Ctrl Pts',(2.06673442137547,7.85800842414933,43.0015356877026));
#166724=CARTESIAN_POINT('Ctrl Pts',(1.86759042655388,7.91038527674255,43.0095954629266));
#166725=CARTESIAN_POINT('Ctrl Pts',(1.66644686737592,7.9551895715948,43.0176552381506));
#166726=CARTESIAN_POINT('Ctrl Pts',(1.46390689294527,7.99228779332222,43.0257150133746));
#166727=CARTESIAN_POINT('Ctrl Pts',(1.26135162649032,8.02938881601231,43.0337753971218));
#166728=CARTESIAN_POINT('Ctrl Pts',(1.05740004618877,8.05878254864867,43.0418357808691));
#166729=CARTESIAN_POINT('Ctrl Pts',(0.852664321026222,8.08038681735899,
43.0498961646163));
#166730=CARTESIAN_POINT('Ctrl Pts',(0.642781977833522,8.10253417115514,
43.058159169163));
#166731=CARTESIAN_POINT('Ctrl Pts',(0.432075896998746,8.11649526279491,
43.0664221737098));
#166732=CARTESIAN_POINT('Ctrl Pts',(0.221210092009776,8.12223821724609,
43.0746851782565));
#166733=CARTESIAN_POINT('Ctrl Pts',(0.0153458712982696,8.12784495297424,
43.0827521903159));
#166734=CARTESIAN_POINT('Ctrl Pts',(-0.19067026004267,8.12561900844492,
43.0908192023752));
#166735=CARTESIAN_POINT('Ctrl Pts',(-0.396221094634212,8.11558355305808,
43.0988862144346));
#166736=CARTESIAN_POINT('Ctrl Pts',(-0.609262884810202,8.10518237232296,
43.107247215225));
#166737=CARTESIAN_POINT('Ctrl Pts',(-0.821804453695356,8.0863918022516,
43.1156082160154));
#166738=CARTESIAN_POINT('Ctrl Pts',(-1.03316484413242,8.05929636924644,
43.1239692168059));
#166739=CARTESIAN_POINT('Ctrl Pts',(-1.24452523456955,8.03220093624127,
43.1323302175963));
#166740=CARTESIAN_POINT('Ctrl Pts',(-1.45470407869705,7.99680072666137,
43.1406912183867));
#166741=CARTESIAN_POINT('Ctrl Pts',(-1.6630322704497,7.95323904016112,43.1490522191772));
#166742=CARTESIAN_POINT('Ctrl Pts',(-1.85185679999638,7.91375559391954,
43.156630464001));
#166743=CARTESIAN_POINT('Ctrl Pts',(-2.03953933790646,7.86748795352796,
43.1642087088247));
#166744=CARTESIAN_POINT('Ctrl Pts',(-2.22553394789696,7.81451765685242,
43.1717869536485));
#166745=CARTESIAN_POINT('Ctrl Pts',(-2.41139015440928,7.76158677676696,
43.1793595593011));
#166746=CARTESIAN_POINT('Ctrl Pts',(-2.59556058061479,7.70196326254506,
43.1869321649537));
#166747=CARTESIAN_POINT('Ctrl Pts',(-2.77750843885825,7.63577988384757,
43.1945047706063));
#166748=CARTESIAN_POINT('Ctrl Pts',(-2.95935545632893,7.56963318589541,
43.2020731793015));
#166749=CARTESIAN_POINT('Ctrl Pts',(-3.13898201277821,7.49693398313537,
43.2096415879967));
#166750=CARTESIAN_POINT('Ctrl Pts',(-3.31586553502567,7.41786514545317,
43.2172099966919));
#166751=CARTESIAN_POINT('Ctrl Pts',(-3.49270632080368,7.33881541143265,
43.2247765767993));
#166752=CARTESIAN_POINT('Ctrl Pts',(-3.66680505310869,7.2533992480984,43.2323431569066));
#166753=CARTESIAN_POINT('Ctrl Pts',(-3.83765811512838,7.16184806833329,
43.2399097370139));
#166754=CARTESIAN_POINT('Ctrl Pts',(-4.00848086858873,7.07031312933279,
43.2474749748442));
#166755=CARTESIAN_POINT('Ctrl Pts',(-4.17605877515832,6.97264551658212,
43.2550402126745));
#166756=CARTESIAN_POINT('Ctrl Pts',(-4.33991210770841,6.86912297603311,
43.2626054505048));
#166757=CARTESIAN_POINT('Ctrl Pts',(-4.50382241992725,6.76556443572763,
43.2701733191314));
#166758=CARTESIAN_POINT('Ctrl Pts',(-4.66400525755614,6.65614709391517,
43.277741187758));
#166759=CARTESIAN_POINT('Ctrl Pts',(-4.82000882456867,6.54119274242703,
43.2853090563847));
#166760=CARTESIAN_POINT('Ctrl Pts',(-4.97399924960415,6.42772181490706,
43.2927792657442));
#166761=CARTESIAN_POINT('Ctrl Pts',(-5.12391736857331,6.30885616908336,
43.3002494751038));
#166762=CARTESIAN_POINT('Ctrl Pts',(-5.26936004855676,6.18494399660772,
43.3077196844634));
#166763=CARTESIAN_POINT('Ctrl Pts',(-5.4505419208893,6.0305832586422,43.3170255259031));
#166764=CARTESIAN_POINT('Ctrl Pts',(-5.6246911036513,5.86846861385627,43.3263313673427));
#166765=CARTESIAN_POINT('Ctrl Pts',(-5.79124916197024,5.69922106138014,
43.3356372087824));
#166766=CARTESIAN_POINT('Ctrl Pts',(-5.95870143688861,5.52906485295327,
43.3449930114066));
#166767=CARTESIAN_POINT('Ctrl Pts',(-6.11848086444778,5.35169901118755,
43.3543488140308));
#166768=CARTESIAN_POINT('Ctrl Pts',(-6.27006456547053,5.16778268770377,
43.363704616655));
#166769=CARTESIAN_POINT('Ctrl Pts',(-6.42238412276047,4.9829735506895,43.3731058366027));
#166770=CARTESIAN_POINT('Ctrl Pts',(-6.56642818044302,4.79155022730358,
43.3825070565505));
#166771=CARTESIAN_POINT('Ctrl Pts',(-6.70171112354593,4.59420891765283,
43.3919082764983));
#166772=CARTESIAN_POINT('Ctrl Pts',(-6.83714048293256,4.39665402615264,
43.4013196713554));
#166773=CARTESIAN_POINT('Ctrl Pts',(-6.96378974949471,4.19316837376188,
43.4107310662125));
#166774=CARTESIAN_POINT('Ctrl Pts',(-7.08121667856289,3.98447711923945,
43.4201424610697));
#166775=CARTESIAN_POINT('Ctrl Pts',(-7.19850586387032,3.77603066306491,
43.4295428162025));
#166776=CARTESIAN_POINT('Ctrl Pts',(-7.30659432077361,3.5623908439446,43.4389431713354));
#166777=CARTESIAN_POINT('Ctrl Pts',(-7.40508628375777,3.34430630962574,
43.4483435264682));
#166778=CARTESIAN_POINT('Ctrl Pts',(-7.46810347304673,3.20477132663045,
43.4543580675621));
#166779=CARTESIAN_POINT('Ctrl Pts',(-7.52719304454957,3.06341733066499,
43.4603726086561));
#166780=CARTESIAN_POINT('Ctrl Pts',(-7.58226108188434,2.92044593318249,
43.46638714975));
#166781=CARTESIAN_POINT('Ctrl Pts',(-7.65314815031847,2.73640408734998,
43.4741294483094));
#166782=CARTESIAN_POINT('Ctrl Pts',(-7.71740173389768,2.54959454654449,
43.4818717468688));
#166783=CARTESIAN_POINT('Ctrl Pts',(-7.77480000416057,2.36054494932947,
43.4896140454281));
#166784=CARTESIAN_POINT('Ctrl Pts',(-7.83216252049865,2.17161311289453,
43.4973515212366));
#166785=CARTESIAN_POINT('Ctrl Pts',(-7.88267812383826,1.98044433497426,
43.5050889970451));
#166786=CARTESIAN_POINT('Ctrl Pts',(-7.92617358399279,1.7875849291474,43.5128264728536));
#166787=CARTESIAN_POINT('Ctrl Pts',(-7.96964968080811,1.59481138060497,
43.5205605040872));
#166788=CARTESIAN_POINT('Ctrl Pts',(-8.00611178113934,1.40034904700722,
43.5282945353208));
#166789=CARTESIAN_POINT('Ctrl Pts',(-8.03543684367452,1.20475818894004,
43.5360285665544));
#166790=CARTESIAN_POINT('Ctrl Pts',(-8.06475815352443,1.00919236034829,
43.5437616080753));
#166791=CARTESIAN_POINT('Ctrl Pts',(-8.08694418480647,0.812498642957925,
43.5514946495963));
#166792=CARTESIAN_POINT('Ctrl Pts',(-8.10192317652025,0.615246620684689,
43.5592276911173));
#166793=CARTESIAN_POINT('Ctrl Pts',(-8.11690067184377,0.418014303743525,
43.5669599601131));
#166794=CARTESIAN_POINT('Ctrl Pts',(-8.12467253855411,0.220224145668624,
43.5746922291089));
#166795=CARTESIAN_POINT('Ctrl Pts',(-8.12521898577066,0.0224498501542118,
43.5824244981047));
#166796=CARTESIAN_POINT('Ctrl Pts',(-8.12576564318059,-0.175400520128988,
43.5901597413524));
#166797=CARTESIAN_POINT('Ctrl Pts',(-8.11908132728276,-0.373234661977047,
43.5978949846001));
#166798=CARTESIAN_POINT('Ctrl Pts',(-8.10519839534709,-0.570479214838729,
43.6056302278478));
#166799=CARTESIAN_POINT('Ctrl Pts',(-8.09357766856049,-0.735583032214666,
43.6121050235773));
#166800=CARTESIAN_POINT('Ctrl Pts',(-8.0769141260109,-0.900273666263304,
43.6185798193067));
#166801=CARTESIAN_POINT('Ctrl Pts',(-8.05525464508299,-1.06421810047043,
43.6250546150362));
#166802=CARTESIAN_POINT('Ctrl Pts',(-8.02710789116816,-1.27726584896878,
43.6334686893463));
#166803=CARTESIAN_POINT('Ctrl Pts',(-7.9905100417965,-1.48915602392358,
43.6418827636564));
#166804=CARTESIAN_POINT('Ctrl Pts',(-7.94558428195602,-1.69922864289459,
43.6502968379666));
#166805=CARTESIAN_POINT('Ctrl Pts',(-7.90064597559849,-1.909359929314,43.658713262094));
#166806=CARTESIAN_POINT('Ctrl Pts',(-7.84737517101555,-2.11767238822419,
43.6671296862214));
#166807=CARTESIAN_POINT('Ctrl Pts',(-7.78594586514241,-2.32351770976074,
43.6755461103488));
#166808=CARTESIAN_POINT('Ctrl Pts',(-7.72450132523735,-2.52941407947623,
43.6839646216896));
#166809=CARTESIAN_POINT('Ctrl Pts',(-7.65489432029978,-2.73284183743178,
43.6923831330305));
#166810=CARTESIAN_POINT('Ctrl Pts',(-7.57734859494423,-2.93316822449663,
43.7008016443713));
#166811=CARTESIAN_POINT('Ctrl Pts',(-7.49977308459219,-3.13357155610882,
43.709223389228));
#166812=CARTESIAN_POINT('Ctrl Pts',(-7.41425285454955,-3.33087088965249,
43.7176451340847));
#166813=CARTESIAN_POINT('Ctrl Pts',(-7.32106018105627,-3.52445249476458,
43.7260668789414));
#166814=CARTESIAN_POINT('Ctrl Pts',(-7.22785740571858,-3.71805508362124,
43.7344895366934));
#166815=CARTESIAN_POINT('Ctrl Pts',(-7.12698064362,-3.90793890291983,43.7429121944454));
#166816=CARTESIAN_POINT('Ctrl Pts',(-7.01874887651428,-4.09351337739717,
43.7513348521975));
#166817=CARTESIAN_POINT('Ctrl Pts',(-6.91049652679755,-4.27912314287384,
43.7597591117));
#166818=CARTESIAN_POINT('Ctrl Pts',(-6.79488651080306,-4.46042169837938,
43.7681833712025));
#166819=CARTESIAN_POINT('Ctrl Pts',(-6.67228270029433,-4.6368449542607,
43.776607630705));
#166820=CARTESIAN_POINT('Ctrl Pts',(-6.63776893946875,-4.68650923494083,
43.778979113911));
#166821=CARTESIAN_POINT('Ctrl Pts',(-6.60270121405478,-4.73578734269762,
43.7813505971169));
#166822=CARTESIAN_POINT('Ctrl Pts',(-6.56708825637221,-4.78466711438927,
43.7837220803228));
#166823=CARTESIAN_POINT('Ctrl Pts',(-6.4405787570321,-4.95830490936511,
43.7921464059783));
#166824=CARTESIAN_POINT('Ctrl Pts',(-6.30717262978249,-5.12693156576806,
43.8005707316338));
#166825=CARTESIAN_POINT('Ctrl Pts',(-6.16728380939353,-5.29001871233859,
43.8089950572893));
#166826=CARTESIAN_POINT('Ctrl Pts',(-6.02741916346917,-5.45307767549574,
43.8174179271204));
#166827=CARTESIAN_POINT('Ctrl Pts',(-5.88107423370648,-5.61059884060153,
43.8258407969515));
#166828=CARTESIAN_POINT('Ctrl Pts',(-5.72870267265477,-5.76208757750332,
43.8342636667826));
#166829=CARTESIAN_POINT('Ctrl Pts',(-5.57636224899295,-5.91354535742186,
43.8426848153857));
#166830=CARTESIAN_POINT('Ctrl Pts',(-5.41799784042819,-6.05897298485688,
43.8511059639889));
#166831=CARTESIAN_POINT('Ctrl Pts',(-5.25410009696062,-6.19791253032974,
43.8595271125921));
#166832=CARTESIAN_POINT('Ctrl Pts',(-5.09024833777183,-6.3368130939676,
43.8679458984999));
#166833=CARTESIAN_POINT('Ctrl Pts',(-4.92086654555653,-6.46922904080733,
43.8763646844076));
#166834=CARTESIAN_POINT('Ctrl Pts',(-4.7464793583057,-6.59474194064316,
43.8847834703154));
#166835=CARTESIAN_POINT('Ctrl Pts',(-4.57214088504883,-6.72021977921823,
43.8931999044868));
#166836=CARTESIAN_POINT('Ctrl Pts',(-4.39280002251156,-6.83879826683661,
43.9016163386583));
#166837=CARTESIAN_POINT('Ctrl Pts',(-4.20901230268642,-6.95010093439904,
43.9100327728297));
#166838=CARTESIAN_POINT('Ctrl Pts',(-4.02529128734135,-7.0613632054291,
43.9184461523147));
#166839=CARTESIAN_POINT('Ctrl Pts',(-3.83712686331025,-7.1653547932383,
43.9268595317996));
#166840=CARTESIAN_POINT('Ctrl Pts',(-3.64510204044308,-7.26174350120256,
43.9352729112845));
#166841=CARTESIAN_POINT('Ctrl Pts',(-3.59095929284808,-7.28892097445001,
43.9376451227261));
#166842=CARTESIAN_POINT('Ctrl Pts',(-3.53650980442697,-7.31549429527996,
43.9400173341677));
#166843=CARTESIAN_POINT('Ctrl Pts',(-3.48176700930949,-7.34145667121887,
43.9423895456093));
#166844=CARTESIAN_POINT('Ctrl Pts',(-3.3032645331394,-7.42611344445103,
43.950124730037));
#166845=CARTESIAN_POINT('Ctrl Pts',(-3.12156246520276,-7.50430829972414,
43.9578599144647));
#166846=CARTESIAN_POINT('Ctrl Pts',(-2.93717868219316,-7.57579493857708,
43.9655950988925));
#166847=CARTESIAN_POINT('Ctrl Pts',(-2.7528519152153,-7.647259471991,43.9733278914096));
#166848=CARTESIAN_POINT('Ctrl Pts',(-2.56584541356301,-7.71201979231342,
43.9810606839267));
#166849=CARTESIAN_POINT('Ctrl Pts',(-2.37669761634251,-7.76987747670269,
43.9887934764439));
#166850=CARTESIAN_POINT('Ctrl Pts',(-2.18757470220896,-7.82772754970123,
43.9965252516837));
#166851=CARTESIAN_POINT('Ctrl Pts',(-1.99631139158246,-7.87867669292311,
44.0042570269237));
#166852=CARTESIAN_POINT('Ctrl Pts',(-1.80346201542789,-7.92257611647933,
44.0119888021636));
#166853=CARTESIAN_POINT('Ctrl Pts',(-1.61054363246769,-7.96649124845551,
44.0197233440451));
#166854=CARTESIAN_POINT('Ctrl Pts',(-1.41603839399175,-8.00335153823512,
44.0274578859266));
#166855=CARTESIAN_POINT('Ctrl Pts',(-1.22051223209202,-8.0330590346277,
44.0351924278081));
#166856=CARTESIAN_POINT('Ctrl Pts',(-1.02495304799253,-8.06277154828688,
44.042928275968));
#166857=CARTESIAN_POINT('Ctrl Pts',(-0.828372947453864,-8.08532881595842,
44.0506641241278));
#166858=CARTESIAN_POINT('Ctrl Pts',(-0.631343921841026,-8.10068468802819,
44.0583999722877));
#166859=CARTESIAN_POINT('Ctrl Pts',(-0.434153678079574,-8.11605312497391,
44.0661421502718));
#166860=CARTESIAN_POINT('Ctrl Pts',(-0.23651412839142,-8.12420837346987,
44.073884328256));
#166861=CARTESIAN_POINT('Ctrl Pts',(-0.038999148654981,-8.12515640642715,
44.0816265062402));
#166862=CARTESIAN_POINT('Ctrl Pts',(0.126234964240147,-8.12594949758864,
44.0881033411253));
#166863=CARTESIAN_POINT('Ctrl Pts',(0.291381787375085,-8.12169961560909,
44.0945801760104));
#166864=CARTESIAN_POINT('Ctrl Pts',(0.456107788770162,-8.11243818143,44.1010570108955));
#166865=CARTESIAN_POINT('Ctrl Pts',(0.695128841881753,-8.09899963662188,
44.1104550408481));
#166866=CARTESIAN_POINT('Ctrl Pts',(0.933399685667861,-8.07500195327902,
44.1198530708006));
#166867=CARTESIAN_POINT('Ctrl Pts',(1.17008024090096,-8.04055966909973,
44.1292511007531));
#166868=CARTESIAN_POINT('Ctrl Pts',(1.4070975736774,-8.00606837629849,44.1386625033523));
#166869=CARTESIAN_POINT('Ctrl Pts',(1.64252005459376,-7.96110275970635,
44.1480739059515));
#166870=CARTESIAN_POINT('Ctrl Pts',(1.87551474980376,-7.90582898789042,
44.1574853085507));
#166871=CARTESIAN_POINT('Ctrl Pts',(2.10815863109604,-7.8506384403231,44.1668825406513));
#166872=CARTESIAN_POINT('Ctrl Pts',(2.33838199799642,-7.78517076979389,
44.1762797727518));
#166873=CARTESIAN_POINT('Ctrl Pts',(2.56536686952964,-7.70964204014815,
44.1856770048524));
#166874=CARTESIAN_POINT('Ctrl Pts',(2.79177919885259,-7.6343038226961,44.1950505335581));
#166875=CARTESIAN_POINT('Ctrl Pts',(3.01496930701531,-7.54895522985642,
44.2044240622637));
#166876=CARTESIAN_POINT('Ctrl Pts',(3.23413710097516,-7.45386106488416,
44.2137975909694));
#166877=CARTESIAN_POINT('Ctrl Pts',(3.45188162845257,-7.35938443743981,
44.2231102483719));
#166878=CARTESIAN_POINT('Ctrl Pts',(3.66565586421285,-7.25528839971713,
44.2324229057745));
#166879=CARTESIAN_POINT('Ctrl Pts',(3.87468744798139,-7.14188243693184,
44.241735563177));
#166880=CARTESIAN_POINT('Ctrl Pts',(4.0092802862809,-7.06886174725337,44.247731867512));
#166881=CARTESIAN_POINT('Ctrl Pts',(4.14190711030131,-6.99198224877317,
44.2537281718471));
#166882=CARTESIAN_POINT('Ctrl Pts',(4.27236462532949,-6.91133764699231,
44.2597244761822));
#166883=CARTESIAN_POINT('Ctrl Pts',(4.43700901099099,-6.80955983132367,
44.2672921340766));
#166884=CARTESIAN_POINT('Ctrl Pts',(4.59813116368294,-6.7018227134163,44.2748597919709));
#166885=CARTESIAN_POINT('Ctrl Pts',(4.75525822826502,-6.58841458508933,
44.2824274498653));
#166886=CARTESIAN_POINT('Ctrl Pts',(4.91234178719294,-6.4750378574305,44.2899930124115));
#166887=CARTESIAN_POINT('Ctrl Pts',(5.06543216120311,-6.35599345862215,
44.2975585749578));
#166888=CARTESIAN_POINT('Ctrl Pts',(5.21408537593068,-6.23161305401786,
44.305124137504));
#166889=CARTESIAN_POINT('Ctrl Pts',(5.36272556724018,-6.10724354630546,
44.3126890372359));
#166890=CARTESIAN_POINT('Ctrl Pts',(5.5069290915758,-5.9775391998602,44.3202539369678));
#166891=CARTESIAN_POINT('Ctrl Pts',(5.64628503765839,-5.84287196813476,
44.3278188366996));
#166892=CARTESIAN_POINT('Ctrl Pts',(5.78570937880555,-5.7081386425377,44.335387449239));
#166893=CARTESIAN_POINT('Ctrl Pts',(5.92028112157277,-5.56843781904027,
44.3429560617784));
#166894=CARTESIAN_POINT('Ctrl Pts',(6.04962583290827,-5.42417872532874,
44.3505246743178));
#166895=CARTESIAN_POINT('Ctrl Pts',(6.17899930824242,-5.27988755092111,
44.3580949699841));
#166896=CARTESIAN_POINT('Ctrl Pts',(6.30314319972982,-5.13103636841071,
44.3656652656504));
#166897=CARTESIAN_POINT('Ctrl Pts',(6.42172357771468,-4.97806728097595,
44.3732355613167));
#166898=CARTESIAN_POINT('Ctrl Pts',(6.54042411146642,-4.82494319219679,
44.3808135278531));
#166899=CARTESIAN_POINT('Ctrl Pts',(6.65354965238771,-4.6676931595859,44.3883914943895));
#166900=CARTESIAN_POINT('Ctrl Pts',(6.76080929604574,-4.5067887930323,44.3959694609259));
#166901=CARTESIAN_POINT('Ctrl Pts',(6.86659964940591,-4.34808856604691,
44.4034436211068));
#166902=CARTESIAN_POINT('Ctrl Pts',(6.9666836684079,-4.1858338068307,44.4109177812876));
#166903=CARTESIAN_POINT('Ctrl Pts',(7.06082668873177,-4.02049922698577,
44.4183919414685));
#166904=CARTESIAN_POINT('Ctrl Pts',(7.16778999590138,-3.8326495766466,44.4268839240765));
#166905=CARTESIAN_POINT('Ctrl Pts',(7.26728547124287,-3.64047231742024,
44.4353759066845));
#166906=CARTESIAN_POINT('Ctrl Pts',(7.35898571646831,-3.44456336671506,
44.4438678892926));
#166907=CARTESIAN_POINT('Ctrl Pts',(7.45061782538993,-3.24879998281566,
44.4523535620777));
#166908=CARTESIAN_POINT('Ctrl Pts',(7.53446616010904,-3.04931067214259,
44.4608392348629));
#166909=CARTESIAN_POINT('Ctrl Pts',(7.61024988985641,-2.84671462855703,
44.469324907648));
#166910=CARTESIAN_POINT('Ctrl Pts',(7.68597193347051,-2.6442834932781,44.4778036732996));
#166911=CARTESIAN_POINT('Ctrl Pts',(7.7536423872849,-2.43875091019721,44.4862824389512));
#166912=CARTESIAN_POINT('Ctrl Pts',(7.81302862644311,-2.23075575643781,
44.4947612046028));
#166913=CARTESIAN_POINT('Ctrl Pts',(7.87233923567211,-2.02302548994825,
44.5032291723245));
#166914=CARTESIAN_POINT('Ctrl Pts',(7.92338662845627,-1.8128391587275,44.5116971400462));
#166915=CARTESIAN_POINT('Ctrl Pts',(7.9659879565569,-1.60085084829613,44.5201651077679));
#166916=CARTESIAN_POINT('Ctrl Pts',(8.0085517595314,-1.38904926650542,44.5286256165307));
#166917=CARTESIAN_POINT('Ctrl Pts',(8.04268429491224,-1.17544912102911,
44.5370861252935));
#166918=CARTESIAN_POINT('Ctrl Pts',(8.06825326753697,-0.960716801861529,
44.5455466340563));
#166919=CARTESIAN_POINT('Ctrl Pts',(8.09378829972018,-0.746269519946942,
44.5539959122778));
#166920=CARTESIAN_POINT('Ctrl Pts',(8.11078243346433,-0.530693315926462,
44.5624451904993));
#166921=CARTESIAN_POINT('Ctrl Pts',(8.1191548345446,-0.314662255745863,
44.5708944687207));
#166922=CARTESIAN_POINT('Ctrl Pts',(8.12325136298361,-0.208960513407529,
44.5750286123423));
#166923=CARTESIAN_POINT('Ctrl Pts',(8.12528459051782,-0.103150010145808,
44.5791627559639));
#166924=CARTESIAN_POINT('Ctrl Pts',(8.12524955482466,0.00268966942621325,
44.5832968995855));
#166925=CARTESIAN_POINT('',(8.12524981409313,0.00169347021508326,46.5833637857063));
#166926=CARTESIAN_POINT('Ctrl Pts',(8.12524955020566,0.00270358701031778,
44.5832974432124));
#166927=CARTESIAN_POINT('Ctrl Pts',(8.1251775121146,0.219203912218492,44.5917540392692));
#166928=CARTESIAN_POINT('Ctrl Pts',(8.11644813158616,0.435525939744223,
44.600210635326));
#166929=CARTESIAN_POINT('Ctrl Pts',(8.0991293976781,0.65099198318127,44.6086672313829));
#166930=CARTESIAN_POINT('Ctrl Pts',(8.08178443997324,0.866784282438916,
44.6171366323051));
#166931=CARTESIAN_POINT('Ctrl Pts',(8.0558241595595,1.08171775676946,44.6256060332273));
#166932=CARTESIAN_POINT('Ctrl Pts',(8.02136810729963,1.2951220983739,44.6340754341495));
#166933=CARTESIAN_POINT('Ctrl Pts',(7.98683179491984,1.50902353285235,44.6425645632498));
#166934=CARTESIAN_POINT('Ctrl Pts',(7.94376015720404,1.72138845859037,44.6510536923501));
#166935=CARTESIAN_POINT('Ctrl Pts',(7.89232403806732,1.93155606717607,44.6595428214504));
#166936=CARTESIAN_POINT('Ctrl Pts',(7.84083155612169,2.14195397378895,44.6680412527913));
#166937=CARTESIAN_POINT('Ctrl Pts',(7.78095634937928,2.35014951053943,44.6765396841323));
#166938=CARTESIAN_POINT('Ctrl Pts',(7.7129190397752,2.55549749527821,44.6850381154733));
#166939=CARTESIAN_POINT('Ctrl Pts',(7.64475713806993,2.76122151982578,44.693552109414));
#166940=CARTESIAN_POINT('Ctrl Pts',(7.56840332027205,2.96408732389021,44.7020661033548));
#166941=CARTESIAN_POINT('Ctrl Pts',(7.48412725595363,3.16346752459892,44.7105800972955));
#166942=CARTESIAN_POINT('Ctrl Pts',(7.40115518195288,3.359762746751,44.7189623555441));
#166943=CARTESIAN_POINT('Ctrl Pts',(7.31050436684576,3.55267925432863,44.7273446137927));
#166944=CARTESIAN_POINT('Ctrl Pts',(7.21247566442981,3.74164166543347,44.7357268720413));
#166945=CARTESIAN_POINT('Ctrl Pts',(7.11800573674497,3.92374409943778,44.7438048258555));
#166946=CARTESIAN_POINT('Ctrl Pts',(7.01652922040552,4.10247129525327,44.7518827796697));
#166947=CARTESIAN_POINT('Ctrl Pts',(6.90830553088348,4.27726574513027,44.7599607334839));
#166948=CARTESIAN_POINT('Ctrl Pts',(6.80021428578587,4.45184628111825,44.7680288014778));
#166949=CARTESIAN_POINT('Ctrl Pts',(6.68539249179063,4.62250339863331,44.7760968694717));
#166950=CARTESIAN_POINT('Ctrl Pts',(6.56414612554026,4.78870266408918,44.7841649374656));
#166951=CARTESIAN_POINT('Ctrl Pts',(6.44303321409428,4.95471899548157,44.7922241250084));
#166952=CARTESIAN_POINT('Ctrl Pts',(6.31551001255445,5.11628700299728,44.8002833125511));
#166953=CARTESIAN_POINT('Ctrl Pts',(6.18192692576556,5.27289930180681,44.8083425000938));
#166954=CARTESIAN_POINT('Ctrl Pts',(6.04851542357616,5.42931043548973,44.8163913357837));
#166955=CARTESIAN_POINT('Ctrl Pts',(5.90905976844119,5.5807783203165,44.8244401714735));
#166956=CARTESIAN_POINT('Ctrl Pts',(5.76395194930333,5.72682682544376,44.8324890071633));
#166957=CARTESIAN_POINT('Ctrl Pts',(5.61895389027642,5.8727648589216,44.8405317546829));
#166958=CARTESIAN_POINT('Ctrl Pts',(5.4683124106001,6.01329146051201,44.8485745022026));
#166959=CARTESIAN_POINT('Ctrl Pts',(5.31245873268391,6.14796468565252,44.8566172497222));
#166960=CARTESIAN_POINT('Ctrl Pts',(5.15673200583406,6.28252821232606,44.8646534459985));
#166961=CARTESIAN_POINT('Ctrl Pts',(4.99580178793621,6.41124766756013,44.8726896422747));
#166962=CARTESIAN_POINT('Ctrl Pts',(4.8301352056564,6.53371880766066,44.880725838551));
#166963=CARTESIAN_POINT('Ctrl Pts',(4.73620961368876,6.60315450298674,44.8852820048099));
#166964=CARTESIAN_POINT('Ctrl Pts',(4.64076222582698,6.67058243382526,44.8898381710689));
#166965=CARTESIAN_POINT('Ctrl Pts',(4.54388303022122,6.73593457288353,44.8943943373278));
#166966=CARTESIAN_POINT('Ctrl Pts',(4.37300026917792,6.85120755685635,44.9024308436719));
#166967=CARTESIAN_POINT('Ctrl Pts',(4.19779623704759,6.9599286625938,44.910467350016));
#166968=CARTESIAN_POINT('Ctrl Pts',(4.01880742894209,7.06178974563672,44.9185038563602));
#166969=CARTESIAN_POINT('Ctrl Pts',(3.83971049624867,7.16371236150811,44.9265452174432));
#166970=CARTESIAN_POINT('Ctrl Pts',(3.65682450071894,7.25876653088662,44.9345865785263));
#166971=CARTESIAN_POINT('Ctrl Pts',(3.47070955099071,7.34669060020645,44.9426279396094));
#166972=CARTESIAN_POINT('Ctrl Pts',(3.2844594154123,7.43467853376761,44.9506751415893));
#166973=CARTESIAN_POINT('Ctrl Pts',(3.09497593164756,7.51552589990583,44.9587223435693));
#166974=CARTESIAN_POINT('Ctrl Pts',(2.90283869828506,7.58901937368977,44.9667695455493));
#166975=CARTESIAN_POINT('Ctrl Pts',(2.71041827043903,7.66262117081108,44.9748286084433));
#166976=CARTESIAN_POINT('Ctrl Pts',(2.51533657074099,7.72884729907743,44.9828876713373));
#166977=CARTESIAN_POINT('Ctrl Pts',(2.3181895379757,7.78753393755173,44.9909467342313));
#166978=CARTESIAN_POINT('Ctrl Pts',(2.12088294562527,7.8462680736503,44.999012319672));
#166979=CARTESIAN_POINT('Ctrl Pts',(1.92150798975258,7.89745046444227,45.0070779051127));
#166980=CARTESIAN_POINT('Ctrl Pts',(1.72067117894991,7.94096834500876,45.0151434905535));
#166981=CARTESIAN_POINT('Ctrl Pts',(1.51951900875534,7.98455455852824,45.0232217407946));
#166982=CARTESIAN_POINT('Ctrl Pts',(1.31690070611728,8.02045215062923,45.0312999910357));
#166983=CARTESIAN_POINT('Ctrl Pts',(1.11343004629675,8.04859994623311,45.0393782412769));
#166984=CARTESIAN_POINT('Ctrl Pts',(0.998545297293156,8.06449291299209,
45.0439394283893));
#166985=CARTESIAN_POINT('Ctrl Pts',(0.883388868159684,8.07791617415651,
45.0485006155018));
#166986=CARTESIAN_POINT('Ctrl Pts',(0.768071277691702,8.08886605618396,
45.0530618026143));
#166987=CARTESIAN_POINT('Ctrl Pts',(0.563633125916835,8.10827830400114,
45.0611479988259));
#166988=CARTESIAN_POINT('Ctrl Pts',(0.358290620238147,8.11995173760702,
45.0692341950375));
#166989=CARTESIAN_POINT('Ctrl Pts',(0.152655273641481,8.12381584785927,
45.0773203912491));
#166990=CARTESIAN_POINT('Ctrl Pts',(-0.0527966563140229,8.12767651151474,
45.0853993749704));
#166991=CARTESIAN_POINT('Ctrl Pts',(-0.25854059115977,8.12374173451219,
45.0934783586916));
#166992=CARTESIAN_POINT('Ctrl Pts',(-0.463960667191387,8.1119928539046,
45.1015573424129));
#166993=CARTESIAN_POINT('Ctrl Pts',(-0.669225569659059,8.10025284835787,
45.1096302232998));
#166994=CARTESIAN_POINT('Ctrl Pts',(-0.874166786002571,8.08071052779534,
45.1177031041867));
#166995=CARTESIAN_POINT('Ctrl Pts',(-1.07816859310736,8.05339928522961,
45.1257759850737));
#166996=CARTESIAN_POINT('Ctrl Pts',(-1.28204411402979,8.02610494953647,
45.1338438684886));
#166997=CARTESIAN_POINT('Ctrl Pts',(-1.48498107227109,7.99105132484738,
45.1419117519036));
#166998=CARTESIAN_POINT('Ctrl Pts',(-1.68636837788461,7.94832367588102,
45.1499796353186));
#166999=CARTESIAN_POINT('Ctrl Pts',(-1.88765844149699,7.90561665841414,
45.1580436230703));
#167000=CARTESIAN_POINT('Ctrl Pts',(-2.08740003554838,7.85524307286104,
45.166107610822));
#167001=CARTESIAN_POINT('Ctrl Pts',(-2.28499116249876,7.79733947893783,
45.1741715985737));
#167002=CARTESIAN_POINT('Ctrl Pts',(-2.48532807333227,7.73863123979891,
45.1823476458493));
#167003=CARTESIAN_POINT('Ctrl Pts',(-2.68345398019448,7.67218221586229,
45.1905236931249));
#167004=CARTESIAN_POINT('Ctrl Pts',(-2.87875497010913,7.59818776976273,
45.1986997404004));
#167005=CARTESIAN_POINT('Ctrl Pts',(-3.0712879338831,7.52524205649939,45.2067599075025));
#167006=CARTESIAN_POINT('Ctrl Pts',(-3.26107522538182,7.44496351391998,
45.2148200746046));
#167007=CARTESIAN_POINT('Ctrl Pts',(-3.44754624276917,7.35758876714839,
45.2228802417068));
#167008=CARTESIAN_POINT('Ctrl Pts',(-3.6340082503288,7.27021824211284,45.2309400193611));
#167009=CARTESIAN_POINT('Ctrl Pts',(-3.81715401658874,7.17575233124587,
45.2389997970155));
#167010=CARTESIAN_POINT('Ctrl Pts',(-3.99643489526495,7.07447494096973,
45.2470595746698));
#167011=CARTESIAN_POINT('Ctrl Pts',(-4.17572930930138,6.97318990444615,
45.2551199608219));
#167012=CARTESIAN_POINT('Ctrl Pts',(-4.35115797826423,6.86509251914933,
45.2631803469739));
#167013=CARTESIAN_POINT('Ctrl Pts',(-4.5221982233869,6.75051189102696,45.2712407331259));
#167014=CARTESIAN_POINT('Ctrl Pts',(-4.6975379055891,6.63305105070194,45.279503733131));
#167015=CARTESIAN_POINT('Ctrl Pts',(-4.86826535365477,6.508776945701,45.2877667331361));
#167016=CARTESIAN_POINT('Ctrl Pts',(-5.03385030828329,6.37809051647091,
45.2960297331412));
#167017=CARTESIAN_POINT('Ctrl Pts',(-5.19550784286892,6.25050376802187,
45.3040967475152));
#167018=CARTESIAN_POINT('Ctrl Pts',(-5.35226382801139,6.11680564990189,
45.3121637618892));
#167019=CARTESIAN_POINT('Ctrl Pts',(-5.50365920692788,5.97740938003229,
45.3202307762632));
#167020=CARTESIAN_POINT('Ctrl Pts',(-5.6605717420389,5.83293322595942,45.3285917690839));
#167021=CARTESIAN_POINT('Ctrl Pts',(-5.8117253570236,5.68233607149676,45.3369527619045));
#167022=CARTESIAN_POINT('Ctrl Pts',(-5.9566513585496,5.52611908622943,45.3453137547252));
#167023=CARTESIAN_POINT('Ctrl Pts',(-6.10157736007554,5.36990210096216,
45.3536747475458));
#167024=CARTESIAN_POINT('Ctrl Pts',(-6.24027552102279,5.20806558687446,
45.3620357403665));
#167025=CARTESIAN_POINT('Ctrl Pts',(-6.3723239016619,5.04114824765236,45.3703967331871));
#167026=CARTESIAN_POINT('Ctrl Pts',(-6.49201017224205,4.88985738191084,
45.3779749862805));
#167027=CARTESIAN_POINT('Ctrl Pts',(-6.60647314287351,4.73408915259941,
45.3855532393739));
#167028=CARTESIAN_POINT('Ctrl Pts',(-6.7153458748783,4.57425593329178,45.3931314924672));
#167029=CARTESIAN_POINT('Ctrl Pts',(-6.82413759189688,4.41454164997315,
45.4007041063885));
#167030=CARTESIAN_POINT('Ctrl Pts',(-6.92734714018761,4.25076869588969,
45.4082767203098));
#167031=CARTESIAN_POINT('Ctrl Pts',(-7.02464742836837,4.08338291978816,
45.4158493342311));
#167032=CARTESIAN_POINT('Ctrl Pts',(-7.12189378992831,3.91608991370249,
45.4234177511917));
#167033=CARTESIAN_POINT('Ctrl Pts',(-7.21323722427045,3.74518838659905,
45.4309861681524));
#167034=CARTESIAN_POINT('Ctrl Pts',(-7.29839365196104,3.57115354801705,
45.438554585113));
#167035=CARTESIAN_POINT('Ctrl Pts',(-7.38352950497776,3.39716075805245,
45.4461211734658));
#167036=CARTESIAN_POINT('Ctrl Pts',(-7.46248115814338,3.22003648961031,
45.4536877618186));
#167037=CARTESIAN_POINT('Ctrl Pts',(-7.53501018718415,3.04028107936274,
45.4612543501714));
#167038=CARTESIAN_POINT('Ctrl Pts',(-7.60752634987313,2.86055755698647,
45.4688195962426));
#167039=CARTESIAN_POINT('Ctrl Pts',(-7.67362202155401,2.67820416402399,
45.4763848423137));
#167040=CARTESIAN_POINT('Ctrl Pts',(-7.73310680513213,2.4937415068365,45.4839500883848));
#167041=CARTESIAN_POINT('Ctrl Pts',(-7.79261227411411,2.30921470409225,
45.4915179652156));
#167042=CARTESIAN_POINT('Ctrl Pts',(-7.84550214617388,2.1225775211719,45.4990858420464));
#167043=CARTESIAN_POINT('Ctrl Pts',(-7.89163568911035,1.9343664887657,45.5066537188772));
#167044=CARTESIAN_POINT('Ctrl Pts',(-7.93717355244986,1.74858565063447,
45.5141238787426));
#167045=CARTESIAN_POINT('Ctrl Pts',(-7.97612847971321,1.5612717107185,45.521594038608));
#167046=CARTESIAN_POINT('Ctrl Pts',(-8.00841401837734,1.37295028051175,
45.5290641984733));
#167047=CARTESIAN_POINT('Ctrl Pts',(-8.04863283525662,1.13835406718165,
45.5383699435256));
#167048=CARTESIAN_POINT('Ctrl Pts',(-8.07848435405988,0.902309964408368,
45.5476756885779));
#167049=CARTESIAN_POINT('Ctrl Pts',(-8.09793765476928,0.665652538468628,
45.5569814336302));
#167050=CARTESIAN_POINT('Ctrl Pts',(-8.11749538044108,0.427724739795072,
45.5663371317518));
#167051=CARTESIAN_POINT('Ctrl Pts',(-8.12654300334931,0.189177065574376,
45.5756928298733));
#167052=CARTESIAN_POINT('Ctrl Pts',(-8.12510134696751,-0.0491494049483041,
45.5850485279948));
#167053=CARTESIAN_POINT('Ctrl Pts',(-8.12365269291446,-0.288632690862096,
45.594449637839));
#167054=CARTESIAN_POINT('Ctrl Pts',(-8.1116127085664,-0.527892578407454,
45.6038507476832));
#167055=CARTESIAN_POINT('Ctrl Pts',(-8.08905456527946,-0.766083417410555,
45.6132518575274));
#167056=CARTESIAN_POINT('Ctrl Pts',(-8.06647200674089,-1.00453205641074,
45.6226631424317));
#167057=CARTESIAN_POINT('Ctrl Pts',(-8.03334853306665,-1.24190929656614,
45.6320744273359));
#167058=CARTESIAN_POINT('Ctrl Pts',(-7.98980916896147,-1.47737503907411,
45.6414857122402));
#167059=CARTESIAN_POINT('Ctrl Pts',(-7.94632085025944,-1.71256472234232,
45.6508859633858));
#167060=CARTESIAN_POINT('Ctrl Pts',(-7.89244106074854,-1.9458473523388,
45.6602862145315));
#167061=CARTESIAN_POINT('Ctrl Pts',(-7.82834556146667,-2.17639457193891,
45.6696864656771));
#167062=CARTESIAN_POINT('Ctrl Pts',(-7.78733190616315,-2.32391794412263,
45.6757015317048));
#167063=CARTESIAN_POINT('Ctrl Pts',(-7.74213644666728,-2.470321477707,45.6817165977324));
#167064=CARTESIAN_POINT('Ctrl Pts',(-7.69281625609412,-2.61539014536531,
45.68773166376));
#167065=CARTESIAN_POINT('Ctrl Pts',(-7.62933277835497,-2.80211820596099,
45.6954740772793));
#167066=CARTESIAN_POINT('Ctrl Pts',(-7.55898263820285,-2.98672135988384,
45.7032164907985));
#167067=CARTESIAN_POINT('Ctrl Pts',(-7.4819335647481,-3.16865234684964,
45.7109589043177));
#167068=CARTESIAN_POINT('Ctrl Pts',(-7.40493248768656,-3.3504700030407,
45.7186964948338));
#167069=CARTESIAN_POINT('Ctrl Pts',(-7.32124092339205,-3.52961848270866,
45.7264340853499));
#167070=CARTESIAN_POINT('Ctrl Pts',(-7.23107587985975,-3.7055673225851,
45.734171675866));
#167071=CARTESIAN_POINT('Ctrl Pts',(-7.14095097913265,-3.88143782744693,
45.7419058214928));
#167072=CARTESIAN_POINT('Ctrl Pts',(-7.04435849994866,-4.05411121590283,
45.7496399671197));
#167073=CARTESIAN_POINT('Ctrl Pts',(-6.94156292139606,-4.22307847083137,
45.7573741127465));
#167074=CARTESIAN_POINT('Ctrl Pts',(-6.83878050738632,-4.39202408692386,
45.7651072678979));
#167075=CARTESIAN_POINT('Ctrl Pts',(-6.72979675326218,-4.55726420926014,
45.7728404230494));
#167076=CARTESIAN_POINT('Ctrl Pts',(-6.61492148497391,-4.71831551616999,
45.7805735782008));
#167077=CARTESIAN_POINT('Ctrl Pts',(-6.50005769781426,-4.87935072691924,
45.7883059604674));
#167078=CARTESIAN_POINT('Ctrl Pts',(-6.37930377750725,-5.036197670542,45.7960383427341));
#167079=CARTESIAN_POINT('Ctrl Pts',(-6.25301209286992,-5.18840315790153,
45.8037707250007));
#167080=CARTESIAN_POINT('Ctrl Pts',(-6.12667184686641,-5.34066717093857,
45.8115060805039));
#167081=CARTESIAN_POINT('Ctrl Pts',(-5.99478980803626,-5.48828588977686,
45.819241436007));
#167082=CARTESIAN_POINT('Ctrl Pts',(-5.85775816550998,-5.63083979854702,
45.8269767915102));
#167083=CARTESIAN_POINT('Ctrl Pts',(-5.74306941318777,-5.7501504164021,
45.8334509040222));
#167084=CARTESIAN_POINT('Ctrl Pts',(-5.62477420040151,-5.86591373289273,
45.8399250165342));
#167085=CARTESIAN_POINT('Ctrl Pts',(-5.50312178915066,-5.97790415917445,
45.8463991290463));
#167086=CARTESIAN_POINT('Ctrl Pts',(-5.34502286193654,-6.12344641412314,
45.854812856586));
#167087=CARTESIAN_POINT('Ctrl Pts',(-5.18117711555769,-6.26268603461247,
45.8632265841257));
#167088=CARTESIAN_POINT('Ctrl Pts',(-5.01210191567926,-6.39519522370852,
45.8716403116655));
#167089=CARTESIAN_POINT('Ctrl Pts',(-4.84297956428164,-6.52774136683199,
45.880056385617));
#167090=CARTESIAN_POINT('Ctrl Pts',(-4.66862505583531,-6.65355316859082,
45.8884724595685));
#167091=CARTESIAN_POINT('Ctrl Pts',(-4.48958729244214,-6.77224434778029,
45.89688853352));
#167092=CARTESIAN_POINT('Ctrl Pts',(-4.31050515898738,-6.89096494162972,
45.9053066931863));
#167093=CARTESIAN_POINT('Ctrl Pts',(-4.12673767354954,-7.00256124405006,
45.9137248528526));
#167094=CARTESIAN_POINT('Ctrl Pts',(-3.93886197256506,-7.10669078570194,
45.922143012519));
#167095=CARTESIAN_POINT('Ctrl Pts',(-3.75091406528485,-7.21086034747584,
45.9305644075378));
#167096=CARTESIAN_POINT('Ctrl Pts',(-3.55885501763653,-7.30755728468961,
45.9389858025567));
#167097=CARTESIAN_POINT('Ctrl Pts',(-3.3632870383451,-7.3964848313371,45.9474071975756));
#167098=CARTESIAN_POINT('Ctrl Pts',(-3.16769780320298,-7.48542204332276,
45.9558295078972));
#167099=CARTESIAN_POINT('Ctrl Pts',(-2.96859911653299,-7.56658807220789,
45.9642518182189));
#167100=CARTESIAN_POINT('Ctrl Pts',(-2.76661421295655,-7.6397338539485,
45.9726741285405));
#167101=CARTESIAN_POINT('Ctrl Pts',(-2.56459073951853,-7.71289360318186,
45.9810980471375));
#167102=CARTESIAN_POINT('Ctrl Pts',(-2.35968019637371,-7.77802995587455,
45.9895219657345));
#167103=CARTESIAN_POINT('Ctrl Pts',(-2.15252331638041,-7.83494294394916,
45.9979458843315));
#167104=CARTESIAN_POINT('Ctrl Pts',(-2.09415364553419,-7.85097906295663,
46.000319454332));
#167105=CARTESIAN_POINT('Ctrl Pts',(-2.03560572557095,-7.86636261812646,
46.0026930243325));
#167106=CARTESIAN_POINT('Ctrl Pts',(-1.97689409283714,-7.88108985535666,
46.0050665943329));
#167107=CARTESIAN_POINT('Ctrl Pts',(-1.76850020764732,-7.93336341753856,
46.0134914575353));
#167108=CARTESIAN_POINT('Ctrl Pts',(-1.55802131713765,-7.97736981620701,
46.0219163207376));
#167109=CARTESIAN_POINT('Ctrl Pts',(-1.34611384576586,-8.01296855583107,
46.0303411839399));
#167110=CARTESIAN_POINT('Ctrl Pts',(-1.13424294864029,-8.04856115127786,
46.0387645930499));
#167111=CARTESIAN_POINT('Ctrl Pts',(-0.92094422318279,-8.07574894233483,
46.0471880021599));
#167112=CARTESIAN_POINT('Ctrl Pts',(-0.706882971391528,-8.09444278670599,
46.05561141127));
#167113=CARTESIAN_POINT('Ctrl Pts',(-0.492865491282712,-8.11313280852164,
46.0640330979441));
#167114=CARTESIAN_POINT('Ctrl Pts',(-0.278086058892827,-8.12333232910829,
46.0724547846182));
#167115=CARTESIAN_POINT('Ctrl Pts',(-0.0632148695584683,-8.12500408878461,
46.0808764712923));
#167116=CARTESIAN_POINT('Ctrl Pts',(0.151595840548115,-8.12667537791515,
46.0892957875364));
#167117=CARTESIAN_POINT('Ctrl Pts',(0.366497992376845,-8.11982369810707,
46.0977151037805));
#167118=CARTESIAN_POINT('Ctrl Pts',(0.580820601175361,-8.10446389292656,
46.1061344200247));
#167119=CARTESIAN_POINT('Ctrl Pts',(0.795083174252925,-8.08910839031115,
46.1145513778628));
#167120=CARTESIAN_POINT('Ctrl Pts',(1.00876626547239,-8.06524953964482,
46.122968335701));
#167121=CARTESIAN_POINT('Ctrl Pts',(1.22120205190785,-8.03295419574368,
46.1313852935392));
#167122=CARTESIAN_POINT('Ctrl Pts',(1.43356039372482,-8.00067062528538,
46.1397991829297));
#167123=CARTESIAN_POINT('Ctrl Pts',(1.64467207818713,-7.95995674306305,
46.1482130723202));
#167124=CARTESIAN_POINT('Ctrl Pts',(1.85387654835768,-7.91093100121278,
46.1566269617107));
#167125=CARTESIAN_POINT('Ctrl Pts',(1.91278060502567,-7.89712720880918,
46.1589959943468));
#167126=CARTESIAN_POINT('Ctrl Pts',(1.97153351604792,-7.88266478779449,
46.161365026983));
#167127=CARTESIAN_POINT('Ctrl Pts',(2.03012067429592,-7.8675471152257,46.1637340596191));
#167128=CARTESIAN_POINT('Ctrl Pts',(2.22140634855614,-7.81818827487497,
46.1714688946699));
#167129=CARTESIAN_POINT('Ctrl Pts',(2.41100894077351,-7.7618185879595,46.1792037297208));
#167130=CARTESIAN_POINT('Ctrl Pts',(2.5983730610885,-7.69858071321653,46.1869385647716));
#167131=CARTESIAN_POINT('Ctrl Pts',(2.78567924938508,-7.63536239129786,
46.1946710082514));
#167132=CARTESIAN_POINT('Ctrl Pts',(2.97074800970908,-7.56528022338878,
46.2024034517312));
#167133=CARTESIAN_POINT('Ctrl Pts',(3.15303883602665,-7.48852680178202,
46.210135895211));
#167134=CARTESIAN_POINT('Ctrl Pts',(3.33530569256797,-7.41178347263235,
46.2178673219367));
#167135=CARTESIAN_POINT('Ctrl Pts',(3.5147950174207,-7.32837077485111,46.2255987486624));
#167136=CARTESIAN_POINT('Ctrl Pts',(3.69098590082337,-7.23852959118239,
46.2333301753881));
#167137=CARTESIAN_POINT('Ctrl Pts',(3.86723987279149,-7.14865623813415,
46.2410643705012));
#167138=CARTESIAN_POINT('Ctrl Pts',(4.04019272660983,-7.05234995721369,
46.2487985656144));
#167139=CARTESIAN_POINT('Ctrl Pts',(4.20934721600092,-6.94989809836413,
46.2565327607275));
#167140=CARTESIAN_POINT('Ctrl Pts',(4.37853029070763,-6.84742892623644,
46.2642682628376));
#167141=CARTESIAN_POINT('Ctrl Pts',(4.54391342364262,-6.73881229647638,
46.2720037649477));
#167142=CARTESIAN_POINT('Ctrl Pts',(4.70502790461982,-6.62437921463203,
46.2797392670578));
#167143=CARTESIAN_POINT('Ctrl Pts',(4.86627427876861,-6.50985245441681,
46.2874811016831));
#167144=CARTESIAN_POINT('Ctrl Pts',(5.02324473536826,-6.38949993976282,
46.2952229363085));
#167145=CARTESIAN_POINT('Ctrl Pts',(5.17550251143273,-6.26369390349285,
46.3029647709338));
#167146=CARTESIAN_POINT('Ctrl Pts',(5.30292265049419,-6.15841046214334,
46.3094436889244));
#167147=CARTESIAN_POINT('Ctrl Pts',(5.42704275918094,-6.04930841442362,
46.315922606915));
#167148=CARTESIAN_POINT('Ctrl Pts',(5.54762664613986,-5.93662582259813,
46.3224015249056));
#167149=CARTESIAN_POINT('Ctrl Pts',(5.72253925643606,-5.77317441322492,
46.3317995007564));
#167150=CARTESIAN_POINT('Ctrl Pts',(5.89011105866949,-5.60209625368084,
46.3411974766071));
#167151=CARTESIAN_POINT('Ctrl Pts',(6.04977040429898,-5.42401747948586,
46.3505954524579));
#167152=CARTESIAN_POINT('Ctrl Pts',(6.2096566341494,-5.24568564610547,46.3600067833204));
#167153=CARTESIAN_POINT('Ctrl Pts',(6.36160789097475,-5.06033332628138,
46.3694181141828));
#167154=CARTESIAN_POINT('Ctrl Pts',(6.50509109190373,-4.86862171959731,
46.3788294450453));
#167155=CARTESIAN_POINT('Ctrl Pts',(6.64835793060362,-4.67719920006977,
46.3882265843055));
#167156=CARTESIAN_POINT('Ctrl Pts',(6.78318221548041,-4.47943659066402,
46.3976237235656));
#167157=CARTESIAN_POINT('Ctrl Pts',(6.90907431273789,-4.27602381934028,
46.4070208628258));
#167158=CARTESIAN_POINT('Ctrl Pts',(7.03464874314137,-4.07312432483484,
46.4163942900363));
#167159=CARTESIAN_POINT('Ctrl Pts',(7.15133596888961,-3.86460316810055,
46.4257677172467));
#167160=CARTESIAN_POINT('Ctrl Pts',(7.25869131645649,-3.65117623991217,
46.4351411444572));
#167161=CARTESIAN_POINT('Ctrl Pts',(7.36534939771774,-3.43913550634857,
46.4444536918409));
#167162=CARTESIAN_POINT('Ctrl Pts',(7.46279638797377,-3.22225254998496,
46.4537662392247));
#167163=CARTESIAN_POINT('Ctrl Pts',(7.55063753374129,-3.00125980157619,
46.4630787866084));
#167164=CARTESIAN_POINT('Ctrl Pts',(7.60720208155978,-2.85895342822822,
46.4690755211363));
#167165=CARTESIAN_POINT('Ctrl Pts',(7.65978429862617,-2.71494349904361,
46.4750722556643));
#167166=CARTESIAN_POINT('Ctrl Pts',(7.70828810210639,-2.56943225196248,
46.4810689901922));
#167167=CARTESIAN_POINT('Ctrl Pts',(7.76719546373361,-2.3927103654793,46.4883519615073));
#167168=CARTESIAN_POINT('Ctrl Pts',(7.82007886233047,-2.21378882965252,
46.4956349328224));
#167169=CARTESIAN_POINT('Ctrl Pts',(7.8667627137631,-2.03315812662141,46.5029179041375));
#167170=CARTESIAN_POINT('Ctrl Pts',(7.91343787853713,-1.85256103429721,
46.5101995202798));
#167171=CARTESIAN_POINT('Ctrl Pts',(7.95391568214445,-1.67025577966911,
46.5174811364221));
#167172=CARTESIAN_POINT('Ctrl Pts',(7.9880702730007,-1.48674842394486,46.5247627525644));
#167173=CARTESIAN_POINT('Ctrl Pts',(8.02222016869862,-1.30326629458312,
46.5320433677186));
#167174=CARTESIAN_POINT('Ctrl Pts',(8.05004851392273,-1.11858277549143,
46.5393239828727));
#167175=CARTESIAN_POINT('Ctrl Pts',(8.07148061401522,-0.933213941214172,
46.5466045980269));
#167176=CARTESIAN_POINT('Ctrl Pts',(8.09292046468911,-0.747778071217875,
46.5538878461008));
#167177=CARTESIAN_POINT('Ctrl Pts',(8.10795940919785,-0.561656777498488,
46.5611710941748));
#167178=CARTESIAN_POINT('Ctrl Pts',(8.11657465044426,-0.375371158009863,
46.5684543422488));
#167179=CARTESIAN_POINT('Ctrl Pts',(8.12238652308375,-0.249702211073741,
46.5733676475175));
#167180=CARTESIAN_POINT('Ctrl Pts',(8.12527611288442,-0.12395856849932,
46.5782809527863));
#167181=CARTESIAN_POINT('Ctrl Pts',(8.12524982216074,0.00169999318035808,
46.5831942580551));
#167182=CARTESIAN_POINT('',(8.12779981229061,-5.30458549197524E-5,48.5834001493614));
#167183=CARTESIAN_POINT('Ctrl Pts',(8.12524981409313,0.00169347021508326,
46.5833637857063));
#167184=CARTESIAN_POINT('Ctrl Pts',(8.12475676563394,2.24736674679337,46.6713392646829));
#167185=CARTESIAN_POINT('Ctrl Pts',(7.14356931219011,4.47573372637722,46.7593147436594));
#167186=CARTESIAN_POINT('Ctrl Pts',(3.83078204044914,7.50935546634369,46.9352878157772));
#167187=CARTESIAN_POINT('Ctrl Pts',(1.52412477697731,8.29110090552138,47.0232854089184));
#167188=CARTESIAN_POINT('Ctrl Pts',(-2.9510162393256,7.89663306204424,47.1992805952008));
#167189=CARTESIAN_POINT('Ctrl Pts',(-5.08535169588728,6.7234298308579,47.287278188342));
#167190=CARTESIAN_POINT('Ctrl Pts',(-7.81671694684396,3.15661951052958,
47.4632733746244));
#167191=CARTESIAN_POINT('Ctrl Pts',(-8.39290461146698,0.790229551554374,
47.5512709677656));
#167192=CARTESIAN_POINT('Ctrl Pts',(-7.60701611462498,-3.63299000730381,
47.727266154048));
#167193=CARTESIAN_POINT('Ctrl Pts',(-6.25093680401385,-5.65606750609986,
47.8152637471892));
#167194=CARTESIAN_POINT('Ctrl Pts',(-2.45807268688606,-8.06369575488301,
47.9912589334716));
#167195=CARTESIAN_POINT('Ctrl Pts',(-0.0502299510459392,-8.42987470330084,
48.0792565266128));
#167196=CARTESIAN_POINT('Ctrl Pts',(4.28689960880937,-7.25863639434595,
48.2552517128952));
#167197=CARTESIAN_POINT('Ctrl Pts',(6.1830912555711,-5.73015646266433,48.3432493060364));
#167198=CARTESIAN_POINT('Ctrl Pts',(7.81049469094434,-2.58642819611753,
48.4819294849132));
#167199=CARTESIAN_POINT('Ctrl Pts',(8.12523846244703,-1.2938062194213,48.5326120706489));
#167200=CARTESIAN_POINT('Ctrl Pts',(8.1252499996828,-7.11371931539338E-5,
48.5832946563846));
#167201=CARTESIAN_POINT('',(8.11795043021363,-0.00244482526706127,50.5832974432124));
#167202=CARTESIAN_POINT('Ctrl Pts',(8.12779981229061,-5.30458549197522E-5,
48.5834001493614));
#167203=CARTESIAN_POINT('Ctrl Pts',(8.10719593127611,2.35984343847289,48.6759604227372));
#167204=CARTESIAN_POINT('Ctrl Pts',(5.81138593698418,7.42468183755121,48.8742990063037));
#167205=CARTESIAN_POINT('Ctrl Pts',(-2.84362164243682,9.17837728242667,
49.1784159000614));
#167206=CARTESIAN_POINT('Ctrl Pts',(-8.15113057818095,3.70434890315244,
49.4428616755388));
#167207=CARTESIAN_POINT('Ctrl Pts',(-8.24488799843749,-1.87812548990129,
49.6544182959206));
#167208=CARTESIAN_POINT('Ctrl Pts',(-6.36260440029279,-5.60229600309865,
49.8130857612071));
#167209=CARTESIAN_POINT('Ctrl Pts',(-2.90807460908608,-7.94038890968604,
49.9717532264935));
#167210=CARTESIAN_POINT('Ctrl Pts',(2.64399874568358,-8.55485708321899,
50.1833098468754));
#167211=CARTESIAN_POINT('Ctrl Pts',(7.34346692161665,-5.03063998245504,
50.3871579191151));
#167212=CARTESIAN_POINT('Ctrl Pts',(8.11601312705655,-1.16362153771914,
50.5381168362592));
#167213=CARTESIAN_POINT('Ctrl Pts',(8.11226079205514,-0.00435044046600885,
50.5832974432124));
#167214=CARTESIAN_POINT('',(8.12525,1.19476911003558E-13,52.5832974432124));
#167215=CARTESIAN_POINT('Ctrl Pts',(8.12525,6.37338797166611E-14,50.5832974432124));
#167216=CARTESIAN_POINT('Ctrl Pts',(8.12524999999998,2.24624642433412,50.6712950363536));
#167217=CARTESIAN_POINT('Ctrl Pts',(7.14398562317601,4.47535249753447,50.7592926294948));
#167218=CARTESIAN_POINT('Ctrl Pts',(3.83078204044946,7.50935546634353,50.9352878157772));
#167219=CARTESIAN_POINT('Ctrl Pts',(1.52412477697767,8.29110090552131,51.0232854089184));
#167220=CARTESIAN_POINT('Ctrl Pts',(-2.95101623932526,7.89663306204436,
51.1992805952008));
#167221=CARTESIAN_POINT('Ctrl Pts',(-5.08535169588699,6.72342983085812,
51.287278188342));
#167222=CARTESIAN_POINT('Ctrl Pts',(-7.81671694684382,3.15661951052992,
51.4632733746244));
#167223=CARTESIAN_POINT('Ctrl Pts',(-8.39290461146695,0.790229551554735,
51.5512709677656));
#167224=CARTESIAN_POINT('Ctrl Pts',(-7.60701611462514,-3.63299000730349,
51.727266154048));
#167225=CARTESIAN_POINT('Ctrl Pts',(-6.25093680401409,-5.65606750609959,
51.8152637471892));
#167226=CARTESIAN_POINT('Ctrl Pts',(-2.45807268688641,-8.0636957548829,
51.9912589334716));
#167227=CARTESIAN_POINT('Ctrl Pts',(-0.0502299510463028,-8.42987470330084,
52.0792565266128));
#167228=CARTESIAN_POINT('Ctrl Pts',(4.28689960880906,-7.25863639434614,
52.2552517128952));
#167229=CARTESIAN_POINT('Ctrl Pts',(6.18309125557085,-5.7301564626646,52.3432493060364));
#167230=CARTESIAN_POINT('Ctrl Pts',(7.81050559202884,-2.5864071380034,52.4819304138558));
#167231=CARTESIAN_POINT('Ctrl Pts',(8.12525000000002,-1.29375883538179,
52.5326139285341));
#167232=CARTESIAN_POINT('Ctrl Pts',(8.12525,1.19477141073054E-13,52.5832974432124));
#167233=CARTESIAN_POINT('',(8.12525,-4.6183759941365E-13,56.5832974432124));
#167234=CARTESIAN_POINT('Ctrl Pts',(8.12524980819547,0.00176547994832403,
52.5830473882962));
#167235=CARTESIAN_POINT('Ctrl Pts',(8.12524364980434,0.0301081787410185,
52.5841494397994));
#167236=CARTESIAN_POINT('Ctrl Pts',(8.12508919290422,0.05845064286214,52.5852526953861));
#167237=CARTESIAN_POINT('Ctrl Pts',(8.12444520351248,0.118736080490925,
52.5876021191595));
#167238=CARTESIAN_POINT('Ctrl Pts',(8.12391557225265,0.150678096441481,
52.5888486012718));
#167239=CARTESIAN_POINT('Ctrl Pts',(8.12241848601408,0.217272047186492,
52.5914509636609));
#167240=CARTESIAN_POINT('Ctrl Pts',(8.12141762297129,0.251922582637177,
52.5928071001308));
#167241=CARTESIAN_POINT('Ctrl Pts',(8.11855027708299,0.333172424316436,
52.5959920901548));
#167242=CARTESIAN_POINT('Ctrl Pts',(8.11650427598706,0.379764110366802,
52.5978224004088));
#167243=CARTESIAN_POINT('Ctrl Pts',(8.1084684309325,0.532703079706359,52.6038438746892));
#167244=CARTESIAN_POINT('Ctrl Pts',(8.10078858546559,0.638949838364625,
52.6080484828693));
#167245=CARTESIAN_POINT('Ctrl Pts',(8.08063974503247,0.8577707765569,52.6167526943706));
#167246=CARTESIAN_POINT('Ctrl Pts',(8.06790134402783,0.970297412420684,
52.6212532560794));
#167247=CARTESIAN_POINT('Ctrl Pts',(8.0390913503981,1.18461350552756,52.6298659506021));
#167248=CARTESIAN_POINT('Ctrl Pts',(8.02342700255712,1.28643615053409,52.6339756641758));
#167249=CARTESIAN_POINT('Ctrl Pts',(7.97269296883845,1.57907854654426,52.6458250754722));
#167250=CARTESIAN_POINT('Ctrl Pts',(7.93271981166649,1.76897697253052,52.6535626818822));
#167251=CARTESIAN_POINT('Ctrl Pts',(7.87956828591667,1.98312920696857,52.6622845119913));
#167252=CARTESIAN_POINT('Ctrl Pts',(7.87302124809859,2.00896347833129,52.663336561779));
#167253=CARTESIAN_POINT('Ctrl Pts',(7.86153479496716,2.05336979698259,52.6651444331469));
#167254=CARTESIAN_POINT('Ctrl Pts',(7.85665638235957,2.07195737114584,52.6659010230804));
#167255=CARTESIAN_POINT('Ctrl Pts',(7.84718558242081,2.10752829488696,52.6673484896315));
#167256=CARTESIAN_POINT('Ctrl Pts',(7.84260388745124,2.12451437874236,52.6680395125751));
#167257=CARTESIAN_POINT('Ctrl Pts',(7.83345778635271,2.15798966484895,52.6694008784996));
#167258=CARTESIAN_POINT('Ctrl Pts',(7.82889640601104,2.17447955851659,52.6700712499469));
#167259=CARTESIAN_POINT('Ctrl Pts',(7.81615638224685,2.21997640851222,52.6719201965385));
#167260=CARTESIAN_POINT('Ctrl Pts',(7.80786837905136,2.24895247458976,52.6730970546445));
#167261=CARTESIAN_POINT('Ctrl Pts',(7.77781867944381,2.35184201129915,52.6772743654238));
#167262=CARTESIAN_POINT('Ctrl Pts',(7.7551669512367,2.42549169822684,52.6802617312939));
#167263=CARTESIAN_POINT('Ctrl Pts',(7.70104970078162,2.5929338795687,52.6870572082245));
#167264=CARTESIAN_POINT('Ctrl Pts',(7.66891189196776,2.68649646263372,52.6908570679943));
#167265=CARTESIAN_POINT('Ctrl Pts',(7.63057555018146,2.79180537228536,52.6951473183141));
#167266=CARTESIAN_POINT('Ctrl Pts',(7.62604754298188,2.80415037692119,52.6956504584141));
#167267=CARTESIAN_POINT('Ctrl Pts',(7.50826267281147,3.12287970464047,52.7086467029539));
#167268=CARTESIAN_POINT('Ctrl Pts',(7.37666184033898,3.42217014181975,52.7209987710771));
#167269=CARTESIAN_POINT('Ctrl Pts',(7.10194013991312,3.95695900570685,52.7438563981186));
#167270=CARTESIAN_POINT('Ctrl Pts',(6.96417927904945,4.19467312589471,52.7543267985542));
#167271=CARTESIAN_POINT('Ctrl Pts',(6.7552169514716,4.51648556842928,52.7691022334592));
#167272=CARTESIAN_POINT('Ctrl Pts',(6.6939451979396,4.6068096751942,52.773318835394));
#167273=CARTESIAN_POINT('Ctrl Pts',(6.5956544134045,4.74560258961966,52.7799151332479));
#167274=CARTESIAN_POINT('Ctrl Pts',(6.55987756512564,4.79493559538267,52.7822834641372));
#167275=CARTESIAN_POINT('Ctrl Pts',(6.49869709897378,4.87733138658489,52.786280357297));
#167276=CARTESIAN_POINT('Ctrl Pts',(6.47358776137376,4.91060962811642,52.7879062077734));
#167277=CARTESIAN_POINT('Ctrl Pts',(6.42690649413506,4.97149755920482,52.7909026886655));
#167278=CARTESIAN_POINT('Ctrl Pts',(6.40540991914324,4.99916381253992,52.7922726154028));
#167279=CARTESIAN_POINT('Ctrl Pts',(6.36053392030442,5.05615489079459,52.7951122120692));
#167280=CARTESIAN_POINT('Ctrl Pts',(6.3371290482563,5.08545862695046,52.7965820783784));
#167281=CARTESIAN_POINT('Ctrl Pts',(6.28387947523037,5.15119053401777,52.799901579663));
#167282=CARTESIAN_POINT('Ctrl Pts',(6.25391928403291,5.18752337306637,52.8017521633865));
#167283=CARTESIAN_POINT('Ctrl Pts',(6.16135495271028,5.29780904610997,52.8074183505815));
#167284=CARTESIAN_POINT('Ctrl Pts',(6.09774264110756,5.37090402746593,52.8112419931888));
#167285=CARTESIAN_POINT('Ctrl Pts',(5.81855289916133,5.68035746699471,52.8277295692925));
#167286=CARTESIAN_POINT('Ctrl Pts',(5.59043004009725,5.90500681505646,52.8404288021798));
#167287=CARTESIAN_POINT('Ctrl Pts',(5.05543404332821,6.37299682983889,52.8691317044041));
#167288=CARTESIAN_POINT('Ctrl Pts',(4.74302764078544,6.60879483677502,52.8852560908435));
#167289=CARTESIAN_POINT('Ctrl Pts',(4.22292207081797,6.94542282654672,52.9112908980809));
#167290=CARTESIAN_POINT('Ctrl Pts',(4.0258108205282,7.06150228536007,52.9209808249307));
#167291=CARTESIAN_POINT('Ctrl Pts',(3.58411376410034,7.29710746165448,52.9421679662169));
#167292=CARTESIAN_POINT('Ctrl Pts',(3.33787837770958,7.41297663020197,52.9536491842324));
#167293=CARTESIAN_POINT('Ctrl Pts',(2.96920252204968,7.56436023241498,52.9700379370817));
#167294=CARTESIAN_POINT('Ctrl Pts',(2.85100111303177,7.60969800405325,52.9751747443793));
#167295=CARTESIAN_POINT('Ctrl Pts',(2.71167995292251,7.65943438942436,52.9810572929424));
#167296=CARTESIAN_POINT('Ctrl Pts',(2.6915456165161,7.66653282374316,52.9819032603197));
#167297=CARTESIAN_POINT('Ctrl Pts',(2.66223391662965,7.67673706692509,52.983128547788));
#167298=CARTESIAN_POINT('Ctrl Pts',(2.65307869349873,7.67990591535224,52.9835103663421));
#167299=CARTESIAN_POINT('Ctrl Pts',(2.63704505729796,7.68542345979927,52.9841774691844));
#167300=CARTESIAN_POINT('Ctrl Pts',(2.63016912886034,7.68777931165431,52.9844630444677));
#167301=CARTESIAN_POINT('Ctrl Pts',(2.61684589222069,7.69232419351748,52.9850153978052));
#167302=CARTESIAN_POINT('Ctrl Pts',(2.61039897746855,7.69451435118389,52.9852822224627));
#167303=CARTESIAN_POINT('Ctrl Pts',(2.59330113024004,7.70029890147038,52.9859886585913));
#167304=CARTESIAN_POINT('Ctrl Pts',(2.58264545584154,7.70387930689289,52.986427679381));
#167305=CARTESIAN_POINT('Ctrl Pts',(2.54495994649214,7.71645501233108,52.9879758731397));
#167306=CARTESIAN_POINT('Ctrl Pts',(2.51789006627449,7.7253303313814,52.9890798327609));
#167307=CARTESIAN_POINT('Ctrl Pts',(2.0670385329708,7.87052816327125,53.007324847304));
#167308=CARTESIAN_POINT('Ctrl Pts',(1.63279095495319,7.97194318363231,53.0226952712351));
#167309=CARTESIAN_POINT('Ctrl Pts',(0.956991521298055,8.07220542378015,
53.0456933946499));
#167310=CARTESIAN_POINT('Ctrl Pts',(0.720142929848893,8.09677272844999,
53.0535848358485));
#167311=CARTESIAN_POINT('Ctrl Pts',(0.123726161042556,8.13225643387959,
53.0735568585539));
#167312=CARTESIAN_POINT('Ctrl Pts',(-0.236114537315934,8.12976861940751,
53.0857107651117));
#167313=CARTESIAN_POINT('Ctrl Pts',(-0.899715183285292,8.08107663315175,
53.109308456053));
#167314=CARTESIAN_POINT('Ctrl Pts',(-1.2033054909797,8.041475128801,53.1205665819576));
#167315=CARTESIAN_POINT('Ctrl Pts',(-1.52994162646951,7.97995407201859,
53.1333796028177));
#167316=CARTESIAN_POINT('Ctrl Pts',(-1.55593275762511,7.97492705984995,
53.134403944482));
#167317=CARTESIAN_POINT('Ctrl Pts',(-1.59422907750533,7.96732572690989,
53.1359204024423));
#167318=CARTESIAN_POINT('Ctrl Pts',(-1.60655371162721,7.96484970104272,
53.1364095281425));
#167319=CARTESIAN_POINT('Ctrl Pts',(-1.62834828306713,7.96041851496297,
53.1372764342931));
#167320=CARTESIAN_POINT('Ctrl Pts',(-1.63782058250833,7.95847502999453,
53.1376538587581));
#167321=CARTESIAN_POINT('Ctrl Pts',(-1.65633791039776,7.95464126624829,
53.1383929636836));
#167322=CARTESIAN_POINT('Ctrl Pts',(-1.66538323037867,7.95275245707023,
53.1387545989205));
#167323=CARTESIAN_POINT('Ctrl Pts',(-1.68976902745533,7.94761687980665,
53.1397311719023));
#167324=CARTESIAN_POINT('Ctrl Pts',(-1.70510332490954,7.94434113582644,
53.140346991521));
#167325=CARTESIAN_POINT('Ctrl Pts',(-1.76155669317739,7.93211047246434,
53.1426205509197));
#167326=CARTESIAN_POINT('Ctrl Pts',(-1.80261515888727,7.92288060334149,
53.1442866596397));
#167327=CARTESIAN_POINT('Ctrl Pts',(-2.50359534796896,7.75957053081513,
53.1729492991114));
#167328=CARTESIAN_POINT('Ctrl Pts',(-3.14166840407209,7.52386786522178,
53.2026434635012));
#167329=CARTESIAN_POINT('Ctrl Pts',(-4.08816258099939,7.03262804904752,
53.2505134909075));
#167330=CARTESIAN_POINT('Ctrl Pts',(-4.42004227846969,6.82892181270963,
53.2680752781826));
#167331=CARTESIAN_POINT('Ctrl Pts',(-4.86346280159948,6.5108371267576,53.2916706494515));
#167332=CARTESIAN_POINT('Ctrl Pts',(-4.9881969189763,6.41577479799822,53.2983208620974));
#167333=CARTESIAN_POINT('Ctrl Pts',(-5.17537780956116,6.2643595143959,53.3082335444692));
#167334=CARTESIAN_POINT('Ctrl Pts',(-5.23982252973921,6.21055519564037,
53.3116305437736));
#167335=CARTESIAN_POINT('Ctrl Pts',(-5.31509526012769,6.14570477041037,
53.3155848220997));
#167336=CARTESIAN_POINT('Ctrl Pts',(-5.32673453854297,6.13561927678388,
53.3161959406604));
#167337=CARTESIAN_POINT('Ctrl Pts',(-5.34527493106549,6.119461411683,53.3171689964752));
#167338=CARTESIAN_POINT('Ctrl Pts',(-5.3521945013234,6.1134103476423,53.3175320659135));
#167339=CARTESIAN_POINT('Ctrl Pts',(-5.36473441860925,6.1024067625279,53.318189897479));
#167340=CARTESIAN_POINT('Ctrl Pts',(-5.37035820733078,6.09745819198557,
53.3184848655716));
#167341=CARTESIAN_POINT('Ctrl Pts',(-5.38160424078162,6.08753478153266,
53.3190746363133));
#167342=CARTESIAN_POINT('Ctrl Pts',(-5.3872264497955,6.08255991337862,53.3193694369066));
#167343=CARTESIAN_POINT('Ctrl Pts',(-5.40306794553901,6.06850321341805,
53.3201999891223));
#167344=CARTESIAN_POINT('Ctrl Pts',(-5.41327124360715,6.05940334697036,
53.3207348229191));
#167345=CARTESIAN_POINT('Ctrl Pts',(-5.4556021226161,6.02145806877636,53.3229534411135));
#167346=CARTESIAN_POINT('Ctrl Pts',(-5.48752280765111,5.99238227337843,
53.3246257987157));
#167347=CARTESIAN_POINT('Ctrl Pts',(-5.97033212278799,5.54550946973115,
53.3499339597509));
#167348=CARTESIAN_POINT('Ctrl Pts',(-6.37264919323184,5.07809061416835,
53.3713685981259));
#167349=CARTESIAN_POINT('Ctrl Pts',(-6.96678705617603,4.20459128241462,
53.4095269562731));
#167350=CARTESIAN_POINT('Ctrl Pts',(-7.18496127042977,3.81981869399859,
53.4257761720295));
#167351=CARTESIAN_POINT('Ctrl Pts',(-7.39581230987746,3.36529113397211,
53.4449234833113));
#167352=CARTESIAN_POINT('Ctrl Pts',(-7.42024471149788,3.31107119722726,
53.4472057502132));
#167353=CARTESIAN_POINT('Ctrl Pts',(-7.45787772142508,3.22504769761268,
53.450824233195));
#167354=CARTESIAN_POINT('Ctrl Pts',(-7.47147524395176,3.19341986311009,
53.4521540938941));
#167355=CARTESIAN_POINT('Ctrl Pts',(-7.49420432098751,3.13961214663148,
53.4544156671137));
#167356=CARTESIAN_POINT('Ctrl Pts',(-7.50343943801816,3.11747645228425,
53.4553457906309));
#167357=CARTESIAN_POINT('Ctrl Pts',(-7.52147381051481,3.07370538314876,
53.4571845017296));
#167358=CARTESIAN_POINT('Ctrl Pts',(-7.53027806140087,3.05207230873849,
53.4580930060731));
#167359=CARTESIAN_POINT('Ctrl Pts',(-7.53901433962415,3.03033832337175,
53.459005490529));
#167360=CARTESIAN_POINT('Ctrl Pts',(-7.53903978272908,3.03027502408319,
53.4590081480982));
#167361=CARTESIAN_POINT('Ctrl Pts',(-7.53909088779636,3.03014787638837,
53.4590134862864));
#167362=CARTESIAN_POINT('Ctrl Pts',(-7.5391165497118,3.03008402805877,53.4590161669021));
#167363=CARTESIAN_POINT('Ctrl Pts',(-7.53916809297861,3.02995578072195,
53.4590215512489));
#167364=CARTESIAN_POINT('Ctrl Pts',(-7.53919397427158,3.02989138181951,
53.4590242549754));
#167365=CARTESIAN_POINT('Ctrl Pts',(-7.53924595678346,3.02976203199594,
53.4590296855999));
#167366=CARTESIAN_POINT('Ctrl Pts',(-7.53927205799163,3.02969708106049,
53.4590324124985));
#167367=CARTESIAN_POINT('Ctrl Pts',(-7.53932448071584,3.02956662609727,
53.4590378895119));
#167368=CARTESIAN_POINT('Ctrl Pts',(-7.53935080229867,3.0295011218618,53.4590406396355));
#167369=CARTESIAN_POINT('Ctrl Pts',(-7.53940366632769,3.02936955879153,
53.4590461631622));
#167370=CARTESIAN_POINT('Ctrl Pts',(-7.53943020877195,3.02930349991962,
53.4590489365668));
#167371=CARTESIAN_POINT('Ctrl Pts',(-7.53948351511514,3.02917082597877,
53.4590545067226));
#167372=CARTESIAN_POINT('Ctrl Pts',(-7.53951027893799,3.02910421105684,
53.4590573034675));
#167373=CARTESIAN_POINT('Ctrl Pts',(-7.53956401754028,3.02897045101929,
53.4590629192119));
#167374=CARTESIAN_POINT('Ctrl Pts',(-7.53959099232742,3.02890330584792,
53.4590657382133));
#167375=CARTESIAN_POINT('Ctrl Pts',(-7.53964520790905,3.02876834813996,
53.4590714042305));
#167376=CARTESIAN_POINT('Ctrl Pts',(-7.5396724162355,3.02870061638599,53.4590742478543));
#167377=CARTESIAN_POINT('Ctrl Pts',(-7.53972705406999,3.02856459697546,
53.4590799584355));
#167378=CARTESIAN_POINT('Ctrl Pts',(-7.53975448496652,3.0284963058182,53.4590828255399));
#167379=CARTESIAN_POINT('Ctrl Pts',(-7.53980957794039,3.02835914257522,
53.4590885841331));
#167380=CARTESIAN_POINT('Ctrl Pts',(-7.53983724119974,3.02829026749664,
53.4590914757478));
#167381=CARTESIAN_POINT('Ctrl Pts',(-7.53989761676832,3.02813994043697,
53.4590977869927));
#167382=CARTESIAN_POINT('Ctrl Pts',(-7.53993035782358,3.02805841578205,
53.4591012096733));
#167383=CARTESIAN_POINT('Ctrl Pts',(-7.53999694110362,3.02789261680388,
53.4591081704675));
#167384=CARTESIAN_POINT('Ctrl Pts',(-7.54003078327093,3.02780834236157,
53.4591117085859));
#167385=CARTESIAN_POINT('Ctrl Pts',(-7.54009959633272,3.02763697438965,
53.4591189031692));
#167386=CARTESIAN_POINT('Ctrl Pts',(-7.54013456707983,3.02754988094928,
53.4591225596302));
#167387=CARTESIAN_POINT('Ctrl Pts',(-7.54020566465514,3.02737280601586,
53.4591299937933));
#167388=CARTESIAN_POINT('Ctrl Pts',(-7.54024179141008,3.02728282441113,
53.4591337714999));
#167389=CARTESIAN_POINT('Ctrl Pts',(-7.54031522852707,3.02709990369866,
53.4591414510692));
#167390=CARTESIAN_POINT('Ctrl Pts',(-7.54035253877454,3.02700696456519,
53.4591453529327));
#167391=CARTESIAN_POINT('Ctrl Pts',(-7.54042837035463,3.02681805940569,
53.4591532837281));
#167392=CARTESIAN_POINT('Ctrl Pts',(-7.54046689155222,3.02672209338719,
53.4591573126594));
#167393=CARTESIAN_POINT('Ctrl Pts',(-7.54054517236893,3.02652706536018,
53.4591655004903));
#167394=CARTESIAN_POINT('Ctrl Pts',(-7.54058493187534,3.02642800328518,
53.4591696593923));
#167395=CARTESIAN_POINT('Ctrl Pts',(-7.54066571651116,3.02622671432042,
53.4591781100533));
#167396=CARTESIAN_POINT('Ctrl Pts',(-7.54070674153946,3.0261244873162,53.4591824018166));
#167397=CARTESIAN_POINT('Ctrl Pts',(-7.54079008433386,3.02591679981866,
53.4591911210822));
#167398=CARTESIAN_POINT('Ctrl Pts',(-7.54083240195278,3.02581133930582,
53.4591955485848));
#167399=CARTESIAN_POINT('Ctrl Pts',(-7.54091835674091,3.02559711680211,
53.4592045421822));
#167400=CARTESIAN_POINT('Ctrl Pts',(-7.5409619937665,3.02548835476233,53.4592091082786));
#167401=CARTESIAN_POINT('Ctrl Pts',(-7.54105061390349,3.02526746183582,
53.4592183818907));
#167402=CARTESIAN_POINT('Ctrl Pts',(-7.54109559686292,3.02515533089981,
53.4592230894081));
#167403=CARTESIAN_POINT('Ctrl Pts',(-7.54930805871703,3.00468245654526,
53.4600825869985));
#167404=CARTESIAN_POINT('Ctrl Pts',(-7.55739303655472,2.98428874575111,
53.4609385218818));
#167405=CARTESIAN_POINT('Ctrl Pts',(-7.57551424033519,2.93803354119027,
53.4628794789341));
#167406=CARTESIAN_POINT('Ctrl Pts',(-7.5855008042606,2.91215292092137,53.4639652041845));
#167407=CARTESIAN_POINT('Ctrl Pts',(-7.61468345057594,2.83535613696169,
53.4671865292511));
#167408=CARTESIAN_POINT('Ctrl Pts',(-7.63350072338563,2.78429795722043,
53.4693277134119));
#167409=CARTESIAN_POINT('Ctrl Pts',(-7.81365719075656,2.27990929505585,
53.4904840891173));
#167410=CARTESIAN_POINT('Ctrl Pts',(-7.93492731954391,1.81331260290932,
53.5101723806308));
#167411=CARTESIAN_POINT('Ctrl Pts',(-8.0578859729071,1.07724564580059,53.5415444711816));
#167412=CARTESIAN_POINT('Ctrl Pts',(-8.0887443694058,0.813754326795947,
53.5528169504256));
#167413=CARTESIAN_POINT('Ctrl Pts',(-8.13058321827464,0.196211154622309,
53.5790622868739));
#167414=CARTESIAN_POINT('Ctrl Pts',(-8.13141645595455,-0.158007032505852,
53.5939918025026));
#167415=CARTESIAN_POINT('Ctrl Pts',(-8.10614464323266,-0.558925034036176,
53.6101680111357));
#167416=CARTESIAN_POINT('Ctrl Pts',(-8.10271174310439,-0.606663568979511,
53.6120821385718));
#167417=CARTESIAN_POINT('Ctrl Pts',(-8.09775859865418,-0.667966561195639,
53.6145226484334));
#167418=CARTESIAN_POINT('Ctrl Pts',(-8.09662574423342,-0.6815608626115,
53.6150627385459));
#167419=CARTESIAN_POINT('Ctrl Pts',(-8.09474584089639,-0.703453446227345,
53.6159306675297));
#167420=CARTESIAN_POINT('Ctrl Pts',(-8.09402025659813,-0.711753515005144,
53.6162592954643));
#167421=CARTESIAN_POINT('Ctrl Pts',(-8.0926143483367,-0.72755571323603,
53.616884127871));
#167422=CARTESIAN_POINT('Ctrl Pts',(-8.09193635585925,-0.735058038497996,
53.617180419709));
#167423=CARTESIAN_POINT('Ctrl Pts',(-8.09036727638708,-0.752155405516818,
53.617854824384));
#167424=CARTESIAN_POINT('Ctrl Pts',(-8.08946955042374,-0.761749837316664,
53.6182326821159));
#167425=CARTESIAN_POINT('Ctrl Pts',(-8.08710127774096,-0.786584329029695,
53.6192091660627));
#167426=CARTESIAN_POINT('Ctrl Pts',(-8.08560471511598,-0.801821911727744,
53.6198067682296));
#167427=CARTESIAN_POINT('Ctrl Pts',(-8.07590900627188,-0.897752685501701,
53.6235590612171));
#167428=CARTESIAN_POINT('Ctrl Pts',(-8.0665451537695,-0.97832329952201,
53.6266642550969));
#167429=CARTESIAN_POINT('Ctrl Pts',(-7.9808792123672,-1.63015319844165,
53.6513915846882));
#167430=CARTESIAN_POINT('Ctrl Pts',(-7.84519476196112,-2.19200057581035,
53.6704387144985));
#167431=CARTESIAN_POINT('Ctrl Pts',(-7.52317004892309,-3.09293663648932,
53.7026340557152));
#167432=CARTESIAN_POINT('Ctrl Pts',(-7.37017093402944,-3.44164338884954,
53.7155355568344));
#167433=CARTESIAN_POINT('Ctrl Pts',(-7.07175799200144,-4.00977104690499,
53.7384189845445));
#167434=CARTESIAN_POINT('Ctrl Pts',(-6.93910643618912,-4.23518762216387,
53.7480331063399));
#167435=CARTESIAN_POINT('Ctrl Pts',(-6.76954146201848,-4.49391761185007,
53.7598605949337));
#167436=CARTESIAN_POINT('Ctrl Pts',(-6.74290170676816,-4.53379130408999,
53.7617063909744));
#167437=CARTESIAN_POINT('Ctrl Pts',(-6.70693207382814,-4.58661140496663,
53.764182958554));
#167438=CARTESIAN_POINT('Ctrl Pts',(-6.69791455914659,-4.59976983968183,
53.7648025440128));
#167439=CARTESIAN_POINT('Ctrl Pts',(-6.68299538066868,-4.62140313709725,
53.7658255435798));
#167440=CARTESIAN_POINT('Ctrl Pts',(-6.67711618734289,-4.62989347970297,
53.7662281485481));
#167441=CARTESIAN_POINT('Ctrl Pts',(-6.66565615059951,-4.64637607887285,
53.7670119112615));
#167442=CARTESIAN_POINT('Ctrl Pts',(-6.66007707842383,-4.65436954839298,
53.7673930047172));
#167443=CARTESIAN_POINT('Ctrl Pts',(-6.64710938159008,-4.67287808423019,
53.768277730539));
#167444=CARTESIAN_POINT('Ctrl Pts',(-6.63971017654716,-4.6833856867158,
53.7687817458024));
#167445=CARTESIAN_POINT('Ctrl Pts',(-6.61571360933007,-4.71729201711857,
53.7704137808348));
#167446=CARTESIAN_POINT('Ctrl Pts',(-6.59901733310505,-4.74062029194703,
53.7715453958729));
#167447=CARTESIAN_POINT('Ctrl Pts',(-6.43646655468301,-4.96521579061872,
53.7825255226603));
#167448=CARTESIAN_POINT('Ctrl Pts',(-6.28158171166152,-5.1597662209341,
53.7927080582552));
#167449=CARTESIAN_POINT('Ctrl Pts',(-5.74159481102126,-5.77762989287939,
53.8273480140395));
#167450=CARTESIAN_POINT('Ctrl Pts',(-5.3207525944797,-6.16736531919509,
53.8531512935697));
#167451=CARTESIAN_POINT('Ctrl Pts',(-4.44069035079091,-6.82474932264212,
53.9026677062644));
#167452=CARTESIAN_POINT('Ctrl Pts',(-3.98914149207106,-7.09815935361309,
53.9262034684646));
#167453=CARTESIAN_POINT('Ctrl Pts',(-3.48899896729561,-7.3380758693166,
53.9483984446961));
#167454=CARTESIAN_POINT('Ctrl Pts',(-3.46369560122287,-7.35005333778223,
53.9495119384426));
#167455=CARTESIAN_POINT('Ctrl Pts',(-3.42852960117716,-7.366477404413,53.9510471099722));
#167456=CARTESIAN_POINT('Ctrl Pts',(-3.4187194247629,-7.37103534601368,
53.9514740479467));
#167457=CARTESIAN_POINT('Ctrl Pts',(-3.40210986448248,-7.37871208205247,
53.9521947013737));
#167458=CARTESIAN_POINT('Ctrl Pts',(-3.3953152398686,-7.38184109435135,
53.9524888862204));
#167459=CARTESIAN_POINT('Ctrl Pts',(-3.38183377594752,-7.38802693091668,
53.9530713795946));
#167460=CARTESIAN_POINT('Ctrl Pts',(-3.37514708995806,-7.39108407080477,
53.9533597021996));
#167461=CARTESIAN_POINT('Ctrl Pts',(-3.36036066512558,-7.397820145331,53.9539959949062));
#167462=CARTESIAN_POINT('Ctrl Pts',(-3.35225900885114,-7.40149486528041,
53.9543437785741));
#167463=CARTESIAN_POINT('Ctrl Pts',(-3.32374531574716,-7.41437158261301,
53.955564870252));
#167464=CARTESIAN_POINT('Ctrl Pts',(-3.30330118722569,-7.42350255390154,
53.9564351128522));
#167465=CARTESIAN_POINT('Ctrl Pts',(-2.96812674576461,-7.57154290765394,
53.9706202156254));
#167466=CARTESIAN_POINT('Ctrl Pts',(-2.64490304387577,-7.69041967842869,
53.9831348263974));
#167467=CARTESIAN_POINT('Ctrl Pts',(-1.75029168147407,-7.95634108712757,
54.0167136835833));
#167468=CARTESIAN_POINT('Ctrl Pts',(-1.16890894714928,-8.0622912723805,
54.0375727501024));
#167469=CARTESIAN_POINT('Ctrl Pts',(-0.176676835861371,-8.13344560927159,
54.0746605155247));
#167470=CARTESIAN_POINT('Ctrl Pts',(0.229420777241419,-8.13212734769299,
54.0901700021729));
#167471=CARTESIAN_POINT('Ctrl Pts',(0.729896328458756,-8.09297531033613,
54.1096013996823));
#167472=CARTESIAN_POINT('Ctrl Pts',(0.825950943604796,-8.08373693700102,
54.1133483580759));
#167473=CARTESIAN_POINT('Ctrl Pts',(0.968565452347753,-8.06745203739496,
54.1189435908539));
#167474=CARTESIAN_POINT('Ctrl Pts',(1.01526583984839,-8.06170804860475,
54.1207809197321));
#167475=CARTESIAN_POINT('Ctrl Pts',(1.09913153172508,-8.05065256276127,
54.1240903654974));
#167476=CARTESIAN_POINT('Ctrl Pts',(1.13631496230111,-8.04548849380078,
54.1255611881129));
#167477=CARTESIAN_POINT('Ctrl Pts',(1.21584084841255,-8.03388155805482,
54.128714828822));
#167478=CARTESIAN_POINT('Ctrl Pts',(1.25817083177055,-8.02736121001849,
54.1303982707186));
#167479=CARTESIAN_POINT('Ctrl Pts',(1.37227592879423,-8.00886017768247,
54.1349498576967));
#167480=CARTESIAN_POINT('Ctrl Pts',(1.44394466066106,-7.99624951405341,
54.1378233522897));
#167481=CARTESIAN_POINT('Ctrl Pts',(1.89348683523406,-7.91090829203186,
54.1559459271916));
#167482=CARTESIAN_POINT('Ctrl Pts',(2.26595581947577,-7.81237446075199,
54.1714180780486));
#167483=CARTESIAN_POINT('Ctrl Pts',(3.0126659260573,-7.55692245166015,54.2034241673218));
#167484=CARTESIAN_POINT('Ctrl Pts',(3.38499690252614,-7.3976369110117,54.219927284617));
#167485=CARTESIAN_POINT('Ctrl Pts',(3.82004468955709,-7.17177128653606,
54.2396220297491));
#167486=CARTESIAN_POINT('Ctrl Pts',(3.89554088451969,-7.1310452423553,54.2430548394567));
#167487=CARTESIAN_POINT('Ctrl Pts',(4.02172702588589,-7.06037272412983,
54.2488126731674));
#167488=CARTESIAN_POINT('Ctrl Pts',(4.07276181134012,-7.03105700376996,
54.2511470433447));
#167489=CARTESIAN_POINT('Ctrl Pts',(4.14438712530256,-6.98887201163811,
54.2544296980245));
#167490=CARTESIAN_POINT('Ctrl Pts',(4.16524512180752,-6.97646111732856,
54.2553864212102));
#167491=CARTESIAN_POINT('Ctrl Pts',(4.20036359491391,-6.95535133882824,
54.2569984343586));
#167492=CARTESIAN_POINT('Ctrl Pts',(4.21465338516476,-6.94670162168263,
54.257654695852));
#167493=CARTESIAN_POINT('Ctrl Pts',(4.24464069325903,-6.9284234903019,54.2590327127431));
#167494=CARTESIAN_POINT('Ctrl Pts',(4.26033236761147,-6.91878564461391,
54.2597542864382));
#167495=CARTESIAN_POINT('Ctrl Pts',(4.30453835918811,-6.89142685985561,
54.261788725878));
#167496=CARTESIAN_POINT('Ctrl Pts',(4.33297586902503,-6.87358238358548,
54.263099418368));
#167497=CARTESIAN_POINT('Ctrl Pts',(4.48010073291159,-6.77998597811191,
54.2698934814721));
#167498=CARTESIAN_POINT('Ctrl Pts',(4.59691600681669,-6.701333925397,54.2753327364994));
#167499=CARTESIAN_POINT('Ctrl Pts',(4.90754315397383,-6.48024185858617,
54.2900199295934));
#167500=CARTESIAN_POINT('Ctrl Pts',(5.09716991908419,-6.33216971881919,
54.2992346229609));
#167501=CARTESIAN_POINT('Ctrl Pts',(5.34771319825525,-6.11797344881262,
54.3119481904637));
#167502=CARTESIAN_POINT('Ctrl Pts',(5.41451794881067,-6.05892984266549,
54.3153935533495));
#167503=CARTESIAN_POINT('Ctrl Pts',(5.53215109279547,-5.95146344872346,
54.3215692070606));
#167504=CARTESIAN_POINT('Ctrl Pts',(5.58334922731551,-5.9034586667603,54.3242953685686));
#167505=CARTESIAN_POINT('Ctrl Pts',(5.66263144601188,-5.82716744779668,
54.3285804460464));
#167506=CARTESIAN_POINT('Ctrl Pts',(5.69114033595974,-5.79932729032866,
54.3301345200194));
#167507=CARTESIAN_POINT('Ctrl Pts',(5.74441198773741,-5.74653410394675,
54.3330639830113));
#167508=CARTESIAN_POINT('Ctrl Pts',(5.76921986082141,-5.72162786977985,
54.3344388234295));
#167509=CARTESIAN_POINT('Ctrl Pts',(5.82522755806615,-5.6646634969339,54.3375673764925));
#167510=CARTESIAN_POINT('Ctrl Pts',(5.85632580090224,-5.63250714422822,
54.3393221752628));
#167511=CARTESIAN_POINT('Ctrl Pts',(5.95338834748967,-5.5304691677471,54.3448559742541));
#167512=CARTESIAN_POINT('Ctrl Pts',(6.0183790741575,-5.45967353919144,54.3486453556684));
#167513=CARTESIAN_POINT('Ctrl Pts',(6.20757599735532,-5.24609347828311,
54.3599339236108));
#167514=CARTESIAN_POINT('Ctrl Pts',(6.32806586628197,-5.10010567051107,
54.3674671502798));
#167515=CARTESIAN_POINT('Ctrl Pts',(6.57137996739337,-4.78338993721634,
54.3834102417702));
#167516=CARTESIAN_POINT('Ctrl Pts',(6.69289812019851,-4.61182924767036,
54.3918194686756));
#167517=CARTESIAN_POINT('Ctrl Pts',(6.86131204173906,-4.35336129611263,
54.4040880818385));
#167518=CARTESIAN_POINT('Ctrl Pts',(6.91349603492676,-4.27000355426077,
54.4079860718544));
#167519=CARTESIAN_POINT('Ctrl Pts',(6.97907978094137,-4.16088601147033,
54.4130030875769));
#167520=CARTESIAN_POINT('Ctrl Pts',(6.99387225281498,-4.13597363511027,
54.4141428264914));
#167521=CARTESIAN_POINT('Ctrl Pts',(7.0185679885778,-4.09387157548053,54.4160590542634));
#167522=CARTESIAN_POINT('Ctrl Pts',(7.02854209568946,-4.07672381928628,
54.4168367541));
#167523=CARTESIAN_POINT('Ctrl Pts',(7.0479523348723,-4.04307023457226,54.4183578259819));
#167524=CARTESIAN_POINT('Ctrl Pts',(7.05739353045289,-4.02656747060298,
54.4191012760194));
#167525=CARTESIAN_POINT('Ctrl Pts',(7.08016606869002,-3.98643600637395,
54.420903484131));
#167526=CARTESIAN_POINT('Ctrl Pts',(7.09343717530291,-3.96277335212363,
54.4219613318108));
#167527=CARTESIAN_POINT('Ctrl Pts',(7.14436662771634,-3.87088946925784,
54.4260514465524));
#167528=CARTESIAN_POINT('Ctrl Pts',(7.18116151213758,-3.80219400696609,
54.4290720116325));
#167529=CARTESIAN_POINT('Ctrl Pts',(7.41042626853166,-3.35895686149777,
54.448357485444));
#167530=CARTESIAN_POINT('Ctrl Pts',(7.57452243004856,-2.97045851589731,
54.4643694992375));
#167531=CARTESIAN_POINT('Ctrl Pts',(7.77144712261527,-2.38008380501974,
54.488336553349));
#167532=CARTESIAN_POINT('Ctrl Pts',(7.82801146504211,-2.18687552143272,
54.4961195618154));
#167533=CARTESIAN_POINT('Ctrl Pts',(7.89543080501839,-1.92023541996281,
54.5068237724786));
#167534=CARTESIAN_POINT('Ctrl Pts',(7.91254248276351,-1.84845964385544,
54.5097013779439));
#167535=CARTESIAN_POINT('Ctrl Pts',(7.94070087922207,-1.72278351086976,
54.5147347202849));
#167536=CARTESIAN_POINT('Ctrl Pts',(7.95218216816694,-1.66898538526603,
54.516887676653));
#167537=CARTESIAN_POINT('Ctrl Pts',(7.9755349218177,-1.55384478924321,54.5214923484539));
#167538=CARTESIAN_POINT('Ctrl Pts',(7.98724692976988,-1.49247357309473,
54.5239447895776));
#167539=CARTESIAN_POINT('Ctrl Pts',(8.02249802562068,-1.29544192400184,
54.5318124285837));
#167540=CARTESIAN_POINT('Ctrl Pts',(8.04329719357104,-1.15931633250214,
54.5372394604156));
#167541=CARTESIAN_POINT('Ctrl Pts',(8.07606386219592,-0.901066095978931,
54.547513096205));
#167542=CARTESIAN_POINT('Ctrl Pts',(8.08874391057554,-0.779069683750958,
54.5523569417624));
#167543=CARTESIAN_POINT('Ctrl Pts',(8.10413328956513,-0.58932085915289,
54.5598675185954));
#167544=CARTESIAN_POINT('Ctrl Pts',(8.10876440015107,-0.521742642218499,
54.5625377387602));
#167545=CARTESIAN_POINT('Ctrl Pts',(8.11550561902531,-0.401313773201119,
54.5672855645311));
#167546=CARTESIAN_POINT('Ctrl Pts',(8.11794568117978,-0.348485494709742,
54.5693646229922));
#167547=CARTESIAN_POINT('Ctrl Pts',(8.12132835570185,-0.255578071603307,
54.573013217846));
#167548=CARTESIAN_POINT('Ctrl Pts',(8.12249040205009,-0.215508905339158,
54.57458408784));
#167549=CARTESIAN_POINT('Ctrl Pts',(8.12461691524859,-0.11704134067931,
54.5784389024037));
#167550=CARTESIAN_POINT('Ctrl Pts',(8.12524832286776,-0.0586380201683644,
54.5807206687261));
#167551=CARTESIAN_POINT('Ctrl Pts',(8.12525491971375,0.171550475355112,
54.589703608444));
#167552=CARTESIAN_POINT('Ctrl Pts',(8.11981210020081,0.343291064673441,
54.5963838175675));
#167553=CARTESIAN_POINT('Ctrl Pts',(8.10033545336368,0.650121364090579,
54.6083574108132));
#167554=CARTESIAN_POINT('Ctrl Pts',(8.08835174174705,0.785275842340364,
54.6136449609056));
#167555=CARTESIAN_POINT('Ctrl Pts',(8.06595498332815,0.981792965271103,
54.6213765104582));
#167556=CARTESIAN_POINT('Ctrl Pts',(8.05821240080725,1.04343667327795,54.6238079401888));
#167557=CARTESIAN_POINT('Ctrl Pts',(8.04227267466351,1.1595567866989,54.6284021290327));
#167558=CARTESIAN_POINT('Ctrl Pts',(8.03422697667461,1.21405048364178,54.6305639763526));
#167559=CARTESIAN_POINT('Ctrl Pts',(8.01400737120932,1.34198142321735,54.635654673723));
#167560=CARTESIAN_POINT('Ctrl Pts',(8.00137718659765,1.41534142009171,54.6385859157454));
#167561=CARTESIAN_POINT('Ctrl Pts',(7.94967077612587,1.69281042539589,54.6497238707111));
#167562=CARTESIAN_POINT('Ctrl Pts',(7.90377761902846,1.89556601208526,54.6579701059781));
#167563=CARTESIAN_POINT('Ctrl Pts',(7.79371943108897,2.30770138678517,54.6749784275962));
#167564=CARTESIAN_POINT('Ctrl Pts',(7.72876273184253,2.5166990655296,54.6837380667358));
#167565=CARTESIAN_POINT('Ctrl Pts',(7.64706873457894,2.74638911102583,54.693496128925));
#167566=CARTESIAN_POINT('Ctrl Pts',(7.63857679674621,2.7699201976613,54.6944973403019));
#167567=CARTESIAN_POINT('Ctrl Pts',(7.62561224975355,2.80533180085954,54.6960062718883));
#167568=CARTESIAN_POINT('Ctrl Pts',(7.6212202501178,2.81724166443451,54.6965141458834));
#167569=CARTESIAN_POINT('Ctrl Pts',(7.54144306083189,3.03202307098823,54.705679831278));
#167570=CARTESIAN_POINT('Ctrl Pts',(7.45800909820819,3.23181519351035,54.7143166417663));
#167571=CARTESIAN_POINT('Ctrl Pts',(7.35024820374394,3.46338837896831,54.724398390452));
#167572=CARTESIAN_POINT('Ctrl Pts',(7.33354439619643,3.4986189176203,54.7259341040434));
#167573=CARTESIAN_POINT('Ctrl Pts',(7.30681650733137,3.55395904038534,54.728348817017));
#167574=CARTESIAN_POINT('Ctrl Pts',(7.29696152200569,3.57414953290101,54.7292303196149));
#167575=CARTESIAN_POINT('Ctrl Pts',(7.27917835967306,3.61020282547512,54.7308051531294));
#167576=CARTESIAN_POINT('Ctrl Pts',(7.27128176127388,3.62608102275784,54.7314989934957));
#167577=CARTESIAN_POINT('Ctrl Pts',(7.25202795780423,3.66448007626066,54.7331774993387));
#167578=CARTESIAN_POINT('Ctrl Pts',(7.24061775785639,3.68697412758726,54.7341611879483));
#167579=CARTESIAN_POINT('Ctrl Pts',(7.19927691140022,3.76754134875716,54.737686770168));
#167580=CARTESIAN_POINT('Ctrl Pts',(7.16875067865304,3.82530648033681,54.7402189113684));
#167581=CARTESIAN_POINT('Ctrl Pts',(7.11024974095552,3.93284827446323,54.7449486534155));
#167582=CARTESIAN_POINT('Ctrl Pts',(7.08244063637543,3.98271033436281,54.7471480212174));
#167583=CARTESIAN_POINT('Ctrl Pts',(6.91596063943906,4.27395233157063,54.7600467535308));
#167584=CARTESIAN_POINT('Ctrl Pts',(6.76548408037174,4.50837071384147,54.7706502379134));
#167585=CARTESIAN_POINT('Ctrl Pts',(6.50139478530221,4.87669166387859,54.7880457239908));
#167586=CARTESIAN_POINT('Ctrl Pts',(6.39495785568427,5.01545300206225,54.7947818405298));
#167587=CARTESIAN_POINT('Ctrl Pts',(6.2488257688162,5.19374291722215,54.8037267873984));
#167588=CARTESIAN_POINT('Ctrl Pts',(6.21308136641001,5.23645002586101,54.8058921952017));
#167589=CARTESIAN_POINT('Ctrl Pts',(6.1552990878859,5.30406318459684,54.8093581709499));
#167590=CARTESIAN_POINT('Ctrl Pts',(6.13354240118779,5.32920732675398,54.8106556001825));
#167591=CARTESIAN_POINT('Ctrl Pts',(6.08808076059829,5.38110003307974,54.8133511958206));
#167592=CARTESIAN_POINT('Ctrl Pts',(6.06435242413952,5.40782715870297,54.8147496004526));
#167593=CARTESIAN_POINT('Ctrl Pts',(6.00756070051975,5.47095237726221,54.8180766800091));
#167594=CARTESIAN_POINT('Ctrl Pts',(5.97434176569944,5.50720854182416,54.8200070548782));
#167595=CARTESIAN_POINT('Ctrl Pts',(5.85357816175083,5.63663504446512,54.8269693346248));
#167596=CARTESIAN_POINT('Ctrl Pts',(5.76416712152762,5.72803708736207,54.8320214866746));
#167597=CARTESIAN_POINT('Ctrl Pts',(5.58711683662652,5.90068481994672,54.8418310596393));
#167598=CARTESIAN_POINT('Ctrl Pts',(5.49976804789478,5.98218246830628,54.8465848177993));
#167599=CARTESIAN_POINT('Ctrl Pts',(5.22557466854112,6.22692564815762,54.8612341714903));
#167600=CARTESIAN_POINT('Ctrl Pts',(5.03302522813126,6.38356416823953,54.8711510601231));
#167601=CARTESIAN_POINT('Ctrl Pts',(4.80191457551451,6.55460593272378,54.8825288926992));
#167602=CARTESIAN_POINT('Ctrl Pts',(4.77004753158206,6.57783316068726,54.8840865404307));
#167603=CARTESIAN_POINT('Ctrl Pts',(4.71857719517437,6.61477808901411,54.8865835918864));
#167604=CARTESIAN_POINT('Ctrl Pts',(4.69908025486382,6.62864274774648,54.8875251893748));
#167605=CARTESIAN_POINT('Ctrl Pts',(4.66432560948276,6.65312706390264,54.8891958274031));
#167606=CARTESIAN_POINT('Ctrl Pts',(4.64909217144247,6.66378084152205,54.8899254406974));
#167607=CARTESIAN_POINT('Ctrl Pts',(4.61601560144214,6.68674490632637,54.8915037931138));
#167608=CARTESIAN_POINT('Ctrl Pts',(4.598159559891,6.69903620970059,54.892352151513));
#167609=CARTESIAN_POINT('Ctrl Pts',(4.54378563311166,6.73614497482338,54.8949245681965));
#167610=CARTESIAN_POINT('Ctrl Pts',(4.50711437256985,6.76073642943636,54.8966445897787));
#167611=CARTESIAN_POINT('Ctrl Pts',(4.42115019818308,6.81737302276155,54.9006440927892));
#167612=CARTESIAN_POINT('Ctrl Pts',(4.37170619913412,6.84918454881104,54.9029198739501));
#167613=CARTESIAN_POINT('Ctrl Pts',(3.96075286205719,7.10732262570993,54.9216494705733));
#167614=CARTESIAN_POINT('Ctrl Pts',(3.58227712442212,7.30540201743851,54.9377415406392));
#167615=CARTESIAN_POINT('Ctrl Pts',(2.81297508839463,7.63380058022156,54.9695405034757));
#167616=CARTESIAN_POINT('Ctrl Pts',(2.42431493264281,7.76597885469104,54.9851957795141));
#167617=CARTESIAN_POINT('Ctrl Pts',(1.95608643892728,7.88662342581524,55.0039757342705));
#167618=CARTESIAN_POINT('Ctrl Pts',(1.88457698294298,7.90401624055325,55.0068410308658));
#167619=CARTESIAN_POINT('Ctrl Pts',(1.77091281975116,7.93003186948286,55.0113924993629));
#167620=CARTESIAN_POINT('Ctrl Pts',(1.72890877170877,7.93929544161359,55.0130738408235));
#167621=CARTESIAN_POINT('Ctrl Pts',(1.65013063668587,7.95601434130762,55.0162262855057));
#167622=CARTESIAN_POINT('Ctrl Pts',(1.6133745850648,7.96354931893501,55.0176967803366));
#167623=CARTESIAN_POINT('Ctrl Pts',(1.53066932644215,7.97990777237776,55.0210049299776));
#167624=CARTESIAN_POINT('Ctrl Pts',(1.48469346556338,7.98858948354417,55.0228434969444));
#167625=CARTESIAN_POINT('Ctrl Pts',(1.3450865663206,8.0137048997076,55.0284254019004));
#167626=CARTESIAN_POINT('Ctrl Pts',(1.25124005771281,8.02889296626107,55.0321764205572));
#167627=CARTESIAN_POINT('Ctrl Pts',(0.766701645013365,8.09860860288,55.0515391838316));
#167628=CARTESIAN_POINT('Ctrl Pts',(0.372689014007289,8.12627747082148,
55.0672063488518));
#167629=CARTESIAN_POINT('Ctrl Pts',(-0.34289161676561,8.12436064912986,
55.096319247919));
#167630=CARTESIAN_POINT('Ctrl Pts',(-0.663673446429851,8.10446396591863,
55.1096228669449));
#167631=CARTESIAN_POINT('Ctrl Pts',(-1.5373082662281,7.9980517858644,55.1466075546246));
#167632=CARTESIAN_POINT('Ctrl Pts',(-2.08372021081485,7.8733883833925,55.1706924029175));
#167633=CARTESIAN_POINT('Ctrl Pts',(-2.68480165772514,7.66924235424176,
55.1964420545646));
#167634=CARTESIAN_POINT('Ctrl Pts',(-2.75626291818493,7.64385068982573,
55.1994877887156));
#167635=CARTESIAN_POINT('Ctrl Pts',(-2.84114273002132,7.6123460051626,55.203078528361));
#167636=CARTESIAN_POINT('Ctrl Pts',(-2.85491217903827,7.60719266011208,
55.2036601754846));
#167637=CARTESIAN_POINT('Ctrl Pts',(-2.87729287426484,7.59874715114003,
55.204604102707));
#167638=CARTESIAN_POINT('Ctrl Pts',(-2.88591260645369,7.59547766635075,
55.2049672913469));
#167639=CARTESIAN_POINT('Ctrl Pts',(-2.90125704990698,7.58962759121779,
55.2056131633811));
#167640=CARTESIAN_POINT('Ctrl Pts',(-2.90798392131558,7.58705271873085,
55.2058960819924));
#167641=CARTESIAN_POINT('Ctrl Pts',(-2.92214022231411,7.58161245976892,
55.2064909777932));
#167642=CARTESIAN_POINT('Ctrl Pts',(-2.92956888516327,7.57874508851252,
55.2068028710785));
#167643=CARTESIAN_POINT('Ctrl Pts',(-2.94914063198376,7.57115756201886,
55.2076238205742));
#167644=CARTESIAN_POINT('Ctrl Pts',(-2.96127662933375,7.56641910174797,
55.2081320878101));
#167645=CARTESIAN_POINT('Ctrl Pts',(-3.01581145079337,7.54497485695481,
55.2104123536861));
#167646=CARTESIAN_POINT('Ctrl Pts',(-3.05808125307775,7.52794151589894,
55.21216969965));
#167647=CARTESIAN_POINT('Ctrl Pts',(-3.39265507183691,7.3898361380272,55.2259858337095));
#167648=CARTESIAN_POINT('Ctrl Pts',(-3.67782491947923,7.25213198888382,
55.2371924239793));
#167649=CARTESIAN_POINT('Ctrl Pts',(-4.44722685057959,6.82351108149312,
55.2673899993585));
#167650=CARTESIAN_POINT('Ctrl Pts',(-4.91025224341217,6.49827517588439,
55.2856005167446));
#167651=CARTESIAN_POINT('Ctrl Pts',(-5.66659133634096,5.83967224588078,
55.3200851109417));
#167652=CARTESIAN_POINT('Ctrl Pts',(-5.97344608767826,5.52538865518179,
55.3358161660439));
#167653=CARTESIAN_POINT('Ctrl Pts',(-6.2737571496323,5.16339736061569,55.3539019320307));
#167654=CARTESIAN_POINT('Ctrl Pts',(-6.29393966021838,5.13877656670567,
55.3551316121641));
#167655=CARTESIAN_POINT('Ctrl Pts',(-6.32187159770565,5.1042907832107,55.3568535728849));
#167656=CARTESIAN_POINT('Ctrl Pts',(-6.32974377103172,5.09452536443244,
55.3573411372647));
#167657=CARTESIAN_POINT('Ctrl Pts',(-6.34329324678662,5.07763737480393,
55.3581842443098));
#167658=CARTESIAN_POINT('Ctrl Pts',(-6.34898125319001,5.070523402047,55.358539377));
#167659=CARTESIAN_POINT('Ctrl Pts',(-6.36072408551017,5.05578593781766,
55.3592750379849));
#167660=CARTESIAN_POINT('Ctrl Pts',(-6.36677719494577,5.04816109986301,
55.3596556307584));
#167661=CARTESIAN_POINT('Ctrl Pts',(-6.38088260977397,5.03032739921414,
55.3605457524435));
#167662=CARTESIAN_POINT('Ctrl Pts',(-6.38892413232806,5.02011006377935,
55.3610556891497));
#167663=CARTESIAN_POINT('Ctrl Pts',(-6.41466302881888,4.98724492173958,
55.3626958628609));
#167664=CARTESIAN_POINT('Ctrl Pts',(-6.43226467724993,4.96452261389915,
55.3638297078879));
#167665=CARTESIAN_POINT('Ctrl Pts',(-6.69254279793944,4.62481663760166,
55.3807798045638));
#167666=CARTESIAN_POINT('Ctrl Pts',(-6.91163133368011,4.29049605428955,
55.397481762485));
#167667=CARTESIAN_POINT('Ctrl Pts',(-7.43295379304438,3.35070995430275,
55.4442273647866));
#167668=CARTESIAN_POINT('Ctrl Pts',(-7.68568069993485,2.72144926764525,
55.47546426592));
#167669=CARTESIAN_POINT('Ctrl Pts',(-7.91968314750162,1.83241794263414,
55.5153206380395));
#167670=CARTESIAN_POINT('Ctrl Pts',(-7.97110905701792,1.59392341402694,
55.5255777670406));
#167671=CARTESIAN_POINT('Ctrl Pts',(-8.01531084491505,1.33226893738488,
55.5361733570518));
#167672=CARTESIAN_POINT('Ctrl Pts',(-8.01880301558406,1.31108606560518,
55.5370269631362));
#167673=CARTESIAN_POINT('Ctrl Pts',(-8.02377739468524,1.28014890325953,
55.5382678151921));
#167674=CARTESIAN_POINT('Ctrl Pts',(-8.0253258401415,1.27040546860291,55.5386577706184));
#167675=CARTESIAN_POINT('Ctrl Pts',(-8.02803401729628,1.25316199048123,
55.539346439498));
#167676=CARTESIAN_POINT('Ctrl Pts',(-8.02920099246855,1.24566310866684,
55.5396454424723));
#167677=CARTESIAN_POINT('Ctrl Pts',(-8.03159842356689,1.23011407745162,
55.5402644375711));
#167678=CARTESIAN_POINT('Ctrl Pts',(-8.03282728697256,1.2220636887081,55.5405843667977));
#167679=CARTESIAN_POINT('Ctrl Pts',(-8.0359559134222,1.20135917002332,55.5414057931157));
#167680=CARTESIAN_POINT('Ctrl Pts',(-8.03783789490505,1.18870234935667,
55.5419066038318));
#167681=CARTESIAN_POINT('Ctrl Pts',(-8.04550795507297,1.13626803710548,
55.543975995905));
#167682=CARTESIAN_POINT('Ctrl Pts',(-8.05103077262727,1.09645194651257,
55.5455346457859));
#167683=CARTESIAN_POINT('Ctrl Pts',(-8.08949968271721,0.803136973157356,
55.556932177959));
#167684=CARTESIAN_POINT('Ctrl Pts',(-8.11076321836762,0.548238389725825,
55.5663763775683));
#167685=CARTESIAN_POINT('Ctrl Pts',(-8.1494928135335,-0.525989991370179,
55.6054683896953));
#167686=CARTESIAN_POINT('Ctrl Pts',(-8.05501936117255,-1.34447685449076,
55.634135299819));
#167687=CARTESIAN_POINT('Ctrl Pts',(-7.81927449074317,-2.21013542941061,
55.6684858824329));
#167688=CARTESIAN_POINT('Ctrl Pts',(-7.79773282169068,-2.2849758915302,
55.6714840406774));
#167689=CARTESIAN_POINT('Ctrl Pts',(-7.76664232282143,-2.38742678497604,
55.6756278248987));
#167690=CARTESIAN_POINT('Ctrl Pts',(-7.75801536502182,-2.41531306677976,
55.6767597791747));
#167691=CARTESIAN_POINT('Ctrl Pts',(-7.74294592405669,-2.46311061742236,
55.6787069143481));
#167692=CARTESIAN_POINT('Ctrl Pts',(-7.73657642861731,-2.48304463455409,
55.6795210518575));
#167693=CARTESIAN_POINT('Ctrl Pts',(-7.72407583305769,-2.52165151156284,
55.6811018465898));
#167694=CARTESIAN_POINT('Ctrl Pts',(-7.71795384489583,-2.54032719669085,
55.6818683647127));
#167695=CARTESIAN_POINT('Ctrl Pts',(-7.70379612539194,-2.58299301474311,
55.6836237854757));
#167696=CARTESIAN_POINT('Ctrl Pts',(-7.69571598805979,-2.60696817790623,
55.6846133063275));
#167697=CARTESIAN_POINT('Ctrl Pts',(-7.67296609160513,-2.67344354111665,
55.6873658459873));
#167698=CARTESIAN_POINT('Ctrl Pts',(-7.65805540371864,-2.71586015961871,
55.6891323500269));
#167699=CARTESIAN_POINT('Ctrl Pts',(-7.6242407406841,-2.809560076873,55.693058418425));
#167700=CARTESIAN_POINT('Ctrl Pts',(-7.60516985278962,-2.86078068651013,
55.6952205065328));
#167701=CARTESIAN_POINT('Ctrl Pts',(-7.45094295529511,-3.26255936846552,
55.7123125074208));
#167702=CARTESIAN_POINT('Ctrl Pts',(-7.29214365340171,-3.6035345337436,
55.7276463139283));
#167703=CARTESIAN_POINT('Ctrl Pts',(-6.7830002427891,-4.52416421359069,
55.7715917645383));
#167704=CARTESIAN_POINT('Ctrl Pts',(-6.38306439301049,-5.07282897109627,
55.8010419421066));
#167705=CARTESIAN_POINT('Ctrl Pts',(-5.90946767918903,-5.5765676541628,
55.8289626428903));
#167706=CARTESIAN_POINT('Ctrl Pts',(-5.89910576315515,-5.58752774051972,
55.82957045944));
#167707=CARTESIAN_POINT('Ctrl Pts',(-5.85913223703797,-5.62957371053287,
55.8319033096499));
#167708=CARTESIAN_POINT('Ctrl Pts',(-5.82930465890093,-5.66045386916352,
55.8336189596199));
#167709=CARTESIAN_POINT('Ctrl Pts',(-5.78967839095846,-5.70083307875243,
55.8358639240323));
#167710=CARTESIAN_POINT('Ctrl Pts',(-5.78009881232172,-5.71054562935977,
55.8364040334341));
#167711=CARTESIAN_POINT('Ctrl Pts',(-5.76521356238555,-5.72556166829836,
55.8372391953913));
#167712=CARTESIAN_POINT('Ctrl Pts',(-5.75992495335559,-5.73088198880345,
55.8375351260863));
#167713=CARTESIAN_POINT('Ctrl Pts',(-5.74933954637718,-5.74150141332026,
55.83812584505));
#167714=CARTESIAN_POINT('Ctrl Pts',(-5.74404277199276,-5.74680053009074,
55.8384206339817));
#167715=CARTESIAN_POINT('Ctrl Pts',(-5.73222283931056,-5.75859302243623,
55.8390766761705));
#167716=CARTESIAN_POINT('Ctrl Pts',(-5.72569595602653,-5.76508266181649,
55.8394377279647));
#167717=CARTESIAN_POINT('Ctrl Pts',(-5.70720188104462,-5.78340881894663,
55.840457325942));
#167718=CARTESIAN_POINT('Ctrl Pts',(-5.69520887529767,-5.79521930130685,
55.8411144404594));
#167719=CARTESIAN_POINT('Ctrl Pts',(-5.60937887075496,-5.87921928882449,
55.8457877036063));
#167720=CARTESIAN_POINT('Ctrl Pts',(-5.53421195294095,-5.95002941592452,
55.8497204248492));
#167721=CARTESIAN_POINT('Ctrl Pts',(-5.3822153303341,-6.08784279986626,
55.8573663618184));
#167722=CARTESIAN_POINT('Ctrl Pts',(-5.30543993508116,-6.15486636356064,
55.8610852528738));
#167723=CARTESIAN_POINT('Ctrl Pts',(-4.91198153066215,-6.48551446248936,
55.8795331863471));
#167724=CARTESIAN_POINT('Ctrl Pts',(-4.57681865562434,-6.72623393890671,
55.8933181545188));
#167725=CARTESIAN_POINT('Ctrl Pts',(-3.63790663158238,-7.29776995294777,
55.9302711589322));
#167726=CARTESIAN_POINT('Ctrl Pts',(-3.00810306977071,-7.5791186369829,
55.953628626276));
#167727=CARTESIAN_POINT('Ctrl Pts',(-2.30904047697838,-7.7903715590882,
55.9815891295643));
#167728=CARTESIAN_POINT('Ctrl Pts',(-2.26755376810707,-7.80254809624716,
55.9832545725002));
#167729=CARTESIAN_POINT('Ctrl Pts',(-2.21072098795639,-7.81873722219118,
55.9855448271214));
#167730=CARTESIAN_POINT('Ctrl Pts',(-2.19545712486625,-7.82303694518714,
55.9861607917615));
#167731=CARTESIAN_POINT('Ctrl Pts',(-2.17124500805291,-7.82978088589587,
55.9871392418767));
#167732=CARTESIAN_POINT('Ctrl Pts',(-2.16230495512371,-7.83225452130359,
55.9875008220774));
#167733=CARTESIAN_POINT('Ctrl Pts',(-2.14497992602915,-7.83701628317341,
55.9882021154146));
#167734=CARTESIAN_POINT('Ctrl Pts',(-2.13659547308613,-7.8393062760449,
55.9885417706599));
#167735=CARTESIAN_POINT('Ctrl Pts',(-2.11665117056621,-7.84471916433469,
55.9893503495815));
#167736=CARTESIAN_POINT('Ctrl Pts',(-2.10508807518004,-7.84782996371639,
55.9898196437291));
#167737=CARTESIAN_POINT('Ctrl Pts',(-2.07081646886335,-7.85696880027689,
55.9912120842996));
#167738=CARTESIAN_POINT('Ctrl Pts',(-2.04808872985772,-7.86292389125557,
55.9921374641323));
#167739=CARTESIAN_POINT('Ctrl Pts',(-1.86563847357267,-7.9098845363327,
55.999582078006));
#167740=CARTESIAN_POINT('Ctrl Pts',(-1.70473351549258,-7.94611603410732,
56.0062467606417));
#167741=CARTESIAN_POINT('Ctrl Pts',(-1.24320039350266,-8.03537705489935,
56.0256574111411));
#167742=CARTESIAN_POINT('Ctrl Pts',(-0.940551602083811,-8.07639597431814,
56.0387456574778));
#167743=CARTESIAN_POINT('Ctrl Pts',(-0.218983071062598,-8.13307983714946,
56.0705906156286));
#167744=CARTESIAN_POINT('Ctrl Pts',(0.200263853118031,-8.13356089963595,
56.089613541702));
#167745=CARTESIAN_POINT('Ctrl Pts',(1.07816644292469,-8.0666315613289,56.1291822371697));
#167746=CARTESIAN_POINT('Ctrl Pts',(1.53491561674973,-7.99231828318995,
56.14959530881));
#167747=CARTESIAN_POINT('Ctrl Pts',(2.01254697376187,-7.87212009879678,
56.1693375757093));
#167748=CARTESIAN_POINT('Ctrl Pts',(2.04212029594849,-7.86450029599521,
56.170553727011));
#167749=CARTESIAN_POINT('Ctrl Pts',(2.08284474932164,-7.85376211394954,
56.1722207175643));
#167750=CARTESIAN_POINT('Ctrl Pts',(2.09403297249518,-7.85078642584977,
56.1726778826741));
#167751=CARTESIAN_POINT('Ctrl Pts',(2.11185495863049,-7.84600557355632,
56.173404878649));
#167752=CARTESIAN_POINT('Ctrl Pts',(2.1184928304322,-7.84421589162311,56.1736753782817));
#167753=CARTESIAN_POINT('Ctrl Pts',(2.13141330219778,-7.84071471854976,
56.1742013818009));
#167754=CARTESIAN_POINT('Ctrl Pts',(2.13769612968913,-7.83900409617749,
56.1744569223436));
#167755=CARTESIAN_POINT('Ctrl Pts',(2.15273871210266,-7.83488903011752,
56.1750681893285));
#167756=CARTESIAN_POINT('Ctrl Pts',(2.16149651632871,-7.83247744252098,
56.1754236160871));
#167757=CARTESIAN_POINT('Ctrl Pts',(2.18781774030315,-7.82518200568449,
56.1764905210807));
#167758=CARTESIAN_POINT('Ctrl Pts',(2.20536885342132,-7.82025371161029,
56.1772001752968));
#167759=CARTESIAN_POINT('Ctrl Pts',(2.34551024136531,-7.78039316920706,
56.1828535174552));
#167760=CARTESIAN_POINT('Ctrl Pts',(2.46728332245264,-7.74263850564397,
56.187686133726));
#167761=CARTESIAN_POINT('Ctrl Pts',(2.85035960308856,-7.61391306115816,
56.2027667160194));
#167762=CARTESIAN_POINT('Ctrl Pts',(3.10793576483658,-7.51245411920426,
56.2127314092396));
#167763=CARTESIAN_POINT('Ctrl Pts',(3.81836550529207,-7.18981095470229,
56.2407122165747));
#167764=CARTESIAN_POINT('Ctrl Pts',(4.25652565444596,-6.93940048920717,
56.2586536535914));
#167765=CARTESIAN_POINT('Ctrl Pts',(5.00822790389797,-6.41166551928036,
56.2927587094915));
#167766=CARTESIAN_POINT('Ctrl Pts',(5.32900554474826,-6.14763984322507,
56.3085862666471));
#167767=CARTESIAN_POINT('Ctrl Pts',(5.70857292842675,-5.78310468659756,
56.328926373727));
#167768=CARTESIAN_POINT('Ctrl Pts',(5.78734592750742,-5.70427309262744,
56.3332485922348));
#167769=CARTESIAN_POINT('Ctrl Pts',(5.89848256171367,-5.58838129907681,
56.3395040260937));
#167770=CARTESIAN_POINT('Ctrl Pts',(5.93217042103995,-5.55260804870382,
56.3414218643622));
#167771=CARTESIAN_POINT('Ctrl Pts',(5.99124531570703,-5.4887249457577,56.3448245520158));
#167772=CARTESIAN_POINT('Ctrl Pts',(6.01676422519282,-5.46073898006491,
56.3463078357722));
#167773=CARTESIAN_POINT('Ctrl Pts',(6.06543322164883,-5.40660953903579,
56.3491630405478));
#167774=CARTESIAN_POINT('Ctrl Pts',(6.08861228823701,-5.3804932178072,56.3505345918358));
#167775=CARTESIAN_POINT('Ctrl Pts',(6.13814215006504,-5.3239570028834,56.353491098669));
#167776=CARTESIAN_POINT('Ctrl Pts',(6.16443672784731,-5.29348911730637,
56.3550766522827));
#167777=CARTESIAN_POINT('Ctrl Pts',(6.2647213375988,-5.17552737701982,56.3611865364457));
#167778=CARTESIAN_POINT('Ctrl Pts',(6.3370833423599,-5.08666800640684,56.3657287357331));
#167779=CARTESIAN_POINT('Ctrl Pts',(6.50787466341803,-4.86763581384776,
56.3767888679848));
#167780=CARTESIAN_POINT('Ctrl Pts',(6.60430830654675,-4.73597105989008,
56.3833256951038));
#167781=CARTESIAN_POINT('Ctrl Pts',(7.01254854543007,-4.1418450403868,56.4123545398637));
#167782=CARTESIAN_POINT('Ctrl Pts',(7.28022082534449,-3.65090335351244,
56.4351960478313));
#167783=CARTESIAN_POINT('Ctrl Pts',(7.5438338686116,-3.02091686176344,56.4626326684866));
#167784=CARTESIAN_POINT('Ctrl Pts',(7.58949460401749,-2.90429690182776,
56.4676346598135));
#167785=CARTESIAN_POINT('Ctrl Pts',(7.6438482206309,-2.75542700515786,56.4739103569023));
#167786=CARTESIAN_POINT('Ctrl Pts',(7.65506235796125,-2.7241170888217,56.475224184652));
#167787=CARTESIAN_POINT('Ctrl Pts',(7.67193958023488,-2.67606854074539,
56.4772308200315));
#167788=CARTESIAN_POINT('Ctrl Pts',(7.67774077721127,-2.65937893480693,
56.4779260487926));
#167789=CARTESIAN_POINT('Ctrl Pts',(7.68931437094285,-2.62572904746364,
56.4793242356882));
#167790=CARTESIAN_POINT('Ctrl Pts',(7.6950851883416,-2.60876838234592,56.4800271776854));
#167791=CARTESIAN_POINT('Ctrl Pts',(7.70683181963275,-2.57386644163167,
56.4814702067843));
#167792=CARTESIAN_POINT('Ctrl Pts',(7.71280119168006,-2.55592310838589,
56.4822101850719));
#167793=CARTESIAN_POINT('Ctrl Pts',(7.72171698176592,-2.52880747040263,
56.483325725167));
#167794=CARTESIAN_POINT('Ctrl Pts',(7.72470980743395,-2.5196505234156,56.4837019788923));
#167795=CARTESIAN_POINT('Ctrl Pts',(7.74835873990877,-2.44685530865725,
56.4866895129049));
#167796=CARTESIAN_POINT('Ctrl Pts',(7.76824449742634,-2.3829690706462,56.4892897268689));
#167797=CARTESIAN_POINT('Ctrl Pts',(7.82714837271466,-2.18515308620252,
56.4972873416449));
#167798=CARTESIAN_POINT('Ctrl Pts',(7.86350860015525,-2.05045814927303,
56.5026581446648));
#167799=CARTESIAN_POINT('Ctrl Pts',(7.96321282977818,-1.63931106426365,
56.5189282563003));
#167800=CARTESIAN_POINT('Ctrl Pts',(8.01556938038562,-1.36042112700604,
56.5298048188836));
#167801=CARTESIAN_POINT('Ctrl Pts',(8.06217360284147,-1.01270340509562,
56.5434073140678));
#167802=CARTESIAN_POINT('Ctrl Pts',(8.07028029365234,-0.945931978640632,
56.5460207023135));
#167803=CARTESIAN_POINT('Ctrl Pts',(8.08180460768298,-0.840037644324885,
56.5501698536874));
#167804=CARTESIAN_POINT('Ctrl Pts',(8.08576925024965,-0.800977264886989,
56.5517012806729));
#167805=CARTESIAN_POINT('Ctrl Pts',(8.09265254853609,-0.72789306859219,
56.5545689145146));
#167806=CARTESIAN_POINT('Ctrl Pts',(8.095640114529,-0.693876586676744,56.5559045404415));
#167807=CARTESIAN_POINT('Ctrl Pts',(8.10118014524423,-0.625882379252799,
56.5585763387248));
#167808=CARTESIAN_POINT('Ctrl Pts',(8.10373348998193,-0.591905408462573,
56.5599124769073));
#167809=CARTESIAN_POINT('Ctrl Pts',(8.10909810953572,-0.513961422844948,
56.562980201026));
#167810=CARTESIAN_POINT('Ctrl Pts',(8.11176565111623,-0.469985633929632,
56.5647128937034));
#167811=CARTESIAN_POINT('Ctrl Pts',(8.12151373445906,-0.284308500723278,
56.5720373795651));
#167812=CARTESIAN_POINT('Ctrl Pts',(8.12523976150824,-0.142458168230421,
56.5776547667235));
#167813=CARTESIAN_POINT('Ctrl Pts',(8.12524997892878,-0.000585164859018793,
56.5832945039328));
#167814=CARTESIAN_POINT('',(8.12525,-6.37027323252548E-13,58.5832974432124));
#167815=CARTESIAN_POINT('Ctrl Pts',(8.12525,-4.61836819862331E-13,56.5832974432124));
#167816=CARTESIAN_POINT('Ctrl Pts',(8.12525000000013,2.24624642433368,56.6712950363536));
#167817=CARTESIAN_POINT('Ctrl Pts',(7.14398562317623,4.47535249753416,56.7592926294948));
#167818=CARTESIAN_POINT('Ctrl Pts',(3.83078204044967,7.50935546634344,56.9352878157772));
#167819=CARTESIAN_POINT('Ctrl Pts',(1.52412477697781,8.29110090552131,57.0232854089184));
#167820=CARTESIAN_POINT('Ctrl Pts',(-2.95101623932528,7.89663306204438,
57.1992805952008));
#167821=CARTESIAN_POINT('Ctrl Pts',(-5.08535169588709,6.72342983085807,
57.287278188342));
#167822=CARTESIAN_POINT('Ctrl Pts',(-7.81671694684393,3.1566195105297,57.4632733746244));
#167823=CARTESIAN_POINT('Ctrl Pts',(-8.392904611467,0.790229551554399,57.5512709677656));
#167824=CARTESIAN_POINT('Ctrl Pts',(-7.60701611462495,-3.63299000730394,
57.727266154048));
#167825=CARTESIAN_POINT('Ctrl Pts',(-6.25093680401372,-5.65606750610003,
57.8152637471892));
#167826=CARTESIAN_POINT('Ctrl Pts',(-2.45807268688572,-8.06369575488313,
57.9912589334716));
#167827=CARTESIAN_POINT('Ctrl Pts',(-0.0502299510454843,-8.42987470330086,
58.0792565266128));
#167828=CARTESIAN_POINT('Ctrl Pts',(4.2868996088099,-7.25863639434566,58.2552517128952));
#167829=CARTESIAN_POINT('Ctrl Pts',(6.18309125557158,-5.73015646266383,
58.3432493060364));
#167830=CARTESIAN_POINT('Ctrl Pts',(7.81050559202891,-2.5864071380029,58.4819304138558));
#167831=CARTESIAN_POINT('Ctrl Pts',(8.1252499999999,-1.29375883538193,58.5326139285341));
#167832=CARTESIAN_POINT('Ctrl Pts',(8.12525,-6.37027053055327E-13,58.5832974432124));
#167833=CARTESIAN_POINT('',(8.1189210508199,-0.00515126165391927,62.5832974432123));
#167834=CARTESIAN_POINT('Ctrl Pts',(8.12524831310126,0.00523573729693267,
58.5811705099486));
#167835=CARTESIAN_POINT('Ctrl Pts',(8.12517639820438,0.116839196648762,
58.5855840757637));
#167836=CARTESIAN_POINT('Ctrl Pts',(8.12280511641629,0.228429150564323,
58.5900170165289));
#167837=CARTESIAN_POINT('Ctrl Pts',(8.09554846868868,0.879357742915142,
58.6160064250618));
#167838=CARTESIAN_POINT('Ctrl Pts',(8.01925291345264,1.41518046884007,58.6379906428653));
#167839=CARTESIAN_POINT('Ctrl Pts',(7.8456709357679,2.12137481707722,58.6674904038425));
#167840=CARTESIAN_POINT('Ctrl Pts',(7.79467526836033,2.30169989202382,58.6750639744105));
#167841=CARTESIAN_POINT('Ctrl Pts',(7.71662152594249,2.54521411760971,58.6853079485774));
#167842=CARTESIAN_POINT('Ctrl Pts',(7.69493002073038,2.61006030061168,58.6880373903059));
#167843=CARTESIAN_POINT('Ctrl Pts',(7.66101751902347,2.7073416043261,58.6921318486831));
#167844=CARTESIAN_POINT('Ctrl Pts',(7.64940336487783,2.73998470227198,58.693505721117));
#167845=CARTESIAN_POINT('Ctrl Pts',(7.63013644960529,2.7930594821971,58.6957390767557));
#167846=CARTESIAN_POINT('Ctrl Pts',(7.62260958606683,2.81353631822115,58.6966006228165));
#167847=CARTESIAN_POINT('Ctrl Pts',(7.60904562803237,2.84998309925561,58.6981337943674));
#167848=CARTESIAN_POINT('Ctrl Pts',(7.60304050095886,2.86596479045633,58.6988059757282));
#167849=CARTESIAN_POINT('Ctrl Pts',(7.59040562475238,2.89927130679426,58.7002065697299));
#167850=CARTESIAN_POINT('Ctrl Pts',(7.58376683666184,2.91659257162282,58.7009348254452));
#167851=CARTESIAN_POINT('Ctrl Pts',(7.56855970114562,2.95586652972008,58.7025859823375));
#167852=CARTESIAN_POINT('Ctrl Pts',(7.55995504196469,2.97780500712256,58.7035082647737));
#167853=CARTESIAN_POINT('Ctrl Pts',(7.53716482510704,3.03517554669036,58.7059204603003));
#167854=CARTESIAN_POINT('Ctrl Pts',(7.52282481877938,3.07054571155132,58.7074080005668));
#167855=CARTESIAN_POINT('Ctrl Pts',(7.44326500322929,3.26287981344836,58.7155032849761));
#167856=CARTESIAN_POINT('Ctrl Pts',(7.37338074734861,3.41787009532359,58.7220513151932));
#167857=CARTESIAN_POINT('Ctrl Pts',(7.20307136067912,3.76600494777748,58.7369582573678));
#167858=CARTESIAN_POINT('Ctrl Pts',(7.0996444986761,3.95753433021788,58.745306083062));
#167859=CARTESIAN_POINT('Ctrl Pts',(6.93023548385204,4.24318749720711,58.7581288463335));
#167860=CARTESIAN_POINT('Ctrl Pts',(6.8697395515003,4.34044723752279,58.7625632697958));
#167861=CARTESIAN_POINT('Ctrl Pts',(6.7813201258849,4.4761180747232,58.7688597814188));
#167862=CARTESIAN_POINT('Ctrl Pts',(6.75508479004031,4.51561348265956,58.7707063442652));
#167863=CARTESIAN_POINT('Ctrl Pts',(6.70963848219389,4.58274717955366,58.7738692413421));
#167864=CARTESIAN_POINT('Ctrl Pts',(6.69059868554859,4.6104999179843,58.7751839201951));
#167865=CARTESIAN_POINT('Ctrl Pts',(6.65025187452325,4.66853386462594,58.7779484252841));
#167866=CARTESIAN_POINT('Ctrl Pts',(6.62890920167816,4.69878933598517,58.7793985716873));
#167867=CARTESIAN_POINT('Ctrl Pts',(6.57387285159557,4.77568780614257,58.7831075219588));
#167868=CARTESIAN_POINT('Ctrl Pts',(6.5398892255511,4.82212060867021,58.7853691163673));
#167869=CARTESIAN_POINT('Ctrl Pts',(6.36558813767213,5.05504113104128,58.7968281630274));
#167870=CARTESIAN_POINT('Ctrl Pts',(6.21777712093239,5.23578059801488,58.8060992719619));
#167871=CARTESIAN_POINT('Ctrl Pts',(5.94843837352386,5.53760430764653,58.8222394875947));
#167872=CARTESIAN_POINT('Ctrl Pts',(5.8304767478359,5.66167125450615,58.8290847258098));
#167873=CARTESIAN_POINT('Ctrl Pts',(5.63631903988984,5.85336972774976,58.8399678629975));
#167874=CARTESIAN_POINT('Ctrl Pts',(5.56261740700668,5.92345484252977,58.8440164441594));
#167875=CARTESIAN_POINT('Ctrl Pts',(5.4551653617551,6.02185976800279,58.8497915404399));
#167876=CARTESIAN_POINT('Ctrl Pts',(5.42247032911268,6.05131719103418,58.8515323651981));
#167877=CARTESIAN_POINT('Ctrl Pts',(5.37054119072963,6.09734526217226,58.8542704580458));
#167878=CARTESIAN_POINT('Ctrl Pts',(5.35146604192433,6.1140938114996,58.8552706191594));
#167879=CARTESIAN_POINT('Ctrl Pts',(5.31833511189125,6.1429099268764,58.8569978108813));
#167880=CARTESIAN_POINT('Ctrl Pts',(5.30431597924443,6.15501931180698,58.8577256047691));
#167881=CARTESIAN_POINT('Ctrl Pts',(5.27678165517953,6.17863885185846,58.8591489703175));
#167882=CARTESIAN_POINT('Ctrl Pts',(5.26326993962654,6.190152844888,58.8598446303911));
#167883=CARTESIAN_POINT('Ctrl Pts',(5.23269824573322,6.21603201615392,58.8614124453043));
#167884=CARTESIAN_POINT('Ctrl Pts',(5.21561662497796,6.23037143212756,58.8622841278934));
#167885=CARTESIAN_POINT('Ctrl Pts',(5.16910103062298,6.26909427178939,58.8646465134454));
#167886=CARTESIAN_POINT('Ctrl Pts',(5.13955363439077,6.29334067977217,58.8661349215696));
#167887=CARTESIAN_POINT('Ctrl Pts',(4.97341868307297,6.42771959657778,58.8744394122587));
#167888=CARTESIAN_POINT('Ctrl Pts',(4.83346157034619,6.53361484987605,58.8811950796788));
#167889=CARTESIAN_POINT('Ctrl Pts',(4.67850676352344,6.64315185392802,58.8884819117514));
#167890=CARTESIAN_POINT('Ctrl Pts',(4.66680683580172,6.65137625219593,58.8890309448283));
#167891=CARTESIAN_POINT('Ctrl Pts',(4.38269759554519,6.84997057429744,58.9023356537205));
#167892=CARTESIAN_POINT('Ctrl Pts',(4.09888596099478,7.02347977651387,58.9150289364623));
#167893=CARTESIAN_POINT('Ctrl Pts',(3.65446067558194,7.25904468311497,58.9344345847304));
#167894=CARTESIAN_POINT('Ctrl Pts',(3.50119302349636,7.33419792147085,58.9410450961357));
#167895=CARTESIAN_POINT('Ctrl Pts',(3.28159910007937,7.4334203897415,58.9504284333985));
#167896=CARTESIAN_POINT('Ctrl Pts',(3.21715146298764,7.4615392346003,58.9531717537745));
#167897=CARTESIAN_POINT('Ctrl Pts',(3.10374022027842,7.50927862605939,58.9579821030075));
#167898=CARTESIAN_POINT('Ctrl Pts',(3.05493529813128,7.52926551130056,58.9600466663165));
#167899=CARTESIAN_POINT('Ctrl Pts',(2.95163296167352,7.57040073213325,58.9644053616558));
#167900=CARTESIAN_POINT('Ctrl Pts',(2.89709489965346,7.59143896106725,58.9666999981994));
#167901=CARTESIAN_POINT('Ctrl Pts',(2.72414353771271,7.65602027560811,58.9739563878941));
#167902=CARTESIAN_POINT('Ctrl Pts',(2.60494088674676,7.69739483554199,58.9789279968587));
#167903=CARTESIAN_POINT('Ctrl Pts',(2.34134770668796,7.78206191617339,58.9898521127108));
#167904=CARTESIAN_POINT('Ctrl Pts',(2.19661740383074,7.82414651867458,58.9958054318505));
#167905=CARTESIAN_POINT('Ctrl Pts',(1.9922889655688,7.8774443066285,59.0041331661356));
#167906=CARTESIAN_POINT('Ctrl Pts',(1.93360857502958,7.8920530934995,59.0065159067674));
#167907=CARTESIAN_POINT('Ctrl Pts',(1.87346085416673,7.90631607020695,59.0089481548735));
#167908=CARTESIAN_POINT('Ctrl Pts',(1.87215113534358,7.9066263033319,59.0090011122884));
#167909=CARTESIAN_POINT('Ctrl Pts',(1.86953208979945,7.90724598945849,59.0091070014892));
#167910=CARTESIAN_POINT('Ctrl Pts',(1.86822276318755,7.90755544272094,59.0091599332747));
#167911=CARTESIAN_POINT('Ctrl Pts',(1.8656041969171,7.90817364202238,59.0092657835395));
#167912=CARTESIAN_POINT('Ctrl Pts',(1.86429495732805,7.90848238817119,59.0093187020179));
#167913=CARTESIAN_POINT('Ctrl Pts',(1.86167624904031,7.90909924807504,59.0094245384235));
#167914=CARTESIAN_POINT('Ctrl Pts',(1.86036678037349,7.90940736178287,59.0094774563488));
#167915=CARTESIAN_POINT('Ctrl Pts',(1.85774728717747,7.91002303348357,59.0095833048255));
#167916=CARTESIAN_POINT('Ctrl Pts',(1.85643726262336,7.91033059127112,59.0096362353749));
#167917=CARTESIAN_POINT('Ctrl Pts',(1.85470348126303,7.91073718110188,59.0097062809692));
#167918=CARTESIAN_POINT('Ctrl Pts',(1.85427979291708,7.91083650453328,59.0097233976647));
#167919=CARTESIAN_POINT('Ctrl Pts',(1.85339565177952,7.91104369499479,59.0097591152349));
#167920=CARTESIAN_POINT('Ctrl Pts',(1.85293519751876,7.91115155587025,59.0097777160754));
#167921=CARTESIAN_POINT('Ctrl Pts',(1.85197463397678,7.91137647830131,59.0098165184163));
#167922=CARTESIAN_POINT('Ctrl Pts',(1.85147452301665,7.91149353263548,59.0098367198748));
#167923=CARTESIAN_POINT('Ctrl Pts',(1.85043157463926,7.91173753741028,59.00987884718));
#167924=CARTESIAN_POINT('Ctrl Pts',(1.84988873526236,7.91186447940296,59.0099007729775));
#167925=CARTESIAN_POINT('Ctrl Pts',(1.84875707272207,7.91212899377904,59.0099464801304));
#167926=CARTESIAN_POINT('Ctrl Pts',(1.84816824723772,7.91226655630618,59.0099702614295));
#167927=CARTESIAN_POINT('Ctrl Pts',(1.84694116460128,7.91255308522884,59.0100198183735));
#167928=CARTESIAN_POINT('Ctrl Pts',(1.84630290477098,7.91270204013126,59.0100455939515));
#167929=CARTESIAN_POINT('Ctrl Pts',(1.84497331089033,7.91301216658495,59.0100992860132));
#167930=CARTESIAN_POINT('Ctrl Pts',(1.84428197373153,7.91317332476599,59.0101272024187));
#167931=CARTESIAN_POINT('Ctrl Pts',(1.84284238426513,7.91350870976285,59.0101853306024));
#167932=CARTESIAN_POINT('Ctrl Pts',(1.84209412833682,7.91368292106043,59.0102155422902));
#167933=CARTESIAN_POINT('Ctrl Pts',(1.84053665857069,7.91404530320573,59.0102784235363));
#167934=CARTESIAN_POINT('Ctrl Pts',(1.83972744055999,7.91423345607052,59.0103110929886));
#167935=CARTESIAN_POINT('Ctrl Pts',(1.8380437987702,7.91462465074278,59.0103790604062));
#167936=CARTESIAN_POINT('Ctrl Pts',(1.83716937017526,7.91482767175841,59.0104143582479));
#167937=CARTESIAN_POINT('Ctrl Pts',(1.83535085093715,7.91524957001853,59.0104877613445));
#167938=CARTESIAN_POINT('Ctrl Pts',(1.83440675472972,7.91546842327834,59.0105258664567));
#167939=CARTESIAN_POINT('Ctrl Pts',(1.83244423187037,7.91592299055131,59.0106050713787));
#167940=CARTESIAN_POINT('Ctrl Pts',(1.83142579884042,7.91615867694652,59.0106461710223));
#167941=CARTESIAN_POINT('Ctrl Pts',(1.82930971754439,7.91664795155981,59.010731560823));
#167942=CARTESIAN_POINT('Ctrl Pts',(1.82821206193691,7.91690150805397,59.0107758507886));
#167943=CARTESIAN_POINT('Ctrl Pts',(1.82593242896765,7.91742759983886,59.0108678257664));
#167944=CARTESIAN_POINT('Ctrl Pts',(1.82475044324223,7.91770009874921,59.0109155105558));
#167945=CARTESIAN_POINT('Ctrl Pts',(1.82229681518712,7.91826518768737,59.0110144886661));
#167946=CARTESIAN_POINT('Ctrl Pts',(1.82102516329836,7.91855773609168,59.0110657817302));
#167947=CARTESIAN_POINT('Ctrl Pts',(1.81838663144945,7.9191640712823,59.0111721991246));
#167948=CARTESIAN_POINT('Ctrl Pts',(1.8170197405945,7.91947781053858,59.0112273231591));
#167949=CARTESIAN_POINT('Ctrl Pts',(1.81418491251236,7.92012770942205,59.0113416348503));
#167950=CARTESIAN_POINT('Ctrl Pts',(1.81271696291293,7.92046381487289,59.011400822166));
#167951=CARTESIAN_POINT('Ctrl Pts',(1.80967394008507,7.92115966278591,59.0115235028407));
#167952=CARTESIAN_POINT('Ctrl Pts',(1.8080988528043,7.92151934361447,59.0115869958082));
#167953=CARTESIAN_POINT('Ctrl Pts',(1.80483520448675,7.92226359358714,59.0117185407826));
#167954=CARTESIAN_POINT('Ctrl Pts',(1.80314662755011,7.92264809272674,59.0117865923393));
#167955=CARTESIAN_POINT('Ctrl Pts',(1.76554242181326,7.93119815210983,59.0133018963152));
#167956=CARTESIAN_POINT('Ctrl Pts',(1.7295717167814,7.93911996776487,59.0147475443942));
#167957=CARTESIAN_POINT('Ctrl Pts',(1.64670008571176,7.9567808076879,59.0180688043332));
#167958=CARTESIAN_POINT('Ctrl Pts',(1.59976440767895,7.96635022167018,59.0199431663738));
#167959=CARTESIAN_POINT('Ctrl Pts',(1.2743947319643,8.02969627556278,59.0328983584521));
#167960=CARTESIAN_POINT('Ctrl Pts',(0.993395927647598,8.06927937728133,
59.0438996042274));
#167961=CARTESIAN_POINT('Ctrl Pts',(0.626014712685072,8.10154644718201,
59.0582869832803));
#167962=CARTESIAN_POINT('Ctrl Pts',(0.541014108906461,8.10766630546251,
59.0616154960695));
#167963=CARTESIAN_POINT('Ctrl Pts',(0.402785371362971,8.11543499276543,
59.0670337438848));
#167964=CARTESIAN_POINT('Ctrl Pts',(0.34960956935855,8.11789962395833,59.0691193917072));
#167965=CARTESIAN_POINT('Ctrl Pts',(0.269876817884071,8.12081025510544,
59.0722496580054));
#167966=CARTESIAN_POINT('Ctrl Pts',(0.24333557722588,8.12164887754905,59.0732921508082));
#167967=CARTESIAN_POINT('Ctrl Pts',(0.208106929980383,8.12258915188453,
59.0746766355035));
#167968=CARTESIAN_POINT('Ctrl Pts',(0.199422766000694,8.12280700157982,
59.0750179845692));
#167969=CARTESIAN_POINT('Ctrl Pts',(0.118948716521843,8.12469663109209,
59.0781817799492));
#167970=CARTESIAN_POINT('Ctrl Pts',(0.0471401921666107,8.12543056615178,
59.0810093219135));
#167971=CARTESIAN_POINT('Ctrl Pts',(-0.20714062953554,8.12465856179557,
59.0910420715853));
#167972=CARTESIAN_POINT('Ctrl Pts',(-0.389540940211746,8.11795792411037,
59.0982766459217));
#167973=CARTESIAN_POINT('Ctrl Pts',(-0.942294311702755,8.07897870548056,
59.1203444063101));
#167974=CARTESIAN_POINT('Ctrl Pts',(-1.31079637625268,8.02742959643593,
59.135269770985));
#167975=CARTESIAN_POINT('Ctrl Pts',(-1.76517645901725,7.93173574998711,
59.1537872496946));
#167976=CARTESIAN_POINT('Ctrl Pts',(-1.8555487450105,7.91108203533322,59.1574746838856));
#167977=CARTESIAN_POINT('Ctrl Pts',(-1.98785592553225,7.87845258841415,
59.1628733588026));
#167978=CARTESIAN_POINT('Ctrl Pts',(-2.03007914073925,7.86767850619569,
59.1645962537011));
#167979=CARTESIAN_POINT('Ctrl Pts',(-2.09781448000107,7.84981292515265,
59.1673593458153));
#167980=CARTESIAN_POINT('Ctrl Pts',(-2.12338208731236,7.84293548809502,
59.1684021243841));
#167981=CARTESIAN_POINT('Ctrl Pts',(-2.1680709757334,7.83068006799212,59.170224222229));
#167982=CARTESIAN_POINT('Ctrl Pts',(-2.18720698095181,7.82535671446688,
59.1710042780461));
#167983=CARTESIAN_POINT('Ctrl Pts',(-2.22551015953701,7.81454986113021,
59.172565199465));
#167984=CARTESIAN_POINT('Ctrl Pts',(-2.24467706129464,7.80906587859042,
59.173346052295));
#167985=CARTESIAN_POINT('Ctrl Pts',(-2.28479759050127,7.79742678469476,
59.1749799438289));
#167986=CARTESIAN_POINT('Ctrl Pts',(-2.30574690615566,7.79125764567903,
59.1758327192332));
#167987=CARTESIAN_POINT('Ctrl Pts',(-2.36789795393136,7.77268282505951,
59.17836169248));
#167988=CARTESIAN_POINT('Ctrl Pts',(-2.40902633978774,7.76003422317414,
59.1800340612331));
#167989=CARTESIAN_POINT('Ctrl Pts',(-2.62815632246915,7.69073309558562,
59.1889442195982));
#167990=CARTESIAN_POINT('Ctrl Pts',(-2.80426671610509,7.62828098713956,
59.1961062011256));
#167991=CARTESIAN_POINT('Ctrl Pts',(-3.1270413609876,7.50112901419255,59.2093880004823));
#167992=CARTESIAN_POINT('Ctrl Pts',(-3.27424594026636,7.43805334788783,
59.2155073190374));
#167993=CARTESIAN_POINT('Ctrl Pts',(-3.53748853251465,7.31592665324726,
59.2266361830694));
#167994=CARTESIAN_POINT('Ctrl Pts',(-3.65415432155833,7.25835820050681,
59.2316367364208));
#167995=CARTESIAN_POINT('Ctrl Pts',(-3.85206786767999,7.15471672900817,
59.2402649880761));
#167996=CARTESIAN_POINT('Ctrl Pts',(-3.93399596570049,7.10999816416011,
59.2438806966601));
#167997=CARTESIAN_POINT('Ctrl Pts',(-4.05361217227407,7.04200786180014,
59.2492308977332));
#167998=CARTESIAN_POINT('Ctrl Pts',(-4.09190982239516,7.0198233847916,59.2509548245374));
#167999=CARTESIAN_POINT('Ctrl Pts',(-4.15902370420061,6.98021083709141,
59.2539957817299));
#168000=CARTESIAN_POINT('Ctrl Pts',(-4.18791645523312,6.9629144226491,59.2553114960037));
#168001=CARTESIAN_POINT('Ctrl Pts',(-4.2497020330876,6.92540328801208,59.2581394609702));
#168002=CARTESIAN_POINT('Ctrl Pts',(-4.28255997790765,6.90513273539684,
59.2596522308104));
#168003=CARTESIAN_POINT('Ctrl Pts',(-4.37032702626561,6.85012051796895,
59.2637171308492));
#168004=CARTESIAN_POINT('Ctrl Pts',(-4.42496579079804,6.81495319969432,
59.2662733153385));
#168005=CARTESIAN_POINT('Ctrl Pts',(-4.65862133612102,6.66057000033471,
59.2773168565769));
#168006=CARTESIAN_POINT('Ctrl Pts',(-4.83328585317899,6.53492858624563,
59.2858633508653));
#168007=CARTESIAN_POINT('Ctrl Pts',(-5.14542407679601,6.29103163774024,
59.3016535114714));
#168008=CARTESIAN_POINT('Ctrl Pts',(-5.28432440690271,6.17481851671146,
59.3088842936542));
#168009=CARTESIAN_POINT('Ctrl Pts',(-5.46507540606076,6.01302127662469,
59.3185288515002));
#168010=CARTESIAN_POINT('Ctrl Pts',(-5.51045682054391,5.97146043681014,
59.3209710186146));
#168011=CARTESIAN_POINT('Ctrl Pts',(-5.57888727382927,5.90734657992605,
59.324682536134));
#168012=CARTESIAN_POINT('Ctrl Pts',(-5.60228133131514,5.88516530987907,
59.3259566494335));
#168013=CARTESIAN_POINT('Ctrl Pts',(-5.6435284955051,5.84558765187151,59.3282119643844));
#168014=CARTESIAN_POINT('Ctrl Pts',(-5.66143470810622,5.82824724310359,
59.3291940470956));
#168015=CARTESIAN_POINT('Ctrl Pts',(-5.69330490854421,5.79709862086708,
59.3309471322092));
#168016=CARTESIAN_POINT('Ctrl Pts',(-5.7072991557919,5.78332167107031,59.3317187046542));
#168017=CARTESIAN_POINT('Ctrl Pts',(-5.73329025026406,5.75754794224224,
59.3331549323709));
#168018=CARTESIAN_POINT('Ctrl Pts',(-5.74529972021392,5.74556407403909,
59.3338198388954));
#168019=CARTESIAN_POINT('Ctrl Pts',(-5.77398545076476,5.71675962397565,
59.3354110584742));
#168020=CARTESIAN_POINT('Ctrl Pts',(-5.79062585951541,5.69990357328113,
59.336336614615));
#168021=CARTESIAN_POINT('Ctrl Pts',(-5.85388624917053,5.63526044983365,
59.3398653112408));
#168022=CARTESIAN_POINT('Ctrl Pts',(-5.89999058582909,5.58697196639273,
59.3424581262394));
#168023=CARTESIAN_POINT('Ctrl Pts',(-5.95571411938024,5.52714950828046,
59.3456216211734));
#168024=CARTESIAN_POINT('Ctrl Pts',(-5.96590302162596,5.51615024236272,
59.3462012976702));
#168025=CARTESIAN_POINT('Ctrl Pts',(-6.26436743077006,5.19215353939417,
59.3632192968626));
#168026=CARTESIAN_POINT('Ctrl Pts',(-6.52764693208651,4.85701489405826,
59.3792790636033));
#168027=CARTESIAN_POINT('Ctrl Pts',(-6.99716044568987,4.15177805421225,
59.4114802274014));
#168028=CARTESIAN_POINT('Ctrl Pts',(-7.2031682621337,3.78310348790634,59.4275758609787));
#168029=CARTESIAN_POINT('Ctrl Pts',(-7.40190662686562,3.35176079300264,
59.4460235178255));
#168030=CARTESIAN_POINT('Ctrl Pts',(-7.42370998418252,3.30318818206961,
59.4480952492352));
#168031=CARTESIAN_POINT('Ctrl Pts',(-7.46051997127221,3.21897874192921,
59.4516779830287));
#168032=CARTESIAN_POINT('Ctrl Pts',(-7.47575253349082,3.18344254369155,
59.4531871529378));
#168033=CARTESIAN_POINT('Ctrl Pts',(-7.5055482448697,3.11253850860205,59.456193162822));
#168034=CARTESIAN_POINT('Ctrl Pts',(-7.52011645598667,3.07717384962502,
59.4576899235039));
#168035=CARTESIAN_POINT('Ctrl Pts',(-7.54849214588069,3.00688610544065,
59.4606599320223));
#168036=CARTESIAN_POINT('Ctrl Pts',(-7.56230829711621,2.97196751944103,
59.4621330770831));
#168037=CARTESIAN_POINT('Ctrl Pts',(-7.59294888873917,2.89293003211595,
59.4654624123954));
#168038=CARTESIAN_POINT('Ctrl Pts',(-7.60963180729591,2.84875775306758,
59.4673195440113));
#168039=CARTESIAN_POINT('Ctrl Pts',(-7.66709289784579,2.69250774835765,
59.4738766236124));
#168040=CARTESIAN_POINT('Ctrl Pts',(-7.70578737788031,2.57968061904721,
59.4785897004082));
#168041=CARTESIAN_POINT('Ctrl Pts',(-7.93796827582238,1.8507636398737,59.5089030704495));
#168042=CARTESIAN_POINT('Ctrl Pts',(-8.05989870723231,1.214348575592,59.5348486980382));
#168043=CARTESIAN_POINT('Ctrl Pts',(-8.14252652616689,0.039914066182005,
59.5842067721203));
#168044=CARTESIAN_POINT('Ctrl Pts',(-8.12769819033082,-0.492782213575494,
59.6070710319487));
#168045=CARTESIAN_POINT('Ctrl Pts',(-8.04442315318636,-1.15076697046135,
59.6343405564969));
#168046=CARTESIAN_POINT('Ctrl Pts',(-8.02472805810492,-1.28091764975282,
59.6396779210998));
#168047=CARTESIAN_POINT('Ctrl Pts',(-7.9987968435175,-1.42802379475317,
59.645606815264));
#168048=CARTESIAN_POINT('Ctrl Pts',(-7.99565676758626,-1.44550190702236,
59.6463095647355));
#168049=CARTESIAN_POINT('Ctrl Pts',(-7.99084120059462,-1.47181019253954,
59.6473646815934));
#168050=CARTESIAN_POINT('Ctrl Pts',(-7.98920832673511,-1.48064805029021,
59.6477186770873));
#168051=CARTESIAN_POINT('Ctrl Pts',(-7.9863696512218,-1.49587084245384,
59.6483276132234));
#168052=CARTESIAN_POINT('Ctrl Pts',(-7.98517084967779,-1.50225706356726,
59.6485828282269));
#168053=CARTESIAN_POINT('Ctrl Pts',(-7.98268105076628,-1.51543346180957,
59.6491088882593));
#168054=CARTESIAN_POINT('Ctrl Pts',(-7.98138904706195,-1.52222344457988,
59.6493796928077));
#168055=CARTESIAN_POINT('Ctrl Pts',(-7.97824966358184,-1.53860824807813,
59.6500324738051));
#168056=CARTESIAN_POINT('Ctrl Pts',(-7.9763936345962,-1.54820141537254,
59.6504140975156));
#168057=CARTESIAN_POINT('Ctrl Pts',(-7.96948600636523,-1.5835623932717,
59.6518186080484));
#168058=CARTESIAN_POINT('Ctrl Pts',(-7.96432677457999,-1.60930920234527,
59.6528369868329));
#168059=CARTESIAN_POINT('Ctrl Pts',(-7.8818453352122,-2.01081437587897,
59.6686464048692));
#168060=CARTESIAN_POINT('Ctrl Pts',(-7.77812968353715,-2.3806656808802,
59.6821215020093));
#168061=CARTESIAN_POINT('Ctrl Pts',(-7.4645410449366,-3.25546685099195,
59.7137134929888));
#168062=CARTESIAN_POINT('Ctrl Pts',(-7.22913812289554,-3.7492683997744,
59.7313928219961));
#168063=CARTESIAN_POINT('Ctrl Pts',(-6.73128452625287,-4.5695491060633,
59.7645459658327));
#168064=CARTESIAN_POINT('Ctrl Pts',(-6.48985689610431,-4.90639207327964,
59.7794574271049));
#168065=CARTESIAN_POINT('Ctrl Pts',(-6.2029620518516,-5.24823816199646,
59.7966180179185));
#168066=CARTESIAN_POINT('Ctrl Pts',(-6.18193817944885,-5.27298609311895,
59.7978724119289));
#168067=CARTESIAN_POINT('Ctrl Pts',(-6.15185584776279,-5.30796985474002,
59.7996630137157));
#168068=CARTESIAN_POINT('Ctrl Pts',(-6.14291892634242,-5.31831001472116,
59.8001944408744));
#168069=CARTESIAN_POINT('Ctrl Pts',(-6.1274948305561,-5.33606519160659,
59.8011107298327));
#168070=CARTESIAN_POINT('Ctrl Pts',(-6.12102016774566,-5.34349106229028,
59.8014950968996));
#168071=CARTESIAN_POINT('Ctrl Pts',(-6.10863493613453,-5.35764378853692,
59.8022298368414));
#168072=CARTESIAN_POINT('Ctrl Pts',(-6.10272671912686,-5.36437268828977,
59.8025801162743));
#168073=CARTESIAN_POINT('Ctrl Pts',(-6.08891647591992,-5.38004890389295,
59.8033983766707));
#168074=CARTESIAN_POINT('Ctrl Pts',(-6.08100584135918,-5.3889885892341,
59.8038666997749));
#168075=CARTESIAN_POINT('Ctrl Pts',(-6.0530310297287,-5.42046245966269,
59.8055215208989));
#168076=CARTESIAN_POINT('Ctrl Pts',(-6.03286117932124,-5.44290215699766,
59.8067122357431));
#168077=CARTESIAN_POINT('Ctrl Pts',(-5.80624333030887,-5.69221559395739,
59.8200644011216));
#168078=CARTESIAN_POINT('Ctrl Pts',(-5.58724796413447,-5.90731880299207,
59.8327403495164));
#168079=CARTESIAN_POINT('Ctrl Pts',(-4.88342893180304,-6.52440518962173,
59.8727616542604));
#168080=CARTESIAN_POINT('Ctrl Pts',(-4.36364372775441,-6.88289445994197,
59.9015269300672));
#168081=CARTESIAN_POINT('Ctrl Pts',(-3.64323174787055,-7.26507038820137,
59.9377466407012));
#168082=CARTESIAN_POINT('Ctrl Pts',(-3.4757203903129,-7.3466834564493,59.9459221489585));
#168083=CARTESIAN_POINT('Ctrl Pts',(-3.21601039246639,-7.46234356474603,
59.9580930532736));
#168084=CARTESIAN_POINT('Ctrl Pts',(-3.12575717343265,-7.50059580841624,
59.9622323647537));
#168085=CARTESIAN_POINT('Ctrl Pts',(-2.9394603794391,-7.57560760137472,
59.9705645527356));
#168086=CARTESIAN_POINT('Ctrl Pts',(-2.84337236156653,-7.6121937065427,
59.9747445293338));
#168087=CARTESIAN_POINT('Ctrl Pts',(-2.73051069950441,-7.65273097270264,
59.9795198334238));
#168088=CARTESIAN_POINT('Ctrl Pts',(-2.71439768662875,-7.6584610220005,
59.9801985636401));
#168089=CARTESIAN_POINT('Ctrl Pts',(-2.68968960568818,-7.66715984384577,
59.9812348592112));
#168090=CARTESIAN_POINT('Ctrl Pts',(-2.68110750429582,-7.6701651088701,
59.981593978953));
#168091=CARTESIAN_POINT('Ctrl Pts',(-2.66613321978502,-7.67538057435653,
59.9822191650092));
#168092=CARTESIAN_POINT('Ctrl Pts',(-2.65974329901191,-7.67759720814684,
59.982485499397));
#168093=CARTESIAN_POINT('Ctrl Pts',(-2.64537098649015,-7.68256280035275,
59.9830835475612));
#168094=CARTESIAN_POINT('Ctrl Pts',(-2.63738705574452,-7.68530730396571,
59.9834150783817));
#168095=CARTESIAN_POINT('Ctrl Pts',(-2.61602531767918,-7.69261326673342,
59.9843003074837));
#168096=CARTESIAN_POINT('Ctrl Pts',(-2.60263982886829,-7.69715228240273,
59.9848531032011));
#168097=CARTESIAN_POINT('Ctrl Pts',(-2.54465803824693,-7.7166453511911,
59.987239669946));
#168098=CARTESIAN_POINT('Ctrl Pts',(-2.49994371702045,-7.73124708715311,
59.9890597583787));
#168099=CARTESIAN_POINT('Ctrl Pts',(-2.37823574098254,-7.76982527599007,
59.9939640395288));
#168100=CARTESIAN_POINT('Ctrl Pts',(-2.30100708425179,-7.79304541804587,
59.997022238823));
#168101=CARTESIAN_POINT('Ctrl Pts',(-2.15937250927729,-7.83334126813685,
60.0025506266885));
#168102=CARTESIAN_POINT('Ctrl Pts',(-2.09507818407863,-7.8507816583953,
60.0050303494735));
#168103=CARTESIAN_POINT('Ctrl Pts',(-1.61517915015586,-7.97464313812339,
60.0233561451848));
#168104=CARTESIAN_POINT('Ctrl Pts',(-1.19193274729973,-8.04879214485667,
60.0385434078481));
#168105=CARTESIAN_POINT('Ctrl Pts',(-0.465948569070224,-8.11743133820707,
60.0648236965058));
#168106=CARTESIAN_POINT('Ctrl Pts',(-0.165766683720586,-8.12910289491409,
60.075746083675));
#168107=CARTESIAN_POINT('Ctrl Pts',(0.373160939472013,-8.120189442957,60.0958253469322));
#168108=CARTESIAN_POINT('Ctrl Pts',(0.611657436581887,-8.10571373840304,
60.1048741211254));
#168109=CARTESIAN_POINT('Ctrl Pts',(0.894816408537628,-8.07595804100068,
60.1158538008365));
#168110=CARTESIAN_POINT('Ctrl Pts',(0.9404267494293,-8.07077395143491,60.117629545636));
#168111=CARTESIAN_POINT('Ctrl Pts',(1.0114116462029,-8.06209587745681,60.1204043658754));
#168112=CARTESIAN_POINT('Ctrl Pts',(1.03681788903874,-8.05886791763399,
60.1213997357525));
#168113=CARTESIAN_POINT('Ctrl Pts',(1.08377055353067,-8.05267669541091,
60.1232433613864));
#168114=CARTESIAN_POINT('Ctrl Pts',(1.10532120207574,-8.0497469282953,60.1240911541939));
#168115=CARTESIAN_POINT('Ctrl Pts',(1.15123488338224,-8.04331720154573,
60.1259008230983));
#168116=CARTESIAN_POINT('Ctrl Pts',(1.17559431982952,-8.03979299178773,
60.1268630268368));
#168117=CARTESIAN_POINT('Ctrl Pts',(1.2407801075633,-8.03005962701958,60.1294437409101));
#168118=CARTESIAN_POINT('Ctrl Pts',(1.28157564139201,-8.02364983878517,
60.1310650082413));
#168119=CARTESIAN_POINT('Ctrl Pts',(1.46542766922892,-7.99332510095756,
60.1384013311545));
#168120=CARTESIAN_POINT('Ctrl Pts',(1.60787466974781,-7.96589367899812,
60.1441676671664));
#168121=CARTESIAN_POINT('Ctrl Pts',(1.88031086007134,-7.90582440702586,
60.155380815686));
#168122=CARTESIAN_POINT('Ctrl Pts',(2.01037739300699,-7.87375451079556,
60.1608165218205));
#168123=CARTESIAN_POINT('Ctrl Pts',(2.36061578150293,-7.77815357524732,
60.1756896800348));
#168124=CARTESIAN_POINT('Ctrl Pts',(2.57898525312594,-7.70850245319125,
60.185222346982));
#168125=CARTESIAN_POINT('Ctrl Pts',(3.04702246722017,-7.53710038884906,
60.2061817216031));
#168126=CARTESIAN_POINT('Ctrl Pts',(3.29516675451728,-7.43196483340922,
60.2176363306343));
#168127=CARTESIAN_POINT('Ctrl Pts',(3.7852460693421,-7.1949465738268,60.2407137793849));
#168128=CARTESIAN_POINT('Ctrl Pts',(4.02663034233093,-7.06269067610335,
60.2523200457162));
#168129=CARTESIAN_POINT('Ctrl Pts',(4.3560101466378,-6.85983631708373,60.2681792884972));
#168130=CARTESIAN_POINT('Ctrl Pts',(4.44995721182366,-6.79926913172143,
60.2727043118282));
#168131=CARTESIAN_POINT('Ctrl Pts',(4.55729139929475,-6.72689345013379,
60.277853420046));
#168132=CARTESIAN_POINT('Ctrl Pts',(4.57192361571225,-6.716957260947,60.2785549084256));
#168133=CARTESIAN_POINT('Ctrl Pts',(4.59413112549058,-6.70177078906364,
60.2796187437192));
#168134=CARTESIAN_POINT('Ctrl Pts',(4.6017300743744,-6.6965552958806,60.2799826188173));
#168135=CARTESIAN_POINT('Ctrl Pts',(4.61549099049545,-6.68707608955959,
60.2806412707466));
#168136=CARTESIAN_POINT('Ctrl Pts',(4.62165595963973,-6.68281676406811,
60.2809362452689));
#168137=CARTESIAN_POINT('Ctrl Pts',(4.6339700651062,-6.67428386219464,60.2815252133562));
#168138=CARTESIAN_POINT('Ctrl Pts',(4.64011920309531,-6.67001030126386,
60.2818192071481));
#168139=CARTESIAN_POINT('Ctrl Pts',(4.65741955220217,-6.65795130945561,
60.2826460139374));
#168140=CARTESIAN_POINT('Ctrl Pts',(4.66855716753571,-6.6501463518201,60.2831779053486));
#168141=CARTESIAN_POINT('Ctrl Pts',(4.71436248197956,-6.61787536747372,
60.2853636300905));
#168142=CARTESIAN_POINT('Ctrl Pts',(4.74885827629627,-6.59316563983728,
60.2870055083312));
#168143=CARTESIAN_POINT('Ctrl Pts',(5.42577472048383,-6.10021386232247,
60.319117905093));
#168144=CARTESIAN_POINT('Ctrl Pts',(5.99628601953395,-5.5404330838178,60.3442318471266));
#168145=CARTESIAN_POINT('Ctrl Pts',(6.69034809712383,-4.62432950240726,
60.383559920268));
#168146=CARTESIAN_POINT('Ctrl Pts',(6.88556738290989,-4.32829298294416,
60.3960108975434));
#168147=CARTESIAN_POINT('Ctrl Pts',(7.13490191877061,-3.890406886666,60.4146729180675));
#168148=CARTESIAN_POINT('Ctrl Pts',(7.20535389791209,-3.75831926306457,
60.4203287834228));
#168149=CARTESIAN_POINT('Ctrl Pts',(7.28235312750977,-3.60382397219841,
60.4269944232643));
#168150=CARTESIAN_POINT('Ctrl Pts',(7.29250342731437,-3.58323988155288,
60.4278835105397));
#168151=CARTESIAN_POINT('Ctrl Pts',(7.307766978784,-3.55195298847042,60.4292364571187));
#168152=CARTESIAN_POINT('Ctrl Pts',(7.31294426415695,-3.54128146811638,
60.4296982047086));
#168153=CARTESIAN_POINT('Ctrl Pts',(7.32226617083568,-3.52195935470619,
60.4305347659852));
#168154=CARTESIAN_POINT('Ctrl Pts',(7.32641888008075,-3.51331267688973,
60.4309093127197));
#168155=CARTESIAN_POINT('Ctrl Pts',(7.33467401194234,-3.49604574335888,
60.4316576345313));
#168156=CARTESIAN_POINT('Ctrl Pts',(7.33877657325894,-3.48742557027033,
60.43203140426));
#168157=CARTESIAN_POINT('Ctrl Pts',(7.35023308661733,-3.46324376560453,
60.4330804500256));
#168158=CARTESIAN_POINT('Ctrl Pts',(7.35755277856995,-3.44766600960279,
60.4337568471992));
#168159=CARTESIAN_POINT('Ctrl Pts',(7.38714915755802,-3.38415553453078,
60.4365170510512));
#168160=CARTESIAN_POINT('Ctrl Pts',(7.40900713264573,-3.33602975677801,
60.438614498745));
#168161=CARTESIAN_POINT('Ctrl Pts',(7.81088310252495,-2.42776515590612,
60.4783150648214));
#168162=CARTESIAN_POINT('Ctrl Pts',(8.03915331135233,-1.50839245211736,
60.5214962649045));
#168163=CARTESIAN_POINT('Ctrl Pts',(8.11850364623206,-0.381530010472146,
60.5718018417503));
#168164=CARTESIAN_POINT('Ctrl Pts',(8.1251981936156,-0.191901387870314,
60.5801413526158));
#168165=CARTESIAN_POINT('Ctrl Pts',(8.12530306403285,0.194326991449929,
60.5966839027687));
#168166=CARTESIAN_POINT('Ctrl Pts',(8.11822602146609,0.390818134203802,
60.6048590059351));
#168167=CARTESIAN_POINT('Ctrl Pts',(8.10272852958194,0.604814845894541,
60.6134027297524));
#168168=CARTESIAN_POINT('Ctrl Pts',(8.1013707875472,0.622737498476672,60.6141157964287));
#168169=CARTESIAN_POINT('Ctrl Pts',(8.09922980642484,0.649806406814116,
60.6151891873091));
#168170=CARTESIAN_POINT('Ctrl Pts',(8.09849052636244,0.65895600686685,60.6155513897293));
#168171=CARTESIAN_POINT('Ctrl Pts',(8.09718030352455,0.674836517362658,
60.6161790064022));
#168172=CARTESIAN_POINT('Ctrl Pts',(8.09661647011617,0.681567993079212,
60.6164447177712));
#168173=CARTESIAN_POINT('Ctrl Pts',(8.09542535404755,0.695578374583006,
60.6169970874));
#168174=CARTESIAN_POINT('Ctrl Pts',(8.0947966471583,0.702857154572223,60.6172836867319));
#168175=CARTESIAN_POINT('Ctrl Pts',(8.09329245904479,0.720001971922734,
60.6179579011816));
#168176=CARTESIAN_POINT('Ctrl Pts',(8.09240875191283,0.729867289501645,
60.6183451832726));
#168177=CARTESIAN_POINT('Ctrl Pts',(8.08945608577587,0.762164866478486,
60.6196109662545));
#168178=CARTESIAN_POINT('Ctrl Pts',(8.08731186460905,0.784590252594031,
60.6204864948873));
#168179=CARTESIAN_POINT('Ctrl Pts',(8.04959316163622,1.16247877565269,60.6351875377156));
#168180=CARTESIAN_POINT('Ctrl Pts',(7.99070464209756,1.51524848438325,60.6481515544868));
#168181=CARTESIAN_POINT('Ctrl Pts',(7.76002520682446,2.49451911717093,60.6843124984819));
#168182=CARTESIAN_POINT('Ctrl Pts',(7.53617244632897,3.10591721774189,60.7073417412755));
#168183=CARTESIAN_POINT('Ctrl Pts',(7.09240190137212,3.97823703329178,60.7441617809294));
#168184=CARTESIAN_POINT('Ctrl Pts',(6.92503953666495,4.26290403670386,60.7568113105691));
#168185=CARTESIAN_POINT('Ctrl Pts',(6.68596816716871,4.6181356778367,60.7733823145035));
#168186=CARTESIAN_POINT('Ctrl Pts',(6.62961783598603,4.69867157964452,60.7771983939031));
#168187=CARTESIAN_POINT('Ctrl Pts',(6.54395786805605,4.81648709215843,60.7828759674642));
#168188=CARTESIAN_POINT('Ctrl Pts',(6.51576044127776,4.85456469053098,60.7847260303116));
#168189=CARTESIAN_POINT('Ctrl Pts',(6.4646104734408,4.92238869114325,60.7880493238095));
#168190=CARTESIAN_POINT('Ctrl Pts',(6.44178157100305,4.95222668893286,60.7895212153291));
#168191=CARTESIAN_POINT('Ctrl Pts',(6.39261883240736,5.01556855269947,60.7926673891941));
#168192=CARTESIAN_POINT('Ctrl Pts',(6.36622671122521,5.04902573625479,60.7943422631618));
#168193=CARTESIAN_POINT('Ctrl Pts',(6.2934754699579,5.13977484044467,60.7989217096145));
#168194=CARTESIAN_POINT('Ctrl Pts',(6.24659827876539,5.19664591299531,60.8018318728236));
#168195=CARTESIAN_POINT('Ctrl Pts',(5.92853158999695,5.57199889022977,60.8213178883067));
#168196=CARTESIAN_POINT('Ctrl Pts',(5.63387517310721,5.86976098877403,60.8381604705478));
#168197=CARTESIAN_POINT('Ctrl Pts',(4.98792958335573,6.42887020666397,60.8728401923948));
#168198=CARTESIAN_POINT('Ctrl Pts',(4.63580441709636,6.68723699102904,60.8906314874597));
#168199=CARTESIAN_POINT('Ctrl Pts',(4.20270195468915,6.95429943598463,60.9109386054428));
#168200=CARTESIAN_POINT('Ctrl Pts',(4.1402424497911,6.99166482188269,60.9138308674267));
#168201=CARTESIAN_POINT('Ctrl Pts',(4.05608661621247,7.04048647163382,60.9176768333862));
#168202=CARTESIAN_POINT('Ctrl Pts',(4.0348286814298,7.05269068611266,60.9186440399612));
#168203=CARTESIAN_POINT('Ctrl Pts',(3.99862944204557,7.0732554931069,60.920283640733));
#168204=CARTESIAN_POINT('Ctrl Pts',(3.98371643483754,7.08166534469235,60.9209569680551));
#168205=CARTESIAN_POINT('Ctrl Pts',(3.95183295451385,7.0995127239852,60.9223920395896));
#168206=CARTESIAN_POINT('Ctrl Pts',(3.93485504261444,7.10893665855741,60.9231535329103));
#168207=CARTESIAN_POINT('Ctrl Pts',(3.89265361590535,7.13216391676713,60.9250399910602));
#168208=CARTESIAN_POINT('Ctrl Pts',(3.86739026549029,7.145894405407,60.9261636854468));
#168209=CARTESIAN_POINT('Ctrl Pts',(3.76718415291409,7.19966881054316,60.9306000446703));
#168210=CARTESIAN_POINT('Ctrl Pts',(3.69168765298413,7.23867045021743,60.9338968721704));
#168211=CARTESIAN_POINT('Ctrl Pts',(3.53881622261458,7.31463036213173,60.9404988412214));
#168212=CARTESIAN_POINT('Ctrl Pts',(3.46144028852124,7.35156233927766,60.9438033754844));
#168213=CARTESIAN_POINT('Ctrl Pts',(3.12042252938551,7.50775436805165,60.9582407352219));
#168214=CARTESIAN_POINT('Ctrl Pts',(2.85110361184242,7.61410665018196,60.9693253760213));
#168215=CARTESIAN_POINT('Ctrl Pts',(2.49957767473549,7.73164986578451,60.9836739687851));
#168216=CARTESIAN_POINT('Ctrl Pts',(2.42208611300805,7.75627468273187,60.9868289832247));
#168217=CARTESIAN_POINT('Ctrl Pts',(2.30355538468195,7.79199111500701,60.9916470954672));
#168218=CARTESIAN_POINT('Ctrl Pts',(2.262776973388,7.80393063131779,60.9933032783038));
#168219=CARTESIAN_POINT('Ctrl Pts',(2.18822778203746,7.82512445230124,60.9963290597273));
#168220=CARTESIAN_POINT('Ctrl Pts',(2.15448721024098,7.83448137219025,60.9976977777518));
#168221=CARTESIAN_POINT('Ctrl Pts',(2.08058319454352,7.85446287412851,61.0006944766805));
#168222=CARTESIAN_POINT('Ctrl Pts',(2.04039663839111,7.86499809357729,61.0023231565775));
#168223=CARTESIAN_POINT('Ctrl Pts',(1.9240154531896,7.89455631508567,61.0070380098315));
#168224=CARTESIAN_POINT('Ctrl Pts',(1.84762384795223,7.9127833840856,61.0101305728496));
#168225=CARTESIAN_POINT('Ctrl Pts',(1.71672453836261,7.94201705726832,61.0154271511196));
#168226=CARTESIAN_POINT('Ctrl Pts',(1.66234593583963,7.95357680749427,61.0176266898467));
#168227=CARTESIAN_POINT('Ctrl Pts',(1.43069327443569,8.00034180636538,61.0269934516233));
#168228=CARTESIAN_POINT('Ctrl Pts',(1.25239064457378,8.0301848728818,61.034196511095));
#168229=CARTESIAN_POINT('Ctrl Pts',(0.806384689260168,8.0896173607951,61.0521648470201));
#168230=CARTESIAN_POINT('Ctrl Pts',(0.537922820619334,8.11189287267858,
61.0629408866666));
#168231=CARTESIAN_POINT('Ctrl Pts',(0.229097062707495,8.12211697465617,
61.0751453871078));
#168232=CARTESIAN_POINT('Ctrl Pts',(0.189334548041407,8.12314114532041,
61.0767129549097));
#168233=CARTESIAN_POINT('Ctrl Pts',(0.12825480132642,8.12426566457234,61.0791141682226));
#168234=CARTESIAN_POINT('Ctrl Pts',(0.106942205005658,8.12457415811716,
61.0799507334359));
#168235=CARTESIAN_POINT('Ctrl Pts',(0.0655175388263775,8.125010739147,61.0815742895506));
#168236=CARTESIAN_POINT('Ctrl Pts',(0.0454057952675497,8.12514802179986,
61.0823614260348));
#168237=CARTESIAN_POINT('Ctrl Pts',(-0.00238654562119118,8.12529679894001,
61.0842295373541));
#168238=CARTESIAN_POINT('Ctrl Pts',(-0.0300671314041179,8.12524151898409,
61.0853096116265));
#168239=CARTESIAN_POINT('Ctrl Pts',(-0.12470551894208,8.12456889754107,
61.0889966447027));
#168240=CARTESIAN_POINT('Ctrl Pts',(-0.1916559813614,8.12326531097501,61.0915952690033));
#168241=CARTESIAN_POINT('Ctrl Pts',(-0.314055257674444,8.119368026531,61.0963344456969));
#168242=CARTESIAN_POINT('Ctrl Pts',(-0.369508150382494,8.11703342482815,
61.0984771469826));
#168243=CARTESIAN_POINT('Ctrl Pts',(-0.654072942869756,8.10213091073416,
61.1094594950965));
#168244=CARTESIAN_POINT('Ctrl Pts',(-0.882602861258377,8.08043005540727,
61.118237715875));
#168245=CARTESIAN_POINT('Ctrl Pts',(-1.27684366261096,8.02606722899659,
61.1334959867371));
#168246=CARTESIAN_POINT('Ctrl Pts',(-1.44302195346336,7.99786047271005,
61.1399628680115));
#168247=CARTESIAN_POINT('Ctrl Pts',(-1.790222260089,7.92775340092446,61.15361313872));
#168248=CARTESIAN_POINT('Ctrl Pts',(-1.97092745133505,7.8847709987417,61.1607986235292));
#168249=CARTESIAN_POINT('Ctrl Pts',(-2.213872798011,7.81810985601866,61.1706037138418));
#168250=CARTESIAN_POINT('Ctrl Pts',(-2.27752896207104,7.79980360418615,
61.1731863647071));
#168251=CARTESIAN_POINT('Ctrl Pts',(-2.393748786298,7.76483701738787,61.1779276210929));
#168252=CARTESIAN_POINT('Ctrl Pts',(-2.44638041629265,7.74841596651649,
61.1800846211835));
#168253=CARTESIAN_POINT('Ctrl Pts',(-2.55585042449841,7.71303479738341,
61.184592085886));
#168254=CARTESIAN_POINT('Ctrl Pts',(-2.61265445561199,7.69397906433219,
61.1869429709098));
#168255=CARTESIAN_POINT('Ctrl Pts',(-2.77921725039197,7.63604587752053,
61.1938718693162));
#168256=CARTESIAN_POINT('Ctrl Pts',(-2.88835681674073,7.59543546485952,
61.1984579551067));
#168257=CARTESIAN_POINT('Ctrl Pts',(-3.20393541744128,7.47022407232345,
61.211849373212));
#168258=CARTESIAN_POINT('Ctrl Pts',(-3.40780943167426,7.37945017508381,
61.2206686170383));
#168259=CARTESIAN_POINT('Ctrl Pts',(-3.65432236401248,7.25729455322159,
61.231497151881));
#168260=CARTESIAN_POINT('Ctrl Pts',(-3.70073221946383,7.23373881452888,
61.2335430629632));
#168261=CARTESIAN_POINT('Ctrl Pts',(-3.77898769953057,7.19306931765594,
61.2370039827339));
#168262=CARTESIAN_POINT('Ctrl Pts',(-3.81095110631346,7.17618602831645,
61.2384206652219));
#168263=CARTESIAN_POINT('Ctrl Pts',(-3.90334956624565,7.12658909806216,
61.2425258509384));
#168264=CARTESIAN_POINT('Ctrl Pts',(-3.9634836441215,7.09332132791915,61.245210127954));
#168265=CARTESIAN_POINT('Ctrl Pts',(-4.16241521353036,6.9799475050825,61.2541430255104));
#168266=CARTESIAN_POINT('Ctrl Pts',(-4.29926419472592,6.8964987592677,61.2603757542781));
#168267=CARTESIAN_POINT('Ctrl Pts',(-4.54931819830307,6.73368204634625,
61.2719959728997));
#168268=CARTESIAN_POINT('Ctrl Pts',(-4.6631390338507,6.6553665652407,61.277379406449));
#168269=CARTESIAN_POINT('Ctrl Pts',(-4.82557431433687,6.53738796790606,
61.2852265057699));
#168270=CARTESIAN_POINT('Ctrl Pts',(-4.8758138151174,6.50000373182439,61.2876771244317));
#168271=CARTESIAN_POINT('Ctrl Pts',(-4.96934372167773,6.42871165930659,
61.2922864760169));
#168272=CARTESIAN_POINT('Ctrl Pts',(-5.01273186602575,6.39493782898225,
61.2944442294149));
#168273=CARTESIAN_POINT('Ctrl Pts',(-5.11333929060061,6.31497080087364,
61.2994951898391));
#168274=CARTESIAN_POINT('Ctrl Pts',(-5.17028082684087,6.268436090637,61.3023906635151));
#168275=CARTESIAN_POINT('Ctrl Pts',(-5.37880171119411,6.09325075291125,
61.3131365448601));
#168276=CARTESIAN_POINT('Ctrl Pts',(-5.52627451862615,5.9598239295092,61.3210226859123));
#168277=CARTESIAN_POINT('Ctrl Pts',(-5.95846946899684,5.53894556536053,
61.3450649901976));
#168278=CARTESIAN_POINT('Ctrl Pts',(-6.2267599271406,5.23552628451184,61.3613267992789));
#168279=CARTESIAN_POINT('Ctrl Pts',(-6.52768190762045,4.83918772183988,
61.3811102124871));
#168280=CARTESIAN_POINT('Ctrl Pts',(-6.58274446637141,4.76401557689418,
61.3848016987598));
#168281=CARTESIAN_POINT('Ctrl Pts',(-6.65503588600647,4.66167532206538,
61.3897400641955));
#168282=CARTESIAN_POINT('Ctrl Pts',(-6.67341377276085,4.63532826048087,
61.3910037986421));
#168283=CARTESIAN_POINT('Ctrl Pts',(-6.70236428483002,4.59329493334236,
61.3930074995878));
#168284=CARTESIAN_POINT('Ctrl Pts',(-6.71303917450127,4.57767958638977,
61.393749172534));
#168285=CARTESIAN_POINT('Ctrl Pts',(-6.73482202202277,4.54557533835347,
61.3952683860332));
#168286=CARTESIAN_POINT('Ctrl Pts',(-6.74592419590036,4.52908264139374,
61.396045819375));
#168287=CARTESIAN_POINT('Ctrl Pts',(-6.77332663990799,4.48805098437757,
61.3979723519062));
#168288=CARTESIAN_POINT('Ctrl Pts',(-6.789554221519,4.46346377751756,61.3991200727112));
#168289=CARTESIAN_POINT('Ctrl Pts',(-6.86235012980001,4.35185150329611,
61.4043015663394));
#168290=CARTESIAN_POINT('Ctrl Pts',(-6.91738191672716,4.26383496120505,
61.4083097916253));
#168291=CARTESIAN_POINT('Ctrl Pts',(-7.09139901944629,3.97327569708988,
61.4213408157735));
#168292=CARTESIAN_POINT('Ctrl Pts',(-7.20329100990146,3.766624420254,61.430300693717));
#168293=CARTESIAN_POINT('Ctrl Pts',(-7.4032688075017,3.35568725227628,61.4478084145931));
#168294=CARTESIAN_POINT('Ctrl Pts',(-7.4922323670626,3.15205940236069,61.4563445519342));
#168295=CARTESIAN_POINT('Ctrl Pts',(-7.59388198332121,2.89068264474098,
61.4672220906932));
#168296=CARTESIAN_POINT('Ctrl Pts',(-7.61443729055391,2.83609492637373,
61.4694893131216));
#168297=CARTESIAN_POINT('Ctrl Pts',(-7.64594744584925,2.7496022722373,61.4730758178265));
#168298=CARTESIAN_POINT('Ctrl Pts',(-7.65729446891351,2.71784223370749,
61.4743915424886));
#168299=CARTESIAN_POINT('Ctrl Pts',(-7.68017015305105,2.6525331977834,61.4770948144507));
#168300=CARTESIAN_POINT('Ctrl Pts',(-7.69167750233672,2.61897749788778,
61.4784825210875));
#168301=CARTESIAN_POINT('Ctrl Pts',(-7.71805447015741,2.54038812243124,
61.4817299911465));
#168302=CARTESIAN_POINT('Ctrl Pts',(-7.73275027307521,2.49529753853598,
61.483591229651));
#168303=CARTESIAN_POINT('Ctrl Pts',(-7.7816063112487,2.34081685393292,61.4899616302422));
#168304=CARTESIAN_POINT('Ctrl Pts',(-7.81384649241907,2.23083459619634,
61.4944866694988));
#168305=CARTESIAN_POINT('Ctrl Pts',(-7.89616719113295,1.92628761384265,
61.5069882655948));
#168306=CARTESIAN_POINT('Ctrl Pts',(-7.9413751586908,1.73049123072408,61.5149958773726));
#168307=CARTESIAN_POINT('Ctrl Pts',(-8.01456379929508,1.34959891103702,
61.5304664603936));
#168308=CARTESIAN_POINT('Ctrl Pts',(-8.04349837003739,1.1648110698877,61.5379238851092));
#168309=CARTESIAN_POINT('Ctrl Pts',(-8.07060514929345,0.941520024572059,
61.5468227200769));
#168310=CARTESIAN_POINT('Ctrl Pts',(-8.07491412840532,0.903819267864985,
61.5483213019505));
#168311=CARTESIAN_POINT('Ctrl Pts',(-8.081464064806,0.842720893481965,61.5507427927173));
#168312=CARTESIAN_POINT('Ctrl Pts',(-8.08386786482879,0.819341372071401,
61.5516676962131));
#168313=CARTESIAN_POINT('Ctrl Pts',(-8.08798672413963,0.777497379011614,
61.5533198168065));
#168314=CARTESIAN_POINT('Ctrl Pts',(-8.08974007471084,0.759036857161392,
61.5540475622623));
#168315=CARTESIAN_POINT('Ctrl Pts',(-8.09343964543737,0.718615560348982,
61.5556384288328));
#168316=CARTESIAN_POINT('Ctrl Pts',(-8.09535970569644,0.696652607591544,
61.5565011205808));
#168317=CARTESIAN_POINT('Ctrl Pts',(-8.10102148066233,0.6287028654175,61.5591651635049));
#168318=CARTESIAN_POINT('Ctrl Pts',(-8.10446091661238,0.582691696398901,
61.5609620435754));
#168319=CARTESIAN_POINT('Ctrl Pts',(-8.11161904785845,0.474550026943905,
61.5651710623397));
#168320=CARTESIAN_POINT('Ctrl Pts',(-8.11501612977759,0.412401017819403,
61.5675789537567));
#168321=CARTESIAN_POINT('Ctrl Pts',(-8.12466965400848,0.188642614285465,
61.5762169056599));
#168322=CARTESIAN_POINT('Ctrl Pts',(-8.12681491848019,0.0268928378850284,
61.5824026345489));
#168323=CARTESIAN_POINT('Ctrl Pts',(-8.11640160148237,-0.600631030495562,
61.6063234648979));
#168324=CARTESIAN_POINT('Ctrl Pts',(-8.0686231312327,-1.06491898245423,
61.6238855130451));
#168325=CARTESIAN_POINT('Ctrl Pts',(-7.94036252037984,-1.7372724846345,
61.650129710661));
#168326=CARTESIAN_POINT('Ctrl Pts',(-7.89075246024864,-1.95025543985168,
61.6585610244123));
#168327=CARTESIAN_POINT('Ctrl Pts',(-7.81546766088394,-2.22313068525872,
61.6695676930288));
#168328=CARTESIAN_POINT('Ctrl Pts',(-7.79758040967125,-2.28507866428104,
61.6720801559474));
#168329=CARTESIAN_POINT('Ctrl Pts',(-7.76729093995983,-2.38547912761291,
61.6761756109967));
#168330=CARTESIAN_POINT('Ctrl Pts',(-7.75533587486127,-2.42406366853103,
61.6777551963373));
#168331=CARTESIAN_POINT('Ctrl Pts',(-7.73186485078844,-2.49786431916701,
61.6807876126248));
#168332=CARTESIAN_POINT('Ctrl Pts',(-7.72039474993824,-2.53309398226664,
61.6822400754721));
#168333=CARTESIAN_POINT('Ctrl Pts',(-7.69319068409944,-2.61474804579395,
61.685618131188));
#168334=CARTESIAN_POINT('Ctrl Pts',(-7.67727678440134,-2.66111093315479,
61.6875449330664));
#168335=CARTESIAN_POINT('Ctrl Pts',(-7.62510262732157,-2.8087485604071,
61.6937090947627));
#168336=CARTESIAN_POINT('Ctrl Pts',(-7.58725052254165,-2.90944803295918,
61.697956628087));
#168337=CARTESIAN_POINT('Ctrl Pts',(-7.35701012323633,-3.48688491761813,
61.7225670745153));
#168338=CARTESIAN_POINT('Ctrl Pts',(-7.1217296056915,-3.9452385944691,61.74306203922));
#168339=CARTESIAN_POINT('Ctrl Pts',(-6.42948745332216,-5.02744712178074,
61.7961337332576));
#168340=CARTESIAN_POINT('Ctrl Pts',(-5.9240538288087,-5.61417367647944,
61.8297851861502));
#168341=CARTESIAN_POINT('Ctrl Pts',(-5.30485199531406,-6.154744630721,61.8628724365981));
#168342=CARTESIAN_POINT('Ctrl Pts',(-5.26576161399473,-6.1882219515441,
61.8649287898478));
#168343=CARTESIAN_POINT('Ctrl Pts',(-5.21558854318688,-6.23037089137512,
61.8675243805212));
#168344=CARTESIAN_POINT('Ctrl Pts',(-5.20479824939517,-6.23938782910821,
61.8680800456619));
#168345=CARTESIAN_POINT('Ctrl Pts',(-5.18762092233689,-6.25366654103752,
61.8689605128334));
#168346=CARTESIAN_POINT('Ctrl Pts',(-5.18124919080095,-6.25894662573627,
61.869286217994));
#168347=CARTESIAN_POINT('Ctrl Pts',(-5.16934985855267,-6.26877666361825,
61.8698927956179));
#168348=CARTESIAN_POINT('Ctrl Pts',(-5.16382429226536,-6.27332906019362,
61.8701737910381));
#168349=CARTESIAN_POINT('Ctrl Pts',(-5.15153816340792,-6.28342410945336,
61.8707970755344));
#168350=CARTESIAN_POINT('Ctrl Pts',(-5.14477465182072,-6.28896317138708,
61.8711391806417));
#168351=CARTESIAN_POINT('Ctrl Pts',(-5.12515731084194,-6.30497621134719,
61.8721284820466));
#168352=CARTESIAN_POINT('Ctrl Pts',(-5.11228029668986,-6.31542181172606,
61.8727741942987));
#168353=CARTESIAN_POINT('Ctrl Pts',(-5.01635829319294,-6.39274637971109,
61.8775563378679));
#168354=CARTESIAN_POINT('Ctrl Pts',(-4.93204316401295,-6.45801885898859,
61.8815990186006));
#168355=CARTESIAN_POINT('Ctrl Pts',(-4.7023167011064,-6.62873715179465,
61.8922119454725));
#168356=CARTESIAN_POINT('Ctrl Pts',(-4.55465719690427,-6.73105055102272,
61.8986259138178));
#168357=CARTESIAN_POINT('Ctrl Pts',(-3.94976983885492,-7.12115074926514,
61.9237254026474));
#168358=CARTESIAN_POINT('Ctrl Pts',(-3.46774181000144,-7.367922266777,61.941195900664));
#168359=CARTESIAN_POINT('Ctrl Pts',(-2.47039456857689,-7.75878826284801,
61.9774627123021));
#168360=CARTESIAN_POINT('Ctrl Pts',(-1.95826305640002,-7.90359242045759,
61.9961720515824));
#168361=CARTESIAN_POINT('Ctrl Pts',(-1.40358744084232,-8.00316773933742,
62.0178344742494));
#168362=CARTESIAN_POINT('Ctrl Pts',(-1.37144739569775,-8.0087379517326,
62.0190941457293));
#168363=CARTESIAN_POINT('Ctrl Pts',(-1.32677351539151,-8.01620360585699,
62.0208514264824));
#168364=CARTESIAN_POINT('Ctrl Pts',(-1.31426729447796,-8.01826350830555,
62.0213440596437));
#168365=CARTESIAN_POINT('Ctrl Pts',(-1.29273146244183,-8.02175894193811,
62.0221935796831));
#168366=CARTESIAN_POINT('Ctrl Pts',(-1.28370413815077,-8.02320851290605,
62.0225500418148));
#168367=CARTESIAN_POINT('Ctrl Pts',(-1.26507876432179,-8.02616706044107,
62.0232862553839));
#168368=CARTESIAN_POINT('Ctrl Pts',(-1.25548041802125,-8.02767406421343,
62.0236660657362));
#168369=CARTESIAN_POINT('Ctrl Pts',(-1.23315170565159,-8.03113879398552,
62.0245505860221));
#168370=CARTESIAN_POINT('Ctrl Pts',(-1.22041935786317,-8.03308347065552,
62.0250556884332));
#168371=CARTESIAN_POINT('Ctrl Pts',(-1.17990761924513,-8.03917249738859,
62.0266651555246));
#168372=CARTESIAN_POINT('Ctrl Pts',(-1.15211147716946,-8.04320306579887,
62.0277729411678));
#168373=CARTESIAN_POINT('Ctrl Pts',(-0.850935757889427,-8.08528168418689,
62.0398142675268));
#168374=CARTESIAN_POINT('Ctrl Pts',(-0.575827172519357,-8.10951765209312,
62.051163082099));
#168375=CARTESIAN_POINT('Ctrl Pts',(0.108007341429484,-8.13478621513484,
62.0802124984239));
#168376=CARTESIAN_POINT('Ctrl Pts',(0.516577756190515,-8.11908359996046,
62.09832791996));
#168377=CARTESIAN_POINT('Ctrl Pts',(1.53296842456235,-8.00297389323821,
62.144229421143));
#168378=CARTESIAN_POINT('Ctrl Pts',(2.13392133622353,-7.86410624761655,
62.1721642797551));
#168379=CARTESIAN_POINT('Ctrl Pts',(2.74694008616192,-7.64691212908519,
62.1983431121043));
#168380=CARTESIAN_POINT('Ctrl Pts',(2.78028635467762,-7.63485119625819,
62.1997601833476));
#168381=CARTESIAN_POINT('Ctrl Pts',(2.82541572315839,-7.61819358190449,
62.201669690669));
#168382=CARTESIAN_POINT('Ctrl Pts',(2.83726828905259,-7.61378723884296,
62.2021704152822));
#168383=CARTESIAN_POINT('Ctrl Pts',(2.85594416800136,-7.60679457568051,
62.2029582300159));
#168384=CARTESIAN_POINT('Ctrl Pts',(2.86277433628951,-7.60422671330217,
62.2032461038299));
#168385=CARTESIAN_POINT('Ctrl Pts',(2.87594082822761,-7.59925640016529,
62.2038005753312));
#168386=CARTESIAN_POINT('Ctrl Pts',(2.88227762093635,-7.59685521772761,
62.2040672257314));
#168387=CARTESIAN_POINT('Ctrl Pts',(2.89725171383319,-7.59115969562443,
62.2046968566993));
#168388=CARTESIAN_POINT('Ctrl Pts',(2.90588642082837,-7.58785853372879,
62.2050595553486));
#168389=CARTESIAN_POINT('Ctrl Pts',(2.93114843689675,-7.57815108782815,
62.2061196296936));
#168390=CARTESIAN_POINT('Ctrl Pts',(2.94776038654476,-7.57170481322532,
62.2068153862158));
#168391=CARTESIAN_POINT('Ctrl Pts',(3.07158039100774,-7.52318715694141,
62.2119921693351));
#168392=CARTESIAN_POINT('Ctrl Pts',(3.17790714084202,-7.47889421341075,
62.2163864025545));
#168393=CARTESIAN_POINT('Ctrl Pts',(3.5344628780798,-7.32138494577898,62.2310430045235));
#168394=CARTESIAN_POINT('Ctrl Pts',(3.77988828380747,-7.19774685280098,
62.2410030044885));
#168395=CARTESIAN_POINT('Ctrl Pts',(4.33586457388257,-6.88136816541448,
62.264036540786));
#168396=CARTESIAN_POINT('Ctrl Pts',(4.64061072891498,-6.67964673342571,
62.2770423221525));
#168397=CARTESIAN_POINT('Ctrl Pts',(5.00087763164712,-6.40458375290102,
62.2935778118405));
#168398=CARTESIAN_POINT('Ctrl Pts',(5.07011877668137,-6.34991066875522,
62.2968117389642));
#168399=CARTESIAN_POINT('Ctrl Pts',(5.37332602181805,-6.10237541592036,
62.3112457567115));
#168400=CARTESIAN_POINT('Ctrl Pts',(5.5972708239307,-5.89764075144378,62.3226541829803));
#168401=CARTESIAN_POINT('Ctrl Pts',(5.84451849234334,-5.64480615125514,
62.3362735916627));
#168402=CARTESIAN_POINT('Ctrl Pts',(5.87945525899085,-5.60840785769787,
62.3382233727168));
#168403=CARTESIAN_POINT('Ctrl Pts',(5.93226733259062,-5.55235063656264,
62.3412097870372));
#168404=CARTESIAN_POINT('Ctrl Pts',(5.9503890798934,-5.5329253643324,62.3422416921391));
#168405=CARTESIAN_POINT('Ctrl Pts',(5.98295131148275,-5.49767587979276,
62.3441088538814));
#168406=CARTESIAN_POINT('Ctrl Pts',(5.99742512800038,-5.48188273354477,
62.3449434929718));
#168407=CARTESIAN_POINT('Ctrl Pts',(6.02554345695251,-5.45095668493241,
62.3465741429988));
#168408=CARTESIAN_POINT('Ctrl Pts',(6.03919386560688,-5.43582930039243,
62.3473700550967));
#168409=CARTESIAN_POINT('Ctrl Pts',(6.07494585111884,-5.39590804924719,
62.3494661271424));
#168410=CARTESIAN_POINT('Ctrl Pts',(6.09695250085984,-5.37102978557374,
62.3507679913123));
#168411=CARTESIAN_POINT('Ctrl Pts',(6.17728190776458,-5.27908843628185,
62.3555640942276));
#168412=CARTESIAN_POINT('Ctrl Pts',(6.2346552311554,-5.21120526665049,62.3590759736546));
#168413=CARTESIAN_POINT('Ctrl Pts',(6.5683907136943,-4.8029329699844,62.3800484434053));
#168414=CARTESIAN_POINT('Ctrl Pts',(6.8179305137607,-4.44158831263069,62.3980628078057));
#168415=CARTESIAN_POINT('Ctrl Pts',(7.34050314382295,-3.53625029271457,
62.4420281554622));
#168416=CARTESIAN_POINT('Ctrl Pts',(7.58405825412809,-2.9782718641043,62.4683149604618));
#168417=CARTESIAN_POINT('Ctrl Pts',(7.77870682761077,-2.3482258212521,62.494919088341));
#168418=CARTESIAN_POINT('Ctrl Pts',(7.79371892678636,-2.29790988672862,
62.4970219239637));
#168419=CARTESIAN_POINT('Ctrl Pts',(7.81227323311432,-2.23344730287871,
62.4996855633942));
#168420=CARTESIAN_POINT('Ctrl Pts',(7.81626636487498,-2.21943236890466,
62.5002628407396));
#168421=CARTESIAN_POINT('Ctrl Pts',(7.82256263188266,-2.19710623555054,
62.5011794744542));
#168422=CARTESIAN_POINT('Ctrl Pts',(7.8248902663525,-2.18880201485997,62.5015197611022));
#168423=CARTESIAN_POINT('Ctrl Pts',(7.82921502550224,-2.17327765490255,
62.5021546683733));
#168424=CARTESIAN_POINT('Ctrl Pts',(7.83121539384655,-2.16605843330477,
62.5024494147007));
#168425=CARTESIAN_POINT('Ctrl Pts',(7.83564625099783,-2.14998133955712,
62.5031046796966));
#168426=CARTESIAN_POINT('Ctrl Pts',(7.83807171155595,-2.1411220835328,62.5034649992353));
#168427=CARTESIAN_POINT('Ctrl Pts',(7.84508411590936,-2.11533692393796,
62.5045114679244));
#168428=CARTESIAN_POINT('Ctrl Pts',(7.84963131031478,-2.09840019676589,
62.5051960086753));
#168429=CARTESIAN_POINT('Ctrl Pts',(7.88364562920719,-1.97005081474732,
62.5103616014667));
#168430=CARTESIAN_POINT('Ctrl Pts',(7.91079249308458,-1.85804518721877,
62.5147368436552));
#168431=CARTESIAN_POINT('Ctrl Pts',(7.9569571824244,-1.64816556709156,62.5227047770965));
#168432=CARTESIAN_POINT('Ctrl Pts',(7.97657224980911,-1.55045587653565,
62.5263263750937));
#168433=CARTESIAN_POINT('Ctrl Pts',(8.08114970837706,-0.974837606639548,
62.5472557002737));
#168434=CARTESIAN_POINT('Ctrl Pts',(8.12494782477393,-0.490442646926205,
62.5632724758603));
#168435=CARTESIAN_POINT('Ctrl Pts',(8.12524844182851,-0.00503200391139533,
62.5796456772854));
#168436=CARTESIAN_POINT('',(8.120871211716,0.00172117854336219,64.5832974432123));
#168437=CARTESIAN_POINT('Ctrl Pts',(8.1189210508199,-0.00515126165391927,
62.5832974432123));
#168438=CARTESIAN_POINT('Ctrl Pts',(8.10078544928883,2.03703630869922,62.6634709337063));
#168439=CARTESIAN_POINT('Ctrl Pts',(6.80819671928344,5.43726497504401,62.7965335792958));
#168440=CARTESIAN_POINT('Ctrl Pts',(2.61913853473347,8.04100520042313,62.9824853799807));
#168441=CARTESIAN_POINT('Ctrl Pts',(-1.52043507705924,8.33340792156297,
63.1411528452671));
#168442=CARTESIAN_POINT('Ctrl Pts',(-5.33310408397482,6.58368385109608,
63.2998203105535));
#168443=CARTESIAN_POINT('Ctrl Pts',(-7.82264342903578,3.23476629007734,
63.45848777584));
#168444=CARTESIAN_POINT('Ctrl Pts',(-8.42537801125607,-0.894369939753464,
63.6171552411264));
#168445=CARTESIAN_POINT('Ctrl Pts',(-6.96195299981465,-4.8258285132288,
63.7758227064128));
#168446=CARTESIAN_POINT('Ctrl Pts',(-3.82482145636898,-7.54243940143088,
63.9344901716993));
#168447=CARTESIAN_POINT('Ctrl Pts',(1.64131973131632,-8.81124817329279,
64.1460467920811));
#168448=CARTESIAN_POINT('Ctrl Pts',(6.87712117603622,-5.734150059192,64.3576034124631));
#168449=CARTESIAN_POINT('Ctrl Pts',(8.08738294886851,-1.59563522457139,
64.5209833478719));
#168450=CARTESIAN_POINT('Ctrl Pts',(8.12076539718447,-0.119070448189842,
64.5785849730899));
#168451=CARTESIAN_POINT('Ctrl Pts',(8.120871211716,0.00172117854336219,
64.5832974432123));
#168452=CARTESIAN_POINT('',(8.12588319212561,0.00333877610560675,66.5832974432123));
#168453=CARTESIAN_POINT('Ctrl Pts',(8.12524981744152,0.00172240138683085,
64.5832974547079));
#168454=CARTESIAN_POINT('Ctrl Pts',(8.12520564937343,0.210080679493343,
64.5914218031291));
#168455=CARTESIAN_POINT('Ctrl Pts',(8.11714269539066,0.418310872283689,
64.5995461515503));
#168456=CARTESIAN_POINT('Ctrl Pts',(8.101116090879,0.625784023926309,64.6076704999715));
#168457=CARTESIAN_POINT('Ctrl Pts',(8.08507493566357,0.833445542379041,
64.6158022245644));
#168458=CARTESIAN_POINT('Ctrl Pts',(8.0610557220093,1.04034834560792,64.6239339491573));
#168459=CARTESIAN_POINT('Ctrl Pts',(8.02916518697421,1.24587076487951,64.6320656737502));
#168460=CARTESIAN_POINT('Ctrl Pts',(7.99721833306486,1.45175613796399,64.640211759017));
#168461=CARTESIAN_POINT('Ctrl Pts',(7.95737241127435,1.6562559525216,64.6483578442838));
#168462=CARTESIAN_POINT('Ctrl Pts',(7.90978530245305,1.85875873410125,64.6565039295506));
#168463=CARTESIAN_POINT('Ctrl Pts',(7.862154855686,2.06144593652047,64.6646574335199));
#168464=CARTESIAN_POINT('Ctrl Pts',(7.80676922922532,2.26213218325287,64.6728109374892));
#168465=CARTESIAN_POINT('Ctrl Pts',(7.74383589681935,2.46022217810345,64.6809644414584));
#168466=CARTESIAN_POINT('Ctrl Pts',(7.68078585008095,2.65867954491142,64.6891330666796));
#168467=CARTESIAN_POINT('Ctrl Pts',(7.61016020825909,2.85453074518204,64.6973016919008));
#168468=CARTESIAN_POINT('Ctrl Pts',(7.53221508499273,3.04719928391759,64.705470317122));
#168469=CARTESIAN_POINT('Ctrl Pts',(7.46110425208086,3.22297449205448,64.7129227107918));
#168470=CARTESIAN_POINT('Ctrl Pts',(7.38390187156463,3.39610080444314,64.7203751044616));
#168471=CARTESIAN_POINT('Ctrl Pts',(7.30083524784918,3.56615931307941,64.7278274981315));
#168472=CARTESIAN_POINT('Ctrl Pts',(7.21070409780524,3.75068070413351,64.7359136918636));
#168473=CARTESIAN_POINT('Ctrl Pts',(7.11349959723325,3.93193487294235,64.7439998855958));
#168474=CARTESIAN_POINT('Ctrl Pts',(7.00948073055911,4.10936338748723,64.752086079328));
#168475=CARTESIAN_POINT('Ctrl Pts',(6.90555464377817,4.28663364421642,64.7601650605591));
#168476=CARTESIAN_POINT('Ctrl Pts',(6.79482646948925,4.46008477850942,64.7682440417901));
#168477=CARTESIAN_POINT('Ctrl Pts',(6.67760168871661,4.62918170407568,64.7763230230212));
#168478=CARTESIAN_POINT('Ctrl Pts',(6.56046545921777,4.79815089429405,64.7843959014123));
#168479=CARTESIAN_POINT('Ctrl Pts',(6.43684258907658,4.96277217521777,64.7924687798034));
#168480=CARTESIAN_POINT('Ctrl Pts',(6.30708289096697,5.12253774695431,64.8005416581945));
#168481=CARTESIAN_POINT('Ctrl Pts',(6.17740351990848,5.28220441666322,64.8086095391131));
#168482=CARTESIAN_POINT('Ctrl Pts',(6.04159509627907,5.43702112650239,64.8166774200318));
#168483=CARTESIAN_POINT('Ctrl Pts',(5.90004926268348,5.58651109910363,64.8247453009504));
#168484=CARTESIAN_POINT('Ctrl Pts',(5.75857177593739,5.73592888894683,64.8328092862105));
#168485=CARTESIAN_POINT('Ctrl Pts',(5.61136262212376,5.88002484189713,64.8408732714705));
#168486=CARTESIAN_POINT('Ctrl Pts',(5.45885245468371,6.01835670598658,64.8489372567306));
#168487=CARTESIAN_POINT('Ctrl Pts',(5.30422288429272,6.15861094001294,64.8571133055628));
#168488=CARTESIAN_POINT('Ctrl Pts',(5.14414408985453,6.29293944186506,64.8652893543951));
#168489=CARTESIAN_POINT('Ctrl Pts',(4.97910310419053,6.42092048232496,64.8734654032273));
#168490=CARTESIAN_POINT('Ctrl Pts',(4.81640134625806,6.54708756852527,64.8815255678742));
#168491=CARTESIAN_POINT('Ctrl Pts',(4.64887739338601,6.66708574316072,64.8895857325212));
#168492=CARTESIAN_POINT('Ctrl Pts',(4.47703087278741,6.78055175679741,64.8976458971681));
#168493=CARTESIAN_POINT('Ctrl Pts',(4.30519265494977,6.89401228832608,64.9057056723884));
#168494=CARTESIAN_POINT('Ctrl Pts',(4.12903255032156,7.0009411138893,64.9137654476087));
#168495=CARTESIAN_POINT('Ctrl Pts',(3.94907906025992,7.10101838740871,64.9218252228289));
#168496=CARTESIAN_POINT('Ctrl Pts',(3.7691119834814,7.20110321688929,64.9298856065724));
#168497=CARTESIAN_POINT('Ctrl Pts',(3.58535122715576,7.29433530912716,64.937945990316));
#168498=CARTESIAN_POINT('Ctrl Pts',(3.39835029725013,7.38044055728924,64.9460063740595));
#168499=CARTESIAN_POINT('Ctrl Pts',(3.20664856386755,7.46871030725432,64.9542693786132));
#168500=CARTESIAN_POINT('Ctrl Pts',(3.01154193451114,7.54949005618894,64.9625323831669));
#168501=CARTESIAN_POINT('Ctrl Pts',(2.81364914934523,7.62253671863172,64.9707953877207));
#168502=CARTESIAN_POINT('Ctrl Pts',(2.6204502380647,7.69385076701802,64.9788623997765));
#168503=CARTESIAN_POINT('Ctrl Pts',(2.42459615555917,7.75779433221035,64.9869294118323));
#168504=CARTESIAN_POINT('Ctrl Pts',(2.2266789549132,7.81419147412237,64.9949964238881));
#168505=CARTESIAN_POINT('Ctrl Pts',(2.02154899328362,7.87264391543959,65.0033574246908));
#168506=CARTESIAN_POINT('Ctrl Pts',(1.8142030762292,7.9229894697624,65.0117184254935));
#168507=CARTESIAN_POINT('Ctrl Pts',(1.60531331324235,7.96508987575324,65.0200794262962));
#168508=CARTESIAN_POINT('Ctrl Pts',(1.39642355025551,8.00719028174409,65.0284404270989));
#168509=CARTESIAN_POINT('Ctrl Pts',(1.18599031746624,8.04104550326096,65.0368014279016));
#168510=CARTESIAN_POINT('Ctrl Pts',(0.974693342527283,8.06657674918754,
65.0451624287043));
#168511=CARTESIAN_POINT('Ctrl Pts',(0.783177967084079,8.0897177626856,65.0527406735337));
#168512=CARTESIAN_POINT('Ctrl Pts',(0.590569177841376,8.10606658349232,
65.0603189183632));
#168513=CARTESIAN_POINT('Ctrl Pts',(0.397410233080106,8.1155254093092,65.0678971631926));
#168514=CARTESIAN_POINT('Ctrl Pts',(0.204395022967877,8.1249771965651,65.0754697688509));
#168515=CARTESIAN_POINT('Ctrl Pts',(0.0108308363557188,8.1275491704616,
65.0830423745091));
#168516=CARTESIAN_POINT('Ctrl Pts',(-0.182731308424958,8.12319498912967,
65.0906149801674));
#168517=CARTESIAN_POINT('Ctrl Pts',(-0.376186175457095,8.11884322101118,
65.0981833888682));
#168518=CARTESIAN_POINT('Ctrl Pts',(-0.569638636746874,8.1075729443288,
65.105751797569));
#168519=CARTESIAN_POINT('Ctrl Pts',(-0.762535075129235,8.08938982999939,
65.1133202062698));
#168520=CARTESIAN_POINT('Ctrl Pts',(-0.955384908191962,8.07121110885558,
65.1208867863826));
#168521=CARTESIAN_POINT('Ctrl Pts',(-1.14767861953453,8.04612290088425,
65.1284533664954));
#168522=CARTESIAN_POINT('Ctrl Pts',(-1.33886498399562,8.01418293509266,
65.1360199466082));
#168523=CARTESIAN_POINT('Ctrl Pts',(-1.53001743286074,7.98224863530648,
65.1435851844439));
#168524=CARTESIAN_POINT('Ctrl Pts',(-1.72006256367128,7.94346506070241,
65.1511504222797));
#168525=CARTESIAN_POINT('Ctrl Pts',(-1.90845692468996,7.8979414868118,65.1587156601155));
#168526=CARTESIAN_POINT('Ctrl Pts',(-2.09691679946813,7.85240208219007,
65.1662835287474));
#168527=CARTESIAN_POINT('Ctrl Pts',(-2.28372439897868,7.80011807910052,
65.1738513973794));
#168528=CARTESIAN_POINT('Ctrl Pts',(-2.46834860628678,7.74124942889338,
65.1814192660114));
#168529=CARTESIAN_POINT('Ctrl Pts',(-2.65059033673784,7.68314044719758,
65.1888894753378));
#168530=CARTESIAN_POINT('Ctrl Pts',(-2.83070437198839,7.61861589268249,
65.1963596846642));
#168531=CARTESIAN_POINT('Ctrl Pts',(-3.00819722506586,7.54787632500732,
65.2038298939906));
#168532=CARTESIAN_POINT('Ctrl Pts',(-3.22930486420425,7.45975413568458,
65.2131357354338));
#168533=CARTESIAN_POINT('Ctrl Pts',(-3.44623709793891,7.36203258265992,
65.2224415768769));
#168534=CARTESIAN_POINT('Ctrl Pts',(-3.65826586947159,7.25512083915625,
65.2317474183201));
#168535=CARTESIAN_POINT('Ctrl Pts',(-3.87143298070287,7.14763510807062,
65.2411032209485));
#168536=CARTESIAN_POINT('Ctrl Pts',(-4.07964382046493,7.03086030960335,
65.250459023577));
#168537=CARTESIAN_POINT('Ctrl Pts',(-4.28219177836065,6.90525315508711,
65.2598148262055));
#168538=CARTESIAN_POINT('Ctrl Pts',(-4.48572299623879,6.77903624626959,
65.2692160461584));
#168539=CARTESIAN_POINT('Ctrl Pts',(-4.68353619515957,6.64390106325968,
65.2786172661114));
#168540=CARTESIAN_POINT('Ctrl Pts',(-4.87494818340455,6.50035135755142,
65.2880184860643));
#168541=CARTESIAN_POINT('Ctrl Pts',(-5.06656733622119,6.35664628846407,
65.297429880927));
#168542=CARTESIAN_POINT('Ctrl Pts',(-5.25177139773545,6.20450851170978,
65.3068412757897));
#168543=CARTESIAN_POINT('Ctrl Pts',(-5.42990897238826,6.04448311388802,
65.3162526706524));
#168544=CARTESIAN_POINT('Ctrl Pts',(-5.60783758867829,5.88464542854186,
65.3256530257911));
#168545=CARTESIAN_POINT('Ctrl Pts',(-5.77871626236403,5.71693864341223,
65.3350533809298));
#168546=CARTESIAN_POINT('Ctrl Pts',(-5.94193009243925,5.54194499603387,
65.3444537360684));
#168547=CARTESIAN_POINT('Ctrl Pts',(-6.04635766667792,5.42998045176408,
65.350468277138));
#168548=CARTESIAN_POINT('Ctrl Pts',(-6.14764816864232,5.31503366556899,
65.3564828182076));
#168549=CARTESIAN_POINT('Ctrl Pts',(-6.24564800006565,5.19726549464003,
65.3624973592772));
#168550=CARTESIAN_POINT('Ctrl Pts',(-6.37179959516469,5.0456668398382,65.3702396577965));
#168551=CARTESIAN_POINT('Ctrl Pts',(-6.49255525770672,4.88931979925239,
65.3779819563158));
#168552=CARTESIAN_POINT('Ctrl Pts',(-6.60753570050326,4.72865303538703,
65.385724254835));
#168553=CARTESIAN_POINT('Ctrl Pts',(-6.72244452089595,4.56808635236642,
65.3934617306034));
#168554=CARTESIAN_POINT('Ctrl Pts',(-6.83158507970928,4.40320558982517,
65.4011992063718));
#168555=CARTESIAN_POINT('Ctrl Pts',(-6.93461813499328,4.23447268078592,
65.4089366821402));
#168556=CARTESIAN_POINT('Ctrl Pts',(-7.03760532195016,4.06581488838033,
65.4166707133338));
#168557=CARTESIAN_POINT('Ctrl Pts',(-7.13449023674341,3.89330866577138,
65.4244047445273));
#168558=CARTESIAN_POINT('Ctrl Pts',(-7.22497670516621,3.71744524805754,
65.4321387757209));
#168559=CARTESIAN_POINT('Ctrl Pts',(-7.31545159417055,3.54160433532307,
65.439871817202));
#168560=CARTESIAN_POINT('Ctrl Pts',(-7.39952949935549,3.36240739363301,
65.4476048586831));
#168561=CARTESIAN_POINT('Ctrl Pts',(-7.4769598305001,3.18037093050289,65.4553379001642));
#168562=CARTESIAN_POINT('Ctrl Pts',(-7.5543824264124,2.99835265267963,65.4630701691203));
#168563=CARTESIAN_POINT('Ctrl Pts',(-7.62515863606883,2.81349574505808,
65.4708024380763));
#168564=CARTESIAN_POINT('Ctrl Pts',(-7.68908577496729,2.62633727988155,
65.4785347070324));
#168565=CARTESIAN_POINT('Ctrl Pts',(-7.75303750372862,2.43910682335563,
65.4862699502406));
#168566=CARTESIAN_POINT('Ctrl Pts',(-7.81013478380173,2.24957337519464,
65.4940051934488));
#168567=CARTESIAN_POINT('Ctrl Pts',(-7.86022443591833,2.05829040212803,
65.5017404366571));
#168568=CARTESIAN_POINT('Ctrl Pts',(-7.90215204813046,1.89817672637618,
65.5082152326258));
#168569=CARTESIAN_POINT('Ctrl Pts',(-7.9391705845897,1.73683761587606,65.5146900285946));
#168570=CARTESIAN_POINT('Ctrl Pts',(-7.97121767767376,1.57460353665337,
65.5211648245634));
#168571=CARTESIAN_POINT('Ctrl Pts',(-8.0128632569568,1.36377841778982,65.5295788990678));
#168572=CARTESIAN_POINT('Ctrl Pts',(-8.04613274282637,1.15134020973383,
65.5379929735722));
#168573=CARTESIAN_POINT('Ctrl Pts',(-8.07093121654614,0.937953549106291,
65.5464070480766));
#168574=CARTESIAN_POINT('Ctrl Pts',(-8.09573661579727,0.724507295455871,
65.5548234724005));
#168575=CARTESIAN_POINT('Ctrl Pts',(-8.11206624965703,0.510112322727504,
65.5632398967244));
#168576=CARTESIAN_POINT('Ctrl Pts',(-8.11987707135234,0.295438502275071,
65.5716563210483));
#168577=CARTESIAN_POINT('Ctrl Pts',(-8.127689830077,0.0807114442110189,
65.5800748325867));
#168578=CARTESIAN_POINT('Ctrl Pts',(-8.12697954942962,-0.134294335862574,
65.5884933441252));
#168579=CARTESIAN_POINT('Ctrl Pts',(-8.11775528991404,-0.348907746507043,
65.5969118556637));
#168580=CARTESIAN_POINT('Ctrl Pts',(-8.10852748739891,-0.563603589266107,
65.6053336007173));
#168581=CARTESIAN_POINT('Ctrl Pts',(-8.09077918113527,-0.777906497569484,
65.6137553457709));
#168582=CARTESIAN_POINT('Ctrl Pts',(-8.06457150215843,-0.991147844205967,
65.6221770908245));
#168583=CARTESIAN_POINT('Ctrl Pts',(-8.03836098234078,-1.20441230562191,
65.6305997487723));
#168584=CARTESIAN_POINT('Ctrl Pts',(-8.00368929417285,-1.41661471401595,
65.63902240672));
#168585=CARTESIAN_POINT('Ctrl Pts',(-7.9606692324782,-1.62709340038455,
65.6474450646678));
#168586=CARTESIAN_POINT('Ctrl Pts',(-7.91764098960571,-1.83761211374279,
65.6558693243627));
#168587=CARTESIAN_POINT('Ctrl Pts',(-7.86626125443626,-2.04640619163457,
65.6642935840577));
#168588=CARTESIAN_POINT('Ctrl Pts',(-7.80669383373301,-2.2528246600335,
65.6727178437526));
#168589=CARTESIAN_POINT('Ctrl Pts',(-7.78992523055216,-2.31093275578307,
65.675089325785));
#168590=CARTESIAN_POINT('Ctrl Pts',(-7.77250809447315,-2.36885267483412,
65.6774608078175));
#168591=CARTESIAN_POINT('Ctrl Pts',(-7.75444679713041,-2.42657009644764,
65.6798322898499));
#168592=CARTESIAN_POINT('Ctrl Pts',(-7.69028681589047,-2.63160236061273,
65.6882566150701));
#168593=CARTESIAN_POINT('Ctrl Pts',(-7.6179876353172,-2.83409919470438,
65.6966809402902));
#168594=CARTESIAN_POINT('Ctrl Pts',(-7.53777193415858,-3.03342740659986,
65.7051052655103));
#168595=CARTESIAN_POINT('Ctrl Pts',(-7.45757009525431,-3.23272117214219,
65.713528134904));
#168596=CARTESIAN_POINT('Ctrl Pts',(-7.36945456670468,-3.4288471644451,
65.7219510042977));
#168597=CARTESIAN_POINT('Ctrl Pts',(-7.27369646623844,-3.62119141713475,
65.7303738736913));
#168598=CARTESIAN_POINT('Ctrl Pts',(-7.17795793410072,-3.8134963639536,
65.7387950218575));
#168599=CARTESIAN_POINT('Ctrl Pts',(-7.07458006635887,-4.0020208782696,
65.7472161700237));
#168600=CARTESIAN_POINT('Ctrl Pts',(-6.96388079188532,-4.1861738949679,
65.7556373181899));
#168601=CARTESIAN_POINT('Ctrl Pts',(-6.8532125758928,-4.37027524454368,
65.7640561036661));
#168602=CARTESIAN_POINT('Ctrl Pts',(-6.73522719171313,-4.55000732009851,
65.7724748891422));
#168603=CARTESIAN_POINT('Ctrl Pts',(-6.61028742604854,-4.72480557351565,
65.7808936746184));
#168604=CARTESIAN_POINT('Ctrl Pts',(-6.48538256147108,-4.89955499821088,
65.7893101083632));
#168605=CARTESIAN_POINT('Ctrl Pts',(-6.35352734749046,-5.0693731380007,
65.797726542108));
#168606=CARTESIAN_POINT('Ctrl Pts',(-6.21512728728488,-5.23372528562083,
65.8061429758528));
#168607=CARTESIAN_POINT('Ctrl Pts',(-6.07677745825526,-5.39801778296601,
65.8145563549215));
#168608=CARTESIAN_POINT('Ctrl Pts',(-5.93188769648226,-5.55684804811031,
65.8229697339901));
#168609=CARTESIAN_POINT('Ctrl Pts',(-5.78090372687759,-5.70971449926113,
65.8313831130587));
#168610=CARTESIAN_POINT('Ctrl Pts',(-5.73833268764744,-5.75281631799033,
65.8337553270847));
#168611=CARTESIAN_POINT('Ctrl Pts',(-5.69527739883983,-5.7954442227784,
65.8361275411106));
#168612=CARTESIAN_POINT('Ctrl Pts',(-5.65174840765014,-5.83758747250301,
65.8384997551366));
#168613=CARTESIAN_POINT('Ctrl Pts',(-5.50981146935305,-5.97500586131276,
65.8462349400473));
#168614=CARTESIAN_POINT('Ctrl Pts',(-5.36277205502693,-6.10732929945869,
65.853970124958));
#168615=CARTESIAN_POINT('Ctrl Pts',(-5.21104173523728,-6.23415845131604,
65.8617053098687));
#168616=CARTESIAN_POINT('Ctrl Pts',(-5.05935833421132,-6.36094838446606,
65.8694381028691));
#168617=CARTESIAN_POINT('Ctrl Pts',(-4.90298718710356,-6.482247188371,65.8771708958695));
#168618=CARTESIAN_POINT('Ctrl Pts',(-4.74237469106222,-6.59769428301073,
65.8849036888699));
#168619=CARTESIAN_POINT('Ctrl Pts',(-4.58178332418309,-6.71312619016226,
65.892635464593));
#168620=CARTESIAN_POINT('Ctrl Pts',(-4.41695200700344,-6.82270771587853,
65.9003672403161));
#168621=CARTESIAN_POINT('Ctrl Pts',(-4.24835810269068,-6.9261201977588,
65.9080990160393));
#168622=CARTESIAN_POINT('Ctrl Pts',(-4.07970387087586,-7.02956968344856,
65.9158335584029));
#168623=CARTESIAN_POINT('Ctrl Pts',(-3.90728466128152,-7.12684552647708,
65.9235681007666));
#168624=CARTESIAN_POINT('Ctrl Pts',(-3.73160512545452,-7.21767349983231,
65.9313026431302));
#168625=CARTESIAN_POINT('Ctrl Pts',(-3.5558959193128,-7.30851681301947,
65.9390384917717));
#168626=CARTESIAN_POINT('Ctrl Pts',(-3.37692560721234,-7.39290993116816,
65.9467743404133));
#168627=CARTESIAN_POINT('Ctrl Pts',(-3.1952211884978,-7.47062575150667,
65.9545101890549));
#168628=CARTESIAN_POINT('Ctrl Pts',(-3.01336809100004,-7.54840516244847,
65.9622523675181));
#168629=CARTESIAN_POINT('Ctrl Pts',(-2.82877674517088,-7.61949622739521,
65.9699945459813));
#168630=CARTESIAN_POINT('Ctrl Pts',(-2.6419926466829,-7.68372061031461,
65.9777367244445));
#168631=CARTESIAN_POINT('Ctrl Pts',(-2.48573569257516,-7.73744845190108,
65.9842135564373));
#168632=CARTESIAN_POINT('Ctrl Pts',(-2.32794456532243,-7.78637155989766,
65.99069038843));
#168633=CARTESIAN_POINT('Ctrl Pts',(-2.16894526312171,-7.83041276102875,
65.9971672204228));
#168634=CARTESIAN_POINT('Ctrl Pts',(-1.93823370989737,-7.89431753154146,
66.0065652488942));
#168635=CARTESIAN_POINT('Ctrl Pts',(-1.70484733732744,-7.94798006146225,
66.0159632773656));
#168636=CARTESIAN_POINT('Ctrl Pts',(-1.46961859860419,-7.99123949942289,
66.025361305837));
#168637=CARTESIAN_POINT('Ctrl Pts',(-1.23405514907411,-8.03456049194298,
66.0347727069163));
#168638=CARTESIAN_POINT('Ctrl Pts',(-0.996644126168747,-8.06744877566463,
66.0441841079956));
#168639=CARTESIAN_POINT('Ctrl Pts',(-0.758227768568692,-8.08979469538451,
66.053595509075));
#168640=CARTESIAN_POINT('Ctrl Pts',(-0.520170387033364,-8.11210696955085,
66.0629927397016));
#168641=CARTESIAN_POINT('Ctrl Pts',(-0.281110732766663,-8.12390860495421,
66.0723899703282));
#168642=CARTESIAN_POINT('Ctrl Pts',(-0.0418928781699178,-8.12514200179041,
66.0817872009548));
#168643=CARTESIAN_POINT('Ctrl Pts',(0.196721579760263,-8.12637228753968,
66.0911607282603));
#168644=CARTESIAN_POINT('Ctrl Pts',(0.435493403104585,-8.11708756041705,
66.1005342555657));
#168645=CARTESIAN_POINT('Ctrl Pts',(0.67357983644703,-8.09728212219582,
66.1099077828712));
#168646=CARTESIAN_POINT('Ctrl Pts',(0.910120150477342,-8.07760529932695,
66.119220439041));
#168647=CARTESIAN_POINT('Ctrl Pts',(1.1459839011936,-8.04754394588073,66.1285330952107));
#168648=CARTESIAN_POINT('Ctrl Pts',(1.38034027614664,-8.00714357836472,
66.1378457513805));
#168649=CARTESIAN_POINT('Ctrl Pts',(1.5312396315234,-7.98113024966235,66.1438420628234));
#168650=CARTESIAN_POINT('Ctrl Pts',(1.68151395299948,-7.95083147595598,
66.1498383742664));
#168651=CARTESIAN_POINT('Ctrl Pts',(1.83094063365618,-7.91627083660777,
66.1558346857094));
#168652=CARTESIAN_POINT('Ctrl Pts',(2.019524908843,-7.87265350473082,66.1634023439234));
#168653=CARTESIAN_POINT('Ctrl Pts',(2.20668353749748,-7.82226218231101,
66.1709700021374));
#168654=CARTESIAN_POINT('Ctrl Pts',(2.39187619588993,-7.76521833730611,
66.1785376603514));
#168655=CARTESIAN_POINT('Ctrl Pts',(2.5770175777641,-7.70819028671654,66.1861032232169));
#168656=CARTESIAN_POINT('Ctrl Pts',(2.76019372147561,-7.64451348672376,
66.1936687860824));
#168657=CARTESIAN_POINT('Ctrl Pts',(2.9408777532014,-7.5743597487329,66.2012343489479));
#168658=CARTESIAN_POINT('Ctrl Pts',(3.12154595529721,-7.50421215687296,
66.2087992489985));
#168659=CARTESIAN_POINT('Ctrl Pts',(3.2997221375484,-7.42758889031082,66.2163641490491));
#168660=CARTESIAN_POINT('Ctrl Pts',(3.47489782680054,-7.34471052226001,
66.2239290490998));
#168661=CARTESIAN_POINT('Ctrl Pts',(3.65015949119813,-7.26179147801846,
66.2314976619566));
#168662=CARTESIAN_POINT('Ctrl Pts',(3.82241738636469,-7.1726113536418,66.2390662748134));
#168663=CARTESIAN_POINT('Ctrl Pts',(3.99118564096093,-7.07743772433833,
66.2466348876702));
#168664=CARTESIAN_POINT('Ctrl Pts',(4.15999142665,-6.98224293009288,66.2542051836535));
#168665=CARTESIAN_POINT('Ctrl Pts',(4.32530571129203,-6.88105216643253,
66.2617754796367));
#168666=CARTESIAN_POINT('Ctrl Pts',(4.48667044834525,-6.77417713456368,
66.26934577562));
#168667=CARTESIAN_POINT('Ctrl Pts',(4.64819869387933,-6.66719380781938,
66.2769237424712));
#168668=CARTESIAN_POINT('Ctrl Pts',(4.8057690958993,-6.55451491788855,66.2845017093224));
#168669=CARTESIAN_POINT('Ctrl Pts',(4.95895490144321,-6.43649390957161,
66.2920796761737));
#168670=CARTESIAN_POINT('Ctrl Pts',(5.11004225487672,-6.32008964004515,
66.2995538344476));
#168671=CARTESIAN_POINT('Ctrl Pts',(5.2568641558625,-6.19848894671413,66.3070279927216));
#168672=CARTESIAN_POINT('Ctrl Pts',(5.3990461284708,-6.07206624347466,66.3145021509956));
#168673=CARTESIAN_POINT('Ctrl Pts',(5.55066229334044,-5.93725502186904,
66.3224722416642));
#168674=CARTESIAN_POINT('Ctrl Pts',(5.69734896901088,-5.79665286581093,
66.3304423323328));
#168675=CARTESIAN_POINT('Ctrl Pts',(5.83864923950696,-5.65065152177205,
66.3384124230014));
#168676=CARTESIAN_POINT('Ctrl Pts',(5.97984530484417,-5.50475784980767,
66.3463766359419));
#168677=CARTESIAN_POINT('Ctrl Pts',(6.11566265520476,-5.35347316287123,
66.3543408488824));
#168678=CARTESIAN_POINT('Ctrl Pts',(6.24567951906185,-5.1972276174583,66.362305061823));
#168679=CARTESIAN_POINT('Ctrl Pts',(6.37562157182863,-5.04107197499536,
66.3702646921929));
#168680=CARTESIAN_POINT('Ctrl Pts',(6.49976958184366,-4.87996141738763,
66.3782243225629));
#168681=CARTESIAN_POINT('Ctrl Pts',(6.61774022143442,-4.71436124242819,
66.3861839529329));
#168682=CARTESIAN_POINT('Ctrl Pts',(6.73946700311993,-4.54348841835689,
66.3943970150279));
#168683=CARTESIAN_POINT('Ctrl Pts',(6.85461631368951,-4.36783563087224,
66.4026100771228));
#168684=CARTESIAN_POINT('Ctrl Pts',(6.96281284365788,-4.18794995990794,
66.4108231392178));
#168685=CARTESIAN_POINT('Ctrl Pts',(7.06761032618024,-4.01371548617374,
66.4187781839092));
#168686=CARTESIAN_POINT('Ctrl Pts',(7.16588506826533,-3.83551035095584,
66.4267332286006));
#168687=CARTESIAN_POINT('Ctrl Pts',(7.25734064468932,-3.65386019566163,
66.434688273292));
#168688=CARTESIAN_POINT('Ctrl Pts',(7.34879156817336,-3.47221928209216,
66.4426429132586));
#168689=CARTESIAN_POINT('Ctrl Pts',(7.43342386938551,-3.28713399200113,
66.4505975532251));
#168690=CARTESIAN_POINT('Ctrl Pts',(7.51098757048573,-3.0991536390616,66.4585521931917));
#168691=CARTESIAN_POINT('Ctrl Pts',(7.58855872367093,-2.91115522554034,
66.4665075974159));
#168692=CARTESIAN_POINT('Ctrl Pts',(7.65905979750801,-2.7202614992951,66.4744630016401));
#168693=CARTESIAN_POINT('Ctrl Pts',(7.72228919296004,-2.52704119135257,
66.4824184058643));
#168694=CARTESIAN_POINT('Ctrl Pts',(7.78553395553669,-2.33377392359758,
66.4903757435513));
#168695=CARTESIAN_POINT('Ctrl Pts',(7.84150341454393,-2.13817926000058,
66.4983330812384));
#168696=CARTESIAN_POINT('Ctrl Pts',(7.8900458824695,-1.94084093501404,66.5062904189255));
#168697=CARTESIAN_POINT('Ctrl Pts',(7.93862466296796,-1.74335498954962,
66.5142537091613));
#168698=CARTESIAN_POINT('Ctrl Pts',(7.97976527492132,-1.5441230970558,66.5222169993971));
#168699=CARTESIAN_POINT('Ctrl Pts',(8.01336696446453,-1.34374009962063,
66.5301802896329));
#168700=CARTESIAN_POINT('Ctrl Pts',(8.0469835021482,-1.14326855559952,66.5381470987409));
#168701=CARTESIAN_POINT('Ctrl Pts',(8.07305442770735,-0.941645218064171,
66.5461139078489));
#168702=CARTESIAN_POINT('Ctrl Pts',(8.09153080529629,-0.739470614318915,
66.5540807169569));
#168703=CARTESIAN_POINT('Ctrl Pts',(8.11002432341238,-0.537108453285023,
66.5620549168701));
#168704=CARTESIAN_POINT('Ctrl Pts',(8.12090920015154,-0.334194332843433,
66.5700291167833));
#168705=CARTESIAN_POINT('Ctrl Pts',(8.12418856789581,-0.131330406878931,
66.5780033166966));
#168706=CARTESIAN_POINT('Ctrl Pts',(8.12491429954366,-0.0864361520226109,
66.5797680255351));
#168707=CARTESIAN_POINT('Ctrl Pts',(8.12526775567514,-0.0415443442075146,
66.5815327343737));
#168708=CARTESIAN_POINT('Ctrl Pts',(8.12524931413266,0.00333851565678357,
66.5832974432123));
#168709=CARTESIAN_POINT('',(8.12804752138609,-0.000138485946060349,68.5832974432123));
#168710=CARTESIAN_POINT('Ctrl Pts',(8.12588319212561,0.00333877610560675,
66.5832974432123));
#168711=CARTESIAN_POINT('Ctrl Pts',(8.1295781066157,0.41488469301549,66.5994773226644));
#168712=CARTESIAN_POINT('Ctrl Pts',(8.00961219341291,2.17106617787553,66.6685463572119));
#168713=CARTESIAN_POINT('Ctrl Pts',(6.72405806064653,5.12185486701279,66.790504546855));
#168714=CARTESIAN_POINT('Ctrl Pts',(2.38173522129256,8.63148943733764,67.0020611672368));
#168715=CARTESIAN_POINT('Ctrl Pts',(-3.67416070295623,8.17511883464795,
67.2136177876189));
#168716=CARTESIAN_POINT('Ctrl Pts',(-7.44199729007036,4.01675585914095,
67.4251744080006));
#168717=CARTESIAN_POINT('Ctrl Pts',(-8.47097384492055,-0.00353968824724416,
67.5838418732871));
#168718=CARTESIAN_POINT('Ctrl Pts',(-7.43229334537619,-4.06791197667408,
67.7425093385735));
#168719=CARTESIAN_POINT('Ctrl Pts',(-4.58332861377674,-7.11692082205451,
67.9011768038601));
#168720=CARTESIAN_POINT('Ctrl Pts',(-0.628874882635375,-8.44934367887127,
68.0598442691463));
#168721=CARTESIAN_POINT('Ctrl Pts',(3.5010973142339,-7.7136066795621,68.2185117344329));
#168722=CARTESIAN_POINT('Ctrl Pts',(6.73558121933879,-5.11366765981602,
68.3771791997192));
#168723=CARTESIAN_POINT('Ctrl Pts',(8.01567158785016,-2.15330402273112,
68.4987744359791));
#168724=CARTESIAN_POINT('Ctrl Pts',(8.13188959766798,-0.403006519366052,
68.5674805171434));
#168725=CARTESIAN_POINT('Ctrl Pts',(8.12804752138609,-0.000138485946060349,
68.5832974432123));
#168726=CARTESIAN_POINT('',(8.12524925928675,-0.00225863613891466,70.5832974432123));
#168727=CARTESIAN_POINT('Ctrl Pts',(8.12524999882064,-0.000138438281777881,
68.5832974432123));
#168728=CARTESIAN_POINT('Ctrl Pts',(8.12525344319759,0.202019689155656,
68.5912370693852));
#168729=CARTESIAN_POINT('Ctrl Pts',(8.11770794645236,0.40434051216219,68.5991766955581));
#168730=CARTESIAN_POINT('Ctrl Pts',(8.10260312143478,0.606226211092314,
68.607116321731));
#168731=CARTESIAN_POINT('Ctrl Pts',(8.08750875266733,0.807972155516052,
68.6150504517318));
#168732=CARTESIAN_POINT('Ctrl Pts',(8.06486551056691,1.00928324548818,68.6229845817327));
#168733=CARTESIAN_POINT('Ctrl Pts',(8.03471506847395,1.20956245433532,68.6309187117335));
#168734=CARTESIAN_POINT('Ctrl Pts',(8.00458042802503,1.40973669819528,68.6388486835101));
#168735=CARTESIAN_POINT('Ctrl Pts',(7.96694648021616,1.60887981058078,68.6467786552868));
#168736=CARTESIAN_POINT('Ctrl Pts',(7.92190669876364,1.80640023765051,68.6547086270634));
#168737=CARTESIAN_POINT('Ctrl Pts',(7.87493732643615,2.01238281976186,68.6629783340849));
#168738=CARTESIAN_POINT('Ctrl Pts',(7.81991362556992,2.21660024398525,68.6712480411063));
#168739=CARTESIAN_POINT('Ctrl Pts',(7.75700099036818,2.4183926889418,68.6795177481278));
#168740=CARTESIAN_POINT('Ctrl Pts',(7.69669787882304,2.61181507982017,68.6874444398545));
#168741=CARTESIAN_POINT('Ctrl Pts',(7.62914716804387,2.80300925359413,68.6953711315812));
#168742=CARTESIAN_POINT('Ctrl Pts',(7.55454566102255,2.99140893527202,68.703297823308));
#168743=CARTESIAN_POINT('Ctrl Pts',(7.47994280837504,3.17981201521298,68.7112246580126));
#168744=CARTESIAN_POINT('Ctrl Pts',(7.39828902825326,3.36542019290255,68.7191514927172));
#168745=CARTESIAN_POINT('Ctrl Pts',(7.30982958087123,3.54768643782395,68.7270783274218));
#168746=CARTESIAN_POINT('Ctrl Pts',(7.22135505292155,3.72998375549695,68.7350065134932));
#168747=CARTESIAN_POINT('Ctrl Pts',(7.12607269037901,3.90893770524193,68.7429346995647));
#168748=CARTESIAN_POINT('Ctrl Pts',(7.02427426820815,4.08402480005801,68.7508628856362));
#168749=CARTESIAN_POINT('Ctrl Pts',(6.92244297212418,4.25916843600526,68.7587936319684));
#168750=CARTESIAN_POINT('Ctrl Pts',(6.81409158925194,4.43044244026811,68.7667243783005));
#168751=CARTESIAN_POINT('Ctrl Pts',(6.69955607677724,4.59735096948418,68.7746551246327));
#168752=CARTESIAN_POINT('Ctrl Pts',(6.58491859003713,4.76440810217083,68.7825929319367));
#168753=CARTESIAN_POINT('Ctrl Pts',(6.46408616331075,4.92709172093237,68.7905307392408));
#168754=CARTESIAN_POINT('Ctrl Pts',(6.3374367117051,5.08493692071322,68.7984685465448));
#168755=CARTESIAN_POINT('Ctrl Pts',(6.21072145558343,5.24286413369543,68.8064104781744));
#168756=CARTESIAN_POINT('Ctrl Pts',(6.07818336292514,5.39594766144925,68.814352409804));
#168757=CARTESIAN_POINT('Ctrl Pts',(5.94023870550447,5.54375790273408,68.8222943414336));
#168758=CARTESIAN_POINT('Ctrl Pts',(5.80214559088934,5.69172721863727,68.8302448202364));
#168759=CARTESIAN_POINT('Ctrl Pts',(5.65863452315447,5.83441167634531,68.8381952990393));
#168760=CARTESIAN_POINT('Ctrl Pts',(5.51015728330688,5.97141978726334,68.8461457778421));
#168761=CARTESIAN_POINT('Ctrl Pts',(5.46635871370853,6.01183513501455,68.8484910504209));
#168762=CARTESIAN_POINT('Ctrl Pts',(5.42212821852692,6.05175682146519,68.8508363229997));
#168763=CARTESIAN_POINT('Ctrl Pts',(5.37747790964115,6.09117549359904,68.8531815955785));
#168764=CARTESIAN_POINT('Ctrl Pts',(5.22368644638327,6.22694734867524,68.8612595442115));
#168765=CARTESIAN_POINT('Ctrl Pts',(5.06457738629581,6.3570440359296,68.8693374928446));
#168766=CARTESIAN_POINT('Ctrl Pts',(4.90059376393837,6.48103913916189,68.8774154414776));
#168767=CARTESIAN_POINT('Ctrl Pts',(4.73681082423041,6.60488249757064,68.8854835043421));
#168768=CARTESIAN_POINT('Ctrl Pts',(4.56816546328188,6.72263896752202,68.8935515672066));
#168769=CARTESIAN_POINT('Ctrl Pts',(4.39513582047105,6.83392044745271,68.9016196300711));
#168770=CARTESIAN_POINT('Ctrl Pts',(4.22229662866159,6.94507944161194,68.9096788125459));
#168771=CARTESIAN_POINT('Ctrl Pts',(4.04508303914585,7.04977748374946,68.9177379950208));
#168772=CARTESIAN_POINT('Ctrl Pts',(3.86400487316773,7.14766772469426,68.9257971774957));
#168773=CARTESIAN_POINT('Ctrl Pts',(3.68315929576284,7.24543222904707,68.9338460082324));
#168774=CARTESIAN_POINT('Ctrl Pts',(3.49845932115371,7.33640622748188,68.9418948389691));
#168775=CARTESIAN_POINT('Ctrl Pts',(3.31044228304972,7.42028701959005,68.9499436697058));
#168776=CARTESIAN_POINT('Ctrl Pts',(3.12256746018415,7.50410436464593,68.9579864123433));
#168777=CARTESIAN_POINT('Ctrl Pts',(2.93138086200307,7.58083906962743,68.9660291549808));
#168778=CARTESIAN_POINT('Ctrl Pts',(2.73744408463825,7.65023447000019,68.9740718976183));
#168779=CARTESIAN_POINT('Ctrl Pts',(2.54366527608003,7.7195733452067,68.9821080891391));
#168780=CARTESIAN_POINT('Ctrl Pts',(2.34714105325024,7.78158473475308,68.99014428066));
#168781=CARTESIAN_POINT('Ctrl Pts',(2.1484529019483,7.83606008722559,68.9981804721808));
#168782=CARTESIAN_POINT('Ctrl Pts',(2.03580473979545,7.86694541329283,69.0027366684089));
#168783=CARTESIAN_POINT('Ctrl Pts',(1.92246136079458,7.89540920653068,69.007292864637));
#168784=CARTESIAN_POINT('Ctrl Pts',(1.80853123420579,7.92142047472561,69.0118490608651));
#168785=CARTESIAN_POINT('Ctrl Pts',(1.60757388525393,7.96730083715331,69.0198855753737));
#168786=CARTESIAN_POINT('Ctrl Pts',(1.40494924650344,8.00551172220066,69.0279220898824));
#168787=CARTESIAN_POINT('Ctrl Pts',(1.20126884395045,8.03595922880734,69.035958604391));
#168788=CARTESIAN_POINT('Ctrl Pts',(0.997465398160986,8.06642512873862,
69.0439999737544));
#168789=CARTESIAN_POINT('Ctrl Pts',(0.792605228504791,8.08911824702432,
69.0520413431177));
#168790=CARTESIAN_POINT('Ctrl Pts',(0.587305116801611,8.10399656109741,
69.060082712481));
#168791=CARTESIAN_POINT('Ctrl Pts',(0.381855881596666,8.11888568230682,
69.0681299228405));
#168792=CARTESIAN_POINT('Ctrl Pts',(0.175966381454576,8.12594865147517,
69.0761771332));
#168793=CARTESIAN_POINT('Ctrl Pts',(-0.0297458548209949,8.12519555128496,
69.0842243435594));
#168794=CARTESIAN_POINT('Ctrl Pts',(-0.235761296243941,8.12444134107885,
69.0922834149323));
#168795=CARTESIAN_POINT('Ctrl Pts',(-0.441598635417027,8.11584803745462,
69.1003424863052));
#168796=CARTESIAN_POINT('Ctrl Pts',(-0.646642958207808,8.09947778854293,
69.1084015576781));
#168797=CARTESIAN_POINT('Ctrl Pts',(-0.851853233428813,8.08309429038565,
69.1164671516529));
#168798=CARTESIAN_POINT('Ctrl Pts',(-1.05626889843344,8.05892132320359,
69.1245327456277));
#168799=CARTESIAN_POINT('Ctrl Pts',(-1.25928359552268,8.02707246688028,
69.1325983396025));
#168800=CARTESIAN_POINT('Ctrl Pts',(-1.46261707206923,7.99517360057602,
69.1406765984025));
#168801=CARTESIAN_POINT('Ctrl Pts',(-1.66454487389827,7.95557481397755,
69.1487548572026));
#168802=CARTESIAN_POINT('Ctrl Pts',(-1.86447247307778,7.90844042524411,
69.1568331160026));
#168803=CARTESIAN_POINT('Ctrl Pts',(-1.97735535239345,7.88182746366776,
69.1613942527189));
#168804=CARTESIAN_POINT('Ctrl Pts',(-2.08960086992019,7.8528130957757,69.1659553894351));
#168805=CARTESIAN_POINT('Ctrl Pts',(-2.20110462444749,7.82143375569568,
69.1705165261514));
#168806=CARTESIAN_POINT('Ctrl Pts',(-2.398783627965,7.76580301299692,69.1786027198836));
#168807=CARTESIAN_POINT('Ctrl Pts',(-2.59451489447767,7.70262817661812,
69.1866889136157));
#168808=CARTESIAN_POINT('Ctrl Pts',(-2.78770264090589,7.63206404247149,
69.1947751073479));
#168809=CARTESIAN_POINT('Ctrl Pts',(-2.98071807303147,7.56156284818411,
69.202854088579));
#168810=CARTESIAN_POINT('Ctrl Pts',(-3.17119421250627,7.48368560593843,
69.2109330698101));
#168811=CARTESIAN_POINT('Ctrl Pts',(-3.35854991814908,7.39863703730632,
69.2190120510412));
#168812=CARTESIAN_POINT('Ctrl Pts',(-3.54576409581162,7.313652714127,69.2270849294323));
#168813=CARTESIAN_POINT('Ctrl Pts',(-3.72986225259659,7.22150799738674,
69.2351578078233));
#168814=CARTESIAN_POINT('Ctrl Pts',(-3.91028215388211,7.12245611004596,
69.2432306862144));
#168815=CARTESIAN_POINT('Ctrl Pts',(-4.09059036718786,7.02346554024892,
69.2512985671331));
#168816=CARTESIAN_POINT('Ctrl Pts',(-4.2672245889835,6.91757647912846,69.2593664480517));
#168817=CARTESIAN_POINT('Ctrl Pts',(-4.43964561493808,6.80508885880714,
69.2674343289704));
#168818=CARTESIAN_POINT('Ctrl Pts',(-4.61198338564122,6.6926555542809,69.2754983142305));
#168819=CARTESIAN_POINT('Ctrl Pts',(-4.78011175321662,6.57363021815613,
69.2835622994905));
#168820=CARTESIAN_POINT('Ctrl Pts',(-4.94351849471029,6.44835734547624,
69.2916262847506));
#168821=CARTESIAN_POINT('Ctrl Pts',(-5.10919606664058,6.32134358102184,
69.2998023335828));
#168822=CARTESIAN_POINT('Ctrl Pts',(-5.27001952312414,6.18790751886747,
69.307978382415));
#168823=CARTESIAN_POINT('Ctrl Pts',(-5.42548673598591,6.04845279721524,
69.3161544312473));
#168824=CARTESIAN_POINT('Ctrl Pts',(-5.57875041610606,5.91097465338595,
69.3242145958942));
#168825=CARTESIAN_POINT('Ctrl Pts',(-5.72680844615076,5.76764755740925,
69.3322747605412));
#168826=CARTESIAN_POINT('Ctrl Pts',(-5.86921397705197,5.61889801064922,
69.3403349251881));
#168827=CARTESIAN_POINT('Ctrl Pts',(-6.01161262763258,5.47015565072081,
69.3483947004084));
#168828=CARTESIAN_POINT('Ctrl Pts',(-6.14835910480783,5.31599159142366,
69.3564544756286));
#168829=CARTESIAN_POINT('Ctrl Pts',(-6.27904409057477,5.15686851404203,
69.3645142508489));
#168830=CARTESIAN_POINT('Ctrl Pts',(-6.40973894322415,4.99773342266593,
69.3725746345924));
#168831=CARTESIAN_POINT('Ctrl Pts',(-6.53437119109374,4.83363881160464,
69.3806350183359));
#168832=CARTESIAN_POINT('Ctrl Pts',(-6.65257203831887,4.66508015338193,
69.3886954020794));
#168833=CARTESIAN_POINT('Ctrl Pts',(-6.77374420207106,4.4922842909537,69.3969584066332));
#168834=CARTESIAN_POINT('Ctrl Pts',(-6.88815717651778,4.31479728879599,
69.4052214111869));
#168835=CARTESIAN_POINT('Ctrl Pts',(-6.99546100379646,4.13318435432816,
69.4134844157406));
#168836=CARTESIAN_POINT('Ctrl Pts',(-7.10021966181955,3.95587914744978,
69.4215514277964));
#168837=CARTESIAN_POINT('Ctrl Pts',(-7.19820245827846,3.77464180923979,
69.4296184398521));
#168838=CARTESIAN_POINT('Ctrl Pts',(-7.28913027432016,3.59002331559133,
69.4376854519079));
#168839=CARTESIAN_POINT('Ctrl Pts',(-7.3833718023676,3.39867671006777,69.4460464527106));
#168840=CARTESIAN_POINT('Ctrl Pts',(-7.47003431566797,3.20369821651608,
69.4544074535133));
#168841=CARTESIAN_POINT('Ctrl Pts',(-7.54886142882182,3.00572432051681,
69.462768454316));
#168842=CARTESIAN_POINT('Ctrl Pts',(-7.62768854197567,2.80775042451753,
69.4711294551187));
#168843=CARTESIAN_POINT('Ctrl Pts',(-7.69868015206915,2.60678148964838,
69.4794904559214));
#168844=CARTESIAN_POINT('Ctrl Pts',(-7.76163701836296,2.40347214622466,
69.4878514567241));
#168845=CARTESIAN_POINT('Ctrl Pts',(-7.81869986977612,2.21919660111488,
69.4954297015536));
#168846=CARTESIAN_POINT('Ctrl Pts',(-7.86927612804514,2.03262899477647,
69.503007946383));
#168847=CARTESIAN_POINT('Ctrl Pts',(-7.91317228702314,1.84428628970369,
69.5105861912125));
#168848=CARTESIAN_POINT('Ctrl Pts',(-7.95703578171511,1.65608373538968,
69.5181587968707));
#168849=CARTESIAN_POINT('Ctrl Pts',(-7.99422898302738,1.46610906559233,
69.5257314025289));
#168850=CARTESIAN_POINT('Ctrl Pts',(-8.02460762374933,1.27489609277155,
69.5333040081872));
#168851=CARTESIAN_POINT('Ctrl Pts',(-8.05496942774856,1.08378909571946,
69.540872416888));
#168852=CARTESIAN_POINT('Ctrl Pts',(-8.07852412904685,0.891445523010382,
69.5484408255888));
#168853=CARTESIAN_POINT('Ctrl Pts',(-8.09517816705029,0.698411058197308,
69.5560092342896));
#168854=CARTESIAN_POINT('Ctrl Pts',(-8.11182818130514,0.505423232052618,
69.5635758144024));
#168855=CARTESIAN_POINT('Ctrl Pts',(-8.12158081122413,0.311745211072521,
69.5711423945152));
#168856=CARTESIAN_POINT('Ctrl Pts',(-8.12439414114411,0.117929647854879,
69.578708974628));
#168857=CARTESIAN_POINT('Ctrl Pts',(-8.12720697199211,-0.0758515333592844,
69.5862742124638));
#168858=CARTESIAN_POINT('Ctrl Pts',(-8.12308295086828,-0.269769840524452,
69.5938394502995));
#168859=CARTESIAN_POINT('Ctrl Pts',(-8.11203226742937,-0.463271038037836,
69.6014046881353));
#168860=CARTESIAN_POINT('Ctrl Pts',(-8.10097774113757,-0.656839525202663,
69.6089725567673));
#168861=CARTESIAN_POINT('Ctrl Pts',(-8.08299175809912,-0.849990245181151,
69.6165404253993));
#168862=CARTESIAN_POINT('Ctrl Pts',(-8.05813657349613,-1.04217202293288,
69.6241082940312));
#168863=CARTESIAN_POINT('Ctrl Pts',(-8.03360213178454,-1.23187379741549,
69.6315785033577));
#168864=CARTESIAN_POINT('Ctrl Pts',(-8.0023748037713,-1.42063114910066,
69.6390487126842));
#168865=CARTESIAN_POINT('Ctrl Pts',(-7.96456353516324,-1.60792265263227,
69.6465189220106));
#168866=CARTESIAN_POINT('Ctrl Pts',(-7.91746101700683,-1.84123673519016,
69.6558247634538));
#168867=CARTESIAN_POINT('Ctrl Pts',(-7.86016659033934,-2.07216192790768,
69.665130604897));
#168868=CARTESIAN_POINT('Ctrl Pts',(-7.79295243627307,-2.29990866959661,
69.6744364463401));
#168869=CARTESIAN_POINT('Ctrl Pts',(-7.72537742297348,-2.52887813759577,
69.6837922489686));
#168870=CARTESIAN_POINT('Ctrl Pts',(-7.64777594680264,-2.75463490548582,
69.6931480515972));
#168871=CARTESIAN_POINT('Ctrl Pts',(-7.56047079908319,-2.97640199884195,
69.7025038542257));
#168872=CARTESIAN_POINT('Ctrl Pts',(-7.47274183243766,-3.1992456506119,
69.7119050741787));
#168873=CARTESIAN_POINT('Ctrl Pts',(-7.3752147911953,-3.41806076796294,
69.7213062941316));
#168874=CARTESIAN_POINT('Ctrl Pts',(-7.26826294017853,-3.6320849928006,
69.7307075140846));
#168875=CARTESIAN_POINT('Ctrl Pts',(-7.16119533552177,-3.84634085535968,
69.7401189089474));
#168876=CARTESIAN_POINT('Ctrl Pts',(-7.04468254438493,-4.05579542565818,
69.7495303038101));
#168877=CARTESIAN_POINT('Ctrl Pts',(-6.91914419246585,-4.25971022563344,
69.7589416986728));
#168878=CARTESIAN_POINT('Ctrl Pts',(-6.79375309913894,-4.46338583012853,
69.7683420538115));
#168879=CARTESIAN_POINT('Ctrl Pts',(-6.65935762960811,-4.66153462439478,
69.7777424089503));
#168880=CARTESIAN_POINT('Ctrl Pts',(-6.51642049528494,-4.85344738213266,
69.787142764089));
#168881=CARTESIAN_POINT('Ctrl Pts',(-6.42496636913281,-4.97623712210801,
69.7931573051584));
#168882=CARTESIAN_POINT('Ctrl Pts',(-6.33001643253913,-5.09647454965942,
69.7991718462278));
#168883=CARTESIAN_POINT('Ctrl Pts',(-6.2317014366177,-5.21397974366577,
69.8051863872972));
#168884=CARTESIAN_POINT('Ctrl Pts',(-6.1051441417948,-5.36523987790784,
69.8129286858165));
#168885=CARTESIAN_POINT('Ctrl Pts',(-5.97294893326488,-5.51204162850269,
69.8206709843357));
#168886=CARTESIAN_POINT('Ctrl Pts',(-5.83546962283214,-5.65393507598941,
69.828413282855));
#168887=CARTESIAN_POINT('Ctrl Pts',(-5.69807594956039,-5.79574013670746,
69.8361507586234));
#168888=CARTESIAN_POINT('Ctrl Pts',(-5.55540497295844,-5.93264272934101,
69.8438882343919));
#168889=CARTESIAN_POINT('Ctrl Pts',(-5.40785040869798,-6.06422637437333,
69.8516257101603));
#168890=CARTESIAN_POINT('Ctrl Pts',(-5.26036153288048,-6.19575144090756,
69.8593597413539));
#168891=CARTESIAN_POINT('Ctrl Pts',(-5.10799366244056,-6.32196204114079,
69.8670937725474));
#168892=CARTESIAN_POINT('Ctrl Pts',(-4.95117705388402,-6.44247881980161,
69.874827803741));
#168893=CARTESIAN_POINT('Ctrl Pts',(-4.79438051291575,-6.56298017610943,
69.8825608452221));
#168894=CARTESIAN_POINT('Ctrl Pts',(-4.63313664303813,-6.67778894092404,
69.8902938867033));
#168895=CARTESIAN_POINT('Ctrl Pts',(-4.4679087276712,-6.78656608040469,
69.8980269281844));
#168896=CARTESIAN_POINT('Ctrl Pts',(-4.30269731844904,-6.89533235313072,
69.9057591971405));
#168897=CARTESIAN_POINT('Ctrl Pts',(-4.13350295367036,-6.99806800943472,
69.9134914660965));
#168898=CARTESIAN_POINT('Ctrl Pts',(-3.96081772784706,-7.09447746414578,
69.9212237350526));
#168899=CARTESIAN_POINT('Ctrl Pts',(-3.7880660778721,-7.19092400318882,
69.9289589782609));
#168900=CARTESIAN_POINT('Ctrl Pts',(-3.61182119289309,-7.28103930645225,
69.9366942214691));
#168901=CARTESIAN_POINT('Ctrl Pts',(-3.4326001621191,-7.36457355788642,
69.9444294646774));
#168902=CARTESIAN_POINT('Ctrl Pts',(-3.28258295175857,-7.43449601796597,
69.9509042606461));
#168903=CARTESIAN_POINT('Ctrl Pts',(-3.13048101536807,-7.49980820338466,
69.9573790566147));
#168904=CARTESIAN_POINT('Ctrl Pts',(-2.97660830846107,-7.56038957597428,
69.9638538525834));
#168905=CARTESIAN_POINT('Ctrl Pts',(-2.7766488925416,-7.63911579144238,
69.9722679270878));
#168906=CARTESIAN_POINT('Ctrl Pts',(-2.57360250103078,-7.7098901782334,
69.9806820015921));
#168907=CARTESIAN_POINT('Ctrl Pts',(-2.36810602907813,-7.77250033113822,
69.9890960760964));
#168908=CARTESIAN_POINT('Ctrl Pts',(-2.16255216761608,-7.83512796933574,
69.9975125004202));
#168909=CARTESIAN_POINT('Ctrl Pts',(-1.95454711231985,-7.88958674496606,
70.005928924744));
#168910=CARTESIAN_POINT('Ctrl Pts',(-1.74474219750444,-7.93571434886283,
70.0143453490678));
#168911=CARTESIAN_POINT('Ctrl Pts',(-1.53488525253141,-7.98185339208409,
70.0227638606061));
#168912=CARTESIAN_POINT('Ctrl Pts',(-1.32322781472788,-8.01965708218385,
70.0311823721446));
#168913=CARTESIAN_POINT('Ctrl Pts',(-1.11043174996157,-8.04901415647763,
70.039600883683));
#168914=CARTESIAN_POINT('Ctrl Pts',(-0.897553951114326,-8.0783825067012,
70.0480226287365));
#168915=CARTESIAN_POINT('Ctrl Pts',(-0.683536912744339,-8.09929772052912,
70.0564443737901));
#168916=CARTESIAN_POINT('Ctrl Pts',(-0.469049400935833,-8.11170020538122,
70.0648661188436));
#168917=CARTESIAN_POINT('Ctrl Pts',(-0.254538639266971,-8.12410403462879,
70.0732887767913));
#168918=CARTESIAN_POINT('Ctrl Pts',(-0.0395575660154435,-8.12799328029952,
70.0817114347391));
#168919=CARTESIAN_POINT('Ctrl Pts',(0.175222646691773,-8.1233604245156,
70.0901340926868));
#168920=CARTESIAN_POINT('Ctrl Pts',(0.390043704415167,-8.11872668769582,
70.0985583523817));
#168921=CARTESIAN_POINT('Ctrl Pts',(0.60466356141743,-8.10556761748978,
70.1069826120766));
#168922=CARTESIAN_POINT('Ctrl Pts',(0.818412432624915,-8.08392779857817,
70.1154068717715));
#168923=CARTESIAN_POINT('Ctrl Pts',(0.878584082831494,-8.07783605359385,
70.1177783538043));
#168924=CARTESIAN_POINT('Ctrl Pts',(0.938686735209647,-8.07107256111987,
70.1201498358372));
#168925=CARTESIAN_POINT('Ctrl Pts',(0.998705517655859,-8.0636390576156,
70.1225213178701));
#168926=CARTESIAN_POINT('Ctrl Pts',(1.21191301222614,-8.03723267958807,
70.1309456430902));
#168927=CARTESIAN_POINT('Ctrl Pts',(1.42408360115664,-8.00236463516795,
70.1393699683103));
#168928=CARTESIAN_POINT('Ctrl Pts',(1.63455445124467,-7.95914061368539,
70.1477942935305));
#168929=CARTESIAN_POINT('Ctrl Pts',(1.84498892939666,-7.91592406184219,
70.1562171629242));
#168930=CARTESIAN_POINT('Ctrl Pts',(2.05372399698473,-7.86435447014295,
70.1646400323179));
#168931=CARTESIAN_POINT('Ctrl Pts',(2.26010706148907,-7.80458862676997,
70.1730629017116));
#168932=CARTESIAN_POINT('Ctrl Pts',(2.46644795126601,-7.74483499664792,
70.1814840498778));
#168933=CARTESIAN_POINT('Ctrl Pts',(2.67043754439279,-7.67688853292304,
70.189905198044));
#168934=CARTESIAN_POINT('Ctrl Pts',(2.87143739663591,-7.60095617930407,
70.1983263462101));
#168935=CARTESIAN_POINT('Ctrl Pts',(3.07238085510465,-7.52504512974066,
70.2067451316864));
#168936=CARTESIAN_POINT('Ctrl Pts',(3.27033600131845,-7.44115275850611,
70.2151639171626));
#168937=CARTESIAN_POINT('Ctrl Pts',(3.46468244641396,-7.34953489059076,
70.2235827026388));
#168938=CARTESIAN_POINT('Ctrl Pts',(3.65897460213065,-7.25794261551369,
70.2319991363836));
#168939=CARTESIAN_POINT('Ctrl Pts',(3.84965983089612,-7.15862926501837,
70.2404155701284));
#168940=CARTESIAN_POINT('Ctrl Pts',(4.03613945280823,-7.05189803386187,
70.2488320038733));
#168941=CARTESIAN_POINT('Ctrl Pts',(4.22255139345792,-6.94520553993782,
70.2572453829419));
#168942=CARTESIAN_POINT('Ctrl Pts',(4.4047605465545,-6.83110067273071,70.2656587620106));
#168943=CARTESIAN_POINT('Ctrl Pts',(4.58219361943055,-6.70993213054722,
70.2740721410792));
#168944=CARTESIAN_POINT('Ctrl Pts',(4.63222217759542,-6.67576777008093,
70.2764443551049));
#168945=CARTESIAN_POINT('Ctrl Pts',(4.6818712003028,-6.64104212099621,70.2788165691306));
#168946=CARTESIAN_POINT('Ctrl Pts',(4.73112823130388,-6.60576363651164,
70.2811887831563));
#168947=CARTESIAN_POINT('Ctrl Pts',(4.89174284651827,-6.49072949629494,
70.2889239680669));
#168948=CARTESIAN_POINT('Ctrl Pts',(5.0482586039032,-6.36976297473629,70.2966591529776));
#168949=CARTESIAN_POINT('Ctrl Pts',(5.20020892040662,-6.24319747778519,
70.3043943378882));
#168950=CARTESIAN_POINT('Ctrl Pts',(5.35211225011853,-6.11667111801232,
70.3121271308886));
#168951=CARTESIAN_POINT('Ctrl Pts',(5.49945267918814,-5.98454945651013,
70.319859923889));
#168952=CARTESIAN_POINT('Ctrl Pts',(5.64179551706581,-5.84720710306349,
70.3275927168894));
#168953=CARTESIAN_POINT('Ctrl Pts',(5.78411962922179,-5.70988281750649,
70.3353244926126));
#168954=CARTESIAN_POINT('Ctrl Pts',(5.92144720608923,-5.56733945381257,
70.3430562683357));
#168955=CARTESIAN_POINT('Ctrl Pts',(6.05337925185845,-5.41998959368647,
70.3507880440589));
#168956=CARTESIAN_POINT('Ctrl Pts',(6.18535850651505,-5.27258700775814,
70.3585225864225));
#168957=CARTESIAN_POINT('Ctrl Pts',(6.31193813369625,-5.12037474985404,
70.366257128786));
#168958=CARTESIAN_POINT('Ctrl Pts',(6.43275796798117,-4.96380020628095,
70.3739916711496));
#168959=CARTESIAN_POINT('Ctrl Pts',(6.55359820738985,-4.80719921901209,
70.3817275197912));
#168960=CARTESIAN_POINT('Ctrl Pts',(6.6686765057568,-4.64623476253393,70.3894633684328));
#168961=CARTESIAN_POINT('Ctrl Pts',(6.77767505817898,-4.48138464854765,
70.3971992170744));
#168962=CARTESIAN_POINT('Ctrl Pts',(6.88676279815156,-4.31639964673467,
70.4049413955375));
#168963=CARTESIAN_POINT('Ctrl Pts',(6.98976066427123,-4.14752293417595,
70.4126835740007));
#168964=CARTESIAN_POINT('Ctrl Pts',(7.08639551780897,-3.97525925288867,
70.4204257524639));
#168965=CARTESIAN_POINT('Ctrl Pts',(7.16723680996016,-3.83114956496384,
70.4269025844569));
#168966=CARTESIAN_POINT('Ctrl Pts',(7.24362577073828,-3.68467008855548,
70.4333794164498));
#168967=CARTESIAN_POINT('Ctrl Pts',(7.31542809573629,-3.53612773222521,
70.4398562484428));
#168968=CARTESIAN_POINT('Ctrl Pts',(7.420184286902,-3.31941147023267,70.4493056395373));
#168969=CARTESIAN_POINT('Ctrl Pts',(7.51523505090712,-3.09818594224481,
70.4587550306319));
#168970=CARTESIAN_POINT('Ctrl Pts',(7.60027053186312,-2.87325171277997,
70.4682044217264));
#168971=CARTESIAN_POINT('Ctrl Pts',(7.68658112354406,-2.64494458478887,
70.4777955068503));
#168972=CARTESIAN_POINT('Ctrl Pts',(7.76257371473142,-2.41281668831467,
70.4873865919741));
#168973=CARTESIAN_POINT('Ctrl Pts',(7.82797664972721,-2.17772108724364,
70.4969776770979));
#168974=CARTESIAN_POINT('Ctrl Pts',(7.89244276833816,-1.94599294072337,
70.5064313817557));
#168975=CARTESIAN_POINT('Ctrl Pts',(7.94662053333941,-1.71138155118103,
70.5158850864134));
#168976=CARTESIAN_POINT('Ctrl Pts',(7.99029987438044,-1.47471877996312,
70.5253387910712));
#168977=CARTESIAN_POINT('Ctrl Pts',(8.03493133236088,-1.23289726257288,
70.534998566428));
#168978=CARTESIAN_POINT('Ctrl Pts',(8.06860144480357,-0.988933912655596,
70.5446583417849));
#168979=CARTESIAN_POINT('Ctrl Pts',(8.09114023723057,-0.743731957070907,
70.5543181171418));
#168980=CARTESIAN_POINT('Ctrl Pts',(8.11367902965756,-0.498530001486218,
70.5639778924986));
#168981=CARTESIAN_POINT('Ctrl Pts',(8.12508640368432,-0.252089453203025,
70.5736376678555));
#168982=CARTESIAN_POINT('Ctrl Pts',(8.1252482522699,-0.00532930436001966,
70.5832974432123));
#168983=CARTESIAN_POINT('',(8.12479782686935,0.00219746833035057,72.5832974432123));
#168984=CARTESIAN_POINT('Ctrl Pts',(8.12525,-1.9191019467627E-12,70.5832974432123));
#168985=CARTESIAN_POINT('Ctrl Pts',(8.12525000000053,2.24624642433222,70.6712950363535));
#168986=CARTESIAN_POINT('Ctrl Pts',(7.14398562317703,4.47535249753288,70.7592926294947));
#168987=CARTESIAN_POINT('Ctrl Pts',(3.83078204045102,7.50935546634275,70.9352878157771));
#168988=CARTESIAN_POINT('Ctrl Pts',(1.5241247769793,8.29110090552103,71.0232854089183));
#168989=CARTESIAN_POINT('Ctrl Pts',(-2.95101623932386,7.89663306204491,
71.1992805952007));
#168990=CARTESIAN_POINT('Ctrl Pts',(-5.08535169588588,6.72342983085899,
71.2872781883419));
#168991=CARTESIAN_POINT('Ctrl Pts',(-7.81671694684337,3.1566195105311,71.4632733746243));
#168992=CARTESIAN_POINT('Ctrl Pts',(-8.39290461146686,0.790229551555905,
71.5512709677655));
#168993=CARTESIAN_POINT('Ctrl Pts',(-7.6070161146256,-3.63299000730257,
71.7272661540479));
#168994=CARTESIAN_POINT('Ctrl Pts',(-6.25093680401474,-5.65606750609891,
71.8152637471891));
#168995=CARTESIAN_POINT('Ctrl Pts',(-2.45807268688716,-8.0636957548827,
71.9912589334715));
#168996=CARTESIAN_POINT('Ctrl Pts',(-0.0502299510469964,-8.42987470330086,
72.0792565266128));
#168997=CARTESIAN_POINT('Ctrl Pts',(4.2868996088086,-7.25863639434643,72.2552517128951));
#168998=CARTESIAN_POINT('Ctrl Pts',(6.18309125557056,-5.73015646266494,
72.3432493060364));
#168999=CARTESIAN_POINT('Ctrl Pts',(7.81050559202848,-2.58640713800423,
72.4819304138558));
#169000=CARTESIAN_POINT('Ctrl Pts',(8.1252499999997,-1.29375883538323,72.5326139285341));
#169001=CARTESIAN_POINT('Ctrl Pts',(8.12525,-1.86335868540631E-12,72.5832974432123));
#169002=CARTESIAN_POINT('',(8.12465437257904,-0.000424865306044762,74.5832974342377));
#169003=CARTESIAN_POINT('Ctrl Pts',(8.12479782686935,0.00219746833035057,
72.5832974432123));
#169004=CARTESIAN_POINT('Ctrl Pts',(8.12460569558819,0.666438545426072,
72.6092652162925));
#169005=CARTESIAN_POINT('Ctrl Pts',(7.88015377287088,2.68210296929945,72.6881221444681));
#169006=CARTESIAN_POINT('Ctrl Pts',(6.23719048967404,5.71096367462421,72.8198682277392));
#169007=CARTESIAN_POINT('Ctrl Pts',(1.56871213603112,8.82446412344862,73.0314248481213));
#169008=CARTESIAN_POINT('Ctrl Pts',(-4.41553899415216,7.78962694628819,
73.2429814685029));
#169009=CARTESIAN_POINT('Ctrl Pts',(-7.77043274392739,3.32666936346098,
73.4545380888851));
#169010=CARTESIAN_POINT('Ctrl Pts',(-8.68429813962366,-2.18133867002485,
73.6660947092667));
#169011=CARTESIAN_POINT('Ctrl Pts',(-5.3027347685792,-7.22585834388306,
73.8776513296489));
#169012=CARTESIAN_POINT('Ctrl Pts',(0.172450800896261,-8.455052455108,74.0892079500306));
#169013=CARTESIAN_POINT('Ctrl Pts',(4.17773714921753,-7.36911953511191,
74.2478754153172));
#169014=CARTESIAN_POINT('Ctrl Pts',(7.20239531903236,-4.46233054468999,
74.4065428806035));
#169015=CARTESIAN_POINT('Ctrl Pts',(8.0825323422617,-1.65664906305872,74.5183502202438));
#169016=CARTESIAN_POINT('Ctrl Pts',(8.12471506055508,-0.154179418476278,
74.5772684047885));
#169017=CARTESIAN_POINT('Ctrl Pts',(8.12465437257904,-0.000424865306044762,
74.5832974342377));
#169018=CARTESIAN_POINT('',(8.12525,-2.44467206894639E-12,76.5832974432123));
#169019=CARTESIAN_POINT('Ctrl Pts',(8.12524998890234,-0.000424667563621383,
74.5832974432123));
#169020=CARTESIAN_POINT('Ctrl Pts',(8.12526121818894,0.21442753365117,74.5917216186074));
#169021=CARTESIAN_POINT('Ctrl Pts',(8.11674625019481,0.42929425617801,74.6001457940026));
#169022=CARTESIAN_POINT('Ctrl Pts',(8.09972773850733,0.643504564517582,
74.6085699693977));
#169023=CARTESIAN_POINT('Ctrl Pts',(8.08271252175064,0.857673399892047,
74.6169925137997));
#169024=CARTESIAN_POINT('Ctrl Pts',(8.05719707002555,1.07118581207959,74.6254150582018));
#169025=CARTESIAN_POINT('Ctrl Pts',(8.02325601111973,1.28337466958447,74.6338376026038));
#169026=CARTESIAN_POINT('Ctrl Pts',(7.98932386718398,1.49550779349196,74.6422579347375));
#169027=CARTESIAN_POINT('Ctrl Pts',(7.94697057779809,1.70631779677591,74.6506782668711));
#169028=CARTESIAN_POINT('Ctrl Pts',(7.89632228242461,1.91514541865222,74.6590985990048));
#169029=CARTESIAN_POINT('Ctrl Pts',(7.84568798915987,2.12391530853482,74.6675166032732));
#169030=CARTESIAN_POINT('Ctrl Pts',(7.78676333104568,2.33070365518239,74.6759346075416));
#169031=CARTESIAN_POINT('Ctrl Pts',(7.71972520522185,2.53486297822238,74.68435261181));
#169032=CARTESIAN_POINT('Ctrl Pts',(7.65271138678992,2.73894827501815,74.6927675637895));
#169033=CARTESIAN_POINT('Ctrl Pts',(7.57759005811987,2.94040620159464,74.7011825157691));
#169034=CARTESIAN_POINT('Ctrl Pts',(7.49458777931377,3.13860503737896,74.7095974677486));
#169035=CARTESIAN_POINT('Ctrl Pts',(7.44763559826222,3.25072084619541,74.7143575822245));
#169036=CARTESIAN_POINT('Ctrl Pts',(7.39816251895578,3.36179408452685,74.7191176967005));
#169037=CARTESIAN_POINT('Ctrl Pts',(7.34621646707142,3.47171300389717,74.7238778111764));
#169038=CARTESIAN_POINT('Ctrl Pts',(7.26180414490245,3.65033122217884,74.7316129960871));
#169039=CARTESIAN_POINT('Ctrl Pts',(7.17082132822503,3.8259791903351,74.7393481809978));
#169040=CARTESIAN_POINT('Ctrl Pts',(7.07351247945622,3.99813816237973,74.7470833659085));
#169041=CARTESIAN_POINT('Ctrl Pts',(6.9762337209877,4.17024389861659,74.7548161589088));
#169042=CARTESIAN_POINT('Ctrl Pts',(6.87263299960399,4.3388624800516,74.7625489519092));
#169043=CARTESIAN_POINT('Ctrl Pts',(6.76300102670223,4.50349915902341,74.7702817449096));
#169044=CARTESIAN_POINT('Ctrl Pts',(6.65338347628829,4.66811417943675,74.7780135206328));
#169045=CARTESIAN_POINT('Ctrl Pts',(6.53773645116441,4.82874804722673,74.7857452963559));
#169046=CARTESIAN_POINT('Ctrl Pts',(6.41639441292734,4.98493433259204,74.793477072079));
#169047=CARTESIAN_POINT('Ctrl Pts',(6.29500895519558,5.14117650567513,74.8012116144426));
#169048=CARTESIAN_POINT('Ctrl Pts',(6.16792462657411,5.29296763483897,74.8089461568063));
#169049=CARTESIAN_POINT('Ctrl Pts',(6.03551708426173,5.43987326029612,74.8166806991699));
#169050=CARTESIAN_POINT('Ctrl Pts',(5.90308717979186,5.58680369647536,74.8244165478114));
#169051=CARTESIAN_POINT('Ctrl Pts',(5.76533251254015,5.72884672747131,74.832152396453));
#169052=CARTESIAN_POINT('Ctrl Pts',(5.62266625905238,5.86560412078874,74.8398882450946));
#169053=CARTESIAN_POINT('Ctrl Pts',(5.47988326957604,6.00247341519781,74.8476304235578));
#169054=CARTESIAN_POINT('Ctrl Pts',(5.33218092480499,6.1340481917291,74.855372602021));
#169055=CARTESIAN_POINT('Ctrl Pts',(5.18000689493983,6.25996933945173,74.8631147804842));
#169056=CARTESIAN_POINT('Ctrl Pts',(5.05270349709213,6.3653105069307,74.8695916124771));
#169057=CARTESIAN_POINT('Ctrl Pts',(4.92227130998829,6.46669568781958,74.8760684444699));
#169058=CARTESIAN_POINT('Ctrl Pts',(4.78898823029079,6.56393778860192,74.8825452764627));
#169059=CARTESIAN_POINT('Ctrl Pts',(4.59559149263344,6.70503825759569,74.8919433049343));
#169060=CARTESIAN_POINT('Ctrl Pts',(4.39608249754805,6.83749589950495,74.9013413334058));
#169061=CARTESIAN_POINT('Ctrl Pts',(4.19118362917435,6.96086685327632,74.9107393618773));
#169062=CARTESIAN_POINT('Ctrl Pts',(3.98599320686122,7.08441335358861,74.9201507629567));
#169063=CARTESIAN_POINT('Ctrl Pts',(3.77539760211755,7.19884728328956,74.9295621640361));
#169064=CARTESIAN_POINT('Ctrl Pts',(3.56014639662484,7.30376924588251,74.9389735651155));
#169065=CARTESIAN_POINT('Ctrl Pts',(3.34521928815028,7.40853323075293,74.9483707957422));
#169066=CARTESIAN_POINT('Ctrl Pts',(3.12565062332381,7.50381386007424,74.957768026369));
#169067=CARTESIAN_POINT('Ctrl Pts',(2.90221004236492,7.58925980794545,74.9671652569957));
#169068=CARTESIAN_POINT('Ctrl Pts',(2.6793330619013,7.6744902292622,74.9765387843013));
#169069=CARTESIAN_POINT('Ctrl Pts',(2.45260370146824,7.74993548690382,74.9859123116069));
#169070=CARTESIAN_POINT('Ctrl Pts',(2.22280865699228,7.81529329180295,74.9952858389125));
#169071=CARTESIAN_POINT('Ctrl Pts',(1.99450588804002,7.88022666695531,75.0045984950823));
#169072=CARTESIAN_POINT('Ctrl Pts',(1.76317715952728,7.9352031459061,75.0139111512521));
#169073=CARTESIAN_POINT('Ctrl Pts',(1.5296160366041,7.97997257783907,75.0232238074218));
#169074=CARTESIAN_POINT('Ctrl Pts',(1.37922873481097,8.00879909651198,75.0292201188643));
#169075=CARTESIAN_POINT('Ctrl Pts',(1.22791634454046,8.03339478576714,75.0352164303068));
#169076=CARTESIAN_POINT('Ctrl Pts',(1.07589550392231,8.05370327409321,75.0412127417492));
#169077=CARTESIAN_POINT('Ctrl Pts',(0.884037263361776,8.07933364702656,
75.0487803999632));
#169078=CARTESIAN_POINT('Ctrl Pts',(0.691126325427681,8.09812214564439,
75.0563480581772));
#169079=CARTESIAN_POINT('Ctrl Pts',(0.497711160093764,8.10999205693927,
75.0639157163912));
#169080=CARTESIAN_POINT('Ctrl Pts',(0.304349547942123,8.1218586816691,75.0714812792567));
#169081=CARTESIAN_POINT('Ctrl Pts',(0.110484352777653,8.12681050822314,
75.0790468421222));
#169082=CARTESIAN_POINT('Ctrl Pts',(-0.0833308035016124,8.12482267743043,
75.0866124049877));
#169083=CARTESIAN_POINT('Ctrl Pts',(-0.277128979739505,8.1228350207905,
75.0941773050383));
#169084=CARTESIAN_POINT('Ctrl Pts',(-0.470876758184223,8.11390892154314,
75.1017422050889));
#169085=CARTESIAN_POINT('Ctrl Pts',(-0.664020555561341,8.09807163862435,
75.1093071051395));
#169086=CARTESIAN_POINT('Ctrl Pts',(-0.857259146720918,8.08222658286494,
75.1168757179963));
#169087=CARTESIAN_POINT('Ctrl Pts',(-1.04989279736519,8.0594635938141,75.1244443308531));
#169088=CARTESIAN_POINT('Ctrl Pts',(-1.24137251463595,8.02986188190098,
75.13201294371));
#169089=CARTESIAN_POINT('Ctrl Pts',(-1.43289481362932,8.00025358708758,
75.1395832396932));
#169090=CARTESIAN_POINT('Ctrl Pts',(-1.62326230649332,7.96380360742398,
75.1471535356765));
#169091=CARTESIAN_POINT('Ctrl Pts',(-1.81193649217937,7.92064225368175,
75.1547238316597));
#169092=CARTESIAN_POINT('Ctrl Pts',(-2.00080185860319,7.87743716518365,
75.1623017985109));
#169093=CARTESIAN_POINT('Ctrl Pts',(-2.18797013393669,7.82750720887086,
75.1698797653621));
#169094=CARTESIAN_POINT('Ctrl Pts',(-2.37291739471902,7.77103278852559,
75.1774577322134));
#169095=CARTESIAN_POINT('Ctrl Pts',(-2.55533111156246,7.71533199642853,
75.1849318904875));
#169096=CARTESIAN_POINT('Ctrl Pts',(-2.73558397890251,7.65326507251006,
75.1924060487616));
#169097=CARTESIAN_POINT('Ctrl Pts',(-2.91319360868311,7.58505046527891,
75.1998802070357));
#169098=CARTESIAN_POINT('Ctrl Pts',(-3.1050771385112,7.51135367509069,75.2079550387546));
#169099=CARTESIAN_POINT('Ctrl Pts',(-3.29428537116136,7.43032439323175,
75.2160298704734));
#169100=CARTESIAN_POINT('Ctrl Pts',(-3.4802415242175,7.34217995527298,75.2241047021923));
#169101=CARTESIAN_POINT('Ctrl Pts',(-3.66607464898251,7.25409383353228,
75.2321741916155));
#169102=CARTESIAN_POINT('Ctrl Pts',(-3.84865969923146,7.15890207792939,
75.2402436810388));
#169103=CARTESIAN_POINT('Ctrl Pts',(-4.0274398828275,7.05687009606315,75.248313170462));
#169104=CARTESIAN_POINT('Ctrl Pts',(-4.20612614116181,6.95489171846339,
75.2563784204394));
#169105=CARTESIAN_POINT('Ctrl Pts',(-4.38101124477215,6.8460804379753,75.2644436704168));
#169106=CARTESIAN_POINT('Ctrl Pts',(-4.55156247338365,6.73074784948788,
75.2725089203942));
#169107=CARTESIAN_POINT('Ctrl Pts',(-4.72204730994814,6.61546015757904,
75.2805710307374));
#169108=CARTESIAN_POINT('Ctrl Pts',(-4.88820137433582,6.49365639807545,
75.2886331410807));
#169109=CARTESIAN_POINT('Ctrl Pts',(-5.04951991933688,6.36569211843615,
75.296695251424));
#169110=CARTESIAN_POINT('Ctrl Pts',(-5.21079760254913,6.2377602519913,75.3047553196446));
#169111=CARTESIAN_POINT('Ctrl Pts',(-5.36724196165026,6.10367117481134,
75.3128153878652));
#169112=CARTESIAN_POINT('Ctrl Pts',(-5.51837991333216,5.9638218194906,75.3208754560859));
#169113=CARTESIAN_POINT('Ctrl Pts',(-5.67178213693864,5.82187731225466,
75.3290562761493));
#169114=CARTESIAN_POINT('Ctrl Pts',(-5.81971742717136,5.6739987614407,75.3372370962128));
#169115=CARTESIAN_POINT('Ctrl Pts',(-5.96172796739798,5.52064191967245,
75.3454179162762));
#169116=CARTESIAN_POINT('Ctrl Pts',(-6.10165596409755,5.36953401166393,
75.3534787669779));
#169117=CARTESIAN_POINT('Ctrl Pts',(-6.23583158313026,5.21310763681955,
75.3615396176796));
#169118=CARTESIAN_POINT('Ctrl Pts',(-6.36385553227013,5.05183435267773,
75.3696004683814));
#169119=CARTESIAN_POINT('Ctrl Pts',(-6.49190071301743,4.89053432282871,
75.3776626559018));
#169120=CARTESIAN_POINT('Ctrl Pts',(-6.61379199197732,4.72438602863369,
75.3857248434224));
#169121=CARTESIAN_POINT('Ctrl Pts',(-6.72917134119584,4.55389290863636,
75.3937870309428));
#169122=CARTESIAN_POINT('Ctrl Pts',(-6.84458411847528,4.38335039284647,
75.4018515542651));
#169123=CARTESIAN_POINT('Ctrl Pts',(-6.95348102549767,4.20846080295797,
75.4099160775875));
#169124=CARTESIAN_POINT('Ctrl Pts',(-7.05554789537656,4.02975575668643,
75.4179806009098));
#169125=CARTESIAN_POINT('Ctrl Pts',(-7.16020957365056,3.84650755792217,
75.4262501456347));
#169126=CARTESIAN_POINT('Ctrl Pts',(-7.25768916636869,3.65924764453877,
75.4345196903596));
#169127=CARTESIAN_POINT('Ctrl Pts',(-7.34769865973584,3.46857491892795,
75.4427892350845));
#169128=CARTESIAN_POINT('Ctrl Pts',(-7.43559520996231,3.28237817260136,
75.4508646549771));
#169129=CARTESIAN_POINT('Ctrl Pts',(-7.51636834507555,3.09292735041873,
75.4589400748697));
#169130=CARTESIAN_POINT('Ctrl Pts',(-7.5897990200549,2.90079961349862,75.4670154947624));
#169131=CARTESIAN_POINT('Ctrl Pts',(-7.66587749248386,2.70174404523337,
75.4753821019034));
#169132=CARTESIAN_POINT('Ctrl Pts',(-7.73407402572994,2.49981528299274,
75.4837487090444));
#169133=CARTESIAN_POINT('Ctrl Pts',(-7.79420162147424,2.29567172006545,
75.4921153161855));
#169134=CARTESIAN_POINT('Ctrl Pts',(-7.85432921721853,2.09152815713822,
75.5004819233265));
#169135=CARTESIAN_POINT('Ctrl Pts',(-7.9063878198325,1.88517016642369,75.5088485304675));
#169136=CARTESIAN_POINT('Ctrl Pts',(-7.95024914288406,1.67726745886612,
75.5172151376086));
#169137=CARTESIAN_POINT('Ctrl Pts',(-7.99259719492189,1.47653765716584,
75.5252930862416));
#169138=CARTESIAN_POINT('Ctrl Pts',(-8.02738648986898,1.2739776759411,75.5333710348747));
#169139=CARTESIAN_POINT('Ctrl Pts',(-8.05446432528133,1.07018315968358,
75.5414489835078));
#169140=CARTESIAN_POINT('Ctrl Pts',(-8.08150902292244,0.86663804652487,
75.5495170463723));
#169141=CARTESIAN_POINT('Ctrl Pts',(-8.10086103143785,0.661861720375482,
75.5575851092368));
#169142=CARTESIAN_POINT('Ctrl Pts',(-8.11241828749152,0.456461489364734,
75.5656531721012));
#169143=CARTESIAN_POINT('Ctrl Pts',(-8.12396282265557,0.251287339151645,
75.5737123545761));
#169144=CARTESIAN_POINT('Ctrl Pts',(-8.12772969136781,0.0454909664028391,
75.5817715370509));
#169145=CARTESIAN_POINT('Ctrl Pts',(-8.1236683387382,-0.160313083316861,
75.5898307195258));
#169146=CARTESIAN_POINT('Ctrl Pts',(-8.11961220277405,-0.365852784929534,
75.5978795502625));
#169147=CARTESIAN_POINT('Ctrl Pts',(-8.10774791116926,-0.571399829657183,
75.6059283809991));
#169148=CARTESIAN_POINT('Ctrl Pts',(-8.0880768829438,-0.776337489813555,
75.6139772117358));
#169149=CARTESIAN_POINT('Ctrl Pts',(-8.06842073379543,-0.981120136047483,
75.6220199543732));
#169150=CARTESIAN_POINT('Ctrl Pts',(-8.04096964817437,-1.18529400354725,
75.6300626970107));
#169151=CARTESIAN_POINT('Ctrl Pts',(-8.0057770593636,-1.38824394047571,
75.6381054396481));
#169152=CARTESIAN_POINT('Ctrl Pts',(-7.97061313624094,-1.59102856704221,
75.6461416311689));
#169153=CARTESIAN_POINT('Ctrl Pts',(-7.92772034221117,-1.79259094153851,
75.6541778226897));
#169154=CARTESIAN_POINT('Ctrl Pts',(-7.87720377732173,-1.99232231655631,
75.6622140142105));
#169155=CARTESIAN_POINT('Ctrl Pts',(-7.84856292402568,-2.10556194444909,
75.6667702104386));
#169156=CARTESIAN_POINT('Ctrl Pts',(-7.81747240184501,-2.21821312517741,
75.6713264066668));
#169157=CARTESIAN_POINT('Ctrl Pts',(-7.78395869918434,-2.33016620263286,
75.6758826028949));
#169158=CARTESIAN_POINT('Ctrl Pts',(-7.72484505609539,-2.5276363040543,
75.6839191174036));
#169159=CARTESIAN_POINT('Ctrl Pts',(-7.65823628448052,-2.72277750295707,
75.6919556319122));
#169160=CARTESIAN_POINT('Ctrl Pts',(-7.58435204968958,-2.91501141487807,
75.6999921464209));
#169161=CARTESIAN_POINT('Ctrl Pts',(-7.51042318146776,-3.10736145521329,
75.7080335157842));
#169162=CARTESIAN_POINT('Ctrl Pts',(-7.42921019490425,-3.2968004098709,
75.7160748851474));
#169163=CARTESIAN_POINT('Ctrl Pts',(-7.34098048664703,-3.48277088783738,
75.7241162545107));
#169164=CARTESIAN_POINT('Ctrl Pts',(-7.25268669112098,-3.66887644887565,
75.7321634648703));
#169165=CARTESIAN_POINT('Ctrl Pts',(-7.15736614066776,-3.8515082217538,
75.7402106752298));
#169166=CARTESIAN_POINT('Ctrl Pts',(-7.05533193849933,-4.03013384394256,
75.7482578855894));
#169167=CARTESIAN_POINT('Ctrl Pts',(-6.95314734520363,-4.20902274754197,
75.7563169569623));
#169168=CARTESIAN_POINT('Ctrl Pts',(-6.84422947939705,-4.38389342425324,
75.7643760283352));
#169169=CARTESIAN_POINT('Ctrl Pts',(-6.72893545953539,-4.5542414454997,
75.7724350997082));
#169170=CARTESIAN_POINT('Ctrl Pts',(-6.6135481265664,-4.72472733775812,
75.780500693683));
#169171=CARTESIAN_POINT('Ctrl Pts',(-6.49177452771158,-4.89068301576979,
75.7885662876579));
#169172=CARTESIAN_POINT('Ctrl Pts',(-6.36401231705863,-5.0516368427299,
75.7966318816327));
#169173=CARTESIAN_POINT('Ctrl Pts',(-6.23604949054567,-5.21284340397075,
75.8047101404328));
#169174=CARTESIAN_POINT('Ctrl Pts',(-6.10207946156526,-5.36903217561216,
75.8127883992329));
#169175=CARTESIAN_POINT('Ctrl Pts',(-5.96253820325935,-5.51976681909415,
75.8208666580329));
#169176=CARTESIAN_POINT('Ctrl Pts',(-5.88375058671614,-5.60487443124139,
75.8254277947491));
#169177=CARTESIAN_POINT('Ctrl Pts',(-5.80318753412615,-5.68824399586726,
75.8299889314653));
#169178=CARTESIAN_POINT('Ctrl Pts',(-5.72093219888738,-5.76980262558726,
75.8345500681814));
#169179=CARTESIAN_POINT('Ctrl Pts',(-5.5751061433143,-5.91439352945372,
75.8426362619136));
#169180=CARTESIAN_POINT('Ctrl Pts',(-5.42367561358374,-6.05357177239314,
75.8507224556458));
#169181=CARTESIAN_POINT('Ctrl Pts',(-5.26706891578806,-6.18689523095706,
75.858808649378));
#169182=CARTESIAN_POINT('Ctrl Pts',(-5.11060190373566,-6.32009977132228,
75.8668876306091));
#169183=CARTESIAN_POINT('Ctrl Pts',(-4.94896816933937,-6.44745973549497,
75.8749666118402));
#169184=CARTESIAN_POINT('Ctrl Pts',(-4.78263224479084,-6.56857034472395,
75.8830455930712));
#169185=CARTESIAN_POINT('Ctrl Pts',(-4.6164219699377,-6.68958946733511,
75.8911184714623));
#169186=CARTESIAN_POINT('Ctrl Pts',(-4.44551684314378,-6.80436846275911,
75.8991913498534));
#169187=CARTESIAN_POINT('Ctrl Pts',(-4.27041428169032,-6.91254290585131,
75.9072642282445));
#169188=CARTESIAN_POINT('Ctrl Pts',(-4.09542011654648,-7.0206503841297,
75.9153321091632));
#169189=CARTESIAN_POINT('Ctrl Pts',(-3.91623396748329,-7.12216129762214,
75.9233999900818));
#169190=CARTESIAN_POINT('Ctrl Pts',(-3.73338254514489,-7.21675427973736,
75.9314678710005));
#169191=CARTESIAN_POINT('Ctrl Pts',(-3.5506194144819,-7.31130158666577,
75.9395318562605));
#169192=CARTESIAN_POINT('Ctrl Pts',(-3.36419482129698,-7.39893747930425,
75.9475958415205));
#169193=CARTESIAN_POINT('Ctrl Pts',(-3.17466095491389,-7.47938602987205,
75.9556598267805));
#169194=CARTESIAN_POINT('Ctrl Pts',(-2.98249317472273,-7.56095255767644,
75.9638358756128));
#169195=CARTESIAN_POINT('Ctrl Pts',(-2.78712934937982,-7.63513033457791,
75.972011924445));
#169196=CARTESIAN_POINT('Ctrl Pts',(-2.58916815565461,-7.70168136345851,
75.9801879732773));
#169197=CARTESIAN_POINT('Ctrl Pts',(-2.39401278808359,-7.76728912354027,
75.9882481379242));
#169198=CARTESIAN_POINT('Ctrl Pts',(-2.19633350453126,-7.82548480685165,
75.9963083025712));
#169199=CARTESIAN_POINT('Ctrl Pts',(-1.99672163313582,-7.87608978378659,
76.0043684672182));
#169200=CARTESIAN_POINT('Ctrl Pts',(-1.79711940598434,-7.92669231574297,
76.0124282424384));
#169201=CARTESIAN_POINT('Ctrl Pts',(-1.59558508428954,-7.96970479506945,
76.0204880176586));
#169202=CARTESIAN_POINT('Ctrl Pts',(-1.39272298146644,-8.00499907928759,
76.0285477928789));
#169203=CARTESIAN_POINT('Ctrl Pts',(-1.18984556229635,-8.04029602826912,
76.0366081766224));
#169204=CARTESIAN_POINT('Ctrl Pts',(-0.985640474229856,-8.06787356616393,
76.044668560366));
#169205=CARTESIAN_POINT('Ctrl Pts',(-0.780720593302095,-8.08765497024286,
76.0527289441095));
#169206=CARTESIAN_POINT('Ctrl Pts',(-0.570649464788704,-8.10793363651782,
76.0609919486633));
#169207=CARTESIAN_POINT('Ctrl Pts',(-0.359827483434094,-8.12001903408977,
76.069254953217));
#169208=CARTESIAN_POINT('Ctrl Pts',(-0.148918920099594,-8.1238851984587,
76.0775179577707));
#169209=CARTESIAN_POINT('Ctrl Pts',(0.0569870444951847,-8.12765966020212,
76.0855849698265));
#169210=CARTESIAN_POINT('Ctrl Pts',(0.262975208159651,-8.12360039996556,
76.0936519818823));
#169211=CARTESIAN_POINT('Ctrl Pts',(0.468428594148711,-8.11173607895892,
76.1017189939381));
#169212=CARTESIAN_POINT('Ctrl Pts',(0.68136938477779,-8.09943938263888,
76.1100799947408));
#169213=CARTESIAN_POINT('Ctrl Pts',(0.89373531404555,-8.07875808080631,
76.1184409955435));
#169214=CARTESIAN_POINT('Ctrl Pts',(1.10484620398487,-8.04978275657425,
76.1268019963462));
#169215=CARTESIAN_POINT('Ctrl Pts',(1.31595709392427,-8.02080743234219,
76.1351629971489));
#169216=CARTESIAN_POINT('Ctrl Pts',(1.52581257745678,-7.98353817534003,
76.1435239979516));
#169217=CARTESIAN_POINT('Ctrl Pts',(1.73374485028036,-7.93812423413909,
76.1518849987543));
#169218=CARTESIAN_POINT('Ctrl Pts',(1.92221052664872,-7.89696194110606,
76.1594632435837));
#169219=CARTESIAN_POINT('Ctrl Pts',(2.1094738818728,-7.84902588551748,76.1670414884132));
#169220=CARTESIAN_POINT('Ctrl Pts',(2.29498972691959,-7.79440246047338,
76.1746197332426));
#169221=CARTESIAN_POINT('Ctrl Pts',(2.48036752474854,-7.73981968215601,
76.1821923389008));
#169222=CARTESIAN_POINT('Ctrl Pts',(2.66400004911832,-7.67855953702154,
76.1897649445591));
#169223=CARTESIAN_POINT('Ctrl Pts',(2.84535171518964,-7.61075956651945,
76.1973375502173));
#169224=CARTESIAN_POINT('Ctrl Pts',(3.02660287091369,-7.54299717272524,
76.2049059589181));
#169225=CARTESIAN_POINT('Ctrl Pts',(3.20557534069263,-7.46870229418943,
76.2124743676188));
#169226=CARTESIAN_POINT('Ctrl Pts',(3.38174819945708,-7.38806244410324,
76.2200427763196));
#169227=CARTESIAN_POINT('Ctrl Pts',(3.55787849345241,-7.30744207724861,
76.2276093564324));
#169228=CARTESIAN_POINT('Ctrl Pts',(3.73121018565105,-7.22047993559738,
76.2351759365452));
#169229=CARTESIAN_POINT('Ctrl Pts',(3.90124173860089,-7.12741190471677,
76.2427425166581));
#169230=CARTESIAN_POINT('Ctrl Pts',(4.07124312872238,-7.03436038368383,
76.2503077544938));
#169231=CARTESIAN_POINT('Ctrl Pts',(4.23794522380528,-6.93520530868187,
76.2578729923295));
#169232=CARTESIAN_POINT('Ctrl Pts',(4.40087078746796,-6.83022868391031,
76.2654382301652));
#169233=CARTESIAN_POINT('Ctrl Pts',(4.56385300816716,-6.72521555372897,
76.2730060987972));
#169234=CARTESIAN_POINT('Ctrl Pts',(4.72305576251727,-6.61437702603606,
76.2805739674291));
#169235=CARTESIAN_POINT('Ctrl Pts',(4.87803013611122,-6.49803890059845,
76.2881418360611));
#169236=CARTESIAN_POINT('Ctrl Pts',(5.0310046481298,-6.38320205657543,76.2956120453876));
#169237=CARTESIAN_POINT('Ctrl Pts',(5.17985900604571,-6.26300694868819,
76.3030822547141));
#169238=CARTESIAN_POINT('Ctrl Pts',(5.32419319157848,-6.13780534240451,
76.3105524640406));
#169239=CARTESIAN_POINT('Ctrl Pts',(5.50399418331556,-5.9818383211906,76.3198583054837));
#169240=CARTESIAN_POINT('Ctrl Pts',(5.67669375945295,-5.8181802863734,76.3291641469269));
#169241=CARTESIAN_POINT('Ctrl Pts',(5.84173903370327,-5.64745718218452,
76.33846998837));
#169242=CARTESIAN_POINT('Ctrl Pts',(6.00767040273525,-5.47581750009047,
76.3478257909985));
#169243=CARTESIAN_POINT('Ctrl Pts',(6.16586506739252,-5.29703675329165,
76.357181593627));
#169244=CARTESIAN_POINT('Ctrl Pts',(6.31580603520619,-5.11177872057791,
76.3665373962555));
#169245=CARTESIAN_POINT('Ctrl Pts',(6.46647488472674,-4.92562136104888,
76.3759386162085));
#169246=CARTESIAN_POINT('Ctrl Pts',(6.60880970056182,-4.73292372339899,
76.3853398361614));
#169247=CARTESIAN_POINT('Ctrl Pts',(6.74233108267822,-4.53438630181099,
76.3947410561144));
#169248=CARTESIAN_POINT('Ctrl Pts',(6.8759969745523,-4.3356340038172,76.4041524509772));
#169249=CARTESIAN_POINT('Ctrl Pts',(7.00083034152809,-4.13102931665845,
76.4135638458399));
#169250=CARTESIAN_POINT('Ctrl Pts',(7.11639540987006,-3.9213013060565,76.4229752407027));
#169251=CARTESIAN_POINT('Ctrl Pts',(7.23182491844797,-3.71181930992968,
76.4323755958414));
#169252=CARTESIAN_POINT('Ctrl Pts',(7.3380078455462,-3.49722603675443,76.44177595098));
#169253=CARTESIAN_POINT('Ctrl Pts',(7.43455510377921,-3.27827362667769,
76.4511763061187));
#169254=CARTESIAN_POINT('Ctrl Pts',(7.49632803057009,-3.13818335952877,
76.4571908471882));
#169255=CARTESIAN_POINT('Ctrl Pts',(7.55415730715697,-2.99630910459338,
76.4632053882577));
#169256=CARTESIAN_POINT('Ctrl Pts',(7.60795081508343,-2.85285330113054,
76.4692199293272));
#169257=CARTESIAN_POINT('Ctrl Pts',(7.67698634659788,-2.66875027415507,
76.4769386495883));
#169258=CARTESIAN_POINT('Ctrl Pts',(7.73940628958672,-2.48195035722015,
76.4846573698495));
#169259=CARTESIAN_POINT('Ctrl Pts',(7.79499388679409,-2.2929801279869,76.4923760901106));
#169260=CARTESIAN_POINT('Ctrl Pts',(7.85054225373071,-2.10414326219491,
76.5000893629787));
#169261=CARTESIAN_POINT('Ctrl Pts',(7.89926778015739,-1.91313947503296,
76.5078026358469));
#169262=CARTESIAN_POINT('Ctrl Pts',(7.94100250815688,-1.72051350705134,
76.5155159087151));
#169263=CARTESIAN_POINT('Ctrl Pts',(7.98271957203336,-1.5279690675463,76.5232259169591));
#169264=CARTESIAN_POINT('Ctrl Pts',(8.01745165377216,-1.33380416112158,
76.5309359252031));
#169265=CARTESIAN_POINT('Ctrl Pts',(8.04508109285943,-1.13857708207028,
76.5386459334471));
#169266=CARTESIAN_POINT('Ctrl Pts',(8.07270748774194,-0.943371513090242,
76.5463550922043));
#169267=CARTESIAN_POINT('Ctrl Pts',(8.09323274058048,-0.747104355328392,
76.5540642509615));
#169268=CARTESIAN_POINT('Ctrl Pts',(8.1065905525326,-0.550342780537027,
76.5617734097188));
#169269=CARTESIAN_POINT('Ctrl Pts',(8.11902225880618,-0.367222812049529,
76.56894808755));
#169270=CARTESIAN_POINT('Ctrl Pts',(8.12524640000166,-0.183674920503634,
76.5761227653811));
#169271=CARTESIAN_POINT('Ctrl Pts',(8.12524999843797,-0.000159322667913658,
76.5832974432123));
#169272=CARTESIAN_POINT('',(8.12525,-2.38892889845022E-12,78.5832974432123));
#169273=CARTESIAN_POINT('Ctrl Pts',(8.12525,-2.44467264634169E-12,76.5832974432123));
#169274=CARTESIAN_POINT('Ctrl Pts',(8.12525000000068,2.24624642433177,76.6712950363535));
#169275=CARTESIAN_POINT('Ctrl Pts',(7.14398562317725,4.47535249753257,76.7592926294947));
#169276=CARTESIAN_POINT('Ctrl Pts',(3.83078204045118,7.50935546634272,76.9352878157771));
#169277=CARTESIAN_POINT('Ctrl Pts',(1.52412477697928,8.29110090552108,77.0232854089183));
#169278=CARTESIAN_POINT('Ctrl Pts',(-2.9510162393241,7.89663306204484,77.1992805952007));
#169279=CARTESIAN_POINT('Ctrl Pts',(-5.08535169588616,6.7234298308588,77.2872781883419));
#169280=CARTESIAN_POINT('Ctrl Pts',(-7.81671694684357,3.15661951053066,
77.4632733746244));
#169281=CARTESIAN_POINT('Ctrl Pts',(-8.39290461146693,0.790229551555331,
77.5512709677655));
#169282=CARTESIAN_POINT('Ctrl Pts',(-7.6070161146253,-3.63299000730324,
77.727266154048));
#169283=CARTESIAN_POINT('Ctrl Pts',(-6.2509368040142,-5.65606750609953,
77.8152637471892));
#169284=CARTESIAN_POINT('Ctrl Pts',(-2.45807268688625,-8.063695754883,77.9912589334716));
#169285=CARTESIAN_POINT('Ctrl Pts',(-0.0502299510459386,-8.42987470330088,
78.0792565266128));
#169286=CARTESIAN_POINT('Ctrl Pts',(4.28689960880965,-7.25863639434584,
78.2552517128952));
#169287=CARTESIAN_POINT('Ctrl Pts',(6.18309125557145,-5.730156462664,78.3432493060364));
#169288=CARTESIAN_POINT('Ctrl Pts',(7.81050559202861,-2.58640713800351,
78.4819304138558));
#169289=CARTESIAN_POINT('Ctrl Pts',(8.12524999999962,-1.29375883538314,
78.5326139285341));
#169290=CARTESIAN_POINT('Ctrl Pts',(8.12525,-2.3889293849853E-12,78.5832974432123));
#169291=CARTESIAN_POINT('',(8.11704416097363,-0.0053549714695382,82.5832974432122));
#169292=CARTESIAN_POINT('Ctrl Pts',(8.1252484868335,0.00495880126088338,
78.5812557146917));
#169293=CARTESIAN_POINT('Ctrl Pts',(8.12477749880775,0.776696675441153,
78.6119376937694));
#169294=CARTESIAN_POINT('Ctrl Pts',(8.01436124269951,1.54444684412075,78.6436553120502));
#169295=CARTESIAN_POINT('Ctrl Pts',(7.77796842233457,2.35109110530625,78.6773309709204));
#169296=CARTESIAN_POINT('Ctrl Pts',(7.7577793397255,2.41687442786724,78.6800779117451));
#169297=CARTESIAN_POINT('Ctrl Pts',(7.72612508359144,2.51552972253561,78.6841958640216));
#169298=CARTESIAN_POINT('Ctrl Pts',(7.71528036328135,2.54859716833381,78.6855758448654));
#169299=CARTESIAN_POINT('Ctrl Pts',(7.6972722113551,2.60233870357997,78.6878177626792));
#169300=CARTESIAN_POINT('Ctrl Pts',(7.69023714527696,2.62305525640478,78.6886817836851));
#169301=CARTESIAN_POINT('Ctrl Pts',(7.67756133222762,2.65989309058917,78.6902177006716));
#169302=CARTESIAN_POINT('Ctrl Pts',(7.67195326884685,2.67602546847662,78.6908901601028));
#169303=CARTESIAN_POINT('Ctrl Pts',(7.66015077416166,2.7096349371009,78.6922907467429));
#169304=CARTESIAN_POINT('Ctrl Pts',(7.65394730689467,2.7271087256561,78.6930187182664));
#169305=CARTESIAN_POINT('Ctrl Pts',(7.63974981109642,2.7666698634588,78.6946666265749));
#169306=CARTESIAN_POINT('Ctrl Pts',(7.63171970137749,2.7887441106567,78.6955859538465));
#169307=CARTESIAN_POINT('Ctrl Pts',(7.61048348997913,2.84634238020573,78.6979848156215));
#169308=CARTESIAN_POINT('Ctrl Pts',(7.59712433962746,2.88180944636591,78.6994620189326));
#169309=CARTESIAN_POINT('Ctrl Pts',(7.51537771402441,3.09431829686392,78.7083181421541));
#169310=CARTESIAN_POINT('Ctrl Pts',(7.44105181310255,3.26901471641379,78.7156217416426));
#169311=CARTESIAN_POINT('Ctrl Pts',(7.27838352742002,3.61698513847938,78.7303906863481));
#169312=CARTESIAN_POINT('Ctrl Pts',(7.18980251307043,3.79001157867117,78.7378511297545));
#169313=CARTESIAN_POINT('Ctrl Pts',(7.03787832489437,4.06223401694974,78.7498852960312));
#169314=CARTESIAN_POINT('Ctrl Pts',(6.97843688778892,4.1635195253785,78.7544311753763));
#169315=CARTESIAN_POINT('Ctrl Pts',(6.89173159576991,4.30418511863206,78.7608555763941));
#169316=CARTESIAN_POINT('Ctrl Pts',(6.86628288265661,4.3446672226043,78.7627176708181));
#169317=CARTESIAN_POINT('Ctrl Pts',(6.82236196422982,4.4131838524819,78.765892734708));
#169318=CARTESIAN_POINT('Ctrl Pts',(6.80407060200713,4.44133287663768,78.7672039853806));
#169319=CARTESIAN_POINT('Ctrl Pts',(6.76533655143993,4.50014074379178,78.769958055071));
#169320=CARTESIAN_POINT('Ctrl Pts',(6.74485868853405,4.53077549966468,78.7714011837903));
#169321=CARTESIAN_POINT('Ctrl Pts',(6.69233422672486,4.60820647632772,78.7750706931421));
#169322=CARTESIAN_POINT('Ctrl Pts',(6.66000479870735,4.65480830647563,78.7772997474766));
#169323=CARTESIAN_POINT('Ctrl Pts',(6.5090320874639,4.86763759191837,78.7875766809654));
#169324=CARTESIAN_POINT('Ctrl Pts',(6.38463732858639,5.02969173769954,78.795679589695));
#169325=CARTESIAN_POINT('Ctrl Pts',(6.09452636068742,5.37950332377518,78.8137935221507));
#169326=CARTESIAN_POINT('Ctrl Pts',(5.9259689934141,5.564638249596,78.8238153869677));
#169327=CARTESIAN_POINT('Ctrl Pts',(5.69795651131389,5.79294613699492,78.8366557270218));
#169328=CARTESIAN_POINT('Ctrl Pts',(5.64609230262538,5.84350709378457,78.8395315702991));
#169329=CARTESIAN_POINT('Ctrl Pts',(5.56794372104095,5.91768007663899,78.8437944767271));
#169330=CARTESIAN_POINT('Ctrl Pts',(5.54217029858227,5.94182490206339,78.8451892701938));
#169331=CARTESIAN_POINT('Ctrl Pts',(5.50006927953073,5.98075334338627,78.8474490941621));
#169332=CARTESIAN_POINT('Ctrl Pts',(5.48383758780031,5.99563991154673,78.8483159263131));
#169333=CARTESIAN_POINT('Ctrl Pts',(5.45413578313851,6.02265880203591,78.849893892359));
#169334=CARTESIAN_POINT('Ctrl Pts',(5.44068526620947,6.03481234362897,78.850605416075));
#169335=CARTESIAN_POINT('Ctrl Pts',(5.41239075878761,6.06020705092514,78.8520958134319));
#169336=CARTESIAN_POINT('Ctrl Pts',(5.39753862384278,6.07343889680216,78.8528745159899));
#169337=CARTESIAN_POINT('Ctrl Pts',(5.36325199331854,6.10375993531316,78.8546640746883));
#169338=CARTESIAN_POINT('Ctrl Pts',(5.34378412456139,6.12081110052114,78.8556742421444));
#169339=CARTESIAN_POINT('Ctrl Pts',(5.29090489456037,6.16668142427111,78.8584026345208));
#169340=CARTESIAN_POINT('Ctrl Pts',(5.25733963487427,6.19532197572334,78.8601179516351));
#169341=CARTESIAN_POINT('Ctrl Pts',(5.01930906386066,6.39510109020361,78.8721734109165));
#169342=CARTESIAN_POINT('Ctrl Pts',(4.80675958453488,6.55635925223577,78.8823823729737));
#169343=CARTESIAN_POINT('Ctrl Pts',(4.37927593135916,6.84870466585796,78.9022326648068));
#169344=CARTESIAN_POINT('Ctrl Pts',(4.16542086773223,6.98083670686255,78.9118620738936));
#169345=CARTESIAN_POINT('Ctrl Pts',(3.8055670544256,7.18074349052698,78.927754498019));
#169346=CARTESIAN_POINT('Ctrl Pts',(3.6630699598506,7.25447003421125,78.9339712985295));
#169347=CARTESIAN_POINT('Ctrl Pts',(3.45631166783953,7.35379867145922,78.9429051765762));
#169348=CARTESIAN_POINT('Ctrl Pts',(3.39376055687149,7.382874404501,78.9455968238417));
#169349=CARTESIAN_POINT('Ctrl Pts',(3.28219105739829,7.43301789509689,78.9503792480907));
#169350=CARTESIAN_POINT('Ctrl Pts',(3.23332102904393,7.45440596326667,78.9524678366587));
#169351=CARTESIAN_POINT('Ctrl Pts',(3.13102052168822,7.49798271510535,78.9568273112413));
#169352=CARTESIAN_POINT('Ctrl Pts',(3.07755650463511,7.52008512164437,78.9590985679526));
#169353=CARTESIAN_POINT('Ctrl Pts',(2.89908932310429,7.59164273879105,78.966656887129));
#169354=CARTESIAN_POINT('Ctrl Pts',(2.77309561098332,7.63856654613175,78.9719554886181));
#169355=CARTESIAN_POINT('Ctrl Pts',(2.47319707476751,7.74185931113206,78.9844731127395));
#169356=CARTESIAN_POINT('Ctrl Pts',(2.29843876235628,7.79552876851279,78.9916946558399));
#169357=CARTESIAN_POINT('Ctrl Pts',(2.12076571874434,7.84359879238489,78.9989427769223));
#169358=CARTESIAN_POINT('Ctrl Pts',(2.11951179332774,7.84393772334074,78.9989939257237));
#169359=CARTESIAN_POINT('Ctrl Pts',(2.11704256139804,7.84460451139439,78.9990946386954));
#169360=CARTESIAN_POINT('Ctrl Pts',(2.11582725988835,7.84493238678788,78.9991442029502));
#169361=CARTESIAN_POINT('Ctrl Pts',(2.11343223482167,7.84557794199921,78.9992418716805));
#169362=CARTESIAN_POINT('Ctrl Pts',(2.11225251570302,7.84589563817123,78.9992899762333));
#169363=CARTESIAN_POINT('Ctrl Pts',(2.10992588347078,7.84652163313258,78.9993848393332));
#169364=CARTESIAN_POINT('Ctrl Pts',(2.10877897433242,7.84682994656895,78.9994315979499));
#169365=CARTESIAN_POINT('Ctrl Pts',(2.10651542697061,7.84743790387041,78.9995238731988));
#169366=CARTESIAN_POINT('Ctrl Pts',(2.10539879229764,7.84773756088715,78.9995693898945));
#169367=CARTESIAN_POINT('Ctrl Pts',(2.10319346793509,7.84832887111911,78.9996592767118));
#169368=CARTESIAN_POINT('Ctrl Pts',(2.10210478145191,7.84862053615817,78.9997036468904));
#169369=CARTESIAN_POINT('Ctrl Pts',(2.0999532127669,7.84919647334802,78.9997913284593));
#169370=CARTESIAN_POINT('Ctrl Pts',(2.09889033343613,7.84948075615436,78.9998346399021));
#169371=CARTESIAN_POINT('Ctrl Pts',(2.0967884027551,7.85004249117029,78.9999202850193));
#169372=CARTESIAN_POINT('Ctrl Pts',(2.09574935399928,7.85031995299039,78.9999626187411));
#169373=CARTESIAN_POINT('Ctrl Pts',(2.09369325441383,7.85086856512302,79.0000463834175));
#169374=CARTESIAN_POINT('Ctrl Pts',(2.09267620591767,7.85113972411655,79.0000878144157));
#169375=CARTESIAN_POINT('Ctrl Pts',(2.09066240711839,7.85167621122216,79.0001698432837));
#169376=CARTESIAN_POINT('Ctrl Pts',(2.08966565893997,7.85194154717527,79.0002104411923));
#169377=CARTESIAN_POINT('Ctrl Pts',(2.08769087740094,7.85246683450753,79.0002908687322));
#169378=CARTESIAN_POINT('Ctrl Pts',(2.08671284593358,7.85272679298343,79.0003306983999));
#169379=CARTESIAN_POINT('Ctrl Pts',(2.08477401840881,7.85324174101474,79.0004096500308));
#169380=CARTESIAN_POINT('Ctrl Pts',(2.08381322408138,7.85349673698234,79.0004487720264));
#169381=CARTESIAN_POINT('Ctrl Pts',(2.08190748445999,7.85400214822219,79.0005263650583));
#169382=CARTESIAN_POINT('Ctrl Pts',(2.08096254071612,7.85425256929428,79.0005648361245));
#169383=CARTESIAN_POINT('Ctrl Pts',(2.07908719917799,7.85474919440275,79.0006411806151));
#169384=CARTESIAN_POINT('Ctrl Pts',(2.07815680278088,7.85499540367861,79.0006790540668));
#169385=CARTESIAN_POINT('Ctrl Pts',(2.07630932741173,7.85548394684647,79.0007542535774));
#169386=CARTESIAN_POINT('Ctrl Pts',(2.07539224972451,7.85572628545846,79.0007915796602));
#169387=CARTESIAN_POINT('Ctrl Pts',(2.07357025005561,7.85620740920747,79.0008657319323));
#169388=CARTESIAN_POINT('Ctrl Pts',(2.07266532921069,7.8564461985996,79.0009025581441));
#169389=CARTESIAN_POINT('Ctrl Pts',(2.07086654127337,7.85692052812117,79.0009757557131));
#169390=CARTESIAN_POINT('Ctrl Pts',(2.06997267520172,7.85715607207187,79.0010121270905));
#169391=CARTESIAN_POINT('Ctrl Pts',(2.0681949482745,7.8576241990653,79.0010844578299));
#169392=CARTESIAN_POINT('Ctrl Pts',(2.067311088327,7.85785678552906,79.0011204172102));
#169393=CARTESIAN_POINT('Ctrl Pts',(2.06555237277822,7.85831927170412,79.0011919648306));
#169394=CARTESIAN_POINT('Ctrl Pts',(2.06467751798638,7.85854917446267,79.0012275530872));
#169395=CARTESIAN_POINT('Ctrl Pts',(2.06293585429693,7.85900655468996,79.0012983975867));
#169396=CARTESIAN_POINT('Ctrl Pts',(2.06206904612585,7.85923403485437,79.0013336538439));
#169397=CARTESIAN_POINT('Ctrl Pts',(2.06034255487005,7.85968682002717,79.001403871919));
#169398=CARTESIAN_POINT('Ctrl Pts',(2.05948287241317,7.85991212740665,79.0014388337498));
#169399=CARTESIAN_POINT('Ctrl Pts',(2.05776974498611,7.86036080707388,79.0015084991753));
#169400=CARTESIAN_POINT('Ctrl Pts',(2.05691630058446,7.86058418141765,79.0015432027803));
#169401=CARTESIAN_POINT('Ctrl Pts',(2.05521479084541,7.86102922614735,79.0016123867515));
#169402=CARTESIAN_POINT('Ctrl Pts',(2.05436672596706,7.86125089830442,79.0016468671278));
#169403=CARTESIAN_POINT('Ctrl Pts',(2.05267514221329,7.86169276193416,79.0017156385893));
#169404=CARTESIAN_POINT('Ctrl Pts',(2.05183162374219,7.86191295489335,79.0017499296824));
#169405=CARTESIAN_POINT('Ctrl Pts',(2.05014832159025,7.86235207651928,79.0018183556192));
#169406=CARTESIAN_POINT('Ctrl Pts',(2.04930853823697,7.86257100640595,79.0018524904696));
#169407=CARTESIAN_POINT('Ctrl Pts',(2.04763191364724,7.86300781231244,79.0019206361921));
#169408=CARTESIAN_POINT('Ctrl Pts',(2.04679507268266,7.86322568929032,79.001954647069));
#169409=CARTESIAN_POINT('Ctrl Pts',(2.04512355562556,7.86366059469195,79.0020225764719));
#169410=CARTESIAN_POINT('Ctrl Pts',(2.04428887973238,7.86387762382452,79.0020564950015));
#169411=CARTESIAN_POINT('Ctrl Pts',(2.04262092804534,7.86431103453956,79.0021242708142));
#169412=CARTESIAN_POINT('Ctrl Pts',(2.04178765237209,7.86452741658966,79.0021581281001));
#169413=CARTESIAN_POINT('Ctrl Pts',(2.04012174596573,7.864959730605,79.0022258121232));
#169414=CARTESIAN_POINT('Ctrl Pts',(2.03928911530709,7.86517566279295,79.0022596388611));
#169415=CARTESIAN_POINT('Ctrl Pts',(2.03762375069531,7.86560727172827,79.0023272921891));
#169416=CARTESIAN_POINT('Ctrl Pts',(2.03679101674031,7.86582294846434,79.0023611187791));
#169417=CARTESIAN_POINT('Ctrl Pts',(2.03512470156712,7.86625423902115,79.0024288020229));
#169418=CARTESIAN_POINT('Ctrl Pts',(2.03429112031392,7.86646985258692,79.0024626586742));
#169419=CARTESIAN_POINT('Ctrl Pts',(2.03262236831987,7.86690120786833,79.0025304321662));
#169420=CARTESIAN_POINT('Ctrl Pts',(2.03178719746098,7.86711694909821,79.0025643490037));
#169421=CARTESIAN_POINT('Ctrl Pts',(2.03011452325683,7.86754874996369,79.0026322730093));
#169422=CARTESIAN_POINT('Ctrl Pts',(2.02927701972304,7.86776480887791,79.0026662801732));
#169423=CARTESIAN_POINT('Ctrl Pts',(2.02759893389873,7.86819743519649,79.0027344150898));
#169424=CARTESIAN_POINT('Ctrl Pts',(2.02675835136632,7.86841400163635,79.0027685428364));
#169425=CARTESIAN_POINT('Ctrl Pts',(2.02507335555464,7.86884783353704,79.002836949393));
#169426=CARTESIAN_POINT('Ctrl Pts',(2.02422894198711,7.86906509778384,79.0028712281947));
#169427=CARTESIAN_POINT('Ctrl Pts',(2.02253552396981,7.86950051688035,79.00293996765));
#169428=CARTESIAN_POINT('Ctrl Pts',(2.02168651915706,7.86971867026762,79.0029744282942));
#169429=CARTESIAN_POINT('Ctrl Pts',(2.01998314790442,7.87015606088526,79.0030435626371));
#169430=CARTESIAN_POINT('Ctrl Pts',(2.01912878102475,7.87037529639753,79.0030782363251));
#169431=CARTESIAN_POINT('Ctrl Pts',(2.01741390177339,7.870815046775,79.0031478284734));
#169432=CARTESIAN_POINT('Ctrl Pts',(2.01655338891001,7.87103555965058,79.0031827469205));
#169433=CARTESIAN_POINT('Ctrl Pts',(2.01482541820033,7.87147806313634,79.0032528609208));
#169434=CARTESIAN_POINT('Ctrl Pts',(2.01395795979479,7.87170005147822,79.0032880564589));
#169435=CARTESIAN_POINT('Ctrl Pts',(2.01221528033501,7.872145707755,79.0033587576936));
#169436=CARTESIAN_POINT('Ctrl Pts',(2.01134005863004,7.87236937313598,79.003394263374));
#169437=CARTESIAN_POINT('Ctrl Pts',(2.00958101406814,7.87281858945148,79.0034656187715));
#169438=CARTESIAN_POINT('Ctrl Pts',(2.0086971904917,7.87304413752564,79.0035014684702));
#169439=CARTESIAN_POINT('Ctrl Pts',(2.00692008014992,7.87349732991471,79.0035735467168));
#169440=CARTESIAN_POINT('Ctrl Pts',(2.00602679258486,7.87372497104864,79.0036097752439));
#169441=CARTESIAN_POINT('Ctrl Pts',(2.0042298659134,7.87418256560786,79.0036826470056));
#169442=CARTESIAN_POINT('Ctrl Pts',(2.00332622591931,7.87441251551417,79.0037192902172));
#169443=CARTESIAN_POINT('Ctrl Pts',(2.00150767683684,7.87487494968464,79.0037930283672));
#169444=CARTESIAN_POINT('Ctrl Pts',(2.00059276676679,7.87510743007155,79.0038301232804));
#169445=CARTESIAN_POINT('Ctrl Pts',(1.96430039190661,7.88432265877255,79.0053014869552));
#169446=CARTESIAN_POINT('Ctrl Pts',(1.92886275333948,7.89306710411284,79.0067341908905));
#169447=CARTESIAN_POINT('Ctrl Pts',(1.84751121702681,7.91256048203342,79.0100134391076));
#169448=CARTESIAN_POINT('Ctrl Pts',(1.80156024619041,7.92314910739212,79.0118587784646));
#169449=CARTESIAN_POINT('Ctrl Pts',(1.59925465774481,7.96791607261864,79.0199575297382));
#169450=CARTESIAN_POINT('Ctrl Pts',(1.44200162774041,7.99787056927811,79.0261863174386));
#169451=CARTESIAN_POINT('Ctrl Pts',(1.16482065801442,8.04222852501486,79.0371151002937));
#169452=CARTESIAN_POINT('Ctrl Pts',(1.04526520915649,8.05863930071604,79.0418125871291));
#169453=CARTESIAN_POINT('Ctrl Pts',(0.838291908905398,8.08236597885774,
79.049938754268));
#169454=CARTESIAN_POINT('Ctrl Pts',(0.751039242055659,8.09094018783375,
79.0533625500681));
#169455=CARTESIAN_POINT('Ctrl Pts',(0.611656793337977,8.1023630236452,79.0588351771077));
#169456=CARTESIAN_POINT('Ctrl Pts',(0.559608670390351,8.10612414879205,
79.0608794696216));
#169457=CARTESIAN_POINT('Ctrl Pts',(0.451830808887094,8.11286945625869,
79.0651155516643));
#169458=CARTESIAN_POINT('Ctrl Pts',(0.396099278714087,8.11578136892283,
79.0673076140426));
#169459=CARTESIAN_POINT('Ctrl Pts',(0.255272832616235,8.12168534714179,
79.0728525112909));
#169460=CARTESIAN_POINT('Ctrl Pts',(0.170152878208164,8.12391438848635,
79.0762094355119));
#169461=CARTESIAN_POINT('Ctrl Pts',(-0.341651512919927,8.12926965683001,
79.0964376596292));
#169462=CARTESIAN_POINT('Ctrl Pts',(-0.768001583346198,8.10011820440259,
79.1135101408076));
#169463=CARTESIAN_POINT('Ctrl Pts',(-1.34351323394947,8.01490600789059,
79.1367886361178));
#169464=CARTESIAN_POINT('Ctrl Pts',(-1.49626758080993,7.98779881819189,
79.1429855493658));
#169465=CARTESIAN_POINT('Ctrl Pts',(-1.70716256719744,7.9441119764702,79.1515424516805));
#169466=CARTESIAN_POINT('Ctrl Pts',(-1.76603467166353,7.93123198026309,
79.1539312108329));
#169467=CARTESIAN_POINT('Ctrl Pts',(-1.86535327397832,7.9083424439376,79.1579590080064));
#169468=CARTESIAN_POINT('Ctrl Pts',(-1.90587587891874,7.89867458544044,
79.1596017775113));
#169469=CARTESIAN_POINT('Ctrl Pts',(-1.94636051838001,7.88868609443464,
79.1612419353231));
#169470=CARTESIAN_POINT('Ctrl Pts',(-1.94639855748499,7.88867670902132,
79.1612434764038));
#169471=CARTESIAN_POINT('Ctrl Pts',(-1.94647462843851,7.88865793940133,
79.1612465582694));
#169472=CARTESIAN_POINT('Ctrl Pts',(-1.94651266056927,7.88864855512515,
79.1612480990656));
#169473=CARTESIAN_POINT('Ctrl Pts',(-1.94658871778806,7.88862978772703,
79.1612511803709));
#169474=CARTESIAN_POINT('Ctrl Pts',(-1.94662674272849,7.88862040464162,
79.1612527208739));
#169475=CARTESIAN_POINT('Ctrl Pts',(-1.94670278552942,7.88860163963458,
79.1612558015913));
#169476=CARTESIAN_POINT('Ctrl Pts',(-1.9467408035598,7.88859225767112,79.1612573418125));
#169477=CARTESIAN_POINT('Ctrl Pts',(-1.94681683272913,7.88857349486175,
79.1612604219738));
#169478=CARTESIAN_POINT('Ctrl Pts',(-1.9468548436396,7.88856411407233,79.1612619619046));
#169479=CARTESIAN_POINT('Ctrl Pts',(-1.94693085868991,7.88854535358156,
79.1612650414901));
#169480=CARTESIAN_POINT('Ctrl Pts',(-1.94696886266647,7.8885359739206,79.1612665811381));
#169481=CARTESIAN_POINT('Ctrl Pts',(-1.94704486358882,7.88851721575127,
79.1612696601474));
#169482=CARTESIAN_POINT('Ctrl Pts',(-1.94708286077298,7.88850783718416,
79.1612711995184));
#169483=CARTESIAN_POINT('Ctrl Pts',(-1.94715884812554,7.88848908119911,
79.1612742779741));
#169484=CARTESIAN_POINT('Ctrl Pts',(-1.94719683835505,7.8884797037662,79.1612758170614));
#169485=CARTESIAN_POINT('Ctrl Pts',(-1.94727281215009,7.88846094996304,
79.1612788949641));
#169486=CARTESIAN_POINT('Ctrl Pts',(-1.94731079538129,7.88845157367541,
79.1612804337659));
#169487=CARTESIAN_POINT('Ctrl Pts',(-1.94738675498445,7.88843282221134,
79.1612835110898));
#169488=CARTESIAN_POINT('Ctrl Pts',(-1.94742473156101,7.88842344698449,
79.1612850496202));
#169489=CARTESIAN_POINT('Ctrl Pts',(-1.94750067778661,7.88840469765911,
79.1612881263983));
#169490=CARTESIAN_POINT('Ctrl Pts',(-1.9475386475168,7.88839532354065,79.1612896646494));
#169491=CARTESIAN_POINT('Ctrl Pts',(-1.94761458031149,7.88837657636773,
79.1612927408796));
#169492=CARTESIAN_POINT('Ctrl Pts',(-1.94765254317287,7.88836720336352,
79.1612942788505));
#169493=CARTESIAN_POINT('Ctrl Pts',(-1.94772846198207,7.88834845848061,
79.1612973545104));
#169494=CARTESIAN_POINT('Ctrl Pts',(-1.9477664182879,7.88833908651362,79.1612988922138));
#169495=CARTESIAN_POINT('Ctrl Pts',(-1.94784232416707,7.88832034366071,
79.1613019673459));
#169496=CARTESIAN_POINT('Ctrl Pts',(-1.9478802735894,7.88831097281219,79.1613035047686));
#169497=CARTESIAN_POINT('Ctrl Pts',(-1.94795616570425,7.8882922321959,79.1613065793393));
#169498=CARTESIAN_POINT('Ctrl Pts',(-1.94799410854456,7.88828286239173,
79.1613081164934));
#169499=CARTESIAN_POINT('Ctrl Pts',(-1.94806998759181,7.88826412384062,
79.1613111905309));
#169500=CARTESIAN_POINT('Ctrl Pts',(-1.94810792369788,7.88825475511868,
79.1613127274103));
#169501=CARTESIAN_POINT('Ctrl Pts',(-1.94818378933276,7.88823601871847,
79.1613158009006));
#169502=CARTESIAN_POINT('Ctrl Pts',(-1.94822171884716,7.88822665104386,
79.1613173375111));
#169503=CARTESIAN_POINT('Ctrl Pts',(-1.9482975714523,7.88820791670066,79.1613204104697));
#169504=CARTESIAN_POINT('Ctrl Pts',(-1.9483354943024,7.8881985500916,79.1613219468082));
#169505=CARTESIAN_POINT('Ctrl Pts',(-1.94841133337646,7.88817981792983,
79.1613250192149));
#169506=CARTESIAN_POINT('Ctrl Pts',(-1.94844924982359,7.88817045232209,
79.1613265552921));
#169507=CARTESIAN_POINT('Ctrl Pts',(-1.94852507626911,7.8881517221194,79.1613296271834));
#169508=CARTESIAN_POINT('Ctrl Pts',(-1.94856298603782,7.8881423575813,79.1613311629881));
#169509=CARTESIAN_POINT('Ctrl Pts',(-1.94863879914926,7.88812362951256,
79.1613342343354));
#169510=CARTESIAN_POINT('Ctrl Pts',(-1.94867670250201,7.88811426597956,
79.1613357698783));
#169511=CARTESIAN_POINT('Ctrl Pts',(-1.94875250263959,7.88809553995638,
79.1613388406961));
#169512=CARTESIAN_POINT('Ctrl Pts',(-1.94879039957604,7.88808617742885,
79.1613403759772));
#169513=CARTESIAN_POINT('Ctrl Pts',(-1.9488661869626,7.88806745339675,79.1613434462746));
#169514=CARTESIAN_POINT('Ctrl Pts',(-1.94890407741564,7.88805809189157,
79.1613449812912));
#169515=CARTESIAN_POINT('Ctrl Pts',(-1.94897985188041,7.88803936989332,
79.1613480510613));
#169516=CARTESIAN_POINT('Ctrl Pts',(-1.94901773595153,7.88803000938569,
79.1613495858173));
#169517=CARTESIAN_POINT('Ctrl Pts',(-1.94909349773738,7.88801128936186,
79.16135265507));
#169518=CARTESIAN_POINT('Ctrl Pts',(-1.94913137540082,7.88800192985844,
79.1613541895646));
#169519=CARTESIAN_POINT('Ctrl Pts',(-1.94920712440952,7.88798321183387,
79.1613572582959));
#169520=CARTESIAN_POINT('Ctrl Pts',(-1.94924499575073,7.88797385331382,
79.1613587925324));
#169521=CARTESIAN_POINT('Ctrl Pts',(-1.94932073227924,7.88795513721571,
79.1613618607542));
#169522=CARTESIAN_POINT('Ctrl Pts',(-1.94935859723964,7.8879457796938,79.1613633947303));
#169523=CARTESIAN_POINT('Ctrl Pts',(-1.94943432077752,7.88792706564884,
79.1613664624221));
#169524=CARTESIAN_POINT('Ctrl Pts',(-1.94947217963067,7.88791770905775,
79.1613679961489));
#169525=CARTESIAN_POINT('Ctrl Pts',(-1.94954789125288,7.88789899680085,
79.1613710633541));
#169526=CARTESIAN_POINT('Ctrl Pts',(-1.9495857436448,7.88788964122833,79.1613725968172));
#169527=CARTESIAN_POINT('Ctrl Pts',(-1.9496614421218,7.88787093106393,79.161375663486));
#169528=CARTESIAN_POINT('Ctrl Pts',(-1.94969928853972,7.88786157638986,
79.1613771967052));
#169529=CARTESIAN_POINT('Ctrl Pts',(-1.94977497504477,7.88784286802853,
79.1613802628853));
#169530=CARTESIAN_POINT('Ctrl Pts',(-1.94981281519283,7.8878335143263,79.1613817958486));
#169531=CARTESIAN_POINT('Ctrl Pts',(-1.94988848938413,7.88781480785307,
79.1613848615259));
#169532=CARTESIAN_POINT('Ctrl Pts',(-1.94992632333294,7.88780545510551,
79.1613863942362));
#169533=CARTESIAN_POINT('Ctrl Pts',(-1.95000198501738,7.88778675056867,
79.161389459403));
#169534=CARTESIAN_POINT('Ctrl Pts',(-1.95003981294821,7.88777739873124,
79.1613909918675));
#169535=CARTESIAN_POINT('Ctrl Pts',(-1.95011546267391,7.88775869599584,
79.1613940565461));
#169536=CARTESIAN_POINT('Ctrl Pts',(-1.95015328445052,7.88774934510249,
79.1613955887594));
#169537=CARTESIAN_POINT('Ctrl Pts',(-1.95022892202693,7.88773064421619,
79.161398652942));
#169538=CARTESIAN_POINT('Ctrl Pts',(-1.95026673772477,7.88772129424854,
79.1614001849072));
#169539=CARTESIAN_POINT('Ctrl Pts',(-1.95034236313225,7.88770259521673,
79.1614032485929));
#169540=CARTESIAN_POINT('Ctrl Pts',(-1.95038017284784,7.88769324615118,
79.1614047803138));
#169541=CARTESIAN_POINT('Ctrl Pts',(-1.9504557863384,7.88767454891209,79.161407843513));
#169542=CARTESIAN_POINT('Ctrl Pts',(-1.95049359004318,7.88766520075599,
79.1614093749885));
#169543=CARTESIAN_POINT('Ctrl Pts',(-1.95056919144303,7.88764650535312,
79.161412437694));
#169544=CARTESIAN_POINT('Ctrl Pts',(-1.9506069892577,7.88763715807688,79.161413968929));
#169545=CARTESIAN_POINT('Ctrl Pts',(-1.95068257902129,7.88761846439839,
79.1614170311593));
#169546=CARTESIAN_POINT('Ctrl Pts',(-1.95072037082725,7.8876091180316,79.1614185621489));
#169547=CARTESIAN_POINT('Ctrl Pts',(-1.95079594871376,7.88759042613757,
79.1614216238943));
#169548=CARTESIAN_POINT('Ctrl Pts',(-1.95083373462223,7.88758108065299,
79.161423154643));
#169549=CARTESIAN_POINT('Ctrl Pts',(-1.95090930040535,7.88756239059993,
79.1614262158943));
#169550=CARTESIAN_POINT('Ctrl Pts',(-1.95094708063404,7.88755304594398,
79.161427746411));
#169551=CARTESIAN_POINT('Ctrl Pts',(-1.95102263538902,7.88753435746646,
79.1614308072117));
#169552=CARTESIAN_POINT('Ctrl Pts',(-1.9510604095568,7.88752501373366,79.161432337481));
#169553=CARTESIAN_POINT('Ctrl Pts',(-1.95113595207191,7.88750632713192,
79.161435397782));
#169554=CARTESIAN_POINT('Ctrl Pts',(-1.95117372064528,7.88749698420716,
79.1614369278227));
#169555=CARTESIAN_POINT('Ctrl Pts',(-1.95124925209198,7.88747829919194,
79.1614399876715));
#169556=CARTESIAN_POINT('Ctrl Pts',(-1.95128701476653,7.88746895715075,
79.1614415174714));
#169557=CARTESIAN_POINT('Ctrl Pts',(-1.95136253439556,7.88745027390792,
79.1614445768376));
#169558=CARTESIAN_POINT('Ctrl Pts',(-1.95140029144312,7.88744093268333,
79.1614461064076));
#169559=CARTESIAN_POINT('Ctrl Pts',(-1.9514757999335,7.88742225104541,79.1614491653187));
#169560=CARTESIAN_POINT('Ctrl Pts',(-1.95151355120057,7.88741291067565,
79.1614506946526));
#169561=CARTESIAN_POINT('Ctrl Pts',(-1.95158904806635,7.88739423076338,
79.161453753089));
#169562=CARTESIAN_POINT('Ctrl Pts',(-1.951626793769,7.88738489119523,79.1614552821956));
#169563=CARTESIAN_POINT('Ctrl Pts',(-1.95170227959926,7.88736621286336,
79.1614583401811));
#169564=CARTESIAN_POINT('Ctrl Pts',(-1.95174001959997,7.88735687413112,
79.1614598690548));
#169565=CARTESIAN_POINT('Ctrl Pts',(-1.95181549381266,7.88733819752417,
79.1614629265658));
#169566=CARTESIAN_POINT('Ctrl Pts',(-1.95185322838488,7.88732885956042,
79.1614644552177));
#169567=CARTESIAN_POINT('Ctrl Pts',(-1.9519286921361,7.88731018439281,79.1614675123011));
#169568=CARTESIAN_POINT('Ctrl Pts',(-1.95196642088589,7.88730084729526,
79.1614690407152));
#169569=CARTESIAN_POINT('Ctrl Pts',(-1.95204187253894,7.88728217397253,
79.1614720973047));
#169570=CARTESIAN_POINT('Ctrl Pts',(-1.95207959614115,7.88727283757445,
79.1614736255083));
#169571=CARTESIAN_POINT('Ctrl Pts',(-1.95215503791157,7.88725416554876,
79.1614766816936));
#169572=CARTESIAN_POINT('Ctrl Pts',(-1.95219275564322,7.8872448300293,79.1614782096576));
#169573=CARTESIAN_POINT('Ctrl Pts',(-1.95226818567163,7.88722615976135,
79.1614812653633));
#169574=CARTESIAN_POINT('Ctrl Pts',(-1.95230589815237,7.8872168249674,79.1614827931126));
#169575=CARTESIAN_POINT('Ctrl Pts',(-1.95238131772789,7.8871981561386,79.1614858483912));
#169576=CARTESIAN_POINT('Ctrl Pts',(-1.95241902467326,7.8871888221408,79.1614873759143));
#169577=CARTESIAN_POINT('Ctrl Pts',(-1.95249443332005,7.88717015486941,
79.1614904307462));
#169578=CARTESIAN_POINT('Ctrl Pts',(-1.95253213487561,7.88716082163199,
79.1614919580491));
#169579=CARTESIAN_POINT('Ctrl Pts',(-1.95260753258819,7.88714215591984,
79.1614950124343));
#169580=CARTESIAN_POINT('Ctrl Pts',(-1.95264522888111,7.88713282341156,
79.161496539522));
#169581=CARTESIAN_POINT('Ctrl Pts',(-1.95272061609433,7.88711415915149,
79.161499593478));
#169582=CARTESIAN_POINT('Ctrl Pts',(-1.95275830702106,7.8871048273982,79.1615011203465));
#169583=CARTESIAN_POINT('Ctrl Pts',(-1.95283368340743,7.88708616467176,
79.1615041738601));
#169584=CARTESIAN_POINT('Ctrl Pts',(-1.95287136913025,7.88707683363352,
79.1615057005158));
#169585=CARTESIAN_POINT('Ctrl Pts',(-1.9529467353201,7.88705817228512,79.1615087536125));
#169586=CARTESIAN_POINT('Ctrl Pts',(-1.95298441565574,7.88704884200755,
79.1615102800481));
#169587=CARTESIAN_POINT('Ctrl Pts',(-1.95305977119553,7.88703018214994,
79.1615133327095));
#169588=CARTESIAN_POINT('Ctrl Pts',(-1.9530974463303,7.88702085258715,79.1615148589325));
#169589=CARTESIAN_POINT('Ctrl Pts',(-1.9531727913719,7.88700219418319,79.1615179111648));
#169590=CARTESIAN_POINT('Ctrl Pts',(-1.95321046137423,7.88699286531846,
79.161519437178));
#169591=CARTESIAN_POINT('Ctrl Pts',(-1.95328579625346,7.88697420828547,
79.1615224889947));
#169592=CARTESIAN_POINT('Ctrl Pts',(-1.95332346104062,7.8869648801395,79.1615240147947));
#169593=CARTESIAN_POINT('Ctrl Pts',(-1.95339878559046,7.88694622451928,
79.1615270661892));
#169594=CARTESIAN_POINT('Ctrl Pts',(-1.95343644525625,7.88693689706909,
79.1615285917798));
#169595=CARTESIAN_POINT('Ctrl Pts',(-1.95351175959471,7.88691824283288,
79.1615316427568));
#169596=CARTESIAN_POINT('Ctrl Pts',(-1.95354941417775,7.88690891606912,
79.1615331681396));
#169597=CARTESIAN_POINT('Ctrl Pts',(-1.95362471823248,7.88689026323528,
79.1615362186962));
#169598=CARTESIAN_POINT('Ctrl Pts',(-1.95366236783991,7.88688093713165,
79.1615377438755));
#169599=CARTESIAN_POINT('Ctrl Pts',(-1.97298584429292,7.88209421330181,
79.1623205341811));
#169600=CARTESIAN_POINT('Ctrl Pts',(-1.99225412139981,7.8772460827388,79.1631008368244));
#169601=CARTESIAN_POINT('Ctrl Pts',(-2.03082277879275,7.86739117920091,
79.1646621290709));
#169602=CARTESIAN_POINT('Ctrl Pts',(-2.05012290505404,7.86238393891958,
79.1654431062218));
#169603=CARTESIAN_POINT('Ctrl Pts',(-2.09051212760801,7.85174649653286,
79.1670766859053));
#169604=CARTESIAN_POINT('Ctrl Pts',(-2.11159729117103,7.84610227347256,
79.1679290270509));
#169605=CARTESIAN_POINT('Ctrl Pts',(-2.17411248571074,7.82909751786587,
79.1704548680323));
#169606=CARTESIAN_POINT('Ctrl Pts',(-2.21547549311649,7.81749329487738,
79.1721245535412));
#169607=CARTESIAN_POINT('Ctrl Pts',(-2.43424034113709,7.75424398129068,
79.1809533096732));
#169608=CARTESIAN_POINT('Ctrl Pts',(-2.60993583625333,7.69688651878376,
79.1880382373002));
#169609=CARTESIAN_POINT('Ctrl Pts',(-2.92921653656757,7.58046347814742,
79.2010498932282));
#169610=CARTESIAN_POINT('Ctrl Pts',(-3.073357727662,7.52317807079658,79.2069767897038));
#169611=CARTESIAN_POINT('Ctrl Pts',(-3.28090948526638,7.43373066420509,
79.2156417948539));
#169612=CARTESIAN_POINT('Ctrl Pts',(-3.34567739738918,7.40480663783087,
79.2183646214665));
#169613=CARTESIAN_POINT('Ctrl Pts',(-3.53871969654899,7.31554805655254,
79.2265451623967));
#169614=CARTESIAN_POINT('Ctrl Pts',(-3.66580144257269,7.25270154389465,
79.2320182092772));
#169615=CARTESIAN_POINT('Ctrl Pts',(-3.83645074542028,7.1626778382182,79.2395104028353));
#169616=CARTESIAN_POINT('Ctrl Pts',(-3.88150139102779,7.13836501280901,
79.241502105676));
#169617=CARTESIAN_POINT('Ctrl Pts',(-3.95535999665793,7.09759925304234,
79.2447911043398));
#169618=CARTESIAN_POINT('Ctrl Pts',(-3.9843023699576,7.08139269324333,79.2460860012422));
#169619=CARTESIAN_POINT('Ctrl Pts',(-4.04249282396076,7.04833870913801,
79.2487019642452));
#169620=CARTESIAN_POINT('Ctrl Pts',(-4.07173679310006,7.03148535296479,
79.2500230654698));
#169621=CARTESIAN_POINT('Ctrl Pts',(-4.14401275725236,6.9892304833494,79.2533043747269));
#169622=CARTESIAN_POINT('Ctrl Pts',(-4.1869169736638,6.96361333704036,79.2552666138396));
#169623=CARTESIAN_POINT('Ctrl Pts',(-4.34180636793745,6.8691833905108,79.2624037430102));
#169624=CARTESIAN_POINT('Ctrl Pts',(-4.45235320409623,6.79805218144114,
79.2676000198836));
#169625=CARTESIAN_POINT('Ctrl Pts',(-4.7878828626092,6.57045982335032,79.2836896437482));
#169626=CARTESIAN_POINT('Ctrl Pts',(-5.00671457330853,6.40527690979999,
79.2946457049854));
#169627=CARTESIAN_POINT('Ctrl Pts',(-5.27338084610761,6.18195700106008,
79.3084894821777));
#169628=CARTESIAN_POINT('Ctrl Pts',(-5.32933270083204,6.13378765154651,
79.3114229166483));
#169629=CARTESIAN_POINT('Ctrl Pts',(-5.41178691203125,6.06082221503731,
79.3157844830949));
#169630=CARTESIAN_POINT('Ctrl Pts',(-5.4387920973462,6.03660037102309,79.3172192988634));
#169631=CARTESIAN_POINT('Ctrl Pts',(-5.48444755217761,5.99509541740975,
79.3196551331035));
#169632=CARTESIAN_POINT('Ctrl Pts',(-5.50318053019628,5.97790415398929,
79.3206575215902));
#169633=CARTESIAN_POINT('Ctrl Pts',(-5.53492659049098,5.94849508650658,
79.3223609876884));
#169634=CARTESIAN_POINT('Ctrl Pts',(-5.54798065055964,5.93632182917712,
79.3230628403995));
#169635=CARTESIAN_POINT('Ctrl Pts',(-5.57310411556495,5.91273827755227,
79.3244161766623));
#169636=CARTESIAN_POINT('Ctrl Pts',(-5.58517885566913,5.90133379617661,
79.3250677683967));
#169637=CARTESIAN_POINT('Ctrl Pts',(-5.61384275266395,5.87409423273916,
79.3266172157638));
#169638=CARTESIAN_POINT('Ctrl Pts',(-5.63040001011275,5.85822577548536,
79.3275143464349));
#169639=CARTESIAN_POINT('Ctrl Pts',(-5.68358208450952,5.80682239566888,
79.3304031698857));
#169640=CARTESIAN_POINT('Ctrl Pts',(-5.71993954157433,5.77101233222465,
79.3323892404417));
#169641=CARTESIAN_POINT('Ctrl Pts',(-6.06434917820577,5.42533579981107,
79.3513231294378));
#169642=CARTESIAN_POINT('Ctrl Pts',(-6.34727749853782,5.09143218799429,
79.3678243463143));
#169643=CARTESIAN_POINT('Ctrl Pts',(-6.77660607443729,4.49299824290805,
79.395804094763));
#169644=CARTESIAN_POINT('Ctrl Pts',(-6.93763031206454,4.24013039441526,
79.4072052852121));
#169645=CARTESIAN_POINT('Ctrl Pts',(-7.14236390248337,3.87561264261209,
79.4232863293808));
#169646=CARTESIAN_POINT('Ctrl Pts',(-7.19813685887801,3.77101589898547,
79.4278614429181));
#169647=CARTESIAN_POINT('Ctrl Pts',(-7.28069365319139,3.60767886783991,
79.4349554897496));
#169648=CARTESIAN_POINT('Ctrl Pts',(-7.30909944012245,3.54977635981188,
79.4374607204884));
#169649=CARTESIAN_POINT('Ctrl Pts',(-7.35535626318044,3.4525764267084,79.441651560756));
#169650=CARTESIAN_POINT('Ctrl Pts',(-7.37358898553961,3.4134638120929,79.4433340174387));
#169651=CARTESIAN_POINT('Ctrl Pts',(-7.40864256056318,3.33667576854119,
79.4466298518094));
#169652=CARTESIAN_POINT('Ctrl Pts',(-7.42548974467901,3.29901376354829,
79.4482429706135));
#169653=CARTESIAN_POINT('Ctrl Pts',(-7.44209777836504,3.26111456933565,
79.4498630049378));
#169654=CARTESIAN_POINT('Ctrl Pts',(-7.44214623868653,3.26100397716454,
79.4498677322696));
#169655=CARTESIAN_POINT('Ctrl Pts',(-7.44224334356792,3.26078235893044,
79.4498772054249));
#169656=CARTESIAN_POINT('Ctrl Pts',(-7.44229198810876,3.2606713328585,79.4498819512484));
#169657=CARTESIAN_POINT('Ctrl Pts',(-7.44238946323068,3.26044884255245,
79.4498914615692));
#169658=CARTESIAN_POINT('Ctrl Pts',(-7.44243829377661,3.2603373783454,79.4498962260649));
#169659=CARTESIAN_POINT('Ctrl Pts',(-7.45706657733138,3.22694373788202,
79.4513236163018));
#169660=CARTESIAN_POINT('Ctrl Pts',(-7.4714225898597,3.19356420015875,79.4527479041842));
#169661=CARTESIAN_POINT('Ctrl Pts',(-7.5041163315556,3.11611994700133,79.4560468152676));
#169662=CARTESIAN_POINT('Ctrl Pts',(-7.52229065536023,3.07198774696187,
79.4579225653743));
#169663=CARTESIAN_POINT('Ctrl Pts',(-7.57741300256708,2.93471295172874,
79.4637446934063));
#169664=CARTESIAN_POINT('Ctrl Pts',(-7.61302753758419,2.84104548796949,
79.4676997387034));
#169665=CARTESIAN_POINT('Ctrl Pts',(-7.76073995265698,2.42981596229223,
79.4849895200201));
#169666=CARTESIAN_POINT('Ctrl Pts',(-7.854765118708,2.10612179280337,79.4983623971184));
#169667=CARTESIAN_POINT('Ctrl Pts',(-8.08129933995873,1.0956990328556,79.5402666655479));
#169668=CARTESIAN_POINT('Ctrl Pts',(-8.14556302194663,0.397010978487219,
79.5699204200111));
#169669=CARTESIAN_POINT('Ctrl Pts',(-8.108688417812,-0.597143940885287,
79.6118234874032));
#169670=CARTESIAN_POINT('Ctrl Pts',(-8.0815348683483,-0.892309858572796,
79.6241587852685));
#169671=CARTESIAN_POINT('Ctrl Pts',(-8.03488495953414,-1.20866328992491,
79.6368880368299));
#169672=CARTESIAN_POINT('Ctrl Pts',(-8.03134450689027,-1.23196943421648,
79.6378228340485));
#169673=CARTESIAN_POINT('Ctrl Pts',(-8.02614388101788,-1.26522874202748,
79.639152278399));
#169674=CARTESIAN_POINT('Ctrl Pts',(-8.02456653388719,-1.27519461761843,
79.6395500487517));
#169675=CARTESIAN_POINT('Ctrl Pts',(-8.02180986837902,-1.29240390551888,
79.6402358838933));
#169676=CARTESIAN_POINT('Ctrl Pts',(-8.0206392944218,-1.29964869432815,
79.6405242880794));
#169677=CARTESIAN_POINT('Ctrl Pts',(-8.01837909756845,-1.31351790244831,
79.6410757756098));
#169678=CARTESIAN_POINT('Ctrl Pts',(-8.01729107724848,-1.32014257387951,
79.6413389222361));
#169679=CARTESIAN_POINT('Ctrl Pts',(-8.01472287049419,-1.33565943764376,
79.6419546343519));
#169680=CARTESIAN_POINT('Ctrl Pts',(-8.01323609207674,-1.34455054114052,
79.6423069330853));
#169681=CARTESIAN_POINT('Ctrl Pts',(-8.00811313887119,-1.37487605689249,
79.6435067875559));
#169682=CARTESIAN_POINT('Ctrl Pts',(-8.00440571425925,-1.39629846046266,
79.6443513890976));
#169683=CARTESIAN_POINT('Ctrl Pts',(-7.93907008183659,-1.76501039141687,
79.6588335865131));
#169684=CARTESIAN_POINT('Ctrl Pts',(-7.8549786721865,-2.10793912567164,
79.6713548347689));
#169685=CARTESIAN_POINT('Ctrl Pts',(-7.59824952072826,-2.92181068195103,
79.7005787980686));
#169686=CARTESIAN_POINT('Ctrl Pts',(-7.40381502759464,-3.38436344734547,
79.7168387199858));
#169687=CARTESIAN_POINT('Ctrl Pts',(-6.93130672607255,-4.26959230667677,
79.7509949997151));
#169688=CARTESIAN_POINT('Ctrl Pts',(-6.65395118467857,-4.69012734905862,
79.7688454272494));
#169689=CARTESIAN_POINT('Ctrl Pts',(-6.32196444513039,-5.10423766924018,
79.7892914992691));
#169690=CARTESIAN_POINT('Ctrl Pts',(-6.30428058851691,-5.12606309676613,
79.7903779201944));
#169691=CARTESIAN_POINT('Ctrl Pts',(-6.27832336961615,-5.15776202841568,
79.7919688572227));
#169692=CARTESIAN_POINT('Ctrl Pts',(-6.27013906135957,-5.16770835328576,
79.7924699401367));
#169693=CARTESIAN_POINT('Ctrl Pts',(-6.25573982002624,-5.18512307166601,
79.7933505995412));
#169694=CARTESIAN_POINT('Ctrl Pts',(-6.24953506809218,-5.19259986866516,
79.7937297816029));
#169695=CARTESIAN_POINT('Ctrl Pts',(-6.2374655889381,-5.20709075989434,
79.7944667878446));
#169696=CARTESIAN_POINT('Ctrl Pts',(-6.23160240244877,-5.21410612206178,
79.7948245519877));
#169697=CARTESIAN_POINT('Ctrl Pts',(-6.21758312453061,-5.23082290768202,
79.7956793683499));
#169698=CARTESIAN_POINT('Ctrl Pts',(-6.20941616135637,-5.24051515934319,
79.7961768436944));
#169699=CARTESIAN_POINT('Ctrl Pts',(-6.18467455248069,-5.26973855393352,
79.7976824423594));
#169700=CARTESIAN_POINT('Ctrl Pts',(-6.16803026223607,-5.28921037740669,
79.7986932866373));
#169701=CARTESIAN_POINT('Ctrl Pts',(-5.99335275549731,-5.49161630846467,
79.8092813739953));
#169702=CARTESIAN_POINT('Ctrl Pts',(-5.8273321890406,-5.6674786537219,79.8191760323589));
#169703=CARTESIAN_POINT('Ctrl Pts',(-5.54283205088212,-5.94310870958965,
79.8358662453626));
#169704=CARTESIAN_POINT('Ctrl Pts',(-5.4289002055741,-6.04736042238196,
79.8424855703851));
#169705=CARTESIAN_POINT('Ctrl Pts',(-4.79948178503529,-6.5911717327529,
79.8786451579491));
#169706=CARTESIAN_POINT('Ctrl Pts',(-4.23356660802693,-6.96817019509298,
79.909969508988));
#169707=CARTESIAN_POINT('Ctrl Pts',(-3.54362613275228,-7.31239915819436,
79.9434093858311));
#169708=CARTESIAN_POINT('Ctrl Pts',(-3.45906120635346,-7.35277933857432,
79.9474291721293));
#169709=CARTESIAN_POINT('Ctrl Pts',(-3.24717809390565,-7.44948990554553,
79.9572770793459));
#169710=CARTESIAN_POINT('Ctrl Pts',(-3.11906883995627,-7.50403104082421,
79.9630306492516));
#169711=CARTESIAN_POINT('Ctrl Pts',(-2.96152567164898,-7.56637068065159,
79.9698290985873));
#169712=CARTESIAN_POINT('Ctrl Pts',(-2.93338255546748,-7.57732580785143,
79.9710335451564));
#169713=CARTESIAN_POINT('Ctrl Pts',(-2.89448076384879,-7.59221969472611,
79.972685399136));
#169714=CARTESIAN_POINT('Ctrl Pts',(-2.88377408540563,-7.59629289926265,
79.9731386711016));
#169715=CARTESIAN_POINT('Ctrl Pts',(-2.86571253794426,-7.60312047067602,
79.9739010789906));
#169716=CARTESIAN_POINT('Ctrl Pts',(-2.85836224385052,-7.60588683358021,
79.9742107241688));
#169717=CARTESIAN_POINT('Ctrl Pts',(-2.84382928529955,-7.61133242783804,
79.9748217410348));
#169718=CARTESIAN_POINT('Ctrl Pts',(-2.83664681789742,-7.61401215930237,
79.9751231333656));
#169719=CARTESIAN_POINT('Ctrl Pts',(-2.82082577767653,-7.61988939177973,
79.9757857536848));
#169720=CARTESIAN_POINT('Ctrl Pts',(-2.81218553165092,-7.62308237836851,
79.9761467967505));
#169721=CARTESIAN_POINT('Ctrl Pts',(-2.78209646027183,-7.6341436198291,
79.9774012715646));
#169722=CARTESIAN_POINT('Ctrl Pts',(-2.76061978548504,-7.64193613784793,
79.9782916733892));
#169723=CARTESIAN_POINT('Ctrl Pts',(-2.50724267697428,-7.73266302876462,
79.9887402592492));
#169724=CARTESIAN_POINT('Ctrl Pts',(-2.27170853626954,-7.80510695827477,
79.997903124035));
#169725=CARTESIAN_POINT('Ctrl Pts',(-1.24319359192606,-8.07093700430364,
80.036717518111));
#169726=CARTESIAN_POINT('Ctrl Pts',(-0.426899983947643,-8.15496136964204,
80.065109091841));
#169727=CARTESIAN_POINT('Ctrl Pts',(0.494831248385932,-8.11087049864078,
80.1002571489554));
#169728=CARTESIAN_POINT('Ctrl Pts',(0.601324214880989,-8.10367119843295,
80.1043537111171));
#169729=CARTESIAN_POINT('Ctrl Pts',(0.743084156623056,-8.09127796786457,
80.1098561276645));
#169730=CARTESIAN_POINT('Ctrl Pts',(0.778504157261536,-8.08794686409379,
80.1112350434894));
#169731=CARTESIAN_POINT('Ctrl Pts',(0.837154975236383,-8.0820421514253,
80.1135250930859));
#169732=CARTESIAN_POINT('Ctrl Pts',(0.860398673824311,-8.07960072696592,
80.1144344127519));
#169733=CARTESIAN_POINT('Ctrl Pts',(0.905441327269623,-8.07467305397167,
80.1161999191652));
#169734=CARTESIAN_POINT('Ctrl Pts',(0.927241410210268,-8.07219872709752,
80.1170559305187));
#169735=CARTESIAN_POINT('Ctrl Pts',(0.976548503732556,-8.06639995657468,
80.1189956446018));
#169736=CARTESIAN_POINT('Ctrl Pts',(1.00404903735945,-8.06302305353095,
80.1200800454552));
#169737=CARTESIAN_POINT('Ctrl Pts',(1.08531684146909,-8.05262163196699,
80.123292539672));
#169738=CARTESIAN_POINT('Ctrl Pts',(1.13903142057696,-8.04519950966483,
80.1254261664822));
#169739=CARTESIAN_POINT('Ctrl Pts',(1.74556550477174,-7.95519431031257,
80.1496458110455));
#169740=CARTESIAN_POINT('Ctrl Pts',(2.28848124585185,-7.81632195398078,
80.1726743097189));
#169741=CARTESIAN_POINT('Ctrl Pts',(2.9498773626595,-7.57226902120199,80.2024754480087));
#169742=CARTESIAN_POINT('Ctrl Pts',(3.08555978973163,-7.51800206380859,
80.2086771757578));
#169743=CARTESIAN_POINT('Ctrl Pts',(3.58007475896511,-7.30457454173073,
80.2315329771549));
#169744=CARTESIAN_POINT('Ctrl Pts',(3.92871379136949,-7.12312937015013,
80.248174196319));
#169745=CARTESIAN_POINT('Ctrl Pts',(4.30585141668263,-6.89070962195107,
80.2660287494273));
#169746=CARTESIAN_POINT('Ctrl Pts',(4.34857657533092,-6.86382673223187,
80.2680487075212));
#169747=CARTESIAN_POINT('Ctrl Pts',(4.40274650697278,-6.82903390234082,
80.2706038552923));
#169748=CARTESIAN_POINT('Ctrl Pts',(4.41442480561729,-6.82149063492429,
80.2711543571048));
#169749=CARTESIAN_POINT('Ctrl Pts',(4.43312023609077,-6.80934673359565,
80.2720350073022));
#169750=CARTESIAN_POINT('Ctrl Pts',(4.44014967542445,-6.80476515586194,
80.272365986127));
#169751=CARTESIAN_POINT('Ctrl Pts',(4.45346705308614,-6.79605586684041,
80.2729927409777));
#169752=CARTESIAN_POINT('Ctrl Pts',(4.45975637865332,-6.7919302986462,80.2732886123013));
#169753=CARTESIAN_POINT('Ctrl Pts',(4.47400451186946,-6.78255571923566,
80.2739585998714));
#169754=CARTESIAN_POINT('Ctrl Pts',(4.48195983645202,-6.77730141591512,
80.2743324738295));
#169755=CARTESIAN_POINT('Ctrl Pts',(4.50592873408012,-6.76140986702241,
80.2754582651974));
#169756=CARTESIAN_POINT('Ctrl Pts',(4.5219138892313,-6.75072973337289,80.2762081685908));
#169757=CARTESIAN_POINT('Ctrl Pts',(4.64961327478309,-6.66475307450011,
80.2821907617029));
#169758=CARTESIAN_POINT('Ctrl Pts',(4.75946565288033,-6.58675372179188,
80.2872750161332));
#169759=CARTESIAN_POINT('Ctrl Pts',(4.90163552238049,-6.48039282188968,
80.2938017440323));
#169760=CARTESIAN_POINT('Ctrl Pts',(4.93572683987588,-6.45446531932871,
80.2953633030543));
#169761=CARTESIAN_POINT('Ctrl Pts',(5.04254554154338,-6.37188516063423,
80.3002496549951));
#169762=CARTESIAN_POINT('Ctrl Pts',(5.11451567354246,-6.314262909118,80.303532295113));
#169763=CARTESIAN_POINT('Ctrl Pts',(5.76082675676988,-5.77849772200924,
80.3330539952394));
#169764=CARTESIAN_POINT('Ctrl Pts',(6.26762705064367,-5.22447338285556,
80.3568081953172));
#169765=CARTESIAN_POINT('Ctrl Pts',(6.86659777771854,-4.35485119343471,
80.3943050864318));
#169766=CARTESIAN_POINT('Ctrl Pts',(7.02699372817844,-4.09099407240808,
80.4056604054243));
#169767=CARTESIAN_POINT('Ctrl Pts',(7.18444551444592,-3.79527764830921,
80.418576512421));
#169768=CARTESIAN_POINT('Ctrl Pts',(7.19678498398481,-3.77182656764837,
80.4196019478341));
#169769=CARTESIAN_POINT('Ctrl Pts',(7.21481127316018,-3.73715721205776,
80.4211197223189));
#169770=CARTESIAN_POINT('Ctrl Pts',(7.2205871703039,-3.725985325965,80.4216090859016));
#169771=CARTESIAN_POINT('Ctrl Pts',(7.23075864020387,-3.70619893958151,
80.4224762887091));
#169772=CARTESIAN_POINT('Ctrl Pts',(7.23516482077516,-3.6975899053385,80.4228537736425));
#169773=CARTESIAN_POINT('Ctrl Pts',(7.24375045343898,-3.6807407268815,80.4235928986079));
#169774=CARTESIAN_POINT('Ctrl Pts',(7.24793124234487,-3.67250127784988,
80.4239544934289));
#169775=CARTESIAN_POINT('Ctrl Pts',(7.25916614117057,-3.65026576399187,
80.4249307379771));
#169776=CARTESIAN_POINT('Ctrl Pts',(7.26619380696334,-3.6362564223695,80.4255462637295));
#169777=CARTESIAN_POINT('Ctrl Pts',(7.29191839136537,-3.58460323738164,
80.4278174319999));
#169778=CARTESIAN_POINT('Ctrl Pts',(7.31036351679667,-3.54683512214842,
80.4294813843808));
#169779=CARTESIAN_POINT('Ctrl Pts',(7.62902417998136,-2.88130117491019,
80.458863744309));
#169780=CARTESIAN_POINT('Ctrl Pts',(7.84762000705927,-2.21776596444659,
80.4894339262253));
#169781=CARTESIAN_POINT('Ctrl Pts',(8.05421590018177,-1.14361082310715,
80.538737387914));
#169782=CARTESIAN_POINT('Ctrl Pts',(8.10057891496814,-0.747581756129389,
80.5567974548414));
#169783=CARTESIAN_POINT('Ctrl Pts',(8.12269738095583,-0.234200122211309,
80.5790892261596));
#169784=CARTESIAN_POINT('Ctrl Pts',(8.12520814609431,-0.11856077287903,
80.5840358250579));
#169785=CARTESIAN_POINT('Ctrl Pts',(8.12529666042017,0.129105673270558,
80.5944232779334));
#169786=CARTESIAN_POINT('Ctrl Pts',(8.1221269073351,0.261102652816135,80.5998289460686));
#169787=CARTESIAN_POINT('Ctrl Pts',(8.11485051036185,0.411373115696335,
80.6058136959489));
#169788=CARTESIAN_POINT('Ctrl Pts',(8.11389737312719,0.429762809132297,
80.6065434389428));
#169789=CARTESIAN_POINT('Ctrl Pts',(8.11237862533107,0.457256824481047,
80.6076306948971));
#169790=CARTESIAN_POINT('Ctrl Pts',(8.11186019030103,0.46636361157105,80.6079902063516));
#169791=CARTESIAN_POINT('Ctrl Pts',(8.11090559125271,0.482648702346258,
80.6086320217353));
#169792=CARTESIAN_POINT('Ctrl Pts',(8.11047523086395,0.489827326796356,
80.6089145660402));
#169793=CARTESIAN_POINT('Ctrl Pts',(8.10954493707778,0.505007676343931,
80.6095112769365));
#169794=CARTESIAN_POINT('Ctrl Pts',(8.10904268973662,0.513009255549799,
80.6098253488854));
#169795=CARTESIAN_POINT('Ctrl Pts',(8.10767755195224,0.534255021866719,
80.6106580926137));
#169796=CARTESIAN_POINT('Ctrl Pts',(8.10679405041784,0.547497891841711,
80.6111759399136));
#169797=CARTESIAN_POINT('Ctrl Pts',(8.10256105203657,0.608688916857114,
80.6135633505826));
#169798=CARTESIAN_POINT('Ctrl Pts',(8.09881854971916,0.656609482743975,
80.615417699697));
#169799=CARTESIAN_POINT('Ctrl Pts',(8.06232803287315,1.07588594626633,80.6315283753008));
#169800=CARTESIAN_POINT('Ctrl Pts',(8.00448149591947,1.44463542380424,80.6449428211977));
#169801=CARTESIAN_POINT('Ctrl Pts',(7.81282683882899,2.28428722419117,80.6758177467193));
#169802=CARTESIAN_POINT('Ctrl Pts',(7.66143275245466,2.74966762476547,80.6932327669446));
#169803=CARTESIAN_POINT('Ctrl Pts',(7.30323188719196,3.58610676120484,80.7269901137275));
#169804=CARTESIAN_POINT('Ctrl Pts',(7.10740349901889,3.96006894938149,80.7430652641163));
#169805=CARTESIAN_POINT('Ctrl Pts',(6.82408408530577,4.41180841967697,80.7636739943391));
#169806=CARTESIAN_POINT('Ctrl Pts',(6.76275853439752,4.50524958718629,80.7680086994423));
#169807=CARTESIAN_POINT('Ctrl Pts',(6.67169259382201,4.63795485454312,80.7742787784615));
#169808=CARTESIAN_POINT('Ctrl Pts',(6.64349197906995,4.67826053093083,80.776198672709));
#169809=CARTESIAN_POINT('Ctrl Pts',(6.59292970082035,4.74914734523146,80.7796037148111));
#169810=CARTESIAN_POINT('Ctrl Pts',(6.57071686423912,4.77983288656315,80.7810872898421));
#169811=CARTESIAN_POINT('Ctrl Pts',(6.52390466738483,4.84355779156074,80.7841887699726));
#169812=CARTESIAN_POINT('Ctrl Pts',(6.49926701705495,4.87656768773171,80.7858070437115));
#169813=CARTESIAN_POINT('Ctrl Pts',(6.43388540231772,4.96279133168555,80.7900655123056));
#169814=CARTESIAN_POINT('Ctrl Pts',(6.39273231220045,5.01569064848147,80.7927100227115));
#169815=CARTESIAN_POINT('Ctrl Pts',(6.18610467256461,5.2746208583289,80.8058173005992));
#169816=CARTESIAN_POINT('Ctrl Pts',(6.01130449031638,5.47300011999977,80.8163808359492));
#169817=CARTESIAN_POINT('Ctrl Pts',(5.62068189614564,5.87498069793229,80.8389777022667));
#169818=CARTESIAN_POINT('Ctrl Pts',(5.40274579160056,6.07600184752323,80.8510182949538));
#169819=CARTESIAN_POINT('Ctrl Pts',(4.91751006313996,6.4767836980718,80.8765940861616));
#169820=CARTESIAN_POINT('Ctrl Pts',(4.64789412919812,6.67290936117833,80.8901054505419));
#169821=CARTESIAN_POINT('Ctrl Pts',(4.32111236860767,6.88117987047064,80.905520331601));
#169822=CARTESIAN_POINT('Ctrl Pts',(4.27493222371801,6.90996404221723,80.9076773794519));
#169823=CARTESIAN_POINT('Ctrl Pts',(4.20859309488172,6.95039375502747,80.9107444677031));
#169824=CARTESIAN_POINT('Ctrl Pts',(4.18866802644074,6.96241979191648,80.9116616517794));
#169825=CARTESIAN_POINT('Ctrl Pts',(4.15284425202332,6.98383226018462,80.9133033574825));
#169826=CARTESIAN_POINT('Ctrl Pts',(4.13696472367219,6.99325041007904,80.9140285112471));
#169827=CARTESIAN_POINT('Ctrl Pts',(4.10198888064589,7.01383376681524,80.9156203092729));
#169828=CARTESIAN_POINT('Ctrl Pts',(4.08287877856378,7.02497528606073,80.9164865118778));
#169829=CARTESIAN_POINT('Ctrl Pts',(4.02762828412385,7.05688567436464,80.9189811771923));
#169830=CARTESIAN_POINT('Ctrl Pts',(3.99137316627603,7.07745471840137,80.9206062908325));
#169831=CARTESIAN_POINT('Ctrl Pts',(3.81747246452006,7.17435459822572,80.9283498449519));
#169832=CARTESIAN_POINT('Ctrl Pts',(3.67778542959045,7.24695488587093,80.9344178344348));
#169833=CARTESIAN_POINT('Ctrl Pts',(3.2716870945602,7.4432510076197,80.9517730955065));
#169834=CARTESIAN_POINT('Ctrl Pts',(3.00056496329956,7.55662166852448,80.963026573868));
#169835=CARTESIAN_POINT('Ctrl Pts',(2.655899843565,7.67926386047105,80.9772017949938));
#169836=CARTESIAN_POINT('Ctrl Pts',(2.58757817016605,7.70255389820744,80.9800048079079));
#169837=CARTESIAN_POINT('Ctrl Pts',(2.48030765741858,7.73753280854493,80.9843980784981));
#169838=CARTESIAN_POINT('Ctrl Pts',(2.44156585693646,7.74984491393775,80.9859831892342));
#169839=CARTESIAN_POINT('Ctrl Pts',(2.36924125897723,7.77223343902952,80.9889399345093));
#169840=CARTESIAN_POINT('Ctrl Pts',(2.3356824498974,7.78238422704716,80.9903109163695));
#169841=CARTESIAN_POINT('Ctrl Pts',(2.2602814232518,7.80465970763496,80.9933894612701));
#169842=CARTESIAN_POINT('Ctrl Pts',(2.21840531223,7.81666572880469,80.9950979692793));
#169843=CARTESIAN_POINT('Ctrl Pts',(2.09031882062074,7.85227635580488,81.0003206102493));
#169844=CARTESIAN_POINT('Ctrl Pts',(2.00381412016627,7.87479558796864,81.0038434942154));
#169845=CARTESIAN_POINT('Ctrl Pts',(1.85220985007238,7.91160194768301,81.0100115572356));
#169846=CARTESIAN_POINT('Ctrl Pts',(1.78727307790877,7.9265239288191,81.0126516041767));
#169847=CARTESIAN_POINT('Ctrl Pts',(1.48378140644731,7.99234494070813,81.0249807900875));
#169848=CARTESIAN_POINT('Ctrl Pts',(1.24319657371835,8.03328362040867,81.034732580768));
#169849=CARTESIAN_POINT('Ctrl Pts',(0.81466573281204,8.08648965914828,81.0519761769169));
#169850=CARTESIAN_POINT('Ctrl Pts',(0.627445408230941,8.10316658532627,
81.0594661245974));
#169851=CARTESIAN_POINT('Ctrl Pts',(0.405978431881623,8.11517204411552,
81.0682162877837));
#169852=CARTESIAN_POINT('Ctrl Pts',(0.372131306239305,8.11679457044921,
81.0695505095287));
#169853=CARTESIAN_POINT('Ctrl Pts',(0.319929534305792,8.11896974947659,
81.0716029425798));
#169854=CARTESIAN_POINT('Ctrl Pts',(0.301581661774526,8.1196719885897,81.0723233004479));
#169855=CARTESIAN_POINT('Ctrl Pts',(0.262936815650409,8.12101989705131,
81.0738384725647));
#169856=CARTESIAN_POINT('Ctrl Pts',(0.242639518906035,8.12165167958616,
81.0746330893633));
#169857=CARTESIAN_POINT('Ctrl Pts',(0.193602941383203,8.12299402329623,
81.0765501768139));
#169858=CARTESIAN_POINT('Ctrl Pts',(0.1648618075648,8.1236281669237,81.0776716227412));
#169859=CARTESIAN_POINT('Ctrl Pts',(0.0621024395873807,8.12534987967175,
81.0816743273612));
#169860=CARTESIAN_POINT('Ctrl Pts',(-0.0119268664681597,8.12557845625808,
81.0845452538756));
#169861=CARTESIAN_POINT('Ctrl Pts',(-0.369994541686901,8.12179058581634,
81.098391877387));
#169862=CARTESIAN_POINT('Ctrl Pts',(-0.653688961810558,8.10389236920271,
81.1092478177369));
#169863=CARTESIAN_POINT('Ctrl Pts',(-1.08978901644335,8.05332595479917,
81.1260819407022));
#169864=CARTESIAN_POINT('Ctrl Pts',(-1.24317143395505,8.03107860112409,
81.1320297526505));
#169865=CARTESIAN_POINT('Ctrl Pts',(-1.58221447599178,7.97195603875809,
81.1452899149938));
#169866=CARTESIAN_POINT('Ctrl Pts',(-1.76741206402433,7.93295274603368,
81.1526097747279));
#169867=CARTESIAN_POINT('Ctrl Pts',(-2.01583687268292,7.87150173927167,
81.1625693127194));
#169868=CARTESIAN_POINT('Ctrl Pts',(-2.08039616855866,7.85468584093349,
81.1651704116254));
#169869=CARTESIAN_POINT('Ctrl Pts',(-2.19801190844992,7.82249842111764,
81.1699338931605));
#169870=CARTESIAN_POINT('Ctrl Pts',(-2.25113280011631,7.80737721562312,
81.1720946097677));
#169871=CARTESIAN_POINT('Ctrl Pts',(-2.36132569144571,7.77479197617668,
81.1765965837412));
#169872=CARTESIAN_POINT('Ctrl Pts',(-2.41836778989625,7.75723832918322,
81.1789382242761));
#169873=CARTESIAN_POINT('Ctrl Pts',(-2.58397954931485,7.70427011446431,
81.1857696217646));
#169874=CARTESIAN_POINT('Ctrl Pts',(-2.69200208731398,7.66719328768862,
81.1902670756382));
#169875=CARTESIAN_POINT('Ctrl Pts',(-2.97427919277889,7.56360554216872,
81.2021261824926));
#169876=CARTESIAN_POINT('Ctrl Pts',(-3.14708771209144,7.49335068137522,
81.2094959931763));
#169877=CARTESIAN_POINT('Ctrl Pts',(-3.37894138490143,7.38965483751212,
81.2195083376915));
#169878=CARTESIAN_POINT('Ctrl Pts',(-3.4402116620601,7.36133053613394,81.2221662148209));
#169879=CARTESIAN_POINT('Ctrl Pts',(-3.53497466023058,7.31608153362273,
81.2262934579289));
#169880=CARTESIAN_POINT('Ctrl Pts',(-3.56871502384484,7.29968272919635,
81.2277662436392));
#169881=CARTESIAN_POINT('Ctrl Pts',(-3.64326353097164,7.26280956611457,
81.2310270058664));
#169882=CARTESIAN_POINT('Ctrl Pts',(-3.68401513931543,7.24222372074472,
81.2328140322197));
#169883=CARTESIAN_POINT('Ctrl Pts',(-3.85591077897572,7.15356359273791,
81.2403754576911));
#169884=CARTESIAN_POINT('Ctrl Pts',(-3.9853588513958,7.08226200656618,81.2461285044163));
#169885=CARTESIAN_POINT('Ctrl Pts',(-4.27382331106329,6.91295782530399,
81.259151107472));
#169886=CARTESIAN_POINT('Ctrl Pts',(-4.43154955123481,6.81292300257379,
81.2664172139082));
#169887=CARTESIAN_POINT('Ctrl Pts',(-4.63996055441071,6.67044044216308,
81.2762813878693));
#169888=CARTESIAN_POINT('Ctrl Pts',(-4.69377976955234,6.63267978098273,
81.2788532106595));
#169889=CARTESIAN_POINT('Ctrl Pts',(-4.7871010189209,6.56549895226251,81.2833586103617));
#169890=CARTESIAN_POINT('Ctrl Pts',(-4.82680489320903,6.53636498081505,
81.2852903033399));
#169891=CARTESIAN_POINT('Ctrl Pts',(-4.91932878920685,6.4671698872635,81.289828160186));
#169892=CARTESIAN_POINT('Ctrl Pts',(-4.97192817960097,6.42681975912757,
81.2924361771976));
#169893=CARTESIAN_POINT('Ctrl Pts',(-5.135339957683,6.29825616889112,81.3006313859687));
#169894=CARTESIAN_POINT('Ctrl Pts',(-5.24434262832098,6.20778681756965,
81.3062347090037));
#169895=CARTESIAN_POINT('Ctrl Pts',(-5.43445159165915,6.04141898500454,
81.3162672446698));
#169896=CARTESIAN_POINT('Ctrl Pts',(-5.5164720412083,5.96661909978844,81.3206870843479));
#169897=CARTESIAN_POINT('Ctrl Pts',(-5.74376736746391,5.75063916943936,
81.3331994109807));
#169898=CARTESIAN_POINT('Ctrl Pts',(-5.88533182185289,5.60567420615562,
81.3413110445535));
#169899=CARTESIAN_POINT('Ctrl Pts',(-6.03694456536234,5.43833877674629,
81.3503487414014));
#169900=CARTESIAN_POINT('Ctrl Pts',(-6.05248440961696,5.42103872038097,
81.3512793635894));
#169901=CARTESIAN_POINT('Ctrl Pts',(-6.11121937347249,5.35508342212963,
81.3548129633114));
#169902=CARTESIAN_POINT('Ctrl Pts',(-6.15390387138072,5.30597661662688,
81.3574144780495));
#169903=CARTESIAN_POINT('Ctrl Pts',(-6.30057988257971,5.13308068204843,
81.3664685577532));
#169904=CARTESIAN_POINT('Ctrl Pts',(-6.40146403186574,5.00670383906051,
81.3729023536171));
#169905=CARTESIAN_POINT('Ctrl Pts',(-6.52111926621317,4.84727856949658,
81.3807682647321));
#169906=CARTESIAN_POINT('Ctrl Pts',(-6.54351747562544,4.8169995931263,81.3822513989634));
#169907=CARTESIAN_POINT('Ctrl Pts',(-6.57877179243205,4.76864145295588,
81.3846024443188));
#169908=CARTESIAN_POINT('Ctrl Pts',(-6.59176573309836,4.75066354609143,
81.3854726492595));
#169909=CARTESIAN_POINT('Ctrl Pts',(-6.61617220563892,4.71660278146744,
81.3871139664015));
#169910=CARTESIAN_POINT('Ctrl Pts',(-6.62760012110755,4.70053114986841,
81.3878853525227));
#169911=CARTESIAN_POINT('Ctrl Pts',(-6.654746910764,4.66205748988672,81.389724514324));
#169912=CARTESIAN_POINT('Ctrl Pts',(-6.670411348865,4.63961732567824,81.3907912131702));
#169913=CARTESIAN_POINT('Ctrl Pts',(-6.7329011502954,4.54912662986257,81.3950698449066));
#169914=CARTESIAN_POINT('Ctrl Pts',(-6.77880122275737,4.48044251888115,
81.3982658041701));
#169915=CARTESIAN_POINT('Ctrl Pts',(-6.90670688812173,4.28258054662003,
81.4073493506183));
#169916=CARTESIAN_POINT('Ctrl Pts',(-6.98612223603341,4.15176984356778,
81.4132084872747));
#169917=CARTESIAN_POINT('Ctrl Pts',(-7.21590606495064,3.74799531883072,
81.4309890038107));
#169918=CARTESIAN_POINT('Ctrl Pts',(-7.35430936779103,3.46855886464907,
81.4428958805196));
#169919=CARTESIAN_POINT('Ctrl Pts',(-7.50284778443874,3.11954332282749,
81.457588352001));
#169920=CARTESIAN_POINT('Ctrl Pts',(-7.52859200701767,3.05689020745503,
81.4602184085665));
#169921=CARTESIAN_POINT('Ctrl Pts',(-7.56806601876324,2.95729882396646,
81.4643894495567));
#169922=CARTESIAN_POINT('Ctrl Pts',(-7.58231569140425,2.92056986559936,
81.4659256615787));
#169923=CARTESIAN_POINT('Ctrl Pts',(-7.60754859683111,2.85410175856874,
81.4687023920728));
#169924=CARTESIAN_POINT('Ctrl Pts',(-7.61862597983699,2.8243991702804,81.4699420329541));
#169925=CARTESIAN_POINT('Ctrl Pts',(-7.64453396318579,2.75366868562953,
81.4728913319673));
#169926=CARTESIAN_POINT('Ctrl Pts',(-7.65920849768165,2.71258472931922,
81.4746023374135));
#169927=CARTESIAN_POINT('Ctrl Pts',(-7.70325829742431,2.58605169799811,
81.4798660164617));
#169928=CARTESIAN_POINT('Ctrl Pts',(-7.73153954278329,2.50022957247542,
81.4834278997582));
#169929=CARTESIAN_POINT('Ctrl Pts',(-7.7962164734376,2.29235965878099,81.4920361103963));
#169930=CARTESIAN_POINT('Ctrl Pts',(-7.83118552209573,2.16989333244498,
81.4970922375113));
#169931=CARTESIAN_POINT('Ctrl Pts',(-7.92392564316205,1.81358545422193,
81.5117479636237));
#169932=CARTESIAN_POINT('Ctrl Pts',(-7.97419697936925,1.57793289309484,
81.5213774945733));
#169933=CARTESIAN_POINT('Ctrl Pts',(-8.02698230663629,1.26234132770517,
81.5340897875249));
#169934=CARTESIAN_POINT('Ctrl Pts',(-8.03889664921228,1.18409939204704,
81.5372260899323));
#169935=CARTESIAN_POINT('Ctrl Pts',(-8.05320510462085,1.07993121567006,
81.5413757022493));
#169936=CARTESIAN_POINT('Ctrl Pts',(-8.05662036561507,1.05414997904124,
81.5424006064654));
#169937=CARTESIAN_POINT('Ctrl Pts',(-8.06218889979259,1.01050552427739,
81.5441317949691));
#169938=CARTESIAN_POINT('Ctrl Pts',(-8.06440671861917,0.992650769178743,
81.5448389284957));
#169939=CARTESIAN_POINT('Ctrl Pts',(-8.06880676114472,0.956239567780087,
81.5462786516932));
#169940=CARTESIAN_POINT('Ctrl Pts',(-8.0709843207416,0.937682653378452,
81.5470111645334));
#169941=CARTESIAN_POINT('Ctrl Pts',(-8.07616680013874,0.892162220894048,
81.5488048744853));
#169942=CARTESIAN_POINT('Ctrl Pts',(-8.07910071872581,0.865190844377972,
81.5498649929472));
#169943=CARTESIAN_POINT('Ctrl Pts',(-8.08999607218282,0.760138822116573,
81.5539844571854));
#169944=CARTESIAN_POINT('Ctrl Pts',(-8.09696116041502,0.681958663565181,
81.5570294799938));
#169945=CARTESIAN_POINT('Ctrl Pts',(-8.10802951141499,0.533397899484663,
81.5627854375292));
#169946=CARTESIAN_POINT('Ctrl Pts',(-8.11235163682892,0.463040922240359,
81.5654985421627));
#169947=CARTESIAN_POINT('Ctrl Pts',(-8.13085809759842,0.0805140055900297,
81.5801976460154));
#169948=CARTESIAN_POINT('Ctrl Pts',(-8.1279402115312,-0.232222304050683,
81.5920324053402));
#169949=CARTESIAN_POINT('Ctrl Pts',(-8.09080517474827,-0.78561704156093,
81.613098804559));
#169950=CARTESIAN_POINT('Ctrl Pts',(-8.06380055018787,-1.02637316650304,
81.6223051959032));
#169951=CARTESIAN_POINT('Ctrl Pts',(-7.98942409005349,-1.49806236256277,
81.6405942038987));
#169952=CARTESIAN_POINT('Ctrl Pts',(-7.94267825250679,-1.72885739461075,
81.6496643996561));
#169953=CARTESIAN_POINT('Ctrl Pts',(-7.87009051064721,-2.0213149239379,
81.6613787439906));
#169954=CARTESIAN_POINT('Ctrl Pts',(-7.85342172396327,-2.08513928417403,
81.6639487289844));
#169955=CARTESIAN_POINT('Ctrl Pts',(-7.82520583494853,-2.18803572628742,
81.6681150423225));
#169956=CARTESIAN_POINT('Ctrl Pts',(-7.81413875724294,-2.22723644182065,
81.6697077370789));
#169957=CARTESIAN_POINT('Ctrl Pts',(-7.79246853100146,-2.3018444183806,
81.6727496501274));
#169958=CARTESIAN_POINT('Ctrl Pts',(-7.78191763001751,-2.33726582202524,
81.6741984561183));
#169959=CARTESIAN_POINT('Ctrl Pts',(-7.75701439363559,-2.41883247333226,
81.6775455221723));
#169960=CARTESIAN_POINT('Ctrl Pts',(-7.74249133222642,-2.46492409342769,
81.679444919971));
#169961=CARTESIAN_POINT('Ctrl Pts',(-7.69555339661151,-2.60938147193878,
81.6854236316002));
#169962=CARTESIAN_POINT('Ctrl Pts',(-7.66166862545484,-2.70725828762598,
81.689512287444));
#169963=CARTESIAN_POINT('Ctrl Pts',(-7.46407230654591,-3.24456461400162,
81.7121703928581));
#169964=CARTESIAN_POINT('Ctrl Pts',(-7.26443325304684,-3.66981835377763,
81.7308338806236));
#169965=CARTESIAN_POINT('Ctrl Pts',(-6.63490858955856,-4.75560213046735,
81.7823936501349));
#169966=CARTESIAN_POINT('Ctrl Pts',(-6.14400767792136,-5.37482346916863,
81.8166454670327));
#169967=CARTESIAN_POINT('Ctrl Pts',(-5.51183074622765,-5.97044549045938,
81.8519448270577));
#169968=CARTESIAN_POINT('Ctrl Pts',(-5.45090795953746,-6.02611819264225,
81.855263620101));
#169969=CARTESIAN_POINT('Ctrl Pts',(-5.37783255506363,-6.09088114479934,
81.8591371718244));
#169970=CARTESIAN_POINT('Ctrl Pts',(-5.36649053925253,-6.10087660965179,
81.8597353817757));
#169971=CARTESIAN_POINT('Ctrl Pts',(-5.34809238586035,-6.11699948713437,
81.860700812379));
#169972=CARTESIAN_POINT('Ctrl Pts',(-5.34105348542202,-6.12314645913878,
81.8610690102268));
#169973=CARTESIAN_POINT('Ctrl Pts',(-5.32855836589666,-6.13402033065851,
81.8617205337273));
#169974=CARTESIAN_POINT('Ctrl Pts',(-5.32310642958805,-6.13875212200346,
81.8620041094347));
#169975=CARTESIAN_POINT('Ctrl Pts',(-5.31167658836193,-6.14864552241621,
81.8625971400557));
#169976=CARTESIAN_POINT('Ctrl Pts',(-5.30569744643427,-6.15380569624585,
81.8629065202685));
#169977=CARTESIAN_POINT('Ctrl Pts',(-5.290055314261,-6.16726556848658,81.863713670438));
#169978=CARTESIAN_POINT('Ctrl Pts',(-5.28038029080375,-6.17555129580364,
81.8642106998065));
#169979=CARTESIAN_POINT('Ctrl Pts',(-5.23809285415745,-6.21159438856918,
81.8663733242762));
#169980=CARTESIAN_POINT('Ctrl Pts',(-5.20528035224113,-6.23911677638299,
81.8680260939126));
#169981=CARTESIAN_POINT('Ctrl Pts',(-4.95913456579828,-6.44228481318374,
81.8802269082415));
#169982=CARTESIAN_POINT('Ctrl Pts',(-4.73717089428763,-6.60721405815946,
81.8901235807326));
#169983=CARTESIAN_POINT('Ctrl Pts',(-4.02491825212102,-7.08207138350816,
81.9197726119515));
#169984=CARTESIAN_POINT('Ctrl Pts',(-3.50958010288958,-7.35109459795958,
81.938425203669));
#169985=CARTESIAN_POINT('Ctrl Pts',(-2.5360514171208,-7.73339985513728,
81.9742047373154));
#169986=CARTESIAN_POINT('Ctrl Pts',(-2.08829588195924,-7.86612937666202,
81.9908397617143));
#169987=CARTESIAN_POINT('Ctrl Pts',(-1.60017175882261,-7.96618922166575,
82.009997076446));
#169988=CARTESIAN_POINT('Ctrl Pts',(-1.56865124500534,-7.97245593382428,
82.0112383060995));
#169989=CARTESIAN_POINT('Ctrl Pts',(-1.5247278302872,-7.98091794339299,
82.0129738767691));
#169990=CARTESIAN_POINT('Ctrl Pts',(-1.51235557918698,-7.98327168371586,
82.0134634022728));
#169991=CARTESIAN_POINT('Ctrl Pts',(-1.49101300960358,-7.98728057434275,
82.0143089887137));
#169992=CARTESIAN_POINT('Ctrl Pts',(-1.48204526876412,-7.9889494045676,
82.0146646339771));
#169993=CARTESIAN_POINT('Ctrl Pts',(-1.46350828072555,-7.99236671471007,
82.0154004985665));
#169994=CARTESIAN_POINT('Ctrl Pts',(-1.45393866745994,-7.99411311782941,
82.0157807802016));
#169995=CARTESIAN_POINT('Ctrl Pts',(-1.43161806382726,-7.9981451033015,
82.0166686950485));
#169996=CARTESIAN_POINT('Ctrl Pts',(-1.41886471442816,-8.000417382513,82.0171767300198));
#169997=CARTESIAN_POINT('Ctrl Pts',(-1.37884611446021,-8.00744884459757,
82.0187731189416));
#169998=CARTESIAN_POINT('Ctrl Pts',(-1.351562080047,-8.01209919631529,82.0198647579263));
#169999=CARTESIAN_POINT('Ctrl Pts',(-1.07882516095381,-8.05715230755174,
82.0308098872083));
#170000=CARTESIAN_POINT('Ctrl Pts',(-0.831678526566427,-8.08639997640681,
82.0409992817011));
#170001=CARTESIAN_POINT('Ctrl Pts',(-0.200168510864236,-8.13187529847885,
82.0677140292404));
#170002=CARTESIAN_POINT('Ctrl Pts',(0.184704455621429,-8.13223896171834,
82.0846469081139));
#170003=CARTESIAN_POINT('Ctrl Pts',(1.22774153279123,-8.05912905421342,
82.1314375727189));
#170004=CARTESIAN_POINT('Ctrl Pts',(1.87931155853566,-7.93254612609118,
82.1617356762533));
#170005=CARTESIAN_POINT('Ctrl Pts',(2.54579791579657,-7.71622629644003,
82.189999038119));
#170006=CARTESIAN_POINT('Ctrl Pts',(2.58312918384015,-7.7038093812577,82.1915730767375));
#170007=CARTESIAN_POINT('Ctrl Pts',(2.63285733338629,-7.68686697420724,
82.1936593039519));
#170008=CARTESIAN_POINT('Ctrl Pts',(2.64533508307752,-7.68258185235168,
82.1941818907385));
#170009=CARTESIAN_POINT('Ctrl Pts',(2.66480141105156,-7.67584365772699,
82.1949958521376));
#170010=CARTESIAN_POINT('Ctrl Pts',(2.67179713225404,-7.67341139929175,
82.1952881037621));
#170011=CARTESIAN_POINT('Ctrl Pts',(2.68580781571798,-7.66851870980025,
82.195872893064));
#170012=CARTESIAN_POINT('Ctrl Pts',(2.69282274582029,-7.66605821042096,
82.196165427482));
#170013=CARTESIAN_POINT('Ctrl Pts',(2.70864268636155,-7.66048494399679,
82.1968245757013));
#170014=CARTESIAN_POINT('Ctrl Pts',(2.71744573570807,-7.65736661352736,
82.1971909616567));
#170015=CARTESIAN_POINT('Ctrl Pts',(2.7434581876743,-7.64810163886216,82.1982724751819));
#170016=CARTESIAN_POINT('Ctrl Pts',(2.76065231390488,-7.64191208495024,
82.1989858823365));
#170017=CARTESIAN_POINT('Ctrl Pts',(2.89816330922583,-7.59188611192789,
82.2046805553654));
#170018=CARTESIAN_POINT('Ctrl Pts',(3.01745291989317,-7.54526772258471,
82.2095542987271));
#170019=CARTESIAN_POINT('Ctrl Pts',(3.32049265316782,-7.41850294610265,
82.2218630097274));
#170020=CARTESIAN_POINT('Ctrl Pts',(3.50247137403872,-7.33434084950595,
82.2291859021828));
#170021=CARTESIAN_POINT('Ctrl Pts',(4.08780251824189,-7.03687625635104,
82.252945175192));
#170022=CARTESIAN_POINT('Ctrl Pts',(4.4763228269596,-6.79634426738865,82.2690974605615));
#170023=CARTESIAN_POINT('Ctrl Pts',(5.13019258780814,-6.31102835920279,
82.2989079481626));
#170024=CARTESIAN_POINT('Ctrl Pts',(5.4033380341403,-6.07880543496155,82.312310288064));
#170025=CARTESIAN_POINT('Ctrl Pts',(5.69770053235318,-5.79298013793138,
82.3281056855524));
#170026=CARTESIAN_POINT('Ctrl Pts',(5.73478446015894,-5.75627113441738,
82.3301216939825));
#170027=CARTESIAN_POINT('Ctrl Pts',(5.7906725216542,-5.69987195502733,82.3332000600365));
#170028=CARTESIAN_POINT('Ctrl Pts',(5.80973566851486,-5.68044012475289,
82.3342573153322));
#170029=CARTESIAN_POINT('Ctrl Pts',(5.84337091792872,-5.64580793616629,
82.3361356302649));
#170030=CARTESIAN_POINT('Ctrl Pts',(5.85798228876853,-5.63064600527697,
82.3369559478849));
#170031=CARTESIAN_POINT('Ctrl Pts',(5.88857494256762,-5.59865264147786,
82.3386827028612));
#170032=CARTESIAN_POINT('Ctrl Pts',(5.90454339442634,-5.58180916484072,
82.3395893739593));
#170033=CARTESIAN_POINT('Ctrl Pts',(5.94427987994433,-5.53953391110842,
82.3418592316745));
#170034=CARTESIAN_POINT('Ctrl Pts',(5.96795701514219,-5.51401743666631,
82.3432240871158));
#170035=CARTESIAN_POINT('Ctrl Pts',(6.05943343448763,-5.41415532959612,
82.3485466174853));
#170036=CARTESIAN_POINT('Ctrl Pts',(6.12601266472768,-5.33870582326983,
82.3525275336655));
#170037=CARTESIAN_POINT('Ctrl Pts',(6.65123883721597,-4.72073904252836,
82.3848541129689));
#170038=CARTESIAN_POINT('Ctrl Pts',(7.03830096881737,-4.12146893670269,
82.4148973364547));
#170039=CARTESIAN_POINT('Ctrl Pts',(7.4960163322414,-3.15562523039783,82.4601712042922));
#170040=CARTESIAN_POINT('Ctrl Pts',(7.62795014290625,-2.8218131247775,82.4752415196864));
#170041=CARTESIAN_POINT('Ctrl Pts',(7.74453635437266,-2.45812727999125,
82.4904748333208));
#170042=CARTESIAN_POINT('Ctrl Pts',(7.7515702989922,-2.43585528750969,82.491403011818));
#170043=CARTESIAN_POINT('Ctrl Pts',(7.76126912307547,-2.40467784859556,
82.4926954925195));
#170044=CARTESIAN_POINT('Ctrl Pts',(7.76401486746026,-2.39579779928162,
82.4930628479599));
#170045=CARTESIAN_POINT('Ctrl Pts',(7.76900381790987,-2.3795643181103,82.4937329718357));
#170046=CARTESIAN_POINT('Ctrl Pts',(7.77125183462766,-2.37221238299013,
82.4940359260861));
#170047=CARTESIAN_POINT('Ctrl Pts',(7.77576769238533,-2.3573683697006,82.4946465139725));
#170048=CARTESIAN_POINT('Ctrl Pts',(7.77803514828598,-2.34987618162453,
82.4949541322155));
#170049=CARTESIAN_POINT('Ctrl Pts',(7.78355807190093,-2.33153161578746,
82.4957059393094));
#170050=CARTESIAN_POINT('Ctrl Pts',(7.78680167959969,-2.32067566417503,
82.4961496512707));
#170051=CARTESIAN_POINT('Ctrl Pts',(7.79837464934966,-2.2816449294646,82.4977405804065));
#170052=CARTESIAN_POINT('Ctrl Pts',(7.80657395121732,-2.2534315897656,82.498882424986));
#170053=CARTESIAN_POINT('Ctrl Pts',(7.85102631555817,-2.09731871251159,
82.5051534347117));
#170054=CARTESIAN_POINT('Ctrl Pts',(7.88428828445487,-1.96859293647769,
82.5101386823629));
#170055=CARTESIAN_POINT('Ctrl Pts',(8.05410122680693,-1.23782263518701,
82.5375828932488));
#170056=CARTESIAN_POINT('Ctrl Pts',(8.12485328113968,-0.622553316611473,
82.5576087136251));
#170057=CARTESIAN_POINT('Ctrl Pts',(8.12524833638065,-0.0051994849222721,
82.5785614930982));
#170058=CARTESIAN_POINT('',(8.12115743020385,0.00265292485629474,84.5832974432122));
#170059=CARTESIAN_POINT('Ctrl Pts',(8.11704416097363,-0.0053549714695382,
82.5832974432122));
#170060=CARTESIAN_POINT('Ctrl Pts',(8.10035380767694,1.97061005880897,82.6608378090696));
#170061=CARTESIAN_POINT('Ctrl Pts',(6.8826360504109,5.30498188964725,82.7912673300224));
#170062=CARTESIAN_POINT('Ctrl Pts',(2.81786210763212,7.9735377618551,82.9745860060708));
#170063=CARTESIAN_POINT('Ctrl Pts',(-1.31318116064729,8.36857010785244,
83.1332534713571));
#170064=CARTESIAN_POINT('Ctrl Pts',(-5.16809395608702,6.7139926335042,83.2919209366436));
#170065=CARTESIAN_POINT('Ctrl Pts',(-7.73996699874804,3.42788185729169,
83.45058840193));
#170066=CARTESIAN_POINT('Ctrl Pts',(-8.44497665565605,-0.68502664701191,
83.6092558672165));
#170067=CARTESIAN_POINT('Ctrl Pts',(-7.07955773652491,-4.65158818748283,
83.7679233325027));
#170068=CARTESIAN_POINT('Ctrl Pts',(-4.01080233417694,-7.44520758162714,
83.9265907977894));
#170069=CARTESIAN_POINT('Ctrl Pts',(1.42217143211323,-8.84926286475008,
84.138147418171));
#170070=CARTESIAN_POINT('Ctrl Pts',(6.73271600913051,-5.90303377185105,
84.3497040385533));
#170071=CARTESIAN_POINT('Ctrl Pts',(8.06645284195508,-1.72963063830897,
84.5157170985985));
#170072=CARTESIAN_POINT('Ctrl Pts',(8.12089038625466,-0.185607932903464,
84.5759518484531));
#170073=CARTESIAN_POINT('Ctrl Pts',(8.12115743020385,0.00265292485629474,
84.5832974432122));
#170074=CARTESIAN_POINT('',(8.12771990326932,0.00255226563719405,86.5832974432122));
#170075=CARTESIAN_POINT('Ctrl Pts',(8.12115743020385,0.00265292485629474,
84.5832974432122));
#170076=CARTESIAN_POINT('Ctrl Pts',(8.12281313442001,1.16989261279775,84.6288410035486));
#170077=CARTESIAN_POINT('Ctrl Pts',(7.31450585013189,5.04406336557019,84.7801628740762));
#170078=CARTESIAN_POINT('Ctrl Pts',(2.62992883968332,8.56828449165683,84.9843738996985));
#170079=CARTESIAN_POINT('Ctrl Pts',(-2.94483553187362,7.92752136468721,
85.1959305200809));
#170080=CARTESIAN_POINT('Ctrl Pts',(-6.36979470017048,5.58418533793423,
85.354597985367));
#170081=CARTESIAN_POINT('Ctrl Pts',(-8.26960761947702,1.84403959870158,
85.5132654506537));
#170082=CARTESIAN_POINT('Ctrl Pts',(-8.139005581661,-2.3268114042503,85.6719329159399));
#170083=CARTESIAN_POINT('Ctrl Pts',(-6.04529291051799,-5.93644050317469,
85.8306003812265));
#170084=CARTESIAN_POINT('Ctrl Pts',(-2.45563682176731,-8.10723493000542,
85.9892678465127));
#170085=CARTESIAN_POINT('Ctrl Pts',(1.6903925653843,-8.28614652732205,86.1479353117993));
#170086=CARTESIAN_POINT('Ctrl Pts',(6.43672742380675,-6.03729498712186,
86.3459451773656));
#170087=CARTESIAN_POINT('Ctrl Pts',(8.10769023119457,-2.34268520044924,
86.4910658878367));
#170088=CARTESIAN_POINT('Ctrl Pts',(8.12771990326932,0.00255226563719405,
86.5832974432122));
#170089=CARTESIAN_POINT('',(8.12607929659711,-0.000602397288300138,88.5832974432122));
#170090=CARTESIAN_POINT('Ctrl Pts',(8.12771990326932,0.00255226563719405,
86.5832974432122));
#170091=CARTESIAN_POINT('Ctrl Pts',(8.13066181458726,0.347015251300818,
86.5968441980277));
#170092=CARTESIAN_POINT('Ctrl Pts',(8.03485269117909,2.03602439612352,86.6632801079386));
#170093=CARTESIAN_POINT('Ctrl Pts',(6.84908166713345,4.95342653106158,86.782605172945));
#170094=CARTESIAN_POINT('Ctrl Pts',(2.59518421047726,8.5697311209224,86.9941617933268));
#170095=CARTESIAN_POINT('Ctrl Pts',(-3.4701714152711,8.2637724545391,87.2057184137089));
#170096=CARTESIAN_POINT('Ctrl Pts',(-7.34003372474683,4.20018525983518,
87.4172750340907));
#170097=CARTESIAN_POINT('Ctrl Pts',(-8.46845332731791,0.206660721371377,
87.5759424993771));
#170098=CARTESIAN_POINT('Ctrl Pts',(-7.53094626422849,-3.88223396860557,
87.7346099646635));
#170099=CARTESIAN_POINT('Ctrl Pts',(-4.75851708790345,-7.00099837833069,
87.8932774299501));
#170100=CARTESIAN_POINT('Ctrl Pts',(-0.838343829035965,-8.43113704348407,
88.0519448952363));
#170101=CARTESIAN_POINT('Ctrl Pts',(3.30861330952905,-7.79810799993996,
88.2106123605229));
#170102=CARTESIAN_POINT('Ctrl Pts',(6.60661632725936,-5.27923024708605,
88.3692798258093));
#170103=CARTESIAN_POINT('Ctrl Pts',(7.98907354300744,-2.28814380995307,
88.4935081867057));
#170104=CARTESIAN_POINT('Ctrl Pts',(8.13073112681308,-0.470635535525396,
88.5648473925067));
#170105=CARTESIAN_POINT('Ctrl Pts',(8.12607929659711,-0.000602397288300138,
88.5832974432122));
#170106=CARTESIAN_POINT('',(8.12524838875447,-0.00511698572615098,90.5832974432122));
#170107=CARTESIAN_POINT('Ctrl Pts',(8.12524997767401,-0.000602335809762239,
88.5832974432122));
#170108=CARTESIAN_POINT('Ctrl Pts',(8.12526495996985,0.201502365521601,
88.5912314058029));
#170109=CARTESIAN_POINT('Ctrl Pts',(8.11773499501211,0.403761566827383,
88.5991653683936));
#170110=CARTESIAN_POINT('Ctrl Pts',(8.1026516106303,0.605577773081411,88.6070993309843));
#170111=CARTESIAN_POINT('Ctrl Pts',(8.08757794812149,0.80726390033737,88.6150281798037));
#170112=CARTESIAN_POINT('Ctrl Pts',(8.06496059500274,1.00850727033384,88.6229570286232));
#170113=CARTESIAN_POINT('Ctrl Pts',(8.0348431432226,1.20871139082447,88.6308858774427));
#170114=CARTESIAN_POINT('Ctrl Pts',(8.00474001668687,1.40882028503302,88.6388109549372));
#170115=CARTESIAN_POINT('Ctrl Pts',(7.96714395263145,1.60789058619621,88.6467360324317));
#170116=CARTESIAN_POINT('Ctrl Pts',(7.92215032532402,1.8053314890813,88.6546611099263));
#170117=CARTESIAN_POINT('Ctrl Pts',(7.87705752094983,2.00320760047877,88.6626036562489));
#170118=CARTESIAN_POINT('Ctrl Pts',(7.82453454514041,2.1994467879691,88.6705462025715));
#170119=CARTESIAN_POINT('Ctrl Pts',(7.76472901475924,2.39346420275216,88.6784887488941));
#170120=CARTESIAN_POINT('Ctrl Pts',(7.70507301351653,2.58699652432234,88.6864114368173));
#170121=CARTESIAN_POINT('Ctrl Pts',(7.63817094197432,2.77831785387582,88.6943341247405));
#170122=CARTESIAN_POINT('Ctrl Pts',(7.56421939868302,2.9668623916669,88.7022568126636));
#170123=CARTESIAN_POINT('Ctrl Pts',(7.49026357116724,3.1554178523825,88.7101799595708));
#170124=CARTESIAN_POINT('Ctrl Pts',(7.40925757941404,3.34119589022874,88.718103106478));
#170125=CARTESIAN_POINT('Ctrl Pts',(7.3214464610705,3.52364999399462,88.7260262533852));
#170126=CARTESIAN_POINT('Ctrl Pts',(7.23361680925743,3.7061426066377,88.7339510725567));
#170127=CARTESIAN_POINT('Ctrl Pts',(7.13897931252366,3.88530958647883,88.7418758917282));
#170128=CARTESIAN_POINT('Ctrl Pts',(7.03782549592002,4.06062801195555,88.7498007108997));
#170129=CARTESIAN_POINT('Ctrl Pts',(6.93626356518562,4.23665377531849,88.7577575034638));
#170130=CARTESIAN_POINT('Ctrl Pts',(6.82813278577759,4.40879956737382,88.7657142960279));
#170131=CARTESIAN_POINT('Ctrl Pts',(6.71377261423615,4.57656474299585,88.7736710885919));
#170132=CARTESIAN_POINT('Ctrl Pts',(6.5997274412337,4.74386781905558,88.7816059646268));
#170133=CARTESIAN_POINT('Ctrl Pts',(6.47948737991197,4.90681413481764,88.7895408406618));
#170134=CARTESIAN_POINT('Ctrl Pts',(6.35343012263957,5.0649396086465,88.7974757166967));
#170135=CARTESIAN_POINT('Ctrl Pts',(6.22685060058172,5.22372020831619,88.8054434675254));
#170136=CARTESIAN_POINT('Ctrl Pts',(6.09440579693078,5.37763967607004,88.813411218354));
#170137=CARTESIAN_POINT('Ctrl Pts',(5.95651623194406,5.52626473678984,88.8213789691827));
#170138=CARTESIAN_POINT('Ctrl Pts',(5.81862666695735,5.67488979750964,88.8293467200114));
#170139=CARTESIAN_POINT('Ctrl Pts',(5.67529260705918,5.81822024134434,88.83731447084));
#170140=CARTESIAN_POINT('Ctrl Pts',(5.52696893801207,5.95586281916816,88.8452822216686));
#170141=CARTESIAN_POINT('Ctrl Pts',(5.37659388168858,6.09540905966868,88.8533601703017));
#170142=CARTESIAN_POINT('Ctrl Pts',(5.22076204191132,6.229413831033,88.8614381189348));
#170143=CARTESIAN_POINT('Ctrl Pts',(5.0599057357018,6.35743985487177,88.8695160675679));
#170144=CARTESIAN_POINT('Ctrl Pts',(4.89924628494258,6.48530920085832,88.8775841304324));
#170145=CARTESIAN_POINT('Ctrl Pts',(4.73357486969886,6.60721418909075,88.8856521932968));
#170146=CARTESIAN_POINT('Ctrl Pts',(4.56335985174343,6.72275497292562,88.8937202561613));
#170147=CARTESIAN_POINT('Ctrl Pts',(4.39333218677518,6.83816858284098,88.9017794386362));
#170148=CARTESIAN_POINT('Ctrl Pts',(4.21877114854755,6.94723177676903,88.9098386211111));
#170149=CARTESIAN_POINT('Ctrl Pts',(4.04017779458328,7.04958516160037,88.917897803586));
#170150=CARTESIAN_POINT('Ctrl Pts',(3.86181383753915,7.15180707708683,88.9259466343227));
#170151=CARTESIAN_POINT('Ctrl Pts',(3.67942817004831,7.24733622083707,88.9339954650594));
#170152=CARTESIAN_POINT('Ctrl Pts',(3.49355044913783,7.33585665221376,88.9420442957961));
#170153=CARTESIAN_POINT('Ctrl Pts',(3.30781332529625,7.4243101271358,88.9500870384336));
#170154=CARTESIAN_POINT('Ctrl Pts',(3.11858969677777,7.50576532146182,88.958129781071));
#170155=CARTESIAN_POINT('Ctrl Pts',(2.92643461789832,7.57995171420414,88.9661725237085));
#170156=CARTESIAN_POINT('Ctrl Pts',(2.73443605656447,7.65407767933676,88.9742087152293));
#170157=CARTESIAN_POINT('Ctrl Pts',(2.5395111015908,7.72094653995816,88.9822449067502));
#170158=CARTESIAN_POINT('Ctrl Pts',(2.34223588471881,7.78033537984292,88.990281098271));
#170159=CARTESIAN_POINT('Ctrl Pts',(2.23038879936087,7.81400645494918,88.994837294499));
#170160=CARTESIAN_POINT('Ctrl Pts',(2.11778662314369,7.84527399401388,88.9993934907269));
#170161=CARTESIAN_POINT('Ctrl Pts',(2.00453702288502,7.8741043228029,89.0039496869549));
#170162=CARTESIAN_POINT('Ctrl Pts',(1.80478003041979,7.92495712720595,89.0119862014635));
#170163=CARTESIAN_POINT('Ctrl Pts',(1.60316595060972,7.96818418802857,89.0200227159722));
#170164=CARTESIAN_POINT('Ctrl Pts',(1.4003037910848,8.00367645867657,89.0280592304809));
#170165=CARTESIAN_POINT('Ctrl Pts',(1.19731908262425,8.03919017018866,89.0361005998442));
#170166=CARTESIAN_POINT('Ctrl Pts',(0.993085101348456,8.06695971503978,
89.0441419692075));
#170167=CARTESIAN_POINT('Ctrl Pts',(0.788217396409137,8.08692777873637,
89.0521833385708));
#170168=CARTESIAN_POINT('Ctrl Pts',(0.583200882053333,8.10691034660242,
89.0602305489303));
#170169=CARTESIAN_POINT('Ctrl Pts',(0.377550039657457,8.11908009699181,
89.0682777592898));
#170170=CARTESIAN_POINT('Ctrl Pts',(0.17188245807031,8.12343178608079,89.0763249696493));
#170171=CARTESIAN_POINT('Ctrl Pts',(-0.034088262845772,8.12778988924874,
89.0843840410223));
#170172=CARTESIAN_POINT('Ctrl Pts',(-0.240075456148502,8.12430689334256,
89.0924431123952));
#170173=CARTESIAN_POINT('Ctrl Pts',(-0.445462854899655,8.11302966883547,
89.1005021837682));
#170174=CARTESIAN_POINT('Ctrl Pts',(-0.651016483748779,8.10174331711734,
89.1085677777429));
#170175=CARTESIAN_POINT('Ctrl Pts',(-0.855969035467893,8.08265017736779,
89.1166333717177));
#170176=CARTESIAN_POINT('Ctrl Pts',(-1.05971152068651,8.05584874829613,
89.1246989656925));
#170177=CARTESIAN_POINT('Ctrl Pts',(-1.26377392815683,8.02900523485739,
89.1327772244926));
#170178=CARTESIAN_POINT('Ctrl Pts',(-1.46662216008448,7.99442929154823,
89.1408554832927));
#170179=CARTESIAN_POINT('Ctrl Pts',(-1.66765779420039,7.95227043327518,
89.1489337420928));
#170180=CARTESIAN_POINT('Ctrl Pts',(-1.78116629086201,7.92846674969148,
89.153494878809));
#170181=CARTESIAN_POINT('Ctrl Pts',(-1.89409721064808,7.90224658368573,
89.1580560155253));
#170182=CARTESIAN_POINT('Ctrl Pts',(-2.006345280416,7.87364376754832,89.1626171522415));
#170183=CARTESIAN_POINT('Ctrl Pts',(-2.20534384035217,7.82293537467142,
89.1707033459737));
#170184=CARTESIAN_POINT('Ctrl Pts',(-2.40258246267606,7.76463687978641,
89.1787895397059));
#170185=CARTESIAN_POINT('Ctrl Pts',(-2.59746170664314,7.69888824733951,
89.1868757334381));
#170186=CARTESIAN_POINT('Ctrl Pts',(-2.79216712757233,7.63319825955275,
89.1949547146692));
#170187=CARTESIAN_POINT('Ctrl Pts',(-2.98451706749501,7.56007148483361,
89.2030336959002));
#170188=CARTESIAN_POINT('Ctrl Pts',(-3.17392548419789,7.47969816124014,
89.2111126771313));
#170189=CARTESIAN_POINT('Ctrl Pts',(-3.36319082230855,7.39938555143222,
89.2191855555224));
#170190=CARTESIAN_POINT('Ctrl Pts',(-3.5495187775071,7.31183743171238,89.2272584339135));
#170191=CARTESIAN_POINT('Ctrl Pts',(-3.73234100480123,7.2172929957415,89.2353313123046));
#170192=CARTESIAN_POINT('Ctrl Pts',(-3.91505005696813,7.12280708700075,
89.2433991932233));
#170193=CARTESIAN_POINT('Ctrl Pts',(-4.09425742853882,7.02133364442052,
89.251467074142));
#170194=CARTESIAN_POINT('Ctrl Pts',(-4.26941663867616,6.9131591279165,89.2595349550606));
#170195=CARTESIAN_POINT('Ctrl Pts',(-4.4444912714021,6.80503684458125,89.2675989403207));
#170196=CARTESIAN_POINT('Ctrl Pts',(-4.61552137226379,6.69022010702722,
89.2756629255808));
#170197=CARTESIAN_POINT('Ctrl Pts',(-4.78198632770572,6.56904059388702,
89.2837269108408));
#170198=CARTESIAN_POINT('Ctrl Pts',(-4.95076461296472,6.44617707356212,
89.2919029596731));
#170199=CARTESIAN_POINT('Ctrl Pts',(-5.11484964076951,6.31677278271794,
89.3000790085053));
#170200=CARTESIAN_POINT('Ctrl Pts',(-5.27372942165282,6.18121877542717,
89.3082550573375));
#170201=CARTESIAN_POINT('Ctrl Pts',(-5.43035730136214,6.0475860587277,89.3163152219845));
#170202=CARTESIAN_POINT('Ctrl Pts',(-5.58192627019638,5.90797701751488,
89.3243753866314));
#170203=CARTESIAN_POINT('Ctrl Pts',(-5.72797903344587,5.76280693368297,
89.3324355512784));
#170204=CARTESIAN_POINT('Ctrl Pts',(-5.87402474015856,5.61764386374121,
89.3404953264986));
#170205=CARTESIAN_POINT('Ctrl Pts',(-6.01455454827871,5.46692051044645,
89.3485551017189));
#170206=CARTESIAN_POINT('Ctrl Pts',(-6.14914778483428,5.31108925577114,
89.3566148769391));
#170207=CARTESIAN_POINT('Ctrl Pts',(-6.28375118335059,5.15524623563768,
89.3646752606826));
#170208=CARTESIAN_POINT('Ctrl Pts',(-6.41241690972039,4.99429478505011,
89.3727356444262));
#170209=CARTESIAN_POINT('Ctrl Pts',(-6.53476398694848,4.82872107264244,
89.3807960281697));
#170210=CARTESIAN_POINT('Ctrl Pts',(-6.66018660805889,4.65898519118419,
89.3890590327234));
#170211=CARTESIAN_POINT('Ctrl Pts',(-6.77896852738852,4.48439189149325,
89.3973220372771));
#170212=CARTESIAN_POINT('Ctrl Pts',(-6.89074586973728,4.30549752307425,
89.4055850418309));
#170213=CARTESIAN_POINT('Ctrl Pts',(-6.99987193428575,4.13084639982123,
89.4136520538867));
#170214=CARTESIAN_POINT('Ctrl Pts',(-7.10232179584241,3.95209621931569,
89.4217190659425));
#170215=CARTESIAN_POINT('Ctrl Pts',(-7.19780274954632,3.76979086172209,
89.4297860779983));
#170216=CARTESIAN_POINT('Ctrl Pts',(-7.29676334673353,3.58084169062526,
89.4381470788009));
#170217=CARTESIAN_POINT('Ctrl Pts',(-7.38823738479246,3.38807368363205,
89.4465080796036));
#170218=CARTESIAN_POINT('Ctrl Pts',(-7.4719527634726,3.19211676837395,89.4548690804063));
#170219=CARTESIAN_POINT('Ctrl Pts',(-7.55566814215268,2.99615985311599,
89.4632300812089));
#170220=CARTESIAN_POINT('Ctrl Pts',(-7.63162474954995,2.7970143905052,89.4715910820116));
#170221=CARTESIAN_POINT('Ctrl Pts',(-7.69960716223356,2.59532986531225,
89.4799520828143));
#170222=CARTESIAN_POINT('Ctrl Pts',(-7.76122506893775,2.41252702312928,
89.4875303276438));
#170223=CARTESIAN_POINT('Ctrl Pts',(-7.81641525518899,2.22727186671854,
89.4951085724732));
#170224=CARTESIAN_POINT('Ctrl Pts',(-7.86497144648169,2.04007639771841,
89.5026868173026));
#170225=CARTESIAN_POINT('Ctrl Pts',(-7.913491505836,1.85302022578778,89.5102594229609));
#170226=CARTESIAN_POINT('Ctrl Pts',(-7.95538729909704,1.66402696692475,
89.5178320286192));
#170227=CARTESIAN_POINT('Ctrl Pts',(-7.99050135741784,1.47362668936324,
89.5254046342774));
#170228=CARTESIAN_POINT('Ctrl Pts',(-8.02559595451032,1.28333193715117,
89.5329730429782));
#170229=CARTESIAN_POINT('Ctrl Pts',(-8.05391622939255,1.09163207813576,
89.5405414516791));
#170230=CARTESIAN_POINT('Ctrl Pts',(-8.07535510965074,0.899070306226197,
89.5481098603799));
#170231=CARTESIAN_POINT('Ctrl Pts',(-8.09678881010417,0.706555058779329,
89.5556764404927));
#170232=CARTESIAN_POINT('Ctrl Pts',(-8.11134437658088,0.513178676856518,
89.5632430206055));
#170233=CARTESIAN_POINT('Ctrl Pts',(-8.11896619276522,0.319492602786696,
89.5708096007183));
#170234=CARTESIAN_POINT('Ctrl Pts',(-8.12658665687383,0.125840887750647,
89.5783748385541));
#170235=CARTESIAN_POINT('Ctrl Pts',(-8.12727580763376,-0.0681200425285449,
89.5859400763897));
#170236=CARTESIAN_POINT('Ctrl Pts',(-8.12103007872434,-0.261835870259456,
89.5935053142255));
#170237=CARTESIAN_POINT('Ctrl Pts',(-8.11478217787525,-0.455619062280116,
89.6010731828574));
#170238=CARTESIAN_POINT('Ctrl Pts',(-8.10159458808534,-0.64915661338977,
89.6086410514894));
#170239=CARTESIAN_POINT('Ctrl Pts',(-8.08151586847249,-0.841895973459506,
89.6162089201214));
#170240=CARTESIAN_POINT('Ctrl Pts',(-8.06169625401975,-1.03214813495714,
89.6236791294478));
#170241=CARTESIAN_POINT('Ctrl Pts',(-8.03516237914344,-1.22162224219535,
89.6311493387742));
#170242=CARTESIAN_POINT('Ctrl Pts',(-8.00201021732005,-1.40979432698729,
89.6386195481007));
#170243=CARTESIAN_POINT('Ctrl Pts',(-7.96071167427457,-1.64420537339614,
89.6479253895438));
#170244=CARTESIAN_POINT('Ctrl Pts',(-7.90916508289916,-1.8764811682522,
89.657231230987));
#170245=CARTESIAN_POINT('Ctrl Pts',(-7.8476229482722,-2.10582563956553,
89.6665370724301));
#170246=CARTESIAN_POINT('Ctrl Pts',(-7.78575040634027,-2.33640141507615,
89.6758928750586));
#170247=CARTESIAN_POINT('Ctrl Pts',(-7.71377476869098,-2.56401427705064,
89.685248677687));
#170248=CARTESIAN_POINT('Ctrl Pts',(-7.63199944735815,-2.78787948054159,
89.6946044803154));
#170249=CARTESIAN_POINT('Ctrl Pts',(-7.54982715139329,-3.01283142762868,
89.7040057002684));
#170250=CARTESIAN_POINT('Ctrl Pts',(-7.45775983349303,-3.23399921083646,
89.7134069202213));
#170251=CARTESIAN_POINT('Ctrl Pts',(-7.35615172633996,-3.45061144459437,
89.7228081401743));
#170252=CARTESIAN_POINT('Ctrl Pts',(-7.25443364906327,-3.66745811706775,
89.7322195350369));
#170253=CARTESIAN_POINT('Ctrl Pts',(-7.14315415404235,-3.87973934917524,
89.7416309298996));
#170254=CARTESIAN_POINT('Ctrl Pts',(-7.02271441312066,-4.08670647762319,
89.7510423247623));
#170255=CARTESIAN_POINT('Ctrl Pts',(-6.90241595003536,-4.29343083015775,
89.760442679901));
#170256=CARTESIAN_POINT('Ctrl Pts',(-6.77297874069724,-4.49485350946098,
89.7698430350397));
#170257=CARTESIAN_POINT('Ctrl Pts',(-6.63484775525196,-4.69025402586342,
89.7792433901783));
#170258=CARTESIAN_POINT('Ctrl Pts',(-6.54646870225914,-4.81527530576154,
89.785257931248));
#170259=CARTESIAN_POINT('Ctrl Pts',(-6.45453158198816,-4.93783180441181,
89.7912724723176));
#170260=CARTESIAN_POINT('Ctrl Pts',(-6.35916264071753,-5.05774041162676,
89.7972870133872));
#170261=CARTESIAN_POINT('Ctrl Pts',(-6.23639769419285,-5.21209437169454,
89.8050293119065));
#170262=CARTESIAN_POINT('Ctrl Pts',(-6.10788593933289,-5.36213122049771,
89.8127716104258));
#170263=CARTESIAN_POINT('Ctrl Pts',(-5.97396991466535,-5.50739239760281,
89.8205139089451));
#170264=CARTESIAN_POINT('Ctrl Pts',(-5.84013730755455,-5.65256309014855,
89.8282513847135));
#170265=CARTESIAN_POINT('Ctrl Pts',(-5.70090737190607,-5.79296377552294,
89.8359888604819));
#170266=CARTESIAN_POINT('Ctrl Pts',(-5.55666336760916,-5.92816833276269,
89.8437263362503));
#170267=CARTESIAN_POINT('Ctrl Pts',(-5.41248357795749,-6.06331269954447,
89.8514603674439));
#170268=CARTESIAN_POINT('Ctrl Pts',(-5.26329442247845,-6.19326530414008,
89.8591943986375));
#170269=CARTESIAN_POINT('Ctrl Pts',(-5.10951661184736,-6.31763623167367,
89.8669284298311));
#170270=CARTESIAN_POINT('Ctrl Pts',(-4.95575847993428,-6.4419912436444,
89.8746614713122));
#170271=CARTESIAN_POINT('Ctrl Pts',(-4.79741313216581,-6.5607657732854,
89.8823945127933));
#170272=CARTESIAN_POINT('Ctrl Pts',(-4.63493529650067,-6.67360939520379,
89.8901275542745));
#170273=CARTESIAN_POINT('Ctrl Pts',(-4.47247369224984,-6.78644174412871,
89.8978598232305));
#170274=CARTESIAN_POINT('Ctrl Pts',(-4.30588071473477,-6.89334416688666,
89.9055920921866));
#170275=CARTESIAN_POINT('Ctrl Pts',(-4.13564097227291,-6.99400895845563,
89.9133243611426));
#170276=CARTESIAN_POINT('Ctrl Pts',(-3.96533574632521,-7.09471247119134,
89.9210596043509));
#170277=CARTESIAN_POINT('Ctrl Pts',(-3.79138125728361,-7.18917337900908,
89.9287948475591));
#170278=CARTESIAN_POINT('Ctrl Pts',(-3.61428823618453,-7.27712911169495,
89.9365300907673));
#170279=CARTESIAN_POINT('Ctrl Pts',(-3.46605227924917,-7.35075257873911,
89.943004886736));
#170280=CARTESIAN_POINT('Ctrl Pts',(-3.31561783853691,-7.41981892123465,
89.9494796827047));
#170281=CARTESIAN_POINT('Ctrl Pts',(-3.16329578184691,-7.48419984761561,
89.9559544786735));
#170282=CARTESIAN_POINT('Ctrl Pts',(-2.96535145435842,-7.56786362850521,
89.9643685531779));
#170283=CARTESIAN_POINT('Ctrl Pts',(-2.76412378459261,-7.64365462963771,
89.9727826276823));
#170284=CARTESIAN_POINT('Ctrl Pts',(-2.56024420095133,-7.71134470724757,
89.9811967021867));
#170285=CARTESIAN_POINT('Ctrl Pts',(-2.35630767935196,-7.77905368883365,
89.9896131265106));
#170286=CARTESIAN_POINT('Ctrl Pts',(-2.14971801597115,-7.83865714726906,
89.9980295508345));
#170287=CARTESIAN_POINT('Ctrl Pts',(-1.94112231701676,-7.8899766611112,
90.0064459751584));
#170288=CARTESIAN_POINT('Ctrl Pts',(-1.7324748877817,-7.94130890183539,
90.0148644866969));
#170289=CARTESIAN_POINT('Ctrl Pts',(-1.5218206860995,-7.98435303358087,
90.0232829982354));
#170290=CARTESIAN_POINT('Ctrl Pts',(-1.30981861315874,-8.01898140433827,
90.0317015097739));
#170291=CARTESIAN_POINT('Ctrl Pts',(-1.0977351111085,-8.05362307570802,
90.0401232548275));
#170292=CARTESIAN_POINT('Ctrl Pts',(-0.88430296362602,-8.07984248270811,
90.0485449998811));
#170293=CARTESIAN_POINT('Ctrl Pts',(-0.670189252137193,-8.0975634563009,
90.0569667449347));
#170294=CARTESIAN_POINT('Ctrl Pts',(-0.456052331306254,-8.11528635079887,
90.0653894028824));
#170295=CARTESIAN_POINT('Ctrl Pts',(-0.241233962254784,-8.12450895384322,
90.0738120608302));
#170296=CARTESIAN_POINT('Ctrl Pts',(-0.0264049238957141,-8.12520709536034,
90.082234718778));
#170297=CARTESIAN_POINT('Ctrl Pts',(0.188464968764381,-8.12590536964389,
90.0906589784729));
#170298=CARTESIAN_POINT('Ctrl Pts',(0.403345270857372,-8.11807594302261,
90.0990832381678));
#170299=CARTESIAN_POINT('Ctrl Pts',(0.617565297220088,-8.10174676635659,
90.1075074978628));
#170300=CARTESIAN_POINT('Ctrl Pts',(0.67786958055097,-8.09715000053153,
90.1098789798952));
#170301=CARTESIAN_POINT('Ctrl Pts',(0.738121556086772,-8.09187998194235,
90.1122504619276));
#170302=CARTESIAN_POINT('Ctrl Pts',(0.798306313214766,-8.08593807747632,
90.1146219439599));
#170303=CARTESIAN_POINT('Ctrl Pts',(1.01210340735999,-8.0648303756404,90.1230462691801));
#170304=CARTESIAN_POINT('Ctrl Pts',(1.22507388350962,-8.03523788305068,
90.1314705944002));
#170305=CARTESIAN_POINT('Ctrl Pts',(1.43655248997595,-7.9972498089058,90.1398949196204));
#170306=CARTESIAN_POINT('Ctrl Pts',(1.64799455035247,-7.95926829956477,
90.1483177890141));
#170307=CARTESIAN_POINT('Ctrl Pts',(1.85794499633917,-7.91289415311656,
90.1567406584078));
#170308=CARTESIAN_POINT('Ctrl Pts',(2.06574754580753,-7.85826791599079,
90.1651635278016));
#170309=CARTESIAN_POINT('Ctrl Pts',(2.27350763047813,-7.80365284182772,
90.1735846759679));
#170310=CARTESIAN_POINT('Ctrl Pts',(2.47912044003013,-7.7407891115347,90.1820058241342));
#170311=CARTESIAN_POINT('Ctrl Pts',(2.68194259170222,-7.66986776270058,
90.1904269723005));
#170312=CARTESIAN_POINT('Ctrl Pts',(2.88470783832014,-7.59896631200462,
90.1988457577767));
#170313=CARTESIAN_POINT('Ctrl Pts',(3.0846837418909,-7.5200118450343,90.2072645432528));
#170314=CARTESIAN_POINT('Ctrl Pts',(3.28124375652037,-7.4332447136359,90.215683328729));
#170315=CARTESIAN_POINT('Ctrl Pts',(3.4777488634247,-7.34650182005521,90.2240997624738));
#170316=CARTESIAN_POINT('Ctrl Pts',(3.67083974529905,-7.25195072597193,
90.2325161962186));
#170317=CARTESIAN_POINT('Ctrl Pts',(3.85991038308934,-7.1498796771008,90.2409326299634));
#170318=CARTESIAN_POINT('Ctrl Pts',(4.04891239923137,-7.04784567408563,
90.2493460090321));
#170319=CARTESIAN_POINT('Ctrl Pts',(4.23389685306091,-6.93829729192304,
90.2577593881008));
#170320=CARTESIAN_POINT('Ctrl Pts',(4.41428197581336,-6.82156889582663,
90.2661727671695));
#170321=CARTESIAN_POINT('Ctrl Pts',(4.46514288612388,-6.78865646716311,
90.2685449811952));
#170322=CARTESIAN_POINT('Ctrl Pts',(4.51563830569596,-6.75517350489252,
90.2709171952209));
#170323=CARTESIAN_POINT('Ctrl Pts',(4.56575557235752,-6.72112815054037,
90.2732894092466));
#170324=CARTESIAN_POINT('Ctrl Pts',(4.72917519665905,-6.61011493317934,
90.2810245941572));
#170325=CARTESIAN_POINT('Ctrl Pts',(4.8886444317497,-6.49306945181757,90.2887597790678));
#170326=CARTESIAN_POINT('Ctrl Pts',(5.0436885650882,-6.37031343191986,90.2964949639785));
#170327=CARTESIAN_POINT('Ctrl Pts',(5.19868475495004,-6.24759537121639,
90.3042277569788));
#170328=CARTESIAN_POINT('Ctrl Pts',(5.34925829135822,-6.11917050754268,
90.3119605499792));
#170329=CARTESIAN_POINT('Ctrl Pts',(5.49496532201888,-5.98540254889426,
90.3196933429795));
#170330=CARTESIAN_POINT('Ctrl Pts',(5.64065318438487,-5.85165218791176,
90.3274251187026));
#170331=CARTESIAN_POINT('Ctrl Pts',(5.78147555653655,-5.7125603714665,90.3351568944257));
#170332=CARTESIAN_POINT('Ctrl Pts',(5.91702332769113,-5.56852965351348,
90.3428886701488));
#170333=CARTESIAN_POINT('Ctrl Pts',(6.05261960154003,-5.42444739743612,
90.3506232125123));
#170334=CARTESIAN_POINT('Ctrl Pts',(6.18293725807404,-5.27542296363728,
90.3583577548759));
#170335=CARTESIAN_POINT('Ctrl Pts',(6.30760514129895,-5.12189466349701,
90.3660922972394));
#170336=CARTESIAN_POINT('Ctrl Pts',(6.43229407953972,-4.96834043413813,
90.373828145881));
#170337=CARTESIAN_POINT('Ctrl Pts',(6.55133112635587,-4.81028110195774,
90.3815639945225));
#170338=CARTESIAN_POINT('Ctrl Pts',(6.66438671824976,-4.64818644549853,
90.3892998431641));
#170339=CARTESIAN_POINT('Ctrl Pts',(6.77753481734768,-4.48595915585234,
90.3970420216272));
#170340=CARTESIAN_POINT('Ctrl Pts',(6.88469148693914,-4.31969023923898,
90.4047842000904));
#170341=CARTESIAN_POINT('Ctrl Pts',(6.98557114769636,-4.14987750457434,
90.4125263785536));
#170342=CARTESIAN_POINT('Ctrl Pts',(7.06996349506373,-4.00781819168956,
90.4190032105467));
#170343=CARTESIAN_POINT('Ctrl Pts',(7.14996368609586,-3.86327933956513,
90.4254800425397));
#170344=CARTESIAN_POINT('Ctrl Pts',(7.22542984209037,-3.71656442962179,
90.4319568745328));
#170345=CARTESIAN_POINT('Ctrl Pts',(7.33517417439504,-3.50320879200267,
90.4413756079129));
#170346=CARTESIAN_POINT('Ctrl Pts',(7.43539163973831,-3.28513213101952,
90.4507943412929));
#170347=CARTESIAN_POINT('Ctrl Pts',(7.52575430349025,-3.06312091272904,
90.460213074673));
#170348=CARTESIAN_POINT('Ctrl Pts',(7.61625700988186,-2.84076562493291,
90.4696464050584));
#170349=CARTESIAN_POINT('Ctrl Pts',(7.69687434893898,-2.61446360933155,
90.4790797354438));
#170350=CARTESIAN_POINT('Ctrl Pts',(7.76732641855281,-2.38502156597202,
90.4885130658292));
#170351=CARTESIAN_POINT('Ctrl Pts',(7.83768238437844,-2.15589250489473,
90.4979335281926));
#170352=CARTESIAN_POINT('Ctrl Pts',(7.89790079023532,-1.92363200655743,
90.5073539905559));
#170353=CARTESIAN_POINT('Ctrl Pts',(7.9477522333787,-1.68905950141607,90.5167744529193));
#170354=CARTESIAN_POINT('Ctrl Pts',(7.99747776005718,-1.45507948745949,
90.5261711207595));
#170355=CARTESIAN_POINT('Ctrl Pts',(8.03688860001431,-1.21879915749754,
90.5355677885996));
#170356=CARTESIAN_POINT('Ctrl Pts',(8.06580645547962,-0.981047290013701,
90.5449644564398));
#170357=CARTESIAN_POINT('Ctrl Pts',(8.0945474977085,-0.744749115291,90.5543036699762));
#170358=CARTESIAN_POINT('Ctrl Pts',(8.1129234469417,-0.506997377249942,
90.5636428835126));
#170359=CARTESIAN_POINT('Ctrl Pts',(8.12080848834577,-0.268620658385211,
90.572982097049));
#170360=CARTESIAN_POINT('Ctrl Pts',(8.12371154976798,-0.180856723990185,
90.5764205457701));
#170361=CARTESIAN_POINT('Ctrl Pts',(8.1251930380562,-0.0930082162133875,
90.5798589944911));
#170362=CARTESIAN_POINT('Ctrl Pts',(8.12524838875447,-0.00511698572615098,
90.5832974432122));
#170363=CARTESIAN_POINT('',(8.12456002707784,-1.23182048087155E-6,94.5833205544621));
#170364=CARTESIAN_POINT('Ctrl Pts',(8.12524954479919,-0.0027197868477638,
90.5813566725845));
#170365=CARTESIAN_POINT('Ctrl Pts',(8.1253341132248,0.249924850446765,90.5913649253526));
#170366=CARTESIAN_POINT('Ctrl Pts',(8.11363502343688,0.502437433370498,
90.601402458627));
#170367=CARTESIAN_POINT('Ctrl Pts',(8.03690933001179,1.32569002632119,90.6346645596573));
#170368=CARTESIAN_POINT('Ctrl Pts',(7.923182466773,1.89009932151999,90.6585382981442));
#170369=CARTESIAN_POINT('Ctrl Pts',(7.6411133025716,2.78694483841881,90.6983243100367));
#170370=CARTESIAN_POINT('Ctrl Pts',(7.50782069243921,3.12830785446595,90.7138877135595));
#170371=CARTESIAN_POINT('Ctrl Pts',(7.29973112944332,3.57052705183164,90.7339426923139));
#170372=CARTESIAN_POINT('Ctrl Pts',(7.24498821827151,3.68033766262184,90.7389102610915));
#170373=CARTESIAN_POINT('Ctrl Pts',(7.17962776501885,3.80433150999515,90.7444728201965));
#170374=CARTESIAN_POINT('Ctrl Pts',(7.17142719911711,3.81976766514242,90.7451644655121));
#170375=CARTESIAN_POINT('Ctrl Pts',(7.15896184904297,3.84304990214713,90.7462062567885));
#170376=CARTESIAN_POINT('Ctrl Pts',(7.15473386303412,3.85091556079698,90.7465579706063));
#170377=CARTESIAN_POINT('Ctrl Pts',(7.14711772963658,3.86502861957716,90.7471885769062));
#170378=CARTESIAN_POINT('Ctrl Pts',(7.14373433955709,3.87127856885769,90.7474676774264));
#170379=CARTESIAN_POINT('Ctrl Pts',(7.13696424036494,3.88374550075098,90.7480240693077));
#170380=CARTESIAN_POINT('Ctrl Pts',(7.13357759750108,3.88996251185891,90.7483013632416));
#170381=CARTESIAN_POINT('Ctrl Pts',(7.12413718504379,3.90723890858877,90.7490714495883));
#170382=CARTESIAN_POINT('Ctrl Pts',(7.11806577763847,3.91828867079501,90.7495634354094));
#170383=CARTESIAN_POINT('Ctrl Pts',(7.09380107622702,3.96220711141761,90.7515165500079));
#170384=CARTESIAN_POINT('Ctrl Pts',(7.07540544518844,3.99496392408681,90.7529680782763));
#170385=CARTESIAN_POINT('Ctrl Pts',(6.76178965406594,4.54445315268577,90.777213370273));
#170386=CARTESIAN_POINT('Ctrl Pts',(6.41088085549522,5.02738108313936,90.7969013446664));
#170387=CARTESIAN_POINT('Ctrl Pts',(5.88196255633283,5.6087974189636,90.8231089847327));
#170388=CARTESIAN_POINT('Ctrl Pts',(5.74863875813143,5.7453671278114,90.8294731843692));
#170389=CARTESIAN_POINT('Ctrl Pts',(5.56641321698683,5.91933010160226,90.8379905597227));
#170390=CARTESIAN_POINT('Ctrl Pts',(5.52171914664393,5.96104374585259,90.8400658609274));
#170391=CARTESIAN_POINT('Ctrl Pts',(5.41051971561242,6.06250408925557,90.8452025798158));
#170392=CARTESIAN_POINT('Ctrl Pts',(5.34349136499075,6.1216647359328,90.8482760030133));
#170393=CARTESIAN_POINT('Ctrl Pts',(4.97394466046285,6.43713991054958,90.8651409216937));
#170394=CARTESIAN_POINT('Ctrl Pts',(4.65397725346166,6.67213241189768,90.8794910127026));
#170395=CARTESIAN_POINT('Ctrl Pts',(4.29349658268906,6.89829123204522,90.8958772392701));
#170396=CARTESIAN_POINT('Ctrl Pts',(4.2687568338003,6.91362783932175,90.8970026878825));
#170397=CARTESIAN_POINT('Ctrl Pts',(4.23279002248889,6.93565764787437,90.8986402446615));
#170398=CARTESIAN_POINT('Ctrl Pts',(4.22162826115478,6.94245728872055,90.8991486260085));
#170399=CARTESIAN_POINT('Ctrl Pts',(4.20211435843275,6.95428051455824,90.9000377633864));
#170400=CARTESIAN_POINT('Ctrl Pts',(4.19376948038085,6.95931606561452,90.9004181012211));
#170401=CARTESIAN_POINT('Ctrl Pts',(4.17762406492428,6.96901911092718,90.9011541834696));
#170402=CARTESIAN_POINT('Ctrl Pts',(4.16982471262103,6.97368855496806,90.9015098593127));
#170403=CARTESIAN_POINT('Ctrl Pts',(4.15130418282547,6.98473455102278,90.9023546910264));
#170404=CARTESIAN_POINT('Ctrl Pts',(4.14057613918752,6.99109951298861,90.9028442476185));
#170405=CARTESIAN_POINT('Ctrl Pts',(4.10276776302586,7.01341371716648,90.9045702439637));
#170406=CARTESIAN_POINT('Ctrl Pts',(4.07560975381132,7.0292304267962,90.9058112527841));
#170407=CARTESIAN_POINT('Ctrl Pts',(3.68832818576379,7.25178262342136,90.9235265820499));
#170408=CARTESIAN_POINT('Ctrl Pts',(3.31300405911257,7.43075094818757,90.9409603055985));
#170409=CARTESIAN_POINT('Ctrl Pts',(2.68939320859586,7.6714405464906,90.9701381901769));
#170410=CARTESIAN_POINT('Ctrl Pts',(2.4489789701589,7.75153729684824,90.9814236896893));
#170411=CARTESIAN_POINT('Ctrl Pts',(1.82282870582047,7.92810425647376,91.0106025659424));
#170412=CARTESIAN_POINT('Ctrl Pts',(1.4330313100301,8.00774480003751,91.0285780583772));
#170413=CARTESIAN_POINT('Ctrl Pts',(0.818017106523038,8.08703690328912,
91.0554835865656));
#170414=CARTESIAN_POINT('Ctrl Pts',(0.595965502406689,8.10642737210059,
91.0648991635527));
#170415=CARTESIAN_POINT('Ctrl Pts',(0.333886051134797,8.11848324648465,
91.0754779988639));
#170416=CARTESIAN_POINT('Ctrl Pts',(0.294385398168833,8.12001154150007,
91.0770590146964));
#170417=CARTESIAN_POINT('Ctrl Pts',(0.242161967235993,8.12165050444959,
91.0791331229897));
#170418=CARTESIAN_POINT('Ctrl Pts',(0.229448284910972,8.12201962702541,
91.0796367964425));
#170419=CARTESIAN_POINT('Ctrl Pts',(0.208609968997774,8.1225756682221,91.0804603351901));
#170420=CARTESIAN_POINT('Ctrl Pts',(0.200485857461575,8.12278025227411,
91.080780903893));
#170421=CARTESIAN_POINT('Ctrl Pts',(0.184767936849336,8.12315247090342,
91.0814001699404));
#170422=CARTESIAN_POINT('Ctrl Pts',(0.177174175211805,8.12332164623336,
91.0816989272464));
#170423=CARTESIAN_POINT('Ctrl Pts',(0.159674154426438,8.12368696460186,
91.0823864562268));
#170424=CARTESIAN_POINT('Ctrl Pts',(0.149767740436123,8.12387563662988,
91.0827749402045));
#170425=CARTESIAN_POINT('Ctrl Pts',(0.123248142462953,8.12433218954174,
91.0838130596602));
#170426=CARTESIAN_POINT('Ctrl Pts',(0.106634393732977,8.12456723411067,
91.0844614601777));
#170427=CARTESIAN_POINT('Ctrl Pts',(-0.0108860505627611,8.12586932771147,
91.0890348644747));
#170428=CARTESIAN_POINT('Ctrl Pts',(-0.111806535856592,8.12510744923939,
91.0928936366302));
#170429=CARTESIAN_POINT('Ctrl Pts',(-0.64119356635003,8.11124532021173,
91.1128751751197));
#170430=CARTESIAN_POINT('Ctrl Pts',(-1.06815865345377,8.06613295571054,
91.1281347079424));
#170431=CARTESIAN_POINT('Ctrl Pts',(-1.84031498679005,7.92213471002392,
91.1563404114849));
#170432=CARTESIAN_POINT('Ctrl Pts',(-2.18634734641192,7.83369991186894,
91.1692088331408));
#170433=CARTESIAN_POINT('Ctrl Pts',(-2.69013315855809,7.66895655640531,
91.1888719604313));
#170434=CARTESIAN_POINT('Ctrl Pts',(-2.85305578072236,7.60984767735848,
91.1953769434026));
#170435=CARTESIAN_POINT('Ctrl Pts',(-3.08317118977262,7.51793171080848,
91.2048037533707));
#170436=CARTESIAN_POINT('Ctrl Pts',(-3.15199680286343,7.48933627062847,
91.2076543303865));
#170437=CARTESIAN_POINT('Ctrl Pts',(-3.2575354271195,7.44377490920035,91.212074602061));
#170438=CARTESIAN_POINT('Ctrl Pts',(-3.29453182469556,7.42747480553381,
91.2136335409408));
#170439=CARTESIAN_POINT('Ctrl Pts',(-3.36353660675089,7.39645524135656,
91.2165589622938));
#170440=CARTESIAN_POINT('Ctrl Pts',(-3.39557393805853,7.38180237179491,
91.2179243841977));
#170441=CARTESIAN_POINT('Ctrl Pts',(-3.44834687085139,7.35724944072377,
91.2201854817549));
#170442=CARTESIAN_POINT('Ctrl Pts',(-3.46913763854652,7.34746891894946,
91.2210793586516));
#170443=CARTESIAN_POINT('Ctrl Pts',(-3.50843813325239,7.32877694025304,
91.2227748660566));
#170444=CARTESIAN_POINT('Ctrl Pts',(-3.5269561221458,7.31988320157539,91.2235762242921));
#170445=CARTESIAN_POINT('Ctrl Pts',(-3.56941977876788,7.29929039433775,
91.2254195735402));
#170446=CARTESIAN_POINT('Ctrl Pts',(-3.59334198911172,7.28754356143387,
91.2264622669463));
#170447=CARTESIAN_POINT('Ctrl Pts',(-3.65313981859911,7.2578142325221,91.2290796013047));
#170448=CARTESIAN_POINT('Ctrl Pts',(-3.68894072808748,7.23968329735795,
91.2306565193586));
#170449=CARTESIAN_POINT('Ctrl Pts',(-3.88681141199762,7.1376252875052,91.2394295100787));
#170450=CARTESIAN_POINT('Ctrl Pts',(-4.04614832779095,7.04852315424849,
91.2467105089181));
#170451=CARTESIAN_POINT('Ctrl Pts',(-4.32313510540156,6.88114147954904,
91.259800936259));
#170452=CARTESIAN_POINT('Ctrl Pts',(-4.44199908466109,6.80501638750348,
91.2655671268226));
#170453=CARTESIAN_POINT('Ctrl Pts',(-4.98763161991512,6.43518284315647,
91.2927535891892));
#170454=CARTESIAN_POINT('Ctrl Pts',(-5.38765580249604,6.10419280896148,
91.3148942899855));
#170455=CARTESIAN_POINT('Ctrl Pts',(-5.95303918576735,5.53723117401015,
91.3487087082865));
#170456=CARTESIAN_POINT('Ctrl Pts',(-6.14208203793715,5.32676682290274,
91.3605217508587));
#170457=CARTESIAN_POINT('Ctrl Pts',(-6.34646443358242,5.07384271983327,
91.3735915124818));
#170458=CARTESIAN_POINT('Ctrl Pts',(-6.37289479636829,5.04060539442343,
91.3752877177737));
#170459=CARTESIAN_POINT('Ctrl Pts',(-6.40711216186561,4.99687621269705,
91.3774901961565));
#170460=CARTESIAN_POINT('Ctrl Pts',(-6.41513588741348,4.98657093483233,
91.3780071383945));
#170461=CARTESIAN_POINT('Ctrl Pts',(-6.42815828890906,4.96976215281186,
91.3788468538617));
#170462=CARTESIAN_POINT('Ctrl Pts',(-6.43317200934207,4.96327036757074,
91.3791703266778));
#170463=CARTESIAN_POINT('Ctrl Pts',(-6.44279314792255,4.95077380827444,
91.3797913822087));
#170464=CARTESIAN_POINT('Ctrl Pts',(-6.4474020217203,4.94477016841105,91.3800890338399));
#170465=CARTESIAN_POINT('Ctrl Pts',(-6.4579190241183,4.93103074298908,91.3807685597568));
#170466=CARTESIAN_POINT('Ctrl Pts',(-6.46382166067951,4.92329075419443,
91.3811501691239));
#170467=CARTESIAN_POINT('Ctrl Pts',(-6.48227733611666,4.89899985810939,
91.3823440114544));
#170468=CARTESIAN_POINT('Ctrl Pts',(-6.49478088218957,4.88241132789941,
91.383153805399));
#170469=CARTESIAN_POINT('Ctrl Pts',(-6.62712103369093,4.70542686153701,
91.391733818094));
#170470=CARTESIAN_POINT('Ctrl Pts',(-6.74104921686855,4.54070806477395,
91.3991622497739));
#170471=CARTESIAN_POINT('Ctrl Pts',(-6.94599881146518,4.21964855671273,
91.4128307301745));
#170472=CARTESIAN_POINT('Ctrl Pts',(-7.03811393101973,4.0641468313091,91.4191209705052));
#170473=CARTESIAN_POINT('Ctrl Pts',(-7.31974076196958,3.55038921999287,
91.4391995539626));
#170474=CARTESIAN_POINT('Ctrl Pts',(-7.48766202856566,3.18100523807409,
91.4525869982833));
#170475=CARTESIAN_POINT('Ctrl Pts',(-7.8113688031447,2.29941257463875,91.4845536024729));
#170476=CARTESIAN_POINT('Ctrl Pts',(-7.94553825019126,1.78132736166615,
91.5034123938262));
#170477=CARTESIAN_POINT('Ctrl Pts',(-8.03227314349433,1.22599775034216,
91.5250659142335));
#170478=CARTESIAN_POINT('Ctrl Pts',(-8.03647854079838,1.19812143791007,
91.5261563057583));
#170479=CARTESIAN_POINT('Ctrl Pts',(-8.04239660847886,1.15745874951914,
91.5277519654002));
#170480=CARTESIAN_POINT('Ctrl Pts',(-8.04422405753139,1.14468916100396,
91.5282537969874));
#170481=CARTESIAN_POINT('Ctrl Pts',(-8.04737502680251,1.12229104960988,
91.5291353216633));
#170482=CARTESIAN_POINT('Ctrl Pts',(-8.04871169693577,1.1126643882335,91.5295146205276));
#170483=CARTESIAN_POINT('Ctrl Pts',(-8.05127150739504,1.09398270830026,
91.5302515182297));
#170484=CARTESIAN_POINT('Ctrl Pts',(-8.05249665243197,1.0849279763153,91.5306090565012));
#170485=CARTESIAN_POINT('Ctrl Pts',(-8.05538192712531,1.06332952168318,
91.5314628001086));
#170486=CARTESIAN_POINT('Ctrl Pts',(-8.05702803245808,1.05078396732294,
91.5319594239335));
#170487=CARTESIAN_POINT('Ctrl Pts',(-8.06279626181468,1.00601170750454,
91.5337343630535));
#170488=CARTESIAN_POINT('Ctrl Pts',(-8.06675436645838,0.973764384603706,
91.5350175726263));
#170489=CARTESIAN_POINT('Ctrl Pts',(-8.12948602377688,0.436026697749313,
91.5564970888526));
#170490=CARTESIAN_POINT('Ctrl Pts',(-8.14082950635848,-0.073797495358503,
91.5781562497802));
#170491=CARTESIAN_POINT('Ctrl Pts',(-8.06252297267184,-1.16557713196623,
91.6266813471057));
#170492=CARTESIAN_POINT('Ctrl Pts',(-7.95755304790733,-1.7436107081773,
91.6537035798851));
#170493=CARTESIAN_POINT('Ctrl Pts',(-7.72560158084465,-2.52754297635896,
91.6892723634112));
#170494=CARTESIAN_POINT('Ctrl Pts',(-7.65036684972993,-2.74687102487199,
91.6990816593317));
#170495=CARTESIAN_POINT('Ctrl Pts',(-7.5516070841766,-2.99907382888776,
91.7099854572502));
#170496=CARTESIAN_POINT('Ctrl Pts',(-7.53710173690985,-3.03534361676441,
91.7115446732268));
#170497=CARTESIAN_POINT('Ctrl Pts',(-7.51768119451012,-3.08290586865181,
91.7135793601409));
#170498=CARTESIAN_POINT('Ctrl Pts',(-7.51300125579147,-3.0942933393667,
91.7140657532789));
#170499=CARTESIAN_POINT('Ctrl Pts',(-7.50531299545572,-3.11288054495593,
91.7148584977897));
#170500=CARTESIAN_POINT('Ctrl Pts',(-7.50232016371644,-3.12008663478886,
91.7151655494323));
#170501=CARTESIAN_POINT('Ctrl Pts',(-7.49652701492568,-3.13397875252599,
91.7157569564762));
#170502=CARTESIAN_POINT('Ctrl Pts',(-7.49372812287789,-3.14066536384142,
91.7160413748296));
#170503=CARTESIAN_POINT('Ctrl Pts',(-7.48728185381759,-3.15600795831578,
91.7166934469854));
#170504=CARTESIAN_POINT('Ctrl Pts',(-7.48362840351823,-3.16466138954361,
91.7170608346469));
#170505=CARTESIAN_POINT('Ctrl Pts',(-7.47386126591454,-3.18768398514423,
91.7180372839942));
#170506=CARTESIAN_POINT('Ctrl Pts',(-7.46772113004175,-3.20204193280439,
91.7186452126462));
#170507=CARTESIAN_POINT('Ctrl Pts',(-7.42538910388895,-3.30024608741469,
91.722796758154));
#170508=CARTESIAN_POINT('Ctrl Pts',(-7.38782645017924,-3.38349651198322,
91.726283677079));
#170509=CARTESIAN_POINT('Ctrl Pts',(-7.12269210387363,-3.94563797392302,
91.7497124355835));
#170510=CARTESIAN_POINT('Ctrl Pts',(-6.85011003083093,-4.40191613374934,
91.7682702312719));
#170511=CARTESIAN_POINT('Ctrl Pts',(-6.12207756105125,-5.38727133836705,
91.8123767689571));
#170512=CARTESIAN_POINT('Ctrl Pts',(-5.63919419628615,-5.89083258509883,
91.838322286557));
#170513=CARTESIAN_POINT('Ctrl Pts',(-5.00687095493669,-6.40036604197319,
91.8696914453421));
#170514=CARTESIAN_POINT('Ctrl Pts',(-4.91396794029383,-6.47196731844397,
91.8742385876345));
#170515=CARTESIAN_POINT('Ctrl Pts',(-4.7787956998906,-6.57155700659152,
91.8807782974299));
#170516=CARTESIAN_POINT('Ctrl Pts',(-4.73776355339478,-6.60120036916218,
91.8827536675297));
#170517=CARTESIAN_POINT('Ctrl Pts',(-4.66547667998767,-6.65240229120052,
91.8862175681431));
#170518=CARTESIAN_POINT('Ctrl Pts',(-4.63434279484372,-6.67412883768865,
91.8877043135851));
#170519=CARTESIAN_POINT('Ctrl Pts',(-4.5693197890889,-6.71883028840123,
91.8907991144362));
#170520=CARTESIAN_POINT('Ctrl Pts',(-4.53540698411044,-6.74176885177694,
91.8924074966925));
#170521=CARTESIAN_POINT('Ctrl Pts',(-4.44649713665089,-6.80093284582514,
91.8966099552527));
#170522=CARTESIAN_POINT('Ctrl Pts',(-4.39123064891768,-6.8367475948886,
91.8992081380901));
#170523=CARTESIAN_POINT('Ctrl Pts',(-4.15001610900945,-6.9889320246575,
91.9104908965143));
#170524=CARTESIAN_POINT('Ctrl Pts',(-3.95983596699512,-7.09841539955821,
91.9192428340685));
#170525=CARTESIAN_POINT('Ctrl Pts',(-3.35345079974509,-7.41554022079475,
91.9467527587969));
#170526=CARTESIAN_POINT('Ctrl Pts',(-2.92370650732244,-7.59524855334279,
91.9657197079367));
#170527=CARTESIAN_POINT('Ctrl Pts',(-2.32694514049983,-7.78660232120568,
91.9911036976743));
#170528=CARTESIAN_POINT('Ctrl Pts',(-2.17148148805181,-7.83138037372527,
91.9976295449122));
#170529=CARTESIAN_POINT('Ctrl Pts',(-1.95448342815741,-7.88692312920749,
92.0065920338899));
#170530=CARTESIAN_POINT('Ctrl Pts',(-1.89400735448259,-7.90166426453254,
92.0090742476009));
#170531=CARTESIAN_POINT('Ctrl Pts',(-1.78841617188946,-7.92612037366538,
92.0133789052787));
#170532=CARTESIAN_POINT('Ctrl Pts',(-1.74337670423528,-7.93614858055619,
92.0152058198199));
#170533=CARTESIAN_POINT('Ctrl Pts',(-1.67669387153191,-7.9504007005055,
92.0178962314956));
#170534=CARTESIAN_POINT('Ctrl Pts',(-1.65511496156213,-7.95492099956906,
92.0187646362495));
#170535=CARTESIAN_POINT('Ctrl Pts',(-1.61535298273234,-7.96308144898652,
92.0203605978011));
#170536=CARTESIAN_POINT('Ctrl Pts',(-1.5971753932187,-7.96674727780008,
92.0210886161781));
#170537=CARTESIAN_POINT('Ctrl Pts',(-1.55593137413552,-7.97491802261615,
92.0227370677108));
#170538=CARTESIAN_POINT('Ctrl Pts',(-1.53285760693621,-7.97938515619657,
92.0236568898079));
#170539=CARTESIAN_POINT('Ctrl Pts',(-1.47248185710484,-7.99080249180098,
92.0260579822632));
#170540=CARTESIAN_POINT('Ctrl Pts',(-1.43514992363138,-7.99759163745963,
92.0275369144875));
#170541=CARTESIAN_POINT('Ctrl Pts',(-1.21344547183795,-8.03630822846412,
92.0362906665144));
#170542=CARTESIAN_POINT('Ctrl Pts',(-1.02806049269457,-8.06212086388244,
92.0434923785696));
#170543=CARTESIAN_POINT('Ctrl Pts',(-0.646892079442106,-8.1018317777574,
92.0582279408311));
#170544=CARTESIAN_POINT('Ctrl Pts',(-0.451164538096103,-8.11508458141697,
92.0657565407119));
#170545=CARTESIAN_POINT('Ctrl Pts',(-0.137186733452844,-8.12494901028113,
92.0778823318179));
#170546=CARTESIAN_POINT('Ctrl Pts',(-0.0191574650205549,-8.12608450102143,
92.0824510807092));
#170547=CARTESIAN_POINT('Ctrl Pts',(0.146747456388834,-8.12406590758929,
92.0889016755247));
#170548=CARTESIAN_POINT('Ctrl Pts',(0.194634710108802,-8.12305970632771,
92.0907669059179));
#170549=CARTESIAN_POINT('Ctrl Pts',(0.278036579505863,-8.12056934433482,
92.0940220596989));
#170550=CARTESIAN_POINT('Ctrl Pts',(0.313555601712088,-8.11927544120442,
92.0954104467735));
#170551=CARTESIAN_POINT('Ctrl Pts',(0.382619616057752,-8.11630567385771,
92.0981144332776));
#170552=CARTESIAN_POINT('Ctrl Pts',(0.416164978307712,-8.11465478404261,
92.0994298060961));
#170553=CARTESIAN_POINT('Ctrl Pts',(0.507168194802084,-8.10961039953391,
92.1030039504594));
#170554=CARTESIAN_POINT('Ctrl Pts',(0.564601644293109,-8.1058142928137,
92.1052658794024));
#170555=CARTESIAN_POINT('Ctrl Pts',(0.824377814177232,-8.08586984602522,
92.1155267026));
#170556=CARTESIAN_POINT('Ctrl Pts',(1.0261103598194,-8.06275299475706,92.1235797740209));
#170557=CARTESIAN_POINT('Ctrl Pts',(1.47560394559122,-7.99410074502044,
92.1417023329796));
#170558=CARTESIAN_POINT('Ctrl Pts',(1.72254346647485,-7.94455143425055,
92.1517839883327));
#170559=CARTESIAN_POINT('Ctrl Pts',(2.07071499760272,-7.85769056498425,
92.1660641957238));
#170560=CARTESIAN_POINT('Ctrl Pts',(2.17412444322425,-7.82970911697356,
92.170312999074));
#170561=CARTESIAN_POINT('Ctrl Pts',(2.30549862540778,-7.79135726742405,
92.1757072818471));
#170562=CARTESIAN_POINT('Ctrl Pts',(2.33400033231447,-7.78286672375455,
92.1768773478741));
#170563=CARTESIAN_POINT('Ctrl Pts',(2.38150300854262,-7.76843145817181,
92.1788266529969));
#170564=CARTESIAN_POINT('Ctrl Pts',(2.40052984006783,-7.76257305209962,
92.1796072076169));
#170565=CARTESIAN_POINT('Ctrl Pts',(2.43754222615371,-7.75102775573066,
92.1811253405446));
#170566=CARTESIAN_POINT('Ctrl Pts',(2.45552989513141,-7.7453480432535,92.1818630197784));
#170567=CARTESIAN_POINT('Ctrl Pts',(2.49879883054023,-7.73151974063034,
92.1836373933238));
#170568=CARTESIAN_POINT('Ctrl Pts',(2.52406026451679,-7.72330971042026,
92.1846732347543));
#170569=CARTESIAN_POINT('Ctrl Pts',(2.61917018317242,-7.69188227439443,
92.188573715468));
#170570=CARTESIAN_POINT('Ctrl Pts',(2.68874267649146,-7.6678398723011,92.1914279653892));
#170571=CARTESIAN_POINT('Ctrl Pts',(3.15870745455253,-7.4982497084062,92.2107457472262));
#170572=CARTESIAN_POINT('Ctrl Pts',(3.54744472814665,-7.32235092393076,
92.226941471631));
#170573=CARTESIAN_POINT('Ctrl Pts',(4.09745492448331,-7.01935342607266,
92.2511231719495));
#170574=CARTESIAN_POINT('Ctrl Pts',(4.27061899700236,-6.91536488510482,
92.2589318238872));
#170575=CARTESIAN_POINT('Ctrl Pts',(4.50158122225822,-6.76468094802649,
92.2696646824494));
#170576=CARTESIAN_POINT('Ctrl Pts',(4.5628811060411,-6.72348553748016,92.2725449508586));
#170577=CARTESIAN_POINT('Ctrl Pts',(4.66885159089408,-6.65015332560848,
92.2775812948471));
#170578=CARTESIAN_POINT('Ctrl Pts',(4.71377327380087,-6.61838771366723,
92.2797345793723));
#170579=CARTESIAN_POINT('Ctrl Pts',(4.80898249460813,-6.54960104504977,
92.2843381778087));
#170580=CARTESIAN_POINT('Ctrl Pts',(4.8591728964647,-6.51245155148121,92.2867892123616));
#170581=CARTESIAN_POINT('Ctrl Pts',(5.08634286412471,-6.3402185892092,92.2979946922879));
#170582=CARTESIAN_POINT('Ctrl Pts',(5.25815166319581,-6.19847527952391,
92.3067858570428));
#170583=CARTESIAN_POINT('Ctrl Pts',(5.51804839609459,-5.96546819136099,
92.3205647847534));
#170584=CARTESIAN_POINT('Ctrl Pts',(5.61019339695844,-5.87889437516912,
92.3255517792433));
#170585=CARTESIAN_POINT('Ctrl Pts',(5.73176164639371,-5.75921413886876,
92.3322597964552));
#170586=CARTESIAN_POINT('Ctrl Pts',(5.76298899024911,-5.72796621707271,
92.3339947630447));
#170587=CARTESIAN_POINT('Ctrl Pts',(5.82514426711339,-5.66474715385486,
92.337471147635));
#170588=CARTESIAN_POINT('Ctrl Pts',(5.85606761194972,-5.63277357890716,
92.3392124774255));
#170589=CARTESIAN_POINT('Ctrl Pts',(6.02422758908939,-5.45602088821721,
92.3487518638481));
#170590=CARTESIAN_POINT('Ctrl Pts',(6.15635965288398,-5.30647890731507,
92.3565082839764));
#170591=CARTESIAN_POINT('Ctrl Pts',(6.34826528728209,-5.07246059068834,
92.3682928954916));
#170592=CARTESIAN_POINT('Ctrl Pts',(6.41215114329186,-4.99145732721021,
92.3723113257211));
#170593=CARTESIAN_POINT('Ctrl Pts',(6.52285487101566,-4.8454579727847,92.3794615188229));
#170594=CARTESIAN_POINT('Ctrl Pts',(6.57028665096452,-4.78094466593479,
92.3825900264944));
#170595=CARTESIAN_POINT('Ctrl Pts',(6.64896866988736,-4.67054424316788,
92.3878968735665));
#170596=CARTESIAN_POINT('Ctrl Pts',(6.68071627945109,-4.62501868852769,
92.3900720624526));
#170597=CARTESIAN_POINT('Ctrl Pts',(6.74605808178709,-4.52924288272262,
92.3946225376633));
#170598=CARTESIAN_POINT('Ctrl Pts',(6.77956300703941,-4.4789358258076,92.3969982584681));
#170599=CARTESIAN_POINT('Ctrl Pts',(6.87051117099734,-4.33901976098782,
92.4035684828183));
#170600=CARTESIAN_POINT('Ctrl Pts',(6.92675953684029,-4.2486490032143,92.407770739258));
#170601=CARTESIAN_POINT('Ctrl Pts',(7.033015537159,-4.07021252359226,92.415994616535));
#170602=CARTESIAN_POINT('Ctrl Pts',(7.08318446648694,-3.98226508197325,
92.4200143141625));
#170603=CARTESIAN_POINT('Ctrl Pts',(7.18073410898358,-3.80357965860117,
92.4281167148098));
#170604=CARTESIAN_POINT('Ctrl Pts',(7.22807006447523,-3.71283767155708,
92.4321989093444));
#170605=CARTESIAN_POINT('Ctrl Pts',(7.3898254883973,-3.38793195625791,92.446700232125));
#170606=CARTESIAN_POINT('Ctrl Pts',(7.494680469301,-3.14918532239902,92.4571519571623));
#170607=CARTESIAN_POINT('Ctrl Pts',(7.61723394927021,-2.82916441201045,
92.470832470786));
#170608=CARTESIAN_POINT('Ctrl Pts',(7.6454242080905,-2.752074324828,92.4741031506227));
#170609=CARTESIAN_POINT('Ctrl Pts',(7.70112831188899,-2.59227799434258,
92.4808260325697));
#170610=CARTESIAN_POINT('Ctrl Pts',(7.72848926263153,-2.5095291171007,92.4842765442627));
#170611=CARTESIAN_POINT('Ctrl Pts',(7.76362438178407,-2.39723899532729,
92.4889119563045));
#170612=CARTESIAN_POINT('Ctrl Pts',(7.77257082368621,-2.36807118637777,
92.4901117791782));
#170613=CARTESIAN_POINT('Ctrl Pts',(7.7872982159503,-2.31907323497182,92.4921198897859));
#170614=CARTESIAN_POINT('Ctrl Pts',(7.79316819992216,-2.29927022872789,
92.4929294605231));
#170615=CARTESIAN_POINT('Ctrl Pts',(7.80402734338868,-2.26211642439976,
92.4944444415505));
#170616=CARTESIAN_POINT('Ctrl Pts',(7.80903430975614,-2.24477095648766,
92.4951501238388));
#170617=CARTESIAN_POINT('Ctrl Pts',(7.82256613925013,-2.19729988260506,
92.4970769830871));
#170618=CARTESIAN_POINT('Ctrl Pts',(7.83097476858211,-2.16714142680919,
92.4982962723509));
#170619=CARTESIAN_POINT('Ctrl Pts',(7.86936668682193,-2.02630314055323,
92.5039698199576));
#170620=CARTESIAN_POINT('Ctrl Pts',(7.89717939934593,-1.91504424260237,
92.5083932121764));
#170621=CARTESIAN_POINT('Ctrl Pts',(7.99293483520782,-1.49433619285397,
92.5249774384208));
#170622=CARTESIAN_POINT('Ctrl Pts',(8.04511593132074,-1.18159167699269,
92.5370319689456));
#170623=CARTESIAN_POINT('Ctrl Pts',(8.08909131823104,-0.771629623113678,
92.5528917398022));
#170624=CARTESIAN_POINT('Ctrl Pts',(8.09760301466621,-0.676487903331905,
92.5565751681093));
#170625=CARTESIAN_POINT('Ctrl Pts',(8.10977796270002,-0.506722062901886,
92.5631621022111));
#170626=CARTESIAN_POINT('Ctrl Pts',(8.11409312580478,-0.432155649202921,
92.5660601980145));
#170627=CARTESIAN_POINT('Ctrl Pts',(8.11917468930519,-0.316787010046766,
92.5705545605992));
#170628=CARTESIAN_POINT('Ctrl Pts',(8.12066279951398,-0.276020516578724,
92.5721446860148));
#170629=CARTESIAN_POINT('Ctrl Pts',(8.12285858628993,-0.200210768694241,
92.5751058398568));
#170630=CARTESIAN_POINT('Ctrl Pts',(8.12364663015118,-0.165170768644414,
92.5764761571663));
#170631=CARTESIAN_POINT('Ctrl Pts',(8.12490270687114,-0.0867501420875349,
92.5795468931977));
#170632=CARTESIAN_POINT('Ctrl Pts',(8.12525007127121,-0.0433686906354123,
92.5812482788994));
#170633=CARTESIAN_POINT('Ctrl Pts',(8.12524985383566,0.0889764527132254,
92.5864473873871));
#170634=CARTESIAN_POINT('Ctrl Pts',(8.12378862713576,0.177933077463759,
92.5899539884065));
#170635=CARTESIAN_POINT('Ctrl Pts',(8.11677939641233,0.391242446543852,
92.598391986294));
#170636=CARTESIAN_POINT('Ctrl Pts',(8.10983418366525,0.515526530941922,
92.6033326440291));
#170637=CARTESIAN_POINT('Ctrl Pts',(8.08864399641308,0.783883249664426,
92.6140460936026));
#170638=CARTESIAN_POINT('Ctrl Pts',(8.07339810971291,0.927834816599277,
92.6198216539235));
#170639=CARTESIAN_POINT('Ctrl Pts',(8.0320035369246,1.23904959113875,92.6323415848297));
#170640=CARTESIAN_POINT('Ctrl Pts',(8.00445621357875,1.4060605135341,92.6390818150515));
#170641=CARTESIAN_POINT('Ctrl Pts',(7.96508687842567,1.60569352292279,92.6471213009521));
#170642=CARTESIAN_POINT('Ctrl Pts',(7.958247561075,1.63925484318654,92.6484722158129));
#170643=CARTESIAN_POINT('Ctrl Pts',(7.94737818586265,1.69092030307857,92.650550288916));
#170644=CARTESIAN_POINT('Ctrl Pts',(7.94349801913949,1.70905550610098,92.6512794179468));
#170645=CARTESIAN_POINT('Ctrl Pts',(7.93601015429277,1.74347601450636,92.6526626117487));
#170646=CARTESIAN_POINT('Ctrl Pts',(7.93241433184351,1.75976380582013,92.6533168457235));
#170647=CARTESIAN_POINT('Ctrl Pts',(7.92353869181697,1.79938728081446,92.654907577781));
#170648=CARTESIAN_POINT('Ctrl Pts',(7.91820590241353,1.8227109699445,92.6558432356378));
#170649=CARTESIAN_POINT('Ctrl Pts',(7.89987323290624,1.90129241615368,92.658993720898));
#170650=CARTESIAN_POINT('Ctrl Pts',(7.88639726226582,1.95643764008313,92.6612014228558));
#170651=CARTESIAN_POINT('Ctrl Pts',(7.85211128844485,2.09062575625059,92.6665701503346));
#170652=CARTESIAN_POINT('Ctrl Pts',(7.83068430976363,2.16950481597874,92.6697231299059));
#170653=CARTESIAN_POINT('Ctrl Pts',(7.69764406531527,2.63158917648916,92.6882072536937));
#170654=CARTESIAN_POINT('Ctrl Pts',(7.55910628610006,3.00647705294046,92.7032723456445));
#170655=CARTESIAN_POINT('Ctrl Pts',(7.22930345213665,3.73011679811805,92.7335149763978));
#170656=CARTESIAN_POINT('Ctrl Pts',(7.03888962387209,4.07806615740555,92.7486537649256));
#170657=CARTESIAN_POINT('Ctrl Pts',(6.78408109487753,4.47228154070999,92.766885800197));
#170658=CARTESIAN_POINT('Ctrl Pts',(6.74346728117882,4.53328880927804,92.7697393178074));
#170659=CARTESIAN_POINT('Ctrl Pts',(6.67775421221683,4.62916088756795,92.7742763298372));
#170660=CARTESIAN_POINT('Ctrl Pts',(6.65319413919483,4.66439058955986,92.7759550471731));
#170661=CARTESIAN_POINT('Ctrl Pts',(6.606651131461,4.73003770581762,92.7791051666667));
#170662=CARTESIAN_POINT('Ctrl Pts',(6.58473448989053,4.76050076762459,92.7805759687621));
#170663=CARTESIAN_POINT('Ctrl Pts',(6.53496362109936,4.82867851335447,92.7838882485662));
#170664=CARTESIAN_POINT('Ctrl Pts',(6.5069924275391,4.86630611891308,92.7857306485246));
#170665=CARTESIAN_POINT('Ctrl Pts',(6.42101202943511,4.9799024164317,92.7913369923278));
#170666=CARTESIAN_POINT('Ctrl Pts',(6.36198677642911,5.05509126216758,92.7951087145605));
#170667=CARTESIAN_POINT('Ctrl Pts',(6.05012575904466,5.43823691106428,92.8146500019928));
#170668=CARTESIAN_POINT('Ctrl Pts',(5.77621832778755,5.72832731516129,92.8304763858973));
#170669=CARTESIAN_POINT('Ctrl Pts',(5.06455976488356,6.37887229406972,92.8697243155004));
#170670=CARTESIAN_POINT('Ctrl Pts',(4.60826411107181,6.71592229402071,92.8936052317998));
#170671=CARTESIAN_POINT('Ctrl Pts',(3.84854986467929,7.1629649651361,92.9308907716063));
#170672=CARTESIAN_POINT('Ctrl Pts',(3.56728098702269,7.30711440100533,92.944187588048));
#170673=CARTESIAN_POINT('Ctrl Pts',(3.21397616996505,7.46290771442859,92.959824787232));
#170674=CARTESIAN_POINT('Ctrl Pts',(3.14925469017234,7.49044922582953,92.9626464954614));
#170675=CARTESIAN_POINT('Ctrl Pts',(3.07092310402293,7.52258760444498,92.9660036512485));
#170676=CARTESIAN_POINT('Ctrl Pts',(3.0576490248136,7.52799278835976,92.9665705666569));
#170677=CARTESIAN_POINT('Ctrl Pts',(3.03591817965557,7.53677459424869,92.9674953292482));
#170678=CARTESIAN_POINT('Ctrl Pts',(3.0274699455964,7.54017216033047,92.9678540257405));
#170679=CARTESIAN_POINT('Ctrl Pts',(3.0123409579158,7.54622695182328,92.9684948845284));
#170680=CARTESIAN_POINT('Ctrl Pts',(3.00566236249887,7.54888952219057,92.9687772687676));
#170681=CARTESIAN_POINT('Ctrl Pts',(2.9915204581127,7.55450576384538,92.9693741058088));
#170682=CARTESIAN_POINT('Ctrl Pts',(2.98405628484498,7.55745724941607,92.9696884659009));
#170683=CARTESIAN_POINT('Ctrl Pts',(2.96420047090534,7.5652746387566,92.9705229502921));
#170684=CARTESIAN_POINT('Ctrl Pts',(2.95180119226931,7.57012116915082,92.9710422369641));
#170685=CARTESIAN_POINT('Ctrl Pts',(2.89422577864737,7.59246281907712,92.9734448932125));
#170686=CARTESIAN_POINT('Ctrl Pts',(2.84890464706926,7.60958455219702,92.9753115634284));
#170687=CARTESIAN_POINT('Ctrl Pts',(2.45378369314967,7.75483121988337,92.9913555770271));
#170688=CARTESIAN_POINT('Ctrl Pts',(2.09568169783588,7.85917440021571,93.0043536212772));
#170689=CARTESIAN_POINT('Ctrl Pts',(1.05516167749654,8.0861454356565,93.0404568526428));
#170690=CARTESIAN_POINT('Ctrl Pts',(0.362598493273749,8.14663450538044,
93.0627236651696));
#170691=CARTESIAN_POINT('Ctrl Pts',(-0.585419638428446,8.10818730570098,
93.0967615628309));
#170692=CARTESIAN_POINT('Ctrl Pts',(-0.840937253722497,8.08568052112567,
93.1062621856567));
#170693=CARTESIAN_POINT('Ctrl Pts',(-1.12360348951219,8.04723796083923,
93.1172475852981));
#170694=CARTESIAN_POINT('Ctrl Pts',(-1.15223287427744,8.04318860794345,
93.1183656127763));
#170695=CARTESIAN_POINT('Ctrl Pts',(-1.19244611735059,8.03728171904753,
93.1199437099653));
#170696=CARTESIAN_POINT('Ctrl Pts',(-1.20404863774974,8.03555175769981,
93.1203999324242));
#170697=CARTESIAN_POINT('Ctrl Pts',(-1.22533306186345,8.03233106957042,
93.1212385221845));
#170698=CARTESIAN_POINT('Ctrl Pts',(-1.2350161026939,8.0308479470702,93.1216206595202));
#170699=CARTESIAN_POINT('Ctrl Pts',(-1.2546405225703,8.02780580128416,93.1223964187254));
#170700=CARTESIAN_POINT('Ctrl Pts',(-1.26458173367128,8.02624581370359,
93.1227900691009));
#170701=CARTESIAN_POINT('Ctrl Pts',(-1.28906227447679,8.02235768508244,
93.1237611064198));
#170702=CARTESIAN_POINT('Ctrl Pts',(-1.3035981971649,8.02000848581037,93.1243391279877));
#170703=CARTESIAN_POINT('Ctrl Pts',(-1.35668008998067,8.01128161796277,
93.1264552402919));
#170704=CARTESIAN_POINT('Ctrl Pts',(-1.39518601763755,8.00466551163902,
93.1280005189447));
#170705=CARTESIAN_POINT('Ctrl Pts',(-1.6175676447821,7.96480244331913,93.1369848906469));
#170706=CARTESIAN_POINT('Ctrl Pts',(-1.80029237755123,7.92549965328251,
93.1446064091622));
#170707=CARTESIAN_POINT('Ctrl Pts',(-2.3770855277246,7.78045890836892,93.1694332999153));
#170708=CARTESIAN_POINT('Ctrl Pts',(-2.7645941422359,7.65134290188091,93.1873038718073));
#170709=CARTESIAN_POINT('Ctrl Pts',(-3.7721806164034,7.22904509667764,93.2361142513957));
#170710=CARTESIAN_POINT('Ctrl Pts',(-4.36770081301235,6.8856244915369,93.2675980694527));
#170711=CARTESIAN_POINT('Ctrl Pts',(-4.94405345614466,6.44806412916196,
93.2967781797405));
#170712=CARTESIAN_POINT('Ctrl Pts',(-4.97481482977613,6.42436090787477,
93.298331671286));
#170713=CARTESIAN_POINT('Ctrl Pts',(-5.01574588447303,6.39235114046577,
93.3003950086423));
#170714=CARTESIAN_POINT('Ctrl Pts',(-5.02606673857963,6.38423942397562,
93.3009149625828));
#170715=CARTESIAN_POINT('Ctrl Pts',(-5.04216959115919,6.37152007265509,
93.3017257736861));
#170716=CARTESIAN_POINT('Ctrl Pts',(-5.0479650081613,6.36692951893811,93.3020174963962));
#170717=CARTESIAN_POINT('Ctrl Pts',(-5.05957714493085,6.35770571651672,
93.3026018527));
#170718=CARTESIAN_POINT('Ctrl Pts',(-5.06539378505848,6.35307238004323,
93.3028944813418));
#170719=CARTESIAN_POINT('Ctrl Pts',(-5.07852206594827,6.34258534933163,
93.3035547840228));
#170720=CARTESIAN_POINT('Ctrl Pts',(-5.08582997002368,6.33672697887453,
93.3039222268951));
#170721=CARTESIAN_POINT('Ctrl Pts',(-5.10746863069011,6.31931883318924,
93.3050099227394));
#170722=CARTESIAN_POINT('Ctrl Pts',(-5.12177034237241,6.30773294422095,
93.305728425548));
#170723=CARTESIAN_POINT('Ctrl Pts',(-5.23842675913126,6.21257065238713,
93.3115868846551));
#170724=CARTESIAN_POINT('Ctrl Pts',(-5.33877110104034,6.12655483502121,
93.3166122840362));
#170725=CARTESIAN_POINT('Ctrl Pts',(-5.59297117555916,5.89766276210383,
93.3294163189935));
#170726=CARTESIAN_POINT('Ctrl Pts',(-5.74346918672227,5.75120150716792,
93.3370713668058));
#170727=CARTESIAN_POINT('Ctrl Pts',(-6.41263853746888,5.04748584097122,
93.3721640961438));
#170728=CARTESIAN_POINT('Ctrl Pts',(-6.85702792995148,4.42495441150281,
93.3990550745752));
#170729=CARTESIAN_POINT('Ctrl Pts',(-7.2447176474381,3.67967164622257,93.4312128251604));
#170730=CARTESIAN_POINT('Ctrl Pts',(-7.2801193993134,3.60912434589969,93.4342511024308));
#170731=CARTESIAN_POINT('Ctrl Pts',(-7.32726894840244,3.51164903081612,
93.4384416871382));
#170732=CARTESIAN_POINT('Ctrl Pts',(-7.33990712666235,3.48515602518261,
93.439579905517));
#170733=CARTESIAN_POINT('Ctrl Pts',(-7.3613273987315,3.43962006905566,93.441534966081));
#170734=CARTESIAN_POINT('Ctrl Pts',(-7.37017985566783,3.42061049848573,
93.4423507450559));
#170735=CARTESIAN_POINT('Ctrl Pts',(-7.38718248430694,3.38372699853912,
93.4439328049726));
#170736=CARTESIAN_POINT('Ctrl Pts',(-7.39534163096749,3.36585733743203,
93.4446989415956));
#170737=CARTESIAN_POINT('Ctrl Pts',(-7.41403289695554,3.32452480680324,
93.4464702787413));
#170738=CARTESIAN_POINT('Ctrl Pts',(-7.42451857386444,3.3010411884574,93.4474761502845));
#170739=CARTESIAN_POINT('Ctrl Pts',(-7.45361242283203,3.23504298948758,
93.4503018601173));
#170740=CARTESIAN_POINT('Ctrl Pts',(-7.47196803726678,3.19241834703397,
93.4521254645569));
#170741=CARTESIAN_POINT('Ctrl Pts',(-7.5866068548216,2.91980302174023,93.4637838740343));
#170742=CARTESIAN_POINT('Ctrl Pts',(-7.67262277575293,2.68564813872753,
93.4737814233935));
#170743=CARTESIAN_POINT('Ctrl Pts',(-7.84472732977312,2.14093144407124,
93.4971185373445));
#170744=CARTESIAN_POINT('Ctrl Pts',(-7.9233853814544,1.82846522772179,93.5105695114073));
#170745=CARTESIAN_POINT('Ctrl Pts',(-8.0821245570991,0.990422030426204,
93.546621976284));
#170746=CARTESIAN_POINT('Ctrl Pts',(-8.12956703598508,0.460243031389453,
93.5694736406476));
#170747=CARTESIAN_POINT('Ctrl Pts',(-8.12444251434636,-0.128091216856152,
93.5932478105546));
#170748=CARTESIAN_POINT('Ctrl Pts',(-8.12333664255147,-0.18540631272118,
93.5955459935552));
#170749=CARTESIAN_POINT('Ctrl Pts',(-8.12117453609173,-0.25775656968365,
93.5984210476238));
#170750=CARTESIAN_POINT('Ctrl Pts',(-8.12068291706426,-0.272806266345323,
93.5990176705914));
#170751=CARTESIAN_POINT('Ctrl Pts',(-8.11983993258543,-0.296586191083534,
93.5999580635789));
#170752=CARTESIAN_POINT('Ctrl Pts',(-8.11951631739125,-0.305317329815395,
93.6003028464561));
#170753=CARTESIAN_POINT('Ctrl Pts',(-8.11888934052497,-0.321526756330951,
93.6009419993758));
#170754=CARTESIAN_POINT('Ctrl Pts',(-8.11858972815591,-0.32900517483413,
93.6012365092375));
#170755=CARTESIAN_POINT('Ctrl Pts',(-8.1179051404897,-0.345522119738005,
93.6018861341483));
#170756=CARTESIAN_POINT('Ctrl Pts',(-8.11751540163881,-0.354560446468816,
93.6022410672732));
#170757=CARTESIAN_POINT('Ctrl Pts',(-8.11668392317779,-0.373122705508367,
93.6029688470262));
#170758=CARTESIAN_POINT('Ctrl Pts',(-8.11624051386584,-0.382646552588263,
93.6033416280234));
#170759=CARTESIAN_POINT('Ctrl Pts',(-8.11506270384081,-0.407020820485135,
93.6042940477138));
#170760=CARTESIAN_POINT('Ctrl Pts',(-8.11430429985016,-0.421870085268918,
93.6048727268254));
#170761=CARTESIAN_POINT('Ctrl Pts',(-8.11200793428495,-0.464532869672184,
93.6065306964587));
#170762=CARTESIAN_POINT('Ctrl Pts',(-8.11036768771832,-0.492340846580435,
93.6076057460644));
#170763=CARTESIAN_POINT('Ctrl Pts',(-8.09235482994553,-0.773147473826267,
93.6184013685156));
#170764=CARTESIAN_POINT('Ctrl Pts',(-8.06429209754929,-1.02526214079034,
93.6275711182436));
#170765=CARTESIAN_POINT('Ctrl Pts',(-7.95450336871915,-1.71588537881363,
93.6520617954594));
#170766=CARTESIAN_POINT('Ctrl Pts',(-7.84841013923517,-2.14962086652652,
93.6667677898156));
#170767=CARTESIAN_POINT('Ctrl Pts',(-7.52295331662879,-3.12470753135144,
93.7015353456496));
#170768=CARTESIAN_POINT('Ctrl Pts',(-7.27983978476436,-3.65547154298248,
93.721845101291));
#170769=CARTESIAN_POINT('Ctrl Pts',(-6.96462931177202,-4.18506813867342,
93.7455237581159));
#170770=CARTESIAN_POINT('Ctrl Pts',(-6.946955626451,-4.21434031211697,93.7468438069342));
#170771=CARTESIAN_POINT('Ctrl Pts',(-6.92234382236947,-4.25452827115195,
93.7486719161675));
#170772=CARTESIAN_POINT('Ctrl Pts',(-6.9155635229353,-4.26554052419386,
93.7491744988491));
#170773=CARTESIAN_POINT('Ctrl Pts',(-6.90390855260079,-4.28436916213679,
93.750036646164));
#170774=CARTESIAN_POINT('Ctrl Pts',(-6.89904681773824,-4.29219354481024,
93.7503957597633));
#170775=CARTESIAN_POINT('Ctrl Pts',(-6.889047551509,-4.30822529013419,93.7511332982291));
#170776=CARTESIAN_POINT('Ctrl Pts',(-6.8839086348603,-4.31643176983551,
93.7515117712047));
#170777=CARTESIAN_POINT('Ctrl Pts',(-6.8720174405855,-4.33534590383467,
93.7523862345009));
#170778=CARTESIAN_POINT('Ctrl Pts',(-6.86525479241219,-4.34604699044165,
93.7528825877653));
#170779=CARTESIAN_POINT('Ctrl Pts',(-6.84403052917533,-4.37945870963368,
93.7544373878876));
#170780=CARTESIAN_POINT('Ctrl Pts',(-6.82948108948303,-4.40211318632358,
93.7554989209249));
#170781=CARTESIAN_POINT('Ctrl Pts',(-6.62764356749219,-4.71297898010225,
93.7701670742825));
#170782=CARTESIAN_POINT('Ctrl Pts',(-6.4223808418545,-4.98907000899445,
93.784423026309));
#170783=CARTESIAN_POINT('Ctrl Pts',(-5.84025454190004,-5.67639072802745,
93.8232087044756));
#170784=CARTESIAN_POINT('Ctrl Pts',(-5.43749754265107,-6.06329314558541,
93.848590321199));
#170785=CARTESIAN_POINT('Ctrl Pts',(-4.64553360621117,-6.68124313302881,
93.8936770602743));
#170786=CARTESIAN_POINT('Ctrl Pts',(-4.27047986554562,-6.9269850970865,
93.9133892191095));
#170787=CARTESIAN_POINT('Ctrl Pts',(-3.85204446889236,-7.15417707643722,
93.9324514619052));
#170788=CARTESIAN_POINT('Ctrl Pts',(-3.82698216091663,-7.16761493115945,
93.9335830978271));
#170789=CARTESIAN_POINT('Ctrl Pts',(-3.79192100721013,-7.18617762415684,
93.9351528610127));
#170790=CARTESIAN_POINT('Ctrl Pts',(-3.78198149380261,-7.19141361299281,
93.9355963850568));
#170791=CARTESIAN_POINT('Ctrl Pts',(-3.76600065592939,-7.19978978715145,
93.936307147053));
#170792=CARTESIAN_POINT('Ctrl Pts',(-3.75996621001173,-7.20294301099246,
93.9365749998592));
#170793=CARTESIAN_POINT('Ctrl Pts',(-3.74747918444401,-7.20944798124879,
93.9371281747099));
#170794=CARTESIAN_POINT('Ctrl Pts',(-3.74102605388138,-7.21279865910471,
93.9374134471239));
#170795=CARTESIAN_POINT('Ctrl Pts',(-3.72595631212753,-7.22059770075181,
93.938078250145));
#170796=CARTESIAN_POINT('Ctrl Pts',(-3.71733620686508,-7.22503931630575,
93.938457474001));
#170797=CARTESIAN_POINT('Ctrl Pts',(-3.68967661157573,-7.23922865940013,
93.9396709915774));
#170798=CARTESIAN_POINT('Ctrl Pts',(-3.67060648474689,-7.248916686373,93.9405026426717));
#170799=CARTESIAN_POINT('Ctrl Pts',(-3.6258330165306,-7.27144056570283,
93.9424439714764));
#170800=CARTESIAN_POINT('Ctrl Pts',(-3.60009932956053,-7.28421566167321,
93.9435511130068));
#170801=CARTESIAN_POINT('Ctrl Pts',(-3.30147378708005,-7.43049469349547,
93.9563048419942));
#170802=CARTESIAN_POINT('Ctrl Pts',(-3.02135377311215,-7.54873634024201,
93.9673738301179));
#170803=CARTESIAN_POINT('Ctrl Pts',(-2.43944920029246,-7.75676879931419,
93.9896318832181));
#170804=CARTESIAN_POINT('Ctrl Pts',(-2.13775555837363,-7.84527740623423,
94.0007965906625));
#170805=CARTESIAN_POINT('Ctrl Pts',(-1.19164602508899,-8.06419634275773,
94.0358420535354));
#170806=CARTESIAN_POINT('Ctrl Pts',(-0.53603397468793,-8.13411680021638,
94.0604396781689));
#170807=CARTESIAN_POINT('Ctrl Pts',(0.239665104336485,-8.12258485979519,
94.0903955235954));
#170808=CARTESIAN_POINT('Ctrl Pts',(0.358495527963639,-8.11820822413523,
94.0950035982537));
#170809=CARTESIAN_POINT('Ctrl Pts',(0.524270408883189,-8.10845562908657,
94.1014696155473));
#170810=CARTESIAN_POINT('Ctrl Pts',(0.571329394682538,-8.10527574168545,
94.10330935506));
#170811=CARTESIAN_POINT('Ctrl Pts',(0.65677390625967,-8.0987542243183,94.1066581567038));
#170812=CARTESIAN_POINT('Ctrl Pts',(0.695168489963827,-8.09554894411697,
94.1081660327224));
#170813=CARTESIAN_POINT('Ctrl Pts',(0.768494165665619,-8.08890203938111,
94.1110520554409));
#170814=CARTESIAN_POINT('Ctrl Pts',(0.803428624046099,-8.08550690561616,
94.1124297740295));
#170815=CARTESIAN_POINT('Ctrl Pts',(0.888948745042009,-8.07663584078636,
94.1158094948154));
#170816=CARTESIAN_POINT('Ctrl Pts',(0.93950698948236,-8.07091091264257,
94.1178135852694));
#170817=CARTESIAN_POINT('Ctrl Pts',(1.10705787579913,-8.05034269877351,
94.1244764990593));
#170818=CARTESIAN_POINT('Ctrl Pts',(1.22378020424593,-8.03342743255707,
94.1291528301537));
#170819=CARTESIAN_POINT('Ctrl Pts',(1.50875887478279,-7.9857734874066,94.1406635343539));
#170820=CARTESIAN_POINT('Ctrl Pts',(1.6764915489995,-7.95225166395241,94.1475193163545));
#170821=CARTESIAN_POINT('Ctrl Pts',(2.13492130724615,-7.8454837057301,94.1664892240613));
#170822=CARTESIAN_POINT('Ctrl Pts',(2.42281623106958,-7.76140852331199,
94.1786677504523));
#170823=CARTESIAN_POINT('Ctrl Pts',(3.01965507519996,-7.5506580854287,94.204390600435));
#170824=CARTESIAN_POINT('Ctrl Pts',(3.32678602397583,-7.42046197025177,
94.2179111263362));
#170825=CARTESIAN_POINT('Ctrl Pts',(3.67356996937964,-7.24758648178896,
94.2333292001477));
#170826=CARTESIAN_POINT('Ctrl Pts',(3.72184149484221,-7.22291645301249,
94.2354787341847));
#170827=CARTESIAN_POINT('Ctrl Pts',(3.78938011786363,-7.18754278636198,
94.2384897562336));
#170828=CARTESIAN_POINT('Ctrl Pts',(3.8088558314234,-7.1772411304074,94.2393584422881));
#170829=CARTESIAN_POINT('Ctrl Pts',(3.84469072501032,-7.15809936702538,
94.2409574602725));
#170830=CARTESIAN_POINT('Ctrl Pts',(3.86106187810866,-7.14928209640021,
94.241688207567));
#170831=CARTESIAN_POINT('Ctrl Pts',(3.89293042845703,-7.13197675622056,
94.2431113334868));
#170832=CARTESIAN_POINT('Ctrl Pts',(3.90843069664883,-7.12349417519611,
94.2438038121072));
#170833=CARTESIAN_POINT('Ctrl Pts',(3.94636018847926,-7.10257604891583,
94.2454992554872));
#170834=CARTESIAN_POINT('Ctrl Pts',(3.96875847269916,-7.09008472869666,
94.2465012595828));
#170835=CARTESIAN_POINT('Ctrl Pts',(4.02096185201129,-7.06064649021562,
94.248839082556));
#170836=CARTESIAN_POINT('Ctrl Pts',(4.05071960355491,-7.04361652722853,
94.2501736149221));
#170837=CARTESIAN_POINT('Ctrl Pts',(4.1388733525322,-6.9924239007025,94.2541343625399));
#170838=CARTESIAN_POINT('Ctrl Pts',(4.1969516055638,-6.95771959319506,94.2567535095189));
#170839=CARTESIAN_POINT('Ctrl Pts',(4.44296767693062,-6.80651285286694,
94.2679074882593));
#170840=CARTESIAN_POINT('Ctrl Pts',(4.6265414970018,-6.68309012542854,94.2763835876451));
#170841=CARTESIAN_POINT('Ctrl Pts',(4.95433929213461,-6.44271465951965,
94.2920236600736));
#170842=CARTESIAN_POINT('Ctrl Pts',(5.10002929741213,-6.32801313970813,
94.2991729073603));
#170843=CARTESIAN_POINT('Ctrl Pts',(5.2831451783569,-6.17341163803696,94.3084791637397));
#170844=CARTESIAN_POINT('Ctrl Pts',(5.32427038573578,-6.13797841750926,
94.3105909299399));
#170845=CARTESIAN_POINT('Ctrl Pts',(5.3923105628403,-6.07815705369578,94.3141225691202));
#170846=CARTESIAN_POINT('Ctrl Pts',(5.41942268146581,-6.05399571889103,
94.3155400507038));
#170847=CARTESIAN_POINT('Ctrl Pts',(5.47079098675269,-6.00759655303768,
94.3182456428773));
#170848=CARTESIAN_POINT('Ctrl Pts',(5.49507585450967,-5.9853915251884,94.319533380041));
#170849=CARTESIAN_POINT('Ctrl Pts',(5.54504001266233,-5.93914607760545,
94.322201001542));
#170850=CARTESIAN_POINT('Ctrl Pts',(5.57069942198457,-5.9150851906819,94.3235810875003));
#170851=CARTESIAN_POINT('Ctrl Pts',(5.66201168794523,-5.82834030258141,
94.3285290988506));
#170852=CARTESIAN_POINT('Ctrl Pts',(5.72676903133103,-5.76472404650015,
94.3321071172336));
#170853=CARTESIAN_POINT('Ctrl Pts',(5.83822238763341,-5.65150289343008,
94.3383893736165));
#170854=CARTESIAN_POINT('Ctrl Pts',(5.88538596003253,-5.60237071619785,
94.3410884079341));
#170855=CARTESIAN_POINT('Ctrl Pts',(6.14872933151441,-5.3210396443987,94.3563905975068));
#170856=CARTESIAN_POINT('Ctrl Pts',(6.35178106232219,-5.07692920692795,
94.3691058784524));
#170857=CARTESIAN_POINT('Ctrl Pts',(6.60864429844011,-4.7285172201209,94.3863432994216));
#170858=CARTESIAN_POINT('Ctrl Pts',(6.67525793159644,-4.63400329198903,
94.390932686035));
#170859=CARTESIAN_POINT('Ctrl Pts',(6.75737771400264,-4.51204175914137,
94.396730248853));
#170860=CARTESIAN_POINT('Ctrl Pts',(6.7747718294589,-4.48588241899203,94.3979666117227));
#170861=CARTESIAN_POINT('Ctrl Pts',(6.80192898415205,-4.44452202153799,
94.3999097410327));
#170862=CARTESIAN_POINT('Ctrl Pts',(6.81179373083975,-4.42938822806896,
94.400618275963));
#170863=CARTESIAN_POINT('Ctrl Pts',(6.83180714023567,-4.39846009544633,
94.402061396736));
#170864=CARTESIAN_POINT('Ctrl Pts',(6.84195170517382,-4.38266321764517,
94.402795913185));
#170865=CARTESIAN_POINT('Ctrl Pts',(6.86312160854572,-4.34944529700583,
94.4043352422872));
#170866=CARTESIAN_POINT('Ctrl Pts',(6.87413557813542,-4.33201715854962,
94.4051398721691));
#170867=CARTESIAN_POINT('Ctrl Pts',(6.9002655692591,-4.29031935110828,94.4070581040988));
#170868=CARTESIAN_POINT('Ctrl Pts',(6.91532006909514,-4.26601141706768,
94.4081708075468));
#170869=CARTESIAN_POINT('Ctrl Pts',(6.95585551646879,-4.19978192803541,
94.4111882119207));
#170870=CARTESIAN_POINT('Ctrl Pts',(6.9810856659204,-4.15770816283401,94.413089668434));
#170871=CARTESIAN_POINT('Ctrl Pts',(7.06230665883452,-4.01944026532467,
94.4192925918609));
#170872=CARTESIAN_POINT('Ctrl Pts',(7.11670247667,-3.92232348269673,94.4235776706964));
#170873=CARTESIAN_POINT('Ctrl Pts',(7.29151932019704,-3.59459391538582,
94.4378483277363));
#170874=CARTESIAN_POINT('Ctrl Pts',(7.40285907135733,-3.35932095362181,
94.4477898999218));
#170875=CARTESIAN_POINT('Ctrl Pts',(7.59795942680543,-2.89002618666521,
94.4673169633243));
#170876=CARTESIAN_POINT('Ctrl Pts',(7.68265470320967,-2.65669971974528,
94.4768872953532));
#170877=CARTESIAN_POINT('Ctrl Pts',(7.78026772401202,-2.34381494818529,
94.489633532609));
#170878=CARTESIAN_POINT('Ctrl Pts',(7.80287426860133,-2.2674186712139,94.4927386174087));
#170879=CARTESIAN_POINT('Ctrl Pts',(7.83924191289082,-2.13752732468404,
94.4980078398094));
#170880=CARTESIAN_POINT('Ctrl Pts',(7.85358769691227,-2.08420178779168,
94.5001681864227));
#170881=CARTESIAN_POINT('Ctrl Pts',(7.87962818824257,-1.98331676804297,
94.504250251202));
#170882=CARTESIAN_POINT('Ctrl Pts',(7.89143866391432,-1.93578965378824,
94.5061712255615));
#170883=CARTESIAN_POINT('Ctrl Pts',(7.92462565439062,-1.79688673159534,
94.5117795309055));
#170884=CARTESIAN_POINT('Ctrl Pts',(7.94484967763263,-1.70524402686819,
94.515472274636));
#170885=CARTESIAN_POINT('Ctrl Pts',(7.99102255032171,-1.47732408836588,
94.5246368111807));
#170886=CARTESIAN_POINT('Ctrl Pts',(8.01507757729343,-1.3406935418348,94.5301137549015));
#170887=CARTESIAN_POINT('Ctrl Pts',(8.05471752283239,-1.07602565819084,
94.5406789793507));
#170888=CARTESIAN_POINT('Ctrl Pts',(8.07077518748635,-0.948100011774246,
94.5457658455318));
#170889=CARTESIAN_POINT('Ctrl Pts',(8.08857779114679,-0.772564218716246,
94.5527067790584));
#170890=CARTESIAN_POINT('Ctrl Pts',(8.09295816759113,-0.725240837896785,
94.5545741018293));
#170891=CARTESIAN_POINT('Ctrl Pts',(8.09998200874483,-0.641344923005015,
94.5578766013952));
#170892=CARTESIAN_POINT('Ctrl Pts',(8.1027935563917,-0.604787930219098,
94.5593128928134));
#170893=CARTESIAN_POINT('Ctrl Pts',(8.10893563513252,-0.517173357069507,
94.5627497507151));
#170894=CARTESIAN_POINT('Ctrl Pts',(8.11203152063572,-0.466100895576881,
94.5647487800398));
#170895=CARTESIAN_POINT('Ctrl Pts',(8.12171406204287,-0.276775813883193,
94.5721478635364));
#170896=CARTESIAN_POINT('Ctrl Pts',(8.12525024283596,-0.138391731887678,
94.5775341323858));
#170897=CARTESIAN_POINT('Ctrl Pts',(8.12524999998749,1.42566410947162E-5,
94.5829227676044));
#170898=CARTESIAN_POINT('',(8.12571484367965,-5.65716636902258E-7,96.5832950704718));
#170899=CARTESIAN_POINT('Ctrl Pts',(8.12456002707784,-1.23182048087137E-6,
94.5833205544621));
#170900=CARTESIAN_POINT('Ctrl Pts',(8.12402776914182,1.12776970425289,94.6275398487303));
#170901=CARTESIAN_POINT('Ctrl Pts',(7.60758318760407,3.60567669421567,94.724648298094));
#170902=CARTESIAN_POINT('Ctrl Pts',(5.15483525499198,6.72198816743881,94.8746459025528));
#170903=CARTESIAN_POINT('Ctrl Pts',(1.33775837807665,8.3503280792661,95.0333133678393));
#170904=CARTESIAN_POINT('Ctrl Pts',(-4.25467436631755,7.88859242601584,
95.2448699882213));
#170905=CARTESIAN_POINT('Ctrl Pts',(-8.30012585283032,3.35904394789376,
95.456426608603));
#170906=CARTESIAN_POINT('Ctrl Pts',(-8.15520229705827,-2.22234120788674,
95.6679832289851));
#170907=CARTESIAN_POINT('Ctrl Pts',(-5.44841867805453,-7.10570068667848,
95.8795398493668));
#170908=CARTESIAN_POINT('Ctrl Pts',(0.335793904015422,-8.95641601104346,
96.0910964697489));
#170909=CARTESIAN_POINT('Ctrl Pts',(5.38922504977475,-6.51729066085791,
96.3026530901306));
#170910=CARTESIAN_POINT('Ctrl Pts',(7.66270883609975,-3.43458399987812,
96.4490895720065));
#170911=CARTESIAN_POINT('Ctrl Pts',(8.12424186435146,-1.03981093457564,
96.542636898787));
#170912=CARTESIAN_POINT('Ctrl Pts',(8.12571484367965,-5.65716636902251E-7,
96.5832950704718));
#170913=CARTESIAN_POINT('',(8.12525,-4.14083264205223E-12,98.5832974432122));
#170914=CARTESIAN_POINT('Ctrl Pts',(8.12525,-4.42750847282105E-12,96.5832974432122));
#170915=CARTESIAN_POINT('Ctrl Pts',(8.12525000000122,2.24624642432963,96.6712950363534));
#170916=CARTESIAN_POINT('Ctrl Pts',(7.14398562317848,4.47535249753052,96.7592926294946));
#170917=CARTESIAN_POINT('Ctrl Pts',(3.83078204045361,7.50935546634141,96.935287815777));
#170918=CARTESIAN_POINT('Ctrl Pts',(1.52412477698225,8.29110090552047,97.0232854089182));
#170919=CARTESIAN_POINT('Ctrl Pts',(-2.9510162393209,7.89663306204599,97.1992805952006));
#170920=CARTESIAN_POINT('Ctrl Pts',(-5.08535169588328,6.72342983086093,
97.2872781883418));
#170921=CARTESIAN_POINT('Ctrl Pts',(-7.81671694684208,3.15661951053424,
97.4632733746242));
#170922=CARTESIAN_POINT('Ctrl Pts',(-8.39290461146651,0.790229551559375,
97.5512709677654));
#170923=CARTESIAN_POINT('Ctrl Pts',(-7.60701611462715,-3.63299000729928,
97.7272661540478));
#170924=CARTESIAN_POINT('Ctrl Pts',(-6.25093680401722,-5.65606750609613,
97.815263747189));
#170925=CARTESIAN_POINT('Ctrl Pts',(-2.45807268689086,-8.06369575488155,
97.9912589334714));
#170926=CARTESIAN_POINT('Ctrl Pts',(-0.0502299510509621,-8.42987470330081,
98.0792565266126));
#170927=CARTESIAN_POINT('Ctrl Pts',(4.28689960880504,-7.25863639434851,
98.255251712895));
#170928=CARTESIAN_POINT('Ctrl Pts',(6.18309125556768,-5.73015646266801,
98.3432493060362));
#170929=CARTESIAN_POINT('Ctrl Pts',(7.81050559202745,-2.58640713800765,
98.4819304138557));
#170930=CARTESIAN_POINT('Ctrl Pts',(8.12524999999934,-1.29375883538613,
98.5326139285339));
#170931=CARTESIAN_POINT('Ctrl Pts',(8.12525,-4.14083171691527E-12,98.5832974432122));
#170932=CARTESIAN_POINT('',(2.10208451021631,7.8486258844723,99.));
#170933=CARTESIAN_POINT('Ctrl Pts',(8.12524988254124,0.00138158011351417,
98.5832974432122));
#170934=CARTESIAN_POINT('Ctrl Pts',(8.12521252668128,0.22107618469403,98.5919091350809));
#170935=CARTESIAN_POINT('Ctrl Pts',(8.11626051648965,0.440727213117883,
98.6005208269495));
#170936=CARTESIAN_POINT('Ctrl Pts',(8.0984302060208,0.659633050043605,98.6091325188182));
#170937=CARTESIAN_POINT('Ctrl Pts',(8.08059799267019,0.878562248981262,
98.6177451297416));
#170938=CARTESIAN_POINT('Ctrl Pts',(8.05388560924342,1.09674586882328,98.6263577406649));
#170939=CARTESIAN_POINT('Ctrl Pts',(8.01838132186286,1.31348716769554,98.6349703515883));
#170940=CARTESIAN_POINT('Ctrl Pts',(7.98287816255186,1.53022158009628,98.6435826888652));
#170941=CARTESIAN_POINT('Ctrl Pts',(7.93858369612052,1.74551353666527,98.652195026142));
#170942=CARTESIAN_POINT('Ctrl Pts',(7.88563759671646,1.95867487239507,98.6608073634189));
#170943=CARTESIAN_POINT('Ctrl Pts',(7.84084602861086,2.13900601282445,98.6680932654216));
#170944=CARTESIAN_POINT('Ctrl Pts',(7.78986346722536,2.31781236312912,98.6753791674244));
#170945=CARTESIAN_POINT('Ctrl Pts',(7.73280286670696,2.49468382508658,98.6826650694271));
#170946=CARTESIAN_POINT('Ctrl Pts',(7.66976526129178,2.69008228438749,98.6907141577887));
#170947=CARTESIAN_POINT('Ctrl Pts',(7.59929130474582,2.88317067675791,98.6987632461504));
#170948=CARTESIAN_POINT('Ctrl Pts',(7.52157620346321,3.07336606638323,98.7068123345121));
#170949=CARTESIAN_POINT('Ctrl Pts',(7.44388876653266,3.26349375189272,98.7148585576286));
#170950=CARTESIAN_POINT('Ctrl Pts',(7.35896544557454,3.45073019344213,98.7229047807452));
#170951=CARTESIAN_POINT('Ctrl Pts',(7.26705019905045,3.63451082911867,98.7309510038617));
#170952=CARTESIAN_POINT('Ctrl Pts',(7.17515588441129,3.81824961237937,98.7389953946096));
#170953=CARTESIAN_POINT('Ctrl Pts',(7.07627296281827,3.99853387452038,98.7470397853575));
#170954=CARTESIAN_POINT('Ctrl Pts',(6.97069236811693,4.17482160955128,98.7550841761054));
#170955=CARTESIAN_POINT('Ctrl Pts',(6.86510685785221,4.3511175520898,98.7631289413796));
#170956=CARTESIAN_POINT('Ctrl Pts',(6.75282321108776,4.52341631961701,98.7711737066538));
#170957=CARTESIAN_POINT('Ctrl Pts',(6.63417734572678,4.69120224547456,98.779218471928));
#170958=CARTESIAN_POINT('Ctrl Pts',(6.51553126712269,4.85898847289503,98.7872632516612));
#170959=CARTESIAN_POINT('Ctrl Pts',(6.39052313404091,5.02226158400115,98.7953080313943));
#170960=CARTESIAN_POINT('Ctrl Pts',(6.25953120194918,5.18053633269033,98.8033528111274));
#170961=CARTESIAN_POINT('Ctrl Pts',(6.12849303100207,5.3388669507991,98.8114004305882));
#170962=CARTESIAN_POINT('Ctrl Pts',(5.99146704521336,5.49219543623203,98.8194480500489));
#170963=CARTESIAN_POINT('Ctrl Pts',(5.84887129471538,5.64007022477154,98.8274956695097));
#170964=CARTESIAN_POINT('Ctrl Pts',(5.76714616726557,5.72482089860158,98.832107957911));
#170965=CARTESIAN_POINT('Ctrl Pts',(5.68359223740185,5.80778083579945,98.8367202463123));
#170966=CARTESIAN_POINT('Ctrl Pts',(5.59829361147862,5.88887053705358,98.8413325347136));
#170967=CARTESIAN_POINT('Ctrl Pts',(5.44430442793545,6.03526136990382,98.8496590759386));
#170968=CARTESIAN_POINT('Ctrl Pts',(5.28455978604005,6.17561896389448,98.8579856171636));
#170969=CARTESIAN_POINT('Ctrl Pts',(5.11955079439096,6.30950768492684,98.8663121583885));
#170970=CARTESIAN_POINT('Ctrl Pts',(4.95456136904949,6.44338052980679,98.8746377122754));
#170971=CARTESIAN_POINT('Ctrl Pts',(4.78430905737275,6.57078585768088,98.8829632661622));
#170972=CARTESIAN_POINT('Ctrl Pts',(4.60931796522703,6.69132837767923,98.8912888200491));
#170973=CARTESIAN_POINT('Ctrl Pts',(4.43434348814969,6.81185945239664,98.8996135834406));
#170974=CARTESIAN_POINT('Ctrl Pts',(4.25463135912899,6.92552886226729,98.9079383468321));
#170975=CARTESIAN_POINT('Ctrl Pts',(4.07073537364008,7.03198414960496,98.9162631102236));
#170976=CARTESIAN_POINT('Ctrl Pts',(3.88683996800717,7.1384391012706,98.9245878473657));
#170977=CARTESIAN_POINT('Ctrl Pts',(3.69876097291084,7.23767983421501,98.9329125845077));
#170978=CARTESIAN_POINT('Ctrl Pts',(3.50707849817467,7.32939888190982,98.9412373216498));
#170979=CARTESIAN_POINT('Ctrl Pts',(3.31541142408727,7.42111056047585,98.9495613899443));
#170980=CARTESIAN_POINT('Ctrl Pts',(3.12014170101451,7.50530164139812,98.9578854582389));
#170981=CARTESIAN_POINT('Ctrl Pts',(2.92187192055566,7.58171168288325,98.9662095265334));
#170982=CARTESIAN_POINT('Ctrl Pts',(2.72360002813004,7.65812253828702,98.9745336834958));
#170983=CARTESIAN_POINT('Ctrl Pts',(2.52232827478524,7.7267520876479,98.9828578404582));
#170984=CARTESIAN_POINT('Ctrl Pts',(2.31867805317345,7.78738849989082,98.9911819974205));
#170985=CARTESIAN_POINT('Ctrl Pts',(2.24676734046914,7.80879975879204,98.9941213316137));
#170986=CARTESIAN_POINT('Ctrl Pts',(2.17456021842664,7.82921483522134,98.9970606658068));
#170987=CARTESIAN_POINT('Ctrl Pts',(2.10208451021631,7.8486258844723,99.));
#170988=CARTESIAN_POINT('',(-2.10208451021626,7.84862588447232,99.));
#170989=CARTESIAN_POINT('Origin',(0.,0.,99.));
#170990=CARTESIAN_POINT('',(8.13159794993647,-0.00671758913982503,98.4167025567874));
#170991=CARTESIAN_POINT('Ctrl Pts',(8.12525,-4.14083309504467E-12,98.4167025567874));
#170992=CARTESIAN_POINT('Ctrl Pts',(8.12525000000114,2.24624642432976,98.5047001499286));
#170993=CARTESIAN_POINT('Ctrl Pts',(7.14398562317847,4.47535249753047,98.5926977430698));
#170994=CARTESIAN_POINT('Ctrl Pts',(3.83078204045389,7.50935546634122,98.7686929293522));
#170995=CARTESIAN_POINT('Ctrl Pts',(1.52412477698275,8.29110090552034,98.8566905224934));
#170996=CARTESIAN_POINT('Ctrl Pts',(-1.1822624975838,8.05254244492327,98.9631254104231));
#170997=CARTESIAN_POINT('Ctrl Pts',(-1.6474727139843,7.97038381115747,98.9815627052115));
#170998=CARTESIAN_POINT('Ctrl Pts',(-2.10208451021626,7.84862588447232,
99.));
#170999=CARTESIAN_POINT('',(8.13064101234909,0.00726150239357421,96.4167025567874));
#171000=CARTESIAN_POINT('Ctrl Pts',(8.13064101234909,0.00726150239357421,
96.4167025567874));
#171001=CARTESIAN_POINT('Ctrl Pts',(8.13264513995559,0.458958580512804,
96.4344080025745));
#171002=CARTESIAN_POINT('Ctrl Pts',(7.88034319623196,3.60392890591984,96.5578917585526));
#171003=CARTESIAN_POINT('Ctrl Pts',(4.76217654495404,7.59287955017989,96.734264669626));
#171004=CARTESIAN_POINT('Ctrl Pts',(-0.787795848183394,8.42010700031842,
96.945821290008));
#171005=CARTESIAN_POINT('Ctrl Pts',(-4.70369331914029,7.04503919375108,
97.1044887552944));
#171006=CARTESIAN_POINT('Ctrl Pts',(-7.50785040472023,3.92613790885546,
97.2631562205808));
#171007=CARTESIAN_POINT('Ctrl Pts',(-8.46487839372023,-0.13681273072905,
97.4218236858673));
#171008=CARTESIAN_POINT('Ctrl Pts',(-7.37643864316404,-4.16414405786197,
97.5804911511536));
#171009=CARTESIAN_POINT('Ctrl Pts',(-4.4775289435207,-7.19508636046639,
97.7391586164401));
#171010=CARTESIAN_POINT('Ctrl Pts',(-0.510988490918713,-8.43710679026292,
97.8978260817266));
#171011=CARTESIAN_POINT('Ctrl Pts',(4.99171475646089,-7.44423893657541,
98.1093827021084));
#171012=CARTESIAN_POINT('Ctrl Pts',(7.94889191739487,-3.41866176302103,
98.2823415271287));
#171013=CARTESIAN_POINT('Ctrl Pts',(8.13566645843371,-0.371006238498034,
98.4024111970536));
#171014=CARTESIAN_POINT('Ctrl Pts',(8.13267765453462,-0.00786016460921045,
98.4167025567874));
#171015=CARTESIAN_POINT('',(8.12524935171145,-0.00324576840847315,92.4142818892175));
#171016=CARTESIAN_POINT('Ctrl Pts',(8.1252466584585,0.00736896933301007,
96.4135943073787));
#171017=CARTESIAN_POINT('Ctrl Pts',(8.12590323294949,-0.716589761930001,
96.3874241345655));
#171018=CARTESIAN_POINT('Ctrl Pts',(8.02980597704607,-1.43739644121946,
96.3618774763689));
#171019=CARTESIAN_POINT('Ctrl Pts',(7.8200332504233,-2.20731470784607,96.3315156398167));
#171020=CARTESIAN_POINT('Ctrl Pts',(7.79961632700026,-2.27840804917313,
96.3286862987029));
#171021=CARTESIAN_POINT('Ctrl Pts',(7.76661022777492,-2.38769110653584,
96.3242963068922));
#171022=CARTESIAN_POINT('Ctrl Pts',(7.75470334917227,-2.42608309630499,
96.3227462405774));
#171023=CARTESIAN_POINT('Ctrl Pts',(7.73176683133274,-2.49814418573916,
96.3198219929881));
#171024=CARTESIAN_POINT('Ctrl Pts',(7.72080088515683,-2.53183261314967,
96.3184487876053));
#171025=CARTESIAN_POINT('Ctrl Pts',(7.70225148961179,-2.58757675261307,
96.3161663991105));
#171026=CARTESIAN_POINT('Ctrl Pts',(7.69479275609644,-2.60967352283208,
96.3152590113286));
#171027=CARTESIAN_POINT('Ctrl Pts',(7.68014130838278,-2.65247002760309,
96.3134964652409));
#171028=CARTESIAN_POINT('Ctrl Pts',(7.67295977493772,-2.67317340499203,
96.3126414793574));
#171029=CARTESIAN_POINT('Ctrl Pts',(7.65650346900041,-2.7200019720856,96.3107021738355));
#171030=CARTESIAN_POINT('Ctrl Pts',(7.64717857877076,-2.74610922487601,
96.3096171501307));
#171031=CARTESIAN_POINT('Ctrl Pts',(7.61915204229363,-2.82332634622982,
96.3063961535349));
#171032=CARTESIAN_POINT('Ctrl Pts',(7.60007038372069,-2.87429636535933,
96.3042545846267));
#171033=CARTESIAN_POINT('Ctrl Pts',(7.41331266597301,-3.35828907136431,
96.2837624747453));
#171034=CARTESIAN_POINT('Ctrl Pts',(7.20932935675875,-3.77635202364663,
96.2647893508854));
#171035=CARTESIAN_POINT('Ctrl Pts',(6.8412628694122,-4.3909394887513,96.234717312196));
#171036=CARTESIAN_POINT('Ctrl Pts',(6.70175925037647,-4.60104848629454,
96.224014954117));
#171037=CARTESIAN_POINT('Ctrl Pts',(6.44179153901747,-4.95562344431865,
96.205359532329));
#171038=CARTESIAN_POINT('Ctrl Pts',(6.32565802367751,-5.10303183711418,
96.197410431286));
#171039=CARTESIAN_POINT('Ctrl Pts',(6.05620881317575,-5.42169601839635,
96.179927731469));
#171040=CARTESIAN_POINT('Ctrl Pts',(5.90051415337845,-5.59074179858677,
96.1704456528119));
#171041=CARTESIAN_POINT('Ctrl Pts',(5.7225002426769,-5.76828823659543,96.1604235084261));
#171042=CARTESIAN_POINT('Ctrl Pts',(5.70707847459305,-5.78354679268849,
96.1595616849925));
#171043=CARTESIAN_POINT('Ctrl Pts',(5.68587522695687,-5.80435825180994,
96.1583857334037));
#171044=CARTESIAN_POINT('Ctrl Pts',(5.68014644055117,-5.8099645632584,96.1580688994498));
#171045=CARTESIAN_POINT('Ctrl Pts',(5.66936982645228,-5.82047961161557,
96.1574745757998));
#171046=CARTESIAN_POINT('Ctrl Pts',(5.66432389844026,-5.82539027982304,
96.1571969864832));
#171047=CARTESIAN_POINT('Ctrl Pts',(5.65382391381546,-5.83558226338742,
96.1566207997966));
#171048=CARTESIAN_POINT('Ctrl Pts',(5.64836882349238,-5.84086250783859,
96.1563222585658));
#171049=CARTESIAN_POINT('Ctrl Pts',(5.63578987717447,-5.85300417313695,
96.1556357201409));
#171050=CARTESIAN_POINT('Ctrl Pts',(5.62866086873989,-5.8598602556906,96.1552480073913));
#171051=CARTESIAN_POINT('Ctrl Pts',(5.60649334221101,-5.88110134668094,
96.1540467335736));
#171052=CARTESIAN_POINT('Ctrl Pts',(5.59141199376807,-5.89544167748034,
96.1532356037871));
#171053=CARTESIAN_POINT('Ctrl Pts',(5.41788291487671,-6.05917960744128,
96.1439742893054));
#171054=CARTESIAN_POINT('Ctrl Pts',(5.25355147410591,-6.20220189559256,
96.1359314263433));
#171055=CARTESIAN_POINT('Ctrl Pts',(4.84747804800057,-6.52788759979342,
96.1173597964537));
#171056=CARTESIAN_POINT('Ctrl Pts',(4.60087263335696,-6.70397974772862,
96.1070744403398));
#171057=CARTESIAN_POINT('Ctrl Pts',(4.13040137264405,-7.00171208689419,
96.0883128421078));
#171058=CARTESIAN_POINT('Ctrl Pts',(3.90954649251,-7.12738614042152,96.0798226996423));
#171059=CARTESIAN_POINT('Ctrl Pts',(3.19746122590257,-7.48951635998182,
96.052668199623));
#171060=CARTESIAN_POINT('Ctrl Pts',(2.68819152705082,-7.6870125316506,96.0334640924608));
#171061=CARTESIAN_POINT('Ctrl Pts',(2.13580299627479,-7.83956823180263,
96.0113870163092));
#171062=CARTESIAN_POINT('Ctrl Pts',(2.10855277275215,-7.84694142233613,
96.010295155754));
#171063=CARTESIAN_POINT('Ctrl Pts',(2.06878924091098,-7.85747829832295,
96.0086977673924));
#171064=CARTESIAN_POINT('Ctrl Pts',(2.05630581943573,-7.86075444897327,
96.008195687338));
#171065=CARTESIAN_POINT('Ctrl Pts',(2.03440785833882,-7.86644562008079,
96.0073139038205));
#171066=CARTESIAN_POINT('Ctrl Pts',(2.02499667797925,-7.86887352046825,
96.0069345954987));
#171067=CARTESIAN_POINT('Ctrl Pts',(2.00673251509985,-7.87355038139605,
96.0061978105488));
#171068=CARTESIAN_POINT('Ctrl Pts',(1.99788004914798,-7.87580131187464,
96.0058403948314));
#171069=CARTESIAN_POINT('Ctrl Pts',(1.97676499633044,-7.88113237866811,
96.0049871528677));
#171070=CARTESIAN_POINT('Ctrl Pts',(1.96449899570235,-7.88419882517905,
96.0044909091146));
#171071=CARTESIAN_POINT('Ctrl Pts',(1.92747884955554,-7.8933619443263,96.0029914101063));
#171072=CARTESIAN_POINT('Ctrl Pts',(1.90270322619867,-7.8993707292612,96.0019854758301));
#171073=CARTESIAN_POINT('Ctrl Pts',(1.64789176958249,-7.95990134213067,
95.9916146223507));
#171074=CARTESIAN_POINT('Ctrl Pts',(1.41562248159417,-8.00447238686052,
95.981947227185));
#171075=CARTESIAN_POINT('Ctrl Pts',(0.539940577329719,-8.13320200119173,
95.9446926258298));
#171076=CARTESIAN_POINT('Ctrl Pts',(-0.110812074463072,-8.15034131647273,
95.9151948725943));
#171077=CARTESIAN_POINT('Ctrl Pts',(-1.06398572468673,-8.06120031822383,
95.8721806059189));
#171078=CARTESIAN_POINT('Ctrl Pts',(-1.36952570606803,-8.01495071254373,
95.8584649652962));
#171079=CARTESIAN_POINT('Ctrl Pts',(-1.78268547537017,-7.92808812187126,
95.8405488891613));
#171080=CARTESIAN_POINT('Ctrl Pts',(-1.89316991355354,-7.90243369382721,
95.8358215702062));
#171081=CARTESIAN_POINT('Ctrl Pts',(-2.04153632824587,-7.86469269397984,
95.829588414464));
#171082=CARTESIAN_POINT('Ctrl Pts',(-2.0799146307956,-7.85463028701927,
95.8279868684712));
#171083=CARTESIAN_POINT('Ctrl Pts',(-2.14535436763218,-7.83695937141752,
95.8252738552663));
#171084=CARTESIAN_POINT('Ctrl Pts',(-2.17245126433044,-7.82949124049688,
95.8241555805646));
#171085=CARTESIAN_POINT('Ctrl Pts',(-2.2100709004257,-7.81891261939912,
95.8226094801085));
#171086=CARTESIAN_POINT('Ctrl Pts',(-2.22062670359331,-7.81592124957927,
95.8221763623739));
#171087=CARTESIAN_POINT('Ctrl Pts',(-2.23759642112233,-7.81107511140476,
95.8214811656711));
#171088=CARTESIAN_POINT('Ctrl Pts',(-2.24401414208078,-7.80923380814827,
95.8212185030776));
#171089=CARTESIAN_POINT('Ctrl Pts',(-2.25740695536677,-7.80537341379034,
95.8206708778199));
#171090=CARTESIAN_POINT('Ctrl Pts',(-2.26438162754039,-7.80335287784375,
95.8203859771821));
#171091=CARTESIAN_POINT('Ctrl Pts',(-2.28045233928751,-7.79867389339832,
95.8197301725536));
#171092=CARTESIAN_POINT('Ctrl Pts',(-2.28954646550092,-7.79600887317518,
95.819359545004));
#171093=CARTESIAN_POINT('Ctrl Pts',(-2.31855225387609,-7.78745363875872,
95.8181789013846));
#171094=CARTESIAN_POINT('Ctrl Pts',(-2.33844609857104,-7.7815029771781,
95.8173713693193));
#171095=CARTESIAN_POINT('Ctrl Pts',(-2.52903151197649,-7.72369805045132,
95.8096546258882));
#171096=CARTESIAN_POINT('Ctrl Pts',(-2.69800142772722,-7.66630973680929,
95.802962131267));
#171097=CARTESIAN_POINT('Ctrl Pts',(-3.47677344769397,-7.37286968249113,
95.7722967750393));
#171098=CARTESIAN_POINT('Ctrl Pts',(-4.05855087043088,-7.06932897060372,
95.7496177583046));
#171099=CARTESIAN_POINT('Ctrl Pts',(-4.82773779382544,-6.54144401680282,
95.7152881181103));
#171100=CARTESIAN_POINT('Ctrl Pts',(-5.04950289487799,-6.37181725099528,
95.7048394886654));
#171101=CARTESIAN_POINT('Ctrl Pts',(-5.46136646771455,-6.02175694730635,
95.6842685184291));
#171102=CARTESIAN_POINT('Ctrl Pts',(-5.65234061166466,-5.8428693511192,
95.674204185728));
#171103=CARTESIAN_POINT('Ctrl Pts',(-5.88810219951548,-5.59963431937994,
95.6610633949834));
#171104=CARTESIAN_POINT('Ctrl Pts',(-5.94105980101686,-5.54341594685729,
95.6580593110513));
#171105=CARTESIAN_POINT('Ctrl Pts',(-6.02242793716618,-5.45453224050368,
95.6533576607653));
#171106=CARTESIAN_POINT('Ctrl Pts',(-6.05139265876349,-5.42238020533149,
95.6516664509385));
#171107=CARTESIAN_POINT('Ctrl Pts',(-6.10496004389695,-5.36195439734099,
95.6485051141478));
#171108=CARTESIAN_POINT('Ctrl Pts',(-6.12962663208127,-5.33373878579804,
95.6470357581051));
#171109=CARTESIAN_POINT('Ctrl Pts',(-6.1843747156451,-5.27023217599949,
95.6437433563248));
#171110=CARTESIAN_POINT('Ctrl Pts',(-6.21435105878343,-5.23485230983879,
95.6419191858602));
#171111=CARTESIAN_POINT('Ctrl Pts',(-6.30111174685808,-5.13065669283656,
95.6365751930641));
#171112=CARTESIAN_POINT('Ctrl Pts',(-6.35706724401277,-5.06116026460026,
95.6330463751458));
#171113=CARTESIAN_POINT('Ctrl Pts',(-6.74188379643628,-4.56676783870095,
95.6081770383364));
#171114=CARTESIAN_POINT('Ctrl Pts',(-7.02902650934413,-4.11109780259688,
95.5863854270459));
#171115=CARTESIAN_POINT('Ctrl Pts',(-7.41043995555299,-3.34741080956153,
95.5517012850208));
#171116=CARTESIAN_POINT('Ctrl Pts',(-7.53514955309206,-3.05635517404504,
95.5388792982535));
#171117=CARTESIAN_POINT('Ctrl Pts',(-7.66091133206201,-2.7079591785244,
95.524146037038));
#171118=CARTESIAN_POINT('Ctrl Pts',(-7.67874457654431,-2.65696954202366,
95.5220048793949));
#171119=CARTESIAN_POINT('Ctrl Pts',(-7.70358968506312,-2.58359121735076,
95.5189464652119));
#171120=CARTESIAN_POINT('Ctrl Pts',(-7.71101503735957,-2.5613443179146,
95.5180222118676));
#171121=CARTESIAN_POINT('Ctrl Pts',(-7.72400475790899,-2.52185769139282,
95.5163871683278));
#171122=CARTESIAN_POINT('Ctrl Pts',(-7.72960797905781,-2.50463095261046,
95.5156756759298));
#171123=CARTESIAN_POINT('Ctrl Pts',(-7.74173907873626,-2.46690623495975,
95.5141213702457));
#171124=CARTESIAN_POINT('Ctrl Pts',(-7.74824326129995,-2.44640076508538,
95.513278957571));
#171125=CARTESIAN_POINT('Ctrl Pts',(-7.76628925959023,-2.38871395249166,
95.51091547035));
#171126=CARTESIAN_POINT('Ctrl Pts',(-7.77764542408482,-2.35147504561999,
95.5093972287453));
#171127=CARTESIAN_POINT('Ctrl Pts',(-7.85579281893262,-2.08845505861087,
95.4987203323771));
#171128=CARTESIAN_POINT('Ctrl Pts',(-7.91301066549013,-1.8599435527455,
95.4896807333021));
#171129=CARTESIAN_POINT('Ctrl Pts',(-7.99359042092224,-1.4662496660108,
95.4742337862524));
#171130=CARTESIAN_POINT('Ctrl Pts',(-8.02194070821344,-1.30224529989528,
95.4678368104537));
#171131=CARTESIAN_POINT('Ctrl Pts',(-8.06021267316544,-1.03155473030517,
95.4572760987396));
#171132=CARTESIAN_POINT('Ctrl Pts',(-8.07309627064354,-0.925337709988211,
95.4531318298419));
#171133=CARTESIAN_POINT('Ctrl Pts',(-8.08845378160931,-0.773733624426063,
95.4472060347446));
#171134=CARTESIAN_POINT('Ctrl Pts',(-8.09265033258577,-0.728531998548076,
95.4454379120988));
#171135=CARTESIAN_POINT('Ctrl Pts',(-8.09647177983796,-0.683251259024802,
95.4436649748077));
#171136=CARTESIAN_POINT('Ctrl Pts',(-8.09647569822461,-0.683204824873072,
95.4436631567075));
#171137=CARTESIAN_POINT('Ctrl Pts',(-8.09648353815878,-0.683111909572502,
95.4436595186634));
#171138=CARTESIAN_POINT('Ctrl Pts',(-8.09648745969328,-0.683065428568405,
95.4436576987251));
#171139=CARTESIAN_POINT('Ctrl Pts',(-8.0964953058797,-0.682972420049493,
95.4436540570239));
#171140=CARTESIAN_POINT('Ctrl Pts',(-8.09649923055314,-0.682925892269909,
95.4436522352505));
#171141=CARTESIAN_POINT('Ctrl Pts',(-8.09650708306364,-0.682832789623486,
95.4436485898565));
#171142=CARTESIAN_POINT('Ctrl Pts',(-8.0965110108964,-0.68278621479787,
95.4436467662375));
#171143=CARTESIAN_POINT('Ctrl Pts',(-8.0965188697338,-0.682693017932335,
95.4436431171471));
#171144=CARTESIAN_POINT('Ctrl Pts',(-8.09652280073543,-0.682646395918386,
95.4436412916768));
#171145=CARTESIAN_POINT('Ctrl Pts',(-8.09653066593017,-0.682553104414559,
95.4436376388736));
#171146=CARTESIAN_POINT('Ctrl Pts',(-8.09653460011634,-0.682506434997056,
95.4436358115436));
#171147=CARTESIAN_POINT('Ctrl Pts',(-8.09654247168501,-0.682413048599427,
95.4436321550175));
#171148=CARTESIAN_POINT('Ctrl Pts',(-8.09654640906959,-0.682366331584664,
95.4436303258202));
#171149=CARTESIAN_POINT('Ctrl Pts',(-8.09655428701372,-0.682272850216289,
95.4436266655683));
#171150=CARTESIAN_POINT('Ctrl Pts',(-8.09655822759182,-0.682226085632625,
95.4436248345047));
#171151=CARTESIAN_POINT('Ctrl Pts',(-8.09656611197868,-0.682132508436122,
95.4436211704934));
#171152=CARTESIAN_POINT('Ctrl Pts',(-8.096570055774,-0.682085695972843,
95.4436193375514));
#171153=CARTESIAN_POINT('Ctrl Pts',(-8.09657794661128,-0.681992022797499,
95.4436156697747));
#171154=CARTESIAN_POINT('Ctrl Pts',(-8.09658189364436,-0.681945162180716,
95.4436138349436));
#171155=CARTESIAN_POINT('Ctrl Pts',(-8.09658979091413,-0.6818513931797,
95.4436101634075));
#171156=CARTESIAN_POINT('Ctrl Pts',(-8.09659374117379,-0.681804484512607,
95.4436083266913));
#171157=CARTESIAN_POINT('Ctrl Pts',(-8.09660164495274,-0.681710618715257,
95.4436046513577));
#171158=CARTESIAN_POINT('Ctrl Pts',(-8.09660559845918,-0.681663661727685,
95.4436028127458));
#171159=CARTESIAN_POINT('Ctrl Pts',(-8.09661350875774,-0.681569698950048,
95.4435991336075));
#171160=CARTESIAN_POINT('Ctrl Pts',(-8.0966174655273,-0.68152269341782,
95.4435972930912));
#171161=CARTESIAN_POINT('Ctrl Pts',(-8.0966253823785,-0.681428633206755,
95.4435936101305));
#171162=CARTESIAN_POINT('Ctrl Pts',(-8.09662934244232,-0.681381578729407,
95.443591767694));
#171163=CARTESIAN_POINT('Ctrl Pts',(-8.09663726578714,-0.681287421725458,
95.4435880809358));
#171164=CARTESIAN_POINT('Ctrl Pts',(-8.09664122911381,-0.681240318645962,
95.4435862365926));
#171165=CARTESIAN_POINT('Ctrl Pts',(-8.09664915908324,-0.681146063231411,
95.4435825459737));
#171166=CARTESIAN_POINT('Ctrl Pts',(-8.09665312570642,-0.68109891111903,
95.4435806997068));
#171167=CARTESIAN_POINT('Ctrl Pts',(-8.09666106229329,-0.681004557317679,
95.4435770052281));
#171168=CARTESIAN_POINT('Ctrl Pts',(-8.09666503223838,-0.680957355839471,
95.4435751570246));
#171169=CARTESIAN_POINT('Ctrl Pts',(-8.09667297541666,-0.680862903899152,
95.4435714586957));
#171170=CARTESIAN_POINT('Ctrl Pts',(-8.09667694867352,-0.680815653145048,
95.4435696085589));
#171171=CARTESIAN_POINT('Ctrl Pts',(-8.0966848985099,-0.68072110221058,
95.4435659063464));
#171172=CARTESIAN_POINT('Ctrl Pts',(-8.09668887509022,-0.680673802010453,
95.4435640542698));
#171173=CARTESIAN_POINT('Ctrl Pts',(-8.09669683162049,-0.680579151594057,
95.4435603481544));
#171174=CARTESIAN_POINT('Ctrl Pts',(-8.09670081154848,-0.680531801628782,
95.4435584941255));
#171175=CARTESIAN_POINT('Ctrl Pts',(-8.0967087747729,-0.680437051664694,
95.4435547841047));
#171176=CARTESIAN_POINT('Ctrl Pts',(-8.09671275806207,-0.680389651741915,
95.4435529281159));
#171177=CARTESIAN_POINT('Ctrl Pts',(-8.09672072799703,-0.680294801972369,
95.4435492141796));
#171178=CARTESIAN_POINT('Ctrl Pts',(-8.09672471465569,-0.680247351961756,
95.4435473562257));
#171179=CARTESIAN_POINT('Ctrl Pts',(-8.09673269131513,-0.680152402157842,
95.443543638365));
#171180=CARTESIAN_POINT('Ctrl Pts',(-8.0967366813387,-0.680104902082411,
95.443541778447));
#171181=CARTESIAN_POINT('Ctrl Pts',(-8.09969937347417,-0.644831188649415,
95.4421605957805));
#171182=CARTESIAN_POINT('Ctrl Pts',(-8.10242815214566,-0.609586115160366,
95.4407794897809));
#171183=CARTESIAN_POINT('Ctrl Pts',(-8.10767547243135,-0.535535378499249,
95.4378752338732));
#171184=CARTESIAN_POINT('Ctrl Pts',(-8.11014560882525,-0.496727186674533,
95.4363517322204));
#171185=CARTESIAN_POINT('Ctrl Pts',(-8.11601353655642,-0.392769310157494,
95.4322663123271));
#171186=CARTESIAN_POINT('Ctrl Pts',(-8.11890543664851,-0.327594114750407,
95.4297004439459));
#171187=CARTESIAN_POINT('Ctrl Pts',(-8.13336579607254,0.119953897322484,
95.412046417264));
#171188=CARTESIAN_POINT('Ctrl Pts',(-8.11870198341614,0.50269035343553,
95.3967416973508));
#171189=CARTESIAN_POINT('Ctrl Pts',(-8.06543350083459,0.989980035517573,
95.3771830144089));
#171190=CARTESIAN_POINT('Ctrl Pts',(-8.05160841328838,1.0967589566312,95.3728951412479));
#171191=CARTESIAN_POINT('Ctrl Pts',(-8.02586100660651,1.26871045561272,
95.3660016895167));
#171192=CARTESIAN_POINT('Ctrl Pts',(-8.01525648259005,1.33406698911411,
95.3633843337835));
#171193=CARTESIAN_POINT('Ctrl Pts',(-7.9994898779356,1.42425121339564,95.3597800762875));
#171194=CARTESIAN_POINT('Ctrl Pts',(-7.99500866816353,1.44919502921509,
95.3587839786189));
#171195=CARTESIAN_POINT('Ctrl Pts',(-7.98719229398234,1.49156345442184,
95.3570936327472));
#171196=CARTESIAN_POINT('Ctrl Pts',(-7.98391664570556,1.50899876618673,
95.3563984641469));
#171197=CARTESIAN_POINT('Ctrl Pts',(-7.9769079915668,1.54564204504393,95.3549382289603));
#171198=CARTESIAN_POINT('Ctrl Pts',(-7.97316264757994,1.56484754383909,
95.3541733410966));
#171199=CARTESIAN_POINT('Ctrl Pts',(-7.96242996028624,1.61884400481386,
95.3520238756442));
#171200=CARTESIAN_POINT('Ctrl Pts',(-7.955284011717,1.65360306387427,95.3506414014832));
#171201=CARTESIAN_POINT('Ctrl Pts',(-7.92152226232347,1.81253991893322,
95.3443231450896));
#171202=CARTESIAN_POINT('Ctrl Pts',(-7.89222490437997,1.9361307983205,95.3394186260104));
#171203=CARTESIAN_POINT('Ctrl Pts',(-7.76599481349782,2.41800604682047,
95.3202443616812));
#171204=CARTESIAN_POINT('Ctrl Pts',(-7.6474592633979,2.77016187275368,95.3061005780106));
#171205=CARTESIAN_POINT('Ctrl Pts',(-7.43132567193435,3.29125120820879,
95.2843655672264));
#171206=CARTESIAN_POINT('Ctrl Pts',(-7.3510559341734,3.46683014989748,95.2768985738719));
#171207=CARTESIAN_POINT('Ctrl Pts',(-7.23194987155557,3.70457905097755,
95.2665478925648));
#171208=CARTESIAN_POINT('Ctrl Pts',(-7.19841218491012,3.76933241301281,
95.2637037068278));
#171209=CARTESIAN_POINT('Ctrl Pts',(-7.13809656030164,3.88204598050795,
95.258707328456));
#171210=CARTESIAN_POINT('Ctrl Pts',(-7.11169539030135,3.93020255814595,
95.2565577823005));
#171211=CARTESIAN_POINT('Ctrl Pts',(-7.05397386699905,4.03300218201322,
95.2519367070545));
#171212=CARTESIAN_POINT('Ctrl Pts',(-7.02250226796445,4.08755621092475,
95.2494643844854));
#171213=CARTESIAN_POINT('Ctrl Pts',(-6.91427230551962,4.27022603855155,
95.2411179796271));
#171214=CARTESIAN_POINT('Ctrl Pts',(-6.83461714547703,4.39658959981555,
95.2352295324915));
#171215=CARTESIAN_POINT('Ctrl Pts',(-6.65960295658383,4.65796869777095,
95.2228131515243));
#171216=CARTESIAN_POINT('Ctrl Pts',(-6.56351490662453,4.79241652527088,
95.2162864868903));
#171217=CARTESIAN_POINT('Ctrl Pts',(-6.42775307631851,4.97062744775441,
95.2074634203575));
#171218=CARTESIAN_POINT('Ctrl Pts',(-6.39160423582731,5.01702523015997,
95.2051499608261));
#171219=CARTESIAN_POINT('Ctrl Pts',(-6.33036988774553,5.0938846952232,95.2012918220174));
#171220=CARTESIAN_POINT('Ctrl Pts',(-6.30556060766926,5.12456336074595,
95.199744962259));
#171221=CARTESIAN_POINT('Ctrl Pts',(-6.24762565895189,5.19514684473642,
95.1961695235155));
#171222=CARTESIAN_POINT('Ctrl Pts',(-6.21433944867187,5.23491760704113,
95.1941423124497));
#171223=CARTESIAN_POINT('Ctrl Pts',(-6.10786546506377,5.35968728106748,
95.1877378617262));
#171224=CARTESIAN_POINT('Ctrl Pts',(-6.03329717802386,5.44349093541879,
95.1833695156871));
#171225=CARTESIAN_POINT('Ctrl Pts',(-5.88609241158617,5.60218532463918,
95.1749415368995));
#171226=CARTESIAN_POINT('Ctrl Pts',(-5.81370153745601,5.67727387934029,
95.1708825601207));
#171227=CARTESIAN_POINT('Ctrl Pts',(-5.65943182347899,5.83124683678178,
95.162389623468));
#171228=CARTESIAN_POINT('Ctrl Pts',(-5.57730232749082,5.9098482930487,95.1579556725355));
#171229=CARTESIAN_POINT('Ctrl Pts',(-5.44962052375443,6.02701241512375,
95.1511790849693));
#171230=CARTESIAN_POINT('Ctrl Pts',(-5.40524763783641,6.0668394118841,95.1488447130368));
#171231=CARTESIAN_POINT('Ctrl Pts',(-5.31891794921337,6.14262584314597,
95.1443404496858));
#171232=CARTESIAN_POINT('Ctrl Pts',(-5.27702473755612,6.1786527894317,95.1421711646499));
#171233=CARTESIAN_POINT('Ctrl Pts',(-5.18365868673933,6.25730260170525,
95.1373711044285));
#171234=CARTESIAN_POINT('Ctrl Pts',(-5.13202091270545,6.29972336946721,
95.1347390177204));
#171235=CARTESIAN_POINT('Ctrl Pts',(-4.93175045715165,6.46015019304431,
95.1246131489552));
#171236=CARTESIAN_POINT('Ctrl Pts',(-4.77952493669337,6.57357158384015,
95.1170863150176));
#171237=CARTESIAN_POINT('Ctrl Pts',(-4.32507020188464,6.88804277716103,
95.0950678291337));
#171238=CARTESIAN_POINT('Ctrl Pts',(-4.01317549494579,7.07430462955483,
95.080495768673));
#171239=CARTESIAN_POINT('Ctrl Pts',(-3.60800429955195,7.28082671597766,
95.0623615316293));
#171240=CARTESIAN_POINT('Ctrl Pts',(-3.52542687275876,7.32116781878217,
95.0587060951519));
#171241=CARTESIAN_POINT('Ctrl Pts',(-3.38597464468263,7.38638704813591,
95.0526073617842));
#171242=CARTESIAN_POINT('Ctrl Pts',(-3.32946715488126,7.41202984761432,
95.050156187515));
#171243=CARTESIAN_POINT('Ctrl Pts',(-3.24806490347128,7.44785100967987,
95.0466559682243));
#171244=CARTESIAN_POINT('Ctrl Pts',(-3.22340493779451,7.45855689085699,
95.0455996331649));
#171245=CARTESIAN_POINT('Ctrl Pts',(-3.18032740412013,7.47700503459374,
95.043761587596));
#171246=CARTESIAN_POINT('Ctrl Pts',(-3.16193359357418,7.48480211080803,
95.0429790389893));
#171247=CARTESIAN_POINT('Ctrl Pts',(-3.1235081682538,7.50092359890265,95.0413491381858));
#171248=CARTESIAN_POINT('Ctrl Pts',(-3.10347165885324,7.5092357654427,95.040502024169));
#171249=CARTESIAN_POINT('Ctrl Pts',(-3.0444300571406,7.53345256294429,95.0380138856426));
#171250=CARTESIAN_POINT('Ctrl Pts',(-3.00533425258843,7.54913425173881,
95.0363764995468));
#171251=CARTESIAN_POINT('Ctrl Pts',(-2.74863991589329,7.64978658672482,
95.0256852153991));
#171252=CARTESIAN_POINT('Ctrl Pts',(-2.52758281196608,7.72564456057991,
95.0167526446114));
#171253=CARTESIAN_POINT('Ctrl Pts',(-2.04671251289425,7.86780741645244,
94.9975645396818));
#171254=CARTESIAN_POINT('Ctrl Pts',(-1.78626711341502,7.93099449377891,
94.9873164200191));
#171255=CARTESIAN_POINT('Ctrl Pts',(-1.44585530767933,7.99596065016857,
94.9739108887133));
#171256=CARTESIAN_POINT('Ctrl Pts',(-1.3683215638532,8.00959301578285,94.9708575019063));
#171257=CARTESIAN_POINT('Ctrl Pts',(-1.24954969227803,8.02870114455305,
94.9661765923732));
#171258=CARTESIAN_POINT('Ctrl Pts',(-1.20844706839709,8.0349904895875,94.9645560735697));
#171259=CARTESIAN_POINT('Ctrl Pts',(-1.13264788598394,8.04599417519215,
94.9615660063421));
#171260=CARTESIAN_POINT('Ctrl Pts',(-1.09796561301865,8.05080027097469,
94.9601972742627));
#171261=CARTESIAN_POINT('Ctrl Pts',(-1.0211671471473,8.06093712508518,94.9571648308177));
#171262=CARTESIAN_POINT('Ctrl Pts',(-0.979038083830723,8.06616229003021,
94.9555002698122));
#171263=CARTESIAN_POINT('Ctrl Pts',(-0.856303813839657,8.08040900753404,
94.9506474181269));
#171264=CARTESIAN_POINT('Ctrl Pts',(-0.775602394193254,8.08855405842972,
94.9474520872307));
#171265=CARTESIAN_POINT('Ctrl Pts',(-0.406408244422184,8.12024003497157,
94.9328123847811));
#171266=CARTESIAN_POINT('Ctrl Pts',(-0.116909428030769,8.12956301390118,
94.9212618277416));
#171267=CARTESIAN_POINT('Ctrl Pts',(0.281740298828503,8.12109946594301,
94.9053632595044));
#171268=CARTESIAN_POINT('Ctrl Pts',(0.390958505417069,8.11657475468431,
94.9010096705924));
#171269=CARTESIAN_POINT('Ctrl Pts',(0.566854802641656,8.10572900577889,
94.894016491461));
#171270=CARTESIAN_POINT('Ctrl Pts',(0.633604033701103,8.10078472093421,
94.8913670282648));
#171271=CARTESIAN_POINT('Ctrl Pts',(0.726642104956197,8.09273617007723,
94.8876837515468));
#171272=CARTESIAN_POINT('Ctrl Pts',(0.752988148194098,8.0903273309966,94.88664182752));
#171273=CARTESIAN_POINT('Ctrl Pts',(0.798211765801853,8.08596968056625,
94.8848555120846));
#171274=CARTESIAN_POINT('Ctrl Pts',(0.817095116096069,8.08408332912075,
94.8841102783764));
#171275=CARTESIAN_POINT('Ctrl Pts',(0.853511011673782,8.08031666665382,
94.8826745090915));
#171276=CARTESIAN_POINT('Ctrl Pts',(0.871044324734877,8.07844541150655,
94.8819838605976));
#171277=CARTESIAN_POINT('Ctrl Pts',(0.921407366838671,8.07290451278525,
94.8800018239735));
#171278=CARTESIAN_POINT('Ctrl Pts',(0.954221023103633,8.0690917123435,94.8787125978143));
#171279=CARTESIAN_POINT('Ctrl Pts',(1.10800008849012,8.05027211079362,94.8726791656735));
#171280=CARTESIAN_POINT('Ctrl Pts',(1.22864227339502,8.03274448791166,94.8679702986353));
#171281=CARTESIAN_POINT('Ctrl Pts',(1.58501303494683,7.97275215785025,94.8540817451467));
#171282=CARTESIAN_POINT('Ctrl Pts',(1.81930956446794,7.92257269153464,94.8449770189337));
#171283=CARTESIAN_POINT('Ctrl Pts',(2.32696808158619,7.79013607267649,94.8250480010857));
#171284=CARTESIAN_POINT('Ctrl Pts',(2.5989059435904,7.70368010921243,94.8142386929617));
#171285=CARTESIAN_POINT('Ctrl Pts',(3.12709995054024,7.50459529657127,94.7926694079061));
#171286=CARTESIAN_POINT('Ctrl Pts',(3.38320886979333,7.39267194894809,94.7819271511611));
#171287=CARTESIAN_POINT('Ctrl Pts',(3.69387781346811,7.23737384150959,94.7684261477287));
#171288=CARTESIAN_POINT('Ctrl Pts',(3.75432948736774,7.20620034820655,94.765776331066));
#171289=CARTESIAN_POINT('Ctrl Pts',(3.850939100764,7.1548354113467,94.761503587549));
#171290=CARTESIAN_POINT('Ctrl Pts',(3.88734660059467,7.13512004901262,94.7598845911873));
#171291=CARTESIAN_POINT('Ctrl Pts',(3.95671804393681,7.0968655099599,94.7567825561497));
#171292=CARTESIAN_POINT('Ctrl Pts',(3.98970638033427,7.07837274617624,94.7552999200764));
#171293=CARTESIAN_POINT('Ctrl Pts',(4.06491559190419,7.03551879784878,94.7519022339171));
#171294=CARTESIAN_POINT('Ctrl Pts',(4.10704873066683,7.01100664858279,94.7499860799305));
#171295=CARTESIAN_POINT('Ctrl Pts',(4.24271967082099,6.93043354519203,94.7437741323328));
#171296=CARTESIAN_POINT('Ctrl Pts',(4.33534975960675,6.8728685116897,94.739467788866));
#171297=CARTESIAN_POINT('Ctrl Pts',(4.76649515019372,6.59274767078643,94.7191108638013));
#171298=CARTESIAN_POINT('Ctrl Pts',(5.08920770188082,6.34694821485646,94.7029974764005));
#171299=CARTESIAN_POINT('Ctrl Pts',(5.84015940178961,5.6807365926197,94.662012329591));
#171300=CARTESIAN_POINT('Ctrl Pts',(6.24276819395873,5.23507364640062,94.6365790495493));
#171301=CARTESIAN_POINT('Ctrl Pts',(6.72648419142853,4.56360235496574,94.6016761490449));
#171302=CARTESIAN_POINT('Ctrl Pts',(6.85234395463876,4.37234990882098,94.5920973275313));
#171303=CARTESIAN_POINT('Ctrl Pts',(7.01952575433701,4.09331704746116,94.5788339501143));
#171304=CARTESIAN_POINT('Ctrl Pts',(7.06761128704567,4.009720411998,94.5749476346757));
#171305=CARTESIAN_POINT('Ctrl Pts',(7.12215451680144,3.91086612333966,94.5704695204145));
#171306=CARTESIAN_POINT('Ctrl Pts',(7.13006690067068,3.89642205011866,94.5698181037515));
#171307=CARTESIAN_POINT('Ctrl Pts',(7.14210059287212,3.8742951218012,94.5688247402399));
#171308=CARTESIAN_POINT('Ctrl Pts',(7.14625351839712,3.86662956863853,94.5684814351066));
#171309=CARTESIAN_POINT('Ctrl Pts',(7.15346440586678,3.85326826844846,94.5678845091736));
#171310=CARTESIAN_POINT('Ctrl Pts',(7.15652791804543,3.84757553703061,94.5676306445625));
#171311=CARTESIAN_POINT('Ctrl Pts',(7.16339195976932,3.83478396139085,94.5670612582654));
#171312=CARTESIAN_POINT('Ctrl Pts',(7.16718874073074,3.82768310537471,94.5667459041681));
#171313=CARTESIAN_POINT('Ctrl Pts',(7.17728865322545,3.80872622340325,94.5659059675328));
#171314=CARTESIAN_POINT('Ctrl Pts',(7.18357297842651,3.79686016637839,94.5653822425539));
#171315=CARTESIAN_POINT('Ctrl Pts',(7.21032472243658,3.74604338286372,94.5631482354486));
#171316=CARTESIAN_POINT('Ctrl Pts',(7.23050524338887,3.7069418205877,94.5614514707266));
#171317=CARTESIAN_POINT('Ctrl Pts',(7.63411789193703,2.90906910721405,94.5273088781268));
#171318=CARTESIAN_POINT('Ctrl Pts',(7.89648214933574,2.09484259389513,94.5009850141658));
#171319=CARTESIAN_POINT('Ctrl Pts',(8.07363102489509,0.96139863034817,94.4617702264432));
#171320=CARTESIAN_POINT('Ctrl Pts',(8.10336069915064,0.665835163129001,
94.4513593883833));
#171321=CARTESIAN_POINT('Ctrl Pts',(8.12247881749743,0.245659908234986,
94.4359580657802));
#171322=CARTESIAN_POINT('Ctrl Pts',(8.12527858156364,0.121891094380435,
94.4313492978148));
#171323=CARTESIAN_POINT('Ctrl Pts',(8.1252332658565,-0.072864439355185,
94.4239667210359));
#171324=CARTESIAN_POINT('Ctrl Pts',(8.12428682139369,-0.143833922092723,
94.4212492996346));
#171325=CARTESIAN_POINT('Ctrl Pts',(8.12190662599008,-0.233846238165964,
94.4177663800555));
#171326=CARTESIAN_POINT('Ctrl Pts',(8.12133535770459,-0.25290967991097,
94.4170266757545));
#171327=CARTESIAN_POINT('Ctrl Pts',(8.12032423101039,-0.283100611339073,
94.4158518892959));
#171328=CARTESIAN_POINT('Ctrl Pts',(8.11992860419081,-0.294229560947777,
94.415418128088));
#171329=CARTESIAN_POINT('Ctrl Pts',(8.11915015033784,-0.314928777814457,
94.4146100232922));
#171330=CARTESIAN_POINT('Ctrl Pts',(8.11877327746063,-0.324499256181384,
94.4142358580493));
#171331=CARTESIAN_POINT('Ctrl Pts',(8.11790158491443,-0.345682695317728,
94.4134064955145));
#171332=CARTESIAN_POINT('Ctrl Pts',(8.1173987667325,-0.357295296209357,
94.4129510603431));
#171333=CARTESIAN_POINT('Ctrl Pts',(8.11588010550233,-0.390709641093286,
94.4116383104904));
#171334=CARTESIAN_POINT('Ctrl Pts',(8.11480133861701,-0.412508346953228,
94.4107791214638));
#171335=CARTESIAN_POINT('Ctrl Pts',(8.10703866270235,-0.557530630675659,
94.405044428367));
#171336=CARTESIAN_POINT('Ctrl Pts',(8.09763627391413,-0.680589024523087,
94.4000881387693));
#171337=CARTESIAN_POINT('Ctrl Pts',(8.06176860241798,-1.04156995842637,
94.3852779332295));
#171338=CARTESIAN_POINT('Ctrl Pts',(8.02758980488776,-1.27858188876243,
94.3752023186942));
#171339=CARTESIAN_POINT('Ctrl Pts',(7.81307519824032,-2.40987468887371,
94.3255475141545));
#171340=CARTESIAN_POINT('Ctrl Pts',(7.49350086006586,-3.27091119580164,
94.2822853649384));
#171341=CARTESIAN_POINT('Ctrl Pts',(7.00532913730159,-4.11694644894432,
94.2423841397797));
#171342=CARTESIAN_POINT('Ctrl Pts',(6.97228242873576,-4.17266846676819,
94.2397740537291));
#171343=CARTESIAN_POINT('Ctrl Pts',(6.93112003065592,-4.24022025374476,
94.2366265371217));
#171344=CARTESIAN_POINT('Ctrl Pts',(6.92363524047266,-4.2524308036738,94.2360582552634));
#171345=CARTESIAN_POINT('Ctrl Pts',(6.91122116218759,-4.27256324248015,
94.2351222806942));
#171346=CARTESIAN_POINT('Ctrl Pts',(6.90631046280093,-4.28049651395868,
94.2347537118338));
#171347=CARTESIAN_POINT('Ctrl Pts',(6.89742671745897,-4.2947931867569,94.2340899416659));
#171348=CARTESIAN_POINT('Ctrl Pts',(6.89345850748529,-4.30115956990539,
94.2337945168686));
#171349=CARTESIAN_POINT('Ctrl Pts',(6.88496503773944,-4.31474409098104,
94.2331644575491));
#171350=CARTESIAN_POINT('Ctrl Pts',(6.88043722869696,-4.32196062964471,
94.2328299399603));
#171351=CARTESIAN_POINT('Ctrl Pts',(6.86818393447519,-4.34142218949823,
94.2319282952375));
#171352=CARTESIAN_POINT('Ctrl Pts',(6.8604370369424,-4.35365373573406,94.2313621300092));
#171353=CARTESIAN_POINT('Ctrl Pts',(6.82215501104413,-4.41374117244007,
94.2285831039246));
#171354=CARTESIAN_POINT('Ctrl Pts',(6.79115122845628,-4.46129749096856,
94.22639069999));
#171355=CARTESIAN_POINT('Ctrl Pts',(6.70285863101587,-4.59367494919469,
94.2202981938675));
#171356=CARTESIAN_POINT('Ctrl Pts',(6.64446106022355,-4.67774533402821,
94.2164408622603));
#171357=CARTESIAN_POINT('Ctrl Pts',(6.43096925963876,-4.97302482563275,
94.2028668817703));
#171358=CARTESIAN_POINT('Ctrl Pts',(6.26726346875171,-5.17781396450533,
94.1933996026619));
#171359=CARTESIAN_POINT('Ctrl Pts',(5.92489875760565,-5.56602018377624,
94.1747875683099));
#171360=CARTESIAN_POINT('Ctrl Pts',(5.74690339065847,-5.7496179843282,94.165650643581));
#171361=CARTESIAN_POINT('Ctrl Pts',(5.3910381932999,-6.08362082766119,94.1479920296429));
#171362=CARTESIAN_POINT('Ctrl Pts',(5.21477807264227,-6.23536856154968,
94.1394982494472));
#171363=CARTESIAN_POINT('Ctrl Pts',(4.8381545563583,-6.53246263267437,94.1216622920368));
#171364=CARTESIAN_POINT('Ctrl Pts',(4.63717106284379,-6.67663432112402,
94.1123091392343));
#171365=CARTESIAN_POINT('Ctrl Pts',(4.39311393318093,-6.83536147940509,
94.1010899685688));
#171366=CARTESIAN_POINT('Ctrl Pts',(4.35610178846738,-6.85900821973032,
94.0993923208304));
#171367=CARTESIAN_POINT('Ctrl Pts',(4.29534189896328,-6.89713701925577,
94.0966115677212));
#171368=CARTESIAN_POINT('Ctrl Pts',(4.27170820958984,-6.91179933556675,
94.0955314432904));
#171369=CARTESIAN_POINT('Ctrl Pts',(4.22928543454946,-6.9378176856726,94.0935953092474));
#171370=CARTESIAN_POINT('Ctrl Pts',(4.21052468321154,-6.94921948233819,
94.092740028724));
#171371=CARTESIAN_POINT('Ctrl Pts',(4.17173426726248,-6.9725795043319,94.0909735593724));
#171372=CARTESIAN_POINT('Ctrl Pts',(4.15169882130206,-6.9845278031663,94.0900622149974));
#171373=CARTESIAN_POINT('Ctrl Pts',(4.10115709014258,-7.01437445927886,
94.0877656505479));
#171374=CARTESIAN_POINT('Ctrl Pts',(4.07058494189238,-7.03216017636156,
94.0863786758069));
#171375=CARTESIAN_POINT('Ctrl Pts',(3.94875606315176,-7.10197492393839,
94.0808591977956));
#171376=CARTESIAN_POINT('Ctrl Pts',(3.85661123412561,-7.15243116349059,
94.0767011405074));
#171377=CARTESIAN_POINT('Ctrl Pts',(3.03413836426582,-7.58228146716365,
94.0396804542716));
#171378=CARTESIAN_POINT('Ctrl Pts',(2.25109561383592,-7.85043173666986,
94.0043734641504));
#171379=CARTESIAN_POINT('Ctrl Pts',(1.2238566220196,-8.03558922964224,93.9605762016838));
#171380=CARTESIAN_POINT('Ctrl Pts',(1.00486508784383,-8.06590183130673,
93.9514256666622));
#171381=CARTESIAN_POINT('Ctrl Pts',(0.747756819237211,-8.09085534487136,
93.9410599513374));
#171382=CARTESIAN_POINT('Ctrl Pts',(0.710584905970697,-8.09420469320021,
93.9395705587599));
#171383=CARTESIAN_POINT('Ctrl Pts',(0.660535048642772,-8.09836696056611,
93.9375786350616));
#171384=CARTESIAN_POINT('Ctrl Pts',(0.647676623964324,-8.09940547024974,
93.937068079694));
#171385=CARTESIAN_POINT('Ctrl Pts',(0.627485652389728,-8.10098780264962,
93.936268303769));
#171386=CARTESIAN_POINT('Ctrl Pts',(0.620154775668397,-8.10155230047332,
93.9359783217586));
#171387=CARTESIAN_POINT('Ctrl Pts',(0.606073814318241,-8.10261734922504,
93.9354221078431));
#171388=CARTESIAN_POINT('Ctrl Pts',(0.599323852732836,-8.10311941762201,
93.9351558191581));
#171389=CARTESIAN_POINT('Ctrl Pts',(0.583455715296596,-8.10427976842575,
93.9345306306485));
#171390=CARTESIAN_POINT('Ctrl Pts',(0.574337029812911,-8.10493109863662,
93.9341719967785));
#171391=CARTESIAN_POINT('Ctrl Pts',(0.547927951585274,-8.10677265596026,
93.9331352060121));
#171392=CARTESIAN_POINT('Ctrl Pts',(0.530634761879627,-8.10792295788589,
93.932458611154));
#171393=CARTESIAN_POINT('Ctrl Pts',(0.404434256397985,-8.11591202734003,
93.927538503479));
#171394=CARTESIAN_POINT('Ctrl Pts',(0.295409099186309,-8.12061141652878,
93.9233889791688));
#171395=CARTESIAN_POINT('Ctrl Pts',(0.0266944833661381,-8.12677461621692,
93.9133972613159));
#171396=CARTESIAN_POINT('Ctrl Pts',(-0.133000664167659,-8.12573028806315,
93.9076530519118));
#171397=CARTESIAN_POINT('Ctrl Pts',(-0.925489891047017,-8.09717654579639,
93.8797352788387));
#171398=CARTESIAN_POINT('Ctrl Pts',(-1.55359212828043,-8.00045124508917,
93.8593338913361));
#171399=CARTESIAN_POINT('Ctrl Pts',(-2.5669517980104,-7.72043559500461,
93.8229183591905));
#171400=CARTESIAN_POINT('Ctrl Pts',(-2.96057603497608,-7.57821302013632,
93.8078575081775));
#171401=CARTESIAN_POINT('Ctrl Pts',(-3.37018115486437,-7.39341307223594,
93.7905737100953));
#171402=CARTESIAN_POINT('Ctrl Pts',(-3.39879044657238,-7.38030496303748,
93.7893579635739));
#171403=CARTESIAN_POINT('Ctrl Pts',(-3.43863913486979,-7.36176638054491,
93.7876524704381));
#171404=CARTESIAN_POINT('Ctrl Pts',(-3.44994341229048,-7.35647563660229,
93.7871672862622));
#171405=CARTESIAN_POINT('Ctrl Pts',(-3.46946135796356,-7.34728576517244,
93.7863271860817));
#171406=CARTESIAN_POINT('Ctrl Pts',(-3.47768076844247,-7.34339885214269,
93.7859726704121));
#171407=CARTESIAN_POINT('Ctrl Pts',(-3.49469654455405,-7.33531721166527,
93.785237230924));
#171408=CARTESIAN_POINT('Ctrl Pts',(-3.50349192052005,-7.33112043935655,
93.7848562403534));
#171409=CARTESIAN_POINT('Ctrl Pts',(-3.52405914931612,-7.32126118335225,
93.7839633398338));
#171410=CARTESIAN_POINT('Ctrl Pts',(-3.53582492371385,-7.31558612208675,
93.7834510167629));
#171411=CARTESIAN_POINT('Ctrl Pts',(-3.57373005254434,-7.2971902920139,
93.7817955433889));
#171412=CARTESIAN_POINT('Ctrl Pts',(-3.59981470389926,-7.28435767399418,
93.7806487070129));
#171413=CARTESIAN_POINT('Ctrl Pts',(-3.9806586433076,-7.09445228318185,
93.7637918859624));
#171414=CARTESIAN_POINT('Ctrl Pts',(-4.32202417190279,-6.89180312107808,
93.7472113603622));
#171415=CARTESIAN_POINT('Ctrl Pts',(-5.35582661542184,-6.17098547215181,
93.6923617589405));
#171416=CARTESIAN_POINT('Ctrl Pts',(-5.9810578857684,-5.56711215960124,
93.65147926183));
#171417=CARTESIAN_POINT('Ctrl Pts',(-6.56121040277545,-4.79382970037055,
93.6113784162077));
#171418=CARTESIAN_POINT('Ctrl Pts',(-6.62141984317476,-4.71031706230643,
93.6071941109172));
#171419=CARTESIAN_POINT('Ctrl Pts',(-6.68893916914521,-4.61281097844696,
93.602479341619));
#171420=CARTESIAN_POINT('Ctrl Pts',(-6.6978087358599,-4.59992287697257,
93.6018593950244));
#171421=CARTESIAN_POINT('Ctrl Pts',(-6.71195693504179,-4.57923687220886,
93.6008693966906));
#171422=CARTESIAN_POINT('Ctrl Pts',(-6.71725930432266,-4.57145531195093,
93.6004981225444));
#171423=CARTESIAN_POINT('Ctrl Pts',(-6.72662176390864,-4.55766385445949,
93.599842085078));
#171424=CARTESIAN_POINT('Ctrl Pts',(-6.73068735077529,-4.55165771466889,
93.5995570458177));
#171425=CARTESIAN_POINT('Ctrl Pts',(-6.73910400100001,-4.53918776197313,
93.5989666043461));
#171426=CARTESIAN_POINT('Ctrl Pts',(-6.7434538206387,-4.53272311576684,
93.5986612634594));
#171427=CARTESIAN_POINT('Ctrl Pts',(-6.75462518272094,-4.51606870712732,
93.5978765493515));
#171428=CARTESIAN_POINT('Ctrl Pts',(-6.76143298355118,-4.5058697204403,
93.5973978385143));
#171429=CARTESIAN_POINT('Ctrl Pts',(-6.78961615049801,-4.46343990869116,
93.5954137742493));
#171430=CARTESIAN_POINT('Ctrl Pts',(-6.81078454885842,-4.43107178677248,
93.5939180595367));
#171431=CARTESIAN_POINT('Ctrl Pts',(-6.86515137274642,-4.34663061976467,
93.5900590667336));
#171432=CARTESIAN_POINT('Ctrl Pts',(-6.89798895671689,-4.2943276168054,
93.5877108036029));
#171433=CARTESIAN_POINT('Ctrl Pts',(-7.04314236925637,-4.05716871209813,
93.577229270678));
#171434=CARTESIAN_POINT('Ctrl Pts',(-7.14864941012239,-3.86824118229549,
93.5693262882223));
#171435=CARTESIAN_POINT('Ctrl Pts',(-7.56785470962135,-3.04171028794821,
93.5358419613534));
#171436=CARTESIAN_POINT('Ctrl Pts',(-7.80472498575103,-2.36869735521673,
93.5108373021046));
#171437=CARTESIAN_POINT('Ctrl Pts',(-8.0183415847571,-1.35374603969443,
93.4717992870617));
#171438=CARTESIAN_POINT('Ctrl Pts',(-8.06628519510275,-1.0302730025906,
93.4592708228089));
#171439=CARTESIAN_POINT('Ctrl Pts',(-8.10311417159392,-0.607296120265727,
93.4428388472676));
#171440=CARTESIAN_POINT('Ctrl Pts',(-8.10984176995107,-0.50964116556756,
93.4390384032802));
#171441=CARTESIAN_POINT('Ctrl Pts',(-8.11720153840767,-0.36464320963158,
93.4333794374685));
#171442=CARTESIAN_POINT('Ctrl Pts',(-8.11918696823725,-0.317377433393139,
93.4315322361271));
#171443=CARTESIAN_POINT('Ctrl Pts',(-8.12200815554881,-0.232555421971376,
93.4282120569847));
#171444=CARTESIAN_POINT('Ctrl Pts',(-8.12299644940413,-0.195005572077664,
93.4267404082097));
#171445=CARTESIAN_POINT('Ctrl Pts',(-8.12455100979448,-0.114797281414313,
93.4235925806025));
#171446=CARTESIAN_POINT('Ctrl Pts',(-8.12504175627157,-0.0721385205948915,
93.4219158029972));
#171447=CARTESIAN_POINT('Ctrl Pts',(-8.12546471906561,0.0444452697352801,
93.4173254997582));
#171448=CARTESIAN_POINT('Ctrl Pts',(-8.12472406330371,0.118368394972371,
93.4144063378893));
#171449=CARTESIAN_POINT('Ctrl Pts',(-8.1138633632295,0.577206721251773,
93.3962277407092));
#171450=CARTESIAN_POINT('Ctrl Pts',(-8.0774013825832,0.961000135856553,
93.3807452545336));
#171451=CARTESIAN_POINT('Ctrl Pts',(-7.9563401258764,1.68460155556326,93.3509908422658));
#171452=CARTESIAN_POINT('Ctrl Pts',(-7.8767416614841,2.02439433972723,93.3367772490979));
#171453=CARTESIAN_POINT('Ctrl Pts',(-7.76034705011079,2.40820496382675,
93.320592431989));
#171454=CARTESIAN_POINT('Ctrl Pts',(-7.74464305493016,2.45823950714455,
93.3184801617431));
#171455=CARTESIAN_POINT('Ctrl Pts',(-7.72520492050419,2.51813570075325,
93.3159495198298));
#171456=CARTESIAN_POINT('Ctrl Pts',(-7.72193461703842,2.52814640432777,
93.3155264940729));
#171457=CARTESIAN_POINT('Ctrl Pts',(-7.69125067105442,2.621457837397,93.3115828109803));
#171458=CARTESIAN_POINT('Ctrl Pts',(-7.66250936697679,2.70431664497324,
93.3080764784248));
#171459=CARTESIAN_POINT('Ctrl Pts',(-7.61515553168986,2.83401329190045,
93.3025866425489));
#171460=CARTESIAN_POINT('Ctrl Pts',(-7.59743910679157,2.88117062755141,
93.3005902508787));
#171461=CARTESIAN_POINT('Ctrl Pts',(-7.57095594309598,2.94971996315994,
93.2976888327562));
#171462=CARTESIAN_POINT('Ctrl Pts',(-7.56253470836174,2.9712439388512,93.2967778962677));
#171463=CARTESIAN_POINT('Ctrl Pts',(-7.5473820500382,3.00949110558663,93.2951594834198));
#171464=CARTESIAN_POINT('Ctrl Pts',(-7.54068660591185,3.02622835188119,
93.29445135279));
#171465=CARTESIAN_POINT('Ctrl Pts',(-7.5339286368954,3.04296021285256,93.2937434592611));
#171466=CARTESIAN_POINT('Ctrl Pts',(-7.53392176892502,3.0429772168973,93.2937427398521));
#171467=CARTESIAN_POINT('Ctrl Pts',(-7.53390802701265,3.04301123943888,
93.2937413004224));
#171468=CARTESIAN_POINT('Ctrl Pts',(-7.53390116345209,3.04302823223383,
93.2937405814893));
#171469=CARTESIAN_POINT('Ctrl Pts',(-7.53388744434638,3.04306219764829,
93.2937391444767));
#171470=CARTESIAN_POINT('Ctrl Pts',(-7.53388058877827,3.04307917032505,
93.2937384263947));
#171471=CARTESIAN_POINT('Ctrl Pts',(-7.53386688496685,3.04311309721399,
93.2937369910121));
#171472=CARTESIAN_POINT('Ctrl Pts',(-7.53386003709493,3.04313005050709,
93.2937362737502));
#171473=CARTESIAN_POINT('Ctrl Pts',(-7.53384634929344,3.04316393710107,
93.2937348400724));
#171474=CARTESIAN_POINT('Ctrl Pts',(-7.53383950929199,3.04318087058025,
93.2937341236489));
#171475=CARTESIAN_POINT('Ctrl Pts',(-7.53382583714785,3.04321471775445,
93.2937326916389));
#171476=CARTESIAN_POINT('Ctrl Pts',(-7.53381900506374,3.04323163130483,
93.2937319760585));
#171477=CARTESIAN_POINT('Ctrl Pts',(-7.53380534828561,3.04326543978276,
93.2937305456857));
#171478=CARTESIAN_POINT('Ctrl Pts',(-7.5337985239722,3.0432823337685,93.2937298309331));
#171479=CARTESIAN_POINT('Ctrl Pts',(-7.53378488270275,3.04331610319926,
93.2937284022123));
#171480=CARTESIAN_POINT('Ctrl Pts',(-7.53377806606017,3.04333297786868,
93.293727688277));
#171481=CARTESIAN_POINT('Ctrl Pts',(-7.53376444057693,3.04336670756748,
93.2937262612372));
#171482=CARTESIAN_POINT('Ctrl Pts',(-7.53375763173327,3.04338356260467,
93.2937255481325));
#171483=CARTESIAN_POINT('Ctrl Pts',(-7.5337440216806,3.04341725345418,93.2937241227364));
#171484=CARTESIAN_POINT('Ctrl Pts',(-7.53373722058697,3.04343408898129,
93.2937234104571));
#171485=CARTESIAN_POINT('Ctrl Pts',(-7.53372362601295,3.04346774086474,
93.2937219867097));
#171486=CARTESIAN_POINT('Ctrl Pts',(-7.5337168326701,3.04348455688104,93.2937212752559));
#171487=CARTESIAN_POINT('Ctrl Pts',(-7.53370325345981,3.04351817008514,
93.2937198531449));
#171488=CARTESIAN_POINT('Ctrl Pts',(-7.53369646780441,3.04353496674849,
93.2937191425099));
#171489=CARTESIAN_POINT('Ctrl Pts',(-7.53368290404449,3.04356854106103,
93.2937177220444));
#171490=CARTESIAN_POINT('Ctrl Pts',(-7.53367612608663,3.04358531834758,
93.2937170122293));
#171491=CARTESIAN_POINT('Ctrl Pts',(-7.53366257774988,3.04361885383813,
93.2937155934063));
#171492=CARTESIAN_POINT('Ctrl Pts',(-7.5336558075323,3.04363561164321,93.2937148844153));
#171493=CARTESIAN_POINT('Ctrl Pts',(-7.53364227424431,3.04366910924071,
93.2937134671956));
#171494=CARTESIAN_POINT('Ctrl Pts',(-7.53363551152804,3.04368584815693,
93.2937127590038));
#171495=CARTESIAN_POINT('Ctrl Pts',(-7.53362199400518,3.04371930609046,
93.2937113434621));
#171496=CARTESIAN_POINT('Ctrl Pts',(-7.53361523907891,3.04373602540438,
93.2937106360997));
#171497=CARTESIAN_POINT('Ctrl Pts',(-7.53360173638902,3.04376944598339,
93.2937092221385));
#171498=CARTESIAN_POINT('Ctrl Pts',(-7.53359498894672,3.04378614645354,
93.2937085155734));
#171499=CARTESIAN_POINT('Ctrl Pts',(-7.53358150188086,3.04381952772228,
93.2937071032754));
#171500=CARTESIAN_POINT('Ctrl Pts',(-7.53357476215167,3.04383620878266,
93.2937063975314));
#171501=CARTESIAN_POINT('Ctrl Pts',(-7.53356129005246,3.04386955237036,
93.2937049868276));
#171502=CARTESIAN_POINT('Ctrl Pts',(-7.53355455788635,3.04388621439336,
93.2937042818891));
#171503=CARTESIAN_POINT('Ctrl Pts',(-7.53354110106289,3.0439195195372,93.2937028728118));
#171504=CARTESIAN_POINT('Ctrl Pts',(-7.53353437651803,3.04393616237999,
93.2937021686848));
#171505=CARTESIAN_POINT('Ctrl Pts',(-7.5335209347308,3.04396942967493,93.2937007612089));
#171506=CARTESIAN_POINT('Ctrl Pts',(-7.53351421773309,3.04398605352197,
93.2937000578856));
#171507=CARTESIAN_POINT('Ctrl Pts',(-7.53350079106562,3.04401928276345,
93.2936986520197));
#171508=CARTESIAN_POINT('Ctrl Pts',(-7.5334940815995,3.04403588765431,93.2936979494984));
#171509=CARTESIAN_POINT('Ctrl Pts',(-7.5334806699575,3.04406907907789,93.2936965452325));
#171510=CARTESIAN_POINT('Ctrl Pts',(-7.53347396794667,3.04408566520247,
93.2936958435052));
#171511=CARTESIAN_POINT('Ctrl Pts',(-7.53346057167164,3.04411881796512,
93.293694440875));
#171512=CARTESIAN_POINT('Ctrl Pts',(-7.53345387735365,3.04413538473669,
93.2936937399664));
#171513=CARTESIAN_POINT('Ctrl Pts',(-7.5334404955451,3.04416850106907,93.2936923388775));
#171514=CARTESIAN_POINT('Ctrl Pts',(-7.53343380854309,3.04418504942125,
93.2936916387484));
#171515=CARTESIAN_POINT('Ctrl Pts',(-7.53342044229823,3.04421812661023,
93.2936902393156));
#171516=CARTESIAN_POINT('Ctrl Pts',(-7.53341376300435,3.04423465557371,
93.2936895400067));
#171517=CARTESIAN_POINT('Ctrl Pts',(-7.53340041099827,3.04426769690014,
93.2936881420912));
#171518=CARTESIAN_POINT('Ctrl Pts',(-7.53339373891981,3.0442842076952,93.293687443551));
#171519=CARTESIAN_POINT('Ctrl Pts',(-7.53338040236975,3.04431721014898,
93.2936860472802));
#171520=CARTESIAN_POINT('Ctrl Pts',(-7.5333737377875,3.04433370208186,93.293685349538));
#171521=CARTESIAN_POINT('Ctrl Pts',(-7.53336041606794,3.04436666721303,
93.2936839548463));
#171522=CARTESIAN_POINT('Ctrl Pts',(-7.53335375896608,3.04438314032396,
93.2936832579005));
#171523=CARTESIAN_POINT('Ctrl Pts',(-7.53334045205952,3.04441606817795,
93.2936818647859));
#171524=CARTESIAN_POINT('Ctrl Pts',(-7.53333380243665,3.04443252247144,
93.2936811686362));
#171525=CARTESIAN_POINT('Ctrl Pts',(-7.53332051012661,3.04446541358601,
93.293679777076));
#171526=CARTESIAN_POINT('Ctrl Pts',(-7.53331386781142,3.04448184948703,
93.2936790817045));
#171527=CARTESIAN_POINT('Ctrl Pts',(-7.53330059049022,3.04451470289351,
93.2936776917397));
#171528=CARTESIAN_POINT('Ctrl Pts',(-7.53329395558048,3.04453112016114,
93.2936769971565));
#171529=CARTESIAN_POINT('Ctrl Pts',(-7.53328069287546,3.04456393678375,
93.293675608748));
#171530=CARTESIAN_POINT('Ctrl Pts',(-7.53327406524153,3.04458033573985,
93.2936749149395));
#171531=CARTESIAN_POINT('Ctrl Pts',(-7.52657141531173,3.06116475031661,
93.2929732601048));
#171532=CARTESIAN_POINT('Ctrl Pts',(-7.51982074033722,3.07771066445389,
93.2922732403024));
#171533=CARTESIAN_POINT('Ctrl Pts',(-7.49951067364812,3.127024916758,93.2901866287043));
#171534=CARTESIAN_POINT('Ctrl Pts',(-7.48579124759548,3.15972698015247,
93.2888026046292));
#171535=CARTESIAN_POINT('Ctrl Pts',(-7.39070595606194,3.3822797751389,93.2793770520012));
#171536=CARTESIAN_POINT('Ctrl Pts',(-7.30233962994029,3.56905993468778,
93.2714309709452));
#171537=CARTESIAN_POINT('Ctrl Pts',(-7.08218215340431,3.99191428040401,
93.2531022773816));
#171538=CARTESIAN_POINT('Ctrl Pts',(-6.94553881460965,4.22518318161648,
93.2427307725261));
#171539=CARTESIAN_POINT('Ctrl Pts',(-6.76205928680134,4.50537835645699,
93.2297410019823));
#171540=CARTESIAN_POINT('Ctrl Pts',(-6.72594237976424,4.55912041745257,
93.2272245664502));
#171541=CARTESIAN_POINT('Ctrl Pts',(-6.66718866589827,4.6443282195857,93.2231923978165));
#171542=CARTESIAN_POINT('Ctrl Pts',(-6.64496230267298,4.67607370568202,
93.2216805845555));
#171543=CARTESIAN_POINT('Ctrl Pts',(-6.60200696473175,4.73650122382074,
93.2187840203165));
#171544=CARTESIAN_POINT('Ctrl Pts',(-6.58131603353919,4.76520923592443,
93.2173996678754));
#171545=CARTESIAN_POINT('Ctrl Pts',(-6.56040309806832,4.79382923735388,
93.216011118566));
#171546=CARTESIAN_POINT('Ctrl Pts',(-6.56036792838607,4.79387736704315,
93.2160087834459));
#171547=CARTESIAN_POINT('Ctrl Pts',(-6.56029763279905,4.79397356429252,
93.2160041161725));
#171548=CARTESIAN_POINT('Ctrl Pts',(-6.56026248621184,4.7940216601561,93.2160017826458));
#171549=CARTESIAN_POINT('Ctrl Pts',(-6.56019220978094,4.79411782675084,
93.2159971167638));
#171550=CARTESIAN_POINT('Ctrl Pts',(-6.56015707951682,4.79416589805838,
93.2159947843805));
#171551=CARTESIAN_POINT('Ctrl Pts',(-6.56008683542515,4.79426201596438,
93.215990120765));
#171552=CARTESIAN_POINT('Ctrl Pts',(-6.56005172133166,4.79431006292779,
93.215987789515));
#171553=CARTESIAN_POINT('Ctrl Pts',(-6.5599815094794,4.79440613228813,93.2159831281591));
#171554=CARTESIAN_POINT('Ctrl Pts',(-6.5599464114472,4.79445415506026,93.215980798035));
#171555=CARTESIAN_POINT('Ctrl Pts',(-6.55987623167614,4.79455017609793,
93.2159761389281));
#171556=CARTESIAN_POINT('Ctrl Pts',(-6.55984114962487,4.79459817479195,
93.2159738099246));
#171557=CARTESIAN_POINT('Ctrl Pts',(-6.55977100166118,4.79469414788804,
93.2159691530484));
#171558=CARTESIAN_POINT('Ctrl Pts',(-6.55973593545178,4.79474212269744,
93.215966825156));
#171559=CARTESIAN_POINT('Ctrl Pts',(-6.55966581925036,4.79483804792005,
93.2159621705072));
#171560=CARTESIAN_POINT('Ctrl Pts',(-6.55963076885347,4.79488599888819,
93.215959843724));
#171561=CARTESIAN_POINT('Ctrl Pts',(-6.55956068405944,4.79498187672919,
93.215955191279));
#171562=CARTESIAN_POINT('Ctrl Pts',(-6.55952564935839,4.79502980401886,
93.215952865597));
#171563=CARTESIAN_POINT('Ctrl Pts',(-6.55945559577165,4.79512563475832,
93.2159482153423));
#171564=CARTESIAN_POINT('Ctrl Pts',(-6.55942057662666,4.79517353856386,
93.2159458907522));
#171565=CARTESIAN_POINT('Ctrl Pts',(-6.55935055413489,4.79526932236171,
93.2159412426802));
#171566=CARTESIAN_POINT('Ctrl Pts',(-6.55931555044835,4.79531720281978,
93.2159389191756));
#171567=CARTESIAN_POINT('Ctrl Pts',(-6.55924555892839,4.79541293985073,
93.2159342732778));
#171568=CARTESIAN_POINT('Ctrl Pts',(-6.5592105706757,4.79546079699811,93.2159319508569));
#171569=CARTESIAN_POINT('Ctrl Pts',(-6.55914060973929,4.79555648779942,
93.2159273071075));
#171570=CARTESIAN_POINT('Ctrl Pts',(-6.55910563677732,4.79560432183497,
93.2159249857606));
#171571=CARTESIAN_POINT('Ctrl Pts',(-6.55903570622705,4.79569996668282,
93.2159203441463));
#171572=CARTESIAN_POINT('Ctrl Pts',(-6.5590007483651,4.7957477778704,93.2159180238608));
#171573=CARTESIAN_POINT('Ctrl Pts',(-6.55893084837131,4.79584337653794,
93.2159133843927));
#171574=CARTESIAN_POINT('Ctrl Pts',(-6.55889590569035,4.7958911647699,93.2159110651738));
#171575=CARTESIAN_POINT('Ctrl Pts',(-6.55882603562209,4.79598671812613,
93.21590642781));
#171576=CARTESIAN_POINT('Ctrl Pts',(-6.55879110794696,4.79603448364502,
93.2159041096459));
#171577=CARTESIAN_POINT('Ctrl Pts',(-6.55872126770312,4.79612999183424,
93.2158994743794));
#171578=CARTESIAN_POINT('Ctrl Pts',(-6.55868635487444,4.79617773486104,
93.2158971572597));
#171579=CARTESIAN_POINT('Ctrl Pts',(-6.55861654444349,4.79627319790501,
93.2158925240896));
#171580=CARTESIAN_POINT('Ctrl Pts',(-6.5585816464217,4.79632091849682,93.2158902080113));
#171581=CARTESIAN_POINT('Ctrl Pts',(-6.55851186551032,4.79641633680261,
93.215885576918));
#171582=CARTESIAN_POINT('Ctrl Pts',(-6.55847698221643,4.7964640350704,93.215883261876));
#171583=CARTESIAN_POINT('Ctrl Pts',(-6.55840723056912,4.7965594089933,93.2158786328423));
#171584=CARTESIAN_POINT('Ctrl Pts',(-6.55837236188042,4.7966070851078,93.2158763188283));
#171585=CARTESIAN_POINT('Ctrl Pts',(-6.55830263938441,4.79670241480788,
93.2158716918466));
#171586=CARTESIAN_POINT('Ctrl Pts',(-6.55826778523327,4.7967500688645,93.2158693788561));
#171587=CARTESIAN_POINT('Ctrl Pts',(-6.55819809156584,4.79684535478884,
93.2158647539048));
#171588=CARTESIAN_POINT('Ctrl Pts',(-6.55816325178624,4.79689298701748,
93.2158624419266));
#171589=CARTESIAN_POINT('Ctrl Pts',(-6.55809358692053,4.7969882292086,93.2158578190038));
#171590=CARTESIAN_POINT('Ctrl Pts',(-6.55805876144252,4.79703583970777,
93.2158555080332));
#171591=CARTESIAN_POINT('Ctrl Pts',(-6.55798912515072,4.79713103848287,
93.2158508871237));
#171592=CARTESIAN_POINT('Ctrl Pts',(-6.55795431389782,4.79717862736001,
93.2158485771555));
#171593=CARTESIAN_POINT('Ctrl Pts',(-6.55788470595877,4.79727378302717,
93.2158439582443));
#171594=CARTESIAN_POINT('Ctrl Pts',(-6.55784990884646,4.79732135040067,
93.2158416492729));
#171595=CARTESIAN_POINT('Ctrl Pts',(-6.55778032902798,4.79741646328296,
93.2158370323446));
#171596=CARTESIAN_POINT('Ctrl Pts',(-6.55774554594491,4.79746400930785,
93.2158347243625));
#171597=CARTESIAN_POINT('Ctrl Pts',(-6.55767599410069,4.79755907961091,
93.2158301094071));
#171598=CARTESIAN_POINT('Ctrl Pts',(-6.55764122496623,4.79760660440025,
93.2158278024089));
#171599=CARTESIAN_POINT('Ctrl Pts',(-6.55757170083455,4.79770163248742,
93.2158231894089));
#171600=CARTESIAN_POINT('Ctrl Pts',(-6.55753694551589,4.79774913622549,
93.2158208833857));
#171601=CARTESIAN_POINT('Ctrl Pts',(-6.55746744895978,4.79784412228955,
93.2158162723319));
#171602=CARTESIAN_POINT('Ctrl Pts',(-6.55743270734223,4.79789160513591,
93.2158139672761));
#171603=CARTESIAN_POINT('Ctrl Pts',(-6.55736323827116,4.79798654930612,
93.2158093581623));
#171604=CARTESIAN_POINT('Ctrl Pts',(-6.55732851032321,4.79803401130659,
93.2158070540716));
#171605=CARTESIAN_POINT('Ctrl Pts',(-6.55725906838534,4.79812891406929,
93.2158024468744));
#171606=CARTESIAN_POINT('Ctrl Pts',(-6.55722435398003,4.79817635540009,
93.2158001437403));
#171607=CARTESIAN_POINT('Ctrl Pts',(-6.55715493908768,4.79827121688058,
93.2157955384537));
#171608=CARTESIAN_POINT('Ctrl Pts',(-6.55712023817218,4.79831863761665,
93.2157932362726));
#171609=CARTESIAN_POINT('Ctrl Pts',(-6.5298517047507,4.83558176093202,93.2139841684961));
#171610=CARTESIAN_POINT('Ctrl Pts',(-6.50230160666431,4.87256483241269,
93.21217429565));
#171611=CARTESIAN_POINT('Ctrl Pts',(-6.40778004575286,4.99722060901601,
93.2060239744839));
#171612=CARTESIAN_POINT('Ctrl Pts',(-6.33933876926566,5.08376264253064,
93.2016691383768));
#171613=CARTESIAN_POINT('Ctrl Pts',(-6.16227216960738,5.2985204853865,93.1906420440488));
#171614=CARTESIAN_POINT('Ctrl Pts',(-6.05139276956349,5.42480990028568,
93.1839507857722));
#171615=CARTESIAN_POINT('Ctrl Pts',(-5.764170871239,5.73217765710635,93.1671577996232));
#171616=CARTESIAN_POINT('Ctrl Pts',(-5.58314559313247,5.90863881191473,
93.1570418423535));
#171617=CARTESIAN_POINT('Ctrl Pts',(-5.34745425810077,6.11786944201301,
93.1445487303525));
#171618=CARTESIAN_POINT('Ctrl Pts',(-5.30023847401889,6.15882015901992,
93.1420782065938));
#171619=CARTESIAN_POINT('Ctrl Pts',(-5.23328565854219,6.21554877951916,
93.1386227725085));
#171620=CARTESIAN_POINT('Ctrl Pts',(-5.21394051745968,6.23178543472024,
93.1376298815866));
#171621=CARTESIAN_POINT('Ctrl Pts',(-5.18051694166885,6.25957373948575,
93.1359241157322));
#171622=CARTESIAN_POINT('Ctrl Pts',(-5.16647484431986,6.27116870036991,
93.1352103859523));
#171623=CARTESIAN_POINT('Ctrl Pts',(-5.15229381191995,6.28279842545444,
93.1344924407725));
#171624=CARTESIAN_POINT('Ctrl Pts',(-5.15219376259511,6.28288047092655,
93.1344873757037));
#171625=CARTESIAN_POINT('Ctrl Pts',(-5.15199897010158,6.28304020276687,
93.13447751447));
#171626=CARTESIAN_POINT('Ctrl Pts',(-5.15190427601749,6.28311784930319,
93.1344727207752));
#171627=CARTESIAN_POINT('Ctrl Pts',(-5.15175004632635,6.28324430757024,
93.1344649134199));
#171628=CARTESIAN_POINT('Ctrl Pts',(-5.15169046009297,6.28329316297049,
93.1344618971195));
#171629=CARTESIAN_POINT('Ctrl Pts',(-5.15157204477313,6.28339025015948,
93.1344559029459));
#171630=CARTESIAN_POINT('Ctrl Pts',(-5.15151323383699,6.28343846710465,
93.1344529259903));
#171631=CARTESIAN_POINT('Ctrl Pts',(-5.15139637841243,6.28353426986887,
93.1344470109737));
#171632=CARTESIAN_POINT('Ctrl Pts',(-5.15133833607977,6.28358185395662,
93.1344440730205));
#171633=CARTESIAN_POINT('Ctrl Pts',(-5.15122300631927,6.28367640057621,
93.1344382354205));
#171634=CARTESIAN_POINT('Ctrl Pts',(-5.15116572090976,6.28372336148851,
93.1344353358746));
#171635=CARTESIAN_POINT('Ctrl Pts',(-5.15105189338562,6.2838166713788,93.1344295744978));
#171636=CARTESIAN_POINT('Ctrl Pts',(-5.15099535340933,6.28386301863799,
93.134426712774));
#171637=CARTESIAN_POINT('Ctrl Pts',(-5.15088300493899,6.28395511100634,
93.1344210264398));
#171638=CARTESIAN_POINT('Ctrl Pts',(-5.15082719889353,6.28400085414154,
93.1344182019523));
#171639=CARTESIAN_POINT('Ctrl Pts',(-5.15071630749497,6.2840917472045,93.1344125895411));
#171640=CARTESIAN_POINT('Ctrl Pts',(-5.15066122442699,6.28413689529147,
93.134409801732));
#171641=CARTESIAN_POINT('Ctrl Pts',(-5.15055176750221,6.28422660776392,
93.1344042620932));
#171642=CARTESIAN_POINT('Ctrl Pts',(-5.15049739632682,6.28427116998303,
93.1344015103982));
#171643=CARTESIAN_POINT('Ctrl Pts',(-5.15038935253042,6.28435971954687,
93.1343960424449));
#171644=CARTESIAN_POINT('Ctrl Pts',(-5.1503356825521,6.2844037047562,93.1343933263193));
#171645=CARTESIAN_POINT('Ctrl Pts',(-5.15022903060004,6.28449110903689,
93.1343879289678));
#171646=CARTESIAN_POINT('Ctrl Pts',(-5.15017605137443,6.2845345258857,93.1343852478799));
#171647=CARTESIAN_POINT('Ctrl Pts',(-5.15007076995498,6.2846208025254,93.1343799200454));
#171648=CARTESIAN_POINT('Ctrl Pts',(-5.15001847093487,6.28466365974429,
93.1343772734584));
#171649=CARTESIAN_POINT('Ctrl Pts',(-5.14991453997051,6.28474882536796,
93.1343720141187));
#171650=CARTESIAN_POINT('Ctrl Pts',(-5.1498629110753,6.28479113130228,93.1343694015193));
#171651=CARTESIAN_POINT('Ctrl Pts',(-5.14976031017698,6.28487520278459,
93.1343642096368));
#171652=CARTESIAN_POINT('Ctrl Pts',(-5.14970934139229,6.2849169657227,93.1343616305155));
#171653=CARTESIAN_POINT('Ctrl Pts',(-5.14960805090765,6.28499995932921,
93.1343565050898));
#171654=CARTESIAN_POINT('Ctrl Pts',(-5.14955773254745,6.28504118728773,
93.1343539589535));
#171655=CARTESIAN_POINT('Ctrl Pts',(-5.14945773247267,6.28512311956672,
93.1343488989668));
#171656=CARTESIAN_POINT('Ctrl Pts',(-5.14940805462437,6.28516382074528,
93.1343463853111));
#171657=CARTESIAN_POINT('Ctrl Pts',(-5.14930932652529,6.28524470695378,
93.1343413898253));
#171658=CARTESIAN_POINT('Ctrl Pts',(-5.14926027987475,6.28528488905923,
93.1343389081763));
#171659=CARTESIAN_POINT('Ctrl Pts',(-5.14916280459681,6.28536474503961,
93.1343339762167));
#171660=CARTESIAN_POINT('Ctrl Pts',(-5.14911437979497,6.28540441580493,
93.1343315260988));
#171661=CARTESIAN_POINT('Ctrl Pts',(-5.14901813901997,6.28548325670949,
93.1343266567334));
#171662=CARTESIAN_POINT('Ctrl Pts',(-5.14897032698599,6.28552242364556,
93.1343242376845));
#171663=CARTESIAN_POINT('Ctrl Pts',(-5.14887530233082,6.28560026467516,
93.1343194299783));
#171664=CARTESIAN_POINT('Ctrl Pts',(-5.14882809396667,6.28563893530464,
93.1343170415356));
#171665=CARTESIAN_POINT('Ctrl Pts',(-5.14873426787018,6.28571579098223,
93.1343122945951));
#171666=CARTESIAN_POINT('Ctrl Pts',(-5.1486876543865,6.28575397257269,93.1343099363115));
#171667=CARTESIAN_POINT('Ctrl Pts',(-5.14859500924652,6.28582985745046,
93.1343052492415));
#171668=CARTESIAN_POINT('Ctrl Pts',(-5.14854898195993,6.28586755718052,
93.1343029206754));
#171669=CARTESIAN_POINT('Ctrl Pts',(-5.1484575006427,6.28594248542269,93.1342982926043));
#171670=CARTESIAN_POINT('Ctrl Pts',(-5.14841205109036,6.28597971028821,
93.1342959933252));
#171671=CARTESIAN_POINT('Ctrl Pts',(-5.14832171650406,6.28605369602054,
93.1342914233839));
#171672=CARTESIAN_POINT('Ctrl Pts',(-5.1482768362567,6.28609045298784,93.1342891529631));
#171673=CARTESIAN_POINT('Ctrl Pts',(-5.14820204483236,6.28615170590039,
93.1342853694308));
#171674=CARTESIAN_POINT('Ctrl Pts',(-5.14817213864121,6.28617619820678,
93.1342838565551));
#171675=CARTESIAN_POINT('Ctrl Pts',(-5.14811259760543,6.28622495989124,
93.1342808445564));
#171676=CARTESIAN_POINT('Ctrl Pts',(-5.1480828255236,6.28624934166092,93.1342793384905));
#171677=CARTESIAN_POINT('Ctrl Pts',(-5.14802336814565,6.28629803342165,
93.1342763307739));
#171678=CARTESIAN_POINT('Ctrl Pts',(-5.14799368370544,6.28632234271388,
93.1342748291664));
#171679=CARTESIAN_POINT('Ctrl Pts',(-5.14793440076921,6.28637089021504,
93.134271830324));
#171680=CARTESIAN_POINT('Ctrl Pts',(-5.14790480332331,6.28639512756612,
93.134270333142));
#171681=CARTESIAN_POINT('Ctrl Pts',(-5.1478456949008,6.28644353076116,93.1342673431769));
#171682=CARTESIAN_POINT('Ctrl Pts',(-5.14781618444235,6.2864676961829,93.1342658504199));
#171683=CARTESIAN_POINT('Ctrl Pts',(-5.14775724851596,6.28651595673633,
93.1342628692297));
#171684=CARTESIAN_POINT('Ctrl Pts',(-5.14772782422087,6.28654005090968,
93.1342613808557));
#171685=CARTESIAN_POINT('Ctrl Pts',(-5.1331299317171,6.29849340828202,93.1335229793208));
#171686=CARTESIAN_POINT('Ctrl Pts',(-5.11852001434468,6.3103720156092,93.1327869725556));
#171687=CARTESIAN_POINT('Ctrl Pts',(-5.07617719364443,6.34455508712244,
93.1306622885587));
#171688=CARTESIAN_POINT('Ctrl Pts',(-5.04833881046515,6.36672831407095,
93.1292757989198));
#171689=CARTESIAN_POINT('Ctrl Pts',(-4.90865164174788,6.47649669886406,
93.1223676933497));
#171690=CARTESIAN_POINT('Ctrl Pts',(-4.79466379321652,6.56133143621268,
93.1168858369982));
#171691=CARTESIAN_POINT('Ctrl Pts',(-4.33877319253352,6.88239802625623,
93.0954395140046));
#171692=CARTESIAN_POINT('Ctrl Pts',(-3.98118386244098,7.09524706129059,
93.079611751811));
#171693=CARTESIAN_POINT('Ctrl Pts',(-3.47932482357219,7.34403826428309,
93.0579685553326));
#171694=CARTESIAN_POINT('Ctrl Pts',(-3.3480720322742,7.40479658204466,93.052360809731));
#171695=CARTESIAN_POINT('Ctrl Pts',(-3.15285400606348,7.48891300733574,
93.044081327935));
#171696=CARTESIAN_POINT('Ctrl Pts',(-3.09010455951135,7.51502230023901,
93.0414292061999));
#171697=CARTESIAN_POINT('Ctrl Pts',(-2.97633795826776,7.56069337661883,
93.036636225409));
#171698=CARTESIAN_POINT('Ctrl Pts',(-2.92543692094486,7.58053367335228,
93.0344972597739));
#171699=CARTESIAN_POINT('Ctrl Pts',(-2.81284893249944,7.62311553322266,
93.0297777834811));
#171700=CARTESIAN_POINT('Ctrl Pts',(-2.75107823072608,7.64562476707396,
93.0271961261199));
#171701=CARTESIAN_POINT('Ctrl Pts',(-2.68822626829924,7.6676676922617,93.0245769702192));
#171702=CARTESIAN_POINT('Ctrl Pts',(-2.68741116588213,7.66795341235325,
93.0245430047238));
#171703=CARTESIAN_POINT('Ctrl Pts',(-2.68577273413758,7.66852744300086,
93.0244747335468));
#171704=CARTESIAN_POINT('Ctrl Pts',(-2.68494940390215,7.66881575094744,
93.0244404278537));
#171705=CARTESIAN_POINT('Ctrl Pts',(-2.68329413473645,7.66939508213039,
93.0243714604537));
#171706=CARTESIAN_POINT('Ctrl Pts',(-2.6824621948553,7.66968610260478,93.024336798735));
#171707=CARTESIAN_POINT('Ctrl Pts',(-2.68078931157348,7.67027098758548,
93.0242671029184));
#171708=CARTESIAN_POINT('Ctrl Pts',(-2.67994836716445,7.67056484917341,
93.0242320688079));
#171709=CARTESIAN_POINT('Ctrl Pts',(-2.67825706611632,7.67115554929748,
93.0241616112703));
#171710=CARTESIAN_POINT('Ctrl Pts',(-2.6774067084173,7.67145238474707,93.0241261878301));
#171711=CARTESIAN_POINT('Ctrl Pts',(-2.67569615737389,7.67204916992957,
93.0240549340894));
#171712=CARTESIAN_POINT('Ctrl Pts',(-2.6748359629,7.67234911640361,93.0240191037747));
#171713=CARTESIAN_POINT('Ctrl Pts',(-2.492096908845,7.73603504788378,93.0164076486909));
#171714=CARTESIAN_POINT('Ctrl Pts',(-2.30802234411292,7.7929338269881,93.0088040390402));
#171715=CARTESIAN_POINT('Ctrl Pts',(-1.98937177659332,7.87914933227079,
92.9957716765212));
#171716=CARTESIAN_POINT('Ctrl Pts',(-1.85575197798406,7.91168623429992,
92.9903455786219));
#171717=CARTESIAN_POINT('Ctrl Pts',(-1.68232333873733,7.94928123111285,
92.9833665574352));
#171718=CARTESIAN_POINT('Ctrl Pts',(-1.64321399007387,7.95745761548076,
92.9817969119496));
#171719=CARTESIAN_POINT('Ctrl Pts',(-1.56750947413697,7.97270284489567,
92.97876723469));
#171720=CARTESIAN_POINT('Ctrl Pts',(-1.53092294302146,7.97980899224618,
92.9773070694807));
#171721=CARTESIAN_POINT('Ctrl Pts',(-1.41799428261572,8.00093771863274,
92.9728110332754));
#171722=CARTESIAN_POINT('Ctrl Pts',(-1.34149902368857,8.01411832947137,
92.9697807580378));
#171723=CARTESIAN_POINT('Ctrl Pts',(-1.13707977988039,8.046332184652,92.9617111423394));
#171724=CARTESIAN_POINT('Ctrl Pts',(-1.00887049827884,8.06341072092439,
92.9566791044633));
#171725=CARTESIAN_POINT('Ctrl Pts',(-0.727628800987101,8.09406151263356,
92.9456636036322));
#171726=CARTESIAN_POINT('Ctrl Pts',(-0.574508770834238,8.10636878388756,
92.9396807715246));
#171727=CARTESIAN_POINT('Ctrl Pts',(-0.358147343803119,8.11759791234234,
92.9312129433623));
#171728=CARTESIAN_POINT('Ctrl Pts',(-0.295126334846212,8.12013336094641,
92.9287448844243));
#171729=CARTESIAN_POINT('Ctrl Pts',(-0.177200895026892,8.12350305210914,
92.9241212338898));
#171730=CARTESIAN_POINT('Ctrl Pts',(-0.122305084141662,8.12451496619417,
92.9219666822249));
#171731=CARTESIAN_POINT('Ctrl Pts',(-0.0011607983394269,8.12551995835907,
92.9172055995514));
#171732=CARTESIAN_POINT('Ctrl Pts',(0.0650858149596844,8.12525936384979,
92.9145978103414));
#171733=CARTESIAN_POINT('Ctrl Pts',(0.299956336470427,8.12146285162752,
92.9053335486736));
#171734=CARTESIAN_POINT('Ctrl Pts',(0.468464002800469,8.1134871260525,92.8986520410267));
#171735=CARTESIAN_POINT('Ctrl Pts',(0.912682296226523,8.0785760390206,92.8809237290591));
#171736=CARTESIAN_POINT('Ctrl Pts',(1.18747343697251,8.0427784271147,92.8698355522543));
#171737=CARTESIAN_POINT('Ctrl Pts',(1.52827811647357,7.980531656138,92.8559696532123));
#171738=CARTESIAN_POINT('Ctrl Pts',(1.5964961399566,7.96716509276762,92.8531887688841));
#171739=CARTESIAN_POINT('Ctrl Pts',(1.83833220565102,7.91654919514451,92.8433158307784));
#171740=CARTESIAN_POINT('Ctrl Pts',(2.01089271660614,7.8744858948896,92.8362433860448));
#171741=CARTESIAN_POINT('Ctrl Pts',(2.21809746407732,7.81672184208803,92.8277539945724));
#171742=CARTESIAN_POINT('Ctrl Pts',(2.25418717044016,7.80639077529286,92.8262755148005));
#171743=CARTESIAN_POINT('Ctrl Pts',(2.31011222975119,7.78996146246456,92.8239852292487));
#171744=CARTESIAN_POINT('Ctrl Pts',(2.32999792172498,7.78403672840212,92.82317101046));
#171745=CARTESIAN_POINT('Ctrl Pts',(2.36857504070049,7.77238200491378,92.8215918948963));
#171746=CARTESIAN_POINT('Ctrl Pts',(2.38726891412584,7.76666060083999,92.8208268735176));
#171747=CARTESIAN_POINT('Ctrl Pts',(2.42997436181131,7.75342151726488,92.8190797770516));
#171748=CARTESIAN_POINT('Ctrl Pts',(2.45397200170698,7.74585967088433,92.8180984754768));
#171749=CARTESIAN_POINT('Ctrl Pts',(2.53972591951875,7.71839941720727,92.8145927272703));
#171750=CARTESIAN_POINT('Ctrl Pts',(2.60127881422242,7.69787281904638,92.8120778901396));
#171751=CARTESIAN_POINT('Ctrl Pts',(2.71597094843826,7.65809264378464,92.8073876156239));
#171752=CARTESIAN_POINT('Ctrl Pts',(2.7691678703961,7.63901763870767,92.8052103868164));
#171753=CARTESIAN_POINT('Ctrl Pts',(3.07741597590783,7.52484497215556,92.7925702843117));
#171754=CARTESIAN_POINT('Ctrl Pts',(3.32775878974398,7.41753352558002,92.7822000633599));
#171755=CARTESIAN_POINT('Ctrl Pts',(3.73504505369,7.21817018164117,92.7648005642661));
#171756=CARTESIAN_POINT('Ctrl Pts',(3.89513266216882,7.13305564489591,92.7578195040342));
#171757=CARTESIAN_POINT('Ctrl Pts',(4.10088933551553,7.01466640202612,92.7486090125817));
#171758=CARTESIAN_POINT('Ctrl Pts',(4.14924865296453,6.98617017031193,92.746426655974));
#171759=CARTESIAN_POINT('Ctrl Pts',(4.22584581398583,6.93995860942192,92.7429406525475));
#171760=CARTESIAN_POINT('Ctrl Pts',(4.25427670188204,6.92256658176761,92.741640212816));
#171761=CARTESIAN_POINT('Ctrl Pts',(4.31292910439184,6.88618935412041,92.7389436317364));
#171762=CARTESIAN_POINT('Ctrl Pts',(4.34313415428197,6.86717896863493,92.737547265882));
#171763=CARTESIAN_POINT('Ctrl Pts',(4.4029592112796,6.82897382134527,92.7347660487752));
#171764=CARTESIAN_POINT('Ctrl Pts',(4.43258135641589,6.80978382748622,92.7333812705683));
#171765=CARTESIAN_POINT('Ctrl Pts',(4.53115601596589,6.74500889947469,92.7287471131814));
#171766=CARTESIAN_POINT('Ctrl Pts',(4.59953753612754,6.69856508679117,92.7254894978782));
#171767=CARTESIAN_POINT('Ctrl Pts',(4.89761768860853,6.48939637365424,92.711097253402));
#171768=CARTESIAN_POINT('Ctrl Pts',(5.11947728618505,6.31584306981161,92.6998646672219));
#171769=CARTESIAN_POINT('Ctrl Pts',(5.45433753896578,6.02463497878707,92.6821698788836));
#171770=CARTESIAN_POINT('Ctrl Pts',(5.57357839181492,5.91449483959559,92.6757080672187));
#171771=CARTESIAN_POINT('Ctrl Pts',(5.70571001556667,5.78490104061786,92.6683958583227));
#171772=CARTESIAN_POINT('Ctrl Pts',(5.7219115053002,5.76887645568493,92.6674965821061));
#171773=CARTESIAN_POINT('Ctrl Pts',(5.75441706255619,5.73645417691248,92.6656871336822));
#171774=CARTESIAN_POINT('Ctrl Pts',(5.77071898020844,5.72005460723826,92.6647770041508));
#171775=CARTESIAN_POINT('Ctrl Pts',(5.79942210864063,5.69093194653879,92.6631699893924));
#171776=CARTESIAN_POINT('Ctrl Pts',(5.81185200099476,5.67823736164646,92.6624725525816));
#171777=CARTESIAN_POINT('Ctrl Pts',(5.83885967648232,5.65047297531502,92.6609539615564));
#171778=CARTESIAN_POINT('Ctrl Pts',(5.85342090955712,5.6353873712343,92.6601331860287));
#171779=CARTESIAN_POINT('Ctrl Pts',(5.89585593269314,5.59108228243704,92.6577351148585));
#171780=CARTESIAN_POINT('Ctrl Pts',(5.92357052592392,5.5617111143031,92.6561610838476));
#171781=CARTESIAN_POINT('Ctrl Pts',(5.98674842794419,5.49374895380421,92.6525533033023));
#171782=CARTESIAN_POINT('Ctrl Pts',(6.02205967590957,5.45501893827718,92.650522341185));
#171783=CARTESIAN_POINT('Ctrl Pts',(6.37322186484456,5.06229239902528,92.6301634768993));
#171784=CARTESIAN_POINT('Ctrl Pts',(6.65787326611589,4.68161277993397,92.6123034654986));
#171785=CARTESIAN_POINT('Ctrl Pts',(7.10513223955482,3.95947034164228,92.5799817441187));
#171786=CARTESIAN_POINT('Ctrl Pts',(7.28027274382671,3.62738615802649,92.5656351645238));
#171787=CARTESIAN_POINT('Ctrl Pts',(7.46148979324959,3.21733341453781,92.5482222035637));
#171788=CARTESIAN_POINT('Ctrl Pts',(7.49022031307785,3.14986726956872,92.5453671681984));
#171789=CARTESIAN_POINT('Ctrl Pts',(7.53432659891189,3.0422779777039,92.5408282929988));
#171790=CARTESIAN_POINT('Ctrl Pts',(7.55030413776109,3.00240570276799,92.5391492371062));
#171791=CARTESIAN_POINT('Ctrl Pts',(7.57964661642587,2.92746528063591,92.5359988179278));
#171792=CARTESIAN_POINT('Ctrl Pts',(7.59308623667504,2.89242756024388,92.5345280557786));
#171793=CARTESIAN_POINT('Ctrl Pts',(7.62276544197277,2.81341990380907,92.5312163110182));
#171794=CARTESIAN_POINT('Ctrl Pts',(7.63886823647951,2.7694000405867,92.5293744074653));
#171795=CARTESIAN_POINT('Ctrl Pts',(7.67168473108728,2.67722596756345,92.5255241554226));
#171796=CARTESIAN_POINT('Ctrl Pts',(7.68832801744688,2.62904883323022,92.5235154192683));
#171797=CARTESIAN_POINT('Ctrl Pts',(7.73145188360616,2.50030617258792,92.5181570808077));
#171798=CARTESIAN_POINT('Ctrl Pts',(7.75712626932035,2.41947745070647,92.5148028274475));
#171799=CARTESIAN_POINT('Ctrl Pts',(8.00978404278669,1.57865454717926,92.480011156819));
#171800=CARTESIAN_POINT('Ctrl Pts',(8.12556467337259,0.789785411816207,
92.4478184145232));
#171801=CARTESIAN_POINT('Ctrl Pts',(8.1252493577062,-0.0032307267043824,
92.4142825253168));
#171802=CARTESIAN_POINT('',(8.1252500832311,0.00151305119344404,88.4163212481402));
#171803=CARTESIAN_POINT('Ctrl Pts',(8.12524935171145,-0.00324576840847315,
92.4142818892175));
#171804=CARTESIAN_POINT('Ctrl Pts',(8.12505842335934,-0.481203611965918,
92.3940695088115));
#171805=CARTESIAN_POINT('Ctrl Pts',(8.08269529486795,-0.958231732574647,
92.3736492650366));
#171806=CARTESIAN_POINT('Ctrl Pts',(7.99334777073901,-1.45841875622197,
92.3532464736714));
#171807=CARTESIAN_POINT('Ctrl Pts',(7.98788932123645,-1.48802488929236,
92.3520429987674));
#171808=CARTESIAN_POINT('Ctrl Pts',(7.97940221984289,-1.53266530495396,
92.3502353455617));
#171809=CARTESIAN_POINT('Ctrl Pts',(7.97649536800879,-1.5477223171385,92.349626829814));
#171810=CARTESIAN_POINT('Ctrl Pts',(7.97170884541368,-1.57214403720874,
92.3486418882419));
#171811=CARTESIAN_POINT('Ctrl Pts',(7.96985526499509,-1.5815137829795,92.3482644892345));
#171812=CARTESIAN_POINT('Ctrl Pts',(7.96657571697868,-1.59793952572654,
92.3476037670509));
#171813=CARTESIAN_POINT('Ctrl Pts',(7.96515688782877,-1.6049969267631,92.3473201701683));
#171814=CARTESIAN_POINT('Ctrl Pts',(7.96228214280116,-1.61919850529424,
92.3467500770431));
#171815=CARTESIAN_POINT('Ctrl Pts',(7.96082598570614,-1.62634262899425,
92.3464635905037));
#171816=CARTESIAN_POINT('Ctrl Pts',(7.95799786724277,-1.6401229920588,92.3459115749195));
#171817=CARTESIAN_POINT('Ctrl Pts',(7.95662721641338,-1.6467594916934,92.3456459937473));
#171818=CARTESIAN_POINT('Ctrl Pts',(7.95336334885058,-1.66246347533802,
92.3450181865911));
#171819=CARTESIAN_POINT('Ctrl Pts',(7.95146292315046,-1.67152946380344,
92.3446562548924));
#171820=CARTESIAN_POINT('Ctrl Pts',(7.94475632826809,-1.70325303776969,
92.3433916030867));
#171821=CARTESIAN_POINT('Ctrl Pts',(7.93986875634451,-1.72589344203662,
92.3424922907919));
#171822=CARTESIAN_POINT('Ctrl Pts',(7.85233235732887,-2.12314029701398,
92.3267737934708));
#171823=CARTESIAN_POINT('Ctrl Pts',(7.743352541108,-2.49145438816358,92.313276116538));
#171824=CARTESIAN_POINT('Ctrl Pts',(7.56081438047686,-2.97866578084,92.2955747243282));
#171825=CARTESIAN_POINT('Ctrl Pts',(7.50964603274314,-3.10541158989064,
92.2909837202256));
#171826=CARTESIAN_POINT('Ctrl Pts',(7.40089438557037,-3.35636329896071,
92.2818371013519));
#171827=CARTESIAN_POINT('Ctrl Pts',(7.34332080885891,-3.48052466028751,
92.2772829763544));
#171828=CARTESIAN_POINT('Ctrl Pts',(7.15027688353463,-3.8707000123997,92.2627550196844));
#171829=CARTESIAN_POINT('Ctrl Pts',(7.00327648035908,-4.13072509715393,
92.2527375791108));
#171830=CARTESIAN_POINT('Ctrl Pts',(6.62847214826358,-4.71595725761751,
92.2286158630955));
#171831=CARTESIAN_POINT('Ctrl Pts',(6.39050381607807,-5.03371794372861,
92.2142657717043));
#171832=CARTESIAN_POINT('Ctrl Pts',(6.11120177711919,-5.35478736540524,
92.1978795037557));
#171833=CARTESIAN_POINT('Ctrl Pts',(6.09197905753035,-5.37664635540263,
92.1967540145036));
#171834=CARTESIAN_POINT('Ctrl Pts',(6.06395570710275,-5.40816970613807,
92.1951164092528));
#171835=CARTESIAN_POINT('Ctrl Pts',(6.05524847283763,-5.41791697226722,
92.1946080203855));
#171836=CARTESIAN_POINT('Ctrl Pts',(6.04000713593716,-5.43489616781846,
92.1937188742371));
#171837=CARTESIAN_POINT('Ctrl Pts',(6.03348345825478,-5.44213743994845,
92.1933385351767));
#171838=CARTESIAN_POINT('Ctrl Pts',(6.02085020848902,-5.45610969119068,
92.1926024537384));
#171839=CARTESIAN_POINT('Ctrl Pts',(6.01474233671666,-5.46284219227043,
92.1922467799399));
#171840=CARTESIAN_POINT('Ctrl Pts',(6.00022627861805,-5.47878889601,92.1914019580711));
#171841=CARTESIAN_POINT('Ctrl Pts',(5.99180815773963,-5.48799400152999,
92.1909124093009));
#171842=CARTESIAN_POINT('Ctrl Pts',(5.96657690882266,-5.51545678777282,
92.1894462209484));
#171843=CARTESIAN_POINT('Ctrl Pts',(5.94970135709016,-5.53365677783305,
92.1884670531249));
#171844=CARTESIAN_POINT('Ctrl Pts',(5.78631150996949,-5.70825845471638,
92.1790004757031));
#171845=CARTESIAN_POINT('Ctrl Pts',(5.63375465646632,-5.85887492806857,
92.1702645257141));
#171846=CARTESIAN_POINT('Ctrl Pts',(4.99377777470236,-6.44258064973689,
92.134010909694));
#171847=CARTESIAN_POINT('Ctrl Pts',(4.46104316142138,-6.82228572231415,
92.1044865273501));
#171848=CARTESIAN_POINT('Ctrl Pts',(3.74593597174448,-7.21208117126267,
92.0680491058429));
#171849=CARTESIAN_POINT('Ctrl Pts',(3.60079213519847,-7.28563307253746,
92.0608154351659));
#171850=CARTESIAN_POINT('Ctrl Pts',(3.28357387176181,-7.43458717456244,
92.0454683720216));
#171851=CARTESIAN_POINT('Ctrl Pts',(3.11088863640055,-7.50848334935149,
92.0373957570775));
#171852=CARTESIAN_POINT('Ctrl Pts',(2.86919988791821,-7.60213652636437,
92.0266121992681));
#171853=CARTESIAN_POINT('Ctrl Pts',(2.80226905825337,-7.62706213412633,
92.0236794422539));
#171854=CARTESIAN_POINT('Ctrl Pts',(2.69222961912174,-7.66639757178168,
92.0189526964495));
#171855=CARTESIAN_POINT('Ctrl Pts',(2.64931625455858,-7.68133292821855,
92.0171321637149));
#171856=CARTESIAN_POINT('Ctrl Pts',(2.5935717493254,-7.70021124024953,92.0147943568442));
#171857=CARTESIAN_POINT('Ctrl Pts',(2.58085355038893,-7.7044832738915,92.0142627992657));
#171858=CARTESIAN_POINT('Ctrl Pts',(2.56142101905766,-7.71095712955034,
92.0134533155079));
#171859=CARTESIAN_POINT('Ctrl Pts',(2.55471433552318,-7.71318171411346,
92.0131744312009));
#171860=CARTESIAN_POINT('Ctrl Pts',(2.54160451803625,-7.71751122233762,
92.0126302288682));
#171861=CARTESIAN_POINT('Ctrl Pts',(2.53520165189848,-7.71961693204703,
92.0123648784637));
#171862=CARTESIAN_POINT('Ctrl Pts',(2.52054008381536,-7.72441847142617,
92.0117582588712));
#171863=CARTESIAN_POINT('Ctrl Pts',(2.5122796550617,-7.72710903063499,92.011417204592));
#171864=CARTESIAN_POINT('Ctrl Pts',(2.48989312902347,-7.73436100273797,
92.0104948292934));
#171865=CARTESIAN_POINT('Ctrl Pts',(2.47575878426278,-7.73889697310255,
92.0099145236709));
#171866=CARTESIAN_POINT('Ctrl Pts',(2.40907902657994,-7.76009435626059,
92.0071863026476));
#171867=CARTESIAN_POINT('Ctrl Pts',(2.35637671070558,-7.7762597137135,92.005057475186));
#171868=CARTESIAN_POINT('Ctrl Pts',(1.91880342659443,-7.90561936485096,
91.9875831727675));
#171869=CARTESIAN_POINT('Ctrl Pts',(1.52617644287239,-7.99070989218256,
91.9731565700769));
#171870=CARTESIAN_POINT('Ctrl Pts',(0.65733121480216,-8.11260215404912,
91.9416483270983));
#171871=CARTESIAN_POINT('Ctrl Pts',(0.180920321578308,-8.13717724189745,
91.9246033048994));
#171872=CARTESIAN_POINT('Ctrl Pts',(-0.467285113362848,-8.11363605367949,
91.9004039650091));
#171873=CARTESIAN_POINT('Ctrl Pts',(-0.639429355346308,-8.1018870244104,
91.8938888762583));
#171874=CARTESIAN_POINT('Ctrl Pts',(-0.892866035785481,-8.07646187149219,
91.8841435108361));
#171875=CARTESIAN_POINT('Ctrl Pts',(-0.974535876972609,-8.06701467177951,
91.8809796155121));
#171876=CARTESIAN_POINT('Ctrl Pts',(-1.08841842534227,-8.05208660961738,
91.876534505384));
#171877=CARTESIAN_POINT('Ctrl Pts',(-1.12076326449219,-8.04764829802405,
91.8752682525196));
#171878=CARTESIAN_POINT('Ctrl Pts',(-1.17561965942971,-8.03978385529092,
91.8731143530182));
#171879=CARTESIAN_POINT('Ctrl Pts',(-1.19814521431303,-8.03645780579778,
91.8722280807683));
#171880=CARTESIAN_POINT('Ctrl Pts',(-1.2426108016991,-8.02970105802412,
91.8704749969147));
#171881=CARTESIAN_POINT('Ctrl Pts',(-1.2645513546987,-8.02627501108478,
91.8696082602749));
#171882=CARTESIAN_POINT('Ctrl Pts',(-1.31511424041881,-8.01816707507372,
91.867606699519));
#171883=CARTESIAN_POINT('Ctrl Pts',(-1.34372605850098,-8.01342180215072,
91.8664710247729));
#171884=CARTESIAN_POINT('Ctrl Pts',(-1.42060290601495,-8.00024846206587,
91.863410928862));
#171885=CARTESIAN_POINT('Ctrl Pts',(-1.46881794381011,-7.99153689036157,
91.8614825158935));
#171886=CARTESIAN_POINT('Ctrl Pts',(-1.92590640797534,-7.90467307934542,
91.8431067513998));
#171887=CARTESIAN_POINT('Ctrl Pts',(-2.32826042277422,-7.79564894024238,
91.8261689391368));
#171888=CARTESIAN_POINT('Ctrl Pts',(-3.22416733751635,-7.4773106381599,
91.7864489684192));
#171889=CARTESIAN_POINT('Ctrl Pts',(-3.7089531284197,-7.2490737686522,91.7634258258299));
#171890=CARTESIAN_POINT('Ctrl Pts',(-4.3139440213017,-6.88756549782854,
91.7340924264256));
#171891=CARTESIAN_POINT('Ctrl Pts',(-4.45731175435859,-6.79566384252212,
91.7271033758118));
#171892=CARTESIAN_POINT('Ctrl Pts',(-4.62400444865303,-6.68126402747384,
91.7190092461655));
#171893=CARTESIAN_POINT('Ctrl Pts',(-4.65021237455194,-6.66304968090878,
91.717737662791));
#171894=CARTESIAN_POINT('Ctrl Pts',(-4.68586895780281,-6.63795572681863,
91.7160096606297));
#171895=CARTESIAN_POINT('Ctrl Pts',(-4.69541091837173,-6.63120957520054,
91.7155474339711));
#171896=CARTESIAN_POINT('Ctrl Pts',(-4.71068028661942,-6.62036467283925,
91.7148081211404));
#171897=CARTESIAN_POINT('Ctrl Pts',(-4.71641695818835,-6.61627903288656,
91.7145304440098));
#171898=CARTESIAN_POINT('Ctrl Pts',(-4.72831401106654,-6.60778265228595,
91.7139547602278));
#171899=CARTESIAN_POINT('Ctrl Pts',(-4.73447355181724,-6.60337074188031,
91.713656807878));
#171900=CARTESIAN_POINT('Ctrl Pts',(-4.74857450558232,-6.59324074257283,
91.7129749545951));
#171901=CARTESIAN_POINT('Ctrl Pts',(-4.756511786827,-6.58751690300791,91.7125913249666));
#171902=CARTESIAN_POINT('Ctrl Pts',(-4.78148642007465,-6.56943818676379,
91.711384843472));
#171903=CARTESIAN_POINT('Ctrl Pts',(-4.79848620548932,-6.55703138787556,
91.7105645067883));
#171904=CARTESIAN_POINT('Ctrl Pts',(-4.98886920006526,-6.4169489920769,
91.7013891124866));
#171905=CARTESIAN_POINT('Ctrl Pts',(-5.15715367014994,-6.28250069654908,
91.6934317473731));
#171906=CARTESIAN_POINT('Ctrl Pts',(-5.87158677079353,-5.66364550463093,
91.6596826944939));
#171907=CARTESIAN_POINT('Ctrl Pts',(-6.35638927209257,-5.11359565535511,
91.6365014014358));
#171908=CARTESIAN_POINT('Ctrl Pts',(-6.96999327429432,-4.19292145669815,
91.5978076469144));
#171909=CARTESIAN_POINT('Ctrl Pts',(-7.1567255416074,-3.86557129821749,
91.5841156359475));
#171910=CARTESIAN_POINT('Ctrl Pts',(-7.33190603639712,-3.501939893346,91.5685594299608));
#171911=CARTESIAN_POINT('Ctrl Pts',(-7.34360161942063,-3.47734731964003,
91.5675058694669));
#171912=CARTESIAN_POINT('Ctrl Pts',(-7.36057756978936,-3.44118397465222,
91.5659543218603));
#171913=CARTESIAN_POINT('Ctrl Pts',(-7.36595480182881,-3.42965875328092,
91.5654595059189));
#171914=CARTESIAN_POINT('Ctrl Pts',(-7.37538187151951,-3.40932892714083,
91.5645860693891));
#171915=CARTESIAN_POINT('Ctrl Pts',(-7.3794430632071,-3.40052959996873,
91.5642078204962));
#171916=CARTESIAN_POINT('Ctrl Pts',(-7.38732572975457,-3.38336971487406,
91.5634697871345));
#171917=CARTESIAN_POINT('Ctrl Pts',(-7.39114877953382,-3.37500989378892,
91.5631100547497));
#171918=CARTESIAN_POINT('Ctrl Pts',(-7.40135239532739,-3.35259727309577,
91.5621451185898));
#171919=CARTESIAN_POINT('Ctrl Pts',(-7.40770710860408,-3.33853278332889,
91.5615390748387));
#171920=CARTESIAN_POINT('Ctrl Pts',(-7.43059390892505,-3.28749179378601,
91.5593377737918));
#171921=CARTESIAN_POINT('Ctrl Pts',(-7.44688939061198,-3.25041020180114,
91.557734854294));
#171922=CARTESIAN_POINT('Ctrl Pts',(-7.73127792216534,-2.58989750478238,
91.5291153816929));
#171923=CARTESIAN_POINT('Ctrl Pts',(-7.92046442442058,-1.93551286273028,
91.4993975382645));
#171924=CARTESIAN_POINT('Ctrl Pts',(-8.09555644438102,-0.824904926288004,
91.4487556891042));
#171925=CARTESIAN_POINT('Ctrl Pts',(-8.12862370169037,-0.379477489358884,
91.4284797730138));
#171926=CARTESIAN_POINT('Ctrl Pts',(-8.1233811112236,0.261823261431164,
91.4008583400842));
#171927=CARTESIAN_POINT('Ctrl Pts',(-8.1147350968487,0.457122673885287,
91.3926631373492));
#171928=CARTESIAN_POINT('Ctrl Pts',(-8.09620188454295,0.687361246080819,
91.3833820392998));
#171929=CARTESIAN_POINT('Ctrl Pts',(-8.09311814455134,0.722764965676807,
91.3819650505185));
#171930=CARTESIAN_POINT('Ctrl Pts',(-8.0886938707795,0.769974102839919,
91.3800878142285));
#171931=CARTESIAN_POINT('Ctrl Pts',(-8.08755960782569,0.781798085295039,
91.379618668753));
#171932=CARTESIAN_POINT('Ctrl Pts',(-8.08564664531005,0.801289765365157,
91.3788469212852));
#171933=CARTESIAN_POINT('Ctrl Pts',(-8.08488295965956,0.808958892682614,
91.3785436892213));
#171934=CARTESIAN_POINT('Ctrl Pts',(-8.08337588205804,0.823878041257104,
91.37795458838));
#171935=CARTESIAN_POINT('Ctrl Pts',(-8.08263364524238,0.831128169872339,
91.3776686722867));
#171936=CARTESIAN_POINT('Ctrl Pts',(-8.08088798104674,0.847956215363072,
91.3770058674632));
#171937=CARTESIAN_POINT('Ctrl Pts',(-8.07987727707015,0.857533377723981,
91.3766292739572));
#171938=CARTESIAN_POINT('Ctrl Pts',(-8.07709648076216,0.883442048431894,
91.3756121222586));
#171939=CARTESIAN_POINT('Ctrl Pts',(-8.07529387926842,0.89977007109312,
91.3749728514205));
#171940=CARTESIAN_POINT('Ctrl Pts',(-8.06127609237742,1.02330756896937,
91.3701487009231));
#171941=CARTESIAN_POINT('Ctrl Pts',(-8.04697558324632,1.13027241887401,
91.3660431779149));
#171942=CARTESIAN_POINT('Ctrl Pts',(-8.0123703159676,1.35494222932192,91.3575169787508));
#171943=CARTESIAN_POINT('Ctrl Pts',(-7.99159233698791,1.4725486385397,91.3531103430874));
#171944=CARTESIAN_POINT('Ctrl Pts',(-7.96757220555676,1.59295072033581,
91.3486248255663));
#171945=CARTESIAN_POINT('Ctrl Pts',(-7.96691291260701,1.59624480936779,
91.3485021262096));
#171946=CARTESIAN_POINT('Ctrl Pts',(-7.88108809444698,2.02368190299981,
91.3325833416261));
#171947=CARTESIAN_POINT('Ctrl Pts',(-7.76218618186128,2.44035264961898,
91.3173310721145));
#171948=CARTESIAN_POINT('Ctrl Pts',(-7.38182896381088,3.45763961478734,
91.2780985721355));
#171949=CARTESIAN_POINT('Ctrl Pts',(-7.08000058664505,4.03982268048939,
91.253592491344));
#171950=CARTESIAN_POINT('Ctrl Pts',(-6.64649038920768,4.67517493009015,
91.2238768842545));
#171951=CARTESIAN_POINT('Ctrl Pts',(-6.57919193085595,4.76941593158421,
91.2193870090111));
#171952=CARTESIAN_POINT('Ctrl Pts',(-6.47975507934423,4.9025503421081,91.2129142882603));
#171953=CARTESIAN_POINT('Ctrl Pts',(-6.44923256007434,4.94263341764401,
91.2109481468675));
#171954=CARTESIAN_POINT('Ctrl Pts',(-6.39508052940576,5.01239177137345,
91.2074948308176));
#171955=CARTESIAN_POINT('Ctrl Pts',(-6.37161226910041,5.04219033023428,
91.2060094080097));
#171956=CARTESIAN_POINT('Ctrl Pts',(-6.32231805489744,5.10388737797582,
91.2029119772274));
#171957=CARTESIAN_POINT('Ctrl Pts',(-6.29645733162535,5.13575671233051,
91.2012996255017));
#171958=CARTESIAN_POINT('Ctrl Pts',(-6.22817733832225,5.21861027764631,
91.197074682014));
#171959=CARTESIAN_POINT('Ctrl Pts',(-6.18537345127561,5.26927332587732,
91.1944579002746));
#171960=CARTESIAN_POINT('Ctrl Pts',(-5.99508172952204,5.48899014416312,
91.182958465877));
#171961=CARTESIAN_POINT('Ctrl Pts',(-5.84125077012173,5.65241581467839,
91.1740051426395));
#171962=CARTESIAN_POINT('Ctrl Pts',(-5.23401259267453,6.24623169309774,
91.1398484516222));
#171963=CARTESIAN_POINT('Ctrl Pts',(-4.73824640114135,6.63018173264989,
91.1141958390362));
#171964=CARTESIAN_POINT('Ctrl Pts',(-4.15184689095235,6.98466055711986,
91.0867900268546));
#171965=CARTESIAN_POINT('Ctrl Pts',(-4.09995403835374,7.01524715679656,
91.0843888084354));
#171966=CARTESIAN_POINT('Ctrl Pts',(-4.00871769502457,7.06766537741545,
91.0802108059653));
#171967=CARTESIAN_POINT('Ctrl Pts',(-3.96952413483381,7.08975243779715,
91.0784298880653));
#171968=CARTESIAN_POINT('Ctrl Pts',(-3.91103976647934,7.12207358822692,
91.0757936932892));
#171969=CARTESIAN_POINT('Ctrl Pts',(-3.89188800456705,7.13255718651336,
91.0749337872623));
#171970=CARTESIAN_POINT('Ctrl Pts',(-3.85637062794597,7.15181361078047,
91.0733453668089));
#171971=CARTESIAN_POINT('Ctrl Pts',(-3.84001680119728,7.16060774745978,
91.0726164223651));
#171972=CARTESIAN_POINT('Ctrl Pts',(-3.80268631437019,7.18051724599185,
91.0709577978678));
#171973=CARTESIAN_POINT('Ctrl Pts',(-3.78169077768482,7.19159690146912,
91.0700287576463));
#171974=CARTESIAN_POINT('Ctrl Pts',(-3.72627143019361,7.22053270941013,
91.0675859641771));
#171975=CARTESIAN_POINT('Ctrl Pts',(-3.69176774845453,7.23823474973324,
91.0660746805367));
#171976=CARTESIAN_POINT('Ctrl Pts',(-3.39512288244355,7.38775485034545,
91.0531559956734));
#171977=CARTESIAN_POINT('Ctrl Pts',(-3.12614304794733,7.50553227877203,
91.0419277360358));
#171978=CARTESIAN_POINT('Ctrl Pts',(-2.76144160049649,7.64220863852683,
91.0269438001028));
#171979=CARTESIAN_POINT('Ctrl Pts',(-2.67091266854636,7.67431677780503,
91.0232444129725));
#171980=CARTESIAN_POINT('Ctrl Pts',(-2.47330789031504,7.74048165132348,
91.0151973467297));
#171981=CARTESIAN_POINT('Ctrl Pts',(-2.36605201849586,7.77393759320926,
91.0108469649942));
#171982=CARTESIAN_POINT('Ctrl Pts',(-2.21288901281733,7.81824971347053,
91.0046471449027));
#171983=CARTESIAN_POINT('Ctrl Pts',(-2.16752763443435,7.83094696038992,
91.0028125688925));
#171984=CARTESIAN_POINT('Ctrl Pts',(-2.08785921645127,7.85250193660636,
90.9995924705763));
#171985=CARTESIAN_POINT('Ctrl Pts',(-2.05359981972962,7.86153105587192,
90.9982083871306));
#171986=CARTESIAN_POINT('Ctrl Pts',(-1.98651750758213,7.87874228354845,
90.9954991929199));
#171987=CARTESIAN_POINT('Ctrl Pts',(-1.95370036962425,7.88694406188557,
90.9941742733046));
#171988=CARTESIAN_POINT('Ctrl Pts',(-1.86362464715478,7.90885941642402,
90.9905385586053));
#171989=CARTESIAN_POINT('Ctrl Pts',(-1.80626686255547,7.92215589777895,
90.9882244072334));
#171990=CARTESIAN_POINT('Ctrl Pts',(-1.52288304145017,7.98461132735043,
90.9767938824655));
#171991=CARTESIAN_POINT('Ctrl Pts',(-1.29497611251476,8.02472587421883,
90.9676055432242));
#171992=CARTESIAN_POINT('Ctrl Pts',(-0.899631288846099,8.07702934212261,
90.9516949504627));
#171993=CARTESIAN_POINT('Ctrl Pts',(-0.73295176805845,8.09385699717708,
90.944996700409));
#171994=CARTESIAN_POINT('Ctrl Pts',(-0.483764740867235,8.11125351844492,
90.9350312174432));
#171995=CARTESIAN_POINT('Ctrl Pts',(-0.401575173985077,8.11573776301831,
90.9317523502175));
#171996=CARTESIAN_POINT('Ctrl Pts',(-0.236519235434454,8.12222966207281,
90.9251918044932));
#171997=CARTESIAN_POINT('Ctrl Pts',(-0.1536614963144,8.12421961484203,90.9219106377518));
#171998=CARTESIAN_POINT('Ctrl Pts',(-0.0433915389004529,8.12518032569453,
90.9175667432298));
#171999=CARTESIAN_POINT('Ctrl Pts',(-0.0159945855926529,8.12528044651396,
90.9164893669666));
#172000=CARTESIAN_POINT('Ctrl Pts',(0.0311246126927512,8.1252143224437,
90.9146399868386));
#172001=CARTESIAN_POINT('Ctrl Pts',(0.0508466549068599,8.12511483906767,
90.9138669823192));
#172002=CARTESIAN_POINT('Ctrl Pts',(0.0927379508235669,8.12475099746668,
90.9122271246504));
#172003=CARTESIAN_POINT('Ctrl Pts',(0.114906889447252,8.12446770621411,
90.9113605407372));
#172004=CARTESIAN_POINT('Ctrl Pts',(0.174678528441149,8.12345920433265,
90.9090270437801));
#172005=CARTESIAN_POINT('Ctrl Pts',(0.212277884514604,8.12256364399469,
90.9075623332755));
#172006=CARTESIAN_POINT('Ctrl Pts',(0.410289533637737,8.11647145733545,
90.8998621735274));
#172007=CARTESIAN_POINT('Ctrl Pts',(0.570529328250431,8.10678380248141,
90.8936771121736));
#172008=CARTESIAN_POINT('Ctrl Pts',(0.738146505853616,8.09165546339017,
90.8872105155033));
#172009=CARTESIAN_POINT('Ctrl Pts',(0.745913905541872,8.09094313710647,
90.8869108613));
#172010=CARTESIAN_POINT('Ctrl Pts',(0.758089991739835,8.08980881982631,
90.8864411332733));
#172011=CARTESIAN_POINT('Ctrl Pts',(0.762499378216574,8.08939440719417,
90.8862710296603));
#172012=CARTESIAN_POINT('Ctrl Pts',(0.781046822311683,8.08763594104981,
90.8855555156225));
#172013=CARTESIAN_POINT('Ctrl Pts',(0.795181686806233,8.08625842642055,
90.8850102330142));
#172014=CARTESIAN_POINT('Ctrl Pts',(1.12919074835057,8.05282329303902,90.872124606117));
#172015=CARTESIAN_POINT('Ctrl Pts',(1.44688541287374,8.00184708589281,90.8598458307875));
#172016=CARTESIAN_POINT('Ctrl Pts',(1.93827518125358,7.89277233559349,90.8404401137499));
#172017=CARTESIAN_POINT('Ctrl Pts',(2.11445313590129,7.84741057932555,90.8333994335378));
#172018=CARTESIAN_POINT('Ctrl Pts',(2.35772816594149,7.77598497455932,90.8235285081678));
#172019=CARTESIAN_POINT('Ctrl Pts',(2.42622699535237,7.75488535914606,90.8207325924299));
#172020=CARTESIAN_POINT('Ctrl Pts',(2.54659262998274,7.71605836839085,90.8157890045708));
#172021=CARTESIAN_POINT('Ctrl Pts',(2.59857611638289,7.69870722320487,90.8136437870903));
#172022=CARTESIAN_POINT('Ctrl Pts',(2.71067162346707,7.66002707710682,90.808995434294));
#172023=CARTESIAN_POINT('Ctrl Pts',(2.77071608130908,7.63851345698321,90.8064914001613));
#172024=CARTESIAN_POINT('Ctrl Pts',(3.03093284557207,7.54180715014992,90.7955776631422));
#172025=CARTESIAN_POINT('Ctrl Pts',(3.22834564226186,7.4594364886134,90.7871351198037));
#172026=CARTESIAN_POINT('Ctrl Pts',(3.54045019912149,7.31449767165344,90.773550565359));
#172027=CARTESIAN_POINT('Ctrl Pts',(3.65728548036502,7.25678488788619,90.7684101444369));
#172028=CARTESIAN_POINT('Ctrl Pts',(3.81195001304269,7.17570138576113,90.7615432441467));
#172029=CARTESIAN_POINT('Ctrl Pts',(3.85104835727102,7.15479418616419,90.7598019306484));
#172030=CARTESIAN_POINT('Ctrl Pts',(3.92888211788227,7.11235101013043,90.7563255647697));
#172031=CARTESIAN_POINT('Ctrl Pts',(3.96761638651186,7.09081601890673,90.7545905690342));
#172032=CARTESIAN_POINT('Ctrl Pts',(4.10405017880955,7.01349532079928,90.7484585266022));
#172033=CARTESIAN_POINT('Ctrl Pts',(4.20076544139305,6.95599844363115,90.7440733338596));
#172034=CARTESIAN_POINT('Ctrl Pts',(4.42753385257603,6.8147306344274,90.7336672442611));
#172035=CARTESIAN_POINT('Ctrl Pts',(4.55644995166325,6.7292178913974,90.7276510921494));
#172036=CARTESIAN_POINT('Ctrl Pts',(4.74299420821402,6.59765947673265,90.7187522013933));
#172037=CARTESIAN_POINT('Ctrl Pts',(4.80256259945274,6.55442576203791,90.7158804005881));
#172038=CARTESIAN_POINT('Ctrl Pts',(4.91349660793744,6.47158745378478,90.7104702896059));
#172039=CARTESIAN_POINT('Ctrl Pts',(4.96499144285993,6.43216550043001,90.7079331248165));
#172040=CARTESIAN_POINT('Ctrl Pts',(5.05903336332086,6.3583692872391,90.7032489603322));
#172041=CARTESIAN_POINT('Ctrl Pts',(5.10171594507861,6.3241736974093,90.7011032320043));
#172042=CARTESIAN_POINT('Ctrl Pts',(5.19745837952696,6.24586859217749,90.6962434586398));
#172043=CARTESIAN_POINT('Ctrl Pts',(5.2503080970434,6.20150892200208,90.6935277699459));
#172044=CARTESIAN_POINT('Ctrl Pts',(5.42107198749079,6.05442974433913,90.6846400050332));
#172045=CARTESIAN_POINT('Ctrl Pts',(5.53658609489731,5.94897930780426,90.6784475269729));
#172046=CARTESIAN_POINT('Ctrl Pts',(5.708784618676,5.78242055209065,90.6689219859997));
#172047=CARTESIAN_POINT('Ctrl Pts',(5.76769264749142,5.72366409826613,90.6656076192812));
#172048=CARTESIAN_POINT('Ctrl Pts',(6.05595737740519,5.42717110802156,90.649107262818));
#172049=CARTESIAN_POINT('Ctrl Pts',(6.2715688290078,5.17650747689679,90.6358455569801));
#172050=CARTESIAN_POINT('Ctrl Pts',(6.52492714692229,4.84281646419253,90.6191435876034));
#172051=CARTESIAN_POINT('Ctrl Pts',(6.57737322787202,4.77134228053209,90.6156185724485));
#172052=CARTESIAN_POINT('Ctrl Pts',(6.6636150196082,4.64968600562255,90.609712239386));
#172053=CARTESIAN_POINT('Ctrl Pts',(6.69803878232654,4.59995887194802,90.6073236300737));
#172054=CARTESIAN_POINT('Ctrl Pts',(6.7468094438123,4.52779840622776,90.6038960850108));
#172055=CARTESIAN_POINT('Ctrl Pts',(6.76160614039066,4.50567181318994,90.602850254712));
#172056=CARTESIAN_POINT('Ctrl Pts',(6.78729471093643,4.46684626232615,90.6010243560557));
#172057=CARTESIAN_POINT('Ctrl Pts',(6.79823433602036,4.45017920316605,90.6002434809412));
#172058=CARTESIAN_POINT('Ctrl Pts',(6.82102753581601,4.41517244958797,90.5986096455649));
#172059=CARTESIAN_POINT('Ctrl Pts',(6.83286870397685,4.39682495473045,90.5977569482588));
#172060=CARTESIAN_POINT('Ctrl Pts',(6.8678157767539,4.34219350105677,90.5952285383212));
#172061=CARTESIAN_POINT('Ctrl Pts',(6.89070769285334,4.30577350392393,90.5935566521223));
#172062=CARTESIAN_POINT('Ctrl Pts',(7.01128707904653,4.11051260733063,90.5846595043369));
#172063=CARTESIAN_POINT('Ctrl Pts',(7.10377486359895,3.94852434612612,90.5775097858551));
#172064=CARTESIAN_POINT('Ctrl Pts',(7.29946042047614,3.57662015134091,90.5614204825523));
#172065=CARTESIAN_POINT('Ctrl Pts',(7.39933384346655,3.36514372325678,90.5524925014136));
#172066=CARTESIAN_POINT('Ctrl Pts',(7.5151754928027,3.08966982036721,90.5409917619867));
#172067=CARTESIAN_POINT('Ctrl Pts',(7.53967931108845,3.02938246532366,90.5384828334626));
#172068=CARTESIAN_POINT('Ctrl Pts',(7.59557543996705,2.88697918405588,90.5325712458664));
#172069=CARTESIAN_POINT('Ctrl Pts',(7.62636444839535,2.80463548864361,90.5291642165655));
#172070=CARTESIAN_POINT('Ctrl Pts',(7.67031490120036,2.68101315291072,90.5240612195728));
#172071=CARTESIAN_POINT('Ctrl Pts',(7.68449230917389,2.64010229737503,90.52237441491));
#172072=CARTESIAN_POINT('Ctrl Pts',(7.70955205335733,2.56587662228152,90.5193170146055));
#172073=CARTESIAN_POINT('Ctrl Pts',(7.72054713774887,2.53260095309486,90.5179474597811));
#172074=CARTESIAN_POINT('Ctrl Pts',(7.74389349593736,2.46038011108299,90.5149771127785));
#172075=CARTESIAN_POINT('Ctrl Pts',(7.75616698953386,2.42141082461412,90.5133756762879));
#172076=CARTESIAN_POINT('Ctrl Pts',(7.7896006515906,2.31239347205932,90.5088989331611));
#172077=CARTESIAN_POINT('Ctrl Pts',(7.81010919269671,2.24214990342071,90.5060181752852));
#172078=CARTESIAN_POINT('Ctrl Pts',(7.90802502920438,1.88912243097763,90.4915574114181));
#172079=CARTESIAN_POINT('Ctrl Pts',(7.9710347882669,1.60257423619999,90.4798633240962));
#172080=CARTESIAN_POINT('Ctrl Pts',(8.03709931818856,1.19919940771406,90.4635632038446));
#172081=CARTESIAN_POINT('Ctrl Pts',(8.05334343845133,1.0847600271667,90.4589582474047));
#172082=CARTESIAN_POINT('Ctrl Pts',(8.07542142679531,0.901147770464904,
90.4516179620861));
#172083=CARTESIAN_POINT('Ctrl Pts',(8.08281983295966,0.832179166244986,
90.448871669956));
#172084=CARTESIAN_POINT('Ctrl Pts',(8.09185129570428,0.736443058619626,
90.445078571604));
#172085=CARTESIAN_POINT('Ctrl Pts',(8.0942362859731,0.709749761734331,90.4440230282214));
#172086=CARTESIAN_POINT('Ctrl Pts',(8.09808970661824,0.664073160073507,
90.4422206475326));
#172087=CARTESIAN_POINT('Ctrl Pts',(8.09962355277197,0.645095624372311,
90.4414729304123));
#172088=CARTESIAN_POINT('Ctrl Pts',(8.10263537568211,0.606126529522303,
90.4399400016355));
#172089=CARTESIAN_POINT('Ctrl Pts',(8.1041060961854,0.586134613656314,90.4391549295779));
#172090=CARTESIAN_POINT('Ctrl Pts',(8.10797637599821,0.530723036462772,
90.4369826175858));
#172091=CARTESIAN_POINT('Ctrl Pts',(8.1102178121944,0.495292754092089,90.4355977436771));
#172092=CARTESIAN_POINT('Ctrl Pts',(8.1209324651078,0.30627476080668,90.4282290802179));
#172093=CARTESIAN_POINT('Ctrl Pts',(8.12527528680073,0.152482634071241,
90.4223022292362));
#172094=CARTESIAN_POINT('Ctrl Pts',(8.12518271962617,-0.408164824613424,
90.4008194375387));
#172095=CARTESIAN_POINT('Ctrl Pts',(8.09456184015827,-0.814411358661026,
90.3854750239771));
#172096=CARTESIAN_POINT('Ctrl Pts',(8.01329831773149,-1.35099982575277,
90.3648074063706));
#172097=CARTESIAN_POINT('Ctrl Pts',(7.98958556584053,-1.48481400039786,
90.3596212478413));
#172098=CARTESIAN_POINT('Ctrl Pts',(7.91719876860025,-1.84105174690529,
90.3456915675978));
#172099=CARTESIAN_POINT('Ctrl Pts',(7.8625146010107,-2.06212749824494,90.3369157345911));
#172100=CARTESIAN_POINT('Ctrl Pts',(7.77992147002927,-2.34455711449415,
90.3254753073271));
#172101=CARTESIAN_POINT('Ctrl Pts',(7.76043598262427,-2.40826897211862,
90.3228793279538));
#172102=CARTESIAN_POINT('Ctrl Pts',(7.72766479458903,-2.51089108532431,
90.3186721328723));
#172103=CARTESIAN_POINT('Ctrl Pts',(7.71486341593251,-2.5499528778852,90.3170646257152));
#172104=CARTESIAN_POINT('Ctrl Pts',(7.68968758102669,-2.62484847594072,
90.3139704637209));
#172105=CARTESIAN_POINT('Ctrl Pts',(7.67735765767219,-2.66069614969036,
90.3124841709913));
#172106=CARTESIAN_POINT('Ctrl Pts',(7.64810768966756,-2.74384027633678,
90.3090243208187));
#172107=CARTESIAN_POINT('Ctrl Pts',(7.63099903444572,-2.79106868554986,
90.3070494925645));
#172108=CARTESIAN_POINT('Ctrl Pts',(7.57333148197439,-2.94576505771821,
90.3005490832461));
#172109=CARTESIAN_POINT('Ctrl Pts',(7.53093176954014,-3.05253140006581,
90.2960117301884));
#172110=CARTESIAN_POINT('Ctrl Pts',(7.24063132542835,-3.74063207893818,
90.2664312475233));
#172111=CARTESIAN_POINT('Ctrl Pts',(6.92790189115822,-4.29222494661871,
90.24109092315));
#172112=CARTESIAN_POINT('Ctrl Pts',(6.30402987340626,-5.14377472163197,
90.196923818038));
#172113=CARTESIAN_POINT('Ctrl Pts',(6.02728066116209,-5.46544475642925,
90.1788354203407));
#172114=CARTESIAN_POINT('Ctrl Pts',(5.54484102054954,-5.94475867008302,
90.150300386213));
#172115=CARTESIAN_POINT('Ctrl Pts',(5.35450697115553,-6.11675429334298,
90.1396870958048));
#172116=CARTESIAN_POINT('Ctrl Pts',(5.14095158550991,-6.29211423239948,
90.1286948831446));
#172117=CARTESIAN_POINT('Ctrl Pts',(5.12550340574968,-6.30470455803753,
90.1279047007098));
#172118=CARTESIAN_POINT('Ctrl Pts',(5.10250147082359,-6.32331080563039,
90.1267356930883));
#172119=CARTESIAN_POINT('Ctrl Pts',(5.0949831203597,-6.32937025371377,90.1263547853934));
#172120=CARTESIAN_POINT('Ctrl Pts',(5.08208854918351,-6.33972482777154,
90.1257035608141));
#172121=CARTESIAN_POINT('Ctrl Pts',(5.07671764991323,-6.34402654605534,
90.1254329208068));
#172122=CARTESIAN_POINT('Ctrl Pts',(5.06568701152103,-6.35283834494368,
90.124878349087));
#172123=CARTESIAN_POINT('Ctrl Pts',(5.06002669775017,-6.35734769806882,
90.1245944536989));
#172124=CARTESIAN_POINT('Ctrl Pts',(5.04694262298147,-6.36774273002923,
90.1239398002049));
#172125=CARTESIAN_POINT('Ctrl Pts',(5.03951456869824,-6.37362300645182,
90.1235693162647));
#172126=CARTESIAN_POINT('Ctrl Pts',(5.01621366711223,-6.39200251759296,
90.1224108716322));
#172127=CARTESIAN_POINT('Ctrl Pts',(5.00030439782131,-6.40445561137356,
90.121625305358));
#172128=CARTESIAN_POINT('Ctrl Pts',(4.71661439354119,-6.62481452121287,
90.1077153933778));
#172129=CARTESIAN_POINT('Ctrl Pts',(4.43612901854739,-6.81581818552268,
90.09562272667));
#172130=CARTESIAN_POINT('Ctrl Pts',(3.95773085766111,-7.09952262916357,
90.0765072060474));
#172131=CARTESIAN_POINT('Ctrl Pts',(3.76655789871067,-7.20277030281036,
90.0692263203532));
#172132=CARTESIAN_POINT('Ctrl Pts',(3.32598231851155,-7.41837101108613,
90.0528514664966));
#172133=CARTESIAN_POINT('Ctrl Pts',(3.0745850425301,-7.52604224681035,90.0437827234198));
#172134=CARTESIAN_POINT('Ctrl Pts',(2.32875672566864,-7.80185513884065,
90.0168251869194));
#172135=CARTESIAN_POINT('Ctrl Pts',(1.823023844337,-7.9352732018687,89.9984035940042));
#172136=CARTESIAN_POINT('Ctrl Pts',(1.27586993066572,-8.02451894913138,
89.9770927868911));
#172137=CARTESIAN_POINT('Ctrl Pts',(1.24369254336064,-8.0295689344628,89.9758349492949));
#172138=CARTESIAN_POINT('Ctrl Pts',(1.19896070361978,-8.03631390879297,
89.9740798262728));
#172139=CARTESIAN_POINT('Ctrl Pts',(1.18643116187188,-8.03817324433148,
89.9735875008642));
#172140=CARTESIAN_POINT('Ctrl Pts',(1.16485239359985,-8.04132389716096,
89.9727383706191));
#172141=CARTESIAN_POINT('Ctrl Pts',(1.15580522572121,-8.04262925898276,
89.9723819896282));
#172142=CARTESIAN_POINT('Ctrl Pts',(1.13713608098323,-8.04529076649055,
89.9716458120258));
#172143=CARTESIAN_POINT('Ctrl Pts',(1.12751383723432,-8.04664492382568,
89.9712659561655));
#172144=CARTESIAN_POINT('Ctrl Pts',(1.10512450221637,-8.04975487070984,
89.9703811051861));
#172145=CARTESIAN_POINT('Ctrl Pts',(1.09235563313169,-8.05149755094252,
89.9698757166854));
#172146=CARTESIAN_POINT('Ctrl Pts',(1.05170670172599,-8.05694679221253,
89.9682644424323));
#172147=CARTESIAN_POINT('Ctrl Pts',(1.02381165478707,-8.06053895687019,
89.9671551248516));
#172148=CARTESIAN_POINT('Ctrl Pts',(0.482310945039678,-8.12741405226549,
89.9455503650096));
#172149=CARTESIAN_POINT('Ctrl Pts',(-0.0360949542220756,-8.14162538655109,
89.9235322627249));
#172150=CARTESIAN_POINT('Ctrl Pts',(-1.32616396610698,-8.05373574904508,
89.8662998001465));
#172151=CARTESIAN_POINT('Ctrl Pts',(-2.08855333395648,-7.89046719698669,
89.8301401358532));
#172152=CARTESIAN_POINT('Ctrl Pts',(-2.85440477185994,-7.60747762182899,
89.7971850584204));
#172153=CARTESIAN_POINT('Ctrl Pts',(-2.89245649945786,-7.5930914555651,
89.795556835486));
#172154=CARTESIAN_POINT('Ctrl Pts',(-2.9428712085305,-7.57359725792394,
89.7934100585827));
#172155=CARTESIAN_POINT('Ctrl Pts',(-2.95533147886672,-7.56874376816158,
89.7928803237333));
#172156=CARTESIAN_POINT('Ctrl Pts',(-2.97470799792059,-7.5611411360792,
89.7920578082562));
#172157=CARTESIAN_POINT('Ctrl Pts',(-2.98163251272359,-7.55841322713757,
89.7917641191758));
#172158=CARTESIAN_POINT('Ctrl Pts',(-2.9955271003613,-7.55291739637152,
89.7911752953547));
#172159=CARTESIAN_POINT('Ctrl Pts',(-3.00249710806778,-7.55014933110006,
89.7908801671053));
#172160=CARTESIAN_POINT('Ctrl Pts',(-3.01810397394759,-7.54392619908828,
89.7902198655022));
#172161=CARTESIAN_POINT('Ctrl Pts',(-3.0267387595794,-7.54046593898535,
89.7898549081862));
#172162=CARTESIAN_POINT('Ctrl Pts',(-3.05215445995236,-7.53023028988641,
89.7887817248986));
#172163=CARTESIAN_POINT('Ctrl Pts',(-3.06891876230982,-7.52341363363619,
89.7880751796552));
#172164=CARTESIAN_POINT('Ctrl Pts',(-3.19928011008044,-7.46989821653667,
89.7825904880507));
#172165=CARTESIAN_POINT('Ctrl Pts',(-3.31183102438735,-7.42068389556017,
89.7779111824683));
#172166=CARTESIAN_POINT('Ctrl Pts',(-3.72771337855501,-7.22748650304879,
89.7607044202216));
#172167=CARTESIAN_POINT('Ctrl Pts',(-4.02315272642039,-7.06729555358356,
89.7486366167324));
#172168=CARTESIAN_POINT('Ctrl Pts',(-4.84462124104432,-6.55363441005245,
89.7138484427421));
#172169=CARTESIAN_POINT('Ctrl Pts',(-5.34030911041913,-6.15642295476436,
89.6910921975045));
#172170=CARTESIAN_POINT('Ctrl Pts',(-5.84624133465654,-5.64347342438746,
89.6635593193846));
#172171=CARTESIAN_POINT('Ctrl Pts',(-5.90662120225961,-5.5802469238601,
89.6601975851622));
#172172=CARTESIAN_POINT('Ctrl Pts',(-5.98906348670876,-5.49108035128396,
89.6554997013062));
#172173=CARTESIAN_POINT('Ctrl Pts',(-6.01200125196499,-5.46595698875673,
89.6541806740617));
#172174=CARTESIAN_POINT('Ctrl Pts',(-6.04866033216221,-5.42529496140551,
89.6520532826715));
#172175=CARTESIAN_POINT('Ctrl Pts',(-6.06248118476256,-5.40984649626293,
89.6512467452121));
#172176=CARTESIAN_POINT('Ctrl Pts',(-6.09077363225227,-5.37797760990128,
89.6495864444536));
#172177=CARTESIAN_POINT('Ctrl Pts',(-6.10523830978567,-5.36155124843075,
89.6487325802365));
#172178=CARTESIAN_POINT('Ctrl Pts',(-6.1375795416018,-5.32452335118314,
89.6468119736052));
#172179=CARTESIAN_POINT('Ctrl Pts',(-6.15541906715872,-5.30388985994851,
89.6457445852264));
#172180=CARTESIAN_POINT('Ctrl Pts',(-6.20822378785311,-5.24218980580471,
89.6425608500608));
#172181=CARTESIAN_POINT('Ctrl Pts',(-6.24288418163928,-5.2008646963119,
89.6404389984451));
#172182=CARTESIAN_POINT('Ctrl Pts',(-6.65728776487264,-4.69666512462372,
89.6146659730834));
#172183=CARTESIAN_POINT('Ctrl Pts',(-6.98513006277759,-4.19356681760353,
89.5899124066949));
#172184=CARTESIAN_POINT('Ctrl Pts',(-7.30206009909252,-3.5652012278945,
89.5601061331467));
#172185=CARTESIAN_POINT('Ctrl Pts',(-7.34758055389546,-3.4704180445728,
89.5556436407094));
#172186=CARTESIAN_POINT('Ctrl Pts',(-7.53587425402126,-3.05802784377165,
89.5364055710946));
#172187=CARTESIAN_POINT('Ctrl Pts',(-7.65999263378856,-2.73229944403452,
89.5216399975741));
#172188=CARTESIAN_POINT('Ctrl Pts',(-7.78960354694572,-2.31300265156048,
89.5037336892653));
#172189=CARTESIAN_POINT('Ctrl Pts',(-7.81492387124996,-2.22595378264975,
89.5000754152648));
#172190=CARTESIAN_POINT('Ctrl Pts',(-7.84301194590939,-2.12299538157213,
89.4958302426727));
#172191=CARTESIAN_POINT('Ctrl Pts',(-7.84719518148492,-2.10748038231436,
89.4951927023057));
#172192=CARTESIAN_POINT('Ctrl Pts',(-7.85384187502791,-2.08253460200741,
89.4941712200543));
#172193=CARTESIAN_POINT('Ctrl Pts',(-7.85633442603922,-2.0731116597331,
89.493786189224));
#172194=CARTESIAN_POINT('Ctrl Pts',(-7.86073277071643,-2.05636212280665,
89.4931032684786));
#172195=CARTESIAN_POINT('Ctrl Pts',(-7.86264528963465,-2.04903731605556,
89.4928051206491));
#172196=CARTESIAN_POINT('Ctrl Pts',(-7.86660738779841,-2.03377554427642,
89.4921849685775));
#172197=CARTESIAN_POINT('Ctrl Pts',(-7.86865519940246,-2.02583812576148,
89.4918630337216));
#172198=CARTESIAN_POINT('Ctrl Pts',(-7.8739286966889,-2.00526915955052,
89.4910303414374));
#172199=CARTESIAN_POINT('Ctrl Pts',(-7.87713600710106,-1.99263289417064,
89.4905203179258));
#172200=CARTESIAN_POINT('Ctrl Pts',(-7.89060168345194,-1.93903979467075,
89.4883638223817));
#172201=CARTESIAN_POINT('Ctrl Pts',(-7.90057125945608,-1.89801056811157,
89.4867292523952));
#172202=CARTESIAN_POINT('Ctrl Pts',(-7.96767364179614,-1.61216145065336,
89.4754630653817));
#172203=CARTESIAN_POINT('Ctrl Pts',(-8.01373824124433,-1.36487827364246,
89.466364858333));
#172204=CARTESIAN_POINT('Ctrl Pts',(-8.11173717626938,-0.658045495434903,
89.4413578800126));
#172205=CARTESIAN_POINT('Ctrl Pts',(-8.13603435273741,-0.195644302811646,
89.4261405526653));
#172206=CARTESIAN_POINT('Ctrl Pts',(-8.10888515299584,0.632203037266909,
89.3980883161775));
#172207=CARTESIAN_POINT('Ctrl Pts',(-8.07217407440557,0.996837365785144,
89.3854525729938));
#172208=CARTESIAN_POINT('Ctrl Pts',(-7.97552435984112,1.56709534165181,
89.3644266744));
#172209=CARTESIAN_POINT('Ctrl Pts',(-7.93185036206105,1.77497019717706,
89.3564950543029));
#172210=CARTESIAN_POINT('Ctrl Pts',(-7.87405094778067,2.00489954792567,
89.3473587460818));
#172211=CARTESIAN_POINT('Ctrl Pts',(-7.86790538911031,2.02888277156754,
89.3464013404125));
#172212=CARTESIAN_POINT('Ctrl Pts',(-7.85850276855301,2.06489152452899,
89.3449571304162));
#172213=CARTESIAN_POINT('Ctrl Pts',(-7.85532748201763,2.07693835249014,
89.3444728280881));
#172214=CARTESIAN_POINT('Ctrl Pts',(-7.84978847673069,2.09775856379603,
89.3436338406103));
#172215=CARTESIAN_POINT('Ctrl Pts',(-7.84743772080945,2.10653538749041,
89.3432795532693));
#172216=CARTESIAN_POINT('Ctrl Pts',(-7.84253419964623,2.12472114275437,
89.3425441933551));
#172217=CARTESIAN_POINT('Ctrl Pts',(-7.83997921313987,2.13412945808166,
89.3421630530401));
#172218=CARTESIAN_POINT('Ctrl Pts',(-7.83395520332092,2.15615506516431,
89.3412691138995));
#172219=CARTESIAN_POINT('Ctrl Pts',(-7.8304726252741,2.1687686035123,89.3407558991244));
#172220=CARTESIAN_POINT('Ctrl Pts',(-7.8191221785521,2.20949500011694,89.3390946884782));
#172221=CARTESIAN_POINT('Ctrl Pts',(-7.81113330752014,2.23757373717886,
89.337942970676));
#172222=CARTESIAN_POINT('Ctrl Pts',(-7.69242828774203,2.64640625297348,
89.3210793096807));
#172223=CARTESIAN_POINT('Ctrl Pts',(-7.55414855445613,3.01856015283658,
89.3044967474096));
#172224=CARTESIAN_POINT('Ctrl Pts',(-7.15226094770793,3.89738907133433,
89.2624376826757));
#172225=CARTESIAN_POINT('Ctrl Pts',(-6.86138408668688,4.38928467715351,
89.2363024335274));
#172226=CARTESIAN_POINT('Ctrl Pts',(-6.29179464735972,5.15570291752874,
89.1937509860266));
#172227=CARTESIAN_POINT('Ctrl Pts',(-6.04039578984724,5.448088970018,89.1770341733334));
#172228=CARTESIAN_POINT('Ctrl Pts',(-5.75242219518411,5.73845723051182,
89.1607068087172));
#172229=CARTESIAN_POINT('Ctrl Pts',(-5.73561105045182,5.75526006304766,
89.1597625772463));
#172230=CARTESIAN_POINT('Ctrl Pts',(-5.71207265279435,5.77858125323408,
89.1584524631018));
#172231=CARTESIAN_POINT('Ctrl Pts',(-5.70540760142429,5.7851620023687,89.1580828229311));
#172232=CARTESIAN_POINT('Ctrl Pts',(-5.69388160661996,5.7965029198255,89.1574458540481));
#172233=CARTESIAN_POINT('Ctrl Pts',(-5.68902604513137,5.80126852575976,
89.157178206343));
#172234=CARTESIAN_POINT('Ctrl Pts',(-5.67896664127495,5.81111679136435,
89.1566251218141));
#172235=CARTESIAN_POINT('Ctrl Pts',(-5.6737619468636,5.81619857349645,89.1563397354763));
#172236=CARTESIAN_POINT('Ctrl Pts',(-5.66158972521399,5.82805145306758,
89.1556740961599));
#172237=CARTESIAN_POINT('Ctrl Pts',(-5.65461685455987,5.83481706529293,
89.1552941522696));
#172238=CARTESIAN_POINT('Ctrl Pts',(-5.63249210562934,5.85620727938735,
89.1540928640061));
#172239=CARTESIAN_POINT('Ctrl Pts',(-5.61729543024625,5.87078555891169,
89.1532740570907));
#172240=CARTESIAN_POINT('Ctrl Pts',(-5.47611900656491,6.0051670942049,89.1457237655605));
#172241=CARTESIAN_POINT('Ctrl Pts',(-5.34637635352792,6.12096197293031,
89.1391974955641));
#172242=CARTESIAN_POINT('Ctrl Pts',(-5.0626159403596,6.35830575418146,89.1255550559194));
#172243=CARTESIAN_POINT('Ctrl Pts',(-4.90770986836957,6.47862014829483,
89.1184738842969));
#172244=CARTESIAN_POINT('Ctrl Pts',(-4.50287078323803,6.77019554513883,
89.1005546120604));
#172245=CARTESIAN_POINT('Ctrl Pts',(-4.24744016081709,6.93329973721904,
89.0897750202761));
#172246=CARTESIAN_POINT('Ctrl Pts',(-3.4331266125429,7.39135209565812,89.0559827931577));
#172247=CARTESIAN_POINT('Ctrl Pts',(-2.84856797903184,7.63570676960402,
89.0322819002105));
#172248=CARTESIAN_POINT('Ctrl Pts',(-2.1276827222347,7.8426218416518,89.003321133802));
#172249=CARTESIAN_POINT('Ctrl Pts',(-2.01299352668427,7.87283988335273,
88.99872487553));
#172250=CARTESIAN_POINT('Ctrl Pts',(-1.85187465694265,7.91154014506264,
88.9922728041213));
#172251=CARTESIAN_POINT('Ctrl Pts',(-1.80596976234776,7.92214493713761,
88.9904350909155));
#172252=CARTESIAN_POINT('Ctrl Pts',(-1.72237544491579,7.94069227076996,
88.9870888384705));
#172253=CARTESIAN_POINT('Ctrl Pts',(-1.68471677375682,7.94876721830031,
88.9855814793114));
#172254=CARTESIAN_POINT('Ctrl Pts',(-1.61263649592199,7.96368775760905,
88.9826961432325));
#172255=CARTESIAN_POINT('Ctrl Pts',(-1.57822513552084,7.97057868536676,
88.9813185932865));
#172256=CARTESIAN_POINT('Ctrl Pts',(-1.49382681276644,7.98691159221029,
88.9779394344096));
#172257=CARTESIAN_POINT('Ctrl Pts',(-1.44379383382703,7.99610746931643,
88.9759357383075));
#172258=CARTESIAN_POINT('Ctrl Pts',(-1.26794906118604,8.02672284740343,
88.9688906615199));
#172259=CARTESIAN_POINT('Ctrl Pts',(-1.14172292393769,8.04564744087221,
88.9638280864338));
#172260=CARTESIAN_POINT('Ctrl Pts',(-0.831910395821181,8.08465861124717,
88.9513790554654));
#172261=CARTESIAN_POINT('Ctrl Pts',(-0.647985112404765,8.10147478662085,
88.943968090165));
#172262=CARTESIAN_POINT('Ctrl Pts',(-0.179362750217856,8.12825929532021,
88.9250265478514));
#172263=CARTESIAN_POINT('Ctrl Pts',(0.105579271624881,8.1295523276579,88.9134511427758));
#172264=CARTESIAN_POINT('Ctrl Pts',(0.495012894545222,8.11083864444987,
88.8976078253616));
#172265=CARTESIAN_POINT('Ctrl Pts',(0.599920788761437,8.1037544649407,88.8933381627985));
#172266=CARTESIAN_POINT('Ctrl Pts',(0.864935160890542,8.08068418790813,
88.8825583506172));
#172267=CARTESIAN_POINT('Ctrl Pts',(1.02476030812926,8.06197476037542,88.8760626490737));
#172268=CARTESIAN_POINT('Ctrl Pts',(1.28179714072594,8.02411803545976,88.865655261502));
#172269=CARTESIAN_POINT('Ctrl Pts',(1.37939809289287,8.00791704707015,88.8617127388967));
#172270=CARTESIAN_POINT('Ctrl Pts',(1.5071516391476,7.98430596572611,88.8565713278));
#172271=CARTESIAN_POINT('Ctrl Pts',(1.53759121642721,7.97849992685588,88.8553477302));
#172272=CARTESIAN_POINT('Ctrl Pts',(1.58498171275378,7.96917939150578,88.8534452514913));
#172273=CARTESIAN_POINT('Ctrl Pts',(1.60195574489754,7.96578464418748,88.8527643498375));
#172274=CARTESIAN_POINT('Ctrl Pts',(1.63419410754808,7.95922987226993,88.8514720600122));
#172275=CARTESIAN_POINT('Ctrl Pts',(1.64946038657398,7.95608012627226,88.8508604902488));
#172276=CARTESIAN_POINT('Ctrl Pts',(1.66476845224285,7.95287580474031,88.8502475762809));
#172277=CARTESIAN_POINT('Ctrl Pts',(1.66481937012427,7.95286514597504,88.8502455376023));
#172278=CARTESIAN_POINT('Ctrl Pts',(1.66492108428459,7.95284385288047,88.8502414651214));
#172279=CARTESIAN_POINT('Ctrl Pts',(1.66497188694735,7.95283321721693,88.8502394310633));
#172280=CARTESIAN_POINT('Ctrl Pts',(1.66507338034592,7.95281196830691,88.8502353674359));
#172281=CARTESIAN_POINT('Ctrl Pts',(1.66512407112647,7.95280135505329,88.8502333378648));
#172282=CARTESIAN_POINT('Ctrl Pts',(1.66522534182941,7.952780150746,88.8502292831682));
#172283=CARTESIAN_POINT('Ctrl Pts',(1.66527592187131,7.95276955966952,88.850227258038));
#172284=CARTESIAN_POINT('Ctrl Pts',(1.66537697233916,7.95274839946301,88.8502232121737));
#172285=CARTESIAN_POINT('Ctrl Pts',(1.66542744284085,7.95273783031929,88.8502211914365));
#172286=CARTESIAN_POINT('Ctrl Pts',(1.66552827521413,7.95271671377837,88.8502171543186));
#172287=CARTESIAN_POINT('Ctrl Pts',(1.66557863719679,7.95270616636006,88.8502151379335));
#172288=CARTESIAN_POINT('Ctrl Pts',(1.66567925431037,7.95268509290393,88.8502111094484));
#172289=CARTESIAN_POINT('Ctrl Pts',(1.6657295091604,7.95267456692707,88.8502090973597));
#172290=CARTESIAN_POINT('Ctrl Pts',(1.66582991270533,7.95265353621427,88.8502050774397));
#172291=CARTESIAN_POINT('Ctrl Pts',(1.66588006142232,7.95264303147582,88.8502030696074));
#172292=CARTESIAN_POINT('Ctrl Pts',(1.66598025409047,7.95262204295508,88.8501990581445));
#172293=CARTESIAN_POINT('Ctrl Pts',(1.66603029793201,7.95261155919782,88.8501970545182));
#172294=CARTESIAN_POINT('Ctrl Pts',(1.66613028170609,7.9525906124662,88.850193051433));
#172295=CARTESIAN_POINT('Ctrl Pts',(1.66618022176059,7.9525801494683,88.8501910519692));
#172296=CARTESIAN_POINT('Ctrl Pts',(1.66627999872396,7.95255924410156,88.8501870571781));
#172297=CARTESIAN_POINT('Ctrl Pts',(1.66632983587104,7.95254880168483,88.8501850618413));
#172298=CARTESIAN_POINT('Ctrl Pts',(1.66642940900573,7.95252793707027,88.8501810752249));
#172299=CARTESIAN_POINT('Ctrl Pts',(1.66647914463274,7.95251751494999,88.8501790839597));
#172300=CARTESIAN_POINT('Ctrl Pts',(1.66657851568945,7.95249669073268,88.8501751054478));
#172301=CARTESIAN_POINT('Ctrl Pts',(1.66662815099231,7.95248628866418,88.8501731182062));
#172302=CARTESIAN_POINT('Ctrl Pts',(1.66672732160777,7.95246550451291,88.8501691477331));
#172303=CARTESIAN_POINT('Ctrl Pts',(1.66677685731049,7.95245512235032,88.8501671644861));
#172304=CARTESIAN_POINT('Ctrl Pts',(1.66687583076972,7.95243437758824,88.8501632019203));
#172305=CARTESIAN_POINT('Ctrl Pts',(1.66692526833097,7.95242401503159,88.8501612226094));
#172306=CARTESIAN_POINT('Ctrl Pts',(1.66702404567895,7.95240330945115,88.8501572679089));
#172307=CARTESIAN_POINT('Ctrl Pts',(1.6670733858044,7.95239296635825,88.8501552925058));
#172308=CARTESIAN_POINT('Ctrl Pts',(1.66717197016231,7.95237229931652,88.8501513455456));
#172309=CARTESIAN_POINT('Ctrl Pts',(1.66722121416035,7.9523619754187,88.8501493739979));
#172310=CARTESIAN_POINT('Ctrl Pts',(1.66731960715735,7.95234134658532,88.8501454347127));
#172311=CARTESIAN_POINT('Ctrl Pts',(1.66736875606876,7.95233104166995,88.8501434669787));
#172312=CARTESIAN_POINT('Ctrl Pts',(1.66746695988346,7.9523104505992,88.8501395352811));
#172313=CARTESIAN_POINT('Ctrl Pts',(1.66751601478815,7.95230016444533,88.8501375713175));
#172314=CARTESIAN_POINT('Ctrl Pts',(1.66761403137255,7.9522796107388,88.8501336471293));
#172315=CARTESIAN_POINT('Ctrl Pts',(1.66766299322739,7.95226934315121,88.8501316868978));
#172316=CARTESIAN_POINT('Ctrl Pts',(1.6677608247379,7.95224882636747,88.8501277701326));
#172317=CARTESIAN_POINT('Ctrl Pts',(1.66780969448112,7.95223857715474,88.8501258135955));
#172318=CARTESIAN_POINT('Ctrl Pts',(1.6679073434729,7.95221809676855,88.850121904151));
#172319=CARTESIAN_POINT('Ctrl Pts',(1.66795612242823,7.95220786565833,88.8501199512553));
#172320=CARTESIAN_POINT('Ctrl Pts',(1.66805359009366,7.95218742143006,88.8501160490836));
#172321=CARTESIAN_POINT('Ctrl Pts',(1.66810227901195,7.95217720827008,88.8501140997992));
#172322=CARTESIAN_POINT('Ctrl Pts',(1.66819956810043,7.95215679963338,88.8501102047902));
#172323=CARTESIAN_POINT('Ctrl Pts',(1.66824816817235,7.95214660417899,88.8501082590694));
#172324=CARTESIAN_POINT('Ctrl Pts',(1.66834528020997,7.95212623082394,88.8501043711618));
#172325=CARTESIAN_POINT('Ctrl Pts',(1.66839379229784,7.95211605289932,88.85010242897));
#172326=CARTESIAN_POINT('Ctrl Pts',(1.66849072973474,7.95209571432195,88.8500985480657));
#172327=CARTESIAN_POINT('Ctrl Pts',(1.66853915499677,7.9520855536891,88.8500966093566));
#172328=CARTESIAN_POINT('Ctrl Pts',(1.66863591935687,7.95206524957961,88.8500927353945));
#172329=CARTESIAN_POINT('Ctrl Pts',(1.66868425863351,7.95205510606713,88.8500908001344));
#172330=CARTESIAN_POINT('Ctrl Pts',(1.66878085223562,7.95203483594877,88.8500869330216));
#172331=CARTESIAN_POINT('Ctrl Pts',(1.66882910655204,7.9520247093464,88.8500850011693));
#172332=CARTESIAN_POINT('Ctrl Pts',(1.66892553126456,7.95200447283676,88.8500811408309));
#172333=CARTESIAN_POINT('Ctrl Pts',(1.66897370158346,7.95199436294729,88.8500792123479));
#172334=CARTESIAN_POINT('Ctrl Pts',(1.66906995950465,7.95197415961555,88.8500753586999));
#172335=CARTESIAN_POINT('Ctrl Pts',(1.6691180469154,7.95196406621506,88.8500734335425));
#172336=CARTESIAN_POINT('Ctrl Pts',(1.66921413973107,7.95194389571682,88.8500695865173));
#172337=CARTESIAN_POINT('Ctrl Pts',(1.66926214518335,7.95193381861066,88.8500676646475));
#172338=CARTESIAN_POINT('Ctrl Pts',(1.66935807458162,7.95191368060086,88.8500638241774));
#172339=CARTESIAN_POINT('Ctrl Pts',(1.66940599876927,7.95190361964801,88.8500619055674));
#172340=CARTESIAN_POINT('Ctrl Pts',(1.66950176755887,7.9518835135462,88.8500580715399));
#172341=CARTESIAN_POINT('Ctrl Pts',(1.66954961180593,7.95187346847324,88.8500561561366));
#172342=CARTESIAN_POINT('Ctrl Pts',(1.66964522089916,7.95185339409692,88.8500523285151));
#172343=CARTESIAN_POINT('Ctrl Pts',(1.6696929859104,7.95184336476038,88.8500504162903));
#172344=CARTESIAN_POINT('Ctrl Pts',(1.66978843780129,7.95182332159483,88.8500465949749));
#172345=CARTESIAN_POINT('Ctrl Pts',(1.66983612464723,7.95181330777436,88.8500446858856));
#172346=CARTESIAN_POINT('Ctrl Pts',(1.66993142072348,7.95179329553699,88.8500408708207));
#172347=CARTESIAN_POINT('Ctrl Pts',(1.66997903011656,7.95178329708737,88.8500389648385));
#172348=CARTESIAN_POINT('Ctrl Pts',(1.67007417293841,7.95176331524921,88.8500351559215));
#172349=CARTESIAN_POINT('Ctrl Pts',(1.67012170606736,7.95175333192509,88.8500332529987));
#172350=CARTESIAN_POINT('Ctrl Pts',(1.6702166970154,7.95173338020476,88.8500294501743));
#172351=CARTESIAN_POINT('Ctrl Pts',(1.67026415486125,7.95172341180433,88.8500275502716));
#172352=CARTESIAN_POINT('Ctrl Pts',(1.67035899524484,7.95170348993528,88.8500237534872));
#172353=CARTESIAN_POINT('Ctrl Pts',(1.67040637831794,7.95169353635557,88.8500218565841));
#172354=CARTESIAN_POINT('Ctrl Pts',(1.67050107108084,7.95167364372776,88.8500180657219));
#172355=CARTESIAN_POINT('Ctrl Pts',(1.67054838060708,7.95166370471538,88.8500161717694));
#172356=CARTESIAN_POINT('Ctrl Pts',(1.67064292675272,7.95164384112624,88.8500123867892));
#172357=CARTESIAN_POINT('Ctrl Pts',(1.67069016346372,7.95163391653158,88.8500104957578));
#172358=CARTESIAN_POINT('Ctrl Pts',(1.67078456523525,7.95161408151794,88.8500067165697));
#172359=CARTESIAN_POINT('Ctrl Pts',(1.67083173013139,7.95160417113483,88.8500048284194));
#172360=CARTESIAN_POINT('Ctrl Pts',(1.67092598909531,7.95158436437554,88.8500010549605));
#172361=CARTESIAN_POINT('Ctrl Pts',(1.67097308305781,7.9515744680228,88.8499991696561));
#172362=CARTESIAN_POINT('Ctrl Pts',(1.67106720112198,7.95155468912484,88.8499954018501));
#172363=CARTESIAN_POINT('Ctrl Pts',(1.67111422514948,7.95154480659651,88.8499935193515));
#172364=CARTESIAN_POINT('Ctrl Pts',(1.67120820354349,7.95152505530927,88.8499897571491));
#172365=CARTESIAN_POINT('Ctrl Pts',(1.67125515820758,7.95151518648909,88.8499878774334));
#172366=CARTESIAN_POINT('Ctrl Pts',(1.67134899953809,7.9514954622724,88.8499841207301));
#172367=CARTESIAN_POINT('Ctrl Pts',(1.67139588595541,7.95148560692949,88.8499822437525));
#172368=CARTESIAN_POINT('Ctrl Pts',(1.67148959142806,7.95146590953747,88.8499784925001));
#172369=CARTESIAN_POINT('Ctrl Pts',(1.67153641041523,7.95145606750393,88.849976618228));
#172370=CARTESIAN_POINT('Ctrl Pts',(1.67162998189814,7.95143639655136,88.8499728723515));
#172371=CARTESIAN_POINT('Ctrl Pts',(1.67167673435268,7.95142656764221,88.8499710007489));
#172372=CARTESIAN_POINT('Ctrl Pts',(1.67177017332727,7.951406922825,88.8499672601891));
#172373=CARTESIAN_POINT('Ctrl Pts',(1.6718168599382,7.95139710689904,88.8499653912284));
#172374=CARTESIAN_POINT('Ctrl Pts',(1.67191016873911,7.95137748773359,88.8499616558917));
#172375=CARTESIAN_POINT('Ctrl Pts',(1.6719567906492,7.95136768455413,88.849959789527));
#172376=CARTESIAN_POINT('Ctrl Pts',(1.67204997017649,7.95134809085832,88.8499560593773));
#172377=CARTESIAN_POINT('Ctrl Pts',(1.67209652801234,7.95133830029716,88.8499541955836));
#172378=CARTESIAN_POINT('Ctrl Pts',(1.67218958040073,7.95131873162915,88.8499504705355));
#172379=CARTESIAN_POINT('Ctrl Pts',(1.67223607501202,7.9513089535111,88.8499486092787));
#172380=CARTESIAN_POINT('Ctrl Pts',(1.69051708949392,7.94746417026244,88.8492167909699));
#172381=CARTESIAN_POINT('Ctrl Pts',(1.70873839997131,7.94356644402831,88.8484878191919));
#172382=CARTESIAN_POINT('Ctrl Pts',(1.75275318835579,7.93399277376195,88.8467278101983));
#172383=CARTESIAN_POINT('Ctrl Pts',(1.77853274489257,7.92825367630113,88.845697693053));
#172384=CARTESIAN_POINT('Ctrl Pts',(1.84840750267653,7.91234005446961,88.8429068281838));
#172385=CARTESIAN_POINT('Ctrl Pts',(1.89244652377259,7.90192265322539,88.8411492050519));
#172386=CARTESIAN_POINT('Ctrl Pts',(2.03825877972754,7.86614196765674,88.8353299027209));
#172387=CARTESIAN_POINT('Ctrl Pts',(2.13962821389219,7.83917595433868,88.8312843935935));
#172388=CARTESIAN_POINT('Ctrl Pts',(2.51601643308847,7.73120533239011,88.8162090013297));
#172389=CARTESIAN_POINT('Ctrl Pts',(2.78720745961225,7.63762717267808,88.8052285836044));
#172390=CARTESIAN_POINT('Ctrl Pts',(3.13462478321105,7.49677229173001,88.7907242815448));
#172391=CARTESIAN_POINT('Ctrl Pts',(3.21581968476767,7.46230332718995,88.7873030667635));
#172392=CARTESIAN_POINT('Ctrl Pts',(3.33596618740773,7.4089734499219,88.7821878542553));
#172393=CARTESIAN_POINT('Ctrl Pts',(3.37535461144747,7.39111217709105,88.7805023492889));
#172394=CARTESIAN_POINT('Ctrl Pts',(3.44423749853242,7.35921072591055,88.7775390640543));
#172395=CARTESIAN_POINT('Ctrl Pts',(3.47379343707519,7.34530554866485,88.7762624865879));
#172396=CARTESIAN_POINT('Ctrl Pts',(3.50398791523402,7.33087695265173,88.7749529617756));
#172397=CARTESIAN_POINT('Ctrl Pts',(3.50471110853462,7.3305312393264,88.7749215939515));
#172398=CARTESIAN_POINT('Ctrl Pts',(3.50610889220126,7.32986279256006,88.7748609602919));
#172399=CARTESIAN_POINT('Ctrl Pts',(3.50678348920247,7.32954007299134,88.774831694579));
#172400=CARTESIAN_POINT('Ctrl Pts',(3.50808734786371,7.32891610055553,88.7747751245863));
#172401=CARTESIAN_POINT('Ctrl Pts',(3.50871661530199,7.32861485976219,88.7747478204134));
#172402=CARTESIAN_POINT('Ctrl Pts',(3.50993287252752,7.32803242463337,88.7746950418725));
#172403=CARTESIAN_POINT('Ctrl Pts',(3.51051986735411,7.32775124079955,88.7746695675972));
#172404=CARTESIAN_POINT('Ctrl Pts',(3.51165443745904,7.32720758837244,88.7746203257272));
#172405=CARTESIAN_POINT('Ctrl Pts',(3.51220201709886,7.32694512892754,88.7745965582142));
#172406=CARTESIAN_POINT('Ctrl Pts',(3.51326042580475,7.32643767897748,88.7745506148163));
#172407=CARTESIAN_POINT('Ctrl Pts',(3.51377125869094,7.32619269641907,88.7745284390013));
#172408=CARTESIAN_POINT('Ctrl Pts',(3.51475866454932,7.32571903446287,88.7744855715675));
#172409=CARTESIAN_POINT('Ctrl Pts',(3.51523524084668,7.32549036197752,88.7744648800096));
#172410=CARTESIAN_POINT('Ctrl Pts',(3.51615645644207,7.32504823052992,88.7744248808368));
#172411=CARTESIAN_POINT('Ctrl Pts',(3.51660109862707,7.32483477758398,88.7744055732752));
#172412=CARTESIAN_POINT('Ctrl Pts',(3.51746061155895,7.32442206733422,88.7743682485835));
#172413=CARTESIAN_POINT('Ctrl Pts',(3.51787548479433,7.32422281527564,88.7743502315009));
#172414=CARTESIAN_POINT('Ctrl Pts',(3.51867747786589,7.32383755648087,88.7743154005835));
#172415=CARTESIAN_POINT('Ctrl Pts',(3.51906459991257,7.32365155428646,88.7742985867879));
#172416=CARTESIAN_POINT('Ctrl Pts',(3.51981297099499,7.32329190817685,88.7742660811703));
#172417=CARTESIAN_POINT('Ctrl Pts',(3.52017422191131,7.3231182682341,88.7742503893843));
#172418=CARTESIAN_POINT('Ctrl Pts',(3.52087260222681,7.32278251905136,88.7742200520507));
#172419=CARTESIAN_POINT('Ctrl Pts',(3.52120973332843,7.32262041323657,88.7742054065316));
#172420=CARTESIAN_POINT('Ctrl Pts',(3.52186150570261,7.32230696017691,88.7741770911489));
#172421=CARTESIAN_POINT('Ctrl Pts',(3.52217614837717,7.32215561595136,88.7741634213137));
#172422=CARTESIAN_POINT('Ctrl Pts',(3.52278446350025,7.32186296596925,88.77413699154));
#172423=CARTESIAN_POINT('Ctrl Pts',(3.52307813720634,7.32172166282285,88.7741242316248));
#172424=CARTESIAN_POINT('Ctrl Pts',(3.52364592975664,7.32144842341717,88.7740995604223));
#172425=CARTESIAN_POINT('Ctrl Pts',(3.52392004971366,7.32131648942145,88.7740876491544));
#172426=CARTESIAN_POINT('Ctrl Pts',(3.52445005317281,7.32106136197773,88.7740646181565));
#172427=CARTESIAN_POINT('Ctrl Pts',(3.52470593760193,7.32093817052067,88.7740534984452));
#172428=CARTESIAN_POINT('Ctrl Pts',(3.52520069786971,7.32069994416747,88.7740319973751));
#172429=CARTESIAN_POINT('Ctrl Pts',(3.52543957456747,7.32058491098002,88.7740216160303));
#172430=CARTESIAN_POINT('Ctrl Pts',(3.52590146341588,7.32036245646727,88.7740015421248));
#172431=CARTESIAN_POINT('Ctrl Pts',(3.52612447622289,7.32025503667431,88.7739918495802));
#172432=CARTESIAN_POINT('Ctrl Pts',(3.5267231487737,7.31996663710141,88.7739658293606));
#172433=CARTESIAN_POINT('Ctrl Pts',(3.52709879953588,7.31978563857414,88.7739495015177));
#172434=CARTESIAN_POINT('Ctrl Pts',(3.5278447240471,7.31942616155599,88.7739170778351));
#172435=CARTESIAN_POINT('Ctrl Pts',(3.52821500372824,7.31924768121248,88.7739009817619));
#172436=CARTESIAN_POINT('Ctrl Pts',(3.52895030846885,7.31889318456538,88.7738690163697));
#172437=CARTESIAN_POINT('Ctrl Pts',(3.52931532831221,7.31871717174947,88.7738531473013));
#172438=CARTESIAN_POINT('Ctrl Pts',(3.53004020960219,7.31836756665899,88.7738216318054));
#172439=CARTESIAN_POINT('Ctrl Pts',(3.5304000713832,7.318193975163,88.7738059853862));
#172440=CARTESIAN_POINT('Ctrl Pts',(3.53111473785338,7.31784916664837,88.7737749108517));
#172441=CARTESIAN_POINT('Ctrl Pts',(3.53146954290853,7.31767795036179,88.7737594827425));
#172442=CARTESIAN_POINT('Ctrl Pts',(3.5668227225724,7.30061459459707,88.7722221316159));
#172443=CARTESIAN_POINT('Ctrl Pts',(3.60169938983743,7.283471650579,88.7706980015291));
#172444=CARTESIAN_POINT('Ctrl Pts',(3.71112519627361,7.22870736249288,88.7658918703864));
#172445=CARTESIAN_POINT('Ctrl Pts',(3.78521782309246,7.19018680259269,88.7626020019635));
#172446=CARTESIAN_POINT('Ctrl Pts',(3.95743783503906,7.09725022401292,88.7548691933391));
#172447=CARTESIAN_POINT('Ctrl Pts',(4.05505775975313,7.04193022237695,88.7504191709854));
#172448=CARTESIAN_POINT('Ctrl Pts',(4.30808479402424,6.89153638821055,88.7387100668404));
#172449=CARTESIAN_POINT('Ctrl Pts',(4.4614946859479,6.7932269962844,88.7314319650879));
#172450=CARTESIAN_POINT('Ctrl Pts',(4.63451451329279,6.67396030726475,88.7230376628884));
#172451=CARTESIAN_POINT('Ctrl Pts',(4.6574769082477,6.65795612834693,88.7219197597267));
#172452=CARTESIAN_POINT('Ctrl Pts',(4.83115343290541,6.53557004669835,88.7134360740931));
#172453=CARTESIAN_POINT('Ctrl Pts',(4.97828937697914,6.42420075580505,88.7060839895282));
#172454=CARTESIAN_POINT('Ctrl Pts',(5.1477992327665,6.2865727969523,88.697469812716));
#172455=CARTESIAN_POINT('Ctrl Pts',(5.17395702526198,6.26506210569217,88.6961363628367));
#172456=CARTESIAN_POINT('Ctrl Pts',(5.21408643206903,6.23163921347777,88.6940847981277));
#172457=CARTESIAN_POINT('Ctrl Pts',(5.22815331613201,6.21984224174736,88.6933645398367));
#172458=CARTESIAN_POINT('Ctrl Pts',(5.25641634197733,6.19597627373232,88.6919150691661));
#172459=CARTESIAN_POINT('Ctrl Pts',(5.27061116083888,6.18390594516789,88.691185882192));
#172460=CARTESIAN_POINT('Ctrl Pts',(5.3043333703737,6.15503036428025,88.6894505134672));
#172461=CARTESIAN_POINT('Ctrl Pts',(5.32382262114243,6.13818083752522,88.6884451195529));
#172462=CARTESIAN_POINT('Ctrl Pts',(5.38857805724869,6.08165579572339,88.6850956615029));
#172463=CARTESIAN_POINT('Ctrl Pts',(5.43348362870176,6.04156986390969,88.6827582811085));
#172464=CARTESIAN_POINT('Ctrl Pts',(5.54379938578207,5.94086927430945,88.6769734639496));
#172465=CARTESIAN_POINT('Ctrl Pts',(5.60866511508464,5.87966964567739,88.6735337463379));
#172466=CARTESIAN_POINT('Ctrl Pts',(5.91256680548846,5.58333773235736,88.6571982699304));
#172467=CARTESIAN_POINT('Ctrl Pts',(6.13790438452492,5.33462626158836,88.6444094449906));
#172468=CARTESIAN_POINT('Ctrl Pts',(6.48402356277164,4.90154409291292,88.6230786880931));
#172469=CARTESIAN_POINT('Ctrl Pts',(6.61383529685443,4.72492086223655,88.6146125841701));
#172470=CARTESIAN_POINT('Ctrl Pts',(6.77430694368877,4.48698800709822,88.6034455967781));
#172471=CARTESIAN_POINT('Ctrl Pts',(6.81155823579529,4.43023366088691,88.6007991147627));
#172472=CARTESIAN_POINT('Ctrl Pts',(6.87520499438304,4.33056362971405,88.5961799833609));
#172473=CARTESIAN_POINT('Ctrl Pts',(6.90192068751406,4.28785679194547,88.5942097192014));
#172474=CARTESIAN_POINT('Ctrl Pts',(6.9556547748926,4.2001557546557,88.5901815024958));
#172475=CARTESIAN_POINT('Ctrl Pts',(6.98263784749714,4.15514264255737,88.5881234222509));
#172476=CARTESIAN_POINT('Ctrl Pts',(7.03915699892522,4.05875201792674,88.5837360663347));
#172477=CARTESIAN_POINT('Ctrl Pts',(7.06857091480966,4.00730637640782,88.5814062291663));
#172478=CARTESIAN_POINT('Ctrl Pts',(7.11106552853481,3.93105842705016,88.5779705028089));
#172479=CARTESIAN_POINT('Ctrl Pts',(7.12458487840021,3.90650273469349,88.5768666460595));
#172480=CARTESIAN_POINT('Ctrl Pts',(7.17413269186415,3.81539446600728,88.5727807837816));
#172481=CARTESIAN_POINT('Ctrl Pts',(7.20935785455462,3.74840954342111,88.5697958734544));
#172482=CARTESIAN_POINT('Ctrl Pts',(7.33647824020812,3.49825225653681,88.5587216815198));
#172483=CARTESIAN_POINT('Ctrl Pts',(7.42236997097542,3.31211505759345,88.5506232726255));
#172484=CARTESIAN_POINT('Ctrl Pts',(7.51408843924093,3.09181155545818,88.5412369821999));
#172485=CARTESIAN_POINT('Ctrl Pts',(7.52685018019015,3.06061270648176,88.5399123114768));
#172486=CARTESIAN_POINT('Ctrl Pts',(7.5530628704052,2.9953744962503,88.5371523402626));
#172487=CARTESIAN_POINT('Ctrl Pts',(7.5664786859088,2.96132190103057,88.5357174445022));
#172488=CARTESIAN_POINT('Ctrl Pts',(7.59422610417411,2.88947249994869,88.5327014995566));
#172489=CARTESIAN_POINT('Ctrl Pts',(7.60850663693776,2.85165710006786,88.5311207752705));
#172490=CARTESIAN_POINT('Ctrl Pts',(7.64483038215455,2.75325488886063,88.5270228213042));
#172491=CARTESIAN_POINT('Ctrl Pts',(7.6664357465347,2.69250942985338,88.5245080898386));
#172492=CARTESIAN_POINT('Ctrl Pts',(7.74483358703632,2.46348949941982,88.5150736395329));
#172493=CARTESIAN_POINT('Ctrl Pts',(7.7968269997611,2.2936252049468,88.5081687161023));
#172494=CARTESIAN_POINT('Ctrl Pts',(7.87061194258034,2.02093053441564,88.4971578010027));
#172495=CARTESIAN_POINT('Ctrl Pts',(7.89604774694241,1.91914627884673,88.4930642662152));
#172496=CARTESIAN_POINT('Ctrl Pts',(7.93133437247057,1.76533876374054,88.4868922301827));
#172497=CARTESIAN_POINT('Ctrl Pts',(7.94265939674813,1.71366495137517,88.4848209888653));
#172498=CARTESIAN_POINT('Ctrl Pts',(7.96396641593782,1.6116933966234,88.4807367955979));
#172499=CARTESIAN_POINT('Ctrl Pts',(7.973978487304,1.56140441337418,88.4787240989503));
#172500=CARTESIAN_POINT('Ctrl Pts',(7.99338702442752,1.45885917842703,88.4746218237507));
#172501=CARTESIAN_POINT('Ctrl Pts',(8.00274864987357,1.40659882234479,88.4725321458228));
#172502=CARTESIAN_POINT('Ctrl Pts',(8.02348828981748,1.28390539588085,88.467627176302));
#172503=CARTESIAN_POINT('Ctrl Pts',(8.03445213608582,1.21340686246497,88.4648096100065));
#172504=CARTESIAN_POINT('Ctrl Pts',(8.09819219755517,0.764712417395979,
88.4468758723622));
#172505=CARTESIAN_POINT('Ctrl Pts',(8.12517874796852,0.383346495983037,
88.4316036140856));
#172506=CARTESIAN_POINT('Ctrl Pts',(8.12524985909245,0.00151321447761893,
88.4163208663708));
#172507=CARTESIAN_POINT('',(8.12631724021387,0.00268884911775716,84.4167025567875));
#172508=CARTESIAN_POINT('Ctrl Pts',(8.12524985911998,0.00151306666855575,
88.4163208604548));
#172509=CARTESIAN_POINT('Ctrl Pts',(8.12528447581569,-0.184380461877274,
88.4088805349657));
#172510=CARTESIAN_POINT('Ctrl Pts',(8.11893963366032,-0.370222552557259,
88.4014489082081));
#172511=CARTESIAN_POINT('Ctrl Pts',(8.10137240488833,-0.62648991633224,
88.3912508305079));
#172512=CARTESIAN_POINT('Ctrl Pts',(8.0955911985821,-0.697228592091197,
88.3884412278708));
#172513=CARTESIAN_POINT('Ctrl Pts',(8.08645389199681,-0.793481059717428,
88.3846286508366));
#172514=CARTESIAN_POINT('Ctrl Pts',(8.08390232606959,-0.819067719003989,
88.3836161632892));
#172515=CARTESIAN_POINT('Ctrl Pts',(8.07919089809966,-0.864144964454268,
88.3818343871552));
#172516=CARTESIAN_POINT('Ctrl Pts',(8.07708185707336,-0.88364063095439,
88.3810644295474));
#172517=CARTESIAN_POINT('Ctrl Pts',(8.07275417006443,-0.922334625505273,
88.3795376542191));
#172518=CARTESIAN_POINT('Ctrl Pts',(8.07053756305378,-0.94153305737122,
88.378780812204));
#172519=CARTESIAN_POINT('Ctrl Pts',(8.06563264578545,-0.982725048093576,
88.3771585169738));
#172520=CARTESIAN_POINT('Ctrl Pts',(8.0629228358995,-1.00471580217326,88.3762934389335));
#172521=CARTESIAN_POINT('Ctrl Pts',(8.0544373054714,-1.07133188350332,88.3736757208578));
#172522=CARTESIAN_POINT('Ctrl Pts',(8.04838079891667,-1.11592063498418,
88.3719273377086));
#172523=CARTESIAN_POINT('Ctrl Pts',(8.03093910895339,-1.23679135802114,
88.3671944774183));
#172524=CARTESIAN_POINT('Ctrl Pts',(8.01883767034917,-1.31296549146983,
88.3642189371654));
#172525=CARTESIAN_POINT('Ctrl Pts',(7.96641459473931,-1.61512116312082,
88.352419925684));
#172526=CARTESIAN_POINT('Ctrl Pts',(7.91760916830698,-1.83952275062591,
88.3436623035118));
#172527=CARTESIAN_POINT('Ctrl Pts',(7.81026647807734,-2.24875015665204,
88.3274570707364));
#172528=CARTESIAN_POINT('Ctrl Pts',(7.7544930375797,-2.43412744671116,88.3200254854521));
#172529=CARTESIAN_POINT('Ctrl Pts',(7.6677520194328,-2.68905289181744,88.309606750686));
#172530=CARTESIAN_POINT('Ctrl Pts',(7.64234763733064,-2.76042550688426,
88.3066678798717));
#172531=CARTESIAN_POINT('Ctrl Pts',(7.61454795398322,-2.83520073088127,
88.3035636766145));
#172532=CARTESIAN_POINT('Ctrl Pts',(7.61314407820166,-2.83896829366363,
88.3034072031183));
#172533=CARTESIAN_POINT('Ctrl Pts',(7.61041160073841,-2.84628480480384,
88.3031032036105));
#172534=CARTESIAN_POINT('Ctrl Pts',(7.60908331156872,-2.8498338688956,88.3029556803782));
#172535=CARTESIAN_POINT('Ctrl Pts',(7.60648038184221,-2.85677385983538,
88.3026670886896));
#172536=CARTESIAN_POINT('Ctrl Pts',(7.60520595540433,-2.86016486613274,
88.3025260221496));
#172537=CARTESIAN_POINT('Ctrl Pts',(7.59231493296727,-2.89439589089042,
88.3011014437266));
#172538=CARTESIAN_POINT('Ctrl Pts',(7.58051310331934,-2.92516575537113,
88.2998163062399));
#172539=CARTESIAN_POINT('Ctrl Pts',(7.55674124862312,-2.98603389052831,
88.2972647101583));
#172540=CARTESIAN_POINT('Ctrl Pts',(7.54477778803705,-3.01613408438214,
88.2959983320068));
#172541=CARTESIAN_POINT('Ctrl Pts',(7.51662627282288,-3.08574794222829,
88.2930586963622));
#172542=CARTESIAN_POINT('Ctrl Pts',(7.50030609389936,-3.12520709193206,
88.2913842812909));
#172543=CARTESIAN_POINT('Ctrl Pts',(7.4505167497896,-3.24295179237185,88.2863630038643));
#172544=CARTESIAN_POINT('Ctrl Pts',(7.41612754282025,-3.32084150422497,
88.2830081444316));
#172545=CARTESIAN_POINT('Ctrl Pts',(7.24090391329714,-3.70141085691617,
88.2664501396477));
#172546=CARTESIAN_POINT('Ctrl Pts',(7.08273252838164,-3.99575114803389,
88.2531017579556));
#172547=CARTESIAN_POINT('Ctrl Pts',(6.86541905644188,-4.34648293916053,
88.2366739868948));
#172548=CARTESIAN_POINT('Ctrl Pts',(6.822957997981,-4.41283775025868,88.2335427076409));
#172549=CARTESIAN_POINT('Ctrl Pts',(6.75869344365595,-4.51011981396591,
88.2289227110258));
#172550=CARTESIAN_POINT('Ctrl Pts',(6.7376281136403,-4.54152895175203,88.22742647844));
#172551=CARTESIAN_POINT('Ctrl Pts',(6.69920652735525,-4.59796115204567,
88.224730759666));
#172552=CARTESIAN_POINT('Ctrl Pts',(6.68192742730242,-4.6230358767899,88.22353026769));
#172553=CARTESIAN_POINT('Ctrl Pts',(6.65343084461098,-4.66389542220327,
88.2215700639692));
#172554=CARTESIAN_POINT('Ctrl Pts',(6.64229719596458,-4.67973829147026,
88.2208090256917));
#172555=CARTESIAN_POINT('Ctrl Pts',(6.62037545996508,-4.71069646425686,
88.2193200960542));
#172556=CARTESIAN_POINT('Ctrl Pts',(6.60959197668369,-4.72581488373092,
88.218592136008));
#172557=CARTESIAN_POINT('Ctrl Pts',(6.58528076709651,-4.75965315996799,
88.2169610050705));
#172558=CARTESIAN_POINT('Ctrl Pts',(6.57172487491795,-4.77835255692863,
88.2160583519331));
#172559=CARTESIAN_POINT('Ctrl Pts',(6.52111528509512,-4.84754218246362,
88.2127132548391));
#172560=CARTESIAN_POINT('Ctrl Pts',(6.48355776017713,-4.89766154760364,
88.2102798247592));
#172561=CARTESIAN_POINT('Ctrl Pts',(6.18272568158983,-5.28958723497865,
88.1911497358633));
#172562=CARTESIAN_POINT('Ctrl Pts',(5.89318036540369,-5.61037140955645,
88.1748614639105));
#172563=CARTESIAN_POINT('Ctrl Pts',(5.31313419406721,-6.15829413014251,
88.144542863829));
#172564=CARTESIAN_POINT('Ctrl Pts',(5.03001957651112,-6.39162564790143,
88.1305776398499));
#172565=CARTESIAN_POINT('Ctrl Pts',(4.63853251183464,-6.67210314853453,
88.1119587984729));
#172566=CARTESIAN_POINT('Ctrl Pts',(4.5435223395634,-6.73716177097599,88.1074908367172));
#172567=CARTESIAN_POINT('Ctrl Pts',(4.41341368549829,-6.82224987081573,
88.1014336247855));
#172568=CARTESIAN_POINT('Ctrl Pts',(4.3795012398182,-6.84406915045713,88.0998603356867));
#172569=CARTESIAN_POINT('Ctrl Pts',(4.31591904075648,-6.88431187485521,
88.0969205418535));
#172570=CARTESIAN_POINT('Ctrl Pts',(4.28629018254488,-6.90279824557435,
88.0955546011133));
#172571=CARTESIAN_POINT('Ctrl Pts',(4.22430353780119,-6.9409206673375,88.0927050125827));
#172572=CARTESIAN_POINT('Ctrl Pts',(4.19192586941449,-6.96052279534235,
88.0912211266817));
#172573=CARTESIAN_POINT('Ctrl Pts',(4.11734970791505,-7.00496370545357,
88.087813461613));
#172574=CARTESIAN_POINT('Ctrl Pts',(4.07506130856448,-7.02964867127109,
88.0858885559673));
#172575=CARTESIAN_POINT('Ctrl Pts',(3.93672385041905,-7.1087324572576,88.0796152038327));
#172576=CARTESIAN_POINT('Ctrl Pts',(3.83978928832454,-7.16155638286208,
88.0752559189152));
#172577=CARTESIAN_POINT('Ctrl Pts',(3.37623285978628,-7.40205086205548,
88.0545774866923));
#172578=CARTESIAN_POINT('Ctrl Pts',(2.99677522813437,-7.56363878466678,
88.0381917320845));
#172579=CARTESIAN_POINT('Ctrl Pts',(2.08950818220156,-7.87094868987318,
87.9990458084862));
#172580=CARTESIAN_POINT('Ctrl Pts',(1.55597895186274,-7.9935442207752,87.9759363142304));
#172581=CARTESIAN_POINT('Ctrl Pts',(0.753988148230762,-8.09444190084231,
87.9417653838544));
#172582=CARTESIAN_POINT('Ctrl Pts',(0.492301924895051,-8.11456303479836,
87.9307336702937));
#172583=CARTESIAN_POINT('Ctrl Pts',(0.159308648476984,-8.12399675391221,
87.9171170330251));
#172584=CARTESIAN_POINT('Ctrl Pts',(0.0884964804720896,-8.12507668767316,
87.9142460748373));
#172585=CARTESIAN_POINT('Ctrl Pts',(-0.0108220171985221,-8.12529277722797,
87.9102615073279));
#172586=CARTESIAN_POINT('Ctrl Pts',(-0.0393226227081642,-8.12520483348696,
87.9091229593181));
#172587=CARTESIAN_POINT('Ctrl Pts',(-0.0825631533069317,-8.1248438873621,
87.9074035307122));
#172588=CARTESIAN_POINT('Ctrl Pts',(-0.0973036308914327,-8.12468072450121,
87.9068187887383));
#172589=CARTESIAN_POINT('Ctrl Pts',(-0.124576557891025,-8.12430460702016,
87.9057395877783));
#172590=CARTESIAN_POINT('Ctrl Pts',(-0.137109103134268,-8.12410276660817,
87.9052447218524));
#172591=CARTESIAN_POINT('Ctrl Pts',(-0.157492127605489,-8.12372731267102,
87.9044416327644));
#172592=CARTESIAN_POINT('Ctrl Pts',(-0.165342885362507,-8.12357131757308,
87.9041327395081));
#172593=CARTESIAN_POINT('Ctrl Pts',(-0.180424035645863,-8.12324978290116,
87.9035401953196));
#172594=CARTESIAN_POINT('Ctrl Pts',(-0.187654455465305,-8.12308596986496,
87.9032564774846));
#172595=CARTESIAN_POINT('Ctrl Pts',(-0.204164687799632,-8.12268985688925,
87.9026094800409));
#172596=CARTESIAN_POINT('Ctrl Pts',(-0.213444350695921,-8.12245130739726,
87.902246448785));
#172597=CARTESIAN_POINT('Ctrl Pts',(-0.242455918230452,-8.12165576388315,
87.9011134543929));
#172598=CARTESIAN_POINT('Ctrl Pts',(-0.262186308296341,-8.12104276360221,
87.9003457718306));
#172599=CARTESIAN_POINT('Ctrl Pts',(-0.4663327495355,-8.11395541364044,
87.8924336080277));
#172600=CARTESIAN_POINT('Ctrl Pts',(-0.650473740009095,-8.10127285133589,
87.8855854813605));
#172601=CARTESIAN_POINT('Ctrl Pts',(-0.981905472975947,-8.06707197764009,
87.8736124146225));
#172602=CARTESIAN_POINT('Ctrl Pts',(-1.12934197330756,-8.04775606740036,
87.8684091826339));
#172603=CARTESIAN_POINT('Ctrl Pts',(-1.51538556838731,-7.9863612509755,
87.8549550712973));
#172604=CARTESIAN_POINT('Ctrl Pts',(-1.75278604354459,-7.93763850759876,
87.8468517395734));
#172605=CARTESIAN_POINT('Ctrl Pts',(-2.46971699960628,-7.7567620349263,
87.8221847020955));
#172606=CARTESIAN_POINT('Ctrl Pts',(-2.9395878944736,-7.5911567052562,87.8056869946392));
#172607=CARTESIAN_POINT('Ctrl Pts',(-3.62751949168764,-7.27518588080589,
87.7787290180603));
#172608=CARTESIAN_POINT('Ctrl Pts',(-3.85833001239837,-7.15545275119635,
87.7691745270075));
#172609=CARTESIAN_POINT('Ctrl Pts',(-4.12439682990733,-7.00080932712546,
87.7574101538642));
#172610=CARTESIAN_POINT('Ctrl Pts',(-4.1655821419195,-6.9763819972725,87.7555672160709));
#172611=CARTESIAN_POINT('Ctrl Pts',(-4.22018889365918,-6.94333835025208,
87.7530938174788));
#172612=CARTESIAN_POINT('Ctrl Pts',(-4.23380469234144,-6.93504430900724,
87.7524745953414));
#172613=CARTESIAN_POINT('Ctrl Pts',(-4.25619815055805,-6.92131284343997,
87.7514520362682));
#172614=CARTESIAN_POINT('Ctrl Pts',(-4.2649900393122,-6.91589865000957,
87.7510495126774));
#172615=CARTESIAN_POINT('Ctrl Pts',(-4.28206281600574,-6.90534000905084,
87.7502657971696));
#172616=CARTESIAN_POINT('Ctrl Pts',(-4.29034481465529,-6.90019738640717,
87.7498846696228));
#172617=CARTESIAN_POINT('Ctrl Pts',(-4.30952745063559,-6.88823823656429,
87.7489997026657));
#172618=CARTESIAN_POINT('Ctrl Pts',(-4.32042119129411,-6.88141072596528,
87.7484954776047));
#172619=CARTESIAN_POINT('Ctrl Pts',(-4.35559398299998,-6.85925019165701,
87.7468620978338));
#172620=CARTESIAN_POINT('Ctrl Pts',(-4.37980784313725,-6.84381438768918,
87.7457293228081));
#172621=CARTESIAN_POINT('Ctrl Pts',(-4.61439917920111,-6.69251267963224,
87.7346730375954));
#172622=CARTESIAN_POINT('Ctrl Pts',(-4.81845774330545,-6.54712587155294,
87.7244093458401));
#172623=CARTESIAN_POINT('Ctrl Pts',(-5.333944482254,-6.14268562565857,87.6967460085545));
#172624=CARTESIAN_POINT('Ctrl Pts',(-5.633281277977,-5.86938241784143,87.6788646403132));
#172625=CARTESIAN_POINT('Ctrl Pts',(-6.15798513720825,-5.31304978471058,
87.644595317736));
#172626=CARTESIAN_POINT('Ctrl Pts',(-6.38730718404794,-5.03503649405329,
87.6283082819637));
#172627=CARTESIAN_POINT('Ctrl Pts',(-6.68079648639094,-4.6267742818475,
87.6062415808004));
#172628=CARTESIAN_POINT('Ctrl Pts',(-6.76108564918213,-4.50863675571175,
87.6000569355226));
#172629=CARTESIAN_POINT('Ctrl Pts',(-6.91721355842457,-4.2653528070661,
87.5878031219735));
#172630=CARTESIAN_POINT('Ctrl Pts',(-6.99287346818967,-4.14014571705009,
87.5817458760562));
#172631=CARTESIAN_POINT('Ctrl Pts',(-7.07538410874687,-3.9948791197118,
87.5750390533899));
#172632=CARTESIAN_POINT('Ctrl Pts',(-7.08557891277828,-3.97676890823265,
87.574208224111));
#172633=CARTESIAN_POINT('Ctrl Pts',(-7.10390022212183,-3.94392852385006,
87.5727108834586));
#172634=CARTESIAN_POINT('Ctrl Pts',(-7.1120506536081,-3.92921188959852,
87.5720432299049));
#172635=CARTESIAN_POINT('Ctrl Pts',(-7.12454665448998,-3.90648251160985,
87.571017063655));
#172636=CARTESIAN_POINT('Ctrl Pts',(-7.12892451490402,-3.8984876435866,
87.5706570693742));
#172637=CARTESIAN_POINT('Ctrl Pts',(-7.13687395894839,-3.88391216642691,
87.5700024662749));
#172638=CARTESIAN_POINT('Ctrl Pts',(-7.14044991373662,-3.87733396193181,
87.5697076614465));
#172639=CARTESIAN_POINT('Ctrl Pts',(-7.14761522799176,-3.86410936345416,
87.5691162454736));
#172640=CARTESIAN_POINT('Ctrl Pts',(-7.1512044218469,-3.85746288868348,
87.5688196417732));
#172641=CARTESIAN_POINT('Ctrl Pts',(-7.16137190811097,-3.83857176057073,
87.5679783834972));
#172642=CARTESIAN_POINT('Ctrl Pts',(-7.1679280735745,-3.82631518595839,
87.567434685506));
#172643=CARTESIAN_POINT('Ctrl Pts',(-7.19559384162369,-3.77427413429594,
87.5651348795675));
#172644=CARTESIAN_POINT('Ctrl Pts',(-7.21640413383259,-3.7343309230171,
87.5633912604));
#172645=CARTESIAN_POINT('Ctrl Pts',(-7.27419703675982,-3.62111600748921,
87.5585048477743));
#172646=CARTESIAN_POINT('Ctrl Pts',(-7.31040353164279,-3.54745321748207,
87.5553907482796));
#172647=CARTESIAN_POINT('Ctrl Pts',(-7.54553599649802,-3.05017801127673,
87.5347344655956));
#172648=CARTESIAN_POINT('Ctrl Pts',(-7.70866698695404,-2.61059232671126,
87.5181805695881));
#172649=CARTESIAN_POINT('Ctrl Pts',(-7.96132435096491,-1.6940953109874,
87.4839734067664));
#172650=CARTESIAN_POINT('Ctrl Pts',(-8.04787676111599,-1.21831640895912,
87.4663540323539));
#172651=CARTESIAN_POINT('Ctrl Pts',(-8.09801045833638,-0.668397125700044,
87.4453162399145));
#172652=CARTESIAN_POINT('Ctrl Pts',(-8.1034367853083,-0.599032742184795,
87.4426522405842));
#172653=CARTESIAN_POINT('Ctrl Pts',(-8.11154355113557,-0.47492309711704,
87.437866387093));
#172654=CARTESIAN_POINT('Ctrl Pts',(-8.11456217066969,-0.420204047850183,
87.4357496498337));
#172655=CARTESIAN_POINT('Ctrl Pts',(-8.11825758738527,-0.338126985132404,
87.4325645542927));
#172656=CARTESIAN_POINT('Ctrl Pts',(-8.11935011378706,-0.310789052255108,
87.4315020070198));
#172657=CARTESIAN_POINT('Ctrl Pts',(-8.1210708320833,-0.261493077130119,
87.429583033099));
#172658=CARTESIAN_POINT('Ctrl Pts',(-8.12174809533972,-0.23953697012244,
87.4287272724805));
#172659=CARTESIAN_POINT('Ctrl Pts',(-8.12288609377211,-0.197054798176525,
87.427069437358));
#172660=CARTESIAN_POINT('Ctrl Pts',(-8.1233580826719,-0.176529156950955,
87.4262675032742));
#172661=CARTESIAN_POINT('Ctrl Pts',(-8.12438458729711,-0.123074265723032,
87.424176435659));
#172662=CARTESIAN_POINT('Ctrl Pts',(-8.12481669957023,-0.0901431154560538,
87.4228856609259));
#172663=CARTESIAN_POINT('Ctrl Pts',(-8.12561654486722,0.0234513854260239,
87.4184235712268));
#172664=CARTESIAN_POINT('Ctrl Pts',(-8.12498330821539,0.10411636252658,
87.4152381952756));
#172665=CARTESIAN_POINT('Ctrl Pts',(-8.10434189934501,1.01164611159506,
87.3791804058906));
#172666=CARTESIAN_POINT('Ctrl Pts',(-7.9593797367279,1.83078500486084,87.3438494336284));
#172667=CARTESIAN_POINT('Ctrl Pts',(-7.61450601515398,2.84588988547919,
87.2987379491886));
#172668=CARTESIAN_POINT('Ctrl Pts',(-7.52517321019521,3.07434026356217,
87.2885502621338));
#172669=CARTESIAN_POINT('Ctrl Pts',(-7.40969693742471,3.33430984184497,
87.2771302332658));
#172670=CARTESIAN_POINT('Ctrl Pts',(-7.39348929929894,3.37009597299934,
87.2755622267616));
#172671=CARTESIAN_POINT('Ctrl Pts',(-7.37170526013057,3.41728109022426,
87.2735012623311));
#172672=CARTESIAN_POINT('Ctrl Pts',(-7.36636092467724,3.42878626067399,
87.2729992506694));
#172673=CARTESIAN_POINT('Ctrl Pts',(-7.35755192402838,3.44763443094345,
87.2721777318965));
#172674=CARTESIAN_POINT('Ctrl Pts',(-7.35410316837012,3.45498481527026,
87.2718575806897));
#172675=CARTESIAN_POINT('Ctrl Pts',(-7.3474054863351,3.46920422004098,87.2712386931006));
#172676=CARTESIAN_POINT('Ctrl Pts',(-7.34415793103988,3.47607387513617,
87.2709399003032));
#172677=CARTESIAN_POINT('Ctrl Pts',(-7.33664673587518,3.49190502763618,
87.2702518149167));
#172678=CARTESIAN_POINT('Ctrl Pts',(-7.33237629981278,3.50086330040163,
87.2698628107042));
#172679=CARTESIAN_POINT('Ctrl Pts',(-7.32091171877041,3.5248000336117,87.2688243801532));
#172680=CARTESIAN_POINT('Ctrl Pts',(-7.3136879979854,3.5397643345841,87.2681762420602));
#172681=CARTESIAN_POINT('Ctrl Pts',(-7.25730205859535,3.65566118042444,
87.2631651686594));
#172682=CARTESIAN_POINT('Ctrl Pts',(-7.20610225584859,3.75558027113001,
87.2589029470602));
#172683=CARTESIAN_POINT('Ctrl Pts',(-6.8271664449743,4.45879117447764,87.2292679120403));
#172684=CARTESIAN_POINT('Ctrl Pts',(-6.42617874716781,5.01950327629161,
87.2072239125608));
#172685=CARTESIAN_POINT('Ctrl Pts',(-5.61181927967381,5.89819239449311,
87.1664003312898));
#172686=CARTESIAN_POINT('Ctrl Pts',(-5.2296215962283,6.23956567214487,87.148330877711));
#172687=CARTESIAN_POINT('Ctrl Pts',(-4.78720368337276,6.565350072131,87.1272479344468));
#172688=CARTESIAN_POINT('Ctrl Pts',(-4.75634986417377,6.58773683437069,
87.1257773495951));
#172689=CARTESIAN_POINT('Ctrl Pts',(-4.7134784869283,6.61838505316805,87.1237332820002));
#172690=CARTESIAN_POINT('Ctrl Pts',(-4.70159431124777,6.62683265886101,
87.1231665832133));
#172691=CARTESIAN_POINT('Ctrl Pts',(-4.68149435894232,6.64103898425186,
87.1222079735667));
#172692=CARTESIAN_POINT('Ctrl Pts',(-4.67329051888297,6.64681457153868,
87.1218166756666));
#172693=CARTESIAN_POINT('Ctrl Pts',(-4.65703565493858,6.65821319187969,
87.1210412845406));
#172694=CARTESIAN_POINT('Ctrl Pts',(-4.64898509185847,6.66383685385207,
87.120657215079));
#172695=CARTESIAN_POINT('Ctrl Pts',(-4.631218729918,6.67619955135258,87.1198095363357));
#172696=CARTESIAN_POINT('Ctrl Pts',(-4.62149838371879,6.68293199588982,
87.119345690482));
#172697=CARTESIAN_POINT('Ctrl Pts',(-4.58749232705156,6.70637538192568,
87.1177227157795));
#172698=CARTESIAN_POINT('Ctrl Pts',(-4.56313053069679,6.7229752603836,87.1165596007791));
#172699=CARTESIAN_POINT('Ctrl Pts',(-4.30887055814659,6.89420670736918,
87.104415296259));
#172700=CARTESIAN_POINT('Ctrl Pts',(-4.07131296116644,7.03710480302124,
87.0930173496083));
#172701=CARTESIAN_POINT('Ctrl Pts',(-3.70578960600831,7.23226595116053,
87.0754084330883));
#172702=CARTESIAN_POINT('Ctrl Pts',(-3.58302771708291,7.29386439805088,
87.0694846652135));
#172703=CARTESIAN_POINT('Ctrl Pts',(-2.91549520809578,7.60789303890565,
87.0372728768638));
#172704=CARTESIAN_POINT('Ctrl Pts',(-2.34561249453569,7.80244731666633,
87.0096243291723));
#172705=CARTESIAN_POINT('Ctrl Pts',(-1.4305582352837,8.00541922578056,86.9681547749409));
#172706=CARTESIAN_POINT('Ctrl Pts',(-1.09731273390021,8.05786659227831,
86.9536741406324));
#172707=CARTESIAN_POINT('Ctrl Pts',(-0.738091941583653,8.09169148187367,
86.9392734399311));
#172708=CARTESIAN_POINT('Ctrl Pts',(-0.714455023279688,8.09381274733787,
86.9383309529761));
#172709=CARTESIAN_POINT('Ctrl Pts',(-0.680727218248399,8.0966907066209,
86.9369929422362));
#172710=CARTESIAN_POINT('Ctrl Pts',(-0.670643833424958,8.09753214222121,
86.9365937966184));
#172711=CARTESIAN_POINT('Ctrl Pts',(-0.653239223852168,8.09895178480713,
86.9359063079696));
#172712=CARTESIAN_POINT('Ctrl Pts',(-0.645918753371324,8.09953890420626,
86.9356175933954));
#172713=CARTESIAN_POINT('Ctrl Pts',(-0.631905803922312,8.10064365802685,
86.9350657704985));
#172714=CARTESIAN_POINT('Ctrl Pts',(-0.625213463284364,8.10116292547065,
86.9348025955091));
#172715=CARTESIAN_POINT('Ctrl Pts',(-0.609541214801772,8.10235941976177,
86.934187129163));
#172716=CARTESIAN_POINT('Ctrl Pts',(-0.600560798205658,8.10303001278166,
86.9338351053358));
#172717=CARTESIAN_POINT('Ctrl Pts',(-0.569493241817417,8.10529798353278,
86.93261947011));
#172718=CARTESIAN_POINT('Ctrl Pts',(-0.547400586532317,8.10682000318818,
86.931758828203));
#172719=CARTESIAN_POINT('Ctrl Pts',(-0.21064655863232,8.12863697703152,
86.9186948687164));
#172720=CARTESIAN_POINT('Ctrl Pts',(0.104948463570433,8.13068996839038,
86.9071650388371));
#172721=CARTESIAN_POINT('Ctrl Pts',(0.825560737317496,8.09340203035556,
86.8811369963684));
#172722=CARTESIAN_POINT('Ctrl Pts',(1.22909681658394,8.04201669537234,86.8667543410258));
#172723=CARTESIAN_POINT('Ctrl Pts',(2.2078677524544,7.84196338932469,86.8304435540159));
#172724=CARTESIAN_POINT('Ctrl Pts',(2.77387208118999,7.66006708806928,86.808082885811));
#172725=CARTESIAN_POINT('Ctrl Pts',(3.41806625228943,7.37219453093453,86.7808157477438));
#172726=CARTESIAN_POINT('Ctrl Pts',(3.52015129714024,7.32399915659644,86.7764378925807));
#172727=CARTESIAN_POINT('Ctrl Pts',(3.66587462282651,7.25145099127642,86.7700964709371));
#172728=CARTESIAN_POINT('Ctrl Pts',(3.71034480073954,7.22879794015218,86.7681486642313));
#172729=CARTESIAN_POINT('Ctrl Pts',(3.78818141483897,7.18824058675871,86.7647162861347));
#172730=CARTESIAN_POINT('Ctrl Pts',(3.82163672230387,7.17051001773245,86.7632334008194));
#172731=CARTESIAN_POINT('Ctrl Pts',(3.89127758955365,7.13297607949051,86.7601302834941));
#172732=CARTESIAN_POINT('Ctrl Pts',(3.92743873436089,7.1131296909311,86.7585096731276));
#172733=CARTESIAN_POINT('Ctrl Pts',(4.02219242284411,7.06018301646667,86.7542379811007));
#172734=CARTESIAN_POINT('Ctrl Pts',(4.08052742920507,7.02662877457023,86.7515825339732));
#172735=CARTESIAN_POINT('Ctrl Pts',(4.34092831665612,6.87250998910077,86.7396094866133));
#172736=CARTESIAN_POINT('Ctrl Pts',(4.53811366293543,6.74392864380732,86.7302136659526));
#172737=CARTESIAN_POINT('Ctrl Pts',(5.09062973698568,6.34842374825113,86.7028658904832));
#172738=CARTESIAN_POINT('Ctrl Pts',(5.43001008585655,6.06069127787336,86.6847482294732));
#172739=CARTESIAN_POINT('Ctrl Pts',(5.85951183175969,5.63137698421874,86.6601484149518));
#172740=CARTESIAN_POINT('Ctrl Pts',(5.9713621612949,5.51263282086083,86.6535676460504));
#172741=CARTESIAN_POINT('Ctrl Pts',(6.12108105277673,5.34377866444996,86.6445374320418));
#172742=CARTESIAN_POINT('Ctrl Pts',(6.16205615783314,5.29647691107933,86.6420417377251));
#172743=CARTESIAN_POINT('Ctrl Pts',(6.23241035568607,5.21333821923431,86.6377160470463));
#172744=CARTESIAN_POINT('Ctrl Pts',(6.26203684144825,5.17771463779949,86.6358815228375));
#172745=CARTESIAN_POINT('Ctrl Pts',(6.30533134974046,5.12474114096853,86.6331821487399));
#172746=CARTESIAN_POINT('Ctrl Pts',(6.31923583232925,5.1075858970073,86.6323123444997));
#172747=CARTESIAN_POINT('Ctrl Pts',(6.34468521422652,5.07592364183414,86.6307151254777));
#172748=CARTESIAN_POINT('Ctrl Pts',(6.35625069305915,5.06143343484455,86.6299872439584));
#172749=CARTESIAN_POINT('Ctrl Pts',(6.38234124170239,5.02851453442241,86.628340388655));
#172750=CARTESIAN_POINT('Ctrl Pts',(6.39683629371163,5.010062233692,86.6274220213856));
#172751=CARTESIAN_POINT('Ctrl Pts',(6.43448038961979,4.96171134376934,86.6250274851695));
#172752=CARTESIAN_POINT('Ctrl Pts',(6.45750106243129,4.93171343370384,86.6235536339798));
#172753=CARTESIAN_POINT('Ctrl Pts',(6.6311292593958,4.70216084770847,86.6123584482157));
#172754=CARTESIAN_POINT('Ctrl Pts',(6.77266536786339,4.49590908277067,86.602769009904));
#172755=CARTESIAN_POINT('Ctrl Pts',(6.9677372186389,4.18147454545883,86.5885439436141));
#172756=CARTESIAN_POINT('Ctrl Pts',(7.02873943557042,4.07810165791997,86.5839279384938));
#172757=CARTESIAN_POINT('Ctrl Pts',(7.15011457606172,3.86160336928366,86.5743533456606));
#172758=CARTESIAN_POINT('Ctrl Pts',(7.21014471652478,3.74832387014416,86.569394124825));
#172759=CARTESIAN_POINT('Ctrl Pts',(7.28947857414439,3.58965342932181,86.5624987366147));
#172760=CARTESIAN_POINT('Ctrl Pts',(7.31108719940772,3.54543559558108,86.5605825702454));
#172761=CARTESIAN_POINT('Ctrl Pts',(7.34769540266949,3.46876601569569,86.5572685190499));
#172762=CARTESIAN_POINT('Ctrl Pts',(7.36288501256494,3.43640650730609,86.5558723345331));
#172763=CARTESIAN_POINT('Ctrl Pts',(7.39178592244317,3.37376545333945,86.5531742267215));
#172764=CARTESIAN_POINT('Ctrl Pts',(7.40552591883214,3.34349791601854,86.5518725851418));
#172765=CARTESIAN_POINT('Ctrl Pts',(7.44176488909633,3.26234853958434,86.5483879927027));
#172766=CARTESIAN_POINT('Ctrl Pts',(7.46392760625363,3.21131862439481,86.5462021663001));
#172767=CARTESIAN_POINT('Ctrl Pts',(7.55328028555494,2.99965994768545,86.5371567821627));
#172768=CARTESIAN_POINT('Ctrl Pts',(7.61582209033827,2.8371210233071,86.5302584322811));
#172769=CARTESIAN_POINT('Ctrl Pts',(7.76489655973197,2.40914096803974,86.512221021849));
#172770=CARTESIAN_POINT('Ctrl Pts',(7.84305907181991,2.14102831844453,86.5010390246955));
#172771=CARTESIAN_POINT('Ctrl Pts',(7.92042105053816,1.81380396419408,86.4876537389973));
#172772=CARTESIAN_POINT('Ctrl Pts',(7.93298418599792,1.75804333997136,86.4853822118613));
#172773=CARTESIAN_POINT('Ctrl Pts',(7.95865504425514,1.6382223291081,86.4805242616879));
#172774=CARTESIAN_POINT('Ctrl Pts',(7.97158001145936,1.57412665512835,86.4779397354864));
#172775=CARTESIAN_POINT('Ctrl Pts',(7.98841825196939,1.4850918847796,86.4743725685921));
#172776=CARTESIAN_POINT('Ctrl Pts',(7.99299102015764,1.46028032819162,86.4733809705378));
#172777=CARTESIAN_POINT('Ctrl Pts',(8.0005810696049,1.41799315562026,86.4716953879883));
#172778=CARTESIAN_POINT('Ctrl Pts',(8.00365682011451,1.40052831061949,86.4710004978576));
#172779=CARTESIAN_POINT('Ctrl Pts',(8.01049901802271,1.36091794318792,86.4694271993562));
#172780=CARTESIAN_POINT('Ctrl Pts',(8.01423085739882,1.33876657207378,86.4685492826547));
#172781=CARTESIAN_POINT('Ctrl Pts',(8.0241858073605,1.27814261279842,86.4661514864202));
#172782=CARTESIAN_POINT('Ctrl Pts',(8.0302240700379,1.2396401957144,86.4646340169552));
#172783=CARTESIAN_POINT('Ctrl Pts',(8.06845771199889,0.983836285814555,
86.4545833494757));
#172784=CARTESIAN_POINT('Ctrl Pts',(8.09210663308779,0.765346948980179,
86.4461458027439));
#172785=CARTESIAN_POINT('Ctrl Pts',(8.10736665150992,0.53883900668231,86.437438955625));
#172786=CARTESIAN_POINT('Ctrl Pts',(8.10785037040559,0.531510929589214,
86.4371573140476));
#172787=CARTESIAN_POINT('Ctrl Pts',(8.11963563174538,0.349210351525483,
86.4301519705228));
#172788=CARTESIAN_POINT('Ctrl Pts',(8.12528048587411,0.173918382661803,
86.4234391042784));
#172789=CARTESIAN_POINT('Ctrl Pts',(8.1252264122484,-0.135823388346372,
86.411545053788));
#172790=CARTESIAN_POINT('Ctrl Pts',(8.121868038732,-0.270206437285089,86.406374213703));
#172791=CARTESIAN_POINT('Ctrl Pts',(8.1074111842862,-0.560283775619173,
86.3951602356333));
#172792=CARTESIAN_POINT('Ctrl Pts',(8.09515708620389,-0.715866711354673,
86.3891127780931));
#172793=CARTESIAN_POINT('Ctrl Pts',(8.07103413395062,-0.939604707821945,
86.380349225736));
#172794=CARTESIAN_POINT('Ctrl Pts',(8.06276361074699,-1.00811303921763,
86.3776568454641));
#172795=CARTESIAN_POINT('Ctrl Pts',(8.0463755951923,-1.1307158772914,86.3728212817761));
#172796=CARTESIAN_POINT('Ctrl Pts',(8.03858258780264,-1.18484959685225,
86.3706801456555));
#172797=CARTESIAN_POINT('Ctrl Pts',(8.02035646576807,-1.30298677922978,
86.3659938864546));
#172798=CARTESIAN_POINT('Ctrl Pts',(8.00970246516257,-1.36695236431319,
86.363447728529));
#172799=CARTESIAN_POINT('Ctrl Pts',(7.98532524561101,-1.50322450949963,
86.358004556188));
#172800=CARTESIAN_POINT('Ctrl Pts',(7.97138299240466,-1.57548606780182,
86.3551067844742));
#172801=CARTESIAN_POINT('Ctrl Pts',(7.92510995785551,-1.79895122795273,
86.3461112279545));
#172802=CARTESIAN_POINT('Ctrl Pts',(7.88944369389878,-1.94942849235616,
86.3400042415));
#172803=CARTESIAN_POINT('Ctrl Pts',(7.82043293381461,-2.20752902483832,
86.3294594165057));
#172804=CARTESIAN_POINT('Ctrl Pts',(7.78910373474079,-2.31564652245985,
86.3250207581936));
#172805=CARTESIAN_POINT('Ctrl Pts',(7.74231925083149,-2.46538945194183,
86.3188517928813));
#172806=CARTESIAN_POINT('Ctrl Pts',(7.72875389218584,-2.50759163788982,
86.3171108128746));
#172807=CARTESIAN_POINT('Ctrl Pts',(7.70093454236142,-2.59176764174563,
86.3136344511152));
#172808=CARTESIAN_POINT('Ctrl Pts',(7.68668105281596,-2.6337400676293,86.3118991276364));
#172809=CARTESIAN_POINT('Ctrl Pts',(7.62927066996063,-2.79836046654507,
86.3050818851993));
#172810=CARTESIAN_POINT('Ctrl Pts',(7.58351584488334,-2.92008217537805,
86.3000165198833));
#172811=CARTESIAN_POINT('Ctrl Pts',(7.45466117076445,-3.23938913376595,
86.2866084155519));
#172812=CARTESIAN_POINT('Ctrl Pts',(7.36663157529904,-3.43487320879174,
86.2782735733245));
#172813=CARTESIAN_POINT('Ctrl Pts',(7.24253407845609,-3.68367325162197,
86.2674076722357));
#172814=CARTESIAN_POINT('Ctrl Pts',(7.21342083046097,-3.74036206681567,
86.26491416792));
#172815=CARTESIAN_POINT('Ctrl Pts',(7.1580333224249,-3.84515935821158,86.2602688940297));
#172816=CARTESIAN_POINT('Ctrl Pts',(7.13193325244573,-3.893355826603,86.2581182509079));
#172817=CARTESIAN_POINT('Ctrl Pts',(7.0705427174501,-4.00403068371667,86.2531448656639));
#172818=CARTESIAN_POINT('Ctrl Pts',(7.03490830891644,-4.06631295641659,
86.2503201022861));
#172819=CARTESIAN_POINT('Ctrl Pts',(6.90569745283106,-4.28536601765933,
86.2402877708361));
#172820=CARTESIAN_POINT('Ctrl Pts',(6.80766824340771,-4.4394449330892,86.2330508131913));
#172821=CARTESIAN_POINT('Ctrl Pts',(6.52137986126716,-4.85761322935227,
86.2128717288316));
#172822=CARTESIAN_POINT('Ctrl Pts',(6.32237913536012,-5.11393405816995,
86.1998687631205));
#172823=CARTESIAN_POINT('Ctrl Pts',(6.10601226752327,-5.36062656322044,
86.186754840284));
#172824=CARTESIAN_POINT('Ctrl Pts',(6.10342260098573,-5.36357488203833,
86.1865980212806));
#172825=CARTESIAN_POINT('Ctrl Pts',(5.98322538208023,-5.50021887370896,
86.1793258881665));
#172826=CARTESIAN_POINT('Ctrl Pts',(5.86125568289897,-5.6300156862801,86.1722334135339));
#172827=CARTESIAN_POINT('Ctrl Pts',(5.70797718567077,-5.78274607151557,
86.1636936514307));
#172828=CARTESIAN_POINT('Ctrl Pts',(5.68064412432064,-5.80959878417325,
86.1621846151848));
#172829=CARTESIAN_POINT('Ctrl Pts',(5.63708801682959,-5.85178814999802,
86.1598021970486));
#172830=CARTESIAN_POINT('Ctrl Pts',(5.62099000809967,-5.86725295136704,
86.1589264190496));
#172831=CARTESIAN_POINT('Ctrl Pts',(5.59197786275281,-5.89489492610727,
86.1573567001354));
#172832=CARTESIAN_POINT('Ctrl Pts',(5.57908717754547,-5.90709648432783,
86.1566622680273));
#172833=CARTESIAN_POINT('Ctrl Pts',(5.54756602504395,-5.93673731736012,
86.1549716484984));
#172834=CARTESIAN_POINT('Ctrl Pts',(5.52889319496654,-5.95413123967668,
86.1539764793883));
#172835=CARTESIAN_POINT('Ctrl Pts',(5.46051061801756,-6.01723120837941,
86.1503542124727));
#172836=CARTESIAN_POINT('Ctrl Pts',(5.41031326679808,-6.0624053055443,86.1477375790293));
#172837=CARTESIAN_POINT('Ctrl Pts',(5.27618995971334,-6.18011412080629,
86.140845292473));
#172838=CARTESIAN_POINT('Ctrl Pts',(5.19133158447958,-6.25156522012157,
86.1365846014484));
#172839=CARTESIAN_POINT('Ctrl Pts',(4.81391007484413,-6.55637020452042,
86.117988150356));
#172840=CARTESIAN_POINT('Ctrl Pts',(4.50689161535851,-6.77108905471312,
86.1037381318701));
#172841=CARTESIAN_POINT('Ctrl Pts',(4.12867924434931,-6.9984423170726,86.086643483592));
#172842=CARTESIAN_POINT('Ctrl Pts',(4.0707624413992,-7.03228840739781,86.0840386684656));
#172843=CARTESIAN_POINT('Ctrl Pts',(3.97829232881325,-7.08480199034862,
86.0798981397679));
#172844=CARTESIAN_POINT('Ctrl Pts',(3.94401124247149,-7.10394287707296,
86.0783670773854));
#172845=CARTESIAN_POINT('Ctrl Pts',(3.8817812003564,-7.13809980264651,86.075594501455));
#172846=CARTESIAN_POINT('Ctrl Pts',(3.85388043509571,-7.15320205672022,
86.0743538466508));
#172847=CARTESIAN_POINT('Ctrl Pts',(3.78721489124895,-7.1887838328655,86.0713950207211));
#172848=CARTESIAN_POINT('Ctrl Pts',(3.74837145365251,-7.20911374951846,
86.0696754761794));
#172849=CARTESIAN_POINT('Ctrl Pts',(3.6278625697812,-7.27094852121179,86.0643539482631));
#172850=CARTESIAN_POINT('Ctrl Pts',(3.54565869093387,-7.31138724861882,
86.0607424530594));
#172851=CARTESIAN_POINT('Ctrl Pts',(3.34521615380744,-7.40581580506629,
86.0519800442096));
#172852=CARTESIAN_POINT('Ctrl Pts',(3.2263319109118,-7.45837521763892,86.0468188269849));
#172853=CARTESIAN_POINT('Ctrl Pts',(2.97358391341527,-7.56294226236704,
86.0359291557931));
#172854=CARTESIAN_POINT('Ctrl Pts',(2.83949787963817,-7.6142989575121,86.0301996092331));
#172855=CARTESIAN_POINT('Ctrl Pts',(2.55189051967794,-7.71580217994867,
86.0180386562009));
#172856=CARTESIAN_POINT('Ctrl Pts',(2.39809053954328,-7.76497977743003,
86.0116111321779));
#172857=CARTESIAN_POINT('Ctrl Pts',(2.21029082979619,-7.81891648436137,
86.0038915756531));
#172858=CARTESIAN_POINT('Ctrl Pts',(2.17759609197165,-7.82808506695261,
86.0025523640778));
#172859=CARTESIAN_POINT('Ctrl Pts',(2.1270117690769,-7.84192899302037,86.0004882089541));
#172860=CARTESIAN_POINT('Ctrl Pts',(2.1091621474017,-7.84674865379484,85.9997613347577));
#172861=CARTESIAN_POINT('Ctrl Pts',(2.07516901781517,-7.85580292827603,
85.9983800350702));
#172862=CARTESIAN_POINT('Ctrl Pts',(2.0590286071767,-7.8600488101217,85.997725446521));
#172863=CARTESIAN_POINT('Ctrl Pts',(2.01957600475349,-7.87029731376836,
85.9961286297498));
#172864=CARTESIAN_POINT('Ctrl Pts',(1.99624997003997,-7.87624613056249,
85.9951872594372));
#172865=CARTESIAN_POINT('Ctrl Pts',(1.91697601137904,-7.89608850654348,
85.9919967987102));
#172866=CARTESIAN_POINT('Ctrl Pts',(1.86090654954597,-7.90949035137273,
85.9897550790939));
#172867=CARTESIAN_POINT('Ctrl Pts',(1.72335364169449,-7.94082490809325,
85.9842872225631));
#172868=CARTESIAN_POINT('Ctrl Pts',(1.64172725737698,-7.95810151882606,
85.9810695185201));
#172869=CARTESIAN_POINT('Ctrl Pts',(1.16626473423822,-8.05110862598338,
85.9624511085643));
#172870=CARTESIAN_POINT('Ctrl Pts',(0.767516623718932,-8.09885473613727,
85.9473155089745));
#172871=CARTESIAN_POINT('Ctrl Pts',(-0.0243255284311196,-8.13464478156951,
85.9171679726225));
#172872=CARTESIAN_POINT('Ctrl Pts',(-0.41628519775045,-8.12402211317606,
85.9021982303826));
#172873=CARTESIAN_POINT('Ctrl Pts',(-0.878679879113604,-8.07792997004699,
85.8841487268657));
#172874=CARTESIAN_POINT('Ctrl Pts',(-0.951316307344746,-8.06969814394235,
85.8813024878867));
#172875=CARTESIAN_POINT('Ctrl Pts',(-1.06639268879897,-8.05508130796135,
85.8767744100433));
#172876=CARTESIAN_POINT('Ctrl Pts',(-1.10891031930456,-8.04933824189309,
85.8750973154235));
#172877=CARTESIAN_POINT('Ctrl Pts',(-1.18853382614312,-8.03794025678495,
85.8719486266537));
#172878=CARTESIAN_POINT('Ctrl Pts',(-1.22564991218905,-8.03236444080418,
85.8704776274058));
#172879=CARTESIAN_POINT('Ctrl Pts',(-1.3091006616024,-8.0192360520904,85.8671627580057));
#172880=CARTESIAN_POINT('Ctrl Pts',(-1.35541115833492,-8.01153867704218,
85.8653179592891));
#172881=CARTESIAN_POINT('Ctrl Pts',(-1.49612429180006,-7.98689541510239,
85.8596962835458));
#172882=CARTESIAN_POINT('Ctrl Pts',(-1.59029560049313,-7.96867906386644,
85.8559115665168));
#172883=CARTESIAN_POINT('Ctrl Pts',(-2.07638041669483,-7.8656916822533,
85.836256948119));
#172884=CARTESIAN_POINT('Ctrl Pts',(-2.46194108858474,-7.75366344008687,
85.8203293035835));
#172885=CARTESIAN_POINT('Ctrl Pts',(-3.37548687124406,-7.41317946604918,
85.7806309153384));
#172886=CARTESIAN_POINT('Ctrl Pts',(-3.89055101019032,-7.15630380539908,
85.7563764540706));
#172887=CARTESIAN_POINT('Ctrl Pts',(-4.68172357633412,-6.65088794788272,
85.7166807032628));
#172888=CARTESIAN_POINT('Ctrl Pts',(-4.97567064009896,-6.43393874440525,
85.7013445903703));
#172889=CARTESIAN_POINT('Ctrl Pts',(-5.27103970536602,-6.18355272960974,
85.6859401212494));
#172890=CARTESIAN_POINT('Ctrl Pts',(-5.28797527992036,-6.16907621820978,
85.6850570045303));
#172891=CARTESIAN_POINT('Ctrl Pts',(-5.31157585796183,-6.14873387661932,
85.6838267726132));
#172892=CARTESIAN_POINT('Ctrl Pts',(-5.31829103303334,-6.14292657200925,
85.6834767790813));
#172893=CARTESIAN_POINT('Ctrl Pts',(-5.33054637714349,-6.13229295368243,
85.68283814543));
#172894=CARTESIAN_POINT('Ctrl Pts',(-5.33608953875205,-6.12747011282205,
85.682549329974));
#172895=CARTESIAN_POINT('Ctrl Pts',(-5.34726691223446,-6.11771854273814,
85.681967053782));
#172896=CARTESIAN_POINT('Ctrl Pts',(-5.35290087087729,-6.11278953227413,
85.6816736080965));
#172897=CARTESIAN_POINT('Ctrl Pts',(-5.36667910877039,-6.10070163869284,
85.6809561082513));
#172898=CARTESIAN_POINT('Ctrl Pts',(-5.374815898617,-6.09353421245212,85.6805325078588));
#172899=CARTESIAN_POINT('Ctrl Pts',(-5.40403519406533,-6.06769185160452,
85.6790118720389));
#172900=CARTESIAN_POINT('Ctrl Pts',(-5.42503507490687,-6.04892347843511,
85.677919963998));
#172901=CARTESIAN_POINT('Ctrl Pts',(-5.47489136451968,-6.00389658941814,
85.6753308973395));
#172902=CARTESIAN_POINT('Ctrl Pts',(-5.50365662682912,-5.9775390879655,
85.6738399596867));
#172903=CARTESIAN_POINT('Ctrl Pts',(-5.61319006949324,-5.87571299888941,
85.6681745320842));
#172904=CARTESIAN_POINT('Ctrl Pts',(-5.6926062136657,-5.79880522090453,
85.6640894054649));
#172905=CARTESIAN_POINT('Ctrl Pts',(-5.84121773407335,-5.64889128611627,
85.6564418506644));
#172906=CARTESIAN_POINT('Ctrl Pts',(-5.91067468346907,-5.57617458559884,
85.6528662224986));
#172907=CARTESIAN_POINT('Ctrl Pts',(-6.34754356712884,-5.10146570107805,
85.6302496244705));
#172908=CARTESIAN_POINT('Ctrl Pts',(-6.6751135981627,-4.66467232727422,
85.6126351539017));
#172909=CARTESIAN_POINT('Ctrl Pts',(-7.23816480019743,-3.73172181807925,
85.5758155538352));
#172910=CARTESIAN_POINT('Ctrl Pts',(-7.47210109769261,-3.23796256591509,
85.5566669140636));
#172911=CARTESIAN_POINT('Ctrl Pts',(-7.66589678167533,-2.69347372353281,
85.5344538463291));
#172912=CARTESIAN_POINT('Ctrl Pts',(-7.67676087593777,-2.66235170291672,
85.5331809850603));
#172913=CARTESIAN_POINT('Ctrl Pts',(-7.69155799773127,-2.61911916891191,
85.5314082093794));
#172914=CARTESIAN_POINT('Ctrl Pts',(-7.69565245412017,-2.60706404928158,
85.530913387658));
#172915=CARTESIAN_POINT('Ctrl Pts',(-7.70264339510236,-2.58632097003858,
85.5300610940978));
#172916=CARTESIAN_POINT('Ctrl Pts',(-7.70555356097127,-2.57763762978768,
85.5297040534266));
#172917=CARTESIAN_POINT('Ctrl Pts',(-7.7115184227696,-2.55973932744321,
85.5289675753912));
#172918=CARTESIAN_POINT('Ctrl Pts',(-7.71457129599614,-2.55052377511001,
85.5285880814707));
#172919=CARTESIAN_POINT('Ctrl Pts',(-7.72162018552575,-2.52911721000013,
85.5277058790947));
#172920=CARTESIAN_POINT('Ctrl Pts',(-7.72560385414903,-2.51692217566856,
85.5272027845002));
#172921=CARTESIAN_POINT('Ctrl Pts',(-7.73813365617375,-2.4782552090768,
85.5256059653377));
#172922=CARTESIAN_POINT('Ctrl Pts',(-7.74657269591682,-2.45174892889349,
85.5245088953513));
#172923=CARTESIAN_POINT('Ctrl Pts',(-7.89106860892381,-1.98970546651755,
85.5053419817239));
#172924=CARTESIAN_POINT('Ctrl Pts',(-7.99032053965758,-1.54356379451311,
85.4861025307766));
#172925=CARTESIAN_POINT('Ctrl Pts',(-8.13590802265173,-0.469609953240339,
85.4385355704836));
#172926=CARTESIAN_POINT('Ctrl Pts',(-8.14787813819847,0.159913475862779,
85.4096039041595));
#172927=CARTESIAN_POINT('Ctrl Pts',(-8.06448284348034,1.01960200084586,
85.3722260810903));
#172928=CARTESIAN_POINT('Ctrl Pts',(-8.03143645827967,1.25360762486109,
85.3623071774363));
#172929=CARTESIAN_POINT('Ctrl Pts',(-7.98432659985631,1.50687505881302,
85.3520217253124));
#172930=CARTESIAN_POINT('Ctrl Pts',(-7.98033816105292,1.52785684641247,
85.3511725808549));
#172931=CARTESIAN_POINT('Ctrl Pts',(-7.97439042331957,1.55848704138068,
85.3499369913192));
#172932=CARTESIAN_POINT('Ctrl Pts',(-7.97249626326144,1.56814789324158,
85.3495478695693));
#172933=CARTESIAN_POINT('Ctrl Pts',(-7.96911149423568,1.58524669977727,
85.3488601667896));
#172934=CARTESIAN_POINT('Ctrl Pts',(-7.96762802068115,1.59268604290622,
85.3485612989009));
#172935=CARTESIAN_POINT('Ctrl Pts',(-7.9645286183128,1.60811626304742,85.3479420889311));
#172936=CARTESIAN_POINT('Ctrl Pts',(-7.96291107619187,1.61610680979537,
85.3476218111559));
#172937=CARTESIAN_POINT('Ctrl Pts',(-7.95897655286157,1.63539376606561,
85.3468496432249));
#172938=CARTESIAN_POINT('Ctrl Pts',(-7.95664754081965,1.64668772143583,
85.3463982217424));
#172939=CARTESIAN_POINT('Ctrl Pts',(-7.94724951573237,1.69177560380963,
85.3445988922921));
#172940=CARTESIAN_POINT('Ctrl Pts',(-7.93998912970386,1.72552954802855,
85.3432582473928));
#172941=CARTESIAN_POINT('Ctrl Pts',(-7.85044985771103,2.1292680534052,85.3272896366083));
#172942=CARTESIAN_POINT('Ctrl Pts',(-7.74258969523478,2.49312719942653,
85.3135533762997));
#172943=CARTESIAN_POINT('Ctrl Pts',(-7.51811921254646,3.09287141221511,
85.2905129521433));
#172944=CARTESIAN_POINT('Ctrl Pts',(-7.41477045143502,3.333039007801,85.2811758703354));
#172945=CARTESIAN_POINT('Ctrl Pts',(-7.220812793615,3.72989229437355,85.2652024299151));
#172946=CARTESIAN_POINT('Ctrl Pts',(-7.13622117424427,3.88929037692719,
85.2586310125887));
#172947=CARTESIAN_POINT('Ctrl Pts',(-6.89635065880736,4.30706884877446,
85.2408618566845));
#172948=CARTESIAN_POINT('Ctrl Pts',(-6.73189012375179,4.5598397872675,85.2295215682954));
#172949=CARTESIAN_POINT('Ctrl Pts',(-6.52640662782762,4.84023221912691,
85.216133603404));
#172950=CARTESIAN_POINT('Ctrl Pts',(-6.49871883010637,4.87734404506329,
85.2143447063804));
#172951=CARTESIAN_POINT('Ctrl Pts',(-6.45364879607592,4.93668928062373,
85.2114566968211));
#172952=CARTESIAN_POINT('Ctrl Pts',(-6.43646522025043,4.95907242297123,
85.2103610689039));
#172953=CARTESIAN_POINT('Ctrl Pts',(-6.40562942562689,4.99880852861293,
85.2084046742599));
#172954=CARTESIAN_POINT('Ctrl Pts',(-6.39202238928627,5.01619624956497,
85.2075446796748));
#172955=CARTESIAN_POINT('Ctrl Pts',(-6.36409343928026,5.05158702558722,
85.2057862485123));
#172956=CARTESIAN_POINT('Ctrl Pts',(-6.34976558134437,5.06958517418161,
85.2048877082685));
#172957=CARTESIAN_POINT('Ctrl Pts',(-6.31488409595752,5.11302219748659,
85.2027085512907));
#172958=CARTESIAN_POINT('Ctrl Pts',(-6.29425297713415,5.13839825073588,
85.201426598406));
#172959=CARTESIAN_POINT('Ctrl Pts',(-6.24979714347838,5.1924089529434,85.1986785080433));
#172960=CARTESIAN_POINT('Ctrl Pts',(-6.22592760875505,5.22100569411556,
85.1972115659069));
#172961=CARTESIAN_POINT('Ctrl Pts',(-6.15892012011215,5.30017060423759,
85.1931163830593));
#172962=CARTESIAN_POINT('Ctrl Pts',(-6.11535729561255,5.35037479961232,
85.1904799524653));
#172963=CARTESIAN_POINT('Ctrl Pts',(-5.60168411762606,5.92788998620443,
85.1596732537404));
#172964=CARTESIAN_POINT('Ctrl Pts',(-5.06537503241138,6.39222613976513,
85.1298116893153));
#172965=CARTESIAN_POINT('Ctrl Pts',(-4.17316780741306,6.98111113265038,
85.0845204638603));
#172966=CARTESIAN_POINT('Ctrl Pts',(-3.857403025468,7.16042636672237,85.0692664032416));
#172967=CARTESIAN_POINT('Ctrl Pts',(-3.50968640450292,7.32818759927291,
85.0538675031234));
#172968=CARTESIAN_POINT('Ctrl Pts',(-3.48862468080854,7.33823752665317,
85.0529401141295));
#172969=CARTESIAN_POINT('Ctrl Pts',(-3.45911680872545,7.35216191336045,
85.0516485450925));
#172970=CARTESIAN_POINT('Ctrl Pts',(-3.45070697205153,7.35611278397529,
85.0512813174631));
#172971=CARTESIAN_POINT('Ctrl Pts',(-3.4353272125972,7.36330588771629,85.0506113550815));
#172972=CARTESIAN_POINT('Ctrl Pts',(-3.42835943640434,7.36655266926118,
85.0503084348293));
#172973=CARTESIAN_POINT('Ctrl Pts',(-3.4142862113079,7.37308609191272,85.0496978435257));
#172974=CARTESIAN_POINT('Ctrl Pts',(-3.4071805978904,7.37637236216918,85.0493901880632));
#172975=CARTESIAN_POINT('Ctrl Pts',(-3.3907705473869,7.3839330644471,85.0486811522825));
#172976=CARTESIAN_POINT('Ctrl Pts',(-3.38146274622301,7.38820019371244,
85.0482800816208));
#172977=CARTESIAN_POINT('Ctrl Pts',(-3.3494108166993,7.40282103227189,85.0469027940046));
#172978=CARTESIAN_POINT('Ctrl Pts',(-3.32662686328344,7.41308746646742,
85.0459303657641));
#172979=CARTESIAN_POINT('Ctrl Pts',(-3.04938429850158,7.53647721714288,
85.0341805580989));
#172980=CARTESIAN_POINT('Ctrl Pts',(-2.78932480999776,7.63655019190068,
85.0240793765987));
#172981=CARTESIAN_POINT('Ctrl Pts',(-2.24623406438895,7.81408427715416,
85.0040828902318));
#172982=CARTESIAN_POINT('Ctrl Pts',(-1.96310240896236,7.88997582535356,
84.9942237083096));
#172983=CARTESIAN_POINT('Ctrl Pts',(-1.05389119882884,8.08169909946907,
84.9629814264044));
#172984=CARTESIAN_POINT('Ctrl Pts',(-0.418044833291394,8.13939365751577,
84.9415732731541));
#172985=CARTESIAN_POINT('Ctrl Pts',(0.332034376420807,8.1192648282605,84.9135094626895));
#172986=CARTESIAN_POINT('Ctrl Pts',(0.446021205798871,8.1138013325801,84.9091746689908));
#172987=CARTESIAN_POINT('Ctrl Pts',(0.580351004771784,8.10452358001241,
84.90397493682));
#172988=CARTESIAN_POINT('Ctrl Pts',(0.600843783824984,8.10303008064512,
84.9031791828658));
#172989=CARTESIAN_POINT('Ctrl Pts',(0.633771601765279,8.10050472553897,
84.9018964850236));
#172990=CARTESIAN_POINT('Ctrl Pts',(0.646210366387321,8.09952192492902,
84.9014109987072));
#172991=CARTESIAN_POINT('Ctrl Pts',(0.668302189978918,8.09772521075269,
84.9005470771186));
#172992=CARTESIAN_POINT('Ctrl Pts',(0.677956162722878,8.09692267757574,
84.9001689808299));
#172993=CARTESIAN_POINT('Ctrl Pts',(0.698054429891007,8.09521571526304,
84.8993806451907));
#172994=CARTESIAN_POINT('Ctrl Pts',(0.708498452072714,8.09430833401813,
84.8989703186827));
#172995=CARTESIAN_POINT('Ctrl Pts',(0.735531853613278,8.09190693807378,
84.8979064829684));
#172996=CARTESIAN_POINT('Ctrl Pts',(0.75211841024307,8.09038212293598,84.8972520582982));
#172997=CARTESIAN_POINT('Ctrl Pts',(0.822227995032138,8.08371942848762,
84.8944786309233));
#172998=CARTESIAN_POINT('Ctrl Pts',(0.875703423722341,8.07810138913002,
84.8923453527549));
#172999=CARTESIAN_POINT('Ctrl Pts',(1.24022471970237,8.03614332857444,84.8776791718487));
#173000=CARTESIAN_POINT('Ctrl Pts',(1.54897563088413,7.98238092741736,84.8646239855646));
#173001=CARTESIAN_POINT('Ctrl Pts',(2.18728376632444,7.83280096065651,84.8363617632022));
#173002=CARTESIAN_POINT('Ctrl Pts',(2.51544119488379,7.73366112403378,84.8210940357378));
#173003=CARTESIAN_POINT('Ctrl Pts',(3.05109895483064,7.53412240022367,84.7953545241231));
#173004=CARTESIAN_POINT('Ctrl Pts',(3.26236997469419,7.44507541805762,84.784983184393));
#173005=CARTESIAN_POINT('Ctrl Pts',(3.8561195476993,7.16468758588721,84.7555645357176));
#173006=CARTESIAN_POINT('Ctrl Pts',(4.22770210842211,6.95191042349121,84.7368141046931));
#173007=CARTESIAN_POINT('Ctrl Pts',(4.60406821598988,6.69500058930455,84.7185739507044));
#173008=CARTESIAN_POINT('Ctrl Pts',(4.62719246156382,6.67903937560237,84.7174559658574));
#173009=CARTESIAN_POINT('Ctrl Pts',(4.65847882667002,6.65720389360648,84.7159463933059));
#173010=CARTESIAN_POINT('Ctrl Pts',(4.66671333508219,6.65143407912942,84.7155493632374));
#173011=CARTESIAN_POINT('Ctrl Pts',(4.68065411141514,6.64162732387729,84.7148776518969));
#173012=CARTESIAN_POINT('Ctrl Pts',(4.68636590543443,6.63759828709141,84.714602567414));
#173013=CARTESIAN_POINT('Ctrl Pts',(4.6973584483303,6.62982300598948,84.7140733906467));
#173014=CARTESIAN_POINT('Ctrl Pts',(4.70263993001324,6.62607781208529,84.7138192459152));
#173015=CARTESIAN_POINT('Ctrl Pts',(4.71509489714885,6.61722337814759,84.7132201445937));
#173016=CARTESIAN_POINT('Ctrl Pts',(4.72226457191375,6.61210877398739,84.7128754546932));
#173017=CARTESIAN_POINT('Ctrl Pts',(4.74315949175458,6.59715172277083,84.711871396121));
#173018=CARTESIAN_POINT('Ctrl Pts',(4.7568624288728,6.58727809156614,84.7112135471533));
#173019=CARTESIAN_POINT('Ctrl Pts',(4.85526232029924,6.51590903840302,84.7064932757088));
#173020=CARTESIAN_POINT('Ctrl Pts',(4.9387969619139,6.45282329183333,84.7025057347998));
#173021=CARTESIAN_POINT('Ctrl Pts',(5.31333354294604,6.15843675536292,84.684611365784));
#173022=CARTESIAN_POINT('Ctrl Pts',(5.58948209517873,5.90893990133547,84.6713460422368));
#173023=CARTESIAN_POINT('Ctrl Pts',(6.06029310433106,5.42092166135052,84.6470648268455));
#173024=CARTESIAN_POINT('Ctrl Pts',(6.26035708909408,5.18859034085921,84.6360881806754));
#173025=CARTESIAN_POINT('Ctrl Pts',(6.72256862175774,4.58606596824537,84.6083261918241));
#173026=CARTESIAN_POINT('Ctrl Pts',(6.96775557051908,4.2041979491997,84.5912784181376));
#173027=CARTESIAN_POINT('Ctrl Pts',(7.26204193379715,3.64873549229596,84.567114547839));
#173028=CARTESIAN_POINT('Ctrl Pts',(7.3391992317856,3.49094221534271,84.5603324260626));
#173029=CARTESIAN_POINT('Ctrl Pts',(7.4358127127681,3.27597113800049,84.5511676643614));
#173030=CARTESIAN_POINT('Ctrl Pts',(7.45983397313095,3.22089655835049,84.548826128002));
#173031=CARTESIAN_POINT('Ctrl Pts',(7.49717101063571,3.13263349648626,84.5450823782366));
#173032=CARTESIAN_POINT('Ctrl Pts',(7.51088241760751,3.09961466700231,84.5436838082965));
#173033=CARTESIAN_POINT('Ctrl Pts',(7.53874412654534,3.03124958817437,84.5407917631937));
#173034=CARTESIAN_POINT('Ctrl Pts',(7.55286481414032,2.99589221386206,84.5392980551749));
#173035=CARTESIAN_POINT('Ctrl Pts',(7.58029743367601,2.92577574020036,84.5363395271524));
#173036=CARTESIAN_POINT('Ctrl Pts',(7.59362007026261,2.89102180562507,84.534874844425));
#173037=CARTESIAN_POINT('Ctrl Pts',(7.62404245166368,2.80999952289691,84.5314638981928));
#173038=CARTESIAN_POINT('Ctrl Pts',(7.64096057350713,2.76366461559956,84.529516026765));
#173039=CARTESIAN_POINT('Ctrl Pts',(7.68407732277075,2.64215453634266,84.5244143060415));
#173040=CARTESIAN_POINT('Ctrl Pts',(7.70959481037355,2.5667435851059,84.5212544762741));
#173041=CARTESIAN_POINT('Ctrl Pts',(7.78346736341931,2.33738302898675,84.5116601939234));
#173042=CARTESIAN_POINT('Ctrl Pts',(7.82834829574597,2.18235781850355,84.5051969493021));
#173043=CARTESIAN_POINT('Ctrl Pts',(7.94554339837831,1.72721785349693,84.4862744354011));
#173044=CARTESIAN_POINT('Ctrl Pts',(8.00541104878279,1.42419521916794,84.47373707899));
#173045=CARTESIAN_POINT('Ctrl Pts',(8.08845278629873,0.826692009431081,
84.4492202069406));
#173046=CARTESIAN_POINT('Ctrl Pts',(8.1131083316348,0.532884010314892,84.4372606206839));
#173047=CARTESIAN_POINT('Ctrl Pts',(8.12405743158788,0.159848718546276,
84.4223301803258));
#173048=CARTESIAN_POINT('Ctrl Pts',(8.12522331389318,0.0812831978779437,
84.4192002007009));
#173049=CARTESIAN_POINT('Ctrl Pts',(8.12524954711001,0.00271287458458927,
84.4160871754279));
#173050=CARTESIAN_POINT('',(8.12696554915539,0.00168838483199298,82.4167025567875));
#173051=CARTESIAN_POINT('Ctrl Pts',(8.12696554915539,0.00168838483199298,
82.4167025567875));
#173052=CARTESIAN_POINT('Ctrl Pts',(8.1306575932175,0.773914348629653,82.4468290208393));
#173053=CARTESIAN_POINT('Ctrl Pts',(7.6585312809221,4.25683691476204,82.5827337950821));
#173054=CARTESIAN_POINT('Ctrl Pts',(3.83053466397931,8.09334768555451,82.7715277244204));
#173055=CARTESIAN_POINT('Ctrl Pts',(-1.74999298391506,8.26945455504389,
82.9830843448022));
#173056=CARTESIAN_POINT('Ctrl Pts',(-6.7807722929522,5.84776877811943,83.1946409651841));
#173057=CARTESIAN_POINT('Ctrl Pts',(-8.9610148003001,0.17955105281233,83.406197585566));
#173058=CARTESIAN_POINT('Ctrl Pts',(-6.81611969460216,-5.00581298154604,
83.617754205948));
#173059=CARTESIAN_POINT('Ctrl Pts',(-3.62342745787797,-7.65690432669867,
83.7764216712344));
#173060=CARTESIAN_POINT('Ctrl Pts',(0.494311211966013,-8.45828284271794,
83.9350891365208));
#173061=CARTESIAN_POINT('Ctrl Pts',(4.46947152341248,-7.18896984766675,
84.0937566018073));
#173062=CARTESIAN_POINT('Ctrl Pts',(7.36660492052287,-4.18569279410471,
84.2524240670937));
#173063=CARTESIAN_POINT('Ctrl Pts',(8.11510270816399,-1.4397668579716,84.3600727187538));
#173064=CARTESIAN_POINT('Ctrl Pts',(8.12636183407427,-0.0449434531184864,
84.4148322153184));
#173065=CARTESIAN_POINT('Ctrl Pts',(8.12631724021387,0.00268884911775716,
84.4167025567875));
#173066=CARTESIAN_POINT('',(8.12524999728007,0.000210238465757252,80.4167025567658));
#173067=CARTESIAN_POINT('Ctrl Pts',(8.12524999728006,0.000210239022574176,
80.4167025567875));
#173068=CARTESIAN_POINT('Ctrl Pts',(8.12524459943052,0.208824588488869,
80.4248543423937));
#173069=CARTESIAN_POINT('Ctrl Pts',(8.11720065752198,0.417390467344348,
80.4330061279999));
#173070=CARTESIAN_POINT('Ctrl Pts',(8.10115533523439,0.625275776680494,
80.4411579136061));
#173071=CARTESIAN_POINT('Ctrl Pts',(8.08510346328949,0.833245944239645,
80.4493130267492));
#173072=CARTESIAN_POINT('Ctrl Pts',(8.06104371662649,1.04053468585204,80.4574681398922));
#173073=CARTESIAN_POINT('Ctrl Pts',(8.02906513843042,1.24651536907546,80.4656232530353));
#173074=CARTESIAN_POINT('Ctrl Pts',(7.99707056053867,1.45259910967143,80.4737824463889));
#173075=CARTESIAN_POINT('Ctrl Pts',(7.95714929118456,1.65737318666362,80.4819416397424));
#173076=CARTESIAN_POINT('Ctrl Pts',(7.90944159300706,1.86022075284359,80.4901008330959));
#173077=CARTESIAN_POINT('Ctrl Pts',(7.86170562258791,2.06318852929624,80.4982648617003));
#173078=CARTESIAN_POINT('Ctrl Pts',(7.80617408419124,2.26422722204124,80.5064288903046));
#173079=CARTESIAN_POINT('Ctrl Pts',(7.74303743588964,2.46273401505552,80.514592918909));
#173080=CARTESIAN_POINT('Ctrl Pts',(7.67982447814697,2.66148073120212,80.52276681488));
#173081=CARTESIAN_POINT('Ctrl Pts',(7.60898812947687,2.85768914198913,80.530940710851));
#173082=CARTESIAN_POINT('Ctrl Pts',(7.53076805115067,3.05077369240465,80.539114606822));
#173083=CARTESIAN_POINT('Ctrl Pts',(7.4524980509439,3.24398147388913,80.5472937195644));
#173084=CARTESIAN_POINT('Ctrl Pts',(7.36683503684257,3.43406113856047,80.5554728323067));
#173085=CARTESIAN_POINT('Ctrl Pts',(7.2740657327235,3.62044959618523,80.563651945049));
#173086=CARTESIAN_POINT('Ctrl Pts',(7.18117875495046,3.80707447911331,80.5718414326248));
#173087=CARTESIAN_POINT('Ctrl Pts',(7.08116761105212,3.98999852830687,80.5800309202006));
#173088=CARTESIAN_POINT('Ctrl Pts',(6.97436452454461,4.1686840898866,80.5882204077763));
#173089=CARTESIAN_POINT('Ctrl Pts',(6.90980065891797,4.2767018538343,80.5931710603528));
#173090=CARTESIAN_POINT('Ctrl Pts',(6.84275562068071,4.38317127256495,80.5981217129293));
#173091=CARTESIAN_POINT('Ctrl Pts',(6.77331025023344,4.48797903477529,80.6030723655058));
#173092=CARTESIAN_POINT('Ctrl Pts',(6.659996676596,4.65899320036341,80.6111503141389));
#173093=CARTESIAN_POINT('Ctrl Pts',(6.54007552376464,4.82590562692456,80.6192282627719));
#173094=CARTESIAN_POINT('Ctrl Pts',(6.41386406614782,4.98818958174986,80.627306211405));
#173095=CARTESIAN_POINT('Ctrl Pts',(6.28780706572278,5.15027493397276,80.6353742742695));
#173096=CARTESIAN_POINT('Ctrl Pts',(6.15547529762081,5.30774285812216,80.643442337134));
#173097=CARTESIAN_POINT('Ctrl Pts',(6.0172298773309,5.46009451986468,80.6515103999985));
#173098=CARTESIAN_POINT('Ctrl Pts',(5.87913662159627,5.61227849053428,80.6595695824734));
#173099=CARTESIAN_POINT('Ctrl Pts',(5.73514290059066,5.75935719275781,80.6676287649483));
#173100=CARTESIAN_POINT('Ctrl Pts',(5.58565112702972,5.90086341560383,80.6756879474232));
#173101=CARTESIAN_POINT('Ctrl Pts',(5.43635137042584,6.04218787865351,80.6837367781599));
#173102=CARTESIAN_POINT('Ctrl Pts',(5.281567878021,6.17795392555325,80.6917856088966));
#173103=CARTESIAN_POINT('Ctrl Pts',(5.12174108426708,6.30772984743565,80.6998344396333));
#173104=CARTESIAN_POINT('Ctrl Pts',(4.96203518277804,6.43740760739694,80.7078771822708));
#173105=CARTESIAN_POINT('Ctrl Pts',(4.79729382770052,6.56110407541399,80.7159199249083));
#173106=CARTESIAN_POINT('Ctrl Pts',(4.62799282585794,6.67842571017358,80.7239626675458));
#173107=CARTESIAN_POINT('Ctrl Pts',(4.45882972605523,6.79565178204471,80.7319988590667));
#173108=CARTESIAN_POINT('Ctrl Pts',(4.28511464679758,6.9065131992776,80.7400350505875));
#173109=CARTESIAN_POINT('Ctrl Pts',(4.10735508293929,7.01065772842697,80.7480712421083));
#173110=CARTESIAN_POINT('Ctrl Pts',(4.00657258513179,7.06970347287438,80.7526274383362));
#173111=CARTESIAN_POINT('Ctrl Pts',(3.90449059302425,7.12659087020588,80.7571836345642));
#173112=CARTESIAN_POINT('Ctrl Pts',(3.80120582549754,7.18126185532205,80.7617398307921));
#173113=CARTESIAN_POINT('Ctrl Pts',(3.61902545151273,7.27769408587345,80.7697763453008));
#173114=CARTESIAN_POINT('Ctrl Pts',(3.43324562569166,7.3671517422415,80.7778128598094));
#173115=CARTESIAN_POINT('Ctrl Pts',(3.24443259173022,7.44938552635173,80.785849374318));
#173116=CARTESIAN_POINT('Ctrl Pts',(3.0555054959029,7.53166898785266,80.7938907436814));
#173117=CARTESIAN_POINT('Ctrl Pts',(2.86354182583267,7.60671974469297,80.8019321130447));
#173118=CARTESIAN_POINT('Ctrl Pts',(2.6691263568128,7.67433723873712,80.809973482408));
#173119=CARTESIAN_POINT('Ctrl Pts',(2.47456967054992,7.74200384798869,80.8180206927675));
#173120=CARTESIAN_POINT('Ctrl Pts',(2.27755793023016,7.80222631870286,80.826067903127));
#173121=CARTESIAN_POINT('Ctrl Pts',(2.07869014701708,7.85485422112938,80.8341151134865));
#173122=CARTESIAN_POINT('Ctrl Pts',(1.87952924689276,7.90755969332591,80.8421741848595));
#173123=CARTESIAN_POINT('Ctrl Pts',(1.67850714185685,7.95264814364333,80.8502332562324));
#173124=CARTESIAN_POINT('Ctrl Pts',(1.47623382200582,7.9900201041841,80.8582923276053));
#173125=CARTESIAN_POINT('Ctrl Pts',(1.27379679243258,8.02742231168617,80.8663579215801));
#173126=CARTESIAN_POINT('Ctrl Pts',(1.07010683907458,8.05709552086541,80.8744235155549));
#173127=CARTESIAN_POINT('Ctrl Pts',(0.865779028174559,8.07899215477235,
80.8824891095297));
#173128=CARTESIAN_POINT('Ctrl Pts',(0.6611303759287,8.10092317139723,80.8905673683298));
#173129=CARTESIAN_POINT('Ctrl Pts',(0.455842178950087,8.11505318318403,
80.8986456271299));
#173130=CARTESIAN_POINT('Ctrl Pts',(0.250531238446654,8.12138668338495,
80.9067238859299));
#173131=CARTESIAN_POINT('Ctrl Pts',(0.134608823462328,8.12496269661052,
80.9112850226462));
#173132=CARTESIAN_POINT('Ctrl Pts',(0.0186791101409345,8.12605417183529,
80.9158461593624));
#173133=CARTESIAN_POINT('Ctrl Pts',(-0.0971476232167939,8.12466921799302,
80.9204072960786));
#173134=CARTESIAN_POINT('Ctrl Pts',(-0.302490603172819,8.12221390788602,
80.9284934898108));
#173135=CARTESIAN_POINT('Ctrl Pts',(-0.507909199282271,8.11196749316603,
80.936579683543));
#173136=CARTESIAN_POINT('Ctrl Pts',(-0.712787867911589,8.09392494515844,
80.9446658772752));
#173137=CARTESIAN_POINT('Ctrl Pts',(-0.917483794490565,8.0758984902475,
80.9527448585063));
#173138=CARTESIAN_POINT('Ctrl Pts',(-1.12164043977352,8.05008979489223,
80.9608238397374));
#173139=CARTESIAN_POINT('Ctrl Pts',(-1.32464345182455,8.01654584519033,
80.9689028209685));
#173140=CARTESIAN_POINT('Ctrl Pts',(-1.52749311596407,7.98302723449487,
80.9769756993596));
#173141=CARTESIAN_POINT('Ctrl Pts',(-1.7291905731799,7.94178507272085,80.9850485777507));
#173142=CARTESIAN_POINT('Ctrl Pts',(-1.9291271513624,7.89291809132569,80.9931214561418));
#173143=CARTESIAN_POINT('Ctrl Pts',(-2.1289399598695,7.84408136077547,81.0011893370605));
#173144=CARTESIAN_POINT('Ctrl Pts',(-2.32699375628324,7.7876292988069,81.0092572179792));
#173145=CARTESIAN_POINT('Ctrl Pts',(-2.52268999577819,7.72371172090858,
81.0173250988979));
#173146=CARTESIAN_POINT('Ctrl Pts',(-2.71829174134733,7.65982500626487,
81.025389084158));
#173147=CARTESIAN_POINT('Ctrl Pts',(-2.91153789986559,7.58848006361889,
81.033453069418));
#173148=CARTESIAN_POINT('Ctrl Pts',(-3.10184442633261,7.50987674448318,
81.0415170546781));
#173149=CARTESIAN_POINT('Ctrl Pts',(-3.29479560410711,7.43018109091952,
81.0496931035103));
#173150=CARTESIAN_POINT('Ctrl Pts',(-3.48472452195033,7.34302391677189,
81.0578691523426));
#173151=CARTESIAN_POINT('Ctrl Pts',(-3.67104154432248,7.24866481100888,
81.0660452011748));
#173152=CARTESIAN_POINT('Ctrl Pts',(-3.85471778056681,7.15564311507756,
81.0741053658218));
#173153=CARTESIAN_POINT('Ctrl Pts',(-4.03488354464302,7.05562244642963,
81.0821655304687));
#173154=CARTESIAN_POINT('Ctrl Pts',(-4.21099665840461,6.94889881243101,
81.0902256951157));
#173155=CARTESIAN_POINT('Ctrl Pts',(-4.38710126326462,6.84218033478265,
81.098285470336));
#173156=CARTESIAN_POINT('Ctrl Pts',(-4.55915333750779,6.72875970196976,
81.1063452455563));
#173157=CARTESIAN_POINT('Ctrl Pts',(-4.72663756575908,6.608977597515,81.1144050207765));
#173158=CARTESIAN_POINT('Ctrl Pts',(-4.89413443928235,6.48918644935919,
81.1224654045201));
#173159=CARTESIAN_POINT('Ctrl Pts',(-5.05706252164284,6.36303305635309,
81.1305257882637));
#173160=CARTESIAN_POINT('Ctrl Pts',(-5.2149371278674,6.2309002812507,81.1385861720072));
#173161=CARTESIAN_POINT('Ctrl Pts',(-5.37678036407692,6.09544597074875,
81.1468491765609));
#173162=CARTESIAN_POINT('Ctrl Pts',(-5.53331245352298,5.95370793904956,
81.1551121811146));
#173163=CARTESIAN_POINT('Ctrl Pts',(-5.68404881754922,5.80614128334966,
81.1633751856683));
#173164=CARTESIAN_POINT('Ctrl Pts',(-5.83120982392957,5.66207480210431,
81.1714421977241));
#173165=CARTESIAN_POINT('Ctrl Pts',(-5.97284671912935,5.51245330939077,
81.1795092097799));
#173166=CARTESIAN_POINT('Ctrl Pts',(-6.10854703049046,5.35773653129623,
81.1875762218357));
#173167=CARTESIAN_POINT('Ctrl Pts',(-6.2491927124805,5.19738135928412,81.1959372226383));
#173168=CARTESIAN_POINT('Ctrl Pts',(-6.38346074163059,5.03155283186272,
81.204298223441));
#173169=CARTESIAN_POINT('Ctrl Pts',(-6.51093842226193,4.86079915487292,
81.2126592242436));
#173170=CARTESIAN_POINT('Ctrl Pts',(-6.63841610289319,4.69004547788324,
81.2210202250463));
#173171=CARTESIAN_POINT('Ctrl Pts',(-6.75910324131319,4.51436697576811,
81.2293812258489));
#173172=CARTESIAN_POINT('Ctrl Pts',(-6.87263762475796,4.33434419967556,
81.2377422266515));
#173173=CARTESIAN_POINT('Ctrl Pts',(-6.9755429317437,4.17117513603027,81.245320471481));
#173174=CARTESIAN_POINT('Ctrl Pts',(-7.07277811459327,4.00411003239889,
81.2528987163104));
#173175=CARTESIAN_POINT('Ctrl Pts',(-7.16402220555559,3.8335979706806,81.2604769611398));
#173176=CARTESIAN_POINT('Ctrl Pts',(-7.2551983993909,3.66321279147042,81.268049566798));
#173177=CARTESIAN_POINT('Ctrl Pts',(-7.34039219791648,3.48938607867542,
81.2756221724562));
#173178=CARTESIAN_POINT('Ctrl Pts',(-7.41932581694009,3.31259595854766,
81.2831947781144));
#173179=CARTESIAN_POINT('Ctrl Pts',(-7.49821568866519,3.1359038206264,81.2907631868152));
#173180=CARTESIAN_POINT('Ctrl Pts',(-7.57085213553342,2.95625187796577,
81.298331595516));
#173181=CARTESIAN_POINT('Ctrl Pts',(-7.63700326572716,2.77414287335255,
81.3059000042167));
#173182=CARTESIAN_POINT('Ctrl Pts',(-7.7031384132797,2.59207786772876,81.3134665843295));
#173183=CARTESIAN_POINT('Ctrl Pts',(-7.76279123005642,2.40755732401736,
81.3210331644424));
#173184=CARTESIAN_POINT('Ctrl Pts',(-7.8157778942537,2.22110411061598,81.3285997445552));
#173185=CARTESIAN_POINT('Ctrl Pts',(-7.86875515885646,2.03468397317115,
81.3361649823909));
#173186=CARTESIAN_POINT('Ctrl Pts',(-7.9150685271603,1.84633220301755,81.3437302202266));
#173187=CARTESIAN_POINT('Ctrl Pts',(-7.95458408897748,1.65658671185251,
81.3512954580623));
#173188=CARTESIAN_POINT('Ctrl Pts',(-7.9941133922517,1.46677523707505,81.3588633266942));
#173189=CARTESIAN_POINT('Ctrl Pts',(-8.02684008813676,1.27556943279536,
81.3664311953262));
#173190=CARTESIAN_POINT('Ctrl Pts',(-8.05268134402219,1.08351775903164,
81.3739990639581));
#173191=CARTESIAN_POINT('Ctrl Pts',(-8.07818913229328,0.893944409609616,
81.3814692732848));
#173192=CARTESIAN_POINT('Ctrl Pts',(-8.09698812161514,0.703547240953842,
81.3889394826114));
#173193=CARTESIAN_POINT('Ctrl Pts',(-8.10904828820644,0.512858091518751,
81.396409691938));
#173194=CARTESIAN_POINT('Ctrl Pts',(-8.12407196333666,0.275311469730006,
81.4057155333813));
#173195=CARTESIAN_POINT('Ctrl Pts',(-8.12863291018924,0.0374285285094461,
81.4150213748245));
#173196=CARTESIAN_POINT('Ctrl Pts',(-8.12278920829472,-0.199957595781936,
81.4243272162678));
#173197=CARTESIAN_POINT('Ctrl Pts',(-8.11691413274366,-0.438618198283218,
81.4336830188964));
#173198=CARTESIAN_POINT('Ctrl Pts',(-8.1005224424968,-0.676776590626742,
81.443038821525));
#173199=CARTESIAN_POINT('Ctrl Pts',(-8.07372435994447,-0.913598665793323,
81.4523946241535));
#173200=CARTESIAN_POINT('Ctrl Pts',(-8.04679618730156,-1.15157038310867,
81.4617958441066));
#173201=CARTESIAN_POINT('Ctrl Pts',(-8.00936037089796,-1.38819273836294,
81.4711970640597));
#173202=CARTESIAN_POINT('Ctrl Pts',(-7.96157967035697,-1.62263264944919,
81.4805982840128));
#173203=CARTESIAN_POINT('Ctrl Pts',(-7.91374725691933,-1.85732629408804,
81.4900096788756));
#173204=CARTESIAN_POINT('Ctrl Pts',(-7.8555475825956,-2.08983273577795,
81.4994210737384));
#173205=CARTESIAN_POINT('Ctrl Pts',(-7.7871943750683,-2.3193299306922,81.5088324686013));
#173206=CARTESIAN_POINT('Ctrl Pts',(-7.71892134699995,-2.54855792154732,
81.51823282374));
#173207=CARTESIAN_POINT('Ctrl Pts',(-7.64051860677562,-2.77478368759938,
81.5276331788788));
#173208=CARTESIAN_POINT('Ctrl Pts',(-7.55224908031308,-2.9972022606775,
81.5370335340176));
#173209=CARTESIAN_POINT('Ctrl Pts',(-7.4957724170166,-3.13951025037706,
81.5430480750865));
#173210=CARTESIAN_POINT('Ctrl Pts',(-7.43525758628962,-3.28025997400512,
81.5490626161554));
#173211=CARTESIAN_POINT('Ctrl Pts',(-7.37078419891237,-3.41924375492063,
81.5550771572243));
#173212=CARTESIAN_POINT('Ctrl Pts',(-7.28778996778099,-3.59815248774896,
81.5628194557436));
#173213=CARTESIAN_POINT('Ctrl Pts',(-7.19819439753301,-3.77421770557299,
81.5705617542628));
#173214=CARTESIAN_POINT('Ctrl Pts',(-7.10222249715836,-3.94691311829354,
81.578304052782));
#173215=CARTESIAN_POINT('Ctrl Pts',(-7.00631037858702,-4.1195009574102,
81.5860415285504));
#173216=CARTESIAN_POINT('Ctrl Pts',(-6.90403000922432,-4.28872286342957,
81.5937790043187));
#173217=CARTESIAN_POINT('Ctrl Pts',(-6.79565360961821,-4.45407449203344,
81.601516480087));
#173218=CARTESIAN_POINT('Ctrl Pts',(-6.68732545709304,-4.6193525092843,
81.6092505112805));
#173219=CARTESIAN_POINT('Ctrl Pts',(-6.57290687248712,-4.78076338577519,
81.6169845424741));
#173220=CARTESIAN_POINT('Ctrl Pts',(-6.45271499555188,-4.93782915345194,
81.6247185736676));
#173221=CARTESIAN_POINT('Ctrl Pts',(-6.33253849939175,-5.0948748216568,
81.6324516151486));
#173222=CARTESIAN_POINT('Ctrl Pts',(-6.20659039092785,-5.24757620352785,
81.6401846566297));
#173223=CARTESIAN_POINT('Ctrl Pts',(-6.07523016469535,-5.39548570644717,
81.6479176981108));
#173224=CARTESIAN_POINT('Ctrl Pts',(-5.94388306125145,-5.54338043331749,
81.6556499670668));
#173225=CARTESIAN_POINT('Ctrl Pts',(-5.80712515435242,-5.68648397292756,
81.6633822360228));
#173226=CARTESIAN_POINT('Ctrl Pts',(-5.66535503287332,-5.82438322176666,
81.6711145049788));
#173227=CARTESIAN_POINT('Ctrl Pts',(-5.52353037887633,-5.96233551417499,
81.678849748187));
#173228=CARTESIAN_POINT('Ctrl Pts',(-5.37668991187192,-6.0950792696329,
81.6865849913952));
#173229=CARTESIAN_POINT('Ctrl Pts',(-5.22526823113462,-6.22223910463069,
81.6943202346034));
#173230=CARTESIAN_POINT('Ctrl Pts',(-5.09852050495581,-6.32867841945512,
81.7007950305725));
#173231=CARTESIAN_POINT('Ctrl Pts',(-4.96856363617686,-6.43120594199879,
81.7072698265417));
#173232=CARTESIAN_POINT('Ctrl Pts',(-4.83566957250131,-6.52962382898778,
81.7137446225108));
#173233=CARTESIAN_POINT('Ctrl Pts',(-4.66297215341838,-6.65751904570784,
81.7221586970152));
#173234=CARTESIAN_POINT('Ctrl Pts',(-4.48523094752583,-6.77853522090792,
81.7305727715196));
#173235=CARTESIAN_POINT('Ctrl Pts',(-4.30300596328412,-6.89230202780183,
81.738986846024));
#173236=CARTESIAN_POINT('Ctrl Pts',(-4.12073008861839,-7.00610060663452,
81.747403270348));
#173237=CARTESIAN_POINT('Ctrl Pts',(-3.93396815978001,-7.11264563565909,
81.7558196946719));
#173238=CARTESIAN_POINT('Ctrl Pts',(-3.7433071235897,-7.21161142470825,
81.7642361189958));
#173239=CARTESIAN_POINT('Ctrl Pts',(-3.55259880479061,-7.31060175658367,
81.7726546305343));
#173240=CARTESIAN_POINT('Ctrl Pts',(-3.35798968248173,-7.40200897445001,
81.7810731420728));
#173241=CARTESIAN_POINT('Ctrl Pts',(-3.16009011446938,-7.4855539561834,
81.7894916536113));
#173242=CARTESIAN_POINT('Ctrl Pts',(-2.96211453405986,-7.56913102719518,
81.7979133986649));
#173243=CARTESIAN_POINT('Ctrl Pts',(-2.76084622511553,-7.64483972350749,
81.8063351437186));
#173244=CARTESIAN_POINT('Ctrl Pts',(-2.55691561110987,-7.71244903517441,
81.8147568887722));
#173245=CARTESIAN_POINT('Ctrl Pts',(-2.35296289158296,-7.78006567550594,
81.8231795467199));
#173246=CARTESIAN_POINT('Ctrl Pts',(-2.14634754228693,-7.83958109807804,
81.8316022046677));
#173247=CARTESIAN_POINT('Ctrl Pts',(-1.93771581692596,-7.89081396152101,
81.8400248626155));
#173248=CARTESIAN_POINT('Ctrl Pts',(-1.7290444158138,-7.94205656798049,
81.8484491223104));
#173249=CARTESIAN_POINT('Ctrl Pts',(-1.51835612891157,-7.98501340574969,
81.8568733820054));
#173250=CARTESIAN_POINT('Ctrl Pts',(-1.30630938408856,-8.01955381274683,
81.8652976417003));
#173251=CARTESIAN_POINT('Ctrl Pts',(-1.2466168931683,-8.02927715432785,
81.8676691237326));
#173252=CARTESIAN_POINT('Ctrl Pts',(-1.18681680887079,-8.03833384078446,
81.8700406057649));
#173253=CARTESIAN_POINT('Ctrl Pts',(-1.12692394473616,-8.04672169179973,
81.8724120877972));
#173254=CARTESIAN_POINT('Ctrl Pts',(-0.914163755552061,-8.07651824260159,
81.8808364130173));
#173255=CARTESIAN_POINT('Ctrl Pts',(-0.700210299611324,-8.09787375757291,
81.8892607382374));
#173256=CARTESIAN_POINT('Ctrl Pts',(-0.485731139424045,-8.11071839128285,
81.8976850634575));
#173257=CARTESIAN_POINT('Ctrl Pts',(-0.271289043858642,-8.12356080528299,
81.9061079328512));
#173258=CARTESIAN_POINT('Ctrl Pts',(-0.0563216888205175,-8.12789525985763,
81.9145308022449));
#173259=CARTESIAN_POINT('Ctrl Pts',(0.158499999989702,-8.12370391585656,
81.9229536716386));
#173260=CARTESIAN_POINT('Ctrl Pts',(0.373277789627329,-8.11951342836367,
81.9313748198047));
#173261=CARTESIAN_POINT('Ctrl Pts',(0.587909708756205,-8.10680062662074,
81.9397959679709));
#173262=CARTESIAN_POINT('Ctrl Pts',(0.801725487033302,-8.08559978022294,
81.9482171161371));
#173263=CARTESIAN_POINT('Ctrl Pts',(1.01548127581744,-8.06440488206729,
81.9566359016133));
#173264=CARTESIAN_POINT('Ctrl Pts',(1.22842111863655,-8.0347267216894,81.9650546870894));
#173265=CARTESIAN_POINT('Ctrl Pts',(1.43987950438145,-7.9966514601652,81.9734734725656));
#173266=CARTESIAN_POINT('Ctrl Pts',(1.65127882064198,-7.9585868347104,81.9818899063104));
#173267=CARTESIAN_POINT('Ctrl Pts',(1.8611972465454,-7.91212983823219,81.9903063400551));
#173268=CARTESIAN_POINT('Ctrl Pts',(2.06897795081504,-7.85741801112434,
81.9987227737999));
#173269=CARTESIAN_POINT('Ctrl Pts',(2.27668324276792,-7.80272604122918,
82.0071361528685));
#173270=CARTESIAN_POINT('Ctrl Pts',(2.48225210746732,-7.73978529084876,
82.0155495319372));
#173271=CARTESIAN_POINT('Ctrl Pts',(2.68504042990407,-7.66878383136991,
82.0239629110058));
#173272=CARTESIAN_POINT('Ctrl Pts',(2.74221808692595,-7.64876444835341,
82.0263351250317));
#173273=CARTESIAN_POINT('Ctrl Pts',(2.79917477723441,-7.62810454540091,
82.0287073390576));
#173274=CARTESIAN_POINT('Ctrl Pts',(2.85589627835543,-7.60680905569317,
82.0310795530836));
#173275=CARTESIAN_POINT('Ctrl Pts',(3.04085062681898,-7.53736989512329,
82.0388147379943));
#173276=CARTESIAN_POINT('Ctrl Pts',(3.22338505814561,-7.46113825452443,
82.046549922905));
#173277=CARTESIAN_POINT('Ctrl Pts',(3.40296248152987,-7.37831511334397,
82.0542851078156));
#173278=CARTESIAN_POINT('Ctrl Pts',(3.58248437513806,-7.29551758312505,
82.062017900816));
#173279=CARTESIAN_POINT('Ctrl Pts',(3.75905076128054,-7.20613275912688,
82.0697506938165));
#173280=CARTESIAN_POINT('Ctrl Pts',(3.93214466327643,-7.11040968647846,
82.0774834868169));
#173281=CARTESIAN_POINT('Ctrl Pts',(4.10521579413556,-7.01469920655082,
82.08521526254));
#173282=CARTESIAN_POINT('Ctrl Pts',(4.27481504204639,-6.91265231042138,
82.0929470382632));
#173283=CARTESIAN_POINT('Ctrl Pts',(4.44045005482825,-6.80456397376612,
82.1006788139864));
#173284=CARTESIAN_POINT('Ctrl Pts',(4.60614433633973,-6.69643696015305,
82.10841335635));
#173285=CARTESIAN_POINT('Ctrl Pts',(4.76787125016454,-6.5822643766721,82.1161478987136));
#173286=CARTESIAN_POINT('Ctrl Pts',(4.92516691846625,-6.46238488390668,
82.1238824410772));
#173287=CARTESIAN_POINT('Ctrl Pts',(5.08248915225231,-6.34248514483173,
82.1316182897188));
#173288=CARTESIAN_POINT('Ctrl Pts',(5.23537837285552,-6.21687679627382,
82.1393541383604));
#173289=CARTESIAN_POINT('Ctrl Pts',(5.38340372193394,-6.08593886998282,
82.1470899870019));
#173290=CARTESIAN_POINT('Ctrl Pts',(5.53155019205584,-5.95489380435142,
82.1548321654652));
#173291=CARTESIAN_POINT('Ctrl Pts',(5.67482457935493,-5.81851068804195,
82.1625743439284));
#173292=CARTESIAN_POINT('Ctrl Pts',(5.81283217824947,-5.67720614651323,
82.1703165223916));
#173293=CARTESIAN_POINT('Ctrl Pts',(5.92828444223744,-5.55899577721508,
82.1767933543844));
#173294=CARTESIAN_POINT('Ctrl Pts',(6.04005138833563,-5.4373419236115,82.1832701863773));
#173295=CARTESIAN_POINT('Ctrl Pts',(6.14792370588864,-5.3125061570856,82.1897470183702));
#173296=CARTESIAN_POINT('Ctrl Pts',(6.30444885781006,-5.13136666028106,
82.1991450468417));
#173297=CARTESIAN_POINT('Ctrl Pts',(6.45286304564321,-4.94342492763543,
82.2085430753132));
#173298=CARTESIAN_POINT('Ctrl Pts',(6.59266451167577,-4.74936439947398,
82.2179411037848));
#173299=CARTESIAN_POINT('Ctrl Pts',(6.73266490349367,-4.55502773942305,
82.2273525048642));
#173300=CARTESIAN_POINT('Ctrl Pts',(6.86402803751655,-4.35455489830909,
82.2367639059436));
#173301=CARTESIAN_POINT('Ctrl Pts',(6.98629423363136,-4.14866007810102,
82.2461753070231));
#173302=CARTESIAN_POINT('Ctrl Pts',(7.1083763373526,-3.94307526729443,82.2555725376498));
#173303=CARTESIAN_POINT('Ctrl Pts',(7.22138886300046,-3.7320848268843,82.2649697682766));
#173304=CARTESIAN_POINT('Ctrl Pts',(7.32491838891015,-3.51642690217015,
82.2743669989033));
#173305=CARTESIAN_POINT('Ctrl Pts',(7.42818677473528,-3.30131294719024,
82.2837405262089));
#173306=CARTESIAN_POINT('Ctrl Pts',(7.52201990450268,-3.08155504962869,
82.2931140535145));
#173307=CARTESIAN_POINT('Ctrl Pts',(7.60605182487658,-2.85791238490469,
82.3024875808201));
#173308=CARTESIAN_POINT('Ctrl Pts',(7.68953804689525,-2.6357220425096,82.3118002369899));
#173309=CARTESIAN_POINT('Ctrl Pts',(7.76334990750397,-2.40969725823298,
82.3211128931597));
#173310=CARTESIAN_POINT('Ctrl Pts',(7.82717285021867,-2.18060834064712,
82.3304255493296));
#173311=CARTESIAN_POINT('Ctrl Pts',(7.86826770379246,-2.03310064007533,
82.3364218607719));
#173312=CARTESIAN_POINT('Ctrl Pts',(7.90522212284631,-1.88432309375023,
82.3424181722142));
#173313=CARTESIAN_POINT('Ctrl Pts',(7.93796211318074,-1.73448697089578,
82.3484144836565));
#173314=CARTESIAN_POINT('Ctrl Pts',(7.97744941790813,-1.55377144282478,
82.3556465620641));
#173315=CARTESIAN_POINT('Ctrl Pts',(8.01080108800573,-1.37152414881994,
82.3628786404717));
#173316=CARTESIAN_POINT('Ctrl Pts',(8.03789519688271,-1.18824592001399,
82.3701107188793));
#173317=CARTESIAN_POINT('Ctrl Pts',(8.06498051105206,-1.0050271830497,82.377340449765));
#173318=CARTESIAN_POINT('Ctrl Pts',(8.08581224529326,-0.820778563164806,
82.3845701806507));
#173319=CARTESIAN_POINT('Ctrl Pts',(8.10031960477432,-0.636010898498386,
82.3917999115364));
#173320=CARTESIAN_POINT('Ctrl Pts',(8.11482634946379,-0.451251063899659,
82.3990293360411));
#173321=CARTESIAN_POINT('Ctrl Pts',(8.1230092195426,-0.265972618188351,
82.4062587605459));
#173322=CARTESIAN_POINT('Ctrl Pts',(8.12484932289462,-0.0806910327038236,
82.4134881850507));
#173323=CARTESIAN_POINT('Ctrl Pts',(8.12512204060097,-0.0532308528357421,
82.4145596422963));
#173324=CARTESIAN_POINT('Ctrl Pts',(8.12525552921274,-0.0257706062289944,
82.4156310995419));
#173325=CARTESIAN_POINT('Ctrl Pts',(8.12524982465525,0.00168802838859176,
82.4167025567875));
#173326=CARTESIAN_POINT('',(8.13282513948647,-0.00629553435651024,78.4167025567875));
#173327=CARTESIAN_POINT('Ctrl Pts',(8.12524756561721,-0.00628966863631806,
78.4167025567875));
#173328=CARTESIAN_POINT('Ctrl Pts',(8.12540082558847,0.191697742214765,
78.4244812575649));
#173329=CARTESIAN_POINT('Ctrl Pts',(8.11831345843962,0.389951385898278,
78.4322599583424));
#173330=CARTESIAN_POINT('Ctrl Pts',(8.10395377987199,0.587895140478698,
78.4400386591199));
#173331=CARTESIAN_POINT('Ctrl Pts',(8.08960780372699,0.785650011375491,
78.447809937235));
#173332=CARTESIAN_POINT('Ctrl Pts',(8.06800336055709,0.983095236806884,
78.4555812153501));
#173333=CARTESIAN_POINT('Ctrl Pts',(8.03916077750979,1.17965315065415,78.4633524934652));
#173334=CARTESIAN_POINT('Ctrl Pts',(8.0103452233831,1.37602686642733,78.4711164889711));
#173335=CARTESIAN_POINT('Ctrl Pts',(7.97430509893499,1.57151458453547,78.4788804844771));
#173336=CARTESIAN_POINT('Ctrl Pts',(7.93111265724911,1.76554229077722,78.4866444799831));
#173337=CARTESIAN_POINT('Ctrl Pts',(7.88794352974413,1.95946526580065,78.4944042846818));
#173338=CARTESIAN_POINT('Ctrl Pts',(7.83762984852406,2.15192945898437,78.5021640893806));
#173339=CARTESIAN_POINT('Ctrl Pts',(7.78029529922124,2.34236901862535,78.5099238940794));
#173340=CARTESIAN_POINT('Ctrl Pts',(7.72298367973844,2.53273241572768,78.5176805953976));
#173341=CARTESIAN_POINT('Ctrl Pts',(7.65865688724969,2.72107245920761,78.5254372967158));
#173342=CARTESIAN_POINT('Ctrl Pts',(7.58748904662149,2.90683634384512,78.533193998034));
#173343=CARTESIAN_POINT('Ctrl Pts',(7.56546498063564,2.96432405201403,78.5355944376168));
#173344=CARTESIAN_POINT('Ctrl Pts',(7.54278611068146,3.02156515181753,78.5379948771995));
#173345=CARTESIAN_POINT('Ctrl Pts',(7.51945855803522,3.0785435771629,78.5403953167823));
#173346=CARTESIAN_POINT('Ctrl Pts',(7.44135943959123,3.26930361347196,78.548431831291));
#173347=CARTESIAN_POINT('Ctrl Pts',(7.35602819130241,3.45701454557353,78.5564683457996));
#173348=CARTESIAN_POINT('Ctrl Pts',(7.2637398644644,3.64112218195033,78.5645048603083));
#173349=CARTESIAN_POINT('Ctrl Pts',(7.17139578629167,3.82534103766342,78.5725462296716));
#173350=CARTESIAN_POINT('Ctrl Pts',(7.07208638634842,4.00595197258028,78.5805875990349));
#173351=CARTESIAN_POINT('Ctrl Pts',(6.96613217110615,4.18242634569694,78.5886289683981));
#173352=CARTESIAN_POINT('Ctrl Pts',(6.86010099407507,4.35902890421334,78.5966761787576));
#173353=CARTESIAN_POINT('Ctrl Pts',(6.74741553463572,4.53148863584257,78.6047233891171));
#173354=CARTESIAN_POINT('Ctrl Pts',(6.62843934565627,4.69930626831832,78.6127705994766));
#173355=CARTESIAN_POINT('Ctrl Pts',(6.5092877942703,4.86737125200056,78.6208296708496));
#173356=CARTESIAN_POINT('Ctrl Pts',(6.38382716446754,5.03078020351362,78.6288887422225));
#173357=CARTESIAN_POINT('Ctrl Pts',(6.25246208877077,5.18906594590821,78.6369478135954));
#173358=CARTESIAN_POINT('Ctrl Pts',(6.12099069287306,5.34747979672011,78.6450134075702));
#173359=CARTESIAN_POINT('Ctrl Pts',(5.98360552502437,5.50076192906777,78.653079001545));
#173360=CARTESIAN_POINT('Ctrl Pts',(5.84074836040636,5.64848175644662,78.6611445955198));
#173361=CARTESIAN_POINT('Ctrl Pts',(5.69766687740148,5.79643353770386,78.6692228543199));
#173362=CARTESIAN_POINT('Ctrl Pts',(5.54909645081852,5.93880533756818,78.6773011131199));
#173363=CARTESIAN_POINT('Ctrl Pts',(5.39551354793556,6.0752054382172,78.68537937192));
#173364=CARTESIAN_POINT('Ctrl Pts',(5.30879775500807,6.15221949812321,78.6899405086362));
#173365=CARTESIAN_POINT('Ctrl Pts',(5.22048458220785,6.22733057093386,78.6945016453524));
#173366=CARTESIAN_POINT('Ctrl Pts',(5.13066389792672,6.30047423048546,78.6990627820686));
#173367=CARTESIAN_POINT('Ctrl Pts',(4.97142564232424,6.43014668676428,78.7071489758008));
#173368=CARTESIAN_POINT('Ctrl Pts',(4.80713777818068,6.55388546943611,78.715235169533));
#173369=CARTESIAN_POINT('Ctrl Pts',(4.63826970675071,6.67129235530408,78.7233213632651));
#173370=CARTESIAN_POINT('Ctrl Pts',(4.46955225762668,6.7885945198015,78.7314003444962));
#173371=CARTESIAN_POINT('Ctrl Pts',(4.2962630058349,6.89957586860656,78.7394793257273));
#173372=CARTESIAN_POINT('Ctrl Pts',(4.11890376208171,7.00387887967868,78.7475583069584));
#173373=CARTESIAN_POINT('Ctrl Pts',(3.94167849500881,7.10810310054585,78.7556311853495));
#173374=CARTESIAN_POINT('Ctrl Pts',(3.76038963880158,7.2056588834096,78.7637040637406));
#173375=CARTESIAN_POINT('Ctrl Pts',(3.57556779496498,7.29623207594915,78.7717769421317));
#173376=CARTESIAN_POINT('Ctrl Pts',(3.39086036410816,7.38674919963541,78.7798448230504));
#173377=CARTESIAN_POINT('Ctrl Pts',(3.2026245909936,7.47029221426978,78.787912703969));
#173378=CARTESIAN_POINT('Ctrl Pts',(3.01141602940937,7.54659267883966,78.7959805848877));
#173379=CARTESIAN_POINT('Ctrl Pts',(2.82029979482945,7.62285630095193,78.8040445701478));
#173380=CARTESIAN_POINT('Ctrl Pts',(2.62621392846526,7.69188423081303,78.8121085554078));
#173381=CARTESIAN_POINT('Ctrl Pts',(2.42973490766022,7.75345573541227,78.8201725406679));
#173382=CARTESIAN_POINT('Ctrl Pts',(2.23052545764217,7.81588288675769,78.8283485895001));
#173383=CARTESIAN_POINT('Ctrl Pts',(2.02885614711122,7.87064469852979,78.8365246383323));
#173384=CARTESIAN_POINT('Ctrl Pts',(1.82534601807279,7.91756272326312,78.8447006871646));
#173385=CARTESIAN_POINT('Ctrl Pts',(1.62472036367283,7.9638157498803,78.8527608518115));
#173386=CARTESIAN_POINT('Ctrl Pts',(1.42230604679981,8.00244580329221,78.8608210164585));
#173387=CARTESIAN_POINT('Ctrl Pts',(1.2187090032898,8.03333280325173,78.8688811811054));
#173388=CARTESIAN_POINT('Ctrl Pts',(1.01512179656751,8.06421831090637,78.8769409563257));
#173389=CARTESIAN_POINT('Ctrl Pts',(0.810352290366901,8.087361463868,78.8850007315459));
#173390=CARTESIAN_POINT('Ctrl Pts',(0.605014417715229,8.10269369511502,
78.8930605067662));
#173391=CARTESIAN_POINT('Ctrl Pts',(0.399661041792254,8.11802708396505,
78.9011208905097));
#173392=CARTESIAN_POINT('Ctrl Pts',(0.193739529759944,8.1255483518748,78.9091812742532));
#173393=CARTESIAN_POINT('Ctrl Pts',(-0.0121326807149723,8.12524094169266,
78.9172416579968));
#173394=CARTESIAN_POINT('Ctrl Pts',(-0.223180078303388,8.12492580387595,
78.9255046625505));
#173395=CARTESIAN_POINT('Ctrl Pts',(-0.434175313038718,8.11638322957722,
78.9337676671043));
#173396=CARTESIAN_POINT('Ctrl Pts',(-0.644454750237635,8.09965219237197,
78.942030671658));
#173397=CARTESIAN_POINT('Ctrl Pts',(-0.849746511114368,8.08331800328096,
78.9500976837138));
#173398=CARTESIAN_POINT('Ctrl Pts',(-1.05435572752898,8.05917945067946,
78.9581646957695));
#173399=CARTESIAN_POINT('Ctrl Pts',(-1.25767116318497,8.02732525862712,
78.9662317078253));
#173400=CARTESIAN_POINT('Ctrl Pts',(-1.46839608946059,7.99431019388232,
78.974592708628));
#173401=CARTESIAN_POINT('Ctrl Pts',(-1.67773079525698,7.95300662129811,
78.9829537094307));
#173402=CARTESIAN_POINT('Ctrl Pts',(-1.88500718646095,7.90357105804019,
78.9913147102334));
#173403=CARTESIAN_POINT('Ctrl Pts',(-2.09228357766491,7.85413549478228,
78.9996757110361));
#173404=CARTESIAN_POINT('Ctrl Pts',(-2.29750129769483,7.79656806586894,
79.0080367118388));
#173405=CARTESIAN_POINT('Ctrl Pts',(-2.50001029116285,7.73108246667825,
79.0163977126415));
#173406=CARTESIAN_POINT('Ctrl Pts',(-2.68356041499135,7.67172762206325,
79.0239759574709));
#173407=CARTESIAN_POINT('Ctrl Pts',(-2.86525302554172,7.60574864884786,
79.0315542023004));
#173408=CARTESIAN_POINT('Ctrl Pts',(-3.04455396470433,7.53328472304765,
79.0391324471298));
#173409=CARTESIAN_POINT('Ctrl Pts',(-3.2237214813245,7.46087471955963,79.046705052788));
#173410=CARTESIAN_POINT('Ctrl Pts',(-3.40050052857907,7.38198950015648,
79.0542776584463));
#173411=CARTESIAN_POINT('Ctrl Pts',(-3.57437149736831,7.29681820804801,
79.0618502641045));
#173412=CARTESIAN_POINT('Ctrl Pts',(-3.74814610182904,7.21169412033732,
79.0694186728053));
#173413=CARTESIAN_POINT('Ctrl Pts',(-3.91901550605132,7.1202910535607,79.0769870815061));
#173414=CARTESIAN_POINT('Ctrl Pts',(-4.08647956659481,7.02284645384641,
79.0845554902068));
#173415=CARTESIAN_POINT('Ctrl Pts',(-4.25390316648401,6.92542539752555,
79.0921220703196));
#173416=CARTESIAN_POINT('Ctrl Pts',(-4.41792273901014,6.82196589129611,
79.0996886504324));
#173417=CARTESIAN_POINT('Ctrl Pts',(-4.57806215562732,6.71275163116534,
79.1072552305452));
#173418=CARTESIAN_POINT('Ctrl Pts',(-4.73817316423684,6.60355674514998,
79.114820468381));
#173419=CARTESIAN_POINT('Ctrl Pts',(-4.8944050849753,6.48860934697962,79.1223857062167));
#173420=CARTESIAN_POINT('Ctrl Pts',(-5.04631047429778,6.36823666013541,
79.1299509440525));
#173421=CARTESIAN_POINT('Ctrl Pts',(-5.19826868841348,6.24782211393176,
79.1375188126844));
#173422=CARTESIAN_POINT('Ctrl Pts',(-5.3458970747568,6.12197873603854,79.1450866813164));
#173423=CARTESIAN_POINT('Ctrl Pts',(-5.48878064983627,5.99107457310314,
79.1526545499483));
#173424=CARTESIAN_POINT('Ctrl Pts',(-5.62982038864289,5.86185965852084,
79.1601247592749));
#173425=CARTESIAN_POINT('Ctrl Pts',(-5.76623681665148,5.72771405851611,
79.1675949686015));
#173426=CARTESIAN_POINT('Ctrl Pts',(-5.89766614671137,5.58902689065231,
79.1750651779281));
#173427=CARTESIAN_POINT('Ctrl Pts',(-6.06139121157169,5.41626054128839,
79.1843710193712));
#173428=CARTESIAN_POINT('Ctrl Pts',(-6.21729831841948,5.23653277495086,
79.1936768608144));
#173429=CARTESIAN_POINT('Ctrl Pts',(-6.36489829365976,5.05052049534175,
79.2029827022575));
#173430=CARTESIAN_POINT('Ctrl Pts',(-6.51329070339016,4.86350955332969,
79.2123385048859));
#173431=CARTESIAN_POINT('Ctrl Pts',(-6.65328655720012,4.6701465054957,79.2216943075144));
#173432=CARTESIAN_POINT('Ctrl Pts',(-6.78443609563551,4.47114240734267,
79.2310501101429));
#173433=CARTESIAN_POINT('Ctrl Pts',(-6.91622229362762,4.27117225271375,
79.2404513300959));
#173434=CARTESIAN_POINT('Ctrl Pts',(-7.0390760764616,4.06550619474868,79.2498525500489));
#173435=CARTESIAN_POINT('Ctrl Pts',(-7.15258868013727,3.85488816118862,
79.259253770002));
#173436=CARTESIAN_POINT('Ctrl Pts',(-7.26622413813402,3.64404217641712,
79.2686651648647));
#173437=CARTESIAN_POINT('Ctrl Pts',(-7.37049818697081,3.42823353373309,
79.2780765597275));
#173438=CARTESIAN_POINT('Ctrl Pts',(-7.46504826856119,3.20823033938519,
79.2874879545903));
#173439=CARTESIAN_POINT('Ctrl Pts',(-7.55948744132022,2.9884852124738,79.296888309729));
#173440=CARTESIAN_POINT('Ctrl Pts',(-7.64422543575287,2.76455540382908,
79.3062886648678));
#173441=CARTESIAN_POINT('Ctrl Pts',(-7.71894840877369,2.53722742874779,
79.3156890200065));
#173442=CARTESIAN_POINT('Ctrl Pts',(-7.76675770782843,2.39177830239757,
79.3217035610758));
#173443=CARTESIAN_POINT('Ctrl Pts',(-7.81046810678153,2.2449384901348,79.327718102145));
#173444=CARTESIAN_POINT('Ctrl Pts',(-7.85000767910977,2.09691845344962,
79.3337326432142));
#173445=CARTESIAN_POINT('Ctrl Pts',(-7.9009055229794,1.90637767940598,79.3414749417335));
#173446=CARTESIAN_POINT('Ctrl Pts',(-7.94491300363429,1.71379089693561,
79.3492172402528));
#173447=CARTESIAN_POINT('Ctrl Pts',(-7.98186570632461,1.51970635607644,
79.356959538772));
#173448=CARTESIAN_POINT('Ctrl Pts',(-8.01879539082733,1.32574271231126,
79.3646970145404));
#173449=CARTESIAN_POINT('Ctrl Pts',(-8.04867898148121,1.1302835133879,79.3724344903088));
#173450=CARTESIAN_POINT('Ctrl Pts',(-8.07140237329596,0.933890406232127,
79.3801719660772));
#173451=CARTESIAN_POINT('Ctrl Pts',(-8.09411564909524,0.737584729497141,
79.3879059972707));
#173452=CARTESIAN_POINT('Ctrl Pts',(-8.10967503397298,0.540346322752834,
79.3956400284643));
#173453=CARTESIAN_POINT('Ctrl Pts',(-8.118017811087,0.342745359376757,79.4033740596578));
#173454=CARTESIAN_POINT('Ctrl Pts',(-8.12635952058831,0.1451696827003,79.4111071011389));
#173455=CARTESIAN_POINT('Ctrl Pts',(-8.12748643921373,-0.0527681057730007,
79.41884014262));
#173456=CARTESIAN_POINT('Ctrl Pts',(-8.12138783143314,-0.250494019788233,
79.4265731841011));
#173457=CARTESIAN_POINT('Ctrl Pts',(-8.1152898328989,-0.448200181132632,
79.4343054530572));
#173458=CARTESIAN_POINT('Ctrl Pts',(-8.10196776025479,-0.645694157064347,
79.4420377220132));
#173459=CARTESIAN_POINT('Ctrl Pts',(-8.08146299138581,-0.842403395862962,
79.4497699909693));
#173460=CARTESIAN_POINT('Ctrl Pts',(-8.06095033526488,-1.03918829975874,
79.4575052341775));
#173461=CARTESIAN_POINT('Ctrl Pts',(-8.03324949958436,-1.23518751166042,
79.4652404773857));
#173462=CARTESIAN_POINT('Ctrl Pts',(-7.99845367769798,-1.42983437090443,
79.472975720594));
#173463=CARTESIAN_POINT('Ctrl Pts',(-7.96932778711885,-1.5927637922132,
79.4794505165629));
#173464=CARTESIAN_POINT('Ctrl Pts',(-7.93523169286402,-1.75474569545111,
79.4859253125318));
#173465=CARTESIAN_POINT('Ctrl Pts',(-7.89624744735514,-1.91545394427466,
79.4924001085008));
#173466=CARTESIAN_POINT('Ctrl Pts',(-7.8455869558458,-2.12429622834947,
79.5008141830052));
#173467=CARTESIAN_POINT('Ctrl Pts',(-7.78664655913359,-2.33108810577066,
79.5092282575096));
#173468=CARTESIAN_POINT('Ctrl Pts',(-7.71961898120049,-2.53518645223365,
79.517642332014));
#173469=CARTESIAN_POINT('Ctrl Pts',(-7.65257268430924,-2.73934179774873,
79.5260587563379));
#173470=CARTESIAN_POINT('Ctrl Pts',(-7.57743477981321,-2.94080185974847,
79.5344751806617));
#173471=CARTESIAN_POINT('Ctrl Pts',(-7.49444727281426,-3.13894052787032,
79.5428916049856));
#173472=CARTESIAN_POINT('Ctrl Pts',(-7.41143918549133,-3.33712833300244,
79.5513101165241));
#173473=CARTESIAN_POINT('Ctrl Pts',(-7.32057771134345,-3.53199285640188,
79.5597286280626));
#173474=CARTESIAN_POINT('Ctrl Pts',(-7.2221526656362,-3.72292874451606,
79.5681471396011));
#173475=CARTESIAN_POINT('Ctrl Pts',(-7.12368981528036,-3.91393797030665,
79.5765688846547));
#173476=CARTESIAN_POINT('Ctrl Pts',(-7.01765770776236,-4.10101531008313,
79.5849906297083));
#173477=CARTESIAN_POINT('Ctrl Pts',(-6.90439238921444,-4.2835794959657,
79.593412374762));
#173478=CARTESIAN_POINT('Ctrl Pts',(-6.79111479301389,-4.46616347130972,
79.6018350327098));
#173479=CARTESIAN_POINT('Ctrl Pts',(-6.67060256204162,-4.64423309330062,
79.6102576906577));
#173480=CARTESIAN_POINT('Ctrl Pts',(-6.54323571841143,-4.81723508828507,
79.6186803486056));
#173481=CARTESIAN_POINT('Ctrl Pts',(-6.41584465327461,-4.99026998326805,
79.6271046083005));
#173482=CARTESIAN_POINT('Ctrl Pts',(-6.28159652782727,-5.15823511346599,
79.6355288679954));
#173483=CARTESIAN_POINT('Ctrl Pts',(-6.14091318052228,-5.32060831783244,
79.6439531276903));
#173484=CARTESIAN_POINT('Ctrl Pts',(-6.1013099343659,-5.36631739502537,
79.6463246097227));
#173485=CARTESIAN_POINT('Ctrl Pts',(-6.06119696865709,-5.41158353727088,
79.648696091755));
#173486=CARTESIAN_POINT('Ctrl Pts',(-6.0205842605687,-5.45639557985786,
79.6510675737873));
#173487=CARTESIAN_POINT('Ctrl Pts',(-5.87631386073357,-5.61558346970216,
79.6594918990075));
#173488=CARTESIAN_POINT('Ctrl Pts',(-5.7257193113277,-5.76905470810939,
79.6679162242276));
#173489=CARTESIAN_POINT('Ctrl Pts',(-5.56926842808729,-5.91632797758966,
79.6763405494478));
#173490=CARTESIAN_POINT('Ctrl Pts',(-5.4128445814735,-6.06357579644723,
79.6847634188414));
#173491=CARTESIAN_POINT('Ctrl Pts',(-5.25056661446976,-6.20462760484973,
79.6931862882351));
#173492=CARTESIAN_POINT('Ctrl Pts',(-5.08293824413027,-6.33903986175019,
79.7016091576288));
#173493=CARTESIAN_POINT('Ctrl Pts',(-4.91534412893088,-6.47342465127934,
79.7100303057949));
#173494=CARTESIAN_POINT('Ctrl Pts',(-4.74240199955845,-6.60117243374322,
79.718451453961));
#173495=CARTESIAN_POINT('Ctrl Pts',(-4.56464845453428,-6.72188009778647,
79.7268726021272));
#173496=CARTESIAN_POINT('Ctrl Pts',(-4.3869447811558,-6.84255389533297,
79.7352913876033));
#173497=CARTESIAN_POINT('Ctrl Pts',(-4.20443260646361,-6.95619137133587,
79.7437101730795));
#173498=CARTESIAN_POINT('Ctrl Pts',(-4.01767812023707,-7.06243230655475,
79.7521289585557));
#173499=CARTESIAN_POINT('Ctrl Pts',(-3.83097580262665,-7.16864356407927,
79.7605453923004));
#173500=CARTESIAN_POINT('Ctrl Pts',(-3.64003376881004,-7.26746227575448,
79.7689618260452));
#173501=CARTESIAN_POINT('Ctrl Pts',(-3.44544446140553,-7.3585732330303,
79.7773782597899));
#173502=CARTESIAN_POINT('Ctrl Pts',(-3.25092577860616,-7.44965112232582,
79.7857916388586));
#173503=CARTESIAN_POINT('Ctrl Pts',(-3.05276270453897,-7.53302673188149,
79.7942050179272));
#173504=CARTESIAN_POINT('Ctrl Pts',(-2.85157029193125,-7.60843179851638,
79.8026183969959));
#173505=CARTESIAN_POINT('Ctrl Pts',(-2.7948426134089,-7.62969281091529,
79.8049906110218));
#173506=CARTESIAN_POINT('Ctrl Pts',(-2.73787423246226,-7.65032045579075,
79.8073628250477));
#173507=CARTESIAN_POINT('Ctrl Pts',(-2.68067922986042,-7.67030940895444,
79.8097350390736));
#173508=CARTESIAN_POINT('Ctrl Pts',(-2.49418091383159,-7.73548828708402,
79.8174702239842));
#173509=CARTESIAN_POINT('Ctrl Pts',(-2.30518888622517,-7.79390142900383,
79.8252054088949));
#173510=CARTESIAN_POINT('Ctrl Pts',(-2.1142442949359,-7.84535905002639,
79.8329405938055));
#173511=CARTESIAN_POINT('Ctrl Pts',(-1.92335874843246,-7.89680075908103,
79.8406733868059));
#173512=CARTESIAN_POINT('Ctrl Pts',(-1.73052218134344,-7.94129113859473,
79.8484061798062));
#173513=CARTESIAN_POINT('Ctrl Pts',(-1.53629109203656,-7.97869019595504,
79.8561389728066));
#173514=CARTESIAN_POINT('Ctrl Pts',(-1.34208555454068,-8.01608433333242,
79.8638707485297));
#173515=CARTESIAN_POINT('Ctrl Pts',(-1.14648620721852,-8.04638894070733,
79.8716025242528));
#173516=CARTESIAN_POINT('Ctrl Pts',(-0.9500600678587,-8.06951506783154,
79.8793342999759));
#173517=CARTESIAN_POINT('Ctrl Pts',(-0.753563641862759,-8.0926494701155,
79.8870688423395));
#173518=CARTESIAN_POINT('Ctrl Pts',(-0.556240183493173,-8.10860021463751,
79.8948033847031));
#173519=CARTESIAN_POINT('Ctrl Pts',(-0.358662835275036,-8.11733013577078,
79.9025379270666));
#173520=CARTESIAN_POINT('Ctrl Pts',(-0.161052118446,-8.12606153129039,79.9102737757082));
#173521=CARTESIAN_POINT('Ctrl Pts',(0.0368122202687993,-8.12756966549348,
79.9180096243497));
#173522=CARTESIAN_POINT('Ctrl Pts',(0.234356526461537,-8.12186952499268,
79.9257454729913));
#173523=CARTESIAN_POINT('Ctrl Pts',(0.43206247235047,-8.11616472037883,
79.9334876514544));
#173524=CARTESIAN_POINT('Ctrl Pts',(0.629447509354175,-8.10323987465981,
79.9412298299176));
#173525=CARTESIAN_POINT('Ctrl Pts',(0.825941656388813,-8.08316200151535,
79.9489720083808));
#173526=CARTESIAN_POINT('Ctrl Pts',(0.99032169283829,-8.06636556473023,
79.9554488403739));
#173527=CARTESIAN_POINT('Ctrl Pts',(1.15407823778847,-8.04456408943727,
79.961925672367));
#173528=CARTESIAN_POINT('Ctrl Pts',(1.3168829979073,-8.01782431413427,79.9684025043601));
#173529=CARTESIAN_POINT('Ctrl Pts',(1.5531163559003,-7.97902430050325,79.9778005328316));
#173530=CARTESIAN_POINT('Ctrl Pts',(1.78748001050274,-7.92980496059317,
79.9871985613031));
#173531=CARTESIAN_POINT('Ctrl Pts',(2.01915084346335,-7.87036958686447,
79.9965965897746));
#173532=CARTESIAN_POINT('Ctrl Pts',(2.25115132463096,-7.81084964157304,
80.0060079908541));
#173533=CARTESIAN_POINT('Ctrl Pts',(2.48045128352638,-7.741084594051,80.0154193919336));
#173534=CARTESIAN_POINT('Ctrl Pts',(2.70624020151537,-7.66132831395457,
80.0248307930131));
#173535=CARTESIAN_POINT('Ctrl Pts',(2.93168915618036,-7.58169212039885,
80.0342280236399));
#173536=CARTESIAN_POINT('Ctrl Pts',(3.1536376025266,-7.49209477633976,80.0436252542666));
#173537=CARTESIAN_POINT('Ctrl Pts',(3.37129519995937,-7.3928381719899,80.0530224848934));
#173538=CARTESIAN_POINT('Ctrl Pts',(3.58840378373652,-7.29383192982284,
80.0623960121989));
#173539=CARTESIAN_POINT('Ctrl Pts',(3.80124309432122,-7.18521509110907,
80.0717695395045));
#173540=CARTESIAN_POINT('Ctrl Pts',(4.00904576453681,-7.06733610495139,
80.0811430668101));
#173541=CARTESIAN_POINT('Ctrl Pts',(4.21549897641626,-6.95022261800679,
80.0904557229798));
#173542=CARTESIAN_POINT('Ctrl Pts',(4.41698070153578,-6.82396689213371,
80.0997683791496));
#173543=CARTESIAN_POINT('Ctrl Pts',(4.61275590322929,-6.68895885319407,
80.1090810353193));
#173544=CARTESIAN_POINT('Ctrl Pts',(4.73881328800171,-6.60202874067335,
80.1150773467617));
#173545=CARTESIAN_POINT('Ctrl Pts',(4.86250514511262,-6.51147095877212,
80.121073658204));
#173546=CARTESIAN_POINT('Ctrl Pts',(4.98363930632188,-6.41740031687159,
80.1270699696464));
#173547=CARTESIAN_POINT('Ctrl Pts',(5.13651694433033,-6.29867825369696,
80.1346376278604));
#173548=CARTESIAN_POINT('Ctrl Pts',(5.28525813442047,-6.17440558564283,
80.1422052860744));
#173549=CARTESIAN_POINT('Ctrl Pts',(5.4294233883266,-6.04491929084187,80.1497729442884));
#173550=CARTESIAN_POINT('Ctrl Pts',(5.57354872546522,-5.91546884846848,
80.1573385071538));
#173551=CARTESIAN_POINT('Ctrl Pts',(5.71310037418531,-5.7808078971073,80.1649040700192));
#173552=CARTESIAN_POINT('Ctrl Pts',(5.84767217900044,-5.64131346846142,
80.1724696328847));
#173553=CARTESIAN_POINT('Ctrl Pts',(5.98223219405122,-5.50183126084836,
80.1800345329352));
#173554=CARTESIAN_POINT('Ctrl Pts',(6.11181297891524,-5.35751668399247,
80.1875994329857));
#173555=CARTESIAN_POINT('Ctrl Pts',(6.23604554107561,-5.20878331015324,
80.1951643330362));
#173556=CARTESIAN_POINT('Ctrl Pts',(6.36033907581099,-5.0599769388918,80.202732945893));
#173557=CARTESIAN_POINT('Ctrl Pts',(6.47927890533027,-4.90674771849094,
80.2103015587498));
#173558=CARTESIAN_POINT('Ctrl Pts',(6.59253627508182,-4.74954240156148,
80.2178701716066));
#173559=CARTESIAN_POINT('Ctrl Pts',(6.70581883128138,-4.59230212493312,
80.2254404675898));
#173560=CARTESIAN_POINT('Ctrl Pts',(6.81341620483991,-4.43108429539835,
80.233010763573));
#173561=CARTESIAN_POINT('Ctrl Pts',(6.91504341334367,-4.26636404378158,
80.2405810595562));
#173562=CARTESIAN_POINT('Ctrl Pts',(7.01677359918164,-4.10147688359129,
80.2481590264074));
#173563=CARTESIAN_POINT('Ctrl Pts',(7.11252135029389,-3.93308052975495,
80.2557369932586));
#173564=CARTESIAN_POINT('Ctrl Pts',(7.20204760538713,-3.7616748732762,80.2633149601098));
#173565=CARTESIAN_POINT('Ctrl Pts',(7.29034746383407,-3.59261725785024,
80.2707891183842));
#173566=CARTESIAN_POINT('Ctrl Pts',(7.37259510796375,-3.42063259496863,
80.2782632766586));
#173567=CARTESIAN_POINT('Ctrl Pts',(7.44860772744934,-3.24621787393913,
80.2857374349329));
#173568=CARTESIAN_POINT('Ctrl Pts',(7.54044114432775,-3.03550154953896,
80.2947672183724));
#173569=CARTESIAN_POINT('Ctrl Pts',(7.62332796704879,-2.82088908368092,
80.3037970018119));
#173570=CARTESIAN_POINT('Ctrl Pts',(7.69698348445964,-2.60310061320257,
80.3128267852514));
#173571=CARTESIAN_POINT('Ctrl Pts',(7.77051202053852,-2.38568760774083,
80.3218410014399));
#173572=CARTESIAN_POINT('Ctrl Pts',(7.83484100401659,-2.16510967085444,
80.3308552176283));
#173573=CARTESIAN_POINT('Ctrl Pts',(7.88973559610182,-1.94210189900115,
80.3398694338168));
#173574=CARTESIAN_POINT('Ctrl Pts',(7.94453711375102,-1.71947223948653,
80.3488683662942));
#173575=CARTESIAN_POINT('Ctrl Pts',(7.98993614758686,-1.49442110824226,
80.3578672987715));
#173576=CARTESIAN_POINT('Ctrl Pts',(8.02574813021303,-1.26769653816758,
80.3668662312489));
#173577=CARTESIAN_POINT('Ctrl Pts',(8.06141949001058,-1.04186224693322,
80.3758298276391));
#173578=CARTESIAN_POINT('Ctrl Pts',(8.08757889480169,-0.814367769798356,
80.3847934240293));
#173579=CARTESIAN_POINT('Ctrl Pts',(8.10409343111378,-0.585966912272722,
80.3937570204194));
#173580=CARTESIAN_POINT('Ctrl Pts',(8.11818505523042,-0.391075637619651,
80.4014055325349));
#173581=CARTESIAN_POINT('Ctrl Pts',(8.12525506186471,-0.195524715374751,
80.4090540446503));
#173582=CARTESIAN_POINT('Ctrl Pts',(8.12524999728007,0.000210238465518916,
80.4167025567657));
#173583=CARTESIAN_POINT('',(8.12952934429449,0.00742862902765984,76.4167025567875));
#173584=CARTESIAN_POINT('Ctrl Pts',(8.12952934429449,0.00742862902765984,
76.4167025567875));
#173585=CARTESIAN_POINT('Ctrl Pts',(8.13195251875862,0.526615112398015,
76.4370411272112));
#173586=CARTESIAN_POINT('Ctrl Pts',(7.83647938259965,3.73996568278205,76.5631580078259));
#173587=CARTESIAN_POINT('Ctrl Pts',(4.57239175033108,7.70877801686287,76.742164043536));
#173588=CARTESIAN_POINT('Ctrl Pts',(-0.99660367399542,8.39788261494146,
76.953720663918));
#173589=CARTESIAN_POINT('Ctrl Pts',(-4.87682214009191,6.92632775896648,
77.1123881292042));
#173590=CARTESIAN_POINT('Ctrl Pts',(-7.60342709026179,3.73828686763939,
77.2710555944908));
#173591=CARTESIAN_POINT('Ctrl Pts',(-8.45799212068,-0.346168247782079,77.4297230597773));
#173592=CARTESIAN_POINT('Ctrl Pts',(-7.27250765093393,-4.34712832670027,
77.5883905250636));
#173593=CARTESIAN_POINT('Ctrl Pts',(-4.29449854831541,-7.30169108010175,
77.7470579903501));
#173594=CARTESIAN_POINT('Ctrl Pts',(-0.307003826939667,-8.45123659280709,
77.9057254556364));
#173595=CARTESIAN_POINT('Ctrl Pts',(5.18705264259522,-7.30934400029921,
78.1172820760186));
#173596=CARTESIAN_POINT('Ctrl Pts',(7.9738707902656,-3.29181374846791,78.2876077764021));
#173597=CARTESIAN_POINT('Ctrl Pts',(8.1337744979333,-0.303304450377095,
78.4050443216903));
#173598=CARTESIAN_POINT('Ctrl Pts',(8.13282513948647,-0.00629553435651024,
78.4167025567875));
#173599=CARTESIAN_POINT('',(8.12524972840108,-0.00210085977713058,74.4167026551268));
#173600=CARTESIAN_POINT('Ctrl Pts',(8.12524972905207,-0.0020983420275516,
74.4167027534661));
#173601=CARTESIAN_POINT('Ctrl Pts',(8.12530621810546,0.21663990926585,74.4252463237542));
#173602=CARTESIAN_POINT('Ctrl Pts',(8.11652544175775,0.435225171804719,
74.4337898940423));
#173603=CARTESIAN_POINT('Ctrl Pts',(8.09897060024819,0.652964607628494,
74.4423334643304));
#173604=CARTESIAN_POINT('Ctrl Pts',(8.08139157394798,0.871004016691488,
74.4508888048448));
#173605=CARTESIAN_POINT('Ctrl Pts',(8.05501434439019,1.08819503484192,74.4594441453593));
#173606=CARTESIAN_POINT('Ctrl Pts',(8.01995378981406,1.30385151445515,74.4679994858738));
#173607=CARTESIAN_POINT('Ctrl Pts',(7.98385330648025,1.52590456644559,74.4768085857695));
#173608=CARTESIAN_POINT('Ctrl Pts',(7.93854656671959,1.74633038105455,74.4856176856651));
#173609=CARTESIAN_POINT('Ctrl Pts',(7.88421476674799,1.96439432759641,74.4944267855608));
#173610=CARTESIAN_POINT('Ctrl Pts',(7.83129931122844,2.17677369050512,74.5030062460966));
#173611=CARTESIAN_POINT('Ctrl Pts',(7.76982352019064,2.38691256644583,74.5115857066323));
#173612=CARTESIAN_POINT('Ctrl Pts',(7.70000508393201,2.59414904543306,74.5201651671681));
#173613=CARTESIAN_POINT('Ctrl Pts',(7.62738348873214,2.80970591685749,74.5290890867437));
#173614=CARTESIAN_POINT('Ctrl Pts',(7.54573566105335,3.02212226378135,74.5380130063193));
#173615=CARTESIAN_POINT('Ctrl Pts',(7.45536184516827,3.23067598500828,74.5469369258949));
#173616=CARTESIAN_POINT('Ctrl Pts',(7.36498802928315,3.43922970623527,74.5558608454704));
#173617=CARTESIAN_POINT('Ctrl Pts',(7.26588836458347,3.64392055211116,74.564784765046));
#173618=CARTESIAN_POINT('Ctrl Pts',(7.15841748436445,3.84405341820913,74.5737086846216));
#173619=CARTESIAN_POINT('Ctrl Pts',(7.06715258272108,4.01400742158951,74.581286929451));
#173620=CARTESIAN_POINT('Ctrl Pts',(6.96970326757686,4.18094771215279,74.5888651742805));
#173621=CARTESIAN_POINT('Ctrl Pts',(6.86630212036858,4.34437368953476,74.59644341911));
#173622=CARTESIAN_POINT('Ctrl Pts',(6.76297791667258,4.50767805735015,74.6040160247682));
#173623=CARTESIAN_POINT('Ctrl Pts',(6.65371088678339,4.66747300585524,74.6115886304264));
#173624=CARTESIAN_POINT('Ctrl Pts',(6.53878016623349,4.82328119646486,74.6191612360847));
#173625=CARTESIAN_POINT('Ctrl Pts',(6.42391314361848,4.97900303366146,74.6267296447855));
#173626=CARTESIAN_POINT('Ctrl Pts',(6.30338889389159,5.13074221496769,74.6342980534863));
#173627=CARTESIAN_POINT('Ctrl Pts',(6.17753058885142,5.27804920271733,74.6418664621871));
#173628=CARTESIAN_POINT('Ctrl Pts',(6.05170269218276,5.42532059992243,74.6494330422999));
#173629=CARTESIAN_POINT('Ctrl Pts',(5.92054353767196,5.56816165070676,74.6569996224128));
#173630=CARTESIAN_POINT('Ctrl Pts',(5.78441749887008,5.7061547263692,74.6645662025256));
#173631=CARTESIAN_POINT('Ctrl Pts',(5.64831560821166,5.8441233226843,74.6721314403613));
#173632=CARTESIAN_POINT('Ctrl Pts',(5.5072488475105,5.9772453960949,74.6796966781971));
#173633=CARTESIAN_POINT('Ctrl Pts',(5.36161927736592,6.10513933396103,74.6872619160328));
#173634=CARTESIAN_POINT('Ctrl Pts',(5.21593906483148,6.2330777466866,74.6948297846648));
#173635=CARTESIAN_POINT('Ctrl Pts',(5.06569314741027,6.35578414632546,74.7023976532968));
#173636=CARTESIAN_POINT('Ctrl Pts',(4.91131793613364,6.47291616605005,74.7099655219288));
#173637=CARTESIAN_POINT('Ctrl Pts',(4.75893485456602,6.5885366595753,74.7174357312551));
#173638=CARTESIAN_POINT('Ctrl Pts',(4.60252871783985,6.69872560740381,74.7249059405815));
#173639=CARTESIAN_POINT('Ctrl Pts',(4.44254749923095,6.80319478477405,74.7323761499079));
#173640=CARTESIAN_POINT('Ctrl Pts',(4.24325457593737,6.93333485954801,74.7416819913511));
#173641=CARTESIAN_POINT('Ctrl Pts',(4.03851277875083,7.05453672605251,74.7509878327943));
#173642=CARTESIAN_POINT('Ctrl Pts',(3.82907566883466,7.1664403356784,74.7602936742375));
#173643=CARTESIAN_POINT('Ctrl Pts',(3.61851413333113,7.27894473320685,74.7696494768659));
#173644=CARTESIAN_POINT('Ctrl Pts',(3.40320679896718,7.38205079083557,74.7790052794943));
#173645=CARTESIAN_POINT('Ctrl Pts',(3.18393376850058,7.47544335275853,74.7883610821227));
#173646=CARTESIAN_POINT('Ctrl Pts',(2.96359628693466,7.5692892846878,74.7977623020757));
#173647=CARTESIAN_POINT('Ctrl Pts',(2.73925456139049,7.65332719003012,74.8071635220286));
#173648=CARTESIAN_POINT('Ctrl Pts',(2.5117136941655,7.72728813239428,74.8165647419815));
#173649=CARTESIAN_POINT('Ctrl Pts',(2.28392656020113,7.80132912244544,74.8259761368442));
#173650=CARTESIAN_POINT('Ctrl Pts',(2.052933397635,7.8652713335794,74.8353875317069));
#173651=CARTESIAN_POINT('Ctrl Pts',(1.81955482203533,7.91889561821015,74.8447989265696));
#173652=CARTESIAN_POINT('Ctrl Pts',(1.58645000341915,7.97245700065563,74.8541992817083));
#173653=CARTESIAN_POINT('Ctrl Pts',(1.35096540119324,8.01572464461132,74.8635996368469));
#173654=CARTESIAN_POINT('Ctrl Pts',(1.11393101868102,8.04853062664983,74.8729999919856));
#173655=CARTESIAN_POINT('Ctrl Pts',(0.962271532682516,8.0695205704753,74.8790145330552));
#173656=CARTESIAN_POINT('Ctrl Pts',(0.809977857814596,8.08622883310838,
74.8850290741248));
#173657=CARTESIAN_POINT('Ctrl Pts',(0.657269933840611,8.09862233942102,
74.8910436151944));
#173658=CARTESIAN_POINT('Ctrl Pts',(0.460694614131297,8.11457604635598,
74.8987859137137));
#173659=CARTESIAN_POINT('Ctrl Pts',(0.263340261760429,8.123384379695,74.906528212233));
#173660=CARTESIAN_POINT('Ctrl Pts',(0.06577570720757,8.12498376114324,74.9142705107522));
#173661=CARTESIAN_POINT('Ctrl Pts',(-0.131665782517973,8.12658214632167,
74.9220079865206));
#173662=CARTESIAN_POINT('Ctrl Pts',(-0.329316861931104,8.12098051789449,
74.929745462289));
#173663=CARTESIAN_POINT('Ctrl Pts',(-0.526604529520342,8.10816719314474,
74.9374829380574));
#173664=CARTESIAN_POINT('Ctrl Pts',(-0.723804368448676,8.09535957263981,
74.945216969251));
#173665=CARTESIAN_POINT('Ctrl Pts',(-0.920640765975811,8.07534667275536,
74.9529510004445));
#173666=CARTESIAN_POINT('Ctrl Pts',(-1.11654153437862,8.0481688951281,74.9606850316381));
#173667=CARTESIAN_POINT('Ctrl Pts',(-1.3124172336526,8.02099459540046,74.9684180731192));
#173668=CARTESIAN_POINT('Ctrl Pts',(-1.50735719151998,7.98665728510766,
74.9761511146004));
#173669=CARTESIAN_POINT('Ctrl Pts',(-1.70079477764788,7.94524918972499,
74.9838841560815));
#173670=CARTESIAN_POINT('Ctrl Pts',(-1.89421303950434,7.90384523098036,
74.9916164250375));
#173671=CARTESIAN_POINT('Ctrl Pts',(-2.08612888376544,7.85537197165063,
74.9993486939936));
#173672=CARTESIAN_POINT('Ctrl Pts',(-2.2759864237333,7.79997265132909,75.0070809629496));
#173673=CARTESIAN_POINT('Ctrl Pts',(-2.46591699326275,7.74455202140838,
75.0148162061578));
#173674=CARTESIAN_POINT('Ctrl Pts',(-2.65378733713659,7.68220010679154,
75.0225514493661));
#173675=CARTESIAN_POINT('Ctrl Pts',(-2.83905664342013,7.61311007000109,
75.0302866925743));
#173676=CARTESIAN_POINT('Ctrl Pts',(-2.9941365711183,7.55527815965902,75.0367614885431));
#173677=CARTESIAN_POINT('Ctrl Pts',(-3.14739425040532,7.4927260665029,75.0432362845119));
#173678=CARTESIAN_POINT('Ctrl Pts',(-3.2985235105468,7.42559291995393,75.0497110804807));
#173679=CARTESIAN_POINT('Ctrl Pts',(-3.49491778470703,7.33835259616598,
75.0581251549851));
#173680=CARTESIAN_POINT('Ctrl Pts',(-3.68781206003829,7.24333339033684,
75.0665392294895));
#173681=CARTESIAN_POINT('Ctrl Pts',(-3.876608120588,7.14084007956285,75.0749533039939));
#173682=CARTESIAN_POINT('Ctrl Pts',(-4.06545690668342,7.03831814522687,
75.0833697283178));
#173683=CARTESIAN_POINT('Ctrl Pts',(-4.25020496110848,6.92831806495576,
75.0917861526417));
#173684=CARTESIAN_POINT('Ctrl Pts',(-4.43027963191671,6.811190053546,75.1002025769656));
#173685=CARTESIAN_POINT('Ctrl Pts',(-4.61039895998918,6.69403299520513,
75.1086210885042));
#173686=CARTESIAN_POINT('Ctrl Pts',(-4.78584236942369,6.56974462064712,
75.1170396000427));
#173687=CARTESIAN_POINT('Ctrl Pts',(-4.95606619123124,6.43871846493032,
75.1254581115812));
#173688=CARTESIAN_POINT('Ctrl Pts',(-5.12635539529663,6.30764198261525,
75.1338798566348));
#173689=CARTESIAN_POINT('Ctrl Pts',(-5.29142079539575,6.16982270757484,
75.1423016016885));
#173690=CARTESIAN_POINT('Ctrl Pts',(-5.45075069773424,6.02569534524022,
75.1507233467421));
#173691=CARTESIAN_POINT('Ctrl Pts',(-5.6100978709981,5.88155235989397,75.1591460046898));
#173692=CARTESIAN_POINT('Ctrl Pts',(-5.76370811147268,5.73110010132149,
75.1675686626375));
#173693=CARTESIAN_POINT('Ctrl Pts',(-5.9111051421337,5.57481152696129,75.1759913205852));
#173694=CARTESIAN_POINT('Ctrl Pts',(-6.05853020346894,5.4184932310111,75.1844155802801));
#173695=CARTESIAN_POINT('Ctrl Pts',(-6.19973951345155,5.25633659401228,
75.192839839975));
#173696=CARTESIAN_POINT('Ctrl Pts',(-6.33429489305838,5.08885014224967,
75.20126409967));
#173697=CARTESIAN_POINT('Ctrl Pts',(-6.37217307780808,5.04170165378735,
75.2036355817024));
#173698=CARTESIAN_POINT('Ctrl Pts',(-6.40952420877964,4.99413100456796,
75.2060070637348));
#173699=CARTESIAN_POINT('Ctrl Pts',(-6.44633908841539,4.94615000982258,
75.2083785457672));
#173700=CARTESIAN_POINT('Ctrl Pts',(-6.57711828671848,4.77570490478156,
75.2168028709873));
#173701=CARTESIAN_POINT('Ctrl Pts',(-6.70114073565114,4.60006159722525,
75.2252271962074));
#173702=CARTESIAN_POINT('Ctrl Pts',(-6.81801667296907,4.41976653338339,
75.2336515214275));
#173703=CARTESIAN_POINT('Ctrl Pts',(-6.93487241269567,4.2395026267335,75.2420743908212));
#173704=CARTESIAN_POINT('Ctrl Pts',(-7.04458396399692,4.05458879074625,
75.2504972602149));
#173705=CARTESIAN_POINT('Ctrl Pts',(-7.14680515950424,3.86560002775552,
75.2589201296086));
#173706=CARTESIAN_POINT('Ctrl Pts',(-7.24900546593935,3.6766498849345,75.2673412777748));
#173707=CARTESIAN_POINT('Ctrl Pts',(-7.34371834772962,3.48362671000325,
75.2757624259411));
#173708=CARTESIAN_POINT('Ctrl Pts',(-7.43064330195706,3.28713061522974,
75.2841835741073));
#173709=CARTESIAN_POINT('Ctrl Pts',(-7.51754386797469,3.09068965063179,
75.2926023595834));
#173710=CARTESIAN_POINT('Ctrl Pts',(-7.59666076382036,2.8907779534883,75.3010211450596));
#173711=CARTESIAN_POINT('Ctrl Pts',(-7.66774098444616,2.68801706801587,
75.3094399305357));
#173712=CARTESIAN_POINT('Ctrl Pts',(-7.73880134928791,2.48531282244016,
75.3178563642805));
#173713=CARTESIAN_POINT('Ctrl Pts',(-7.80182943402933,2.27976122651153,
75.3262727980252));
#173714=CARTESIAN_POINT('Ctrl Pts',(-7.85662121798895,2.07200159255388,
75.33468923177));
#173715=CARTESIAN_POINT('Ctrl Pts',(-7.91139311571642,1.86431736326486,
75.3431026108386));
#173716=CARTESIAN_POINT('Ctrl Pts',(-7.95793461498048,1.65442695129161,
75.3515159899072));
#173717=CARTESIAN_POINT('Ctrl Pts',(-7.99609193054374,1.44298350676414,
75.3599293689758));
#173718=CARTESIAN_POINT('Ctrl Pts',(-8.00685066593836,1.38336547449382,
75.3623015830018));
#173719=CARTESIAN_POINT('Ctrl Pts',(-8.01694316794742,1.32362405197726,
75.3646737970278));
#173720=CARTESIAN_POINT('Ctrl Pts',(-8.0263667199826,1.26377404580717,75.3670460110538));
#173721=CARTESIAN_POINT('Ctrl Pts',(-8.05709451971255,1.06861844030229,
75.3747811959645));
#173722=CARTESIAN_POINT('Ctrl Pts',(-8.08071938514722,0.872221018269008,
75.3825163808752));
#173723=CARTESIAN_POINT('Ctrl Pts',(-8.09715150632828,0.675148166009207,
75.3902515657859));
#173724=CARTESIAN_POINT('Ctrl Pts',(-8.11357854629147,0.478136253544567,
75.3979843587863));
#173725=CARTESIAN_POINT('Ctrl Pts',(-8.12281724193719,0.280449678433193,
75.4057171517867));
#173726=CARTESIAN_POINT('Ctrl Pts',(-8.12482951941,0.0826610127197688,75.4134499447871));
#173727=CARTESIAN_POINT('Ctrl Pts',(-8.12684153216034,-0.115101633170138,
75.4211817205102));
#173728=CARTESIAN_POINT('Ctrl Pts',(-8.12162901749148,-0.312965989718375,
75.4289134962333));
#173729=CARTESIAN_POINT('Ctrl Pts',(-8.10920600260128,-0.510358275993785,
75.4366452719565));
#173730=CARTESIAN_POINT('Ctrl Pts',(-8.09677854241716,-0.707821194618828,
75.4443798143201));
#173731=CARTESIAN_POINT('Ctrl Pts',(-8.07713544515563,-0.904811352251254,
75.4521143566838));
#173732=CARTESIAN_POINT('Ctrl Pts',(-8.0503427823418,-1.10075821563922,
75.4598488990474));
#173733=CARTESIAN_POINT('Ctrl Pts',(-8.02354559454599,-1.29673817226739,
75.4675847476889));
#173734=CARTESIAN_POINT('Ctrl Pts',(-7.98959649066467,-1.49167413444426,
75.4753205963305));
#173735=CARTESIAN_POINT('Ctrl Pts',(-7.94861294309523,-1.68500440455182,
75.483056444972));
#173736=CARTESIAN_POINT('Ctrl Pts',(-7.90759586093138,-1.8784928662406,
75.4907986234353));
#173737=CARTESIAN_POINT('Ctrl Pts',(-7.85953291581635,-2.07037266657687,
75.4985408018985));
#173738=CARTESIAN_POINT('Ctrl Pts',(-7.80459210839859,-2.2600950387146,
75.5062829803617));
#173739=CARTESIAN_POINT('Ctrl Pts',(-7.75863057691466,-2.41881004837783,
75.5127598123545));
#173740=CARTESIAN_POINT('Ctrl Pts',(-7.70785656533052,-2.5760153602587,
75.5192366443472));
#173741=CARTESIAN_POINT('Ctrl Pts',(-7.65239452295687,-2.73139993913738,
75.52571347634));
#173742=CARTESIAN_POINT('Ctrl Pts',(-7.57191785567642,-2.95686644775757,
75.5351115048115));
#173743=CARTESIAN_POINT('Ctrl Pts',(-7.48152510899277,-3.17862761966625,
75.5445095332829));
#173744=CARTESIAN_POINT('Ctrl Pts',(-7.38156369033432,-3.39591004710636,
75.5539075617544));
#173745=CARTESIAN_POINT('Ctrl Pts',(-7.28146003494381,-3.61350164925435,
75.5633189628337));
#173746=CARTESIAN_POINT('Ctrl Pts',(-7.17176048805549,-3.82660172531268,
75.5727303639131));
#173747=CARTESIAN_POINT('Ctrl Pts',(-7.05285996042488,-4.03445832065911,
75.5821417649925));
#173748=CARTESIAN_POINT('Ctrl Pts',(-6.93413845760611,-4.24200195282017,
75.5915389956191));
#173749=CARTESIAN_POINT('Ctrl Pts',(-6.80624368370452,-4.44431785359218,
75.6009362262457));
#173750=CARTESIAN_POINT('Ctrl Pts',(-6.66961418037348,-4.64068251957199,
75.6103334568724));
#173751=CARTESIAN_POINT('Ctrl Pts',(-6.53332930761853,-4.83655188061171,
75.6197069841778));
#173752=CARTESIAN_POINT('Ctrl Pts',(-6.3883537188307,-5.02649994834641,
75.6290805114832));
#173753=CARTESIAN_POINT('Ctrl Pts',(-6.23516764793593,-5.20983415903358,
75.6384540387886));
#173754=CARTESIAN_POINT('Ctrl Pts',(-6.08297635838614,-5.3919778081271,
75.6477666949584));
#173755=CARTESIAN_POINT('Ctrl Pts',(-5.92268088945874,-5.56759317338444,
75.6570793511282));
#173756=CARTESIAN_POINT('Ctrl Pts',(-5.75479649173734,-5.73602692646988,
75.6663920072979));
#173757=CARTESIAN_POINT('Ctrl Pts',(-5.6466976725834,-5.84447946917977,
75.6723883187408));
#173758=CARTESIAN_POINT('Ctrl Pts',(-5.53545343527797,-5.94995509218792,
75.6783846301837));
#173759=CARTESIAN_POINT('Ctrl Pts',(-5.42121114614727,-6.05228529329117,
75.6843809416266));
#173760=CARTESIAN_POINT('Ctrl Pts',(-5.27703141066134,-6.18143135154644,
75.6919485998406));
#173761=CARTESIAN_POINT('Ctrl Pts',(-5.12813153575109,-6.30551384389175,
75.6995162580546));
#173762=CARTESIAN_POINT('Ctrl Pts',(-4.97492175438106,-6.42416073119953,
75.7070839162686));
#173763=CARTESIAN_POINT('Ctrl Pts',(-4.82175439404575,-6.54277476731674,
75.7146494791341));
#173764=CARTESIAN_POINT('Ctrl Pts',(-4.6642797920895,-6.65595596814462,
75.7222150419996));
#173765=CARTESIAN_POINT('Ctrl Pts',(-4.50294161846877,-6.76337226116986,
75.729780604865));
#173766=CARTESIAN_POINT('Ctrl Pts',(-4.34161757959845,-6.87077914351156,
75.7373455049156));
#173767=CARTESIAN_POINT('Ctrl Pts',(-4.1764309492916,-6.97242192027236,
75.7449104049662));
#173768=CARTESIAN_POINT('Ctrl Pts',(-4.00785469237258,-7.06801162473061,
75.7524753050168));
#173769=CARTESIAN_POINT('Ctrl Pts',(-3.83919569926737,-7.16364824402569,
75.7600439178736));
#173770=CARTESIAN_POINT('Ctrl Pts',(-3.66714407468579,-7.25322567148377,
75.7676125307304));
#173771=CARTESIAN_POINT('Ctrl Pts',(-3.49219822177283,-7.33650046972987,
75.7751811435872));
#173772=CARTESIAN_POINT('Ctrl Pts',(-3.317213463978,-7.419793786827,75.7827514395705));
#173773=CARTESIAN_POINT('Ctrl Pts',(-3.13933353261881,-7.49678153505065,
75.7903217355537));
#173774=CARTESIAN_POINT('Ctrl Pts',(-2.95907691176168,-7.56726842346556,
75.797892031537));
#173775=CARTESIAN_POINT('Ctrl Pts',(-2.77863763956001,-7.63782673519286,
75.8054699983882));
#173776=CARTESIAN_POINT('Ctrl Pts',(-2.59581721296777,-7.70187090314973,
75.8130479652394));
#173777=CARTESIAN_POINT('Ctrl Pts',(-2.41115025259095,-7.75925524918021,
75.8206259320907));
#173778=CARTESIAN_POINT('Ctrl Pts',(-2.22901299639221,-7.81585350212932,
75.8281000903647));
#173779=CARTESIAN_POINT('Ctrl Pts',(-2.04507981757291,-7.86597320841395,
75.8355742486388));
#173780=CARTESIAN_POINT('Ctrl Pts',(-1.85987240872072,-7.90952351193037,
75.8430484069129));
#173781=CARTESIAN_POINT('Ctrl Pts',(-1.65978049137863,-7.95657380967729,
75.8511232386318));
#173782=CARTESIAN_POINT('Ctrl Pts',(-1.45777415622232,-7.99605722870673,
75.8591980703507));
#173783=CARTESIAN_POINT('Ctrl Pts',(-1.25445250182052,-8.02782887729778,
75.8672729020696));
#173784=CARTESIAN_POINT('Ctrl Pts',(-1.05126536469937,-8.05957950581706,
75.8753423914928));
#173785=CARTESIAN_POINT('Ctrl Pts',(-0.846764955638771,-8.08362848922263,
75.883411880916));
#173786=CARTESIAN_POINT('Ctrl Pts',(-0.641560898076209,-8.09988192361837,
75.8914813703392));
#173787=CARTESIAN_POINT('Ctrl Pts',(-0.436464648012926,-8.11612681899135,
75.8995466203166));
#173788=CARTESIAN_POINT('Ctrl Pts',(-0.23066580179146,-8.12458430800815,
75.907611870294));
#173789=CARTESIAN_POINT('Ctrl Pts',(-0.0247800730888524,-8.12521221325805,
75.9156771202714));
#173790=CARTESIAN_POINT('Ctrl Pts',(0.181025508580555,-8.12583987407748,
75.9237392306147));
#173791=CARTESIAN_POINT('Ctrl Pts',(0.386917588946715,-8.11864402912757,
75.931801340958));
#173792=CARTESIAN_POINT('Ctrl Pts',(0.592278846543603,-8.10363457532711,
75.9398634513013));
#173793=CARTESIAN_POINT('Ctrl Pts',(0.797588086386284,-8.08862892340285,
75.947923519522));
#173794=CARTESIAN_POINT('Ctrl Pts',(1.00236645601473,-8.06581363366268,
75.9559835877426));
#173795=CARTESIAN_POINT('Ctrl Pts',(1.20599952194076,-8.03525063178359,
75.9640436559632));
#173796=CARTESIAN_POINT('Ctrl Pts',(1.41268331489412,-8.00422975055449,
75.9722244760267));
#173797=CARTESIAN_POINT('Ctrl Pts',(1.61818688104359,-7.96522718414051,
75.9804052960902));
#173798=CARTESIAN_POINT('Ctrl Pts',(1.82187530932127,-7.91836207304172,
75.9885861161536));
#173799=CARTESIAN_POINT('Ctrl Pts',(2.02257670567079,-7.87218422525166,
75.9966469668553));
#173800=CARTESIAN_POINT('Ctrl Pts',(2.22151552496948,-7.81837294701084,
76.004707817557));
#173801=CARTESIAN_POINT('Ctrl Pts',(2.41809634264528,-7.75709337575522,
76.0127686682588));
#173802=CARTESIAN_POINT('Ctrl Pts',(2.61470976146192,-7.69580364184001,
76.0208308557793));
#173803=CARTESIAN_POINT('Ctrl Pts',(2.80896409611744,-7.62704323885842,
76.0288930432998));
#173804=CARTESIAN_POINT('Ctrl Pts',(3.00028009424158,-7.55102687841844,
76.0369552308203));
#173805=CARTESIAN_POINT('Ctrl Pts',(3.19165152102717,-7.4749884942839,76.0450197541426));
#173806=CARTESIAN_POINT('Ctrl Pts',(3.38008261892044,-7.39169007678637,
76.053084277465));
#173807=CARTESIAN_POINT('Ctrl Pts',(3.56501453744225,-7.30139431275461,
76.0611488007874));
#173808=CARTESIAN_POINT('Ctrl Pts',(3.75464791193204,-7.20880299281188,
76.0694183455122));
#173809=CARTESIAN_POINT('Ctrl Pts',(3.94060151628308,-7.10885398988861,
76.0776878902371));
#173810=CARTESIAN_POINT('Ctrl Pts',(4.12230025877587,-7.00188032881142,
76.085957434962));
#173811=CARTESIAN_POINT('Ctrl Pts',(4.2997336832766,-6.8974178391106,76.0940328548546));
#173812=CARTESIAN_POINT('Ctrl Pts',(4.4731095158356,-6.78625699138805,76.1021082747472));
#173813=CARTESIAN_POINT('Ctrl Pts',(4.64192191238647,-6.66875164643326,
76.1101836946399));
#173814=CARTESIAN_POINT('Ctrl Pts',(4.81682142488792,-6.54700923906974,
76.1185503017809));
#173815=CARTESIAN_POINT('Ctrl Pts',(4.9868219806478,-6.41845651367071,76.1269169089218));
#173816=CARTESIAN_POINT('Ctrl Pts',(5.15139851814492,-6.28353251521422,
76.1352835160628));
#173817=CARTESIAN_POINT('Ctrl Pts',(5.31597505564203,-6.14860851675773,
76.1436501232038));
#173818=CARTESIAN_POINT('Ctrl Pts',(5.47512731906034,-6.00731352220343,
76.1520167303447));
#173819=CARTESIAN_POINT('Ctrl Pts',(5.62837241333278,-5.86012896951377,
76.1603833374857));
#173820=CARTESIAN_POINT('Ctrl Pts',(5.77633035840448,-5.71802246968975,
76.1684612861188));
#173821=CARTESIAN_POINT('Ctrl Pts',(5.91906960610025,-5.57014972641378,
76.1765392347518));
#173822=CARTESIAN_POINT('Ctrl Pts',(6.05612875466844,-5.41691721086616,
76.1846171833849));
#173823=CARTESIAN_POINT('Ctrl Pts',(6.19302017067409,-5.26387222079763,
76.1926852462494));
#173824=CARTESIAN_POINT('Ctrl Pts',(6.32424513502683,-5.10548076675019,
76.2007533091139));
#173825=CARTESIAN_POINT('Ctrl Pts',(6.44937754428596,-4.94218745635574,
76.2088213719783));
#173826=CARTESIAN_POINT('Ctrl Pts',(6.57437222227587,-4.7790738803325,76.2168805544533));
#173827=CARTESIAN_POINT('Ctrl Pts',(6.69328752288442,-4.61106945295417,
76.2249397369282));
#173828=CARTESIAN_POINT('Ctrl Pts',(6.80573585024926,-4.43865374850663,
76.2329989194032));
#173829=CARTESIAN_POINT('Ctrl Pts',(6.91803974166775,-4.2664595060054,76.2410477501399));
#173830=CARTESIAN_POINT('Ctrl Pts',(7.0238930595349,-4.0898655533672,76.2490965808766));
#173831=CARTESIAN_POINT('Ctrl Pts',(7.12294994496738,-3.90938251441187,
76.2571454116133));
#173832=CARTESIAN_POINT('Ctrl Pts',(7.22193190421692,-3.72903599201603,
76.2651881542507));
#173833=CARTESIAN_POINT('Ctrl Pts',(7.31412752666964,-3.54480652240982,
76.273230896888));
#173834=CARTESIAN_POINT('Ctrl Pts',(7.39923483838501,-3.3572326950823,76.2812736395253));
#173835=CARTESIAN_POINT('Ctrl Pts',(7.48427282699343,-3.16981165369326,
76.2893098310462));
#173836=CARTESIAN_POINT('Ctrl Pts',(7.56223389198272,-2.97905197520006,
76.2973460225671));
#173837=CARTESIAN_POINT('Ctrl Pts',(7.63286237412736,-2.78551602762053,
76.305382214088));
#173838=CARTESIAN_POINT('Ctrl Pts',(7.67290587273076,-2.67578895702119,
76.3099384103161));
#173839=CARTESIAN_POINT('Ctrl Pts',(7.7105932046514,-2.56516990756974,76.3144946065442));
#173840=CARTESIAN_POINT('Ctrl Pts',(7.74588456348531,-2.45376443279708,
76.3190508027724));
#173841=CARTESIAN_POINT('Ctrl Pts',(7.80498441965225,-2.26720183637626,
76.3266807311924));
#173842=CARTESIAN_POINT('Ctrl Pts',(7.85733735241861,-2.07851109462117,
76.3343106596125));
#173843=CARTESIAN_POINT('Ctrl Pts',(7.90280004174291,-1.88823702503904,
76.3419405880325));
#173844=CARTESIAN_POINT('Ctrl Pts',(7.94828568129213,-1.69786690234703,
76.3495743681511));
#173845=CARTESIAN_POINT('Ctrl Pts',(7.98687404736717,-1.5059122071846,76.3572081482697));
#173846=CARTESIAN_POINT('Ctrl Pts',(8.01847276254194,-1.31292883237172,
76.3648419283882));
#173847=CARTESIAN_POINT('Ctrl Pts',(8.05008105541181,-1.1198869635374,76.3724780223357));
#173848=CARTESIAN_POINT('Ctrl Pts',(8.0746954299414,-0.925816151661797,
76.3801141162831));
#173849=CARTESIAN_POINT('Ctrl Pts',(8.09227536083693,-0.731277681111288,
76.3877502102305));
#173850=CARTESIAN_POINT('Ctrl Pts',(8.10986970331353,-0.536579732861084,
76.3953925640539));
#173851=CARTESIAN_POINT('Ctrl Pts',(8.12041807074284,-0.341413720418515,
76.4030349178773));
#173852=CARTESIAN_POINT('Ctrl Pts',(8.12393203108951,-0.146341780561353,
76.4106772717006));
#173853=CARTESIAN_POINT('Ctrl Pts',(8.12485550804272,-0.0950764209942109,
76.4126857000629));
#173854=CARTESIAN_POINT('Ctrl Pts',(8.1252934320321,-0.0438175393908651,
76.4146941284252));
#173855=CARTESIAN_POINT('Ctrl Pts',(8.12524660770978,0.00742471553402487,
76.4167025567875));
#173856=CARTESIAN_POINT('',(8.12524906564331,-0.0038966347636782,72.4167025567875));
#173857=CARTESIAN_POINT('Ctrl Pts',(8.12524906564331,-0.0038966347636782,
72.4167025567875));
#173858=CARTESIAN_POINT('Ctrl Pts',(8.12533820018677,0.181966400879045,
72.4239655139928));
#173859=CARTESIAN_POINT('Ctrl Pts',(8.11904571743255,0.367994713859331,
72.4312284711981));
#173860=CARTESIAN_POINT('Ctrl Pts',(8.10636402924909,0.55366938491884,72.4384914284034));
#173861=CARTESIAN_POINT('Ctrl Pts',(8.0936840973464,0.739318341984484,72.4457533797653));
#173862=CARTESIAN_POINT('Ctrl Pts',(8.07461673634665,0.924613365706575,
72.4530153311273));
#173863=CARTESIAN_POINT('Ctrl Pts',(8.049206453849,1.10903698126604,72.4602772824892));
#173864=CARTESIAN_POINT('Ctrl Pts',(8.02379836453089,1.2934446790921,72.4675386070669));
#173865=CARTESIAN_POINT('Ctrl Pts',(7.99204850192037,1.47698073328401,72.4747999316447));
#173866=CARTESIAN_POINT('Ctrl Pts',(7.95405299875925,1.65913485149008,72.4820612562225));
#173867=CARTESIAN_POINT('Ctrl Pts',(7.91604481293383,1.8413497716158,72.4893250045855));
#173868=CARTESIAN_POINT('Ctrl Pts',(7.87178691239364,2.02218145539832,72.4965887529485));
#173869=CARTESIAN_POINT('Ctrl Pts',(7.82142608333776,2.20113188732154,72.5038525013116));
#173870=CARTESIAN_POINT('Ctrl Pts',(7.80483468765621,2.26008718013709,72.5062455461736));
#173871=CARTESIAN_POINT('Ctrl Pts',(7.78758129581107,2.3188384138625,72.5086385910357));
#173872=CARTESIAN_POINT('Ctrl Pts',(7.76967232571523,2.37736819056597,72.5110316358978));
#173873=CARTESIAN_POINT('Ctrl Pts',(7.70002965467141,2.60497312616041,72.5203374773411));
#173874=CARTESIAN_POINT('Ctrl Pts',(7.62047679462563,2.82920612644778,72.5296433187843));
#173875=CARTESIAN_POINT('Ctrl Pts',(7.53136166697491,3.04930795488435,72.5389491602275));
#173876=CARTESIAN_POINT('Ctrl Pts',(7.44176809818251,3.27059146563297,72.548304962856));
#173877=CARTESIAN_POINT('Ctrl Pts',(7.3425093773523,3.48769930448531,72.5576607654845));
#173878=CARTESIAN_POINT('Ctrl Pts',(7.23398256648911,3.69988969973858,72.567016568113));
#173879=CARTESIAN_POINT('Ctrl Pts',(7.1249289170865,3.91311016375572,72.5764177880661));
#173880=CARTESIAN_POINT('Ctrl Pts',(7.00651701668263,4.12136529862264,72.5858190080192));
#173881=CARTESIAN_POINT('Ctrl Pts',(6.87919273380317,4.32393280402109,72.5952202279722));
#173882=CARTESIAN_POINT('Ctrl Pts',(6.75173064826658,4.52671954757161,72.6046316228351));
#173883=CARTESIAN_POINT('Ctrl Pts',(6.61533691549991,4.7238063233347,72.6140430176979));
#173884=CARTESIAN_POINT('Ctrl Pts',(6.47050121367161,4.91449912059959,72.6234544125607));
#173885=CARTESIAN_POINT('Ctrl Pts',(6.32583540655121,5.10496823201438,72.6328547676995));
#173886=CARTESIAN_POINT('Ctrl Pts',(6.17274744932352,5.28905833020603,72.6422551228383));
#173887=CARTESIAN_POINT('Ctrl Pts',(6.01176704613544,5.46610872060737,72.6516554779771));
#173888=CARTESIAN_POINT('Ctrl Pts',(5.90876846448565,5.5793892114667,72.6576700190462));
#173889=CARTESIAN_POINT('Ctrl Pts',(5.80253978676833,5.68978847537497,72.6636845601153));
#173890=CARTESIAN_POINT('Ctrl Pts',(5.69322869546497,5.79714020734657,72.6696991011844));
#173891=CARTESIAN_POINT('Ctrl Pts',(5.55251652963046,5.93533016164763,72.6774413997037));
#173892=CARTESIAN_POINT('Ctrl Pts',(5.4066283645938,6.06853290350363,72.6851836982229));
#173893=CARTESIAN_POINT('Ctrl Pts',(5.25596022344466,6.19633518235316,72.6929259967422));
#173894=CARTESIAN_POINT('Ctrl Pts',(5.10538593490379,6.32405785195602,72.7006634725106));
#173895=CARTESIAN_POINT('Ctrl Pts',(4.95003786704904,6.4463865290839,72.708400948279));
#173896=CARTESIAN_POINT('Ctrl Pts',(4.79034849363571,6.56294513705715,72.7161384240473));
#173897=CARTESIAN_POINT('Ctrl Pts',(4.6307302108482,6.6794518553886,72.7238724552409));
#173898=CARTESIAN_POINT('Ctrl Pts',(4.46677475637333,6.7901934126344,72.7316064864344));
#173899=CARTESIAN_POINT('Ctrl Pts',(4.29894734816104,6.89483424458044,72.739340517628));
#173900=CARTESIAN_POINT('Ctrl Pts',(4.13114141657244,6.99946168579493,72.7470735591091));
#173901=CARTESIAN_POINT('Ctrl Pts',(3.95946481370844,7.09798976341856,72.7548066005902));
#173902=CARTESIAN_POINT('Ctrl Pts',(3.78441169260494,7.19012626477275,72.7625396420713));
#173903=CARTESIAN_POINT('Ctrl Pts',(3.60937605917799,7.28225356175902,72.7702719110273));
#173904=CARTESIAN_POINT('Ctrl Pts',(3.43096489380225,7.36799039292066,72.7780041799833));
#173905=CARTESIAN_POINT('Ctrl Pts',(3.2496967837625,7.44709059808618,72.7857364489393));
#173906=CARTESIAN_POINT('Ctrl Pts',(3.06835894812452,7.52622122950332,72.7934716921475));
#173907=CARTESIAN_POINT('Ctrl Pts',(2.8841622963857,7.59870999312656,72.8012069353557));
#173908=CARTESIAN_POINT('Ctrl Pts',(2.697645825484,7.66435871829788,72.8089421785639));
#173909=CARTESIAN_POINT('Ctrl Pts',(2.5415219569212,7.71931007401683,72.8154169745329));
#173910=CARTESIAN_POINT('Ctrl Pts',(2.38377314301183,7.76946974238227,72.8218917705019));
#173911=CARTESIAN_POINT('Ctrl Pts',(2.22472360236408,7.81474839361986,72.8283665664708));
#173912=CARTESIAN_POINT('Ctrl Pts',(2.01803682932689,7.87358854036697,72.8367806409753));
#173913=CARTESIAN_POINT('Ctrl Pts',(1.80905368549032,7.92421359863214,72.8451947154797));
#173914=CARTESIAN_POINT('Ctrl Pts',(1.59842875182824,7.96647431978719,72.8536087899841));
#173915=CARTESIAN_POINT('Ctrl Pts',(1.38774499641717,8.00874684319893,72.862025214308));
#173916=CARTESIAN_POINT('Ctrl Pts',(1.17541879473009,8.04265031426947,72.8704416386319));
#173917=CARTESIAN_POINT('Ctrl Pts',(0.962114210042332,8.06808675023606,
72.8788580629558));
#173918=CARTESIAN_POINT('Ctrl Pts',(0.748756727303346,8.09352949426159,
72.8872765744944));
#173919=CARTESIAN_POINT('Ctrl Pts',(0.534420639260289,8.11050097995341,
72.8956950860329));
#173920=CARTESIAN_POINT('Ctrl Pts',(0.31977550978621,8.11895505504501,72.9041135975714));
#173921=CARTESIAN_POINT('Ctrl Pts',(0.10504793601485,8.12741237731153,72.9125353426251));
#173922=CARTESIAN_POINT('Ctrl Pts',(-0.109988652598161,8.12734573973279,
72.9209570876787));
#173923=CARTESIAN_POINT('Ctrl Pts',(-0.324662866439217,8.11876108686883,
72.9293788327324));
#173924=CARTESIAN_POINT('Ctrl Pts',(-0.53936035037808,8.11017550345196,
72.9378014906801));
#173925=CARTESIAN_POINT('Ctrl Pts',(-0.753695117504446,8.09307007479076,
72.9462241486279));
#173926=CARTESIAN_POINT('Ctrl Pts',(-0.966998464671324,8.06750280643418,
72.9546468065757));
#173927=CARTESIAN_POINT('Ctrl Pts',(-1.18034237599743,8.0419306759188,72.9630710662706));
#173928=CARTESIAN_POINT('Ctrl Pts',(-1.39265421346462,8.00789352238933,
72.9714953259656));
#173929=CARTESIAN_POINT('Ctrl Pts',(-1.60327173810763,7.96550107000717,
72.9799195856606));
#173930=CARTESIAN_POINT('Ctrl Pts',(-1.6625618945651,7.95356732831775,72.9822910676927));
#173931=CARTESIAN_POINT('Ctrl Pts',(-1.72171783872473,7.94097177664898,
72.9846625497249));
#173932=CARTESIAN_POINT('Ctrl Pts',(-1.7807249388753,7.92771759427438,72.9870340317571));
#173933=CARTESIAN_POINT('Ctrl Pts',(-1.99033858773114,7.88063414968803,
72.9954583569772));
#173934=CARTESIAN_POINT('Ctrl Pts',(-2.19809465750639,7.82523058662881,
73.0038826821972));
#173935=CARTESIAN_POINT('Ctrl Pts',(-2.40334379003392,7.76167676403787,
73.0123070074173));
#173936=CARTESIAN_POINT('Ctrl Pts',(-2.6085574530005,7.69813392432494,73.0207298768109));
#173937=CARTESIAN_POINT('Ctrl Pts',(-2.81126479202046,7.62644371624108,
73.0291527462045));
#173938=CARTESIAN_POINT('Ctrl Pts',(-3.01083162655915,7.54682585455708,
73.0375756155981));
#173939=CARTESIAN_POINT('Ctrl Pts',(-3.21035767928003,7.46722426291683,
73.0459967637642));
#173940=CARTESIAN_POINT('Ctrl Pts',(-3.40674426409017,7.37969835050973,
73.0544179119303));
#173941=CARTESIAN_POINT('Ctrl Pts',(-3.59937617500349,7.2845163678392,73.0628390600964));
#173942=CARTESIAN_POINT('Ctrl Pts',(-3.79195403990344,7.18936109002087,
73.0712578455725));
#173943=CARTESIAN_POINT('Ctrl Pts',(-3.9807790984489,7.0865541489707,73.0796766310486));
#173944=CARTESIAN_POINT('Ctrl Pts',(-4.16525888331298,6.97641068153834,
73.0880954165248));
#173945=CARTESIAN_POINT('Ctrl Pts',(-4.34968713498416,6.86629798194626,
73.0965118502695));
#173946=CARTESIAN_POINT('Ctrl Pts',(-4.52977231006664,6.74885298302943,
73.1049282840143));
#173947=CARTESIAN_POINT('Ctrl Pts',(-4.70494816856911,6.62443584719319,
73.113344717759));
#173948=CARTESIAN_POINT('Ctrl Pts',(-4.88006044841937,6.50006386754385,
73.1217580968276));
#173949=CARTESIAN_POINT('Ctrl Pts',(-5.05026675490292,6.36872495698999,
73.1301714758962));
#173950=CARTESIAN_POINT('Ctrl Pts',(-5.21503055399626,6.23082208728395,
73.1385848549649));
#173951=CARTESIAN_POINT('Ctrl Pts',(-5.26148691737217,6.19193936024744,
73.1409570689911));
#173952=CARTESIAN_POINT('Ctrl Pts',(-5.30751079024305,6.15253505479862,
73.1433292830174));
#173953=CARTESIAN_POINT('Ctrl Pts',(-5.35309060059216,6.11261879920153,
73.1457014970437));
#173954=CARTESIAN_POINT('Ctrl Pts',(-5.50171473709118,5.98246207026925,
73.1534366819544));
#173955=CARTESIAN_POINT('Ctrl Pts',(-5.64568073970341,5.84680119993373,
73.1611718668651));
#173956=CARTESIAN_POINT('Ctrl Pts',(-5.78455678274856,5.70601352869563,
73.1689070517758));
#173957=CARTESIAN_POINT('Ctrl Pts',(-5.92338988188977,5.56526939248415,
73.1766398447763));
#173958=CARTESIAN_POINT('Ctrl Pts',(-6.05713590802872,5.41940186364829,
73.1843726377767));
#173959=CARTESIAN_POINT('Ctrl Pts',(-6.18539879614912,5.26882617810618,
73.1921054307771));
#173960=CARTESIAN_POINT('Ctrl Pts',(-6.31364481081703,5.11827030134675,
73.1998372065003));
#173961=CARTESIAN_POINT('Ctrl Pts',(-6.43640889579381,4.96300777096174,
73.2075689822235));
#173962=CARTESIAN_POINT('Ctrl Pts',(-6.55333421547803,4.80348813080087,
73.2153007579467));
#173963=CARTESIAN_POINT('Ctrl Pts',(-6.67030137423394,4.64391141015755,
73.2230353003103));
#173964=CARTESIAN_POINT('Ctrl Pts',(-6.78142538102213,4.48007481903832,
73.2307698426739));
#173965=CARTESIAN_POINT('Ctrl Pts',(-6.88639144130183,4.31245875106822,
73.2385043850375));
#173966=CARTESIAN_POINT('Ctrl Pts',(-6.9913752291787,4.14481437461323,73.2462402336791));
#173967=CARTESIAN_POINT('Ctrl Pts',(-7.09019881717135,3.97338955301307,
73.2539760823207));
#173968=CARTESIAN_POINT('Ctrl Pts',(-7.18259253779685,3.79869082691459,
73.2617119309623));
#173969=CARTESIAN_POINT('Ctrl Pts',(-7.27506185914825,3.62384915440786,
73.2694541094256));
#173970=CARTESIAN_POINT('Ctrl Pts',(-7.36109064292379,3.44572854124775,
73.2771962878888));
#173971=CARTESIAN_POINT('Ctrl Pts',(-7.44045630233157,3.2648579717339,73.2849384663521));
#173972=CARTESIAN_POINT('Ctrl Pts',(-7.50685079897228,3.11354806629623,
73.2914152983447));
#173973=CARTESIAN_POINT('Ctrl Pts',(-7.56858298382625,2.96031410241079,
73.2978921303373));
#173974=CARTESIAN_POINT('Ctrl Pts',(-7.62554913898165,2.80547462855686,
73.30436896233));
#173975=CARTESIAN_POINT('Ctrl Pts',(-7.70820830764052,2.58079907955007,
73.3137669908014));
#173976=CARTESIAN_POINT('Ctrl Pts',(-7.7808798634525,2.35261557665354,73.3231650192727));
#173977=CARTESIAN_POINT('Ctrl Pts',(-7.8433350493158,2.12174052765041,73.3325630477441));
#173978=CARTESIAN_POINT('Ctrl Pts',(-7.90587910368191,1.8905369627738,73.3419744488235));
#173979=CARTESIAN_POINT('Ctrl Pts',(-7.95817769973159,1.65663422688744,
73.3513858499029));
#173980=CARTESIAN_POINT('Ctrl Pts',(-8.00005229852206,1.42086268985145,
73.3607972509823));
#173981=CARTESIAN_POINT('Ctrl Pts',(-8.04186384803645,1.18544614665803,
73.3701944816089));
#173982=CARTESIAN_POINT('Ctrl Pts',(-8.07328276631883,0.948166462592412,
73.3795917122355));
#173983=CARTESIAN_POINT('Ctrl Pts',(-8.09418224276287,0.709860115404616,
73.3889889428621));
#173984=CARTESIAN_POINT('Ctrl Pts',(-8.11502900293129,0.472154865718613,
73.3983624701677));
#173985=CARTESIAN_POINT('Ctrl Pts',(-8.12540929805967,0.233428161608197,
73.4077359974733));
#173986=CARTESIAN_POINT('Ctrl Pts',(-8.12524815165165,-0.00548056397160565,
73.4171095247788));
#173987=CARTESIAN_POINT('Ctrl Pts',(-8.12508805171894,-0.242837830319122,
73.4264221809486));
#173988=CARTESIAN_POINT('Ctrl Pts',(-8.11452295540435,-0.480374717166226,
73.4357348371184));
#173989=CARTESIAN_POINT('Ctrl Pts',(-8.09352990955081,-0.717259482827784,
73.4450474932882));
#173990=CARTESIAN_POINT('Ctrl Pts',(-8.08001273048008,-0.869786839692345,
73.451043804731));
#173991=CARTESIAN_POINT('Ctrl Pts',(-8.06217322375856,-1.02204366016996,
73.4570401161738));
#173992=CARTESIAN_POINT('Ctrl Pts',(-8.04001658451643,-1.17380615230997,
73.4630364276166));
#173993=CARTESIAN_POINT('Ctrl Pts',(-8.0120537486039,-1.36533834358738,
73.4706040858306));
#173994=CARTESIAN_POINT('Ctrl Pts',(-7.97722263444777,-1.5560067236132,
73.4781717440446));
#173995=CARTESIAN_POINT('Ctrl Pts',(-7.93559986926388,-1.74526281042113,
73.4857394022586));
#173996=CARTESIAN_POINT('Ctrl Pts',(-7.89398862867558,-1.9344664956201,
73.4933049651241));
#173997=CARTESIAN_POINT('Ctrl Pts',(-7.84558955766252,-2.12225830696251,
73.5008705279896));
#173998=CARTESIAN_POINT('Ctrl Pts',(-7.79053056235515,-2.30809902723222,
73.5084360908551));
#173999=CARTESIAN_POINT('Ctrl Pts',(-7.73547639073627,-2.493923466098,73.5160009909057));
#174000=CARTESIAN_POINT('Ctrl Pts',(-7.67376356141738,-2.67779680184264,
73.5235658909563));
#174001=CARTESIAN_POINT('Ctrl Pts',(-7.60557009024882,-2.85919414605103,
73.531130791007));
#174002=CARTESIAN_POINT('Ctrl Pts',(-7.53734315014629,-3.04068051895429,
73.5386994038638));
#174003=CARTESIAN_POINT('Ctrl Pts',(-7.46262934039782,-3.21968812679239,
73.5462680167206));
#174004=CARTESIAN_POINT('Ctrl Pts',(-7.38165537816871,-3.39571074157575,
73.5538366295774));
#174005=CARTESIAN_POINT('Ctrl Pts',(-7.30066340875383,-3.57177250069438,
73.5614069255607));
#174006=CARTESIAN_POINT('Ctrl Pts',(-7.21340867773382,-3.74484761523026,
73.568977221544));
#174007=CARTESIAN_POINT('Ctrl Pts',(-7.12016416680368,-3.91445395940033,
73.5765475175272));
#174008=CARTESIAN_POINT('Ctrl Pts',(-7.02682517260175,-4.08423216314854,
73.5841254843785));
#174009=CARTESIAN_POINT('Ctrl Pts',(-6.92748445960888,-4.25053425745538,
73.5917034512297));
#174010=CARTESIAN_POINT('Ctrl Pts',(-6.8224591849423,-4.41290587167871,
73.5992814180809));
#174011=CARTESIAN_POINT('Ctrl Pts',(-6.71887262392489,-4.57305319981126,
73.6067555763549));
#174012=CARTESIAN_POINT('Ctrl Pts',(-6.60975649933532,-4.72937680833569,
73.6142297346289));
#174013=CARTESIAN_POINT('Ctrl Pts',(-6.49545316497986,-4.88147270237713,
73.6217038929028));
#174014=CARTESIAN_POINT('Ctrl Pts',(-6.37196364870327,-5.0457920416925,
73.6297787246217));
#174015=CARTESIAN_POINT('Ctrl Pts',(-6.24215632176443,-5.20552794152128,
73.6378535563406));
#174016=CARTESIAN_POINT('Ctrl Pts',(-6.10639835220765,-5.36018532577519,
73.6459283880594));
#174017=CARTESIAN_POINT('Ctrl Pts',(-5.97073019990481,-5.51474038895284,
73.6539978774826));
#174018=CARTESIAN_POINT('Ctrl Pts',(-5.82911946395495,-5.66422339926768,
73.6620673669059));
#174019=CARTESIAN_POINT('Ctrl Pts',(-5.68197406005973,-5.80817168679683,
73.6701368563291));
#174020=CARTESIAN_POINT('Ctrl Pts',(-5.53490596154673,-5.95204434860411,
73.6782021063065));
#174021=CARTESIAN_POINT('Ctrl Pts',(-5.38230921987001,-6.09038786546068,
73.6862673562839));
#174022=CARTESIAN_POINT('Ctrl Pts',(-5.22462956665833,-6.22277538190955,
73.6943326062613));
#174023=CARTESIAN_POINT('Ctrl Pts',(-5.06701129485761,-6.3551113626505,
73.7023947166046));
#174024=CARTESIAN_POINT('Ctrl Pts',(-4.90431430020517,-6.48149576387487,
73.7104568269478));
#174025=CARTESIAN_POINT('Ctrl Pts',(-4.73701891142311,-6.60154068345563,
73.7185189372911));
#174026=CARTESIAN_POINT('Ctrl Pts',(-4.56976589835752,-6.72155519580572,
73.7265790055118));
#174027=CARTESIAN_POINT('Ctrl Pts',(-4.39791707172538,-6.83523324513132,
73.7346390737324));
#174028=CARTESIAN_POINT('Ctrl Pts',(-4.2219838762333,-6.94222872796093,
73.742699141953));
#174029=CARTESIAN_POINT('Ctrl Pts',(-4.04341493908372,-7.05082716269777,
73.7508799620165));
#174030=CARTESIAN_POINT('Ctrl Pts',(-3.86063854733434,-7.15254100888551,
73.7590607820799));
#174031=CARTESIAN_POINT('Ctrl Pts',(-3.67421852464841,-7.24705497396221,
73.7672416021434));
#174032=CARTESIAN_POINT('Ctrl Pts',(-3.49053229771513,-7.34018291905796,
73.7753024528451));
#174033=CARTESIAN_POINT('Ctrl Pts',(-3.30330887018905,-7.4263205744407,
73.7833633035468));
#174034=CARTESIAN_POINT('Ctrl Pts',(-3.11311121644029,-7.50521326256447,
73.7914241542485));
#174035=CARTESIAN_POINT('Ctrl Pts',(-2.92288202013944,-7.58411903432348,
73.799486341769));
#174036=CARTESIAN_POINT('Ctrl Pts',(-2.72967790653201,-7.65577732090503,
73.8075485292895));
#174037=CARTESIAN_POINT('Ctrl Pts',(-2.5340811935733,-7.71998186959517,
73.81561071681));
#174038=CARTESIAN_POINT('Ctrl Pts',(-2.33842781173114,-7.78420501982534,
73.8236752401323));
#174039=CARTESIAN_POINT('Ctrl Pts',(-2.14038074897869,-7.84097002617608,
73.8317397634547));
#174040=CARTESIAN_POINT('Ctrl Pts',(-1.94053739483727,-7.89012054291556,
73.8398042867771));
#174041=CARTESIAN_POINT('Ctrl Pts',(-1.7356134967979,-7.94052059511733,
73.848073831502));
#174042=CARTESIAN_POINT('Ctrl Pts',(-1.52880110969277,-7.98291378675044,
73.8563433762269));
#174043=CARTESIAN_POINT('Ctrl Pts',(-1.32075515694156,-8.01718737325705,
73.8646129209518));
#174044=CARTESIAN_POINT('Ctrl Pts',(-1.11759301424641,-8.05065639863557,
73.8726883408444));
#174045=CARTESIAN_POINT('Ctrl Pts',(-0.91325489095522,-8.07638274216671,
73.880763760737));
#174046=CARTESIAN_POINT('Ctrl Pts',(-0.708355890209745,-8.09431402252872,
73.8888391806297));
#174047=CARTESIAN_POINT('Ctrl Pts',(-0.496068545944349,-8.11289187734247,
73.8972057877707));
#174048=CARTESIAN_POINT('Ctrl Pts',(-0.283179502971089,-8.12310204624144,
73.9055723949118));
#174049=CARTESIAN_POINT('Ctrl Pts',(-0.0703731950607855,-8.12494524141037,
73.9139390020528));
#174050=CARTESIAN_POINT('Ctrl Pts',(0.142433112849518,-8.12678843657929,
73.9223056091939));
#174051=CARTESIAN_POINT('Ctrl Pts',(0.355156311837234,-8.12026470677724,
73.9306722163349));
#174052=CARTESIAN_POINT('Ctrl Pts',(0.567117184088067,-8.10543432901729,
73.939038823476));
#174053=CARTESIAN_POINT('Ctrl Pts',(0.771765138676577,-8.09111561801125,
73.947116772109));
#174054=CARTESIAN_POINT('Ctrl Pts',(0.976100380386021,-8.06902602697114,
73.9551947207421));
#174055=CARTESIAN_POINT('Ctrl Pts',(1.17950822345358,-8.03918204255292,
73.9632726693752));
#174056=CARTESIAN_POINT('Ctrl Pts',(1.38266713663346,-8.00937458111031,
73.9713407322397));
#174057=CARTESIAN_POINT('Ctrl Pts',(1.5849006036307,-7.97183168814913,73.9794087951043));
#174058=CARTESIAN_POINT('Ctrl Pts',(1.78559660822796,-7.92662174669542,
73.9874768579689));
#174059=CARTESIAN_POINT('Ctrl Pts',(1.98607170989304,-7.88146156711242,
73.9955360404437));
#174060=CARTESIAN_POINT('Ctrl Pts',(2.18501241658971,-7.82865123142644,
74.0035952229185));
#174061=CARTESIAN_POINT('Ctrl Pts',(2.38181387656983,-7.76831064130931,
74.0116544053933));
#174062=CARTESIAN_POINT('Ctrl Pts',(2.57836255195641,-7.70804755657017,
74.01970323613));
#174063=CARTESIAN_POINT('Ctrl Pts',(2.77277716191924,-7.64027360548962,
74.0277520668668));
#174064=CARTESIAN_POINT('Ctrl Pts',(2.96446500835067,-7.56515926975529,
74.0358008976035));
#174065=CARTESIAN_POINT('Ctrl Pts',(3.15600786296069,-7.49010175016531,
74.043843640241));
#174066=CARTESIAN_POINT('Ctrl Pts',(3.34482777245157,-7.40771502761441,
74.0518863828785));
#174067=CARTESIAN_POINT('Ctrl Pts',(3.53034781734139,-7.31821917211373,
74.059929125516));
#174068=CARTESIAN_POINT('Ctrl Pts',(3.71571674917015,-7.2287962143567,74.0679653170369));
#174069=CARTESIAN_POINT('Ctrl Pts',(3.89779089454204,-7.13227581143776,
74.0760015085577));
#174070=CARTESIAN_POINT('Ctrl Pts',(4.076013660801,-7.02892596343592,74.0840377000786));
#174071=CARTESIAN_POINT('Ctrl Pts',(4.1770587756715,-6.97033077112463,74.0885938963064));
#174072=CARTESIAN_POINT('Ctrl Pts',(4.27686625954618,-6.90954117291963,
74.0931500925343));
#174073=CARTESIAN_POINT('Ctrl Pts',(4.37533792322839,-6.84661271141135,
74.0977062887621));
#174074=CARTESIAN_POINT('Ctrl Pts',(4.54902863238394,-6.73561540826113,
74.1057428032707));
#174075=CARTESIAN_POINT('Ctrl Pts',(4.71842442093203,-6.61804890458617,
74.1137793177793));
#174076=CARTESIAN_POINT('Ctrl Pts',(4.88302931101169,-6.49428304821253,
74.1218158322879));
#174077=CARTESIAN_POINT('Ctrl Pts',(5.04773363882793,-6.37044242494334,
74.1298572016511));
#174078=CARTESIAN_POINT('Ctrl Pts',(5.20764104170037,-6.24039516724635,
74.1378985710143));
#174079=CARTESIAN_POINT('Ctrl Pts',(5.36228881921625,-6.10455126784994,
74.1459399403775));
#174080=CARTESIAN_POINT('Ctrl Pts',(5.51704892798421,-5.96860869574351,
74.153987150737));
#174081=CARTESIAN_POINT('Ctrl Pts',(5.66654155224571,-5.82686128979284,
74.1620343610965));
#174082=CARTESIAN_POINT('Ctrl Pts',(5.81034059418364,-5.67975613403266,
74.170081571456));
#174083=CARTESIAN_POINT('Ctrl Pts',(5.95435158564125,-5.53243415577711,
74.1781406428289));
#174084=CARTESIAN_POINT('Ctrl Pts',(6.09265200113154,-5.37973887051835,
74.1861997142018));
#174085=CARTESIAN_POINT('Ctrl Pts',(6.22485467574036,-5.2221520303811,74.1942587855747));
#174086=CARTESIAN_POINT('Ctrl Pts',(6.35716434845941,-5.06443764748314,
74.2023243795494));
#174087=CARTESIAN_POINT('Ctrl Pts',(6.48336623842568,-4.90182405822823,
74.2103899735242));
#174088=CARTESIAN_POINT('Ctrl Pts',(6.60311583106907,-4.7348230045045,74.2184555674989));
#174089=CARTESIAN_POINT('Ctrl Pts',(6.72305345793257,-4.56755972097103,
74.226533826299));
#174090=CARTESIAN_POINT('Ctrl Pts',(6.83651836201009,-4.39589546553531,
74.2346120850991));
#174091=CARTESIAN_POINT('Ctrl Pts',(6.94321048164746,-4.22036915092043,
74.2426903438991));
#174092=CARTESIAN_POINT('Ctrl Pts',(7.0034508572392,-4.12126369538565,74.2472514806157));
#174093=CARTESIAN_POINT('Ctrl Pts',(7.06153295399646,-4.02092746171593,
74.2518126173322));
#174094=CARTESIAN_POINT('Ctrl Pts',(7.11740948051487,-3.91946040280763,
74.2563737540487));
#174095=CARTESIAN_POINT('Ctrl Pts',(7.22059852415721,-3.73207780366742,
74.2647969572259));
#174096=CARTESIAN_POINT('Ctrl Pts',(7.31644555401899,-3.54050601147677,
74.2732201604031));
#174097=CARTESIAN_POINT('Ctrl Pts',(7.40462551799961,-3.3453263668421,74.2816433635803));
#174098=CARTESIAN_POINT('Ctrl Pts',(7.4927044203584,-3.15037041442214,74.2900569130614));
#174099=CARTESIAN_POINT('Ctrl Pts',(7.57313368175876,-2.95181510309204,
74.2984704625426));
#174100=CARTESIAN_POINT('Ctrl Pts',(7.64563451223645,-2.75026552678081,
74.3068840120237));
#174101=CARTESIAN_POINT('Ctrl Pts',(7.71805116954088,-2.54894994871891,
74.3152877934076));
#174102=CARTESIAN_POINT('Ctrl Pts',(7.78255767350349,-2.34464729292043,
74.3236915747915));
#174103=CARTESIAN_POINT('Ctrl Pts',(7.8389232237723,-2.13798275350932,74.3320953561754));
#174104=CARTESIAN_POINT('Ctrl Pts',(7.89519516524345,-1.93166143116894,
74.3404851810226));
#174105=CARTESIAN_POINT('Ctrl Pts',(7.94335307174294,-1.7229863121671,74.3488750058699));
#174106=CARTESIAN_POINT('Ctrl Pts',(7.9832158263263,-1.51259797460968,74.3572648307171));
#174107=CARTESIAN_POINT('Ctrl Pts',(8.02303601866255,-1.30243427281829,
74.3656456975833));
#174108=CARTESIAN_POINT('Ctrl Pts',(8.05457867863643,-1.09056126298045,
74.3740265644495));
#174109=CARTESIAN_POINT('Ctrl Pts',(8.07771312413821,-0.877632181853677,
74.3824074313157));
#174110=CARTESIAN_POINT('Ctrl Pts',(8.10081321161226,-0.66501933148655,
74.3907758513716));
#174111=CARTESIAN_POINT('Ctrl Pts',(8.11552997917101,-0.45135380484218,
74.3991442714274));
#174112=CARTESIAN_POINT('Ctrl Pts',(8.12178415220492,-0.237296749857492,
74.4075126914832));
#174113=CARTESIAN_POINT('Ctrl Pts',(8.12407351337415,-0.158940441673543,
74.410575979918));
#174114=CARTESIAN_POINT('Ctrl Pts',(8.12522942505247,-0.0805317558266113,
74.4136392683528));
#174115=CARTESIAN_POINT('Ctrl Pts',(8.12524972775009,-0.00210337752670956,
74.4167025567875));
#174116=CARTESIAN_POINT('',(8.12524985409108,0.00153983533466129,68.4161556904274));
#174117=CARTESIAN_POINT('Ctrl Pts',(8.12524912703364,-0.00376644912560897,
72.4136256277805));
#174118=CARTESIAN_POINT('Ctrl Pts',(8.12504495497945,-0.444220773542676,
72.3949776375295));
#174119=CARTESIAN_POINT('Ctrl Pts',(8.08902685308007,-0.883951672119959,
72.3762872520971));
#174120=CARTESIAN_POINT('Ctrl Pts',(8.01504119253789,-1.33380636191999,
72.3581502401893));
#174121=CARTESIAN_POINT('Ctrl Pts',(8.01249875253361,-1.34899535716882,
72.3575391098091));
#174122=CARTESIAN_POINT('Ctrl Pts',(8.00830498159974,-1.37361953614454,
72.3565504825373));
#174123=CARTESIAN_POINT('Ctrl Pts',(8.00668012898813,-1.38305915325922,
72.3561720026502));
#174124=CARTESIAN_POINT('Ctrl Pts',(8.00380322905308,-1.39959758255951,
72.3555098130235));
#174125=CARTESIAN_POINT('Ctrl Pts',(8.00255842169075,-1.4066976328787,72.355225826995));
#174126=CARTESIAN_POINT('Ctrl Pts',(8.0000346105114,-1.42098100930207,72.3546551326423));
#174127=CARTESIAN_POINT('Ctrl Pts',(7.99875537571469,-1.42816428960903,
72.3543684335725));
#174128=CARTESIAN_POINT('Ctrl Pts',(7.99627075941841,-1.44200808584983,
72.3538165102144));
#174129=CARTESIAN_POINT('Ctrl Pts',(7.99506672788509,-1.44866883537331,
72.3535512324763));
#174130=CARTESIAN_POINT('Ctrl Pts',(7.99220071414338,-1.46441133131637,
72.3529249126987));
#174131=CARTESIAN_POINT('Ctrl Pts',(7.99053157101026,-1.47349177671526,
72.352564161535));
#174132=CARTESIAN_POINT('Ctrl Pts',(7.9855296022346,-1.50044495913771,72.3514949314562));
#174133=CARTESIAN_POINT('Ctrl Pts',(7.98215224871541,-1.51830945103964,
72.3507883069983));
#174134=CARTESIAN_POINT('Ctrl Pts',(7.93918496767691,-1.74147833821821,
72.3419879767086));
#174135=CARTESIAN_POINT('Ctrl Pts',(7.89174591770249,-1.94518638619677,
72.3342784455922));
#174136=CARTESIAN_POINT('Ctrl Pts',(7.80616930297352,-2.25756236921412,
72.3227389680835));
#174137=CARTESIAN_POINT('Ctrl Pts',(7.77349272313415,-2.36763151194455,
72.3187263148649));
#174138=CARTESIAN_POINT('Ctrl Pts',(7.72019059084956,-2.53415661578989,
72.3126962252828));
#174139=CARTESIAN_POINT('Ctrl Pts',(7.7012536796923,-2.59113573193026,72.3106403080961));
#174140=CARTESIAN_POINT('Ctrl Pts',(7.65311041591386,-2.7308016777998,72.3056098318278));
#174141=CARTESIAN_POINT('Ctrl Pts',(7.62319363052296,-2.81323584978403,
72.3026484823864));
#174142=CARTESIAN_POINT('Ctrl Pts',(7.54814618143299,-3.01003130888968,
72.2955702977016));
#174143=CARTESIAN_POINT('Ctrl Pts',(7.50174295869586,-3.12388413911585,
72.2914681881237));
#174144=CARTESIAN_POINT('Ctrl Pts',(7.35398908633463,-3.46410610577125,
72.2790992305006));
#174145=CARTESIAN_POINT('Ctrl Pts',(7.24484276246993,-3.6869279749241,72.2708443731707));
#174146=CARTESIAN_POINT('Ctrl Pts',(6.94753331744447,-4.22952813186986,
72.2498282037025));
#174147=CARTESIAN_POINT('Ctrl Pts',(6.74735584827594,-4.54205792881767,
72.2368684506662));
#174148=CARTESIAN_POINT('Ctrl Pts',(6.4353746976905,-4.96276847347414,72.2175034197649));
#174149=CARTESIAN_POINT('Ctrl Pts',(6.34074444171681,-5.08311670814125,
72.2117242698427));
#174150=CARTESIAN_POINT('Ctrl Pts',(6.2280017313192,-5.21844945028411,72.2049236714721));
#174151=CARTESIAN_POINT('Ctrl Pts',(6.21315379241246,-5.23611880803534,
72.204029683142));
#174152=CARTESIAN_POINT('Ctrl Pts',(6.19054413417771,-5.26279319474105,
72.202670764606));
#174153=CARTESIAN_POINT('Ctrl Pts',(6.1828375498404,-5.27184490654455,72.2022079904825));
#174154=CARTESIAN_POINT('Ctrl Pts',(6.1689325866376,-5.28810445021449,72.2013737501251));
#174155=CARTESIAN_POINT('Ctrl Pts',(6.16274136365834,-5.29531838691089,
72.2010025650811));
#174156=CARTESIAN_POINT('Ctrl Pts',(6.15033126375604,-5.30972723873345,
72.2002590566208));
#174157=CARTESIAN_POINT('Ctrl Pts',(6.14411238660805,-5.31692213443908,
72.1998867333906));
#174158=CARTESIAN_POINT('Ctrl Pts',(6.12672227474124,-5.33697027659267,
72.1988463059439));
#174159=CARTESIAN_POINT('Ctrl Pts',(6.11552327162103,-5.34979931165965,
72.1981771052115));
#174160=CARTESIAN_POINT('Ctrl Pts',(6.07030913853198,-5.40126693413939,
72.1954785580249));
#174161=CARTESIAN_POINT('Ctrl Pts',(6.03596784940917,-5.43961667154546,
72.1934362681541));
#174162=CARTESIAN_POINT('Ctrl Pts',(5.40032434219047,-6.13602371317179,
72.1557623189628));
#174163=CARTESIAN_POINT('Ctrl Pts',(4.69519240538418,-6.69095410946617,
72.1151810558609));
#174164=CARTESIAN_POINT('Ctrl Pts',(3.749174347508,-7.21102644371547,72.0671412255708));
#174165=CARTESIAN_POINT('Ctrl Pts',(3.58089650030489,-7.29605342109991,
72.0588448934444));
#174166=CARTESIAN_POINT('Ctrl Pts',(3.27939061971709,-7.43545085977603,
72.0445708382571));
#174167=CARTESIAN_POINT('Ctrl Pts',(3.14739007965915,-7.49228078923422,
72.0385134903086));
#174168=CARTESIAN_POINT('Ctrl Pts',(2.96970122811621,-7.56325539578843,
72.030670574294));
#174169=CARTESIAN_POINT('Ctrl Pts',(2.92530236746905,-7.58053848604186,
72.0287368087081));
#174170=CARTESIAN_POINT('Ctrl Pts',(2.8498638239487,-7.60914285430796,72.025494010966));
#174171=CARTESIAN_POINT('Ctrl Pts',(2.81890448255758,-7.62066639839367,
72.0241751221225));
#174172=CARTESIAN_POINT('Ctrl Pts',(2.77666048163881,-7.63609760870184,
72.0223907379606));
#174173=CARTESIAN_POINT('Ctrl Pts',(2.76543649514764,-7.64016957359124,
72.0219180964252));
#174174=CARTESIAN_POINT('Ctrl Pts',(2.74762676266306,-7.6465864020851,72.0211703883204));
#174175=CARTESIAN_POINT('Ctrl Pts',(2.7410469220259,-7.64894752257462,72.0208946340961));
#174176=CARTESIAN_POINT('Ctrl Pts',(2.72735758045506,-7.65383989529039,
72.0203219287197));
#174177=CARTESIAN_POINT('Ctrl Pts',(2.72024758158589,-7.65636974092588,
72.0200250362779));
#174178=CARTESIAN_POINT('Ctrl Pts',(2.70395243103713,-7.66214223925022,
72.0193458634097));
#174179=CARTESIAN_POINT('Ctrl Pts',(2.69476494250921,-7.66537829134713,
72.0189638529471));
#174180=CARTESIAN_POINT('Ctrl Pts',(2.66644529609841,-7.67529593741482,
72.0177891127069));
#174181=CARTESIAN_POINT('Ctrl Pts',(2.64729386452627,-7.68192250986928,
72.0169985789499));
#174182=CARTESIAN_POINT('Ctrl Pts',(2.49536096016209,-7.73385705303818,
72.0107566485465));
#174183=CARTESIAN_POINT('Ctrl Pts',(2.36144690896471,-7.77579205445396,
72.0054332755426));
#174184=CARTESIAN_POINT('Ctrl Pts',(1.82242374767841,-7.92937587773068,
71.9845098408519));
#174185=CARTESIAN_POINT('Ctrl Pts',(1.41000022841712,-8.01299917827056,
71.9695884318297));
#174186=CARTESIAN_POINT('Ctrl Pts',(0.660770043793895,-8.10525052058009,
71.9424541737385));
#174187=CARTESIAN_POINT('Ctrl Pts',(0.326390879380124,-8.12558698148869,
71.9303412267286));
#174188=CARTESIAN_POINT('Ctrl Pts',(-0.177154645820925,-8.12507361174617,
71.9116302759429));
#174189=CARTESIAN_POINT('Ctrl Pts',(-0.345975732781222,-8.11963692453342,
71.9052812927844));
#174190=CARTESIAN_POINT('Ctrl Pts',(-0.621379669958194,-8.1021629022256,
71.8947717732055));
#174191=CARTESIAN_POINT('Ctrl Pts',(-0.728111544639003,-8.09326939223116,
71.8906616295401));
#174192=CARTESIAN_POINT('Ctrl Pts',(-0.870298233511019,-8.07858613602711,
71.8851348184977));
#174193=CARTESIAN_POINT('Ctrl Pts',(-0.905936297801803,-8.07466732308913,
71.8837452647594));
#174194=CARTESIAN_POINT('Ctrl Pts',(-0.964819651271658,-8.06779769112256,
71.8814422762498));
#174195=CARTESIAN_POINT('Ctrl Pts',(-0.98808026437187,-8.06498195476041,
71.8805306991771));
#174196=CARTESIAN_POINT('Ctrl Pts',(-1.03308054028227,-8.05933699285622,
71.8787636286209));
#174197=CARTESIAN_POINT('Ctrl Pts',(-1.05482160078324,-8.05652031304778,
71.8779083192658));
#174198=CARTESIAN_POINT('Ctrl Pts',(-1.10387830075651,-8.04996275690394,
71.875974682275));
#174199=CARTESIAN_POINT('Ctrl Pts',(-1.13118680485935,-8.0461707721552,
71.8748956731085));
#174200=CARTESIAN_POINT('Ctrl Pts',(-1.20115881839355,-8.03609138407347,
71.8721239078179));
#174201=CARTESIAN_POINT('Ctrl Pts',(-1.24379240730171,-8.02960320654094,
71.8704283579014));
#174202=CARTESIAN_POINT('Ctrl Pts',(-1.51488356943178,-7.98613644160722,
71.8596010771361));
#174203=CARTESIAN_POINT('Ctrl Pts',(-1.74171806207007,-7.93975188705933,
71.8503291373223));
#174204=CARTESIAN_POINT('Ctrl Pts',(-2.00682622234335,-7.8736322144272,
71.839190830929));
#174205=CARTESIAN_POINT('Ctrl Pts',(-2.04731575041621,-7.86320125134358,
71.8374814050575));
#174206=CARTESIAN_POINT('Ctrl Pts',(-2.30512055736173,-7.79465902595829,
71.8265437792783));
#174207=CARTESIAN_POINT('Ctrl Pts',(-2.52001868938172,-7.72785813238617,
71.817179932485));
#174208=CARTESIAN_POINT('Ctrl Pts',(-2.98688176645549,-7.56118693729032,
71.7963310852899));
#174209=CARTESIAN_POINT('Ctrl Pts',(-3.23718755319796,-7.45745428388846,
71.7848131890206));
#174210=CARTESIAN_POINT('Ctrl Pts',(-3.79231863603349,-7.1941701917563,
71.758770810249));
#174211=CARTESIAN_POINT('Ctrl Pts',(-4.09315265023061,-7.02736675993834,
71.7442911404142));
#174212=CARTESIAN_POINT('Ctrl Pts',(-4.40889168279579,-6.82512577658013,
71.7291961587856));
#174213=CARTESIAN_POINT('Ctrl Pts',(-4.43515730382158,-6.80808691605568,
71.727941394451));
#174214=CARTESIAN_POINT('Ctrl Pts',(-4.47467627769516,-6.78212466724629,
71.726055600984));
#174215=CARTESIAN_POINT('Ctrl Pts',(-4.48800273054334,-6.77331339058104,
71.7254200458083));
#174216=CARTESIAN_POINT('Ctrl Pts',(-4.51238662939472,-6.75708751666462,
71.7242579285532));
#174217=CARTESIAN_POINT('Ctrl Pts',(-4.52345199201722,-6.74968494667762,
71.7237308586995));
#174218=CARTESIAN_POINT('Ctrl Pts',(-4.54131252423564,-6.73767285786067,
71.7228806554447));
#174219=CARTESIAN_POINT('Ctrl Pts',(-4.54811896438835,-6.7330801917622,
71.7225567794492));
#174220=CARTESIAN_POINT('Ctrl Pts',(-4.56114862372824,-6.72425961708287,
71.7219370379099));
#174221=CARTESIAN_POINT('Ctrl Pts',(-4.56737295340548,-6.72003336826816,
71.7216410978728));
#174222=CARTESIAN_POINT('Ctrl Pts',(-4.58148511524971,-6.71042270729361,
71.720970397624));
#174223=CARTESIAN_POINT('Ctrl Pts',(-4.58936935065679,-6.7050330152836,
71.7205958817484));
#174224=CARTESIAN_POINT('Ctrl Pts',(-4.61316303340061,-6.68870593800675,
71.7194662626136));
#174225=CARTESIAN_POINT('Ctrl Pts',(-4.62904308682632,-6.67772569116637,
71.7187131941158));
#174226=CARTESIAN_POINT('Ctrl Pts',(-4.75764884901585,-6.58812216392219,
71.7126221985415));
#174227=CARTESIAN_POINT('Ctrl Pts',(-4.86839046867243,-6.50671585011454,
71.7074391774823));
#174228=CARTESIAN_POINT('Ctrl Pts',(-4.9914715805629,-6.41133628367439,
71.7017214669738));
#174229=CARTESIAN_POINT('Ctrl Pts',(-5.00587793636145,-6.40009434101028,
71.7010527860219));
#174230=CARTESIAN_POINT('Ctrl Pts',(-5.61092781592472,-5.92465332024203,
71.6729879854966));
#174231=CARTESIAN_POINT('Ctrl Pts',(-6.1344268456325,-5.38080118977403,
71.6492218693922));
#174232=CARTESIAN_POINT('Ctrl Pts',(-6.79573739469479,-4.46966222613106,
71.6101699234832));
#174233=CARTESIAN_POINT('Ctrl Pts',(-6.99447620919207,-4.1517704508491,
71.5967066866135));
#174234=CARTESIAN_POINT('Ctrl Pts',(-7.19870656213617,-3.76853932757851,
71.5801715980217));
#174235=CARTESIAN_POINT('Ctrl Pts',(-7.22625143129925,-3.71544814329774,
71.5778751307285));
#174236=CARTESIAN_POINT('Ctrl Pts',(-7.2610135149388,-3.64659708295576,
71.5748883933583));
#174237=CARTESIAN_POINT('Ctrl Pts',(-7.2687702309883,-3.63111096969571,
71.5742160575835));
#174238=CARTESIAN_POINT('Ctrl Pts',(-7.28120825193478,-3.6060791708597,
71.573128370759));
#174239=CARTESIAN_POINT('Ctrl Pts',(-7.28592045725938,-3.59654885744889,
71.5727140429054));
#174240=CARTESIAN_POINT('Ctrl Pts',(-7.29487211851472,-3.57835456242222,
71.5719226338914));
#174241=CARTESIAN_POINT('Ctrl Pts',(-7.29911488010529,-3.56969222288833,
71.5715456627836));
#174242=CARTESIAN_POINT('Ctrl Pts',(-7.30876951742276,-3.54989141489916,
71.570683546783));
#174243=CARTESIAN_POINT('Ctrl Pts',(-7.31417136800568,-3.53874809985087,
71.5701980726932));
#174244=CARTESIAN_POINT('Ctrl Pts',(-7.32813960641714,-3.50976482380475,
71.5689345813134));
#174245=CARTESIAN_POINT('Ctrl Pts',(-7.33666630611144,-3.49190588585062,
71.5681552619687));
#174246=CARTESIAN_POINT('Ctrl Pts',(-7.38873995946633,-3.38180632816902,
71.5633458704179));
#174247=CARTESIAN_POINT('Ctrl Pts',(-7.43061098676327,-3.28878574378801,
71.5592611610081));
#174248=CARTESIAN_POINT('Ctrl Pts',(-7.75767053619448,-2.52403856549157,
71.5254927951342));
#174249=CARTESIAN_POINT('Ctrl Pts',(-7.95288701129577,-1.81755561601874,
71.4927521215064));
#174250=CARTESIAN_POINT('Ctrl Pts',(-8.12210716901295,-0.572953641409007,
71.4361327713641));
#174251=CARTESIAN_POINT('Ctrl Pts',(-8.14217494269334,-0.04549467870958,
71.4125983856602));
#174252=CARTESIAN_POINT('Ctrl Pts',(-8.10938780181966,0.508234116331102,
71.39040356535));
#174253=CARTESIAN_POINT('Ctrl Pts',(-8.10758720757868,0.536192257884405,
71.3892892255849));
#174254=CARTESIAN_POINT('Ctrl Pts',(-8.10489076270286,0.574935099791029,
71.3877530911188));
#174255=CARTESIAN_POINT('Ctrl Pts',(-8.10411792962021,0.58572794767398,
71.3873260272872));
#174256=CARTESIAN_POINT('Ctrl Pts',(-8.102774312729,0.603980103466187,71.3866052254961));
#174257=CARTESIAN_POINT('Ctrl Pts',(-8.10221478379891,0.611440206476997,
71.3863110176697));
#174258=CARTESIAN_POINT('Ctrl Pts',(-8.10108497497928,0.626229860189176,
71.3857285289231));
#174259=CARTESIAN_POINT('Ctrl Pts',(-8.10051504896648,0.633559430173642,
71.3854402337814));
#174260=CARTESIAN_POINT('Ctrl Pts',(-8.09923367861765,0.649754167785704,
71.3848040625161));
#174261=CARTESIAN_POINT('Ctrl Pts',(-8.09851762452955,0.658618968296973,
71.3844563725896));
#174262=CARTESIAN_POINT('Ctrl Pts',(-8.0959488520343,0.689782885721233,
71.383235934421));
#174263=CARTESIAN_POINT('Ctrl Pts',(-8.09401856694579,0.712075624075153,
71.3823662473177));
#174264=CARTESIAN_POINT('Ctrl Pts',(-8.06057194931326,1.08062758120911,
71.3680395665487));
#174265=CARTESIAN_POINT('Ctrl Pts',(-8.00695192987167,1.42454425133131,
71.3553998141502));
#174266=CARTESIAN_POINT('Ctrl Pts',(-7.80412581306698,2.33651838338503,
71.321796061126));
#174267=CARTESIAN_POINT('Ctrl Pts',(-7.6151792680233,2.89356970676521,71.3010230017926));
#174268=CARTESIAN_POINT('Ctrl Pts',(-7.19727977051824,3.79244936429604,
71.2640615559556));
#174269=CARTESIAN_POINT('Ctrl Pts',(-6.99946542087125,4.14619936434816,
71.2485817615133));
#174270=CARTESIAN_POINT('Ctrl Pts',(-6.72293859285824,4.56410735578998,
71.2291846775868));
#174271=CARTESIAN_POINT('Ctrl Pts',(-6.66832016618217,4.64354231640478,
71.2254414632883));
#174272=CARTESIAN_POINT('Ctrl Pts',(-6.58496769142871,4.7602626286742,71.2198506667732));
#174273=CARTESIAN_POINT('Ctrl Pts',(-6.55730194331004,4.79830084412732,
71.2180140037653));
#174274=CARTESIAN_POINT('Ctrl Pts',(-6.50696437873559,4.86626256381853,
71.2147052452221));
#174275=CARTESIAN_POINT('Ctrl Pts',(-6.48441245812721,4.89627325893316,
71.213234441493));
#174276=CARTESIAN_POINT('Ctrl Pts',(-6.43567933738876,4.96019702038749,
71.2100802850006));
#174277=CARTESIAN_POINT('Ctrl Pts',(-6.40943625549527,4.99406146157451,
71.2083963065731));
#174278=CARTESIAN_POINT('Ctrl Pts',(-6.33786449468941,5.08492523309164,
71.203841896057));
#174279=CARTESIAN_POINT('Ctrl Pts',(-6.29203547093929,5.14152511566616,
71.2009661032967));
#174280=CARTESIAN_POINT('Ctrl Pts',(-5.99822354309752,5.49457714782154,
71.1827742683189));
#174281=CARTESIAN_POINT('Ctrl Pts',(-5.73011890938351,5.77362874985495,
71.167233074209));
#174282=CARTESIAN_POINT('Ctrl Pts',(-5.14356787094451,6.30287644120553,
71.1351914507845));
#174283=CARTESIAN_POINT('Ctrl Pts',(-4.82422803895731,6.55052431125194,
71.1187238430818));
#174284=CARTESIAN_POINT('Ctrl Pts',(-4.41676435507607,6.82049442112218,
71.0990870451804));
#174285=CARTESIAN_POINT('Ctrl Pts',(-4.34497857649999,6.86644834670042,
71.0956763271705));
#174286=CARTESIAN_POINT('Ctrl Pts',(-4.22266014119511,6.9420645203891,71.0899516161459));
#174287=CARTESIAN_POINT('Ctrl Pts',(-4.17250573162737,6.97232489772471,
71.0876284093376));
#174288=CARTESIAN_POINT('Ctrl Pts',(-4.10115155948183,7.01433035461302,
71.0843586340783));
#174289=CARTESIAN_POINT('Ctrl Pts',(-4.08021999499516,7.02652682602128,
71.0834037140385));
#174290=CARTESIAN_POINT('Ctrl Pts',(-4.04323723635568,7.04785507970407,
71.0817241538075));
#174291=CARTESIAN_POINT('Ctrl Pts',(-4.02720890193824,7.05702607594547,
71.0809987462373));
#174292=CARTESIAN_POINT('Ctrl Pts',(-3.99220257066058,7.0768976859255,71.079419695486));
#174293=CARTESIAN_POINT('Ctrl Pts',(-3.97321250001097,7.08757678311576,
71.0785664512056));
#174294=CARTESIAN_POINT('Ctrl Pts',(-3.9201492367624,7.11713671174759,71.0761911514856));
#174295=CARTESIAN_POINT('Ctrl Pts',(-3.88598279114167,7.13584912829217,
71.0746719087804));
#174296=CARTESIAN_POINT('Ctrl Pts',(-3.64083412099443,7.26783030831431,
71.0638373832864));
#174297=CARTESIAN_POINT('Ctrl Pts',(-3.42506772951328,7.37197016519568,
71.0546455920066));
#174298=CARTESIAN_POINT('Ctrl Pts',(-2.9794605640374,7.56325006901938,71.0360052580862));
#174299=CARTESIAN_POINT('Ctrl Pts',(-2.74963618815843,7.64979975102331,
71.0265651246789));
#174300=CARTESIAN_POINT('Ctrl Pts',(-2.46205102193899,7.74346442267606,
71.0148228872735));
#174301=CARTESIAN_POINT('Ctrl Pts',(-2.40766959437042,7.76054531492432,
71.0126058024549));
#174302=CARTESIAN_POINT('Ctrl Pts',(-2.31752015566504,7.78782195028811,
71.0089345345016));
#174303=CARTESIAN_POINT('Ctrl Pts',(-2.28185376234295,7.7983468630871,71.0074830912306));
#174304=CARTESIAN_POINT('Ctrl Pts',(-2.21181852071274,7.81849218666112,
71.0046346685808));
#174305=CARTESIAN_POINT('Ctrl Pts',(-2.17745603643589,7.82813173371456,
71.0032378815212));
#174306=CARTESIAN_POINT('Ctrl Pts',(-2.10163344559445,7.84886401523147,
71.0001572058916));
#174307=CARTESIAN_POINT('Ctrl Pts',(-2.06014673256705,7.85985527165133,
70.9984725190217));
#174308=CARTESIAN_POINT('Ctrl Pts',(-1.91599980027263,7.89682506429924,
70.9926215822871));
#174309=CARTESIAN_POINT('Ctrl Pts',(-1.81292075903311,7.92112488179225,
70.98844191024));
#174310=CARTESIAN_POINT('Ctrl Pts',(-1.53134751399616,7.98171861287944,
70.9770337665918));
#174311=CARTESIAN_POINT('Ctrl Pts',(-1.35206154163355,8.01403680447728,
70.9697785863781));
#174312=CARTESIAN_POINT('Ctrl Pts',(-0.972043262195311,8.06942298042583,
70.9544449962139));
#174313=CARTESIAN_POINT('Ctrl Pts',(-0.771227515012711,8.09108545248789,
70.946367644826));
#174314=CARTESIAN_POINT('Ctrl Pts',(-0.504546282224392,8.10983362781094,
70.9357374043058));
#174315=CARTESIAN_POINT('Ctrl Pts',(-0.439225760877315,8.11363354029947,
70.9331415143973));
#174316=CARTESIAN_POINT('Ctrl Pts',(-0.327234507077776,8.11879204502633,
70.9287083012134));
#174317=CARTESIAN_POINT('Ctrl Pts',(-0.28058494286654,8.12053808683788,
70.9268668374692));
#174318=CARTESIAN_POINT('Ctrl Pts',(-0.211503770181915,8.12252773124193,
70.9241489425652));
#174319=CARTESIAN_POINT('Ctrl Pts',(-0.189082215551901,8.1230806047658,
70.9232682351449));
#174320=CARTESIAN_POINT('Ctrl Pts',(-0.146857469901718,8.12394686670683,
70.9216124105504));
#174321=CARTESIAN_POINT('Ctrl Pts',(-0.127054949774831,8.12428069754005,
70.9208369716678));
#174322=CARTESIAN_POINT('Ctrl Pts',(-0.0815579850499752,8.1248812989825,
70.9190577094675));
#174323=CARTESIAN_POINT('Ctrl Pts',(-0.0558630755347635,8.12509859328326,
70.9180545622681));
#174324=CARTESIAN_POINT('Ctrl Pts',(0.0123321477511183,8.12535179092498,
70.9153961902816));
#174325=CARTESIAN_POINT('Ctrl Pts',(0.0548325363598336,8.12517613507318,
70.913743587966));
#174326=CARTESIAN_POINT('Ctrl Pts',(0.466865950002563,8.1202401666167,70.8977536317569));
#174327=CARTESIAN_POINT('Ctrl Pts',(0.835673794229557,8.09060688734209,
70.8836710363049));
#174328=CARTESIAN_POINT('Ctrl Pts',(1.36171574237481,8.01197628077325,70.8632572662452));
#174329=CARTESIAN_POINT('Ctrl Pts',(1.52149125407162,7.98317590727053,70.8570154963416));
#174330=CARTESIAN_POINT('Ctrl Pts',(1.82945705073294,7.91808168022554,70.8448565825756));
#174331=CARTESIAN_POINT('Ctrl Pts',(1.97770017857377,7.88236208344037,70.838945229761));
#174332=CARTESIAN_POINT('Ctrl Pts',(2.19036479600651,7.82474261310355,70.8303622292009));
#174333=CARTESIAN_POINT('Ctrl Pts',(2.25565485830422,7.80617166146281,70.8277130687633));
#174334=CARTESIAN_POINT('Ctrl Pts',(2.3725345149626,7.7713378843036,70.8229441925071));
#174335=CARTESIAN_POINT('Ctrl Pts',(2.42420903188614,7.75537381958172,70.8208264138433));
#174336=CARTESIAN_POINT('Ctrl Pts',(2.53919592216212,7.71858880518702,70.8160925735475));
#174337=CARTESIAN_POINT('Ctrl Pts',(2.6024192577888,7.69750238977082,70.813475199615));
#174338=CARTESIAN_POINT('Ctrl Pts',(2.82017536466298,7.62188630762233,70.8044097103626));
#174339=CARTESIAN_POINT('Ctrl Pts',(2.97331278707267,7.56346155516255,70.7979447823253));
#174340=CARTESIAN_POINT('Ctrl Pts',(3.2308281893675,7.45618434676361,70.7869312597258));
#174341=CARTESIAN_POINT('Ctrl Pts',(3.33612592249368,7.40966933736333,70.7823863691926));
#174342=CARTESIAN_POINT('Ctrl Pts',(3.47248358467956,7.34593762153586,70.77645327592));
#174343=CARTESIAN_POINT('Ctrl Pts',(3.50446886675525,7.33073255225362,70.7750580945332));
#174344=CARTESIAN_POINT('Ctrl Pts',(3.58421397240402,7.29218236606534,70.7715714814167));
#174345=CARTESIAN_POINT('Ctrl Pts',(3.63184610210123,7.26857670913078,70.769481520171));
#174346=CARTESIAN_POINT('Ctrl Pts',(3.7149371627918,7.2263775233482,70.7658240679228));
#174347=CARTESIAN_POINT('Ctrl Pts',(3.75049656320541,7.20798624934944,70.7642552031043));
#174348=CARTESIAN_POINT('Ctrl Pts',(3.83724584712964,7.16230388280299,70.7604178434199));
#174349=CARTESIAN_POINT('Ctrl Pts',(3.88828215720208,7.13472595809677,70.758151477773));
#174350=CARTESIAN_POINT('Ctrl Pts',(4.10309942568018,7.01565793411155,70.7485664893735));
#174351=CARTESIAN_POINT('Ctrl Pts',(4.26398133561234,6.91905662459237,70.7412735337428));
#174352=CARTESIAN_POINT('Ctrl Pts',(4.4726076200251,6.78374509481955,70.7315871315129));
#174353=CARTESIAN_POINT('Ctrl Pts',(4.52346361755219,6.7499402455907,70.7292073185378));
#174354=CARTESIAN_POINT('Ctrl Pts',(4.64547241950542,6.66684073964602,70.7234488329007));
#174355=CARTESIAN_POINT('Ctrl Pts',(4.71622785884208,6.61697620967572,70.7200682410466));
#174356=CARTESIAN_POINT('Ctrl Pts',(4.83167108467573,6.53282573646637,70.714477652273));
#174357=CARTESIAN_POINT('Ctrl Pts',(4.87682321037085,6.49918863573094,70.7122716593564));
#174358=CARTESIAN_POINT('Ctrl Pts',(4.96265734114744,6.43384639466952,70.7080389578296));
#174359=CARTESIAN_POINT('Ctrl Pts',(5.00339426095581,6.40221783162282,70.7060128543733));
#174360=CARTESIAN_POINT('Ctrl Pts',(5.11385168074785,6.31475938120592,70.7004700932477));
#174361=CARTESIAN_POINT('Ctrl Pts',(5.18295689963812,6.2581644842555,70.6969481139968));
#174362=CARTESIAN_POINT('Ctrl Pts',(5.60382537133273,5.90173366450811,70.6751454625246));
#174363=CARTESIAN_POINT('Ctrl Pts',(5.9304020742526,5.57347636726984,70.6566230950635));
#174364=CARTESIAN_POINT('Ctrl Pts',(6.30944666723935,5.12122337965189,70.6330358672515));
#174365=CARTESIAN_POINT('Ctrl Pts',(6.38927806623034,5.02127198022834,70.6279341022965));
#174366=CARTESIAN_POINT('Ctrl Pts',(6.49914869383377,4.87684560901156,70.6207317766775));
#174367=CARTESIAN_POINT('Ctrl Pts',(6.53115805922531,4.83389400885742,70.6186104661968));
#174368=CARTESIAN_POINT('Ctrl Pts',(6.58728505208385,4.75700496202787,70.6148510780976));
#174369=CARTESIAN_POINT('Ctrl Pts',(6.61157095301244,4.72319278933939,70.6132107125388));
#174370=CARTESIAN_POINT('Ctrl Pts',(6.64888530260346,4.67038992424895,70.6106695992693));
#174371=CARTESIAN_POINT('Ctrl Pts',(6.66209461606928,4.65152804389989,70.6097659103944));
#174372=CARTESIAN_POINT('Ctrl Pts',(6.6864211146216,4.6164754904999,70.6080941157472));
#174373=CARTESIAN_POINT('Ctrl Pts',(6.69756011913283,4.60030017828732,70.6073256274008));
#174374=CARTESIAN_POINT('Ctrl Pts',(6.72277274354714,4.56340242331729,70.6055794959634));
#174375=CARTESIAN_POINT('Ctrl Pts',(6.73680938663503,4.54265498684987,70.6046025975057));
#174376=CARTESIAN_POINT('Ctrl Pts',(6.78317023212566,4.4734419520957,70.6013593643055));
#174377=CARTESIAN_POINT('Ctrl Pts',(6.81506928648291,4.42469343445056,70.5991004475842));
#174378=CARTESIAN_POINT('Ctrl Pts',(6.98445761290257,4.15965419069249,70.5869398841881));
#174379=CARTESIAN_POINT('Ctrl Pts',(7.11218036556518,3.93729146884441,70.5771619352727));
#174380=CARTESIAN_POINT('Ctrl Pts',(7.3065276361628,3.55851768801626,70.5608651367569));
#174381=CARTESIAN_POINT('Ctrl Pts',(7.37913996320894,3.4053908853602,70.5543703537443));
#174382=CARTESIAN_POINT('Ctrl Pts',(7.49144532854843,3.14806761629204,70.5435453680393));
#174383=CARTESIAN_POINT('Ctrl Pts',(7.53387679306897,3.04512446454064,70.5392380281772));
#174384=CARTESIAN_POINT('Ctrl Pts',(7.59125404644554,2.89737370259024,70.5330784735375));
#174385=CARTESIAN_POINT('Ctrl Pts',(7.60794558758513,2.85325713557075,70.5312421718113));
#174386=CARTESIAN_POINT('Ctrl Pts',(7.63650474971762,2.77574114584565,70.5280199941431));
#174387=CARTESIAN_POINT('Ctrl Pts',(7.64853974192807,2.74240469417306,70.5266356631243));
#174388=CARTESIAN_POINT('Ctrl Pts',(7.67162879921967,2.67711454483264,70.5239268981184));
#174389=CARTESIAN_POINT('Ctrl Pts',(7.68270229111433,2.64516846646532,70.5226026667168));
#174390=CARTESIAN_POINT('Ctrl Pts',(7.71249874840557,2.55744256647578,70.5189691693249));
#174391=CARTESIAN_POINT('Ctrl Pts',(7.73081568700851,2.50152717171804,70.5166564341745));
#174392=CARTESIAN_POINT('Ctrl Pts',(7.84458082561739,2.14105224307255,70.5017657142116));
#174393=CARTESIAN_POINT('Ctrl Pts',(7.92262001831429,1.83129459579061,70.4890400931874));
#174394=CARTESIAN_POINT('Ctrl Pts',(8.0040754175095,1.40290158378793,70.4716500691821));
#174395=CARTESIAN_POINT('Ctrl Pts',(8.02343272710258,1.28758828974776,70.4669914170889));
#174396=CARTESIAN_POINT('Ctrl Pts',(8.05037215628687,1.10275897164459,70.4595774573658));
#174397=CARTESIAN_POINT('Ctrl Pts',(8.05955711576899,1.03349329748628,70.4568109495476));
#174398=CARTESIAN_POINT('Ctrl Pts',(8.07103589346378,0.937437546265412,
70.4529949806364));
#174399=CARTESIAN_POINT('Ctrl Pts',(8.07409182279171,0.910741890424098,
70.4519366489683));
#174400=CARTESIAN_POINT('Ctrl Pts',(8.07908818077056,0.865092318483335,
70.4501309695083));
#174401=CARTESIAN_POINT('Ctrl Pts',(8.08109446385744,0.846145862850543,
70.4493827341964));
#174402=CARTESIAN_POINT('Ctrl Pts',(8.08481742108188,0.809766434194584,
70.4479484614929));
#174403=CARTESIAN_POINT('Ctrl Pts',(8.08654438991563,0.792334678125103,
70.4472622914036));
#174404=CARTESIAN_POINT('Ctrl Pts',(8.091296918529,0.742728790426684,70.445312704527));
#174405=CARTESIAN_POINT('Ctrl Pts',(8.09418692589185,0.710541978090115,
70.4440513329304));
#174406=CARTESIAN_POINT('Ctrl Pts',(8.1062462310358,0.56659794473718,70.4384249761508));
#174407=CARTESIAN_POINT('Ctrl Pts',(8.11329359178476,0.454674335631456,
70.4340896728578));
#174408=CARTESIAN_POINT('Ctrl Pts',(8.12284981053059,0.228262825703277,
70.4253719529228));
#174409=CARTESIAN_POINT('Ctrl Pts',(8.12525961307041,0.113795876175322,
70.4209914133454));
#174410=CARTESIAN_POINT('Ctrl Pts',(8.12521102066953,-0.463152093049132,
70.3989788627655));
#174411=CARTESIAN_POINT('Ctrl Pts',(8.08568865400911,-0.924772150512832,
70.381553585682));
#174412=CARTESIAN_POINT('Ctrl Pts',(8.00536840918922,-1.3906364203307,70.3634517871324));
#174413=CARTESIAN_POINT('Ctrl Pts',(8.00360443098289,-1.40075305909931,
70.3630584547249));
#174414=CARTESIAN_POINT('Ctrl Pts',(7.96184204267193,-1.63761119523076,
70.3538438034098));
#174415=CARTESIAN_POINT('Ctrl Pts',(7.91224357439764,-1.86255160519841,
70.3449689048758));
#174416=CARTESIAN_POINT('Ctrl Pts',(7.83600451309022,-2.14969542717593,
70.3334186531768));
#174417=CARTESIAN_POINT('Ctrl Pts',(7.81805157208324,-2.21409726839991,
70.3308136797705));
#174418=CARTESIAN_POINT('Ctrl Pts',(7.7877663440834,-2.31777407627084,70.326595535779));
#174419=CARTESIAN_POINT('Ctrl Pts',(7.77592678248519,-2.35718984345461,
70.3249861104559));
#174420=CARTESIAN_POINT('Ctrl Pts',(7.7526120905287,-2.4327205276596,70.3218906733692));
#174421=CARTESIAN_POINT('Ctrl Pts',(7.74118275997524,-2.4688484882497,70.3204050305507));
#174422=CARTESIAN_POINT('Ctrl Pts',(7.71405078766447,-2.55257120005117,
70.3169503174575));
#174423=CARTESIAN_POINT('Ctrl Pts',(7.69815968671359,-2.6001032095624,70.3149799882836));
#174424=CARTESIAN_POINT('Ctrl Pts',(7.64463098599666,-2.75541980893398,
70.3085117226566));
#174425=CARTESIAN_POINT('Ctrl Pts',(7.60516155662379,-2.86255806788374,
70.3040021721219));
#174426=CARTESIAN_POINT('Ctrl Pts',(7.33791659911186,-3.54339676207545,
70.2750337620794));
#174427=CARTESIAN_POINT('Ctrl Pts',(7.0476618457027,-4.09036631971679,70.2503042843223));
#174428=CARTESIAN_POINT('Ctrl Pts',(6.45944268322675,-4.94705537190274,
70.206885575961));
#174429=CARTESIAN_POINT('Ctrl Pts',(6.19385657087972,-5.27578274585069,
70.1888842928901));
#174430=CARTESIAN_POINT('Ctrl Pts',(5.71598413270993,-5.78118165530637,
70.159648903071));
#174431=CARTESIAN_POINT('Ctrl Pts',(5.5180912241296,-5.97036155979792,70.148294836524));
#174432=CARTESIAN_POINT('Ctrl Pts',(5.29418462112617,-6.16374820610839,
70.1365249303017));
#174433=CARTESIAN_POINT('Ctrl Pts',(5.2772838595182,-6.17822448836411,70.135642875744));
#174434=CARTESIAN_POINT('Ctrl Pts',(5.25356075435809,-6.19837605374711,
70.1344138706803));
#174435=CARTESIAN_POINT('Ctrl Pts',(5.24678834259311,-6.2041097985284,70.1340640493713));
#174436=CARTESIAN_POINT('Ctrl Pts',(5.23439196123506,-6.2145701643817,70.1334256332464));
#174437=CARTESIAN_POINT('Ctrl Pts',(5.22877095286869,-6.21930027050853,
70.1331368635155));
#174438=CARTESIAN_POINT('Ctrl Pts',(5.21740836867921,-6.2288356482483,70.1325545822708));
#174439=CARTESIAN_POINT('Ctrl Pts',(5.21166654981927,-6.23364062105183,
70.1322610860705));
#174440=CARTESIAN_POINT('Ctrl Pts',(5.19758783855358,-6.24538917438899,
70.1315432878215));
#174441=CARTESIAN_POINT('Ctrl Pts',(5.18924364966388,-6.25232401791281,
70.131119440424));
#174442=CARTESIAN_POINT('Ctrl Pts',(5.15915753836315,-6.27722682501975,
70.1295969510889));
#174443=CARTESIAN_POINT('Ctrl Pts',(5.13733581759779,-6.29509839819479,
70.1285034534015));
#174444=CARTESIAN_POINT('Ctrl Pts',(5.01894048924274,-6.39103627032841,
70.1226306930314));
#174445=CARTESIAN_POINT('Ctrl Pts',(4.92068208345349,-6.46699280498969,
70.1179797515618));
#174446=CARTESIAN_POINT('Ctrl Pts',(4.7194201191621,-6.61533048007238,70.1088355778977));
#174447=CARTESIAN_POINT('Ctrl Pts',(4.61639659419257,-6.68763095760165,
70.1043445752153));
#174448=CARTESIAN_POINT('Ctrl Pts',(4.26847310631183,-6.91992621151057,
70.0896785612089));
#174449=CARTESIAN_POINT('Ctrl Pts',(4.01661312776997,-7.06909265258483,
70.0798588002836));
#174450=CARTESIAN_POINT('Ctrl Pts',(3.51428884849086,-7.33106733635283,
70.0609437903159));
#174451=CARTESIAN_POINT('Ctrl Pts',(3.26507234615863,-7.44540631990467,
70.05185297893));
#174452=CARTESIAN_POINT('Ctrl Pts',(2.52446720160884,-7.74084221022625,
70.024827851808));
#174453=CARTESIAN_POINT('Ctrl Pts',(2.02083343283141,-7.88731448839574,
70.0063602070289));
#174454=CARTESIAN_POINT('Ctrl Pts',(1.47462488986803,-7.99038362122791,
69.9849932148308));
#174455=CARTESIAN_POINT('Ctrl Pts',(1.4425746555034,-7.99623206980877,69.9837350627376));
#174456=CARTESIAN_POINT('Ctrl Pts',(1.39801453122952,-8.00408666961057,
69.9819795696626));
#174457=CARTESIAN_POINT('Ctrl Pts',(1.38553363883102,-8.00625658957399,
69.9814871914562));
#174458=CARTESIAN_POINT('Ctrl Pts',(1.3640379922249,-8.00994203976023,69.9806379943421));
#174459=CARTESIAN_POINT('Ctrl Pts',(1.35502564541722,-8.01147156420938,
69.9802815994345));
#174460=CARTESIAN_POINT('Ctrl Pts',(1.33642812894035,-8.01459555039709,
69.9795454156831));
#174461=CARTESIAN_POINT('Ctrl Pts',(1.32684264344161,-8.01618803291472,
69.9791655676479));
#174462=CARTESIAN_POINT('Ctrl Pts',(1.30453879484438,-8.01985237673453,
69.9782807734856));
#174463=CARTESIAN_POINT('Ctrl Pts',(1.29181833000483,-8.0219111820242,69.9777754341324));
#174464=CARTESIAN_POINT('Ctrl Pts',(1.25132490882108,-8.02836622228204,
69.9761644704218));
#174465=CARTESIAN_POINT('Ctrl Pts',(1.22353414337463,-8.0326485300445,69.9750554161045));
#174466=CARTESIAN_POINT('Ctrl Pts',(0.685409441237254,-8.11271131149232,
69.9535127482153));
#174467=CARTESIAN_POINT('Ctrl Pts',(0.169091766363293,-8.13985034820149,
69.9315661332443));
#174468=CARTESIAN_POINT('Ctrl Pts',(-1.12268340649487,-8.08475128496889,
69.8743495850356));
#174469=CARTESIAN_POINT('Ctrl Pts',(-1.89037987318308,-7.94041816769533,
69.838114659094));
#174470=CARTESIAN_POINT('Ctrl Pts',(-2.66449371236685,-7.67605521527749,
69.8050954500327));
#174471=CARTESIAN_POINT('Ctrl Pts',(-2.70298427949223,-7.66258614844077,
69.8034632276906));
#174472=CARTESIAN_POINT('Ctrl Pts',(-2.75397260833487,-7.64431171505664,
69.8013119894218));
#174473=CARTESIAN_POINT('Ctrl Pts',(-2.76656178318958,-7.63976456620548,
69.800781733742));
#174474=CARTESIAN_POINT('Ctrl Pts',(-2.78613575062367,-7.63263981665349,
69.7999585949431));
#174475=CARTESIAN_POINT('Ctrl Pts',(-2.79312829918805,-7.63008370179775,
69.7996648010626));
#174476=CARTESIAN_POINT('Ctrl Pts',(-2.80715708583404,-7.62493363215728,
69.7990758875457));
#174477=CARTESIAN_POINT('Ctrl Pts',(-2.81419326522917,-7.622339540177,69.7987807740736));
#174478=CARTESIAN_POINT('Ctrl Pts',(-2.82994463495543,-7.61650755685396,
69.7981206851073));
#174479=CARTESIAN_POINT('Ctrl Pts',(-2.83865788791283,-7.6132644375987,
69.7977559250275));
#174480=CARTESIAN_POINT('Ctrl Pts',(-2.86429221961688,-7.60367307719444,
69.7966838894245));
#174481=CARTESIAN_POINT('Ctrl Pts',(-2.88119776630638,-7.59728330536158,
69.7959782891976));
#174482=CARTESIAN_POINT('Ctrl Pts',(-3.01217327325884,-7.54727857692013,
69.7905216180425));
#174483=CARTESIAN_POINT('Ctrl Pts',(-3.12527129057741,-7.50115209177839,
69.7858682579696));
#174484=CARTESIAN_POINT('Ctrl Pts',(-3.53580520945711,-7.32282020534022,
69.769070096283));
#174485=CARTESIAN_POINT('Ctrl Pts',(-3.82627140615542,-7.17532412275545,
69.7573553566899));
#174486=CARTESIAN_POINT('Ctrl Pts',(-4.31543366197447,-6.88875969781271,
69.7369939457859));
#174487=CARTESIAN_POINT('Ctrl Pts',(-4.51820916486686,-6.7574967925622,
69.7283491849793));
#174488=CARTESIAN_POINT('Ctrl Pts',(-5.08240579768239,-6.35551189765814,
69.7032436953689));
#174489=CARTESIAN_POINT('Ctrl Pts',(-5.42749546570607,-6.06346784630231,
69.6865185591514));
#174490=CARTESIAN_POINT('Ctrl Pts',(-5.78489424545429,-5.70592928269897,
69.6670641678215));
#174491=CARTESIAN_POINT('Ctrl Pts',(-5.822860475225,-5.66717974231265,69.6649687097535));
#174492=CARTESIAN_POINT('Ctrl Pts',(-5.87963071179815,-5.60806546091758,
69.6617913833632));
#174493=CARTESIAN_POINT('Ctrl Pts',(-5.89872337670598,-5.58797978144977,
69.660715121027));
#174494=CARTESIAN_POINT('Ctrl Pts',(-5.93274761434856,-5.55181724297009,
69.6587833489756));
#174495=CARTESIAN_POINT('Ctrl Pts',(-5.94771756087288,-5.53577679879834,
69.6579285559876));
#174496=CARTESIAN_POINT('Ctrl Pts',(-5.97849766303341,-5.50252663626776,
69.6561609267104));
#174497=CARTESIAN_POINT('Ctrl Pts',(-5.99429893369876,-5.48530892277588,
69.6552479285773));
#174498=CARTESIAN_POINT('Ctrl Pts',(-6.0339603650917,-5.44171616413769,
69.6529419619288));
#174499=CARTESIAN_POINT('Ctrl Pts',(-6.05772198622704,-5.41525223955118,
69.6515472082112));
#174500=CARTESIAN_POINT('Ctrl Pts',(-6.15203516966994,-5.30881567487904,
69.6459568513787));
#174501=CARTESIAN_POINT('Ctrl Pts',(-6.22118216170835,-5.22761442520881,
69.641734832547));
#174502=CARTESIAN_POINT('Ctrl Pts',(-6.80567378693081,-4.5132036145341,
69.6049020913526));
#174503=CARTESIAN_POINT('Ctrl Pts',(-7.22443060215095,-3.80703758585675,
69.5698953363403));
#174504=CARTESIAN_POINT('Ctrl Pts',(-7.62326117383189,-2.82243333133104,
69.525297386777));
#174505=CARTESIAN_POINT('Ctrl Pts',(-7.70524212631386,-2.59026915367048,
69.5151134302322));
#174506=CARTESIAN_POINT('Ctrl Pts',(-7.78318193918576,-2.33287125718537,
69.5043889143253));
#174507=CARTESIAN_POINT('Ctrl Pts',(-7.78970998082622,-2.31097984152365,
69.5034812441314));
#174508=CARTESIAN_POINT('Ctrl Pts',(-7.79874055978895,-2.28022325310348,
69.5022124692848));
#174509=CARTESIAN_POINT('Ctrl Pts',(-7.80132044441033,-2.27138101765195,
69.501848456534));
#174510=CARTESIAN_POINT('Ctrl Pts',(-7.80601993238448,-2.25517164412501,
69.5011825489026));
#174511=CARTESIAN_POINT('Ctrl Pts',(-7.80814415422935,-2.24780586272768,
69.5008804764231));
#174512=CARTESIAN_POINT('Ctrl Pts',(-7.81242352860919,-2.23288778347482,
69.5002697603115));
#174513=CARTESIAN_POINT('Ctrl Pts',(-7.81457816214596,-2.22533534376384,
69.4999611372646));
#174514=CARTESIAN_POINT('Ctrl Pts',(-7.81984873207604,-2.20675884686842,
69.4992034178064));
#174515=CARTESIAN_POINT('Ctrl Pts',(-7.82295231619448,-2.19573128160686,
69.4987548159585));
#174516=CARTESIAN_POINT('Ctrl Pts',(-7.83415378797876,-2.1556053158934,
69.4971269457086));
#174517=CARTESIAN_POINT('Ctrl Pts',(-7.84211279301498,-2.12646815769041,
69.4959533920774));
#174518=CARTESIAN_POINT('Ctrl Pts',(-7.8858527843668,-1.9627542960068,69.4894095773776));
#174519=CARTESIAN_POINT('Ctrl Pts',(-7.91833107642896,-1.82732355148469,
69.4841980488634));
#174520=CARTESIAN_POINT('Ctrl Pts',(-7.96649898976188,-1.60096170352779,
69.475755305302));
#174521=CARTESIAN_POINT('Ctrl Pts',(-7.98414908211039,-1.51047960281127,
69.4724492669952));
#174522=CARTESIAN_POINT('Ctrl Pts',(-8.08425921272116,-0.946347622755314,
69.452172700937));
#174523=CARTESIAN_POINT('Ctrl Pts',(-8.12608706776378,-0.466441020489828,
69.4363477489438));
#174524=CARTESIAN_POINT('Ctrl Pts',(-8.12420806368213,0.596718049988053,
69.4003988978025));
#174525=CARTESIAN_POINT('Ctrl Pts',(-8.06057789775269,1.17721256588351,
69.3800983281423));
#174526=CARTESIAN_POINT('Ctrl Pts',(-7.92771808349984,1.78108723886922,
69.3563595479564));
#174527=CARTESIAN_POINT('Ctrl Pts',(-7.91974216543471,1.81622403842902,
69.3549692431946));
#174528=CARTESIAN_POINT('Ctrl Pts',(-7.90852037189623,1.86418022227607,
69.3530590537562));
#174529=CARTESIAN_POINT('Ctrl Pts',(-7.90547646684718,1.87704667070063,
69.352545310608));
#174530=CARTESIAN_POINT('Ctrl Pts',(-7.90024023707496,1.89894130311322,
69.3516689434141));
#174531=CARTESIAN_POINT('Ctrl Pts',(-7.89806380339156,1.90797327890583,
69.351306803821));
#174532=CARTESIAN_POINT('Ctrl Pts',(-7.89382236281962,1.9254432035057,69.3506051359127));
#174533=CARTESIAN_POINT('Ctrl Pts',(-7.89175930468227,1.93388161532513,
69.3502656674043));
#174534=CARTESIAN_POINT('Ctrl Pts',(-7.88682861845043,1.95391004334875,
69.3494586443778));
#174535=CARTESIAN_POINT('Ctrl Pts',(-7.883948972578,1.96549706452093,69.348990723491));
#174536=CARTESIAN_POINT('Ctrl Pts',(-7.87536771486809,1.99970374695952,
69.347606274945));
#174537=CARTESIAN_POINT('Ctrl Pts',(-7.86959424239913,2.02230516219376,
69.3466875522776));
#174538=CARTESIAN_POINT('Ctrl Pts',(-7.82346079782808,2.19971431373903,
69.3394445293105));
#174539=CARTESIAN_POINT('Ctrl Pts',(-7.77863554647648,2.353318377364,69.3329834798282));
#174540=CARTESIAN_POINT('Ctrl Pts',(-7.66990437118594,2.68874786390042,
69.3184425885165));
#174541=CARTESIAN_POINT('Ctrl Pts',(-7.60400611593848,2.86982286334984,
69.3103056836526));
#174542=CARTESIAN_POINT('Ctrl Pts',(-7.29689156039784,3.62862185723587,
69.2750327645425));
#174543=CARTESIAN_POINT('Ctrl Pts',(-6.99578450431915,4.17976247284559,
69.2462802276797));
#174544=CARTESIAN_POINT('Ctrl Pts',(-6.41412665823376,5.00243139365272,
69.2014013177315));
#174545=CARTESIAN_POINT('Ctrl Pts',(-6.17207815084648,5.2981970177237,69.1848421192762));
#174546=CARTESIAN_POINT('Ctrl Pts',(-5.8936089731106,5.59335654494038,69.1686386974851));
#174547=CARTESIAN_POINT('Ctrl Pts',(-5.87705304586395,5.61074965407702,
69.1676846751924));
#174548=CARTESIAN_POINT('Ctrl Pts',(-5.85390396730234,5.63485442608403,
69.1663632241873));
#174549=CARTESIAN_POINT('Ctrl Pts',(-5.84737600522581,5.64162830360981,
69.1659919511869));
#174550=CARTESIAN_POINT('Ctrl Pts',(-5.83609923825769,5.65328927951273,
69.1653529233625));
#174551=CARTESIAN_POINT('Ctrl Pts',(-5.83135603169067,5.6581817599575,69.1650848446888));
#174552=CARTESIAN_POINT('Ctrl Pts',(-5.82154115947836,5.66828006657245,
69.1645315697771));
#174553=CARTESIAN_POINT('Ctrl Pts',(-5.81646865180371,5.67348506718894,
69.1642464222294));
#174554=CARTESIAN_POINT('Ctrl Pts',(-5.80462613185168,5.68560433653809,
69.1635825351703));
#174555=CARTESIAN_POINT('Ctrl Pts',(-5.79785072916694,5.69251333995597,
69.1632040998581));
#174556=CARTESIAN_POINT('Ctrl Pts',(-5.77643571253208,5.71427273343935,
69.1620122990789));
#174557=CARTESIAN_POINT('Ctrl Pts',(-5.76175119704321,5.72907894573721,
69.1612014146334));
#174558=CARTESIAN_POINT('Ctrl Pts',(-5.62588778504759,5.86501760559962,
69.1537554811931));
#174559=CARTESIAN_POINT('Ctrl Pts',(-5.50095799946835,5.98234988834199,
69.1473199099218));
#174560=CARTESIAN_POINT('Ctrl Pts',(-5.22708447628595,6.22372871095469,
69.1338491205783));
#174561=CARTESIAN_POINT('Ctrl Pts',(-5.07722421852103,6.34657453499534,
69.1268489394979));
#174562=CARTESIAN_POINT('Ctrl Pts',(-4.68360841064116,6.64636275139911,
69.1090720866717));
#174563=CARTESIAN_POINT('Ctrl Pts',(-4.43415025674763,6.81532372194114,
69.0983571724786));
#174564=CARTESIAN_POINT('Ctrl Pts',(-3.88156971909406,7.14638530192673,
69.0750731776475));
#174565=CARTESIAN_POINT('Ctrl Pts',(-3.57638547463713,7.30389357314996,
69.0624704409213));
#174566=CARTESIAN_POINT('Ctrl Pts',(-2.96121531300906,7.57356373851832,
69.0371963198603));
#174567=CARTESIAN_POINT('Ctrl Pts',(-2.65254292039627,7.68711056539703,
69.024596737373));
#174568=CARTESIAN_POINT('Ctrl Pts',(-2.24388602237955,7.8098841672753,69.0080829800269));
#174569=CARTESIAN_POINT('Ctrl Pts',(-2.1494116824107,7.83641144922028,69.0042732327988));
#174570=CARTESIAN_POINT('Ctrl Pts',(-2.00866858150771,7.87319377271939,
68.9986031942153));
#174571=CARTESIAN_POINT('Ctrl Pts',(-1.96275286531232,7.88476574272989,
68.9967542892249));
#174572=CARTESIAN_POINT('Ctrl Pts',(-1.88023255802318,7.90479755121464,
68.9934322564218));
#174573=CARTESIAN_POINT('Ctrl Pts',(-1.84366542552282,7.91340613034307,
68.9919604636509));
#174574=CARTESIAN_POINT('Ctrl Pts',(-1.77285825178119,7.92955801857297,
68.9891107608784));
#174575=CARTESIAN_POINT('Ctrl Pts',(-1.73862647552142,7.93713391084969,
68.9877331690328));
#174576=CARTESIAN_POINT('Ctrl Pts',(-1.65580289577095,7.9549022181951,68.9844000091245));
#174577=CARTESIAN_POINT('Ctrl Pts',(-1.6071646971683,7.96487125672831,68.9824425363852));
#174578=CARTESIAN_POINT('Ctrl Pts',(-1.40798595367946,8.00379682227947,
68.9744248176684));
#174579=CARTESIAN_POINT('Ctrl Pts',(-1.25673307356647,8.02893574027641,
68.9683320555353));
#174580=CARTESIAN_POINT('Ctrl Pts',(-0.862835584914242,8.08299957998712,
68.9524377680066));
#174581=CARTESIAN_POINT('Ctrl Pts',(-0.619437882252064,8.10528601764408,
68.942587929458));
#174582=CARTESIAN_POINT('Ctrl Pts',(-0.146004578182886,8.12718336880894,
68.9233792791811));
#174583=CARTESIAN_POINT('Ctrl Pts',(0.0837468794542702,8.12806329111535,
68.9140353986946));
#174584=CARTESIAN_POINT('Ctrl Pts',(0.50732398423374,8.11172239437114,68.8968220247214));
#174585=CARTESIAN_POINT('Ctrl Pts',(0.701093165108121,8.09727654641522,
68.8889533412629));
#174586=CARTESIAN_POINT('Ctrl Pts',(1.01819559679323,8.06216713146995,68.8761361493206));
#174587=CARTESIAN_POINT('Ctrl Pts',(1.14190034348952,8.04557800554014,68.8711513789643));
#174588=CARTESIAN_POINT('Ctrl Pts',(1.29804345678392,8.02096489941695,68.8648919268133));
#174589=CARTESIAN_POINT('Ctrl Pts',(1.33087977954765,8.01558193538709,68.8635774219933));
#174590=CARTESIAN_POINT('Ctrl Pts',(1.38110339077879,8.0070314898736,68.8615700017127));
#174591=CARTESIAN_POINT('Ctrl Pts',(1.39851482991532,8.00400875372883,68.8608746620199));
#174592=CARTESIAN_POINT('Ctrl Pts',(1.43239101391131,7.99801371967724,68.8595229167905));
#174593=CARTESIAN_POINT('Ctrl Pts',(1.44885665619311,7.99504733374806,68.8588664002883));
#174594=CARTESIAN_POINT('Ctrl Pts',(1.46536577108706,7.99202044055815,68.8582085848539));
#174595=CARTESIAN_POINT('Ctrl Pts',(1.46541849174124,7.99201077385633,68.8582064841728));
#174596=CARTESIAN_POINT('Ctrl Pts',(1.46552380950545,7.99199146202823,68.858202287742));
#174597=CARTESIAN_POINT('Ctrl Pts',(1.46557640685287,7.99198181686093,68.8582001919829));
#174598=CARTESIAN_POINT('Ctrl Pts',(1.46568147969507,7.9919625477992,68.8581960053289));
#174599=CARTESIAN_POINT('Ctrl Pts',(1.46573395515897,7.99195292391292,68.8581939144351));
#174600=CARTESIAN_POINT('Ctrl Pts',(1.46583878540066,7.99193369720672,68.8581897374651));
#174601=CARTESIAN_POINT('Ctrl Pts',(1.46589114021679,7.99192409438223,68.8581876513873));
#174602=CARTESIAN_POINT('Ctrl Pts',(1.46599573060775,7.99190490954192,68.8581834839917));
#174603=CARTESIAN_POINT('Ctrl Pts',(1.46604796609892,7.99189532754387,68.8581814026771));
#174604=CARTESIAN_POINT('Ctrl Pts',(1.4661523191496,7.99187618412347,68.8581772447557));
#174605=CARTESIAN_POINT('Ctrl Pts',(1.46620443660733,7.99186662272217,68.8581751681529));
#174606=CARTESIAN_POINT('Ctrl Pts',(1.46630855482179,7.99184752027662,68.8581710196058));
#174607=CARTESIAN_POINT('Ctrl Pts',(1.46636055549897,7.99183797924932,68.8581689476647));
#174608=CARTESIAN_POINT('Ctrl Pts',(1.46646444154669,7.99181891730299,68.8581648083854));
#174609=CARTESIAN_POINT('Ctrl Pts',(1.46651632681758,7.99180939640456,68.8581627410511));
#174610=CARTESIAN_POINT('Ctrl Pts',(1.46661998268906,7.99179037460616,68.8581586109602));
#174611=CARTESIAN_POINT('Ctrl Pts',(1.46667175352282,7.9917808736657,68.8581565481942));
#174612=CARTESIAN_POINT('Ctrl Pts',(1.46677518263982,7.99176189140107,68.8581524271552));
#174613=CARTESIAN_POINT('Ctrl Pts',(1.46682684065998,7.99175241012745,68.8581503688927));
#174614=CARTESIAN_POINT('Ctrl Pts',(1.466930044307,7.99173346717444,68.8581462568544));
#174615=CARTESIAN_POINT('Ctrl Pts',(1.46698159033408,7.99172400542382,68.8581442030626));
#174616=CARTESIAN_POINT('Ctrl Pts',(1.46708457196305,7.99170510116225,68.8581400998872));
#174617=CARTESIAN_POINT('Ctrl Pts',(1.46713600741592,7.99169565868086,68.8581380505095));
#174618=CARTESIAN_POINT('Ctrl Pts',(1.46723876914309,7.99167679273547,68.8581339561127));
#174619=CARTESIAN_POINT('Ctrl Pts',(1.46729009532673,7.99166736929029,68.8581319110971));
#174620=CARTESIAN_POINT('Ctrl Pts',(1.46739263923941,7.99164854129095,68.8581278253954));
#174621=CARTESIAN_POINT('Ctrl Pts',(1.46744385723238,7.99163913669046,68.8581257846989));
#174622=CARTESIAN_POINT('Ctrl Pts',(1.46754618581056,7.99162034619471,68.8581217075936));
#174623=CARTESIAN_POINT('Ctrl Pts',(1.46759729666251,7.99161096025259,68.8581196711743));
#174624=CARTESIAN_POINT('Ctrl Pts',(1.46769941264952,7.9915922067694,68.8581156025559));
#174625=CARTESIAN_POINT('Ctrl Pts',(1.46775041764299,7.99158283925644,68.8581135703625));
#174626=CARTESIAN_POINT('Ctrl Pts',(1.46785232332801,7.99156412237797,68.8581095101397));
#174627=CARTESIAN_POINT('Ctrl Pts',(1.46790322378515,7.99155477305758,68.8581074821196));
#174628=CARTESIAN_POINT('Ctrl Pts',(1.46800492100919,7.99153609245808,68.858103430219));
#174629=CARTESIAN_POINT('Ctrl Pts',(1.46805571791023,7.99152676115637,68.8581014063331));
#174630=CARTESIAN_POINT('Ctrl Pts',(1.46815720941942,7.99150811634365,68.858097362645));
#174631=CARTESIAN_POINT('Ctrl Pts',(1.46820790399562,7.99149880284052,68.8580953428442));
#174632=CARTESIAN_POINT('Ctrl Pts',(1.46830919178887,7.99148019345943,68.858091307289));
#174633=CARTESIAN_POINT('Ctrl Pts',(1.46835978505242,7.99147089757492,68.8580892915328));
#174634=CARTESIAN_POINT('Ctrl Pts',(1.4684608719172,7.99145232312524,68.8580852639993));
#174635=CARTESIAN_POINT('Ctrl Pts',(1.46851136525732,7.99144304461001,68.8580832522324));
#174636=CARTESIAN_POINT('Ctrl Pts',(1.46861225274046,7.99142450481927,68.8580792326588));
#174637=CARTESIAN_POINT('Ctrl Pts',(1.46866264708611,7.99141524350846,68.8580772248441));
#174638=CARTESIAN_POINT('Ctrl Pts',(1.46876333781327,7.99139673790576,68.8580732131258));
#174639=CARTESIAN_POINT('Ctrl Pts',(1.468813634279,7.9913874936003,68.8580712092189));
#174640=CARTESIAN_POINT('Ctrl Pts',(1.46891413041804,7.99136902179866,68.8580672052694));
#174641=CARTESIAN_POINT('Ctrl Pts',(1.46896433005693,7.9913597943107,68.8580652052282));
#174642=CARTESIAN_POINT('Ctrl Pts',(1.46906463404821,7.99134135587287,68.8580612089501));
#174643=CARTESIAN_POINT('Ctrl Pts',(1.46911473808841,7.99133214498226,68.8580592127256));
#174644=CARTESIAN_POINT('Ctrl Pts',(1.4692148519933,7.99131373954044,68.8580552240368));
#174645=CARTESIAN_POINT('Ctrl Pts',(1.46926486165812,7.99130454502781,68.8580532315803));
#174646=CARTESIAN_POINT('Ctrl Pts',(1.46936478718811,7.99128617227837,68.8580492504124));
#174647=CARTESIAN_POINT('Ctrl Pts',(1.46941470336609,7.99127699398584,68.8580472616885));
#174648=CARTESIAN_POINT('Ctrl Pts',(1.46951444294607,7.99125865349378,68.8580432879448));
#174649=CARTESIAN_POINT('Ctrl Pts',(1.46956426659665,7.99124949125033,68.8580413029151));
#174650=CARTESIAN_POINT('Ctrl Pts',(1.46966382280698,7.99123118255187,68.8580373364927));
#174651=CARTESIAN_POINT('Ctrl Pts',(1.46971355520909,7.99122203612762,68.8580353551063));
#174652=CARTESIAN_POINT('Ctrl Pts',(1.46981292962969,7.99120375894277,68.8580313959421));
#174653=CARTESIAN_POINT('Ctrl Pts',(1.4698625717242,7.99119462816994,68.8580294181615));
#174654=CARTESIAN_POINT('Ctrl Pts',(1.469961766682,7.99117638208116,68.8580254661628));
#174655=CARTESIAN_POINT('Ctrl Pts',(1.47001131950453,7.99116726677443,68.8580234919465));
#174656=CARTESIAN_POINT('Ctrl Pts',(1.47011033726559,7.99114905137518,68.858019547023));
#174657=CARTESIAN_POINT('Ctrl Pts',(1.47015980200424,7.99113995132111,68.8580175763238));
#174658=CARTESIAN_POINT('Ctrl Pts',(1.47025864426745,7.991121766309,68.8580136384076));
#174659=CARTESIAN_POINT('Ctrl Pts',(1.47030802186855,7.99111268133854,68.8580116711876));
#174660=CARTESIAN_POINT('Ctrl Pts',(1.47040669086932,7.99109452631231,68.8580077401897));
#174661=CARTESIAN_POINT('Ctrl Pts',(1.47045598235759,7.99108545624189,68.8580057764081));
#174662=CARTESIAN_POINT('Ctrl Pts',(1.47055448006977,7.99106733084824,68.8580018522496));
#174663=CARTESIAN_POINT('Ctrl Pts',(1.47060368638651,7.99105827550955,68.8579998918689));
#174664=CARTESIAN_POINT('Ctrl Pts',(1.47070201509097,7.99104017933849,68.8579959744589));
#174665=CARTESIAN_POINT('Ctrl Pts',(1.47075113733859,7.9910311385335,68.8579940174351));
#174666=CARTESIAN_POINT('Ctrl Pts',(1.47084929892892,7.99101307124614,68.8579901066981));
#174667=CARTESIAN_POINT('Ctrl Pts',(1.47089833816698,7.9910040447846,68.857988152989));
#174668=CARTESIAN_POINT('Ctrl Pts',(1.47099633439392,7.99098600606819,68.8579842488551));
#174669=CARTESIAN_POINT('Ctrl Pts',(1.47104529147504,7.99097699379789,68.8579822984266));
#174670=CARTESIAN_POINT('Ctrl Pts',(1.47114312476577,7.99095898321498,68.8579784007991));
#174671=CARTESIAN_POINT('Ctrl Pts',(1.47119200082598,7.99094998493142,68.857976453606));
#174672=CARTESIAN_POINT('Ctrl Pts',(1.47128967285355,7.99093200218324,68.8579725624181));
#174673=CARTESIAN_POINT('Ctrl Pts',(1.47133846886116,7.99092301771272,68.8579706184217));
#174674=CARTESIAN_POINT('Ctrl Pts',(1.47143598152897,7.99090506245792,68.8579667335976));
#174675=CARTESIAN_POINT('Ctrl Pts',(1.47148469837034,7.99089609164177,68.8579647927625));
#174676=CARTESIAN_POINT('Ctrl Pts',(1.47158205389726,7.99087816348075,68.8579609142136));
#174677=CARTESIAN_POINT('Ctrl Pts',(1.47163069262779,7.99086920612907,68.8579589764979));
#174678=CARTESIAN_POINT('Ctrl Pts',(1.47172789262735,7.99085130477353,68.8579551041598));
#174679=CARTESIAN_POINT('Ctrl Pts',(1.47177645405722,7.99084236074151,68.8579531695311));
#174680=CARTESIAN_POINT('Ctrl Pts',(1.47187350094922,7.99082448575452,68.8579493033074));
#174681=CARTESIAN_POINT('Ctrl Pts',(1.47192198622288,7.9908155548357,68.85794737172));
#174682=CARTESIAN_POINT('Ctrl Pts',(1.47201888142288,7.99079770596513,68.8579435115543));
#174683=CARTESIAN_POINT('Ctrl Pts',(1.47206729136785,7.99078878801136,68.8579415829752));
#174684=CARTESIAN_POINT('Ctrl Pts',(1.47216403713483,7.99077096484954,68.8579377287773));
#174685=CARTESIAN_POINT('Ctrl Pts',(1.47221237281052,7.99076205966986,68.8579358031644));
#174686=CARTESIAN_POINT('Ctrl Pts',(1.47230897074345,7.99074426193059,68.8579319548706));
#174687=CARTESIAN_POINT('Ctrl Pts',(1.47235723302641,7.99073536936765,68.8579300321887));
#174688=CARTESIAN_POINT('Ctrl Pts',(1.47245368517003,7.99071759668244,68.8579261897175));
#174689=CARTESIAN_POINT('Ctrl Pts',(1.47250187504069,7.99070871655967,68.8579242699277));
#174690=CARTESIAN_POINT('Ctrl Pts',(1.47259818306337,7.99069096862921,68.8579204332125));
#174691=CARTESIAN_POINT('Ctrl Pts',(1.47264630134839,7.99068210079834,68.8579185162818));
#174692=CARTESIAN_POINT('Ctrl Pts',(1.47274246731365,7.99066437725036,68.8579146852403));
#174693=CARTESIAN_POINT('Ctrl Pts',(1.4727905149483,7.99065552154298,68.8579127711314));
#174694=CARTESIAN_POINT('Ctrl Pts',(1.47288654070747,7.99063782204418,68.8579089456898));
#174695=CARTESIAN_POINT('Ctrl Pts',(1.47293451864807,7.99062897828795,68.8579070343645));
#174696=CARTESIAN_POINT('Ctrl Pts',(1.47303040614765,7.9906113024873,68.8579032144452));
#174697=CARTESIAN_POINT('Ctrl Pts',(1.47307831550587,7.99060247048116,68.8579013058593));
#174698=CARTESIAN_POINT('Ctrl Pts',(1.47317406575616,7.99058481820011,68.857897491422));
#174699=CARTESIAN_POINT('Ctrl Pts',(1.47322190703322,7.99057599785548,68.8578955855553));
#174700=CARTESIAN_POINT('Ctrl Pts',(1.47331752296717,7.99055836856085,68.8578917764831));
#174701=CARTESIAN_POINT('Ctrl Pts',(1.47336529738919,7.99054955965541,68.8578898732869));
#174702=CARTESIAN_POINT('Ctrl Pts',(1.47346078006895,7.99053195315882,68.8578860695374));
#174703=CARTESIAN_POINT('Ctrl Pts',(1.47350848845103,7.99052315554596,68.8578841689791));
#174704=CARTESIAN_POINT('Ctrl Pts',(1.47360383959436,7.990505571538,68.8578803704838));
#174705=CARTESIAN_POINT('Ctrl Pts',(1.47365148260562,7.99049678509799,68.8578784725368));
#174706=CARTESIAN_POINT('Ctrl Pts',(1.47374670470366,7.99047922312647,68.8578746791964));
#174707=CARTESIAN_POINT('Ctrl Pts',(1.47379428351258,7.99047044764739,68.857872783814));
#174708=CARTESIAN_POINT('Ctrl Pts',(1.47388937762626,7.99045290752376,68.8578689955862));
#174709=CARTESIAN_POINT('Ctrl Pts',(1.47393689298121,7.99044414287112,68.8578671027387));
#174710=CARTESIAN_POINT('Ctrl Pts',(1.47403186113397,7.99042662422917,68.8578633195427));
#174711=CARTESIAN_POINT('Ctrl Pts',(1.47407931392535,7.99041787024219,68.8578614291945));
#174712=CARTESIAN_POINT('Ctrl Pts',(1.47417415777903,7.99040037278226,68.8578576509642));
#174713=CARTESIAN_POINT('Ctrl Pts',(1.47422154883355,7.99039162931187,68.8578557630824));
#174714=CARTESIAN_POINT('Ctrl Pts',(1.4743162703113,7.99037415268596,68.857851989741));
#174715=CARTESIAN_POINT('Ctrl Pts',(1.47436360060736,7.99036541955501,68.8578501042866));
#174716=CARTESIAN_POINT('Ctrl Pts',(1.47445820106574,7.99034796351952,68.8578463357801));
#174717=CARTESIAN_POINT('Ctrl Pts',(1.47450547132981,7.9903392405973,68.857844452724));
#174718=CARTESIAN_POINT('Ctrl Pts',(1.49288185894259,7.98694802258996,68.8571124131317));
#174719=CARTESIAN_POINT('Ctrl Pts',(1.51119932016105,7.98350246306801,68.8563832422862));
#174720=CARTESIAN_POINT('Ctrl Pts',(1.55546114101503,7.97501891430162,68.8546223212223));
#174721=CARTESIAN_POINT('Ctrl Pts',(1.58139312247707,7.96991730470969,68.853591492964));
#174722=CARTESIAN_POINT('Ctrl Pts',(1.65170706747173,7.95572772528308,68.8507980196084));
#174723=CARTESIAN_POINT('Ctrl Pts',(1.69603876069255,7.94639493275195,68.849038506292));
#174724=CARTESIAN_POINT('Ctrl Pts',(1.84292256960197,7.91418750140257,68.8432101401496));
#174725=CARTESIAN_POINT('Ctrl Pts',(1.94510929488157,7.88969438350205,68.8391575098413));
#174726=CARTESIAN_POINT('Ctrl Pts',(2.36154539459447,7.78129633786341,68.8225906315874));
#174727=CARTESIAN_POINT('Ctrl Pts',(2.67109307344107,7.68054232349897,68.8101392688014));
#174728=CARTESIAN_POINT('Ctrl Pts',(3.03429394351043,7.53770375575407,68.7950031265807));
#174729=CARTESIAN_POINT('Ctrl Pts',(3.09453230953841,7.51317425415586,68.7924754702189));
#174730=CARTESIAN_POINT('Ctrl Pts',(3.19023663475632,7.47285648895061,68.7884297585868));
#174731=CARTESIAN_POINT('Ctrl Pts',(3.22589529380331,7.45753266372646,68.7869156704604));
#174732=CARTESIAN_POINT('Ctrl Pts',(3.29251281890573,7.42833747619856,68.7840740483638));
#174733=CARTESIAN_POINT('Ctrl Pts',(3.32349728312093,7.41452656095403,68.7827470659134));
#174734=CARTESIAN_POINT('Ctrl Pts',(3.3547245645171,7.40037234132297,68.7814041705394));
#174735=CARTESIAN_POINT('Ctrl Pts',(3.35505482968569,7.40022261717816,68.7813899672191));
#174736=CARTESIAN_POINT('Ctrl Pts',(3.35571081124885,7.39992517811352,68.7813617549607));
#174737=CARTESIAN_POINT('Ctrl Pts',(3.35603652789243,7.39977746380677,68.7813477460289));
#174738=CARTESIAN_POINT('Ctrl Pts',(3.35668349730532,7.39948400808205,68.7813199189465));
#174739=CARTESIAN_POINT('Ctrl Pts',(3.35700475036275,7.39933826723619,68.7813061008));
#174740=CARTESIAN_POINT('Ctrl Pts',(3.35764287582884,7.39904872277399,68.7812786517574));
#174741=CARTESIAN_POINT('Ctrl Pts',(3.3579597484739,7.3989049197308,68.7812650208671));
#174742=CARTESIAN_POINT('Ctrl Pts',(3.35858919449595,7.39861921597219,68.7812379428836));
#174743=CARTESIAN_POINT('Ctrl Pts',(3.35890176811458,7.39847731580591,68.7812244957954));
#174744=CARTESIAN_POINT('Ctrl Pts',(3.35952269566285,7.39819538364034,68.7811977820384));
#174745=CARTESIAN_POINT('Ctrl Pts',(3.35983104986385,7.39805535215586,68.7811845153729));
#174746=CARTESIAN_POINT('Ctrl Pts',(3.3604436165455,7.39777712385026,68.7811581591512));
#174747=CARTESIAN_POINT('Ctrl Pts',(3.36074782925585,7.39763892754274,68.7811450695997));
#174748=CARTESIAN_POINT('Ctrl Pts',(3.36135218925008,7.39736433677668,68.7811190643663));
#174749=CARTESIAN_POINT('Ctrl Pts',(3.36165233673397,7.3972279428258,68.7811061486899));
#174750=CARTESIAN_POINT('Ctrl Pts',(3.36224864085068,7.39695692467045,68.7810804880395));
#174751=CARTESIAN_POINT('Ctrl Pts',(3.36254479770947,7.39682230094311,68.7810677430693));
#174752=CARTESIAN_POINT('Ctrl Pts',(3.36313319352195,7.39655479180632,68.7810424207326));
#174753=CARTESIAN_POINT('Ctrl Pts',(3.36342543271977,7.39642190684766,68.7810298433688));
#174754=CARTESIAN_POINT('Ctrl Pts',(3.4060567742504,7.37703383311753,68.7791950079598));
#174755=CARTESIAN_POINT('Ctrl Pts',(3.44822964998529,7.35741552327589,68.7773695894421));
#174756=CARTESIAN_POINT('Ctrl Pts',(3.59006026043245,7.28995031233638,68.7711948094611));
#174757=CARTESIAN_POINT('Ctrl Pts',(3.68890873341837,7.24043232769752,68.7668310458188));
#174758=CARTESIAN_POINT('Ctrl Pts',(3.93610346373034,7.11022403658889,68.7557619955943));
#174759=CARTESIAN_POINT('Ctrl Pts',(4.08300137027764,7.02689799338167,68.7490374499538));
#174760=CARTESIAN_POINT('Ctrl Pts',(4.44541235920284,6.8061212850139,68.7320969216525));
#174761=CARTESIAN_POINT('Ctrl Pts',(4.65723765563184,6.662966027469,68.7218664317003));
#174762=CARTESIAN_POINT('Ctrl Pts',(4.90960813340563,6.47448618992539,68.7093850524794));
#174763=CARTESIAN_POINT('Ctrl Pts',(4.9568592080705,6.43838258485717,68.7070352090695));
#174764=CARTESIAN_POINT('Ctrl Pts',(5.02360181144587,6.38621561044771,68.7037000809295));
#174765=CARTESIAN_POINT('Ctrl Pts',(5.04342119368483,6.37057514330391,68.7027076787084));
#174766=CARTESIAN_POINT('Ctrl Pts',(5.07768947766798,6.34327217549735,68.7009884944066));
#174767=CARTESIAN_POINT('Ctrl Pts',(5.09217183743392,6.33165209915655,68.700260889157));
#174768=CARTESIAN_POINT('Ctrl Pts',(5.12295462150942,6.30677927628258,68.6987119345327));
#174769=CARTESIAN_POINT('Ctrl Pts',(5.13924374350542,6.29351274267405,68.697890837169));
#174770=CARTESIAN_POINT('Ctrl Pts',(5.1555872470373,6.28009615527412,68.6970654281444));
#174771=CARTESIAN_POINT('Ctrl Pts',(5.15569322855992,6.2800091492197,68.6970600756081));
#174772=CARTESIAN_POINT('Ctrl Pts',(5.15590553630268,6.27983484513326,68.6970493529933));
#174773=CARTESIAN_POINT('Ctrl Pts',(5.1560118634934,6.27974754627461,68.6970439828652));
#174774=CARTESIAN_POINT('Ctrl Pts',(5.15622487119661,6.27957264940916,68.6970332246297));
#174775=CARTESIAN_POINT('Ctrl Pts',(5.1563315515814,6.27948505147677,68.6970278365282));
#174776=CARTESIAN_POINT('Ctrl Pts',(5.156545272635,6.27930955065525,68.697017041993));
#174777=CARTESIAN_POINT('Ctrl Pts',(5.15665231330758,6.27922164773185,68.6970116355585));
#174778=CARTESIAN_POINT('Ctrl Pts',(5.15686676228843,6.27904553079711,68.6970008039843));
#174779=CARTESIAN_POINT('Ctrl Pts',(5.15697417051611,6.27895731682004,68.6969953788482));
#174780=CARTESIAN_POINT('Ctrl Pts',(5.15718936183999,6.27878057174157,68.6969845095039));
#174781=CARTESIAN_POINT('Ctrl Pts',(5.15729714490241,6.27869204063525,68.6969790652971));
#174782=CARTESIAN_POINT('Ctrl Pts',(5.15751309320959,6.27851465519246,68.6969681574403));
#174783=CARTESIAN_POINT('Ctrl Pts',(5.15762125846492,6.27842580081388,68.6969626937894));
#174784=CARTESIAN_POINT('Ctrl Pts',(5.15783797836242,6.27824776280772,68.6969517466792));
#174785=CARTESIAN_POINT('Ctrl Pts',(5.15794653311332,6.27815857905661,68.6969462632139));
#174786=CARTESIAN_POINT('Ctrl Pts',(5.15816403977227,6.27797987581868,68.6969352760807));
#174787=CARTESIAN_POINT('Ctrl Pts',(5.15827299159601,6.27789035636617,68.6969297724165));
#174788=CARTESIAN_POINT('Ctrl Pts',(5.15849129966275,6.27771097565327,68.6969187445172));
#174789=CARTESIAN_POINT('Ctrl Pts',(5.15860065596855,6.27762111430554,68.6969132202784));
#174790=CARTESIAN_POINT('Ctrl Pts',(5.15881978092106,6.27744104318508,68.6969021508278));
#174791=CARTESIAN_POINT('Ctrl Pts',(5.15892954942596,6.27735083349231,68.6968966056227));
#174792=CARTESIAN_POINT('Ctrl Pts',(5.18800649302797,6.25345361075834,68.6954276987711));
#174793=CARTESIAN_POINT('Ctrl Pts',(5.2168086270516,6.22944629965759,68.6939676604643));
#174794=CARTESIAN_POINT('Ctrl Pts',(5.28210558538231,6.17424916107911,68.6906447536481));
#174795=CARTESIAN_POINT('Ctrl Pts',(5.31849228133803,6.14293350142099,68.6887837565319));
#174796=CARTESIAN_POINT('Ctrl Pts',(5.43553123371574,6.04038625232833,68.6827634459872));
#174797=CARTESIAN_POINT('Ctrl Pts',(5.51504687034231,5.96787433877879,68.6786195231253));
#174798=CARTESIAN_POINT('Ctrl Pts',(5.74935971908633,5.74551625739629,68.6662059149627));
#174799=CARTESIAN_POINT('Ctrl Pts',(5.8996613873873,5.5910723565407,68.6579659858858));
#174800=CARTESIAN_POINT('Ctrl Pts',(6.14589564198877,5.31705331723577,68.6438313971806));
#174801=CARTESIAN_POINT('Ctrl Pts',(6.24490908088331,5.20040377445726,68.6379526604064));
#174802=CARTESIAN_POINT('Ctrl Pts',(6.4252530284798,4.97535421014705,68.6268252387107));
#174803=CARTESIAN_POINT('Ctrl Pts',(6.50728041476446,4.8675791932999,68.6215835161743));
#174804=CARTESIAN_POINT('Ctrl Pts',(6.63600402948093,4.68937773932993,68.6130394889167));
#174805=CARTESIAN_POINT('Ctrl Pts',(6.68436302244405,4.62018440568612,68.6097509392193));
#174806=CARTESIAN_POINT('Ctrl Pts',(6.76009305283663,4.50814949090166,68.6044699526556));
#174807=CARTESIAN_POINT('Ctrl Pts',(6.78815553460128,4.46578261135981,68.6024827005488));
#174808=CARTESIAN_POINT('Ctrl Pts',(6.84449976555352,4.37895951116253,68.5984296651954));
#174809=CARTESIAN_POINT('Ctrl Pts',(6.87275025218304,4.3344858276652,68.5963637782265));
#174810=CARTESIAN_POINT('Ctrl Pts',(6.93139591858326,4.24014718693536,68.5920027948546));
#174811=CARTESIAN_POINT('Ctrl Pts',(6.96169011666517,4.19022293451664,68.5897072406829));
#174812=CARTESIAN_POINT('Ctrl Pts',(7.00735887954088,4.11309917103806,68.5861798497595));
#174813=CARTESIAN_POINT('Ctrl Pts',(7.02311916856769,4.08613024735513,68.5849498667983));
#174814=CARTESIAN_POINT('Ctrl Pts',(7.07722596024238,3.99230514915065,68.5806828966483));
#174815=CARTESIAN_POINT('Ctrl Pts',(7.11477641183433,3.92499481180254,68.5776429897638));
#174816=CARTESIAN_POINT('Ctrl Pts',(7.24831491145606,3.67740793101818,68.5665410162272));
#174817=CARTESIAN_POINT('Ctrl Pts',(7.33845478342522,3.49406351712362,68.5584701306853));
#174818=CARTESIAN_POINT('Ctrl Pts',(7.43548303308128,3.27634617986965,68.5490947127222));
#174819=CARTESIAN_POINT('Ctrl Pts',(7.44917855609185,3.24508722105226,68.5477535867909));
#174820=CARTESIAN_POINT('Ctrl Pts',(7.47705193014619,3.18036207357472,68.5449872780222));
#174821=CARTESIAN_POINT('Ctrl Pts',(7.49120296097507,3.14688523636605,68.543562440069));
#174822=CARTESIAN_POINT('Ctrl Pts',(7.52066919614788,3.07585229118556,68.5405512278604));
#174823=CARTESIAN_POINT('Ctrl Pts',(7.53592875312049,3.03827423292664,68.5389652197135));
#174824=CARTESIAN_POINT('Ctrl Pts',(7.57487957637518,2.9402552895227,68.534844624304));
#174825=CARTESIAN_POINT('Ctrl Pts',(7.59812900545402,2.87964188948989,68.5323125717301));
#174826=CARTESIAN_POINT('Ctrl Pts',(7.68342064584085,2.64905164434503,68.5227305708916));
#174827=CARTESIAN_POINT('Ctrl Pts',(7.74050542177605,2.47729757651487,68.5156958446344));
#174828=CARTESIAN_POINT('Ctrl Pts',(7.82077818122245,2.20580046442253,68.5046598428428));
#174829=CARTESIAN_POINT('Ctrl Pts',(7.84789708810768,2.10728219182212,68.5006723989076));
#174830=CARTESIAN_POINT('Ctrl Pts',(7.88615138613055,1.95731206573724,68.4946185195247));
#174831=CARTESIAN_POINT('Ctrl Pts',(7.8986567719548,1.90622018308294,68.4925588976306));
#174832=CARTESIAN_POINT('Ctrl Pts',(7.92233418071596,1.8052482237899,68.4884926036413));
#174833=CARTESIAN_POINT('Ctrl Pts',(7.93353336705345,1.75537697194322,68.4864861717446));
#174834=CARTESIAN_POINT('Ctrl Pts',(7.95545027779596,1.65328168089871,68.4823814780289));
#174835=CARTESIAN_POINT('Ctrl Pts',(7.96612607420632,1.6010511496219,68.4802830756631));
#174836=CARTESIAN_POINT('Ctrl Pts',(7.99001105265801,1.47803762170106,68.4753431823402));
#174837=CARTESIAN_POINT('Ctrl Pts',(8.00279485494536,1.40717670504677,68.4724993422498));
#174838=CARTESIAN_POINT('Ctrl Pts',(8.0881702828961,0.895070953656037,68.451952704868));
#174839=CARTESIAN_POINT('Ctrl Pts',(8.12516511525461,0.448681294685467,
68.4340257735927));
#174840=CARTESIAN_POINT('Ctrl Pts',(8.12524985409108,0.00153983533466129,
68.4161556904274));
#174841=CARTESIAN_POINT('',(8.12524976787349,0.00315471203378172,64.4160553597947));
#174842=CARTESIAN_POINT('Ctrl Pts',(8.12524985424774,0.00153900849306533,
68.4161556573826));
#174843=CARTESIAN_POINT('Ctrl Pts',(8.12528237179811,-0.170138550527305,
68.4092945351027));
#174844=CARTESIAN_POINT('Ctrl Pts',(8.11987384283798,-0.341777092234551,
68.4024537844651));
#174845=CARTESIAN_POINT('Ctrl Pts',(8.10701627146785,-0.544971023882323,
68.3944096543118));
#174846=CARTESIAN_POINT('Ctrl Pts',(8.10481302331182,-0.576812024049769,
68.3931507326559));
#174847=CARTESIAN_POINT('Ctrl Pts',(8.10078293599201,-0.630461975753339,
68.3910326129349));
#174848=CARTESIAN_POINT('Ctrl Pts',(8.09905549502474,-0.652277986337368,
68.3901721681756));
#174849=CARTESIAN_POINT('Ctrl Pts',(8.0956879270921,-0.692729758567754,
68.3885784377277));
#174850=CARTESIAN_POINT('Ctrl Pts',(8.09407153657532,-0.711367341657171,
68.3878448295472));
#174851=CARTESIAN_POINT('Ctrl Pts',(8.09061230082685,-0.749714626254643,
68.3863369087451));
#174852=CARTESIAN_POINT('Ctrl Pts',(8.08876176397404,-0.769423519400977,
68.3855627149282));
#174853=CARTESIAN_POINT('Ctrl Pts',(8.08453844555367,-0.812703450460102,
68.3838645289267));
#174854=CARTESIAN_POINT('Ctrl Pts',(8.08213456390817,-0.836271291250548,
68.3829410391522));
#174855=CARTESIAN_POINT('Ctrl Pts',(8.07245465411354,-0.927231385424134,
68.3793808909721));
#174856=CARTESIAN_POINT('Ctrl Pts',(8.06443845589282,-0.994542450136126,
68.3767549491114));
#174857=CARTESIAN_POINT('Ctrl Pts',(8.05060544007279,-1.09949505721077,
68.3726671091484));
#174858=CARTESIAN_POINT('Ctrl Pts',(8.04536468118677,-1.1372090807838,68.3711995072183));
#174859=CARTESIAN_POINT('Ctrl Pts',(7.99945485684791,-1.45137474617261,
68.3589791156529));
#174860=CARTESIAN_POINT('Ctrl Pts',(7.94481481446527,-1.72559724645603,
68.3483363392331));
#174861=CARTESIAN_POINT('Ctrl Pts',(7.83788003959037,-2.14746140446812,
68.3316412044999));
#174862=CARTESIAN_POINT('Ctrl Pts',(7.79526973845258,-2.29732955351505,
68.3256469802612));
#174863=CARTESIAN_POINT('Ctrl Pts',(7.72685277196014,-2.51406983012027,
68.3168486942218));
#174864=CARTESIAN_POINT('Ctrl Pts',(7.70442831998608,-2.58197309237309,
68.3140735520567));
#174865=CARTESIAN_POINT('Ctrl Pts',(7.67986724905146,-2.65317567027084,
68.3111420947519));
#174866=CARTESIAN_POINT('Ctrl Pts',(7.6786213741955,-2.65677923285041,68.3109936755857));
#174867=CARTESIAN_POINT('Ctrl Pts',(7.67618647920419,-2.66380589201568,
68.3107041563119));
#174868=CARTESIAN_POINT('Ctrl Pts',(7.67499770467241,-2.66722907286134,
68.3105630583767));
#174869=CARTESIAN_POINT('Ctrl Pts',(7.67265798727234,-2.67395197894404,
68.3102858472728));
#174870=CARTESIAN_POINT('Ctrl Pts',(7.67150720478222,-2.67725175923315,
68.3101497355337));
#174871=CARTESIAN_POINT('Ctrl Pts',(7.65951940125848,-2.71155467204993,
68.3087342708662));
#174872=CARTESIAN_POINT('Ctrl Pts',(7.64849665170215,-2.74249250831835,
68.3074533000525));
#174873=CARTESIAN_POINT('Ctrl Pts',(7.62598414968093,-2.80448744221619,
68.3048774178709));
#174874=CARTESIAN_POINT('Ctrl Pts',(7.61449150591817,-2.8355428337931,68.3035825028963));
#174875=CARTESIAN_POINT('Ctrl Pts',(7.58723475371147,-2.90783515408737,
68.3005572421608));
#174876=CARTESIAN_POINT('Ctrl Pts',(7.57132378381058,-2.94901553597965,
68.2988256225012));
#174877=CARTESIAN_POINT('Ctrl Pts',(7.52070865324648,-3.0769061929997,68.2934214048425));
#174878=CARTESIAN_POINT('Ctrl Pts',(7.48484469518878,-3.16314875957572,
68.2897388545074));
#174879=CARTESIAN_POINT('Ctrl Pts',(7.3212545348328,-3.53816585473537,68.2735557268121));
#174880=CARTESIAN_POINT('Ctrl Pts',(7.17824490486902,-3.81997147494461,
68.2609332763151));
#174881=CARTESIAN_POINT('Ctrl Pts',(6.97790492517623,-4.16356246973784,
68.2450940582139));
#174882=CARTESIAN_POINT('Ctrl Pts',(6.9355373091331,-4.23376096600011,68.2418341586656));
#174883=CARTESIAN_POINT('Ctrl Pts',(6.87156676215497,-4.336215284512,68.2370471372909));
#174884=CARTESIAN_POINT('Ctrl Pts',(6.8507836059003,-4.36897662642505,68.2355119437941));
#174885=CARTESIAN_POINT('Ctrl Pts',(6.81281772358389,-4.42788675532222,
68.2327442325536));
#174886=CARTESIAN_POINT('Ctrl Pts',(6.79571709024347,-4.454087526402,68.2315106710721));
#174887=CARTESIAN_POINT('Ctrl Pts',(6.76831536793371,-4.49554596307694,
68.229555075291));
#174888=CARTESIAN_POINT('Ctrl Pts',(6.75811305171226,-4.51086847610355,
68.2288315057182));
#174889=CARTESIAN_POINT('Ctrl Pts',(6.737706362303,-4.541291963691,68.2273933424948));
#174890=CARTESIAN_POINT('Ctrl Pts',(6.72750306847714,-4.55639355102487,
68.2266787381253));
#174891=CARTESIAN_POINT('Ctrl Pts',(6.70484993590334,-4.58967978954676,
68.2251021344501));
#174892=CARTESIAN_POINT('Ctrl Pts',(6.6923767577114,-4.60784836675312,68.2242405590758));
#174893=CARTESIAN_POINT('Ctrl Pts',(6.64894834335656,-4.6705583855664,68.2212628677662));
#174894=CARTESIAN_POINT('Ctrl Pts',(6.61762098529057,-4.71484064012608,
68.2191533299401));
#174895=CARTESIAN_POINT('Ctrl Pts',(6.39191163066633,-5.02720648675815,
68.2042125084047));
#174896=CARTESIAN_POINT('Ctrl Pts',(6.18174124685891,-5.28350466912997,
68.1916299791438));
#174897=CARTESIAN_POINT('Ctrl Pts',(5.8434269320696,-5.64815868404763,68.1727365288103));
#174898=CARTESIAN_POINT('Ctrl Pts',(5.72662288744624,-5.76655226479261,
68.1664276887652));
#174899=CARTESIAN_POINT('Ctrl Pts',(5.35059155554883,-6.12500031618885,
68.1466632182802));
#174900=CARTESIAN_POINT('Ctrl Pts',(5.07929713680077,-6.35178659747735,
68.1331591686982));
#174901=CARTESIAN_POINT('Ctrl Pts',(4.72423193329506,-6.61126398044991,
68.1161094882838));
#174902=CARTESIAN_POINT('Ctrl Pts',(4.6535401965327,-6.6612117730507,68.1127443077749));
#174903=CARTESIAN_POINT('Ctrl Pts',(4.55091880344635,-6.73128873186888,
68.1078982831813));
#174904=CARTESIAN_POINT('Ctrl Pts',(4.51962563584827,-6.7523398943051,68.1064256699359));
#174905=CARTESIAN_POINT('Ctrl Pts',(4.45622553410183,-6.7943514515029,68.1034522069703));
#174906=CARTESIAN_POINT('Ctrl Pts',(4.4241145178227,-6.8153039828961,68.101951332318));
#174907=CARTESIAN_POINT('Ctrl Pts',(4.36211694310375,-6.85513477839087,
68.0990631826074));
#174908=CARTESIAN_POINT('Ctrl Pts',(4.33225310799632,-6.87404684701336,
68.0976762180631));
#174909=CARTESIAN_POINT('Ctrl Pts',(4.26116988288377,-6.91841497431566,
68.0943847644017));
#174910=CARTESIAN_POINT('Ctrl Pts',(4.21984439854455,-6.94369842078232,
68.0924789995474));
#174911=CARTESIAN_POINT('Ctrl Pts',(4.06728370560869,-7.03517198171976,
68.0854715048558));
#174912=CARTESIAN_POINT('Ctrl Pts',(3.95469796582418,-7.0990707289956,68.0803541086279));
#174913=CARTESIAN_POINT('Ctrl Pts',(3.47688779510555,-7.35535977581938,
68.0588569931837));
#174914=CARTESIAN_POINT('Ctrl Pts',(3.09881441516549,-7.52245985305122,
68.0423935515526));
#174915=CARTESIAN_POINT('Ctrl Pts',(2.21016307782089,-7.83681167644055,
68.0037393787933));
#174916=CARTESIAN_POINT('Ctrl Pts',(1.6945644242408,-7.96422242321409,67.9812694531593));
#174917=CARTESIAN_POINT('Ctrl Pts',(0.921593806983284,-8.07672619712227,
67.9482699891821));
#174918=CARTESIAN_POINT('Ctrl Pts',(0.67135801296593,-8.1013656798774,67.9377170400963));
#174919=CARTESIAN_POINT('Ctrl Pts',(0.352061973250933,-8.1179073393984,
67.9246595686243));
#174920=CARTESIAN_POINT('Ctrl Pts',(0.283702650057588,-8.12058374054772,
67.9218881940336));
#174921=CARTESIAN_POINT('Ctrl Pts',(0.187527340314437,-8.12313325342106,
67.9180299109739));
#174922=CARTESIAN_POINT('Ctrl Pts',(0.15973414087787,-8.12372730844027,
67.9169197177845));
#174923=CARTESIAN_POINT('Ctrl Pts',(0.111169665544383,-8.12451600502814,
67.9149887947233));
#174924=CARTESIAN_POINT('Ctrl Pts',(0.0903997446909679,-8.12477365261168,
67.914165850343));
#174925=CARTESIAN_POINT('Ctrl Pts',(0.0600104991025161,-8.12503408140102,
67.9129661809404));
#174926=CARTESIAN_POINT('Ctrl Pts',(0.0503918816739662,-8.12509942974085,
67.9125871155027));
#174927=CARTESIAN_POINT('Ctrl Pts',(0.0335144987093047,-8.12518412284654,
67.9119231459339));
#174928=CARTESIAN_POINT('Ctrl Pts',(0.0262557905068431,-8.1252108210004,
67.9116379592979));
#174929=CARTESIAN_POINT('Ctrl Pts',(0.0121661504554965,-8.12524376302789,
67.911085136558));
#174930=CARTESIAN_POINT('Ctrl Pts',(0.00533522940645123,-8.12525111978136,
67.9108174570436));
#174931=CARTESIAN_POINT('Ctrl Pts',(-0.0109660751142631,-8.12524811901701,
67.9101794894724));
#174932=CARTESIAN_POINT('Ctrl Pts',(-0.0204364602350505,-8.12522981844067,
67.9098095191954));
#174933=CARTESIAN_POINT('Ctrl Pts',(-0.0542969048736042,-8.12510518658287,
67.9084891472156));
#174934=CARTESIAN_POINT('Ctrl Pts',(-0.0786866475893341,-8.12490559181954,
67.9075425714146));
#174935=CARTESIAN_POINT('Ctrl Pts',(-0.512123510969814,-8.11940665590536,
67.8908050070238));
#174936=CARTESIAN_POINT('Ctrl Pts',(-0.920202038761973,-8.08333301032376,
67.8765166026161));
#174937=CARTESIAN_POINT('Ctrl Pts',(-1.67960378625187,-7.95792978515934,
67.8504518717959));
#174938=CARTESIAN_POINT('Ctrl Pts',(-2.03107546700232,-7.87556046562825,
67.8385918448277));
#174939=CARTESIAN_POINT('Ctrl Pts',(-2.93263516201177,-7.59988518097128,
67.8068520556476));
#174940=CARTESIAN_POINT('Ctrl Pts',(-3.46938307923615,-7.37033869787014,
67.7865082791149));
#174941=CARTESIAN_POINT('Ctrl Pts',(-4.00173824143169,-7.07153341752101,
67.7629940937613));
#174942=CARTESIAN_POINT('Ctrl Pts',(-4.02642609084264,-7.05750570269801,
67.761895992281));
#174943=CARTESIAN_POINT('Ctrl Pts',(-4.06225479286396,-7.03689853169093,
67.7602910874559));
#174944=CARTESIAN_POINT('Ctrl Pts',(-4.07345437557699,-7.03042135264311,
67.7597878039503));
#174945=CARTESIAN_POINT('Ctrl Pts',(-4.093045280803,-7.0190285986269,67.7589045955394));
#174946=CARTESIAN_POINT('Ctrl Pts',(-4.10144335032669,-7.0141246483289,
67.758525072208));
#174947=CARTESIAN_POINT('Ctrl Pts',(-4.11770548553439,-7.00458938050265,
67.7577883739759));
#174948=CARTESIAN_POINT('Ctrl Pts',(-4.12557059474589,-6.99995986575535,
67.7574312617242));
#174949=CARTESIAN_POINT('Ctrl Pts',(-4.1442861747106,-6.98890111050983,
67.7565795483498));
#174950=CARTESIAN_POINT('Ctrl Pts',(-4.15512949370236,-6.98245984730412,
67.7560845310902));
#174951=CARTESIAN_POINT('Ctrl Pts',(-4.19364163322253,-6.95946098004096,
67.7543208191451));
#174952=CARTESIAN_POINT('Ctrl Pts',(-4.22122666817874,-6.94276405096403,
67.7530472891322));
#174953=CARTESIAN_POINT('Ctrl Pts',(-4.67677196270482,-6.66330874395816,
67.7318444279279));
#174954=CARTESIAN_POINT('Ctrl Pts',(-5.07951291141891,-6.36162888214538,
67.710488533981));
#174955=CARTESIAN_POINT('Ctrl Pts',(-5.64190296136223,-5.85272167400217,
67.6769527046995));
#174956=CARTESIAN_POINT('Ctrl Pts',(-5.82375524306836,-5.67179777825154,
67.6654332765996));
#174957=CARTESIAN_POINT('Ctrl Pts',(-6.36389153071405,-5.08100700429423,
67.6294739318485));
#174958=CARTESIAN_POINT('Ctrl Pts',(-6.68983719728844,-4.64349362207447,
67.605100792816));
#174959=CARTESIAN_POINT('Ctrl Pts',(-6.97934853272343,-4.16037732323915,
67.5825268228573));
#174960=CARTESIAN_POINT('Ctrl Pts',(-6.98901572345644,-4.14411687078104,
67.581771489877));
#174961=CARTESIAN_POINT('Ctrl Pts',(-7.00628165217253,-4.11484289567279,
67.580419388186));
#174962=CARTESIAN_POINT('Ctrl Pts',(-7.01390111922076,-4.10184174969319,
67.5798216205588));
#174963=CARTESIAN_POINT('Ctrl Pts',(-7.0260047268843,-4.0810569500542,67.5788702148473));
#174964=CARTESIAN_POINT('Ctrl Pts',(-7.03051218262687,-4.07328696541042,
67.5785154929436));
#174965=CARTESIAN_POINT('Ctrl Pts',(-7.03838572416256,-4.05966249401794,
67.5778951214279));
#174966=CARTESIAN_POINT('Ctrl Pts',(-7.04175740807506,-4.05381126516518,
67.5776292173625));
#174967=CARTESIAN_POINT('Ctrl Pts',(-7.04936853689389,-4.04056474474278,
67.5770284107597));
#174968=CARTESIAN_POINT('Ctrl Pts',(-7.05360365082833,-4.03316696444838,
67.5766937020005));
#174969=CARTESIAN_POINT('Ctrl Pts',(-7.06501154578945,-4.01316703892286,
67.5757910058133));
#174970=CARTESIAN_POINT('Ctrl Pts',(-7.07216226468644,-4.00055230307849,
67.5752239841448));
#174971=CARTESIAN_POINT('Ctrl Pts',(-7.10393023166592,-3.94415839453911,
67.5726993125262));
#174972=CARTESIAN_POINT('Ctrl Pts',(-7.12817529161501,-3.90017016480807,
67.5707573579752));
#174973=CARTESIAN_POINT('Ctrl Pts',(-7.15512691781651,-3.85018044470134,
67.5685784957784));
#174974=CARTESIAN_POINT('Ctrl Pts',(-7.15823562059561,-3.84439767286311,
67.5683268683799));
#174975=CARTESIAN_POINT('Ctrl Pts',(-7.19074635742421,-3.78374543566969,
67.5656920521144));
#174976=CARTESIAN_POINT('Ctrl Pts',(-7.21952429242536,-3.72854286372604,
67.5633313505425));
#174977=CARTESIAN_POINT('Ctrl Pts',(-7.30448361988949,-3.56089942096104,
67.5562610450679));
#174978=CARTESIAN_POINT('Ctrl Pts',(-7.3586938873596,-3.44747894752531,
67.5516100735348));
#174979=CARTESIAN_POINT('Ctrl Pts',(-7.55990469990789,-3.00010651399587,
67.5336431996009));
#174980=CARTESIAN_POINT('Ctrl Pts',(-7.68697892380179,-2.65766123365706,
67.520677545651));
#174981=CARTESIAN_POINT('Ctrl Pts',(-7.92752083770743,-1.84565710448643,
67.4901801584177));
#174982=CARTESIAN_POINT('Ctrl Pts',(-8.02302685049483,-1.37224137682229,
67.4725395280405));
#174983=CARTESIAN_POINT('Ctrl Pts',(-8.08285062260947,-0.831315734765007,
67.4517599623032));
#174984=CARTESIAN_POINT('Ctrl Pts',(-8.08898033100149,-0.76938751113298,
67.449373280676));
#174985=CARTESIAN_POINT('Ctrl Pts',(-8.09875036260817,-0.657593560786433,
67.4450504339902));
#174986=CARTESIAN_POINT('Ctrl Pts',(-8.10264296999869,-0.607752891722415,
67.4431180653179));
#174987=CARTESIAN_POINT('Ctrl Pts',(-8.10786522389545,-0.531872765917759,
67.4401683223207));
#174988=CARTESIAN_POINT('Ctrl Pts',(-8.10952991239581,-0.505857411798655,
67.4391556173412));
#174989=CARTESIAN_POINT('Ctrl Pts',(-8.11236055631888,-0.458008525922321,
67.4372904597392));
#174990=CARTESIAN_POINT('Ctrl Pts',(-8.11356363657743,-0.436177390521669,
67.436438514337));
#174991=CARTESIAN_POINT('Ctrl Pts',(-8.11573929955384,-0.393568105432536,
67.434773824817));
#174992=CARTESIAN_POINT('Ctrl Pts',(-8.11672024076189,-0.372790506428888,
67.4339611826753));
#174993=CARTESIAN_POINT('Ctrl Pts',(-8.11911203607947,-0.317633774258172,
67.4318014025331));
#174994=CARTESIAN_POINT('Ctrl Pts',(-8.12038431223899,-0.28324913788809,
67.4304523994076));
#174995=CARTESIAN_POINT('Ctrl Pts',(-8.12418770521429,-0.159125849185185,
67.4255723975308));
#174996=CARTESIAN_POINT('Ctrl Pts',(-8.12544991887554,-0.0693556589142267,
67.422023492796));
#174997=CARTESIAN_POINT('Ctrl Pts',(-8.12364523334291,0.648873426885906,
67.3934434558375));
#174998=CARTESIAN_POINT('Ctrl Pts',(-8.04915847923988,1.27498319445882,
67.3671476166185));
#174999=CARTESIAN_POINT('Ctrl Pts',(-7.80688433222686,2.2901336481186,67.3228579568412));
#175000=CARTESIAN_POINT('Ctrl Pts',(-7.67964844082461,2.6861077945585,67.3052027981136));
#175001=CARTESIAN_POINT('Ctrl Pts',(-7.50307558741761,3.11869198044984,
67.2863626793351));
#175002=CARTESIAN_POINT('Ctrl Pts',(-7.48299505549403,3.16657039627257,
67.2842844535992));
#175003=CARTESIAN_POINT('Ctrl Pts',(-7.45690258042211,3.22714867952234,
67.2816664668417));
#175004=CARTESIAN_POINT('Ctrl Pts',(-7.45131495144626,3.24002935031666,
67.2811104730396));
#175005=CARTESIAN_POINT('Ctrl Pts',(-7.44232244705243,3.26061268448294,
67.2802231245441));
#175006=CARTESIAN_POINT('Ctrl Pts',(-7.43893894735494,3.26832462008929,
67.2798909171762));
#175007=CARTESIAN_POINT('Ctrl Pts',(-7.43251301171878,3.28290943913169,
67.2792631452908));
#175008=CARTESIAN_POINT('Ctrl Pts',(-7.42947301845861,3.28978338547856,
67.2789674813435));
#175009=CARTESIAN_POINT('Ctrl Pts',(-7.42257632304926,3.30531968211885,
67.2782997202027));
#175010=CARTESIAN_POINT('Ctrl Pts',(-7.41871398279387,3.313979528444,67.2779278588823));
#175011=CARTESIAN_POINT('Ctrl Pts',(-7.40733106292205,3.33938182212979,
67.2768381140802));
#175012=CARTESIAN_POINT('Ctrl Pts',(-7.39976887360642,3.35610563809094,
67.2761220146158));
#175013=CARTESIAN_POINT('Ctrl Pts',(-7.3442575638069,3.47776938096674,67.2709229699835));
#175014=CARTESIAN_POINT('Ctrl Pts',(-7.29413864732273,3.58169533223031,
67.2665464193172));
#175015=CARTESIAN_POINT('Ctrl Pts',(-6.92624758302988,4.3047725925774,67.2364877210908));
#175016=CARTESIAN_POINT('Ctrl Pts',(-6.5322776545076,4.88195575864787,67.2141925393082));
#175017=CARTESIAN_POINT('Ctrl Pts',(-5.72851076755715,5.78506503095518,
67.1729244295603));
#175018=CARTESIAN_POINT('Ctrl Pts',(-5.35200186662086,6.13504840745117,
67.1547320846952));
#175019=CARTESIAN_POINT('Ctrl Pts',(-4.92273492565188,6.46429875265236,
67.1338894137622));
#175020=CARTESIAN_POINT('Ctrl Pts',(-4.90034498303991,6.48128818525221,
67.1328023098433));
#175021=CARTESIAN_POINT('Ctrl Pts',(-4.86756380388422,6.50589549297222,
67.1312105824569));
#175022=CARTESIAN_POINT('Ctrl Pts',(-4.8572417819325,6.51360543941619,67.1307093714129));
#175023=CARTESIAN_POINT('Ctrl Pts',(-4.83910306677747,6.52708690627988,
67.1298285649592));
#175024=CARTESIAN_POINT('Ctrl Pts',(-4.83129426495378,6.53286902498781,
67.1294493617748));
#175025=CARTESIAN_POINT('Ctrl Pts',(-4.81611834134668,6.54406412402888,
67.1287123749738));
#175026=CARTESIAN_POINT('Ctrl Pts',(-4.80875241648433,6.5494787070103,67.1283546511884));
#175027=CARTESIAN_POINT('Ctrl Pts',(-4.79115549978447,6.56236825297716,
67.1275000255716));
#175028=CARTESIAN_POINT('Ctrl Pts',(-4.78091614438116,6.56983172763534,
67.1270027032725));
#175029=CARTESIAN_POINT('Ctrl Pts',(-4.74427406650383,6.59640914370292,
67.1252228816519));
#175030=CARTESIAN_POINT('Ctrl Pts',(-4.71777400173205,6.61538800433101,
67.1239354528301));
#175031=CARTESIAN_POINT('Ctrl Pts',(-4.26146317939659,6.93805316163785,
67.1017613747089));
#175032=CARTESIAN_POINT('Ctrl Pts',(-3.80331990871621,7.19939476466031,
67.0793045265722));
#175033=CARTESIAN_POINT('Ctrl Pts',(-3.07124324612625,7.52750801859559,
67.0436601736648));
#175034=CARTESIAN_POINT('Ctrl Pts',(-2.81371562270016,7.62751013974738,
67.0311853636322));
#175035=CARTESIAN_POINT('Ctrl Pts',(-2.23350135862769,7.81942576983251,
67.0036286497536));
#175036=CARTESIAN_POINT('Ctrl Pts',(-1.90918175208397,7.90487132480282,
66.988583617878));
#175037=CARTESIAN_POINT('Ctrl Pts',(-1.50483030809981,7.9850563451124,66.970841124326));
#175038=CARTESIAN_POINT('Ctrl Pts',(-1.42894622558409,7.99898445276284,
66.9675550811182));
#175039=CARTESIAN_POINT('Ctrl Pts',(-1.26057291326981,8.02741588921456,
66.9603748289545));
#175040=CARTESIAN_POINT('Ctrl Pts',(-1.16800677360788,8.0414060445731,66.9565009404886));
#175041=CARTESIAN_POINT('Ctrl Pts',(-1.02180670860129,8.06092439468,66.9505169889738));
#175042=CARTESIAN_POINT('Ctrl Pts',(-0.968327462287127,8.0675233480576,
66.9483570071883));
#175043=CARTESIAN_POINT('Ctrl Pts',(-0.901075449670824,8.07514340375013,
66.9456732948217));
#175044=CARTESIAN_POINT('Ctrl Pts',(-0.887360828707382,8.07666197881792,
66.9451276958735));
#175045=CARTESIAN_POINT('Ctrl Pts',(-0.865554460247878,8.07902031299955,
66.9442627790811));
#175046=CARTESIAN_POINT('Ctrl Pts',(-0.857465243867065,8.0798828641092,
66.9439424987562));
#175047=CARTESIAN_POINT('Ctrl Pts',(-0.842241128180823,8.08148308758662,
66.9433407663423));
#175048=CARTESIAN_POINT('Ctrl Pts',(-0.835106525419513,8.08222346292072,
66.9430592025743));
#175049=CARTESIAN_POINT('Ctrl Pts',(-0.819083943237819,8.0838647232487,
66.9424278287786));
#175050=CARTESIAN_POINT('Ctrl Pts',(-0.810195431557844,8.08476040049189,
66.9420782308996));
#175051=CARTESIAN_POINT('Ctrl Pts',(-0.787598524540116,8.08699980532536,
66.9411910908572));
#175052=CARTESIAN_POINT('Ctrl Pts',(-0.773888125860028,8.08832334039418,
66.9406543523265));
#175053=CARTESIAN_POINT('Ctrl Pts',(-0.697694262053483,8.09548321688525,
66.9376796439581));
#175054=CARTESIAN_POINT('Ctrl Pts',(-0.635147207728117,8.10063047358791,
66.9352681500204));
#175055=CARTESIAN_POINT('Ctrl Pts',(0.168378862335905,8.15739204640914,
66.904612617782));
#175056=CARTESIAN_POINT('Ctrl Pts',(0.913042336930171,8.10789647634058,
66.8792462508587));
#175057=CARTESIAN_POINT('Ctrl Pts',(1.93143524335923,7.89793545264935,66.8411471898703));
#175058=CARTESIAN_POINT('Ctrl Pts',(2.21868846126042,7.82209940607559,66.8300713915483));
#175059=CARTESIAN_POINT('Ctrl Pts',(2.76815282729282,7.64432964409433,66.808134051918));
#175060=CARTESIAN_POINT('Ctrl Pts',(3.03050839307999,7.54416725991463,66.7973378179631));
#175061=CARTESIAN_POINT('Ctrl Pts',(3.35722349828693,7.39963577098459,66.7834777094646));
#175062=CARTESIAN_POINT('Ctrl Pts',(3.42685684990023,7.36764624488402,66.7804969147674));
#175063=CARTESIAN_POINT('Ctrl Pts',(3.53498910736567,7.3161056924747,66.7758230250501));
#175064=CARTESIAN_POINT('Ctrl Pts',(3.57380252720547,7.29722453882304,66.7741361565688));
#175065=CARTESIAN_POINT('Ctrl Pts',(3.64605904881325,7.26135990660095,66.7709779944127));
#175066=CARTESIAN_POINT('Ctrl Pts',(3.67953859658884,7.24445235914449,66.7695074528438));
#175067=CARTESIAN_POINT('Ctrl Pts',(3.75432431601573,7.20603256776671,66.7662059383096));
#175068=CARTESIAN_POINT('Ctrl Pts',(3.79556497944784,7.1843957922146,66.7643738154981));
#175069=CARTESIAN_POINT('Ctrl Pts',(3.91606353853653,7.11984948401743,66.7589858665454));
#175070=CARTESIAN_POINT('Ctrl Pts',(3.9947958291383,7.07597459109165,66.7554208248923));
#175071=CARTESIAN_POINT('Ctrl Pts',(4.61584434226886,6.71621537012863,66.7269272717926));
#175072=CARTESIAN_POINT('Ctrl Pts',(5.12062435597174,6.33977408667381,66.7013594027734));
#175073=CARTESIAN_POINT('Ctrl Pts',(5.70083759731357,5.79216076383939,66.6690256663079));
#175074=CARTESIAN_POINT('Ctrl Pts',(5.82095447296992,5.67143419109782,66.6621515817681));
#175075=CARTESIAN_POINT('Ctrl Pts',(5.98111482082203,5.50000842620154,66.6527607321199));
#175076=CARTESIAN_POINT('Ctrl Pts',(6.02447930591811,5.45247433561489,66.6501940450774));
#175077=CARTESIAN_POINT('Ctrl Pts',(6.09875713143947,5.36908645007551,66.6457578067695));
#175078=CARTESIAN_POINT('Ctrl Pts',(6.12993011411289,5.33346835557321,66.6438834202816));
#175079=CARTESIAN_POINT('Ctrl Pts',(6.17530749811607,5.28069698466522,66.6411371328361));
#175080=CARTESIAN_POINT('Ctrl Pts',(6.18975533884231,5.26375457191609,66.6402600296525));
#175081=CARTESIAN_POINT('Ctrl Pts',(6.21609387538912,5.23261001498598,66.6386561856895));
#175082=CARTESIAN_POINT('Ctrl Pts',(6.2280059656783,5.21842623125739,66.6379289514342));
#175083=CARTESIAN_POINT('Ctrl Pts',(6.25477770937037,5.18632674848314,66.636290085895));
#175084=CARTESIAN_POINT('Ctrl Pts',(6.26960910197254,5.16838766440655,66.6353790382456));
#175085=CARTESIAN_POINT('Ctrl Pts',(6.30791479290245,5.12164807629578,66.6330173878932));
#175086=CARTESIAN_POINT('Ctrl Pts',(6.33126903934526,5.0927497899076,66.6315690019332));
#175087=CARTESIAN_POINT('Ctrl Pts',(6.49067129220682,4.89271599919196,66.6216188195317));
#175088=CARTESIAN_POINT('Ctrl Pts',(6.61996362658758,4.71630864829569,66.6132184609574));
#175089=CARTESIAN_POINT('Ctrl Pts',(6.84009164238777,4.38904683280956,66.5980576517333));
#175090=CARTESIAN_POINT('Ctrl Pts',(6.9334388927404,4.24004841252845,66.5913032211815));
#175091=CARTESIAN_POINT('Ctrl Pts',(7.07767457367433,3.99230603314086,66.5802320487235));
#175092=CARTESIAN_POINT('Ctrl Pts',(7.13150126140866,3.89534008052208,66.5759373569923));
#175093=CARTESIAN_POINT('Ctrl Pts',(7.20524250760718,3.7558443976771,66.5698017332538));
#175094=CARTESIAN_POINT('Ctrl Pts',(7.22679945369571,3.71419659773013,66.5679752323476));
#175095=CARTESIAN_POINT('Ctrl Pts',(7.26399454420735,3.64078618166893,66.5647643115575));
#175096=CARTESIAN_POINT('Ctrl Pts',(7.27978791652459,3.60910357834949,66.5633813049974));
#175097=CARTESIAN_POINT('Ctrl Pts',(7.31241338045087,3.54256912553104,66.5604823963732));
#175098=CARTESIAN_POINT('Ctrl Pts',(7.32920451778435,3.50769818811195,66.5589661686231));
#175099=CARTESIAN_POINT('Ctrl Pts',(7.37324690396006,3.41453627810188,66.5549231781983));
#175100=CARTESIAN_POINT('Ctrl Pts',(7.40005587672126,3.35603946070945,66.5523926111522));
#175101=CARTESIAN_POINT('Ctrl Pts',(7.56533041145752,2.98380091849978,66.5363372753369));
#175102=CARTESIAN_POINT('Ctrl Pts',(7.68450946102702,2.66187903549099,66.5226431027337));
#175103=CARTESIAN_POINT('Ctrl Pts',(7.83512182606183,2.15951533923086,66.5016970093936));
#175104=CARTESIAN_POINT('Ctrl Pts',(7.88141179793418,1.98393285100065,66.4944568374496));
#175105=CARTESIAN_POINT('Ctrl Pts',(7.93145751486333,1.7645288671942,66.4855625941377));
#175106=CARTESIAN_POINT('Ctrl Pts',(7.94079210969303,1.72203401078657,66.4838470465938));
#175107=CARTESIAN_POINT('Ctrl Pts',(7.95431498374099,1.65802322615973,66.4812747143047));
#175108=CARTESIAN_POINT('Ctrl Pts',(7.95875820721297,1.63656215374422,66.4804143018794));
#175109=CARTESIAN_POINT('Ctrl Pts',(7.96707320447535,1.59556533448844,66.4787745163987));
#175110=CARTESIAN_POINT('Ctrl Pts',(7.97096007350897,1.57603289680016,66.4779948997055));
#175111=CARTESIAN_POINT('Ctrl Pts',(7.97976232870652,1.53093387838883,66.4761983843436));
#175112=CARTESIAN_POINT('Ctrl Pts',(7.98462673092698,1.50535754454683,66.475182191451));
#175113=CARTESIAN_POINT('Ctrl Pts',(7.99750618916814,1.43582001312951,66.4724259462639));
#175114=CARTESIAN_POINT('Ctrl Pts',(8.00528167202,1.3918152665049,66.4706888922711));
#175115=CARTESIAN_POINT('Ctrl Pts',(8.05157034817105,1.11661778278855,66.4598640027488));
#175116=CARTESIAN_POINT('Ctrl Pts',(8.08042845631781,0.883910871926848,
66.4508764259574));
#175117=CARTESIAN_POINT('Ctrl Pts',(8.11659211714811,0.433495816651327,
66.4335543104261));
#175118=CARTESIAN_POINT('Ctrl Pts',(8.12528685465822,0.216100174615363,
66.4252264970346));
#175119=CARTESIAN_POINT('Ctrl Pts',(8.12521409019402,-0.211923570187139,
66.4087511185072));
#175120=CARTESIAN_POINT('Ctrl Pts',(8.11699493825367,-0.422382964632793,
66.4006125534617));
#175121=CARTESIAN_POINT('Ctrl Pts',(8.09538390981195,-0.699256483068275,
66.3898052595378));
#175122=CARTESIAN_POINT('Ctrl Pts',(8.08932606281942,-0.766161911063918,
66.3871861588197));
#175123=CARTESIAN_POINT('Ctrl Pts',(8.07676727611018,-0.888019704309546,
66.382400906296));
#175124=CARTESIAN_POINT('Ctrl Pts',(8.07053331029202,-0.942995592617735,
66.3802364799513));
#175125=CARTESIAN_POINT('Ctrl Pts',(8.05643536843777,-1.05691655480052,
66.3757393629398));
#175126=CARTESIAN_POINT('Ctrl Pts',(8.04848479322796,-1.11584763840538,
66.3734063245012));
#175127=CARTESIAN_POINT('Ctrl Pts',(8.0236705920712,-1.28568315175161,66.366663100997));
#175128=CARTESIAN_POINT('Ctrl Pts',(8.00515628565184,-1.39633220505732,
66.3622455509408));
#175129=CARTESIAN_POINT('Ctrl Pts',(7.96560317565574,-1.60595261680053,
66.3538327016816));
#175130=CARTESIAN_POINT('Ctrl Pts',(7.94499505202998,-1.70498426553291,
66.3498393545942));
#175131=CARTESIAN_POINT('Ctrl Pts',(7.89078443591569,-1.94311063898959,
66.3401975497372));
#175132=CARTESIAN_POINT('Ctrl Pts',(7.85534604560827,-2.08175327420229,
66.3345506808625));
#175133=CARTESIAN_POINT('Ctrl Pts',(7.80378797100673,-2.26333107199899,
66.3271268925674));
#175134=CARTESIAN_POINT('Ctrl Pts',(7.79094019770234,-2.3071681975563,66.3253324659611));
#175135=CARTESIAN_POINT('Ctrl Pts',(7.76524205126199,-2.39218819962183,
66.3218490623778));
#175136=CARTESIAN_POINT('Ctrl Pts',(7.75243201312976,-2.43338167807495,
66.3201598926861));
#175137=CARTESIAN_POINT('Ctrl Pts',(7.70626740455601,-2.57776868670368,
66.3142313315006));
#175138=CARTESIAN_POINT('Ctrl Pts',(7.67117540937297,-2.68039487733141,
66.3100031626101));
#175139=CARTESIAN_POINT('Ctrl Pts',(7.56586223670502,-2.96935306622828,
66.2980227777913));
#175140=CARTESIAN_POINT('Ctrl Pts',(7.49083224236327,-3.15384863120235,
66.2902819749781));
#175141=CARTESIAN_POINT('Ctrl Pts',(7.37643109916493,-3.4079738740167,66.2794060088474));
#175142=CARTESIAN_POINT('Ctrl Pts',(7.34269625096009,-3.4800622686869,66.2762962317874));
#175143=CARTESIAN_POINT('Ctrl Pts',(7.28367215345462,-3.60151102884986,
66.2710103044029));
#175144=CARTESIAN_POINT('Ctrl Pts',(7.25892666212905,-3.65112933474513,
66.2688372431872));
#175145=CARTESIAN_POINT('Ctrl Pts',(7.20607788168896,-3.75443751282017,
66.2642827663701));
#175146=CARTESIAN_POINT('Ctrl Pts',(7.17787789358002,-3.80807410429185,
66.2619008915859));
#175147=CARTESIAN_POINT('Ctrl Pts',(7.09808609249884,-3.95580277367275,
66.2552901750498));
#175148=CARTESIAN_POINT('Ctrl Pts',(7.04522653103298,-4.04919555946854,
66.2510534063102));
#175149=CARTESIAN_POINT('Ctrl Pts',(6.9215124827327,-4.25801466173364,66.2414413001707));
#175150=CARTESIAN_POINT('Ctrl Pts',(6.84959071805755,-4.3727714922219,66.2360597871468));
#175151=CARTESIAN_POINT('Ctrl Pts',(6.53770099839623,-4.84382672177588,
66.2135404342653));
#175152=CARTESIAN_POINT('Ctrl Pts',(6.2725408675276,-5.18260759031173,66.1962574664917));
#175153=CARTESIAN_POINT('Ctrl Pts',(5.9340245562,-5.55085881413701,66.1764179372877));
#175154=CARTESIAN_POINT('Ctrl Pts',(5.88552494959952,-5.60225643702847,
66.173623663906));
#175155=CARTESIAN_POINT('Ctrl Pts',(5.81819010225182,-5.67177517281152,
66.1698122825605));
#175156=CARTESIAN_POINT('Ctrl Pts',(5.79992899526413,-5.69044755125468,
66.1687853421284));
#175157=CARTESIAN_POINT('Ctrl Pts',(5.76840539906206,-5.72237172808484,
66.1670242276754));
#175158=CARTESIAN_POINT('Ctrl Pts',(5.75518650853229,-5.73566624700747,
66.1662892149316));
#175159=CARTESIAN_POINT('Ctrl Pts',(5.72778720485934,-5.76303222101129,
66.1647729869279));
#175160=CARTESIAN_POINT('Ctrl Pts',(5.71360065269636,-5.77709738806742,
66.1639919078419));
#175161=CARTESIAN_POINT('Ctrl Pts',(5.67769241136163,-5.81243673973807,
66.162025014844));
#175162=CARTESIAN_POINT('Ctrl Pts',(5.65590289376746,-5.83364161049239,
66.1608407218886));
#175163=CARTESIAN_POINT('Ctrl Pts',(5.55067145053681,-5.93490572302008,
66.155163386764));
#175164=CARTESIAN_POINT('Ctrl Pts',(5.46564512663863,-6.01330053341449,
66.1507021741328));
#175165=CARTESIAN_POINT('Ctrl Pts',(5.15134202941808,-6.29091442219426,
66.1345828077174));
#175166=CARTESIAN_POINT('Ctrl Pts',(4.91261590221555,-6.47905357528902,
66.1230221806197));
#175167=CARTESIAN_POINT('Ctrl Pts',(4.54107957367375,-6.73949461958504,
66.1055822575981));
#175168=CARTESIAN_POINT('Ctrl Pts',(4.41588098621987,-6.82218336721901,
66.0997942969035));
#175169=CARTESIAN_POINT('Ctrl Pts',(4.24308419578413,-6.92955834317883,
66.0918973619693));
#175170=CARTESIAN_POINT('Ctrl Pts',(4.19742538294049,-6.95731000049822,
66.0898192229814));
#175171=CARTESIAN_POINT('Ctrl Pts',(4.1232537544949,-7.00139596624113,66.0864560319566));
#175172=CARTESIAN_POINT('Ctrl Pts',(4.094909689487,-7.01801123014745,66.0851737748835));
#175173=CARTESIAN_POINT('Ctrl Pts',(4.03525291537851,-7.05249752029697,
66.0824809209811));
#175174=CARTESIAN_POINT('Ctrl Pts',(4.00392046844352,-7.07033296499898,
66.0810700107101));
#175175=CARTESIAN_POINT('Ctrl Pts',(3.92796405792192,-7.11290298887246,
66.0776576076076));
#175176=CARTESIAN_POINT('Ctrl Pts',(3.88322388049436,-7.13742690554507,
66.0756541715074));
#175177=CARTESIAN_POINT('Ctrl Pts',(3.71135679690996,-7.2295399099169,66.0679822541809));
#175178=CARTESIAN_POINT('Ctrl Pts',(3.58267349414296,-7.29416661469247,
66.0622874990506));
#175179=CARTESIAN_POINT('Ctrl Pts',(3.17560203757542,-7.48523188214039,
66.0444301608095));
#175180=CARTESIAN_POINT('Ctrl Pts',(2.89175369627808,-7.59940154113746,
66.0321913243133));
#175181=CARTESIAN_POINT('Ctrl Pts',(2.53477966330553,-7.72008011783607,
66.0172307782375));
#175182=CARTESIAN_POINT('Ctrl Pts',(2.46711333358603,-7.74196983099114,
66.0144142150904));
#175183=CARTESIAN_POINT('Ctrl Pts',(2.37525429729774,-7.77035913429486,
66.0106207974673));
#175184=CARTESIAN_POINT('Ctrl Pts',(2.35130643850876,-7.77763923633915,
66.0096346003467));
#175185=CARTESIAN_POINT('Ctrl Pts',(2.31033218790532,-7.78988878722828,
66.0079521948445));
#175186=CARTESIAN_POINT('Ctrl Pts',(2.29332248590119,-7.79491334870117,
66.0072552298158));
#175187=CARTESIAN_POINT('Ctrl Pts',(2.25821560996518,-7.8051588440548,66.005819850931));
#175188=CARTESIAN_POINT('Ctrl Pts',(2.24011645835406,-7.8103726274337,66.0050815573951));
#175189=CARTESIAN_POINT('Ctrl Pts',(2.19475620293195,-7.82326881469741,
66.0032356071258));
#175190=CARTESIAN_POINT('Ctrl Pts',(2.16747275199456,-7.83087170219616,
66.0021291939289));
#175191=CARTESIAN_POINT('Ctrl Pts',(2.05507102089112,-7.86156146807002,
65.997586096076));
#175192=CARTESIAN_POINT('Ctrl Pts',(1.96961876925467,-7.88340457949319,
65.9941677224519));
#175193=CARTESIAN_POINT('Ctrl Pts',(1.39816802030431,-8.01960581908799,
65.9714986999136));
#175194=CARTESIAN_POINT('Ctrl Pts',(0.902866426919166,-8.09035209126938,
65.9527310908568));
#175195=CARTESIAN_POINT('Ctrl Pts',(0.290640563331582,-8.12084633362458,
65.929376276916));
#175196=CARTESIAN_POINT('Ctrl Pts',(0.176967400717827,-8.1241183801935,
65.9250352451172));
#175197=CARTESIAN_POINT('Ctrl Pts',(-0.17221644250915,-8.12683722238152,
65.9116611181454));
#175198=CARTESIAN_POINT('Ctrl Pts',(-0.407661965790738,-8.11843279466399,
65.9025865897993));
#175199=CARTESIAN_POINT('Ctrl Pts',(-0.709506812354297,-8.09449308979185,
65.8908154373219));
#175200=CARTESIAN_POINT('Ctrl Pts',(-0.776537880727611,-8.08833772507705,
65.8881928263365));
#175201=CARTESIAN_POINT('Ctrl Pts',(-0.884513901156566,-8.07706781409081,
65.8839532090205));
#175202=CARTESIAN_POINT('Ctrl Pts',(-0.925510025313442,-8.07247300978378,
65.8823400203701));
#175203=CARTESIAN_POINT('Ctrl Pts',(-1.00406236014561,-8.06306268486193,
65.879242034595));
#175204=CARTESIAN_POINT('Ctrl Pts',(-1.04162342017547,-8.05829645291117,
65.8777576197378));
#175205=CARTESIAN_POINT('Ctrl Pts',(-1.12860651991741,-8.04664058980043,
65.8743127481626));
#175206=CARTESIAN_POINT('Ctrl Pts',(-1.17800110157287,-8.03955787588657,
65.8723510553864));
#175207=CARTESIAN_POINT('Ctrl Pts',(-1.33886403808096,-8.01497732958864,
65.8659441085504));
#175208=CARTESIAN_POINT('Ctrl Pts',(-1.45003325117336,-7.99561266216185,
65.8614875386447));
#175209=CARTESIAN_POINT('Ctrl Pts',(-2.14166742442192,-7.86023707560376,
65.8335770948069));
#175210=CARTESIAN_POINT('Ctrl Pts',(-2.70838026960999,-7.68340436469641,
65.8098940618716));
#175211=CARTESIAN_POINT('Ctrl Pts',(-3.55252128438107,-7.31489158181805,
65.77150808314));
#175212=CARTESIAN_POINT('Ctrl Pts',(-3.8459185068589,-7.16498073331512,
65.7575626268181));
#175213=CARTESIAN_POINT('Ctrl Pts',(-4.46864879847514,-6.79750156815182,
65.7269634608765));
#175214=CARTESIAN_POINT('Ctrl Pts',(-4.79289827014357,-6.57289871458698,
65.7103468082767));
#175215=CARTESIAN_POINT('Ctrl Pts',(-5.11649168966103,-6.31202598791034,
65.6938132369453));
#175216=CARTESIAN_POINT('Ctrl Pts',(-5.13334579690712,-6.29832677960305,
65.6929523697108));
#175217=CARTESIAN_POINT('Ctrl Pts',(-5.15705283204414,-6.27889906091169,
65.6917420926312));
#175218=CARTESIAN_POINT('Ctrl Pts',(-5.16395147489601,-6.27322664147535,
65.6913899820534));
#175219=CARTESIAN_POINT('Ctrl Pts',(-5.17651930719527,-6.26285794337134,
65.6907486711045));
#175220=CARTESIAN_POINT('Ctrl Pts',(-5.18219148882733,-6.25816531662345,
65.6904592902064));
#175221=CARTESIAN_POINT('Ctrl Pts',(-5.19360646722319,-6.24869548203223,
65.6898770583545));
#175222=CARTESIAN_POINT('Ctrl Pts',(-5.19934906997312,-6.24391804979842,
65.689584219249));
#175223=CARTESIAN_POINT('Ctrl Pts',(-5.21335235794006,-6.23223560787106,
65.6888703166078));
#175224=CARTESIAN_POINT('Ctrl Pts',(-5.22160593682087,-6.22532207376202,
65.6884496962123));
#175225=CARTESIAN_POINT('Ctrl Pts',(-5.25102079105293,-6.20058333940167,
65.6869512847883));
#175226=CARTESIAN_POINT('Ctrl Pts',(-5.27210488589027,-6.18266634995624,
65.6858784212792));
#175227=CARTESIAN_POINT('Ctrl Pts',(-5.69304264548774,-5.82123992251527,
65.6644900534577));
#175228=CARTESIAN_POINT('Ctrl Pts',(-6.05863507432376,-5.43971904231667,
65.6466661385943));
#175229=CARTESIAN_POINT('Ctrl Pts',(-6.57424450685164,-4.78465457191867,
65.6188089320896));
#175230=CARTESIAN_POINT('Ctrl Pts',(-6.75001803475049,-4.53330615418877,
65.6086603655937));
#175231=CARTESIAN_POINT('Ctrl Pts',(-7.17801341021492,-3.84100494506177,
65.581007867879));
#175232=CARTESIAN_POINT('Ctrl Pts',(-7.40380680392797,-3.38537584130643,
65.5630447193436));
#175233=CARTESIAN_POINT('Ctrl Pts',(-7.59726689937952,-2.88136740909345,
65.5422913732803));
#175234=CARTESIAN_POINT('Ctrl Pts',(-7.60872398657461,-2.85097557929176,
65.5410370420098));
#175235=CARTESIAN_POINT('Ctrl Pts',(-7.62439017416096,-2.80865129463363,
65.5392860452217));
#175236=CARTESIAN_POINT('Ctrl Pts',(-7.62875415348125,-2.79677630258508,
65.5387943090215));
#175237=CARTESIAN_POINT('Ctrl Pts',(-7.63622197236423,-2.77630780585556,
65.5379459249085));
#175238=CARTESIAN_POINT('Ctrl Pts',(-7.63933908974433,-2.76771915397871,
65.5375896991179));
#175239=CARTESIAN_POINT('Ctrl Pts',(-7.64574211796224,-2.74998354397871,
65.5368535895245));
#175240=CARTESIAN_POINT('Ctrl Pts',(-7.64902611610913,-2.74083591279153,
65.5364736458324));
#175241=CARTESIAN_POINT('Ctrl Pts',(-7.65663102158317,-2.7195322028468,
65.53558815841));
#175242=CARTESIAN_POINT('Ctrl Pts',(-7.66093940027064,-2.70737169714791,
65.5350822195579));
#175243=CARTESIAN_POINT('Ctrl Pts',(-7.67457278516681,-2.66859801109404,
65.5334674653374));
#175244=CARTESIAN_POINT('Ctrl Pts',(-7.68378816868808,-2.64194665709101,
65.532355197167));
#175245=CARTESIAN_POINT('Ctrl Pts',(-7.86539384528741,-2.10774574820757,
65.5100127789457));
#175246=CARTESIAN_POINT('Ctrl Pts',(-7.98725817670137,-1.58448422945002,
65.4871424845212));
#175247=CARTESIAN_POINT('Ctrl Pts',(-8.1323200153023,-0.474689868414925,
65.4374942058783));
#175248=CARTESIAN_POINT('Ctrl Pts',(-8.14541724627627,0.11016935005052,
65.4107024834253));
#175249=CARTESIAN_POINT('Ctrl Pts',(-8.07867718978711,0.891666298386771,
65.3770688398252));
#175250=CARTESIAN_POINT('Ctrl Pts',(-8.05414508560277,1.09126581436165,
65.368694457187));
#175251=CARTESIAN_POINT('Ctrl Pts',(-8.01892898912319,1.31030437846695,
65.3598397965051));
#175252=CARTESIAN_POINT('Ctrl Pts',(-8.01555041022097,1.33081603872916,
65.3590134768446));
#175253=CARTESIAN_POINT('Ctrl Pts',(-8.01047380964964,1.3609157619988,65.3578048528227));
#175254=CARTESIAN_POINT('Ctrl Pts',(-8.00883722825762,1.37051399799154,
65.3574200365076));
#175255=CARTESIAN_POINT('Ctrl Pts',(-8.00589774452284,1.38756843376153,
65.3567373024246));
#175256=CARTESIAN_POINT('Ctrl Pts',(-8.00460167072762,1.39502578743407,
65.3564391115006));
#175257=CARTESIAN_POINT('Ctrl Pts',(-8.00187959949421,1.41055935570605,
65.3558186886657));
#175258=CARTESIAN_POINT('Ctrl Pts',(-8.00045179083238,1.41863524697295,
65.3554965285343));
#175259=CARTESIAN_POINT('Ctrl Pts',(-7.99753086362955,1.43501176898227,
65.3548440274901));
#175260=CARTESIAN_POINT('Ctrl Pts',(-7.99603704325914,1.44331226535306,
65.3545137141916));
#175261=CARTESIAN_POINT('Ctrl Pts',(-7.98998427507912,1.47664699295352,
65.3531887761207));
#175262=CARTESIAN_POINT('Ctrl Pts',(-7.98532063552413,1.50166221996321,
65.3521981297017));
#175263=CARTESIAN_POINT('Ctrl Pts',(-7.97375262244783,1.56213362192292,
65.3498113650114));
#175264=CARTESIAN_POINT('Ctrl Pts',(-7.96672914681945,1.59756661296886,
65.3484195235397));
#175265=CARTESIAN_POINT('Ctrl Pts',(-7.86692894604569,2.08402103143757,
65.3293908341882));
#175266=CARTESIAN_POINT('Ctrl Pts',(-7.73620633673433,2.52643571023312,
65.3129779518931));
#175267=CARTESIAN_POINT('Ctrl Pts',(-7.35803688400547,3.49491385757805,
65.2756551601418));
#175268=CARTESIAN_POINT('Ctrl Pts',(-7.09030629034492,4.01031793990886,
65.2547006226584));
#175269=CARTESIAN_POINT('Ctrl Pts',(-6.72003636824551,4.56825851802383,
65.2291262086479));
#175270=CARTESIAN_POINT('Ctrl Pts',(-6.66874851808954,4.64280815600138,
65.2256480126999));
#175271=CARTESIAN_POINT('Ctrl Pts',(-6.59620316492399,4.74457387976865,
65.2208139647307));
#175272=CARTESIAN_POINT('Ctrl Pts',(-6.57600094180632,4.77253487055945,
65.2194766195567));
#175273=CARTESIAN_POINT('Ctrl Pts',(-6.54332271204319,4.81716190283916,
65.2173274439717));
#175274=CARTESIAN_POINT('Ctrl Pts',(-6.53095960310399,4.83391017410198,
65.2165175143791));
#175275=CARTESIAN_POINT('Ctrl Pts',(-6.50678342642775,4.86639952391509,
65.2149398307756));
#175276=CARTESIAN_POINT('Ctrl Pts',(-6.49497724629585,4.88214557879501,
65.214172202156));
#175277=CARTESIAN_POINT('Ctrl Pts',(-6.46885533116981,4.91672226116835,
65.2124798627619));
#175278=CARTESIAN_POINT('Ctrl Pts',(-6.45451434601867,4.93553357206189,
65.2115547327507));
#175279=CARTESIAN_POINT('Ctrl Pts',(-6.41445567749221,4.98760599982247,
65.2089812793721));
#175280=CARTESIAN_POINT('Ctrl Pts',(-6.38856175005407,5.02073042327874,
65.2073299110334));
#175281=CARTESIAN_POINT('Ctrl Pts',(-6.33043040879614,5.09391621568159,
65.2036482762663));
#175282=CARTESIAN_POINT('Ctrl Pts',(-6.29806750408878,5.13387545892998,
65.2016157237437));
#175283=CARTESIAN_POINT('Ctrl Pts',(-5.97465714367341,5.52553724375952,
65.1814637391716));
#175284=CARTESIAN_POINT('Ctrl Pts',(-5.65485624178699,5.85240525089714,
65.1627293753417));
#175285=CARTESIAN_POINT('Ctrl Pts',(-4.87586664836254,6.52483658010809,
65.1194447066968));
#175286=CARTESIAN_POINT('Ctrl Pts',(-4.40408307581055,6.85212460011129,
65.0946992205918));
#175287=CARTESIAN_POINT('Ctrl Pts',(-3.84855357837986,7.15625678623129,
65.0689230406342));
#175288=CARTESIAN_POINT('Ctrl Pts',(-3.79495697475135,7.18482272543686,
65.0664699839276));
#175289=CARTESIAN_POINT('Ctrl Pts',(-3.71373590099987,7.2269495361896,65.0628079214012));
#175290=CARTESIAN_POINT('Ctrl Pts',(-3.68634691082636,7.24095852932249,
65.0615823896207));
#175291=CARTESIAN_POINT('Ctrl Pts',(-3.64824415396597,7.2601752057576,65.0598910191015));
#175292=CARTESIAN_POINT('Ctrl Pts',(-3.63759768017609,7.26551529791332,
65.0594198856143));
#175293=CARTESIAN_POINT('Ctrl Pts',(-3.62053489209693,7.27402679972451,
65.0586671896804));
#175294=CARTESIAN_POINT('Ctrl Pts',(-3.61412608281881,7.27721316479831,
65.0583850112067));
#175295=CARTESIAN_POINT('Ctrl Pts',(-3.60091268675825,7.28376090943299,
65.0578043417398));
#175296=CARTESIAN_POINT('Ctrl Pts',(-3.59410758244709,7.2871212319881,65.0575058952136));
#175297=CARTESIAN_POINT('Ctrl Pts',(-3.57828924690416,7.29490468957244,
65.056813586907));
#175298=CARTESIAN_POINT('Ctrl Pts',(-3.56927249435045,7.2993206688475,65.0564200307715));
#175299=CARTESIAN_POINT('Ctrl Pts',(-3.5410239304411,7.31309062189298,65.0551904625854));
#175300=CARTESIAN_POINT('Ctrl Pts',(-3.52176326475132,7.32238543361087,
65.0543570364865));
#175301=CARTESIAN_POINT('Ctrl Pts',(-3.35426453493117,7.40240320267688,
65.0471532159475));
#175302=CARTESIAN_POINT('Ctrl Pts',(-3.20395650283865,7.46868973780232,
65.0410087725186));
#175303=CARTESIAN_POINT('Ctrl Pts',(-2.69949267515121,7.67312716574129,
65.0212422503882));
#175304=CARTESIAN_POINT('Ctrl Pts',(-2.33764703225545,7.7909933326566,65.008376930653));
#175305=CARTESIAN_POINT('Ctrl Pts',(-1.71906298429799,7.94548953476738,
64.9869189938467));
#175306=CARTESIAN_POINT('Ctrl Pts',(-1.46643687724503,7.99597042042751,
64.9783012521853));
#175307=CARTESIAN_POINT('Ctrl Pts',(-0.707475819954939,8.11044631883014,
64.9521167343787));
#175308=CARTESIAN_POINT('Ctrl Pts',(-0.197119007150179,8.13885357084496,
64.9340526506436));
#175309=CARTESIAN_POINT('Ctrl Pts',(0.344775467129954,8.11799606352015,
64.9132014133074));
#175310=CARTESIAN_POINT('Ctrl Pts',(0.377033714500188,8.1165618188947,64.9119542311904));
#175311=CARTESIAN_POINT('Ctrl Pts',(0.421886141373222,8.11429965592282,
64.910211686451));
#175312=CARTESIAN_POINT('Ctrl Pts',(0.434488410269032,8.11363461353964,
64.9097211533254));
#175313=CARTESIAN_POINT('Ctrl Pts',(0.456203697186414,8.11243792446836,
64.9088742932131));
#175314=CARTESIAN_POINT('Ctrl Pts',(0.465317478449534,8.11192027421732,
64.9085183819724));
#175315=CARTESIAN_POINT('Ctrl Pts',(0.484137683759807,8.11081949129409,
64.9077824005763));
#175316=CARTESIAN_POINT('Ctrl Pts',(0.493843970354896,8.11023429065843,
64.9074022695735));
#175317=CARTESIAN_POINT('Ctrl Pts',(0.516454981119869,8.10883031128891,
64.9065154395649));
#175318=CARTESIAN_POINT('Ctrl Pts',(0.529358831163944,8.10799814940859,
64.9060083439557));
#175319=CARTESIAN_POINT('Ctrl Pts',(0.570554391291529,8.10524270882468,
64.9043862531092));
#175320=CARTESIAN_POINT('Ctrl Pts',(0.598837900124074,8.10320213446807,
64.9032677768537));
#175321=CARTESIAN_POINT('Ctrl Pts',(1.19545697479929,8.0570170773446,64.8795717415941));
#175322=CARTESIAN_POINT('Ctrl Pts',(1.75751587621444,7.95334038131988,64.8551312043109));
#175323=CARTESIAN_POINT('Ctrl Pts',(2.62510588459359,7.69679208170392,64.8147642484918));
#175324=CARTESIAN_POINT('Ctrl Pts',(2.94000145813439,7.58209572280094,64.7995588971635));
#175325=CARTESIAN_POINT('Ctrl Pts',(3.65023213176778,7.27248710499434,64.7648018577684));
#175326=CARTESIAN_POINT('Ctrl Pts',(4.03866740606205,7.06417368211481,64.7454453496932));
#175327=CARTESIAN_POINT('Ctrl Pts',(4.43308363825827,6.80942894844569,64.7266367975115));
#175328=CARTESIAN_POINT('Ctrl Pts',(4.45771115355224,6.79333235257426,64.7254656118682));
#175329=CARTESIAN_POINT('Ctrl Pts',(4.49175698062641,6.77081506781141,64.7238502475973));
#175330=CARTESIAN_POINT('Ctrl Pts',(4.50124982769582,6.76450792341948,64.7234002464539));
#175331=CARTESIAN_POINT('Ctrl Pts',(4.51641850197298,6.75438363300913,64.7226817825234));
#175332=CARTESIAN_POINT('Ctrl Pts',(4.52210281269807,6.7505792713384,64.7224126794892));
#175333=CARTESIAN_POINT('Ctrl Pts',(4.53380568988196,6.74272542448886,64.721858911851));
#175334=CARTESIAN_POINT('Ctrl Pts',(4.53982365151768,6.73867504760398,64.7215742917754));
#175335=CARTESIAN_POINT('Ctrl Pts',(4.55378358990197,6.7292521514178,64.7209143694076));
#175336=CARTESIAN_POINT('Ctrl Pts',(4.56172150688043,6.72387361538723,64.7205393602484));
#175337=CARTESIAN_POINT('Ctrl Pts',(4.57835700324922,6.71255879673595,64.7197539110081));
#175338=CARTESIAN_POINT('Ctrl Pts',(4.58705260508955,6.70661962901463,64.7193436092958));
#175339=CARTESIAN_POINT('Ctrl Pts',(4.6383984918679,6.67140338926205,64.7169222675484));
#175340=CARTESIAN_POINT('Ctrl Pts',(4.68078048878368,6.64173606134519,64.7149294048499));
#175341=CARTESIAN_POINT('Ctrl Pts',(4.86677868482135,6.50887293516043,64.7061963888022));
#175342=CARTESIAN_POINT('Ctrl Pts',(5.00729134661894,6.40140601812458,64.6996321227779));
#175343=CARTESIAN_POINT('Ctrl Pts',(5.48888260889117,6.00750803362267,64.6768818301142));
#175344=CARTESIAN_POINT('Ctrl Pts',(5.80982237052869,5.69771614418732,64.6611970011749));
#175345=CARTESIAN_POINT('Ctrl Pts',(6.24265027949436,5.20512022940595,64.6375007784001));
#175346=CARTESIAN_POINT('Ctrl Pts',(6.37533831363412,5.04172766620706,64.6298269637827));
#175347=CARTESIAN_POINT('Ctrl Pts',(6.7672236856133,4.51891595382675,64.6056555662988));
#175348=CARTESIAN_POINT('Ctrl Pts',(7.00347298490783,4.1433382764389,64.5887815533345));
#175349=CARTESIAN_POINT('Ctrl Pts',(7.25983449841712,3.65063540870118,64.5673172911544));
#175350=CARTESIAN_POINT('Ctrl Pts',(7.30966788503088,3.549801535146,64.5629553586286));
#175351=CARTESIAN_POINT('Ctrl Pts',(7.37831507482546,3.403319750806,64.5566533604685));
#175352=CARTESIAN_POINT('Ctrl Pts',(7.39883139843843,3.35848367256796,64.554728999357));
#175353=CARTESIAN_POINT('Ctrl Pts',(7.43439306359846,3.27886010707587,64.551318836131));
#175354=CARTESIAN_POINT('Ctrl Pts',(7.44960550853401,3.24414882208678,64.5498346224841));
#175355=CARTESIAN_POINT('Ctrl Pts',(7.47836546326555,3.17725614963081,64.5469786441879));
#175356=CARTESIAN_POINT('Ctrl Pts',(7.49194948211848,3.145091348337,64.5456072525477));
#175357=CARTESIAN_POINT('Ctrl Pts',(7.52071459765309,3.07573617509593,64.5426539458711));
#175358=CARTESIAN_POINT('Ctrl Pts',(7.53582807019887,3.0385187770293,64.5410714420403));
#175359=CARTESIAN_POINT('Ctrl Pts',(7.57175603477389,2.94812798647438,64.5372330910199));
#175360=CARTESIAN_POINT('Ctrl Pts',(7.59228714338808,2.8948443758837,64.5349747086733));
#175361=CARTESIAN_POINT('Ctrl Pts',(7.7769340225401,2.40015713159284,64.514042895066));
#175362=CARTESIAN_POINT('Ctrl Pts',(7.90294210862582,1.94549302343782,64.4950225567952));
#175363=CARTESIAN_POINT('Ctrl Pts',(7.99033216260217,1.47456587650895,64.4755584402205));
#175364=CARTESIAN_POINT('Ctrl Pts',(7.99179170308602,1.46663491276828,64.4752307202717));
#175365=CARTESIAN_POINT('Ctrl Pts',(8.02475806137802,1.28598935728686,64.4677679779035));
#175366=CARTESIAN_POINT('Ctrl Pts',(8.05067070566752,1.1123003414602,64.4606297618435));
#175367=CARTESIAN_POINT('Ctrl Pts',(8.09853278855276,0.700435081823796,
64.4438321144453));
#175368=CARTESIAN_POINT('Ctrl Pts',(8.11563527370661,0.461855513389096,
64.4342021022195));
#175369=CARTESIAN_POINT('Ctrl Pts',(8.12324142796484,0.184654997777823,
64.4232056083949));
#175370=CARTESIAN_POINT('Ctrl Pts',(8.1240202554274,0.146436607636499,64.4216937683884));
#175371=CARTESIAN_POINT('Ctrl Pts',(8.12479443884191,0.0883121799698593,
64.4194014691192));
#175372=CARTESIAN_POINT('Ctrl Pts',(8.12498639216542,0.0684094130669633,
64.4186177988583));
#175373=CARTESIAN_POINT('Ctrl Pts',(8.12516785655924,0.0380128452778828,
64.4174228851264));
#175374=CARTESIAN_POINT('Ctrl Pts',(8.12521017267948,0.0275195205149921,
64.417010732583));
#175375=CARTESIAN_POINT('Ctrl Pts',(8.12524185021268,0.0124023266316113,
64.4164174421896));
#175376=CARTESIAN_POINT('Ctrl Pts',(8.12524759234423,0.00777851422042358,
64.4162360399775));
#175377=CARTESIAN_POINT('Ctrl Pts',(8.12524938758068,0.00315469804922955,
64.4160547003486));
#175378=CARTESIAN_POINT('',(8.12524999535401,-0.000274771867375941,60.4167025044555));
#175379=CARTESIAN_POINT('Ctrl Pts',(8.12524938756529,0.0031547376877246,
64.4160547019031));
#175380=CARTESIAN_POINT('Ctrl Pts',(8.12525204940757,-0.00370102481534387,
64.4157858284478));
#175381=CARTESIAN_POINT('Ctrl Pts',(8.12524603432191,-0.0105567958430449,
64.4155170925646));
#175382=CARTESIAN_POINT('Ctrl Pts',(8.12519813422269,-0.0329084438924019,
64.4146413753845));
#175383=CARTESIAN_POINT('Ctrl Pts',(8.12512059715649,-0.048404228318903,
64.4140349442452));
#175384=CARTESIAN_POINT('Ctrl Pts',(8.12471932175839,-0.0994273318824331,
64.4120401975096));
#175385=CARTESIAN_POINT('Ctrl Pts',(8.12420689032392,-0.13495285100877,
64.410654606361));
#175386=CARTESIAN_POINT('Ctrl Pts',(8.11947477656758,-0.360448517205846,
64.4018763343925));
#175387=CARTESIAN_POINT('Ctrl Pts',(8.10882517728109,-0.550226757232409,
64.3945617889879));
#175388=CARTESIAN_POINT('Ctrl Pts',(8.07513697308051,-0.918860305201467,
64.3803278025321));
#175389=CARTESIAN_POINT('Ctrl Pts',(8.05278017884501,-1.09766688401897,
64.3734116579737));
#175390=CARTESIAN_POINT('Ctrl Pts',(8.00415582295705,-1.40355555064036,
64.3614663920084));
#175391=CARTESIAN_POINT('Ctrl Pts',(7.98075471087268,-1.53102334966457,
64.356454671678));
#175392=CARTESIAN_POINT('Ctrl Pts',(7.94632772561076,-1.69620039633607,
64.349898106299));
#175393=CARTESIAN_POINT('Ctrl Pts',(7.93806317250455,-1.73446624753435,
64.348374831546));
#175394=CARTESIAN_POINT('Ctrl Pts',(7.9223281029886,-1.80485246180425,64.3455643941418));
#175395=CARTESIAN_POINT('Ctrl Pts',(7.91493795418629,-1.8369899710248,64.3442778938508));
#175396=CARTESIAN_POINT('Ctrl Pts',(7.89925646041881,-1.90333223292204,
64.3416150432594));
#175397=CARTESIAN_POINT('Ctrl Pts',(7.89093810213413,-1.93752989000181,
64.3402384993482));
#175398=CARTESIAN_POINT('Ctrl Pts',(7.87144005493255,-2.01547963905902,
64.3370915458013));
#175399=CARTESIAN_POINT('Ctrl Pts',(7.86011729518225,-2.05919469662068,
64.33531999881));
#175400=CARTESIAN_POINT('Ctrl Pts',(7.82290836486081,-2.19807138964046,
64.3296699459717));
#175401=CARTESIAN_POINT('Ctrl Pts',(7.79565398966512,-2.29285668554399,
64.3257804125679));
#175402=CARTESIAN_POINT('Ctrl Pts',(7.67686491772103,-2.67934590069931,
64.309779680942));
#175403=CARTESIAN_POINT('Ctrl Pts',(7.57062835689682,-2.9662656681853,64.2975559304686));
#175404=CARTESIAN_POINT('Ctrl Pts',(7.39952224714856,-3.35883482445798,
64.2804585812234));
#175405=CARTESIAN_POINT('Ctrl Pts',(7.3480301193725,-3.47003667282726,64.2755736441374));
#175406=CARTESIAN_POINT('Ctrl Pts',(7.27227122521564,-3.62438965903496,
64.2687520887739));
#175407=CARTESIAN_POINT('Ctrl Pts',(7.25009545692704,-3.66854808821287,
64.2667957655264));
#175408=CARTESIAN_POINT('Ctrl Pts',(7.21499875400296,-3.736874538536,64.2637629173039));
#175409=CARTESIAN_POINT('Ctrl Pts',(7.20235608084728,-3.76118401961452,
64.2626827218337));
#175410=CARTESIAN_POINT('Ctrl Pts',(7.18075844045299,-3.80220399056128,
64.2608583554564));
#175411=CARTESIAN_POINT('Ctrl Pts',(7.17186752600412,-3.81894791253493,
64.260113203913));
#175412=CARTESIAN_POINT('Ctrl Pts',(7.15407559281999,-3.85217352162106,
64.2586337764102));
#175413=CARTESIAN_POINT('Ctrl Pts',(7.14517602069198,-3.86865584725983,
64.2578994780146));
#175414=CARTESIAN_POINT('Ctrl Pts',(7.12714118232302,-3.90178249117635,
64.2564227114513));
#175415=CARTESIAN_POINT('Ctrl Pts',(7.11800441306719,-3.91842585988836,
64.2556802726238));
#175416=CARTESIAN_POINT('Ctrl Pts',(7.09571828303957,-3.95868668763129,
64.2538829126784));
#175417=CARTESIAN_POINT('Ctrl Pts',(7.08250922400596,-3.98227087752909,
64.2528288918872));
#175418=CARTESIAN_POINT('Ctrl Pts',(7.03118857839778,-4.0728385636086,64.248775921879));
#175419=CARTESIAN_POINT('Ctrl Pts',(6.99224224111277,-4.13934479879885,
64.2457884052512));
#175420=CARTESIAN_POINT('Ctrl Pts',(6.7339240821858,-4.5664071052158,64.2264978092489));
#175421=CARTESIAN_POINT('Ctrl Pts',(6.48768755617069,-4.90996159105387,
64.2104504594844));
#175422=CARTESIAN_POINT('Ctrl Pts',(6.12907874093593,-5.33593916333049,
64.1890069140588));
#175423=CARTESIAN_POINT('Ctrl Pts',(6.03972662018785,-5.4368699595074,64.1838019477991));
#175424=CARTESIAN_POINT('Ctrl Pts',(5.9267833840165,-5.55822701518685,64.1773740221034));
#175425=CARTESIAN_POINT('Ctrl Pts',(5.90553117334658,-5.58080194855463,
64.1761708503687));
#175426=CARTESIAN_POINT('Ctrl Pts',(5.87193317930073,-5.61608423694732,
64.1742785014447));
#175427=CARTESIAN_POINT('Ctrl Pts',(5.85967413836101,-5.62887381364428,
64.1735900494471));
#175428=CARTESIAN_POINT('Ctrl Pts',(5.83991486298699,-5.6493537104712,64.1724835967761));
#175429=CARTESIAN_POINT('Ctrl Pts',(5.8324410301001,-5.65706943418077,64.1720658179839));
#175430=CARTESIAN_POINT('Ctrl Pts',(5.82071279407045,-5.669129307266,64.1714113593207));
#175431=CARTESIAN_POINT('Ctrl Pts',(5.81646877575139,-5.67348354313539,
64.1711747667798));
#175432=CARTESIAN_POINT('Ctrl Pts',(5.80688973725717,-5.68328930491495,
64.170641282479));
#175433=CARTESIAN_POINT('Ctrl Pts',(5.80155192073177,-5.68873808985793,
64.1703443674562));
#175434=CARTESIAN_POINT('Ctrl Pts',(5.79194368959671,-5.69851847923192,
64.1698105616407));
#175435=CARTESIAN_POINT('Ctrl Pts',(5.78767606791372,-5.70285282069132,
64.1695736945061));
#175436=CARTESIAN_POINT('Ctrl Pts',(5.78004590347647,-5.71058488837986,
64.1691506038999));
#175437=CARTESIAN_POINT('Ctrl Pts',(5.77668522135747,-5.71398444756537,
64.168964396173));
#175438=CARTESIAN_POINT('Ctrl Pts',(5.77070977335725,-5.72001836107062,
64.1686335604088));
#175439=CARTESIAN_POINT('Ctrl Pts',(5.76809619847496,-5.72265389346899,
64.168488942439));
#175440=CARTESIAN_POINT('Ctrl Pts',(5.76346984884242,-5.72731272142231,
64.1682331005509));
#175441=CARTESIAN_POINT('Ctrl Pts',(5.76145781210566,-5.72933674929343,
64.1681218828647));
#175442=CARTESIAN_POINT('Ctrl Pts',(5.75790885942168,-5.73290309266949,
64.1679257983797));
#175443=CARTESIAN_POINT('Ctrl Pts',(5.75637238903329,-5.73444585135656,
64.1678409353406));
#175444=CARTESIAN_POINT('Ctrl Pts',(5.71813460267077,-5.77280927939729,
64.1657296901173));
#175445=CARTESIAN_POINT('Ctrl Pts',(5.68108144517901,-5.80927739912985,
64.1637003779826));
#175446=CARTESIAN_POINT('Ctrl Pts',(5.60593469460557,-5.88183106590527,
64.1596171476276));
#175447=CARTESIAN_POINT('Ctrl Pts',(5.56783641332856,-5.91790825709693,
64.1575632710034));
#175448=CARTESIAN_POINT('Ctrl Pts',(5.48305435021858,-5.99664920821727,
64.1530278682194));
#175449=CARTESIAN_POINT('Ctrl Pts',(5.43621650970671,-6.03914205477017,
64.1505452543575));
#175450=CARTESIAN_POINT('Ctrl Pts',(5.27342822128735,-6.18340051557863,
64.1419947395129));
#175451=CARTESIAN_POINT('Ctrl Pts',(5.15507877583407,-6.28240794851399,
64.1359113623838));
#175452=CARTESIAN_POINT('Ctrl Pts',(4.93314086003644,-6.45757794478466,
64.1247504614391));
#175453=CARTESIAN_POINT('Ctrl Pts',(4.83042503823626,-6.53476745256651,
64.1196765853492));
#175454=CARTESIAN_POINT('Ctrl Pts',(4.66299862665205,-6.65448082229071,
64.1115617008048));
#175455=CARTESIAN_POINT('Ctrl Pts',(4.59943550084666,-6.69857181366465,
64.1085155644984));
#175456=CARTESIAN_POINT('Ctrl Pts',(4.50427363148722,-6.7625883056649,64.1040092861141));
#175457=CARTESIAN_POINT('Ctrl Pts',(4.47315155761274,-6.78321433375243,
64.1025439978163));
#175458=CARTESIAN_POINT('Ctrl Pts',(4.40251628902125,-6.82933003919344,
64.099237843005));
#175459=CARTESIAN_POINT('Ctrl Pts',(4.36292177808266,-6.85469270185865,
64.0973980327873));
#175460=CARTESIAN_POINT('Ctrl Pts',(4.19784317407485,-6.958425680721,64.0897784624167));
#175461=CARTESIAN_POINT('Ctrl Pts',(4.07045016611131,-7.03370535256267,
64.084019063757));
#175462=CARTESIAN_POINT('Ctrl Pts',(3.77697888693032,-7.19648029311263,
64.0709534203922));
#175463=CARTESIAN_POINT('Ctrl Pts',(3.60978196664744,-7.28178356681184,
64.0636501735826));
#175464=CARTESIAN_POINT('Ctrl Pts',(3.3913140943643,-7.38387015225066,64.0542255174533));
#175465=CARTESIAN_POINT('Ctrl Pts',(3.34262320686156,-7.40603941313536,
64.0521324573302));
#175466=CARTESIAN_POINT('Ctrl Pts',(3.24877503240178,-7.44765501977847,
64.0481109177716));
#175467=CARTESIAN_POINT('Ctrl Pts',(3.20365318231655,-7.4671755553558,64.0461829345451));
#175468=CARTESIAN_POINT('Ctrl Pts',(3.09936060646691,-7.51117510599718,
64.0417381805705));
#175469=CARTESIAN_POINT('Ctrl Pts',(3.04007217246704,-7.53536653291677,
64.0392198491847));
#175470=CARTESIAN_POINT('Ctrl Pts',(2.86206881262391,-7.60555438327485,
64.0316811236387));
#175471=CARTESIAN_POINT('Ctrl Pts',(2.74255294244948,-7.64946392738869,
64.0266483374526));
#175472=CARTESIAN_POINT('Ctrl Pts',(2.25776655844223,-7.81474954326695,
64.0063298713251));
#175473=CARTESIAN_POINT('Ctrl Pts',(1.8851152814601,-7.91291066159002,63.9909038048653));
#175474=CARTESIAN_POINT('Ctrl Pts',(1.37368334320369,-8.00943604647141,
63.9700926781856));
#175475=CARTESIAN_POINT('Ctrl Pts',(1.23983811073659,-8.03124358790862,
63.9646816320136));
#175476=CARTESIAN_POINT('Ctrl Pts',(1.05048490881522,-8.05724852629485,
63.957093360949));
#175477=CARTESIAN_POINT('Ctrl Pts',(0.995384196476443,-8.06424098776294,
63.9548931929893));
#175478=CARTESIAN_POINT('Ctrl Pts',(0.909396319193509,-8.07425839542534,
63.9514737343896));
#175479=CARTESIAN_POINT('Ctrl Pts',(0.878556319360719,-8.07767225787237,
63.9502501359119));
#175480=CARTESIAN_POINT('Ctrl Pts',(0.826275490750182,-8.08315658179095,
63.9481809433575));
#175481=CARTESIAN_POINT('Ctrl Pts',(0.804844644263694,-8.08531858461841,
63.9473341902665));
#175482=CARTESIAN_POINT('Ctrl Pts',(0.764802366292209,-8.08919737820714,
63.9457549088741));
#175483=CARTESIAN_POINT('Ctrl Pts',(0.746193122989615,-8.09093521843988,
63.9450220930727));
#175484=CARTESIAN_POINT('Ctrl Pts',(0.707759744308294,-8.0943906284182,
63.9435110663978));
#175485=CARTESIAN_POINT('Ctrl Pts',(0.687934940217948,-8.09609961794608,
63.942732987854));
#175486=CARTESIAN_POINT('Ctrl Pts',(0.643666690664774,-8.09975197157235,
63.9409986803755));
#175487=CARTESIAN_POINT('Ctrl Pts',(0.619220314132326,-8.10165754759993,
63.9400430471894));
#175488=CARTESIAN_POINT('Ctrl Pts',(0.52066865764252,-8.10889090127148,
63.9361981806767));
#175489=CARTESIAN_POINT('Ctrl Pts',(0.446500092807692,-8.11331284414584,
63.9333218985643));
#175490=CARTESIAN_POINT('Ctrl Pts',(0.125294502595008,-8.12804524212464,
63.9209153883458));
#175491=CARTESIAN_POINT('Ctrl Pts',(-0.122082025730928,-8.12809424394012,
63.9114834068664));
#175492=CARTESIAN_POINT('Ctrl Pts',(-0.531230597173478,-8.10949011156463,
63.8958015585012));
#175493=CARTESIAN_POINT('Ctrl Pts',(-0.69312617299227,-8.09725949964694,
63.8895763427644));
#175494=CARTESIAN_POINT('Ctrl Pts',(-0.928650146515136,-8.0723509178624,
63.8804424902982));
#175495=CARTESIAN_POINT('Ctrl Pts',(-1.00264285739792,-8.06349475420231,
63.8775619364667));
#175496=CARTESIAN_POINT('Ctrl Pts',(-1.13618574810246,-8.04564448522457,
63.872339003689));
#175497=CARTESIAN_POINT('Ctrl Pts',(-1.19577776775611,-8.0370037151075,
63.8699996291643));
#175498=CARTESIAN_POINT('Ctrl Pts',(-1.2878575355839,-8.02260547297953,
63.8663700168485));
#175499=CARTESIAN_POINT('Ctrl Pts',(-1.32041564458816,-8.01731115299748,
63.865083751183));
#175500=CARTESIAN_POINT('Ctrl Pts',(-1.38473825371414,-8.00644911668935,
63.8625366319962));
#175501=CARTESIAN_POINT('Ctrl Pts',(-1.41650364793955,-8.0008902565102,
63.8612758761062));
#175502=CARTESIAN_POINT('Ctrl Pts',(-1.48996925976643,-7.98758274206336,
63.8583531952647));
#175503=CARTESIAN_POINT('Ctrl Pts',(-1.53164353265685,-7.97969639315823,
63.8566901354077));
#175504=CARTESIAN_POINT('Ctrl Pts',(-1.65263821544259,-7.95581685323283,
63.8518463519944));
#175505=CARTESIAN_POINT('Ctrl Pts',(-1.7317835384288,-7.93896470136714,
63.848658628572));
#175506=CARTESIAN_POINT('Ctrl Pts',(-2.09291836372321,-7.85641209705464,
63.8340232325431));
#175507=CARTESIAN_POINT('Ctrl Pts',(-2.37152029756464,-7.77685068071387,
63.8224691814695));
#175508=CARTESIAN_POINT('Ctrl Pts',(-2.79714929864855,-7.63029771565671,
63.8045205684309));
#175509=CARTESIAN_POINT('Ctrl Pts',(-2.9474390112876,-7.57351248576873,
63.7981255740526));
#175510=CARTESIAN_POINT('Ctrl Pts',(-3.12730734936599,-7.49938575999014,
63.790439559224));
#175511=CARTESIAN_POINT('Ctrl Pts',(-3.15858611875411,-7.48626554287471,
63.7891018124664));
#175512=CARTESIAN_POINT('Ctrl Pts',(-3.20612307748125,-7.46597468927721,
63.7870675055553));
#175513=CARTESIAN_POINT('Ctrl Pts',(-3.22244135791033,-7.45894596748951,
63.7863689574048));
#175514=CARTESIAN_POINT('Ctrl Pts',(-3.25468018323636,-7.44493429699319,
63.7849885600082));
#175515=CARTESIAN_POINT('Ctrl Pts',(-3.27060164000678,-7.43795366324794,
63.7843066788492));
#175516=CARTESIAN_POINT('Ctrl Pts',(-3.3078954115363,-7.42145961269543,
63.7827092202604));
#175517=CARTESIAN_POINT('Ctrl Pts',(-3.32924930814989,-7.41190487568663,
63.7817943418073));
#175518=CARTESIAN_POINT('Ctrl Pts',(-3.39697023209044,-7.38125164353628,
63.7788919046525));
#175519=CARTESIAN_POINT('Ctrl Pts',(-3.44318042365743,-7.35980918259458,
63.7769098546716));
#175520=CARTESIAN_POINT('Ctrl Pts',(-3.87464215715951,-7.15464920109376,
63.7583769411999));
#175521=CARTESIAN_POINT('Ctrl Pts',(-4.24506479953309,-6.94127473179555,
63.7422494402626));
#175522=CARTESIAN_POINT('Ctrl Pts',(-4.84852728871508,-6.52721324974982,
63.714449338336));
#175523=CARTESIAN_POINT('Ctrl Pts',(-5.09012257526372,-6.34061343858149,
63.7028440259401));
#175524=CARTESIAN_POINT('Ctrl Pts',(-5.41118586621761,-6.06243388068201,
63.6865064216333));
#175525=CARTESIAN_POINT('Ctrl Pts',(-5.49997353340321,-5.98200032070825,
63.6818830476362));
#175526=CARTESIAN_POINT('Ctrl Pts',(-5.65288329967631,-5.83719485623575,
63.6737206436038));
#175527=CARTESIAN_POINT('Ctrl Pts',(-5.71776503104696,-5.77365536606747,
63.6701905117093));
#175528=CARTESIAN_POINT('Ctrl Pts',(-5.80803529048837,-5.68223834361919,
63.6651802468827));
#175529=CARTESIAN_POINT('Ctrl Pts',(-5.83431600503003,-5.65525094684929,
63.6637093804543));
#175530=CARTESIAN_POINT('Ctrl Pts',(-5.88694846925146,-5.60044582380717,
63.6607386431695));
#175531=CARTESIAN_POINT('Ctrl Pts',(-5.91329301984136,-5.5726224845497,
63.6592387453951));
#175532=CARTESIAN_POINT('Ctrl Pts',(-5.96358378557714,-5.51875056893912,
63.656350253589));
#175533=CARTESIAN_POINT('Ctrl Pts',(-5.98755861018893,-5.49272985779891,
63.6549619646227));
#175534=CARTESIAN_POINT('Ctrl Pts',(-6.04404719283613,-5.43061149356175,
63.6516638397119));
#175535=CARTESIAN_POINT('Ctrl Pts',(-6.07640863765134,-5.39437723100798,
63.6497527156917));
#175536=CARTESIAN_POINT('Ctrl Pts',(-6.17476433658124,-5.28224276866908,
63.6438766874999));
#175537=CARTESIAN_POINT('Ctrl Pts',(-6.23967564193039,-5.20540593989818,
63.6399033600526));
#175538=CARTESIAN_POINT('Ctrl Pts',(-6.56490242714283,-4.80560147872492,
63.6194947523112));
#175539=CARTESIAN_POINT('Ctrl Pts',(-6.80162929359192,-4.46425539471723,
63.6029886710398));
#175540=CARTESIAN_POINT('Ctrl Pts',(-7.20251664628805,-3.77977075460938,
63.5705558172725));
#175541=CARTESIAN_POINT('Ctrl Pts',(-7.37072190454711,-3.44025474152612,
63.5547351218701));
#175542=CARTESIAN_POINT('Ctrl Pts',(-7.66828907220903,-2.71665612943567,
63.5216660775127));
#175543=CARTESIAN_POINT('Ctrl Pts',(-7.7938542466089,-2.33210619624823,
63.504436103179));
#175544=CARTESIAN_POINT('Ctrl Pts',(-7.91927117879069,-1.82196566220897,
63.482861504689));
#175545=CARTESIAN_POINT('Ctrl Pts',(-7.94560058857013,-1.70348105245745,
63.4779417661207));
#175546=CARTESIAN_POINT('Ctrl Pts',(-7.9732636753246,-1.56434461232731,
63.4723022967545));
#175547=CARTESIAN_POINT('Ctrl Pts',(-7.97718464863456,-1.54422562895212,
63.4714901912393));
#175548=CARTESIAN_POINT('Ctrl Pts',(-7.98284803600176,-1.51456884711066,
63.4702982397127));
#175549=CARTESIAN_POINT('Ctrl Pts',(-7.9846495614056,-1.50504250474424,
63.4699161428485));
#175550=CARTESIAN_POINT('Ctrl Pts',(-7.98777228687909,-1.48836632601237,
63.4692486632953));
#175551=CARTESIAN_POINT('Ctrl Pts',(-7.98910094674253,-1.48121790789082,
63.4689629889867));
#175552=CARTESIAN_POINT('Ctrl Pts',(-7.99165531064304,-1.4673715693478,
63.4684105231899));
#175553=CARTESIAN_POINT('Ctrl Pts',(-7.99288219344804,-1.46067387484599,
63.4681436848806));
#175554=CARTESIAN_POINT('Ctrl Pts',(-7.99578057124931,-1.4447382984189,
63.4675097661155));
#175555=CARTESIAN_POINT('Ctrl Pts',(-7.99744448054419,-1.43549903380843,
63.4671429940331));
#175556=CARTESIAN_POINT('Ctrl Pts',(-8.00239079824824,-1.40775785143915,
63.466044092619));
#175557=CARTESIAN_POINT('Ctrl Pts',(-8.0056250550691,-1.38924732924432,
63.4653139686099));
#175558=CARTESIAN_POINT('Ctrl Pts',(-8.05104951925469,-1.12384394578858,
63.4548918939583));
#175559=CARTESIAN_POINT('Ctrl Pts',(-8.08186510898217,-0.875145046226254,
63.4457563378864));
#175560=CARTESIAN_POINT('Ctrl Pts',(-8.13987571169031,-0.123724830521734,
63.4192581857281));
#175561=CARTESIAN_POINT('Ctrl Pts',(-8.13192134988833,0.380501029881913,
63.4028745511142));
#175562=CARTESIAN_POINT('Ctrl Pts',(-8.01189465542595,1.48125066983262,
63.3656839765176));
#175563=CARTESIAN_POINT('Ctrl Pts',(-7.87967257195023,2.0724918143441,63.3446719436477));
#175564=CARTESIAN_POINT('Ctrl Pts',(-7.67391061298761,2.67050429610845,
63.3203132846228));
#175565=CARTESIAN_POINT('Ctrl Pts',(-7.66451114472503,2.69736282033,63.3192128460829));
#175566=CARTESIAN_POINT('Ctrl Pts',(-7.65062936392473,2.73637087719036,
63.3176051481124));
#175567=CARTESIAN_POINT('Ctrl Pts',(-7.64625874428789,2.74856006942296,
63.3171014259841));
#175568=CARTESIAN_POINT('Ctrl Pts',(-7.63855409512638,2.76988691287619,
63.3162177087356));
#175569=CARTESIAN_POINT('Ctrl Pts',(-7.63523275558756,2.7790291364945,63.3158381166157));
#175570=CARTESIAN_POINT('Ctrl Pts',(-7.62876438297412,2.79673466483496,
63.3151014766595));
#175571=CARTESIAN_POINT('Ctrl Pts',(-7.6256193266851,2.80529867933497,63.3147444919888));
#175572=CARTESIAN_POINT('Ctrl Pts',(-7.61809634583897,2.82567768656041,
63.3138933873048));
#175573=CARTESIAN_POINT('Ctrl Pts',(-7.61370535524593,2.83748781223489,
63.3133988525227));
#175574=CARTESIAN_POINT('Ctrl Pts',(-7.59800515431709,2.87941665499392,
63.3116384943998));
#175575=CARTESIAN_POINT('Ctrl Pts',(-7.58654462174147,2.90947817855706,
63.3103678597336));
#175576=CARTESIAN_POINT('Ctrl Pts',(-7.39731528067532,3.39711511563414,
63.2896165249454));
#175577=CARTESIAN_POINT('Ctrl Pts',(-7.17863979560322,3.83766805284282,
63.2687758373457));
#175578=CARTESIAN_POINT('Ctrl Pts',(-6.64247001345833,4.70969677116121,
63.2235801981561));
#175579=CARTESIAN_POINT('Ctrl Pts',(-6.31939339008014,5.13506570441792,
63.1991886686126));
#175580=CARTESIAN_POINT('Ctrl Pts',(-5.78028346325522,5.71625220931396,
63.1644909113297));
#175581=CARTESIAN_POINT('Ctrl Pts',(-5.59450124224049,5.89820323550877,
63.1534092167543));
#175582=CARTESIAN_POINT('Ctrl Pts',(-5.36818891090053,6.09951490315464,
63.1411744746036));
#175583=CARTESIAN_POINT('Ctrl Pts',(-5.33585423308989,6.12782130460805,
63.1394540399324));
#175584=CARTESIAN_POINT('Ctrl Pts',(-5.29335428758745,6.16443510346981,
63.1372265058798));
#175585=CARTESIAN_POINT('Ctrl Pts',(-5.28339172345201,6.17297591588093,
63.1367067371201));
#175586=CARTESIAN_POINT('Ctrl Pts',(-5.26715767014812,6.1868251267358,63.1358635867649));
#175587=CARTESIAN_POINT('Ctrl Pts',(-5.26089876643083,6.19214819275304,
63.1355394351994));
#175588=CARTESIAN_POINT('Ctrl Pts',(-5.24886217047174,6.20235364170421,
63.1349177944893));
#175589=CARTESIAN_POINT('Ctrl Pts',(-5.2430857156204,6.20723746609683,63.1346202313172));
#175590=CARTESIAN_POINT('Ctrl Pts',(-5.22988143408974,6.21836971905312,
63.1339417676677));
#175591=CARTESIAN_POINT('Ctrl Pts',(-5.22244920631241,6.2246129249912,63.1335611303777));
#175592=CARTESIAN_POINT('Ctrl Pts',(-5.2027880126816,6.24106868252852,63.132557433755));
#175593=CARTESIAN_POINT('Ctrl Pts',(-5.19054013321589,6.25125863604428,
63.1319354840345));
#175594=CARTESIAN_POINT('Ctrl Pts',(-5.11025100102791,6.3176586990242,63.1278794069582));
#175595=CARTESIAN_POINT('Ctrl Pts',(-5.04132635515106,6.37279420225621,
63.1244957924265));
#175596=CARTESIAN_POINT('Ctrl Pts',(-4.54164333825795,6.75932921596949,
63.1005685158073));
#175597=CARTESIAN_POINT('Ctrl Pts',(-4.07946894131787,7.04791161659307,
63.0814870743557));
#175598=CARTESIAN_POINT('Ctrl Pts',(-3.33112898753213,7.41672437088348,
63.0513920394419));
#175599=CARTESIAN_POINT('Ctrl Pts',(-3.06363186422011,7.53116018788785,
63.0407974046997));
#175600=CARTESIAN_POINT('Ctrl Pts',(-2.5706637747521,7.71143353272238,63.0212294327299));
#175601=CARTESIAN_POINT('Ctrl Pts',(-2.34737804935643,7.78230880486546,
63.0123534670956));
#175602=CARTESIAN_POINT('Ctrl Pts',(-2.07726331331589,7.85536443242926,
63.0015620714131));
#175603=CARTESIAN_POINT('Ctrl Pts',(-2.03307852239784,7.86691584566017,
62.9997953163534));
#175604=CARTESIAN_POINT('Ctrl Pts',(-1.96401611110322,7.88435042384482,
62.9970314634466));
#175605=CARTESIAN_POINT('Ctrl Pts',(-1.93920400436303,7.89048976386617,
62.9960380220522));
#175606=CARTESIAN_POINT('Ctrl Pts',(-1.89322872803482,7.90163562009407,
62.9941963931268));
#175607=CARTESIAN_POINT('Ctrl Pts',(-1.87207358696403,7.90667445708102,
62.9933486625261));
#175608=CARTESIAN_POINT('Ctrl Pts',(-1.82689224060276,7.91724447949351,
62.991537419877));
#175609=CARTESIAN_POINT('Ctrl Pts',(-1.80286055595851,7.92275136658977,
62.9905735750719));
#175610=CARTESIAN_POINT('Ctrl Pts',(-1.73832481455643,7.93723097002044,
62.9879837321676));
#175611=CARTESIAN_POINT('Ctrl Pts',(-1.69777660589826,7.94600297002463,
62.9863549419748));
#175612=CARTESIAN_POINT('Ctrl Pts',(-1.51324324699864,7.98444702922659,
62.9789332451494));
#175613=CARTESIAN_POINT('Ctrl Pts',(-1.36853878936757,8.01051806358963,
62.9730875467613));
#175614=CARTESIAN_POINT('Ctrl Pts',(-1.0941736298121,8.05229829755306,62.9619289755147));
#175615=CARTESIAN_POINT('Ctrl Pts',(-0.964685657689746,8.06883537719088,
62.9566316024408));
#175616=CARTESIAN_POINT('Ctrl Pts',(-0.606834356168358,8.10579971070932,
62.9418956805752));
#175617=CARTESIAN_POINT('Ctrl Pts',(-0.377922659050299,8.11969250849721,
62.9323590304124));
#175618=CARTESIAN_POINT('Ctrl Pts',(0.119685701681321,8.12880292136515,
62.9114326169932));
#175619=CARTESIAN_POINT('Ctrl Pts',(0.388183179612827,8.12041085485493,
62.900015800063));
#175620=CARTESIAN_POINT('Ctrl Pts',(1.00315989691236,8.07061522847358,62.8738589285822));
#175621=CARTESIAN_POINT('Ctrl Pts',(1.34839545407884,8.02016251701541,62.8591632117109));
#175622=CARTESIAN_POINT('Ctrl Pts',(1.72017800583175,7.94113780508695,62.8438598016724));
#175623=CARTESIAN_POINT('Ctrl Pts',(1.7509855809573,7.93440177558938,62.8425958151784));
#175624=CARTESIAN_POINT('Ctrl Pts',(1.80443779045928,7.92238804902876,62.8404107099278));
#175625=CARTESIAN_POINT('Ctrl Pts',(1.82710034318673,7.91719220985915,62.839486766264));
#175626=CARTESIAN_POINT('Ctrl Pts',(1.85977389630223,7.90955338754597,62.8381585456323));
#175627=CARTESIAN_POINT('Ctrl Pts',(1.86980293496711,7.9071885472248,62.8377513796489));
#175628=CARTESIAN_POINT('Ctrl Pts',(1.88725282252336,7.90303882062074,62.837043882874));
#175629=CARTESIAN_POINT('Ctrl Pts',(1.89467569426125,7.90126254660898,62.836743224662));
#175630=CARTESIAN_POINT('Ctrl Pts',(1.90897917882951,7.89781844444394,62.836164460185));
#175631=CARTESIAN_POINT('Ctrl Pts',(1.91586013372285,7.89615207775169,62.8358862974823));
#175632=CARTESIAN_POINT('Ctrl Pts',(1.93212057916416,7.89219176570665,62.8352296023997));
#175633=CARTESIAN_POINT('Ctrl Pts',(1.94149818815987,7.88989008703565,62.8348513766385));
#175634=CARTESIAN_POINT('Ctrl Pts',(1.96932747033105,7.88300693451832,62.8337304643152));
#175635=CARTESIAN_POINT('Ctrl Pts',(1.98776726804379,7.87837739075315,62.8329897314686));
#175636=CARTESIAN_POINT('Ctrl Pts',(2.22054577885077,7.81906612739816,62.8236654189386));
#175637=CARTESIAN_POINT('Ctrl Pts',(2.4325736746376,7.75572063302635,62.8155031024213));
#175638=CARTESIAN_POINT('Ctrl Pts',(3.11200976243386,7.52212474382858,62.789897959343));
#175639=CARTESIAN_POINT('Ctrl Pts',(3.56644896326103,7.31761251325884,62.7735395429903));
#175640=CARTESIAN_POINT('Ctrl Pts',(4.49196538899508,6.79427659383245,62.7376094089114));
#175641=CARTESIAN_POINT('Ctrl Pts',(4.9540993098378,6.46504235961165,62.7179404884031));
#175642=CARTESIAN_POINT('Ctrl Pts',(5.41923087030591,6.05430540045263,62.6942711520381));
#175643=CARTESIAN_POINT('Ctrl Pts',(5.45984842508369,6.01770156678796,62.6921695839031));
#175644=CARTESIAN_POINT('Ctrl Pts',(5.5124295755443,5.96934574661173,62.6894024422877));
#175645=CARTESIAN_POINT('Ctrl Pts',(5.52473097594945,5.95796241237925,62.6887516879447));
#175646=CARTESIAN_POINT('Ctrl Pts',(5.54468630420597,5.93938142713052,62.6876904933898));
#175647=CARTESIAN_POINT('Ctrl Pts',(5.55236167238611,5.93220682436324,62.6872809865011));
#175648=CARTESIAN_POINT('Ctrl Pts',(5.56708175938493,5.91839352755375,62.6864930289483));
#175649=CARTESIAN_POINT('Ctrl Pts',(5.57412857543158,5.911757089601,62.6861146702385));
#175650=CARTESIAN_POINT('Ctrl Pts',(5.59019569895153,5.89657138224248,62.6852493616479));
#175651=CARTESIAN_POINT('Ctrl Pts',(5.59920827467962,5.88801398720893,62.6847620801637));
#175652=CARTESIAN_POINT('Ctrl Pts',(5.62294822765948,5.86536922460854,62.6834734901238));
#175653=CARTESIAN_POINT('Ctrl Pts',(5.63764225517208,5.85124710701203,62.6826707559272));
#175654=CARTESIAN_POINT('Ctrl Pts',(5.73222596136949,5.75965768359682,62.6774701048535));
#175655=CARTESIAN_POINT('Ctrl Pts',(5.81056812256743,5.68061334685429,62.6730068867596));
#175656=CARTESIAN_POINT('Ctrl Pts',(6.54783702410524,4.90552330799002,62.629457466984));
#175657=CARTESIAN_POINT('Ctrl Pts',(7.08027475571478,4.09967731532907,62.5847303324922));
#175658=CARTESIAN_POINT('Ctrl Pts',(7.56706264271846,2.97191484942539,62.5307991778134));
#175659=CARTESIAN_POINT('Ctrl Pts',(7.66172198382725,2.71859464217452,62.5192544220422));
#175660=CARTESIAN_POINT('Ctrl Pts',(7.75641443257763,2.42064381551627,62.5066462132521));
#175661=CARTESIAN_POINT('Ctrl Pts',(7.76892684435691,2.3801800605182,62.5049539791719));
#175662=CARTESIAN_POINT('Ctrl Pts',(7.78477544105883,2.32747069559257,62.5027734304126));
#175663=CARTESIAN_POINT('Ctrl Pts',(7.7883999663594,2.31531303998063,62.5022721169757));
#175664=CARTESIAN_POINT('Ctrl Pts',(7.79423145439123,2.29558397642976,62.5014611869925));
#175665=CARTESIAN_POINT('Ctrl Pts',(7.79645588507414,2.28801778623926,62.5011508072324));
#175666=CARTESIAN_POINT('Ctrl Pts',(7.80069628430694,2.27351648376464,62.5005570946048));
#175667=CARTESIAN_POINT('Ctrl Pts',(7.80271402817571,2.26658190165376,62.5002736858765));
#175668=CARTESIAN_POINT('Ctrl Pts',(7.80732801053588,2.25064539035918,62.4996235240274));
#175669=CARTESIAN_POINT('Ctrl Pts',(7.80991793351598,2.24164163280765,62.4992570367442));
#175670=CARTESIAN_POINT('Ctrl Pts',(7.8178953759522,2.21372674641611,62.4981233384743));
#175671=CARTESIAN_POINT('Ctrl Pts',(7.82322984634526,2.1948004457798,62.4973583053059));
#175672=CARTESIAN_POINT('Ctrl Pts',(7.86655399893867,2.03892472871585,62.4910859259758));
#175673=CARTESIAN_POINT('Ctrl Pts',(7.90101451191266,1.90101500873938,62.4857160076361));
#175674=CARTESIAN_POINT('Ctrl Pts',(8.06032380931102,1.18397563950439,62.4584198726444));
#175675=CARTESIAN_POINT('Ctrl Pts',(8.12518544520022,0.593344303021297,
62.4378250394779));
#175676=CARTESIAN_POINT('Ctrl Pts',(8.12531225746491,-0.571359736175462,
62.3954537244734));
#175677=CARTESIAN_POINT('Ctrl Pts',(8.06492182068399,-1.14198041541291,
62.3738694867536));
#175678=CARTESIAN_POINT('Ctrl Pts',(7.9202586513955,-1.81748889944684,62.3471936005567));
#175679=CARTESIAN_POINT('Ctrl Pts',(7.89287697418633,-1.93293965873061,
62.34259541739));
#175680=CARTESIAN_POINT('Ctrl Pts',(7.8511016152355,-2.09334933675133,62.3361410732562));
#175681=CARTESIAN_POINT('Ctrl Pts',(7.83882943857648,-2.1388457230221,62.3343030290089));
#175682=CARTESIAN_POINT('Ctrl Pts',(7.81580821770263,-2.22133135436604,
62.3309563601047));
#175683=CARTESIAN_POINT('Ctrl Pts',(7.80519056780994,-2.25835587721572,
62.3294489165132));
#175684=CARTESIAN_POINT('Ctrl Pts',(7.78322840658023,-2.33293420686602,
62.3264014384356));
#175685=CARTESIAN_POINT('Ctrl Pts',(7.7718743741075,-2.37048415745722,62.3248613568242));
#175686=CARTESIAN_POINT('Ctrl Pts',(7.74317078945072,-2.46298895674056,
62.3210527992961));
#175687=CARTESIAN_POINT('Ctrl Pts',(7.72550770352769,-2.51784414738833,
62.3187815840866));
#175688=CARTESIAN_POINT('Ctrl Pts',(7.65531858141025,-2.72813165456218,
62.3100236453473));
#175689=CARTESIAN_POINT('Ctrl Pts',(7.59867342313778,-2.8821460828094,62.3035005081099));
#175690=CARTESIAN_POINT('Ctrl Pts',(7.38599250098703,-3.41045312062028,
62.2807167141194));
#175691=CARTESIAN_POINT('Ctrl Pts',(7.2066420450918,-3.77470215026916,62.264263832392));
#175692=CARTESIAN_POINT('Ctrl Pts',(6.92298713874376,-4.25622794409802,
62.2415507475766));
#175693=CARTESIAN_POINT('Ctrl Pts',(6.84138542441196,-4.38619117662682,
62.2353188670386));
#175694=CARTESIAN_POINT('Ctrl Pts',(6.65387746531277,-4.66685090764606,
62.2216618800794));
#175695=CARTESIAN_POINT('Ctrl Pts',(6.54642724378459,-4.81641721516844,
62.2142511119096));
#175696=CARTESIAN_POINT('Ctrl Pts',(6.39921731363512,-5.00728937323294,
62.2046551407293));
#175697=CARTESIAN_POINT('Ctrl Pts',(6.36397352008132,-5.05200655279165,
62.2023966849957));
#175698=CARTESIAN_POINT('Ctrl Pts',(6.31415493373948,-5.11386751144847,
62.1992592772701));
#175699=CARTESIAN_POINT('Ctrl Pts',(6.29997471125366,-5.13132654339272,
62.198372328782));
#175700=CARTESIAN_POINT('Ctrl Pts',(6.27389841592312,-5.16316127890511,
62.1967524778462));
#175701=CARTESIAN_POINT('Ctrl Pts',(6.26202500489671,-5.17755526910597,
62.1960191066999));
#175702=CARTESIAN_POINT('Ctrl Pts',(6.23694484477089,-5.20774716648288,
62.1944786360966));
#175703=CARTESIAN_POINT('Ctrl Pts',(6.22372740342606,-5.22353603974208,
62.1936717627748));
#175704=CARTESIAN_POINT('Ctrl Pts',(6.18831232026624,-5.26551582220743,
62.1915226459226));
#175705=CARTESIAN_POINT('Ctrl Pts',(6.16600841098385,-5.29161662809608,
62.1901824797457));
#175706=CARTESIAN_POINT('Ctrl Pts',(6.02934098069599,-5.4495122330022,62.1820473844686));
#175707=CARTESIAN_POINT('Ctrl Pts',(5.91092053211543,-5.57773752900278,
62.1753208757816));
#175708=CARTESIAN_POINT('Ctrl Pts',(5.56831406656756,-5.92553598374877,
62.1565383245833));
#175709=CARTESIAN_POINT('Ctrl Pts',(5.33540944962258,-6.13608205130694,
62.144516491761));
#175710=CARTESIAN_POINT('Ctrl Pts',(5.04423671565151,-6.37016097234567,
62.1300179431059));
#175711=CARTESIAN_POINT('Ctrl Pts',(4.99714332621086,-6.40717046669309,
62.1276890158747));
#175712=CARTESIAN_POINT('Ctrl Pts',(4.9226796036295,-6.46436920916488,62.124029815501));
#175713=CARTESIAN_POINT('Ctrl Pts',(4.8955842930863,-6.48491311991678,62.1227030830682));
#175714=CARTESIAN_POINT('Ctrl Pts',(4.84004767897333,-6.52647505380922,
62.1199930452544));
#175715=CARTESIAN_POINT('Ctrl Pts',(4.81159651055969,-6.54747868817897,
62.1186096301913));
#175716=CARTESIAN_POINT('Ctrl Pts',(4.74534694402768,-6.59572138182043,
62.1153993321513));
#175717=CARTESIAN_POINT('Ctrl Pts',(4.70744961659883,-6.62282237793359,
62.1135711378423));
#175718=CARTESIAN_POINT('Ctrl Pts',(4.58131145250874,-6.71139612614134,
62.1075123800936));
#175719=CARTESIAN_POINT('Ctrl Pts',(4.49208381136442,-6.7714426340591,62.103268355296));
#175720=CARTESIAN_POINT('Ctrl Pts',(4.26676196698893,-6.91666089700728,
62.0926514134573));
#175721=CARTESIAN_POINT('Ctrl Pts',(4.12928627651811,-6.99960354903399,
62.086261571181));
#175722=CARTESIAN_POINT('Ctrl Pts',(3.78279343433746,-7.19488927112636,
62.0703891672577));
#175723=CARTESIAN_POINT('Ctrl Pts',(3.57114030165288,-7.30225411112304,
62.0608924530032));
#175724=CARTESIAN_POINT('Ctrl Pts',(3.27815767084971,-7.43508612343448,
62.0481123647284));
#175725=CARTESIAN_POINT('Ctrl Pts',(3.20068201581274,-7.46876550654912,
62.0447668893427));
#175726=CARTESIAN_POINT('Ctrl Pts',(3.09898395766114,-7.51110149238733,
62.0404263355929));
#175727=CARTESIAN_POINT('Ctrl Pts',(3.07522632662997,-7.5208596746376,62.0394159295113));
#175728=CARTESIAN_POINT('Ctrl Pts',(3.0346935048254,-7.53728390835473,62.037698452646));
#175729=CARTESIAN_POINT('Ctrl Pts',(3.01794169170144,-7.54400698103875,
62.0369904960387));
#175730=CARTESIAN_POINT('Ctrl Pts',(2.98196926235409,-7.55830494789312,
62.0354740970303));
#175731=CARTESIAN_POINT('Ctrl Pts',(2.96274185863672,-7.5658624788938,62.0346659207762));
#175732=CARTESIAN_POINT('Ctrl Pts',(2.91502799716843,-7.58440713042021,
62.032665931966));
#175733=CARTESIAN_POINT('Ctrl Pts',(2.88650799762047,-7.59530719155618,
62.0314753589515));
#175734=CARTESIAN_POINT('Ctrl Pts',(2.77617384271997,-7.63676460149921,
62.0268869698048));
#175735=CARTESIAN_POINT('Ctrl Pts',(2.69393005716837,-7.66616304398773,
62.0235037932779));
#175736=CARTESIAN_POINT('Ctrl Pts',(2.53324846378231,-7.72069432954278,
62.0169513329304));
#175737=CARTESIAN_POINT('Ctrl Pts',(2.45487094351724,-7.74597169227038,
62.0137812529695));
#175738=CARTESIAN_POINT('Ctrl Pts',(2.12872368156943,-7.8457092115773,62.0006739371023));
#175739=CARTESIAN_POINT('Ctrl Pts',(1.87785249931966,-7.90950617504113,
61.9907871897118));
#175740=CARTESIAN_POINT('Ctrl Pts',(1.3714804935247,-8.01282360825074,61.9709363988586));
#175741=CARTESIAN_POINT('Ctrl Pts',(1.1162828344953,-8.05234197028682,61.9609835006251));
#175742=CARTESIAN_POINT('Ctrl Pts',(0.78095028817407,-8.0880199317794,61.9478681832114));
#175743=CARTESIAN_POINT('Ctrl Pts',(0.702142483920749,-8.09524215925793,
61.9447836955023));
#175744=CARTESIAN_POINT('Ctrl Pts',(0.568260862463784,-8.10554180646614,
61.9395380810763));
#175745=CARTESIAN_POINT('Ctrl Pts',(0.513238168799655,-8.10921173352463,
61.9373806566744));
#175746=CARTESIAN_POINT('Ctrl Pts',(0.398391891898013,-8.11569823152074,
61.9328738532247));
#175747=CARTESIAN_POINT('Ctrl Pts',(0.338565899703413,-8.11841406833795,
61.9305240581155));
#175748=CARTESIAN_POINT('Ctrl Pts',(0.162614985591844,-8.12445315920515,
61.9236068139472));
#175749=CARTESIAN_POINT('Ctrl Pts',(0.046442743288885,-8.12594767860219,
61.9190313378358));
#175750=CARTESIAN_POINT('Ctrl Pts',(-0.306702637332613,-8.12291729740619,
61.9051017399361));
#175751=CARTESIAN_POINT('Ctrl Pts',(-0.543481870822225,-8.11051660733493,
61.8957308207934));
#175752=CARTESIAN_POINT('Ctrl Pts',(-0.825419238152854,-8.08334769458556,
61.8845899582229));
#175753=CARTESIAN_POINT('Ctrl Pts',(-0.871419998375232,-8.078518061831,
61.8827729047744));
#175754=CARTESIAN_POINT('Ctrl Pts',(-0.959825596665691,-8.06847244073484,
61.8792831720209));
#175755=CARTESIAN_POINT('Ctrl Pts',(-1.00223544949722,-8.06331425764931,
61.8776101989663));
#175756=CARTESIAN_POINT('Ctrl Pts',(-1.14664729274457,-8.0445929449074,
61.8719145879527));
#175757=CARTESIAN_POINT('Ctrl Pts',(-1.24843169712396,-8.02942675979171,
61.8679019667794));
#175758=CARTESIAN_POINT('Ctrl Pts',(-1.54561554432345,-7.97935784802296,
61.8561607164715));
#175759=CARTESIAN_POINT('Ctrl Pts',(-1.74005619463509,-7.93922435869023,
61.8484449843567));
#175760=CARTESIAN_POINT('Ctrl Pts',(-2.01370625907561,-7.87220475345948,
61.8374526241279));
#175761=CARTESIAN_POINT('Ctrl Pts',(-2.09427140311719,-7.85115582589881,
61.8341999260927));
#175762=CARTESIAN_POINT('Ctrl Pts',(-2.22834613981786,-7.81391606660522,
61.8287537009817));
#175763=CARTESIAN_POINT('Ctrl Pts',(-2.28203784649393,-7.7984045840702,
61.8265637382998));
#175764=CARTESIAN_POINT('Ctrl Pts',(-2.39258791821276,-7.76522730340484,
61.8220343642352));
#175765=CARTESIAN_POINT('Ctrl Pts',(-2.4494207461888,-7.74748797961997,
61.8196946682721));
#175766=CARTESIAN_POINT('Ctrl Pts',(-2.60249712413585,-7.69785525494417,
61.8133602274957));
#175767=CARTESIAN_POINT('Ctrl Pts',(-2.69834673310783,-7.6647825500432,
61.8093587108608));
#175768=CARTESIAN_POINT('Ctrl Pts',(-3.12289377704863,-7.50934272681272,
61.7914640469587));
#175769=CARTESIAN_POINT('Ctrl Pts',(-3.44407959679674,-7.36756432997102,
61.7774480702845));
#175770=CARTESIAN_POINT('Ctrl Pts',(-3.98374446877178,-7.08632117156818,
61.7530861434291));
#175771=CARTESIAN_POINT('Ctrl Pts',(-4.20659552217092,-6.95634415889652,
61.7427698769314));
#175772=CARTESIAN_POINT('Ctrl Pts',(-4.46003845374512,-6.791885278389,61.7308234533547));
#175773=CARTESIAN_POINT('Ctrl Pts',(-4.49698930193048,-6.7674763310802,
61.7290762995698));
#175774=CARTESIAN_POINT('Ctrl Pts',(-4.55525181108142,-6.72830146036634,
61.7263137215263));
#175775=CARTESIAN_POINT('Ctrl Pts',(-4.57669543941068,-6.7137335712442,
61.7252952677873));
#175776=CARTESIAN_POINT('Ctrl Pts',(-4.61447452854532,-6.68780295186171,
61.7234982001473));
#175777=CARTESIAN_POINT('Ctrl Pts',(-4.63083863865992,-6.67648238248094,
61.7227188695024));
#175778=CARTESIAN_POINT('Ctrl Pts',(-4.66519472401123,-6.65252802048314,
61.7210808459859));
#175779=CARTESIAN_POINT('Ctrl Pts',(-4.68317727619349,-6.63988113448914,
61.7202224409685));
#175780=CARTESIAN_POINT('Ctrl Pts',(-4.73693808579128,-6.60174483752643,
61.717652869569));
#175781=CARTESIAN_POINT('Ctrl Pts',(-4.77256123059647,-6.5760380672491,
61.7159457256849));
#175782=CARTESIAN_POINT('Ctrl Pts',(-4.85654681896081,-6.5143895383639,
61.7119073301713));
#175783=CARTESIAN_POINT('Ctrl Pts',(-4.90472147275561,-6.47819615344555,
61.7095800121605));
#175784=CARTESIAN_POINT('Ctrl Pts',(-5.08931854848621,-6.33626969529422,
61.7006082172586));
#175785=CARTESIAN_POINT('Ctrl Pts',(-5.22276188287721,-6.22673557689064,
61.6940060646147));
#175786=CARTESIAN_POINT('Ctrl Pts',(-5.56354347062184,-5.92834481329625,
61.6766734579828));
#175787=CARTESIAN_POINT('Ctrl Pts',(-5.76476847883351,-5.73286406727149,
61.6659446193856));
#175788=CARTESIAN_POINT('Ctrl Pts',(-6.00262996547609,-5.47657958061562,
61.652404952417));
#175789=CARTESIAN_POINT('Ctrl Pts',(-6.04912250091376,-5.42518269725157,
61.6497147129244));
#175790=CARTESIAN_POINT('Ctrl Pts',(-6.12146995540695,-5.3431171797327,
61.6454560625029));
#175791=CARTESIAN_POINT('Ctrl Pts',(-6.14776514359542,-5.31284098530027,
61.6438926687732));
#175792=CARTESIAN_POINT('Ctrl Pts',(-6.1964469889122,-5.25594349399365,
61.6409685746474));
#175793=CARTESIAN_POINT('Ctrl Pts',(-6.21888893714445,-5.22937067683744,
61.6396085262119));
#175794=CARTESIAN_POINT('Ctrl Pts',(-6.26944326411468,-5.16872517156314,
61.6365169514494));
#175795=CARTESIAN_POINT('Ctrl Pts',(-6.29744977109725,-5.13456571688859,
61.6347843242804));
#175796=CARTESIAN_POINT('Ctrl Pts',(-6.38389496117759,-5.02735752053206,
61.6293731591286));
#175797=CARTESIAN_POINT('Ctrl Pts',(-6.44135133999584,-4.95352715216749,
61.6256846313344));
#175798=CARTESIAN_POINT('Ctrl Pts',(-6.57804371246188,-4.77147917450536,
61.6166799861609));
#175799=CARTESIAN_POINT('Ctrl Pts',(-6.65589974403492,-4.66226026696053,
61.6113527434064));
#175800=CARTESIAN_POINT('Ctrl Pts',(-6.8109787738291,-4.43290372672422,
61.6003274637109));
#175801=CARTESIAN_POINT('Ctrl Pts',(-6.88781038445357,-4.31255554272703,
61.594629493107));
#175802=CARTESIAN_POINT('Ctrl Pts',(-7.04155796220453,-4.057128254136,61.5827435935202));
#175803=CARTESIAN_POINT('Ctrl Pts',(-7.11785046002824,-3.92173860166251,
61.5765591373405));
#175804=CARTESIAN_POINT('Ctrl Pts',(-7.20598200657805,-3.7542851571309,
61.5690831787386));
#175805=CARTESIAN_POINT('Ctrl Pts',(-7.22156222153079,-3.72422781448013,
61.5677479563913));
#175806=CARTESIAN_POINT('Ctrl Pts',(-7.24535112640807,-3.67762365350201,
61.5656885457635));
#175807=CARTESIAN_POINT('Ctrl Pts',(-7.2536919857583,-3.66114480183142,
61.5649624404453));
#175808=CARTESIAN_POINT('Ctrl Pts',(-7.26946435218926,-3.62971820535078,
61.5635817760801));
#175809=CARTESIAN_POINT('Ctrl Pts',(-7.27690612471744,-3.61477571536043,
61.562927056102));
#175810=CARTESIAN_POINT('Ctrl Pts',(-7.29498961651387,-3.57818334004305,
61.5613281079596));
#175811=CARTESIAN_POINT('Ctrl Pts',(-7.30558108080675,-3.55650876532049,
61.5603847438999));
#175812=CARTESIAN_POINT('Ctrl Pts',(-7.34128920710725,-3.48260237703531,
61.5571802417162));
#175813=CARTESIAN_POINT('Ctrl Pts',(-7.36594360049633,-3.43014890166331,
61.5549265616023));
#175814=CARTESIAN_POINT('Ctrl Pts',(-7.42496324921254,-3.30101032549842,
61.5494237355752));
#175815=CARTESIAN_POINT('Ctrl Pts',(-7.45870425400993,-3.22404706107066,
61.5461831614131));
#175816=CARTESIAN_POINT('Ctrl Pts',(-7.64685488975612,-2.77610504818729,
61.5275134563248));
#175817=CARTESIAN_POINT('Ctrl Pts',(-7.77476992081399,-2.39459972790696,
61.5123492254595));
#175818=CARTESIAN_POINT('Ctrl Pts',(-7.97017323991821,-1.6272973329033,
61.482232868238));
#175819=CARTESIAN_POINT('Ctrl Pts',(-8.03907875170318,-1.24296508113117,
61.4673242886985));
#175820=CARTESIAN_POINT('Ctrl Pts',(-8.08780429090186,-0.782584465608853,
61.4493419320412));
#175821=CARTESIAN_POINT('Ctrl Pts',(-8.09450888817357,-0.709889057082839,
61.4464994618613));
#175822=CARTESIAN_POINT('Ctrl Pts',(-8.10359536137866,-0.594364031135042,
61.441976010416));
#175823=CARTESIAN_POINT('Ctrl Pts',(-8.10661928465596,-0.551588741911865,
61.4402997564319));
#175824=CARTESIAN_POINT('Ctrl Pts',(-8.1116548188829,-0.471330579643435,
61.437151806774));
#175825=CARTESIAN_POINT('Ctrl Pts',(-8.1137455781137,-0.433853776364693,
61.4356807033261));
#175826=CARTESIAN_POINT('Ctrl Pts',(-8.11786818376271,-0.349443158880844,
61.4323644819724));
#175827=CARTESIAN_POINT('Ctrl Pts',(-8.11975282665341,-0.302503528540085,
61.4305184322093));
#175828=CARTESIAN_POINT('Ctrl Pts',(-8.12425218016602,-0.159516862081264,
61.4248887483838));
#175829=CARTESIAN_POINT('Ctrl Pts',(-8.12557041786649,-0.0634377752123971,
61.4210972420416));
#175830=CARTESIAN_POINT('Ctrl Pts',(-8.12356828760708,0.434934049148002,
61.4013830069805));
#175831=CARTESIAN_POINT('Ctrl Pts',(-8.09207729568715,0.836542689192359,
61.3854020371046));
#175832=CARTESIAN_POINT('Ctrl Pts',(-7.94312641934823,1.80580367579763,
61.3454643083025));
#175833=CARTESIAN_POINT('Ctrl Pts',(-7.79449744559859,2.36641543206504,
61.3210105496806));
#175834=CARTESIAN_POINT('Ctrl Pts',(-7.45926099603663,3.24159150537307,
61.2813935792335));
#175835=CARTESIAN_POINT('Ctrl Pts',(-7.3088143056645,3.56787654615489,61.2663223215167));
#175836=CARTESIAN_POINT('Ctrl Pts',(-7.12661772412565,3.90275613116896,
61.2511555210289));
#175837=CARTESIAN_POINT('Ctrl Pts',(-7.11587144578774,3.92231553855636,
61.2502709091544));
#175838=CARTESIAN_POINT('Ctrl Pts',(-7.10073471219003,3.94959909810885,
61.2490389504922));
#175839=CARTESIAN_POINT('Ctrl Pts',(-7.09641201802787,3.95736060523233,
61.2486887147537));
#175840=CARTESIAN_POINT('Ctrl Pts',(-7.08849021999816,3.97152967674962,
61.248049775112));
#175841=CARTESIAN_POINT('Ctrl Pts',(-7.08489513882653,3.97793947221306,
61.2477608952793));
#175842=CARTESIAN_POINT('Ctrl Pts',(-7.07762150663957,3.99086674547418,
61.2471786258198));
#175843=CARTESIAN_POINT('Ctrl Pts',(-7.07394263697814,3.99738403716737,
61.246885250874));
#175844=CARTESIAN_POINT('Ctrl Pts',(-7.06491585727204,4.01332391877098,
61.2461681691995));
#175845=CARTESIAN_POINT('Ctrl Pts',(-7.05955808581796,4.02274092898861,
61.2457449149994));
#175846=CARTESIAN_POINT('Ctrl Pts',(-7.04023377764377,4.05654851815236,
61.2442268740445));
#175847=CARTESIAN_POINT('Ctrl Pts',(-7.02615943859548,4.08087749074562,
61.2431371911178));
#175848=CARTESIAN_POINT('Ctrl Pts',(-6.74597066269945,4.55946664879856,
61.2217633867272));
#175849=CARTESIAN_POINT('Ctrl Pts',(-6.43644439311334,4.98689027910571,
61.2039625492203));
#175850=CARTESIAN_POINT('Ctrl Pts',(-5.60872534562217,5.92325868789787,
61.162200081619));
#175851=CARTESIAN_POINT('Ctrl Pts',(-5.05954832784191,6.39872730018576,
61.1383400024782));
#175852=CARTESIAN_POINT('Ctrl Pts',(-4.3646357413689,6.85428640341238,61.107215830422));
#175853=CARTESIAN_POINT('Ctrl Pts',(-4.27340048671877,6.91153633511982,
61.1031206324968));
#175854=CARTESIAN_POINT('Ctrl Pts',(-4.16377144545252,6.97732765980867,
61.0981827127597));
#175855=CARTESIAN_POINT('Ctrl Pts',(-4.14644828723428,6.98763626104161,
61.0974019498304));
#175856=CARTESIAN_POINT('Ctrl Pts',(-4.11844052257241,7.00416219367493,
61.0961387900911));
#175857=CARTESIAN_POINT('Ctrl Pts',(-4.10777973140671,7.01041981980389,
61.0956577902534));
#175858=CARTESIAN_POINT('Ctrl Pts',(-4.08875390511109,7.02152921940628,
61.0947990151759));
#175859=CARTESIAN_POINT('Ctrl Pts',(-4.0803943998404,7.02639044008455,61.094421567099));
#175860=CARTESIAN_POINT('Ctrl Pts',(-4.06308993406297,7.03641203966904,
61.0936399784184));
#175861=CARTESIAN_POINT('Ctrl Pts',(-4.05414377642814,7.04157031090248,
61.0932357662378));
#175862=CARTESIAN_POINT('Ctrl Pts',(-4.03102394421308,7.05484232634771,
61.0921907737771));
#175863=CARTESIAN_POINT('Ctrl Pts',(-4.0168356276749,7.06293039926917,61.0915491141526));
#175864=CARTESIAN_POINT('Ctrl Pts',(-3.98592294802465,7.08042894707689,
61.0901502928308));
#175865=CARTESIAN_POINT('Ctrl Pts',(-3.96918945675955,7.08982304944259,
61.0893925763861));
#175866=CARTESIAN_POINT('Ctrl Pts',(-3.92063466039204,7.11685570550575,
61.0871924160428));
#175867=CARTESIAN_POINT('Ctrl Pts',(-3.88872815607519,7.1343398124449,61.0857447419105));
#175868=CARTESIAN_POINT('Ctrl Pts',(-3.56948260151329,7.30650192572491,
61.0712401536745));
#175869=CARTESIAN_POINT('Ctrl Pts',(-3.27321314273342,7.44393866513744,
61.0576050810417));
#175870=CARTESIAN_POINT('Ctrl Pts',(-2.58247179560257,7.71514166658305,
61.0255476920333));
#175871=CARTESIAN_POINT('Ctrl Pts',(-2.18436564951852,7.83716049459927,
61.0068720976049));
#175872=CARTESIAN_POINT('Ctrl Pts',(-1.26458408332123,8.04351480764306,
60.964533921876));
#175873=CARTESIAN_POINT('Ctrl Pts',(-0.740383610719197,8.1085952819358,
60.9409806207243));
#175874=CARTESIAN_POINT('Ctrl Pts',(-0.1825648725882,8.12325767747229,60.9185733810647));
#175875=CARTESIAN_POINT('Ctrl Pts',(-0.151624703333772,8.12389409172628,
60.9173384552744));
#175876=CARTESIAN_POINT('Ctrl Pts',(-0.108733545335255,8.12453120865442,
60.9156366988931));
#175877=CARTESIAN_POINT('Ctrl Pts',(-0.0967853111397488,8.12468232916457,
60.9151637330466));
#175878=CARTESIAN_POINT('Ctrl Pts',(-0.0776770240843752,8.12488185204107,
60.9144090362036));
#175879=CARTESIAN_POINT('Ctrl Pts',(-0.070517192407656,8.12494714787237,
60.9141266339489));
#175880=CARTESIAN_POINT('Ctrl Pts',(-0.0557722640516926,8.12506212609247,
60.9135458257129));
#175881=CARTESIAN_POINT('Ctrl Pts',(-0.0481871645174521,8.12511065130447,
60.9132474653224));
#175882=CARTESIAN_POINT('Ctrl Pts',(-0.0305899512860504,8.12519858593376,
60.9125562314602));
#175883=CARTESIAN_POINT('Ctrl Pts',(-0.0205777981007368,8.12523011128357,
60.9121636615602));
#175884=CARTESIAN_POINT('Ctrl Pts',(0.0111078971516225,8.12527131348465,
60.9109234918231));
#175885=CARTESIAN_POINT('Ctrl Pts',(0.0327815299780469,8.12521277783753,
60.9100784569328));
#175886=CARTESIAN_POINT('Ctrl Pts',(0.518396730850356,8.12195814959084,
60.8912135749861));
#175887=CARTESIAN_POINT('Ctrl Pts',(0.981254947947732,8.07911744903377,
60.8745905294104));
#175888=CARTESIAN_POINT('Ctrl Pts',(1.83850391449729,7.92497464002435,60.8433212049468));
#175889=CARTESIAN_POINT('Ctrl Pts',(2.2330717166765,7.82295990687601,60.8287294406177));
#175890=CARTESIAN_POINT('Ctrl Pts',(2.87554546160043,7.60425876813392,60.8035885545911));
#175891=CARTESIAN_POINT('Ctrl Pts',(3.12819743219707,7.50385805839592,60.7933336200218));
#175892=CARTESIAN_POINT('Ctrl Pts',(3.42011051805385,7.37054639615745,60.7809705478439));
#175893=CARTESIAN_POINT('Ctrl Pts',(3.4646953526693,7.34969361257639,60.7790679521608));
#175894=CARTESIAN_POINT('Ctrl Pts',(3.53276679155353,7.31709885217607,60.7761410123672));
#175895=CARTESIAN_POINT('Ctrl Pts',(3.55639068008394,7.30564590844781,60.7751211171078));
#175896=CARTESIAN_POINT('Ctrl Pts',(3.5995829255423,7.28444700775809,60.7732488793961));
#175897=CARTESIAN_POINT('Ctrl Pts',(3.61916829301732,7.27473616764047,60.7723970684399));
#175898=CARTESIAN_POINT('Ctrl Pts',(3.65988955042922,7.25434055743921,60.7706200470351));
#175899=CARTESIAN_POINT('Ctrl Pts',(3.68101842361429,7.24364216430808,60.7696946295668));
#175900=CARTESIAN_POINT('Ctrl Pts',(3.73506221449023,7.21598011075325,60.7673186619841));
#175901=CARTESIAN_POINT('Ctrl Pts',(3.76790841166634,7.19888358605946,60.7658660939672));
#175902=CARTESIAN_POINT('Ctrl Pts',(3.90602873709278,7.12578736285463,60.7597205080133));
#175903=CARTESIAN_POINT('Ctrl Pts',(4.01017890308169,7.06769909188581,60.7549937797083));
#175904=CARTESIAN_POINT('Ctrl Pts',(4.2728839759304,6.91350235844712,60.7428109601154));
#175905=CARTESIAN_POINT('Ctrl Pts',(4.42949409816638,6.81422272803062,60.7352977337067));
#175906=CARTESIAN_POINT('Ctrl Pts',(4.96727551700171,6.44692925676997,60.7085560816244));
#175907=CARTESIAN_POINT('Ctrl Pts',(5.32865914823077,6.15159164251842,60.6887909456451));
#175908=CARTESIAN_POINT('Ctrl Pts',(5.94531495419874,5.55231416255085,60.6523221694996));
#175909=CARTESIAN_POINT('Ctrl Pts',(6.20756351610341,5.25748439611811,60.6356834160601));
#175910=CARTESIAN_POINT('Ctrl Pts',(6.46005269871621,4.92826944339104,60.6191368695381));
#175911=CARTESIAN_POINT('Ctrl Pts',(6.47265301497333,4.91170882013923,60.6183096824065));
#175912=CARTESIAN_POINT('Ctrl Pts',(6.4912694697758,4.88704512735089,60.6170855916737));
#175913=CARTESIAN_POINT('Ctrl Pts',(6.49733430545904,4.87897902539082,60.6166864983251));
#175914=CARTESIAN_POINT('Ctrl Pts',(6.50769768075396,4.86514236526821,60.6160040335542));
#175915=CARTESIAN_POINT('Ctrl Pts',(6.51200360423369,4.85937736724523,60.6157203221113));
#175916=CARTESIAN_POINT('Ctrl Pts',(6.52082443768452,4.84753478960648,60.6151388299771));
#175917=CARTESIAN_POINT('Ctrl Pts',(6.52533852323877,4.84145660324821,60.6148410879811));
#175918=CARTESIAN_POINT('Ctrl Pts',(6.53574575209892,4.82740234213295,60.6141542841525));
#175919=CARTESIAN_POINT('Ctrl Pts',(6.54163280889005,4.81942176030033,60.6137655124283));
#175920=CARTESIAN_POINT('Ctrl Pts',(6.56004136314681,4.79437097586078,60.6125490472261));
#175921=CARTESIAN_POINT('Ctrl Pts',(6.57251082754709,4.77726251875835,60.6117238888044));
#175922=CARTESIAN_POINT('Ctrl Pts',(6.76887688357308,4.50561864708963,60.5987133809843));
#175923=CARTESIAN_POINT('Ctrl Pts',(6.93792910374296,4.24068738920564,60.5873947578006));
#175924=CARTESIAN_POINT('Ctrl Pts',(7.4397684916167,3.34354093246848,60.5516780980573));
#175925=CARTESIAN_POINT('Ctrl Pts',(7.70467034127299,2.67722706093914,60.5288058451769));
#175926=CARTESIAN_POINT('Ctrl Pts',(7.89231785046553,1.93234034338486,60.5014377636945));
#175927=CARTESIAN_POINT('Ctrl Pts',(7.90502134347635,1.87969617604864,60.4994959447511));
#175928=CARTESIAN_POINT('Ctrl Pts',(7.97060789579515,1.5954697078088,60.4889638419832));
#175929=CARTESIAN_POINT('Ctrl Pts',(8.0138397396152,1.36179164406858,60.4801287633887));
#175930=CARTESIAN_POINT('Ctrl Pts',(8.05030829620179,1.10130577618197,60.469996262894));
#175931=CARTESIAN_POINT('Ctrl Pts',(8.05372561464904,1.07603056952247,60.4690102117594));
#175932=CARTESIAN_POINT('Ctrl Pts',(8.05865928521796,1.03819941428734,60.4675299132235));
#175933=CARTESIAN_POINT('Ctrl Pts',(8.06026543203758,1.02565523566158,60.4670383471084));
#175934=CARTESIAN_POINT('Ctrl Pts',(8.06298135964844,1.00404313390011,60.466190179523));
#175935=CARTESIAN_POINT('Ctrl Pts',(8.06410514757114,0.994976979138242,
60.4658339967926));
#175936=CARTESIAN_POINT('Ctrl Pts',(8.06633167306843,0.976762920415431,
60.465117649003));
#175937=CARTESIAN_POINT('Ctrl Pts',(8.06743414470222,0.967614997243684,
60.4647574765578));
#175938=CARTESIAN_POINT('Ctrl Pts',(8.06963369641106,0.949098802184107,
60.4640276615495));
#175939=CARTESIAN_POINT('Ctrl Pts',(8.07073002879028,0.939730457217788,
60.4636579972944));
#175940=CARTESIAN_POINT('Ctrl Pts',(8.07321103190454,0.918205262005532,
60.4628076869764));
#175941=CARTESIAN_POINT('Ctrl Pts',(8.07458455921479,0.906047163976217,
60.4623267091662));
#175942=CARTESIAN_POINT('Ctrl Pts',(8.07803815102685,0.874845236051451,
60.4610905531158));
#175943=CARTESIAN_POINT('Ctrl Pts',(8.08007833166224,0.855797116500719,
60.4603341873944));
#175944=CARTESIAN_POINT('Ctrl Pts',(8.11085524543148,0.558524385973172,
60.4485029571617));
#175945=CARTESIAN_POINT('Ctrl Pts',(8.12527172054597,0.279029717082663,
60.437000513906));
#175946=CARTESIAN_POINT('Ctrl Pts',(8.12524997543795,-0.000631779635134194,
60.4251159836211));
#175947=CARTESIAN_POINT('',(8.13321556035325,-0.00564624965199908,58.4167025567876));
#175948=CARTESIAN_POINT('Ctrl Pts',(8.12524804204743,-0.00564071843287404,
58.4167025567876));
#175949=CARTESIAN_POINT('Ctrl Pts',(8.12538636330396,0.193605978980111,
58.4245358486659));
#175950=CARTESIAN_POINT('Ctrl Pts',(8.11819169268104,0.393119237488508,
58.4323691405441));
#175951=CARTESIAN_POINT('Ctrl Pts',(8.10363182462515,0.592316480795924,
58.4402024324224));
#175952=CARTESIAN_POINT('Ctrl Pts',(8.08908683718342,0.791310138651282,
58.4480277184455));
#175953=CARTESIAN_POINT('Ctrl Pts',(8.06719166999482,0.989988084929009,
58.4558530044687));
#175954=CARTESIAN_POINT('Ctrl Pts',(8.03796611065937,1.18776612445018,58.4636782904918));
#175955=CARTESIAN_POINT('Ctrl Pts',(8.00877136902933,1.38533561140653,58.4714953249241));
#175956=CARTESIAN_POINT('Ctrl Pts',(7.97226169411772,1.5820067454906,58.4793123593564));
#175957=CARTESIAN_POINT('Ctrl Pts',(7.92850878668791,1.77719891455983,58.4871293937886));
#175958=CARTESIAN_POINT('Ctrl Pts',(7.88478257898052,1.97227196979093,58.494941657963));
#175959=CARTESIAN_POINT('Ctrl Pts',(7.83382201664854,2.16586752378011,58.5027539221375));
#175960=CARTESIAN_POINT('Ctrl Pts',(7.7757502551909,2.35741288946139,58.5105661863119));
#175961=CARTESIAN_POINT('Ctrl Pts',(7.71770715655588,2.54886371296411,58.5183745945409));
#175962=CARTESIAN_POINT('Ctrl Pts',(7.65255995253317,2.73826603678667,58.5261830027699));
#175963=CARTESIAN_POINT('Ctrl Pts',(7.58048229823073,2.92505994617384,58.533991410999));
#175964=CARTESIAN_POINT('Ctrl Pts',(7.53647218251617,3.03911501145677,58.5387591708967));
#175965=CARTESIAN_POINT('Ctrl Pts',(7.48987921437218,3.15219785171096,58.5435269307944));
#175966=CARTESIAN_POINT('Ctrl Pts',(7.44075200433562,3.2641839979504,58.5482946906921));
#175967=CARTESIAN_POINT('Ctrl Pts',(7.35794340140681,3.45294733929565,58.5563312052008));
#175968=CARTESIAN_POINT('Ctrl Pts',(7.26798055620304,3.63848305674189,58.5643677197096));
#175969=CARTESIAN_POINT('Ctrl Pts',(7.17115218707309,3.82024395455799,58.5724042342183));
#175970=CARTESIAN_POINT('Ctrl Pts',(7.07426532397069,4.00211465404734,58.5804456035816));
#175971=CARTESIAN_POINT('Ctrl Pts',(6.97050481102578,4.18020570571134,58.588486972945));
#175972=CARTESIAN_POINT('Ctrl Pts',(6.86020417375442,4.35399658439259,58.5965283423083));
#175973=CARTESIAN_POINT('Ctrl Pts',(6.74982341759097,4.52791369926795,58.6045755526679));
#175974=CARTESIAN_POINT('Ctrl Pts',(6.6328932283692,4.69752414308522,58.6126227630274));
#175975=CARTESIAN_POINT('Ctrl Pts',(6.50978943598929,4.86233781853773,58.620669973387));
#175976=CARTESIAN_POINT('Ctrl Pts',(6.38650419741034,5.02739441757839,58.62872904476));
#175977=CARTESIAN_POINT('Ctrl Pts',(6.2570273581813,5.18763986421855,58.636788116133));
#175978=CARTESIAN_POINT('Ctrl Pts',(6.12177501879248,5.34261716593921,58.6448471875059));
#175979=CARTESIAN_POINT('Ctrl Pts',(5.98641321304975,5.49771989839352,58.6529127814808));
#175980=CARTESIAN_POINT('Ctrl Pts',(5.84526679511342,5.64754574778535,58.6609783754556));
#175981=CARTESIAN_POINT('Ctrl Pts',(5.69878808873808,5.79167522243409,58.6690439694304));
#175982=CARTESIAN_POINT('Ctrl Pts',(5.55207937732762,5.93603101328741,58.6771222282305));
#175983=CARTESIAN_POINT('Ctrl Pts',(5.40002187451157,6.07467233789709,58.6852004870307));
#175984=CARTESIAN_POINT('Ctrl Pts',(5.24310162096852,6.20721942214848,58.6932787458308));
#175985=CARTESIAN_POINT('Ctrl Pts',(5.15450149715187,6.28205799659028,58.6978398825468));
#175986=CARTESIAN_POINT('Ctrl Pts',(5.06435170617298,6.3549545324053,58.7024010192627));
#175987=CARTESIAN_POINT('Ctrl Pts',(4.97274368742692,6.42584685326811,58.7069621559787));
#175988=CARTESIAN_POINT('Ctrl Pts',(4.81033676276519,6.55152803239476,58.7150483497109));
#175989=CARTESIAN_POINT('Ctrl Pts',(4.64302902299906,6.67115206366083,58.723134543443));
#175990=CARTESIAN_POINT('Ctrl Pts',(4.47129960638425,6.78433249424349,58.7312207371752));
#175991=CARTESIAN_POINT('Ctrl Pts',(4.2997233642602,6.89741197325267,58.7392997184063));
#175992=CARTESIAN_POINT('Ctrl Pts',(4.12373357235079,7.00405913783073,58.7473786996374));
#175993=CARTESIAN_POINT('Ctrl Pts',(3.94384075842282,7.10392902798887,58.7554576808684));
#175994=CARTESIAN_POINT('Ctrl Pts',(3.76408383502655,7.20372347670954,58.7635305592595));
#175995=CARTESIAN_POINT('Ctrl Pts',(3.58043004481467,7.29675070657168,58.7716034376506));
#175996=CARTESIAN_POINT('Ctrl Pts',(3.39341762130824,7.3827098283689,58.7796763160417));
#175997=CARTESIAN_POINT('Ctrl Pts',(3.20652096684773,7.46861573762905,58.7877441969604));
#175998=CARTESIAN_POINT('Ctrl Pts',(3.01627011257903,7.54746213275558,58.7958120778791));
#175999=CARTESIAN_POINT('Ctrl Pts',(2.82322710233959,7.61899444094266,58.8038799587978));
#176000=CARTESIAN_POINT('Ctrl Pts',(2.63027730488765,7.69049220902475,58.8119439440578));
#176001=CARTESIAN_POINT('Ctrl Pts',(2.43453833700815,7.75468282419935,58.8200079293179));
#176002=CARTESIAN_POINT('Ctrl Pts',(2.2365919758216,7.81135992617101,58.8280719145779));
#176003=CARTESIAN_POINT('Ctrl Pts',(2.03589479408909,7.8688246583656,58.8362479634101));
#176004=CARTESIAN_POINT('Ctrl Pts',(1.83292871753126,7.91856537212488,58.8444240122423));
#176005=CARTESIAN_POINT('Ctrl Pts',(1.62831702554787,7.96041903588064,58.8526000610746));
#176006=CARTESIAN_POINT('Ctrl Pts',(1.42660542133468,8.00167948183336,58.8606602257215));
#176007=CARTESIAN_POINT('Ctrl Pts',(1.2232948623812,8.03527491782727,58.8687203903684));
#176008=CARTESIAN_POINT('Ctrl Pts',(1.01899407762534,8.06110033632286,58.8767805550154));
#176009=CARTESIAN_POINT('Ctrl Pts',(0.814703163657677,8.08692450706388,
58.8848403302356));
#176010=CARTESIAN_POINT('Ctrl Pts',(0.609422433575708,8.10497936945029,
58.8929001054559));
#176011=CARTESIAN_POINT('Ctrl Pts',(0.403767332793357,8.11521161174919,
58.9009598806762));
#176012=CARTESIAN_POINT('Ctrl Pts',(0.198096704788882,8.12544462659542,
58.9090202644197));
#176013=CARTESIAN_POINT('Ctrl Pts',(-0.00794803388750687,8.12785382821346,
58.9170806481632));
#176014=CARTESIAN_POINT('Ctrl Pts',(-0.213749224837953,8.12243798569008,
58.9251410319068));
#176015=CARTESIAN_POINT('Ctrl Pts',(-0.42472381762285,8.11688600046745,
58.9334040364605));
#176016=CARTESIAN_POINT('Ctrl Pts',(-0.635442107449402,8.10311040649792,
58.9416670410142));
#176017=CARTESIAN_POINT('Ctrl Pts',(-0.845241631071249,8.08116663283242,
58.9499300455679));
#176018=CARTESIAN_POINT('Ctrl Pts',(-1.05006486157437,8.05974334962373,
58.9579970576237));
#176019=CARTESIAN_POINT('Ctrl Pts',(-1.25401209977637,8.03053504270057,
58.9660640696795));
#176020=CARTESIAN_POINT('Ctrl Pts',(-1.45647449919524,7.9936455760619,58.9741310817353));
#176021=CARTESIAN_POINT('Ctrl Pts',(-1.66631530175634,7.95541173457959,
58.982492082538));
#176022=CARTESIAN_POINT('Ctrl Pts',(-1.87456064031404,7.90892643445054,
58.9908530833407));
#176023=CARTESIAN_POINT('Ctrl Pts',(-2.08054651029981,7.85436272277893,
58.9992140841433));
#176024=CARTESIAN_POINT('Ctrl Pts',(-2.28653238028559,7.79979901110732,
59.007575084946));
#176025=CARTESIAN_POINT('Ctrl Pts',(-2.49025842832984,7.73715702172116,
59.0159360857487));
#176026=CARTESIAN_POINT('Ctrl Pts',(-2.69108010185902,7.66666651471671,
59.0242970865514));
#176027=CARTESIAN_POINT('Ctrl Pts',(-2.87310087245517,7.60277532120567,
59.0318753313809));
#176028=CARTESIAN_POINT('Ctrl Pts',(-3.05310033015549,7.53230813123251,
59.0394535762103));
#176029=CARTESIAN_POINT('Ctrl Pts',(-3.23054793484947,7.45541733259379,
59.0470318210397));
#176030=CARTESIAN_POINT('Ctrl Pts',(-3.40786349611596,7.37858375041967,
59.054604426698));
#176031=CARTESIAN_POINT('Ctrl Pts',(-3.5826306470187,7.29533621379642,59.0621770323562));
#176032=CARTESIAN_POINT('Ctrl Pts',(-3.75433463186656,7.20587670130897,
59.0697496380144));
#176033=CARTESIAN_POINT('Ctrl Pts',(-3.9259434533907,7.11646676987552,59.0773180467152));
#176034=CARTESIAN_POINT('Ctrl Pts',(-4.09449216222265,7.02085188261255,
59.084886455416));
#176035=CARTESIAN_POINT('Ctrl Pts',(-4.25948666092877,6.91928182312802,
59.0924548641167));
#176036=CARTESIAN_POINT('Ctrl Pts',(-4.42444129564691,6.81773630378066,
59.1000214442295));
#176037=CARTESIAN_POINT('Ctrl Pts',(-4.5858431126521,6.71023866162834,59.1075880243423));
#176038=CARTESIAN_POINT('Ctrl Pts',(-4.7432231696582,6.59708432000968,59.1151546044551));
#176039=CARTESIAN_POINT('Ctrl Pts',(-4.9005753081548,6.48395005145887,59.1227198422908));
#176040=CARTESIAN_POINT('Ctrl Pts',(-5.05390680998816,6.36516129799542,
59.1302850801266));
#176041=CARTESIAN_POINT('Ctrl Pts',(-5.20277848913424,6.24105628523746,
59.1378503179623));
#176042=CARTESIAN_POINT('Ctrl Pts',(-5.35170193810663,6.1169081152115,59.1454181865943));
#176043=CARTESIAN_POINT('Ctrl Pts',(-5.49616218113374,5.9874402257623,59.1529860552263));
#176044=CARTESIAN_POINT('Ctrl Pts',(-5.63575349523875,5.85303084763818,
59.1605539238582));
#176045=CARTESIAN_POINT('Ctrl Pts',(-5.77354345794196,5.7203559507979,59.1680241331848));
#176046=CARTESIAN_POINT('Ctrl Pts',(-5.90658918307767,5.58286660992183,
59.1754943425114));
#176047=CARTESIAN_POINT('Ctrl Pts',(-6.03453665110089,5.44096084979667,
59.182964551838));
#176048=CARTESIAN_POINT('Ctrl Pts',(-6.19392426641852,5.26418501315344,
59.1922703932813));
#176049=CARTESIAN_POINT('Ctrl Pts',(-6.34532358992774,5.08064389841133,
59.2015762347245));
#176050=CARTESIAN_POINT('Ctrl Pts',(-6.4882623953925,4.89102633922939,59.2108820761678));
#176051=CARTESIAN_POINT('Ctrl Pts',(-6.63196861046514,4.70039076162852,
59.2202378787963));
#176052=CARTESIAN_POINT('Ctrl Pts',(-6.76712323346971,4.50361338683149,
59.2295936814247));
#176053=CARTESIAN_POINT('Ctrl Pts',(-6.89329428761988,4.30141621175714,
59.2389494840532));
#176054=CARTESIAN_POINT('Ctrl Pts',(-7.02007783349853,4.0982374795571,59.2483507040063));
#176055=CARTESIAN_POINT('Ctrl Pts',(-7.13779037612417,3.88958624743861,
59.2577519239594));
#176056=CARTESIAN_POINT('Ctrl Pts',(-7.24604173723519,3.67621635717289,
59.2671531439124));
#176057=CARTESIAN_POINT('Ctrl Pts',(-7.3544102584414,3.46261553737062,59.2765645387752));
#176058=CARTESIAN_POINT('Ctrl Pts',(-7.45329710928877,3.2442858823815,59.285975933638));
#176059=CARTESIAN_POINT('Ctrl Pts',(-7.542358903169,3.02200425848266,59.2953873285008));
#176060=CARTESIAN_POINT('Ctrl Pts',(-7.63131622607169,2.7999833746557,59.3047876836396));
#176061=CARTESIAN_POINT('Ctrl Pts',(-7.71047151882323,2.57401982332461,
59.3141880387784));
#176062=CARTESIAN_POINT('Ctrl Pts',(-7.77953055161956,2.34490766532882,
59.3235883939172));
#176063=CARTESIAN_POINT('Ctrl Pts',(-7.82371594491667,2.19831698196304,
59.3296029349862));
#176064=CARTESIAN_POINT('Ctrl Pts',(-7.86376919165637,2.05043775128498,
59.3356174760553));
#176065=CARTESIAN_POINT('Ctrl Pts',(-7.8996236098685,1.90148215476986,59.3416320171243));
#176066=CARTESIAN_POINT('Ctrl Pts',(-7.9457776897635,1.70973706880325,59.3493743156435));
#176067=CARTESIAN_POINT('Ctrl Pts',(-7.98499275830769,1.51611758234971,
59.3571166141628));
#176068=CARTESIAN_POINT('Ctrl Pts',(-8.01711805569086,1.32117585643077,
59.364858912682));
#176069=CARTESIAN_POINT('Ctrl Pts',(-8.04922334192284,1.12635556155427,
59.3725963884504));
#176070=CARTESIAN_POINT('Ctrl Pts',(-8.07424759310664,0.930215014276329,
59.3803338642187));
#176071=CARTESIAN_POINT('Ctrl Pts',(-8.0920906761317,0.733318519991388,
59.3880713399871));
#176072=CARTESIAN_POINT('Ctrl Pts',(-8.10992581576069,0.536509680224317,
59.3958053711806));
#176073=CARTESIAN_POINT('Ctrl Pts',(-8.12058612244261,0.338945914785465,
59.4035394023741));
#176074=CARTESIAN_POINT('Ctrl Pts',(-8.12402304696773,0.141198777746593,
59.4112734335676));
#176075=CARTESIAN_POINT('Ctrl Pts',(-8.12745953167473,-0.0565230538854145,
59.4190064750487));
#176076=CARTESIAN_POINT('Ctrl Pts',(-8.12367446159159,-0.254427857503845,
59.4267395165298));
#176077=CARTESIAN_POINT('Ctrl Pts',(-8.1126713474277,-0.451941557201383,
59.4344725580108));
#176078=CARTESIAN_POINT('Ctrl Pts',(-8.10166933246672,-0.64943552542729,
59.4422048269668));
#176079=CARTESIAN_POINT('Ctrl Pts',(-8.08345073299006,-0.846538114910816,
59.4499370959228));
#176080=CARTESIAN_POINT('Ctrl Pts',(-8.05807112147902,-1.04267797698327,
59.4576693648787));
#176081=CARTESIAN_POINT('Ctrl Pts',(-8.03268174758566,-1.23889328514048,
59.4654046080869));
#176082=CARTESIAN_POINT('Ctrl Pts',(-8.00012590370554,-1.4341447752558,
59.4731398512951));
#176083=CARTESIAN_POINT('Ctrl Pts',(-7.96051081565275,-1.62786827365595,
59.4808750945033));
#176084=CARTESIAN_POINT('Ctrl Pts',(-7.92735095169755,-1.79002479450765,
59.4873498904725));
#176085=CARTESIAN_POINT('Ctrl Pts',(-7.8892459262511,-1.95111075807356,
59.4938246864417));
#176086=CARTESIAN_POINT('Ctrl Pts',(-7.84628585923914,-2.1108021644872,
59.5002994824109));
#176087=CARTESIAN_POINT('Ctrl Pts',(-7.79045874031913,-2.31832304972874,
59.5087135569154));
#176088=CARTESIAN_POINT('Ctrl Pts',(-7.72640514464444,-2.52358870154097,
59.5171276314198));
#176089=CARTESIAN_POINT('Ctrl Pts',(-7.65433369538427,-2.7259609759138,
59.5255417059243));
#176090=CARTESIAN_POINT('Ctrl Pts',(-7.58224211855191,-2.9283897672931,
59.5339581302482));
#176091=CARTESIAN_POINT('Ctrl Pts',(-7.50212830660131,-3.12792331937895,
59.5423745545721));
#176092=CARTESIAN_POINT('Ctrl Pts',(-7.41424972646203,-3.32394171972941,
59.550790978896));
#176093=CARTESIAN_POINT('Ctrl Pts',(-7.32634935304548,-3.52000873128116,
59.5592094904346));
#176094=CARTESIAN_POINT('Ctrl Pts',(-7.23068047512863,-3.71255860991952,
59.5676280019733));
#176095=CARTESIAN_POINT('Ctrl Pts',(-7.1275478400223,-3.90099337998586,
59.5760465135119));
#176096=CARTESIAN_POINT('Ctrl Pts',(-7.02437559210323,-4.08950052705732,
59.5844682585656));
#176097=CARTESIAN_POINT('Ctrl Pts',(-6.91373398380659,-4.27388917474599,
59.5928900036192));
#176098=CARTESIAN_POINT('Ctrl Pts',(-6.79597338141109,-4.45358657282553,
59.6013117486728));
#176099=CARTESIAN_POINT('Ctrl Pts',(-6.67820001408728,-4.63330344961323,
59.6097344066207));
#176100=CARTESIAN_POINT('Ctrl Pts',(-6.55330625912476,-4.80832784237316,
59.6181570645685));
#176101=CARTESIAN_POINT('Ctrl Pts',(-6.42168575059229,-4.97811607770851,
59.6265797225164));
#176102=CARTESIAN_POINT('Ctrl Pts',(-6.29004021162703,-5.14793660187985,
59.6350039822113));
#176103=CARTESIAN_POINT('Ctrl Pts',(-6.15166552523974,-5.31251877076992,
59.6434282419063));
#176104=CARTESIAN_POINT('Ctrl Pts',(-6.00699635693191,-5.47135105164225,
59.6518525016013));
#176105=CARTESIAN_POINT('Ctrl Pts',(-5.96627107712832,-5.5160633366165,
59.6542239836332));
#176106=CARTESIAN_POINT('Ctrl Pts',(-5.9250472257413,-5.56032017481485,
59.6565954656652));
#176107=CARTESIAN_POINT('Ctrl Pts',(-5.88333505391349,-5.60411065253825,
59.6589669476971));
#176108=CARTESIAN_POINT('Ctrl Pts',(-5.73515897820208,-5.75966959033143,
59.6673912729172));
#176109=CARTESIAN_POINT('Ctrl Pts',(-5.58080255360596,-5.90935670906184,
59.6758155981372));
#176110=CARTESIAN_POINT('Ctrl Pts',(-5.42074539525802,-6.05270244785657,
59.6842399233572));
#176111=CARTESIAN_POINT('Ctrl Pts',(-5.26071589674424,-6.19602341475479,
59.6926627927509));
#176112=CARTESIAN_POINT('Ctrl Pts',(-5.09498782864397,-6.33300501451064,
59.7010856621445));
#176113=CARTESIAN_POINT('Ctrl Pts',(-4.92407575896629,-6.46321634191991,
59.7095085315381));
#176114=CARTESIAN_POINT('Ctrl Pts',(-4.75319861545562,-6.59340106042684,
59.7179296797043));
#176115=CARTESIAN_POINT('Ctrl Pts',(-4.57713979565663,-6.71681810952512,
59.7263508278705));
#176116=CARTESIAN_POINT('Ctrl Pts',(-4.39644573569564,-6.83307781717606,
59.7347719760367));
#176117=CARTESIAN_POINT('Ctrl Pts',(-4.215802372392,-6.94930490627517,59.7431907615128));
#176118=CARTESIAN_POINT('Ctrl Pts',(-4.03052658815115,-7.05837852195163,
59.751609546989));
#176119=CARTESIAN_POINT('Ctrl Pts',(-3.84119333691809,-7.15995260535404,
59.7600283324651));
#176120=CARTESIAN_POINT('Ctrl Pts',(-3.65191297466052,-7.26149831471663,
59.7684447662099));
#176121=CARTESIAN_POINT('Ctrl Pts',(-3.45857764080911,-7.35554854991029,
59.7768611999547));
#176122=CARTESIAN_POINT('Ctrl Pts',(-3.26178741716566,-7.44180290035417,
59.7852776336994));
#176123=CARTESIAN_POINT('Ctrl Pts',(-3.06506861693375,-7.5280259454829,
59.793691012768));
#176124=CARTESIAN_POINT('Ctrl Pts',(-2.86489767249388,-7.60645865035784,
59.8021043918366));
#176125=CARTESIAN_POINT('Ctrl Pts',(-2.66189610388929,-7.67684809636084,
59.8105177709052));
#176126=CARTESIAN_POINT('Ctrl Pts',(-2.6046583205384,-7.69669491768445,
59.8128899849314));
#176127=CARTESIAN_POINT('Ctrl Pts',(-2.54719562530409,-7.71590259370242,
59.8152621989575));
#176128=CARTESIAN_POINT('Ctrl Pts',(-2.48952222673452,-7.73446615126699,
59.8176344129837));
#176129=CARTESIAN_POINT('Ctrl Pts',(-2.30146398348853,-7.7949971778854,
59.8253695978944));
#176130=CARTESIAN_POINT('Ctrl Pts',(-2.11108068195695,-7.84870267244674,
59.8331047828051));
#176131=CARTESIAN_POINT('Ctrl Pts',(-1.91891801273629,-7.89540633678193,
59.8408399677158));
#176132=CARTESIAN_POINT('Ctrl Pts',(-1.72681476496072,-7.9420955591902,
59.8485727607162));
#176133=CARTESIAN_POINT('Ctrl Pts',(-1.5329335881136,-7.98178717972852,
59.8563055537166));
#176134=CARTESIAN_POINT('Ctrl Pts',(-1.3378342829939,-8.01435505787872,
59.864038346717));
#176135=CARTESIAN_POINT('Ctrl Pts',(-1.14276064390407,-8.04691865160498,
59.8717701224401));
#176136=CARTESIAN_POINT('Ctrl Pts',(-0.946469544243333,-8.07236031221967,
59.8795018981632));
#176137=CARTESIAN_POINT('Ctrl Pts',(-0.749530034423728,-8.09060518688168,
59.8872336738863));
#176138=CARTESIAN_POINT('Ctrl Pts',(-0.552520054268652,-8.10885659005816,
59.8949682162499));
#176139=CARTESIAN_POINT('Ctrl Pts',(-0.35486155216785,-8.11990602540112,
59.9027027586136));
#176140=CARTESIAN_POINT('Ctrl Pts',(-0.157128416396801,-8.12373056072521,
59.9104373009772));
#176141=CARTESIAN_POINT('Ctrl Pts',(0.0406381142961575,-8.12755574197067,
59.9181731496188));
#176142=CARTESIAN_POINT('Ctrl Pts',(0.238478950284186,-8.12415359266938,
59.9259089982604));
#176143=CARTESIAN_POINT('Ctrl Pts',(0.435820985675838,-8.11355332951874,
59.9336448469019));
#176144=CARTESIAN_POINT('Ctrl Pts',(0.633324495256172,-8.10294439275282,
59.9413870253652));
#176145=CARTESIAN_POINT('Ctrl Pts',(0.830328036174533,-8.08512560110551,
59.9491292038284));
#176146=CARTESIAN_POINT('Ctrl Pts',(1.02626346573561,-8.06017809117121,
59.9568713822916));
#176147=CARTESIAN_POINT('Ctrl Pts',(1.19017609894768,-8.03930788890827,
59.9633482142844));
#176148=CARTESIAN_POINT('Ctrl Pts',(1.35334123727867,-8.01344966063173,
59.9698250462772));
#176149=CARTESIAN_POINT('Ctrl Pts',(1.51543234453711,-7.98267827058255,
59.97630187827));
#176150=CARTESIAN_POINT('Ctrl Pts',(1.75063017623512,-7.93802829353992,
59.9856999067414));
#176151=CARTESIAN_POINT('Ctrl Pts',(1.98370033438577,-7.88300859344652,
59.9950979352128));
#176152=CARTESIAN_POINT('Ctrl Pts',(2.21382499870229,-7.81784282507782,
60.0044959636842));
#176153=CARTESIAN_POINT('Ctrl Pts',(2.44427711115741,-7.75258433127435,
60.0139073647636));
#176154=CARTESIAN_POINT('Ctrl Pts',(2.67177531021364,-7.67715090081817,
60.023318765843));
#176155=CARTESIAN_POINT('Ctrl Pts',(2.89551562634762,-7.59181643745927,
60.0327301669224));
#176156=CARTESIAN_POINT('Ctrl Pts',(3.1189190636738,-7.50661045953731,60.0421273975491));
#176157=CARTESIAN_POINT('Ctrl Pts',(3.33857589388081,-7.41153326016449,
60.0515246281758));
#176158=CARTESIAN_POINT('Ctrl Pts',(3.55370351085696,-7.30690624816159,
60.0609218588024));
#176159=CARTESIAN_POINT('Ctrl Pts',(3.76828849573501,-7.20254314451151,
60.0702953861081));
#176160=CARTESIAN_POINT('Ctrl Pts',(3.97836704400503,-7.08867834160937,
60.0796689134137));
#176161=CARTESIAN_POINT('Ctrl Pts',(4.18318067121494,-6.96567922276598,
60.0890424407194));
#176162=CARTESIAN_POINT('Ctrl Pts',(4.38666425075851,-6.84347885297659,
60.0983550968892));
#176163=CARTESIAN_POINT('Ctrl Pts',(4.58495101820729,-6.71226242211352,
60.107667753059));
#176164=CARTESIAN_POINT('Ctrl Pts',(4.77731583887187,-6.5724379752238,60.1169804092288));
#176165=CARTESIAN_POINT('Ctrl Pts',(4.90117731880401,-6.4824066334087,60.1229767206713));
#176166=CARTESIAN_POINT('Ctrl Pts',(5.0225839822251,-6.3888074375956,60.1289730321139));
#176167=CARTESIAN_POINT('Ctrl Pts',(5.1413465689545,-6.29175993028976,60.1349693435564));
#176168=CARTESIAN_POINT('Ctrl Pts',(5.29123115610279,-6.16928090750249,
60.1425370017704));
#176169=CARTESIAN_POINT('Ctrl Pts',(5.43684283592682,-6.04135563105719,
60.1501046599844));
#176170=CARTESIAN_POINT('Ctrl Pts',(5.57775061728474,-5.9083318808171,60.1576723181984));
#176171=CARTESIAN_POINT('Ctrl Pts',(5.71861938381086,-5.77534496246231,
60.1652378810639));
#176172=CARTESIAN_POINT('Ctrl Pts',(5.85478657630854,-5.63726263133551,
60.1728034439293));
#176173=CARTESIAN_POINT('Ctrl Pts',(5.98585552004352,-5.4944718814154,60.1803690067948));
#176174=CARTESIAN_POINT('Ctrl Pts',(6.1169129809003,-5.35169364131449,60.1879339068455));
#176175=CARTESIAN_POINT('Ctrl Pts',(6.24287283401844,-5.20420807489195,
60.1954988068961));
#176176=CARTESIAN_POINT('Ctrl Pts',(6.36337646291,-5.0524377832669,60.2030637069468));
#176177=CARTESIAN_POINT('Ctrl Pts',(6.48393923423736,-4.90059300372137,
60.2106323198036));
#176178=CARTESIAN_POINT('Ctrl Pts',(6.59904019996351,-4.74445958410859,
60.2182009326604));
#176179=CARTESIAN_POINT('Ctrl Pts',(6.70836179251535,-4.58449229721463,
60.2257695455173));
#176180=CARTESIAN_POINT('Ctrl Pts',(6.81770769626733,-4.42448943640853,
60.2333398415005));
#176181=CARTESIAN_POINT('Ctrl Pts',(6.92127146867148,-4.26065131995747,
60.2409101374837));
#176182=CARTESIAN_POINT('Ctrl Pts',(7.0187800049933,-4.09346000395829,60.248480433467));
#176183=CARTESIAN_POINT('Ctrl Pts',(7.1163873452605,-3.92609927549251,60.2560584003182));
#176184=CARTESIAN_POINT('Ctrl Pts',(7.20792701552237,-3.75537888246008,
60.2636363671695));
#176185=CARTESIAN_POINT('Ctrl Pts',(7.29317243242582,-3.58180449402309,
60.2712143340207));
#176186=CARTESIAN_POINT('Ctrl Pts',(7.37725009475724,-3.410607855535,60.2786884922948));
#176187=CARTESIAN_POINT('Ctrl Pts',(7.45520477439366,-3.23663525093396,
60.2861626505689));
#176188=CARTESIAN_POINT('Ctrl Pts',(7.52686604962493,-3.06038805276448,
60.293636808843));
#176189=CARTESIAN_POINT('Ctrl Pts',(7.61514203613323,-2.84327783197196,
60.3028438553662));
#176190=CARTESIAN_POINT('Ctrl Pts',(7.69401223489476,-2.62236632347889,
60.3120509018894));
#176191=CARTESIAN_POINT('Ctrl Pts',(7.76320154708332,-2.39841391379036,
60.3212579484126));
#176192=CARTESIAN_POINT('Ctrl Pts',(7.83225976266042,-2.17488583845505,
60.3304475498628));
#176193=CARTESIAN_POINT('Ctrl Pts',(7.89167371237667,-1.94832846441916,
60.339637151313));
#176194=CARTESIAN_POINT('Ctrl Pts',(7.94121874032326,-1.71951518773132,
60.3488267527632));
#176195=CARTESIAN_POINT('Ctrl Pts',(7.99065588289186,-1.49120015693954,
60.357996343656));
#176196=CARTESIAN_POINT('Ctrl Pts',(8.0302669900568,-1.26063912489709,60.3671659345488));
#176197=CARTESIAN_POINT('Ctrl Pts',(8.05987815615349,-1.02861638644337,
60.3763355254416));
#176198=CARTESIAN_POINT('Ctrl Pts',(8.08934617123157,-0.797715329291968,
60.3854607872367));
#176199=CARTESIAN_POINT('Ctrl Pts',(8.10891065581527,-0.565366758546668,
60.3945860490317));
#176200=CARTESIAN_POINT('Ctrl Pts',(8.11844970807552,-0.332358089939839,
60.4037113108267));
#176201=CARTESIAN_POINT('Ctrl Pts',(8.12297647043886,-0.221783701352419,
60.408041708703));
#176202=CARTESIAN_POINT('Ctrl Pts',(8.12524624889688,-0.11106086174646,
60.4123721065793));
#176203=CARTESIAN_POINT('Ctrl Pts',(8.12524999535401,-0.000274771867375941,
60.4167025044555));
#176204=CARTESIAN_POINT('',(8.12839272166354,0.00745291351919315,56.4167025567876));
#176205=CARTESIAN_POINT('Ctrl Pts',(8.12839272166354,0.00745291351919315,
56.4167025567876));
#176206=CARTESIAN_POINT('Ctrl Pts',(8.13117600423807,0.594204244290565,
56.4396742518479));
#176207=CARTESIAN_POINT('Ctrl Pts',(7.79071024475799,3.87609837964483,56.5684242570992));
#176208=CARTESIAN_POINT('Ctrl Pts',(4.37969769441631,7.81986399754792,56.7500634174461));
#176209=CARTESIAN_POINT('Ctrl Pts',(-1.20468243196269,8.37056697778818,
56.9616200378278));
#176210=CARTESIAN_POINT('Ctrl Pts',(-5.04719085376719,6.80318123386091,
57.1202875031144));
#176211=CARTESIAN_POINT('Ctrl Pts',(-7.69384797429684,3.54846383209959,
57.2789549684008));
#176212=CARTESIAN_POINT('Ctrl Pts',(-8.44679792397339,-0.555938847163704,
57.4376224336872));
#176213=CARTESIAN_POINT('Ctrl Pts',(-7.16239838939218,-4.52625027291816,
57.5962898989736));
#176214=CARTESIAN_POINT('Ctrl Pts',(-4.11199154401565,-7.40600674808037,
57.7549573642601));
#176215=CARTESIAN_POINT('Ctrl Pts',(-0.0971997372447445,-8.45625233235956,
57.9136248295464));
#176216=CARTESIAN_POINT('Ctrl Pts',(5.36683002199323,-7.17838145731046,
58.1251814499284));
#176217=CARTESIAN_POINT('Ctrl Pts',(8.01157082499094,-3.15609430642058,
58.2928740256754));
#176218=CARTESIAN_POINT('Ctrl Pts',(8.13406518936454,-0.235442656146994,
58.407677446327));
#176219=CARTESIAN_POINT('Ctrl Pts',(8.13353216142055,-0.00564646944313244,
58.4167025567876));
#176220=CARTESIAN_POINT('',(8.12524955238746,-0.00269701298808146,54.4167028280926));
#176221=CARTESIAN_POINT('Ctrl Pts',(8.12524955469297,-0.00269006721165242,
54.4167030993976));
#176222=CARTESIAN_POINT('Ctrl Pts',(8.12532117721707,0.213643145395203,
54.4251531671901));
#176223=CARTESIAN_POINT('Ctrl Pts',(8.1167486902665,0.42985406284176,54.4336032349825));
#176224=CARTESIAN_POINT('Ctrl Pts',(8.09958770519598,0.645264727331433,
54.442053302775));
#176225=CARTESIAN_POINT('Ctrl Pts',(8.0824089990312,0.860897833171388,54.450512096433));
#176226=CARTESIAN_POINT('Ctrl Pts',(8.05662409774357,1.07572878194088,54.458970890091));
#176227=CARTESIAN_POINT('Ctrl Pts',(8.02234035055661,1.28908605699205,54.467429683749));
#176228=CARTESIAN_POINT('Ctrl Pts',(7.98802355053444,1.50264902901132,54.475896632499));
#176229=CARTESIAN_POINT('Ctrl Pts',(7.94519157648052,1.71473523844329,54.484363581249));
#176230=CARTESIAN_POINT('Ctrl Pts',(7.8940028471983,1.92468350928801,54.492830529999));
#176231=CARTESIAN_POINT('Ctrl Pts',(7.84274283670313,2.13492413682158,54.5013092691253));
#176232=CARTESIAN_POINT('Ctrl Pts',(7.78310286112371,2.34302062537099,54.5097880082515));
#176233=CARTESIAN_POINT('Ctrl Pts',(7.71529177581499,2.54832501391434,54.5182667473777));
#176234=CARTESIAN_POINT('Ctrl Pts',(7.64743704724449,2.75376153650533,54.5267509434264));
#176235=CARTESIAN_POINT('Ctrl Pts',(7.57140079006321,2.95640213063907,54.535235139475));
#176236=CARTESIAN_POINT('Ctrl Pts',(7.48744068584734,3.15561714065853,54.5437193355236));
#176237=CARTESIAN_POINT('Ctrl Pts',(7.40340079297167,3.35502146795923,54.5522115942425));
#176238=CARTESIAN_POINT('Ctrl Pts',(7.31142210103964,3.5509934704558,54.5607038529614));
#176239=CARTESIAN_POINT('Ctrl Pts',(7.21180989403962,3.74292474072513,54.5691961116802));
#176240=CARTESIAN_POINT('Ctrl Pts',(7.16328015026766,3.8364311055424,54.5733334272973));
#176241=CARTESIAN_POINT('Ctrl Pts',(7.11293928072038,3.92897876777759,54.5774707429144));
#176242=CARTESIAN_POINT('Ctrl Pts',(7.0608264780951,4.02049959690723,54.5816080585314));
#176243=CARTESIAN_POINT('Ctrl Pts',(6.96537197072242,4.18813739834589,54.5891863388038));
#176244=CARTESIAN_POINT('Ctrl Pts',(6.86380968578961,4.35260891314493,54.5967646190762));
#176245=CARTESIAN_POINT('Ctrl Pts',(6.75638455891372,4.51341946361872,54.6043428993485));
#176246=CARTESIAN_POINT('Ctrl Pts',(6.64903936949063,4.6741103513454,54.6119155404521));
#176247=CARTESIAN_POINT('Ctrl Pts',(6.5358402198108,4.83114539062414,54.6194881815556));
#176248=CARTESIAN_POINT('Ctrl Pts',(6.41707800793653,4.98405431376478,54.6270608226592));
#176249=CARTESIAN_POINT('Ctrl Pts',(6.29838161732412,5.13687849060345,54.6346292667982));
#176250=CARTESIAN_POINT('Ctrl Pts',(6.17412852431732,5.28558081247401,54.6421977109373));
#176251=CARTESIAN_POINT('Ctrl Pts',(6.04465295973988,5.42971989690149,54.6497661550763));
#176252=CARTESIAN_POINT('Ctrl Pts',(5.91520867859788,5.57382415494487,54.6573327705542));
#176253=CARTESIAN_POINT('Ctrl Pts',(5.78054467676714,5.71336709163324,54.6648993860321));
#176254=CARTESIAN_POINT('Ctrl Pts',(5.64103558225979,5.84794024611905,54.67246600151));
#176255=CARTESIAN_POINT('Ctrl Pts',(5.50155123616915,5.98248952780635,54.6800312746972));
#176256=CARTESIAN_POINT('Ctrl Pts',(5.35722377501494,6.11207052907319,54.6875965478845));
#176257=CARTESIAN_POINT('Ctrl Pts',(5.20846460849133,6.236311729267,54.6951618210717));
#176258=CARTESIAN_POINT('Ctrl Pts',(5.05965371435143,6.36059613151204,54.7027297249106));
#176259=CARTESIAN_POINT('Ctrl Pts',(4.90640831666732,6.47953678467443,54.7102976287495));
#176260=CARTESIAN_POINT('Ctrl Pts',(4.74917319109061,6.59280225424107,54.7178655325884));
#176261=CARTESIAN_POINT('Ctrl Pts',(4.59397223275593,6.70460239659791,54.7253355296649));
#176262=CARTESIAN_POINT('Ctrl Pts',(4.43488446612516,6.81087314914783,54.7328055267414));
#176263=CARTESIAN_POINT('Ctrl Pts',(4.27236483638971,6.91133751652173,54.7402755238179));
#176264=CARTESIAN_POINT('Ctrl Pts',(4.06990534011865,7.036491414822,54.749581303358));
#176265=CARTESIAN_POINT('Ctrl Pts',(3.86222049824272,7.15257477844018,54.7588870828981));
#176266=CARTESIAN_POINT('Ctrl Pts',(3.65007256103867,7.25924637008916,54.7681928624382));
#176267=CARTESIAN_POINT('Ctrl Pts',(3.43678578333663,7.3664905901132,54.7775485967351));
#176268=CARTESIAN_POINT('Ctrl Pts',(3.21898792955849,7.46422174700156,54.786904331032));
#176269=CARTESIAN_POINT('Ctrl Pts',(2.99746666849595,7.55214414148431,54.7962600653289));
#176270=CARTESIAN_POINT('Ctrl Pts',(2.77487016322118,7.6404933033362,54.8056612115158));
#176271=CARTESIAN_POINT('Ctrl Pts',(2.54851406480698,7.71893825665806,54.8150623577028));
#176272=CARTESIAN_POINT('Ctrl Pts',(2.31920988599594,7.7872301280493,54.8244635038897));
#176273=CARTESIAN_POINT('Ctrl Pts',(2.08965755173713,7.85559590563803,54.8338748240981));
#176274=CARTESIAN_POINT('Ctrl Pts',(1.85715079420815,7.91378662327403,54.8432861443065));
#176275=CARTESIAN_POINT('Ctrl Pts',(1.62251539912165,7.96160356599807,54.852697464515));
#176276=CARTESIAN_POINT('Ctrl Pts',(1.38815517534784,8.00936443086184,54.8620977474912));
#176277=CARTESIAN_POINT('Ctrl Pts',(1.15167134041322,8.04677583537968,54.8714980304675));
#176278=CARTESIAN_POINT('Ctrl Pts',(0.913897794378005,8.07369050583009,
54.8808983134437));
#176279=CARTESIAN_POINT('Ctrl Pts',(0.761755334774513,8.09091220365991,
54.8869132053306));
#176280=CARTESIAN_POINT('Ctrl Pts',(0.609085056009594,8.103837301339,54.8929280972176));
#176281=CARTESIAN_POINT('Ctrl Pts',(0.456107690708852,8.11243818694332,
54.8989429891045));
#176282=CARTESIAN_POINT('Ctrl Pts',(0.259196678160573,8.12350916525328,
54.9066853008478));
#176283=CARTESIAN_POINT('Ctrl Pts',(0.061684181500173,8.12741761380081,
54.914427612591));
#176284=CARTESIAN_POINT('Ctrl Pts',(-0.135859564528569,8.12411408962393,
54.9221699243343));
#176285=CARTESIAN_POINT('Ctrl Pts',(-0.333280259637731,8.12081262322765,
54.9299074133555));
#176286=CARTESIAN_POINT('Ctrl Pts',(-0.530731813611958,8.11030813480075,
54.9376449023768));
#176287=CARTESIAN_POINT('Ctrl Pts',(-0.727641109789703,8.0926031644857,
54.945382391398));
#176288=CARTESIAN_POINT('Ctrl Pts',(-0.92446274644691,8.07490607601899,
54.9531164358659));
#176289=CARTESIAN_POINT('Ctrl Pts',(-1.12074225497299,8.05001492133607,
54.9608504803337));
#176290=CARTESIAN_POINT('Ctrl Pts',(-1.31590862474052,8.01798428869959,
54.9685845248016));
#176291=CARTESIAN_POINT('Ctrl Pts',(-1.51105001943296,7.98595775496323,
54.9763175795583));
#176292=CARTESIAN_POINT('Ctrl Pts',(-1.70507820945395,7.94679361266297,
54.9840506343149));
#176293=CARTESIAN_POINT('Ctrl Pts',(-1.89742902587127,7.90059812003377,
54.9917836890716));
#176294=CARTESIAN_POINT('Ctrl Pts',(-2.08976062681534,7.85440724224464,
54.9995159713111));
#176295=CARTESIAN_POINT('Ctrl Pts',(-2.28041484514974,7.80118649929966,
55.0072482535506));
#176296=CARTESIAN_POINT('Ctrl Pts',(-2.4688395181715,7.74109288124194,55.0149805357901));
#176297=CARTESIAN_POINT('Ctrl Pts',(-2.65733666855023,7.68097614823576,
55.0227157922441));
#176298=CARTESIAN_POINT('Ctrl Pts',(-2.84360222324174,7.61398136575718,
55.030451048698));
#176299=CARTESIAN_POINT('Ctrl Pts',(-3.02710032847934,7.54031505733151,
55.0381863051519));
#176300=CARTESIAN_POINT('Ctrl Pts',(-3.18069551964057,7.4786534357571,55.0446610215648));
#176301=CARTESIAN_POINT('Ctrl Pts',(-3.3323519420771,7.41231841846424,55.0511357379778));
#176302=CARTESIAN_POINT('Ctrl Pts',(-3.48176698343969,7.34145668348791,
55.0576104543907));
#176303=CARTESIAN_POINT('Ctrl Pts',(-3.67593586605389,7.24936994459615,
55.0660245232801));
#176304=CARTESIAN_POINT('Ctrl Pts',(-3.86641280821176,7.14959357787699,
55.0744385921696));
#176305=CARTESIAN_POINT('Ctrl Pts',(-4.05260734156805,7.04244711002992,
55.082852661059));
#176306=CARTESIAN_POINT('Ctrl Pts',(-4.23885387189586,6.93527072029557,
55.0912690796742));
#176307=CARTESIAN_POINT('Ctrl Pts',(-4.42081537713161,6.82072025230835,
55.0996854982895));
#176308=CARTESIAN_POINT('Ctrl Pts',(-4.5979280725388,6.69916002214155,55.1081019169047));
#176309=CARTESIAN_POINT('Ctrl Pts',(-4.77508468938182,6.5775696467622,55.1165204226724));
#176310=CARTESIAN_POINT('Ctrl Pts',(-4.94738987823115,6.44896618817717,
55.12493892844));
#176311=CARTESIAN_POINT('Ctrl Pts',(-5.11430990332206,6.31375655020701,
55.1333574342077));
#176312=CARTESIAN_POINT('Ctrl Pts',(-5.28129404125881,6.17849497913493,
55.1417791734661));
#176313=CARTESIAN_POINT('Ctrl Pts',(-5.44288867607268,6.03662232332008,
55.1502009127246));
#176314=CARTESIAN_POINT('Ctrl Pts',(-5.59859305894425,5.88858585085088,
55.158622651983));
#176315=CARTESIAN_POINT('Ctrl Pts',(-5.75431431990311,5.7405333314827,55.1670453041435));
#176316=CARTESIAN_POINT('Ctrl Pts',(-5.90414386489438,5.58631584549195,
55.1754679563039));
#176317=CARTESIAN_POINT('Ctrl Pts',(-6.04761730014841,5.42641802236481,
55.1838906084644));
#176318=CARTESIAN_POINT('Ctrl Pts',(-6.19111802100276,5.2664897900676,55.1923148624345));
#176319=CARTESIAN_POINT('Ctrl Pts',(-6.32826004101571,5.10087925898032,
55.2007391164045));
#176320=CARTESIAN_POINT('Ctrl Pts',(-6.45861793529407,4.9301056711188,55.2091633703746));
#176321=CARTESIAN_POINT('Ctrl Pts',(-6.4953150588272,4.88203110314082,55.2115348868088));
#176322=CARTESIAN_POINT('Ctrl Pts',(-6.5314747998295,4.83354757078024,55.2139064032431));
#176323=CARTESIAN_POINT('Ctrl Pts',(-6.56708825636936,4.78466711439318,
55.2162779196773));
#176324=CARTESIAN_POINT('Ctrl Pts',(-6.69359774332266,4.6110293364188,55.2247022445406));
#176325=CARTESIAN_POINT('Ctrl Pts',(-6.8132235736821,4.43236261921473,55.2331265694039));
#176326=CARTESIAN_POINT('Ctrl Pts',(-6.92558966475159,4.24922291224947,
55.2415508942672));
#176327=CARTESIAN_POINT('Ctrl Pts',(-7.0379363373458,4.06611485445737,55.2499737632861));
#176328=CARTESIAN_POINT('Ctrl Pts',(-7.14302563848885,3.87853557566106,
55.258396632305));
#176329=CARTESIAN_POINT('Ctrl Pts',(-7.2405257755269,3.68706849087871,55.2668195013239));
#176330=CARTESIAN_POINT('Ctrl Pts',(-7.33800598806478,3.49564053307689,
55.2752406490995));
#176331=CARTESIAN_POINT('Ctrl Pts',(-7.42790001379247,3.30032659087973,
55.2836617968751));
#176332=CARTESIAN_POINT('Ctrl Pts',(-7.50992233352312,3.10173404839142,
55.2920829446507));
#176333=CARTESIAN_POINT('Ctrl Pts',(-7.59192164037156,2.90319722472215,
55.3005017297172));
#176334=CARTESIAN_POINT('Ctrl Pts',(-7.66605355161384,2.70138388175668,
55.3089205147837));
#176335=CARTESIAN_POINT('Ctrl Pts',(-7.73208056312027,2.4969216503362,55.3173392998502));
#176336=CARTESIAN_POINT('Ctrl Pts',(-7.79808913034733,2.29251653430581,
55.3257557331758));
#176337=CARTESIAN_POINT('Ctrl Pts',(-7.85599723723042,2.08546425817583,
55.3341721665014));
#176338=CARTESIAN_POINT('Ctrl Pts',(-7.90561678982064,1.8764089999267,55.342588599827));
#176339=CARTESIAN_POINT('Ctrl Pts',(-7.95521833333483,1.66742961684867,
55.3510019784659));
#176340=CARTESIAN_POINT('Ctrl Pts',(-7.99653726911623,1.45644895996967,
55.3594153571048));
#176341=CARTESIAN_POINT('Ctrl Pts',(-8.02943606656307,1.24412379427298,
55.3678287357437));
#176342=CARTESIAN_POINT('Ctrl Pts',(-8.03871213393285,1.18425709110593,
55.3702009521503));
#176343=CARTESIAN_POINT('Ctrl Pts',(-8.04731910989908,1.12428356740809,
55.3725731685569));
#176344=CARTESIAN_POINT('Ctrl Pts',(-8.05525464611378,1.06421809266818,
55.3749453849636));
#176345=CARTESIAN_POINT('Ctrl Pts',(-8.0811303839952,0.868360063917399,
55.3826805711281));
#176346=CARTESIAN_POINT('Ctrl Pts',(-8.0998745576842,0.67143685392728,55.3904157572926));
#176347=CARTESIAN_POINT('Ctrl Pts',(-8.11141143931543,0.47401690333016,
55.3981509434571));
#176348=CARTESIAN_POINT('Ctrl Pts',(-8.12294475347403,0.276657999582231,
55.4058837377218));
#176349=CARTESIAN_POINT('Ctrl Pts',(-8.1272751931843,0.0788030133886556,
55.4136165319865));
#176350=CARTESIAN_POINT('Ctrl Pts',(-8.12437890424811,-0.118974714574983,
55.4213493262512));
#176351=CARTESIAN_POINT('Ctrl Pts',(-8.12148299632561,-0.316726424409161,
55.4290811032485));
#176352=CARTESIAN_POINT('Ctrl Pts',(-8.11136225933815,-0.514400543104047,
55.4368128802457));
#176353=CARTESIAN_POINT('Ctrl Pts',(-8.09404495409557,-0.711423814318956,
55.444544657243));
#176354=CARTESIAN_POINT('Ctrl Pts',(-8.07672145222333,-0.908517586124225,
55.4522792008923));
#176355=CARTESIAN_POINT('Ctrl Pts',(-8.05219626393886,-1.10495969247385,
55.4600137445417));
#176356=CARTESIAN_POINT('Ctrl Pts',(-8.02054959776511,-1.30018141514555,
55.467748288191));
#176357=CARTESIAN_POINT('Ctrl Pts',(-7.9888975867931,-1.49543610876966,
55.4754841381257));
#176358=CARTESIAN_POINT('Ctrl Pts',(-7.95012176548351,-1.68946966039589,
55.4832199880604));
#176359=CARTESIAN_POINT('Ctrl Pts',(-7.90435350815507,-1.88172346018661,
55.490955837995));
#176360=CARTESIAN_POINT('Ctrl Pts',(-7.85854780113553,-2.07413457086995,
55.4986980177575));
#176361=CARTESIAN_POINT('Ctrl Pts',(-7.8057383160175,-2.26476267798658,
55.5064401975201));
#176362=CARTESIAN_POINT('Ctrl Pts',(-7.74610661894578,-2.45306335230551,
55.5141823772826));
#176363=CARTESIAN_POINT('Ctrl Pts',(-7.69622092294884,-2.61058880699442,
55.5206592016051));
#176364=CARTESIAN_POINT('Ctrl Pts',(-7.6415617019312,-2.76648561514557,
55.5271360259276));
#176365=CARTESIAN_POINT('Ctrl Pts',(-7.58226108443207,-2.92044592656789,
55.5336128502501));
#176366=CARTESIAN_POINT('Ctrl Pts',(-7.49621448058495,-3.14384599361324,
55.5430108761084));
#176367=CARTESIAN_POINT('Ctrl Pts',(-7.40034680045617,-3.36329580948709,
55.5524089019666));
#176368=CARTESIAN_POINT('Ctrl Pts',(-7.29502453550529,-3.5780308255905,
55.5618069278249));
#176369=CARTESIAN_POINT('Ctrl Pts',(-7.18955240745439,-3.79307138824867,
55.5712183261385));
#176370=CARTESIAN_POINT('Ctrl Pts',(-7.07459880091788,-4.00338369818199,
55.5806297244521));
#176371=CARTESIAN_POINT('Ctrl Pts',(-6.95057716370891,-4.20822583208509,
55.5900411227658));
#176372=CARTESIAN_POINT('Ctrl Pts',(-6.82674226255766,-4.41275954067304,
55.599438350589));
#176373=CARTESIAN_POINT('Ctrl Pts',(-6.69386664112265,-4.6118395053296,
55.6088355784123));
#176374=CARTESIAN_POINT('Ctrl Pts',(-6.55240665869331,-4.80475332786311,
55.6182328062355));
#176375=CARTESIAN_POINT('Ctrl Pts',(-6.41130349015302,-4.99718055107653,
55.6276063308082));
#176376=CARTESIAN_POINT('Ctrl Pts',(-6.26165921735419,-5.18347265648011,
55.6369798553809));
#176377=CARTESIAN_POINT('Ctrl Pts',(-6.10397111129621,-5.36294921055209,
55.6463533799536));
#176378=CARTESIAN_POINT('Ctrl Pts',(-5.94730701916723,-5.54126025825905,
55.6556660336086));
#176379=CARTESIAN_POINT('Ctrl Pts',(-5.78270323996381,-5.71284393894928,
55.6649786872636));
#176380=CARTESIAN_POINT('Ctrl Pts',(-5.61069107700621,-5.87705991129093,
55.6742913409186));
#176381=CARTESIAN_POINT('Ctrl Pts',(-5.49993415966061,-5.98279693920071,
55.6802876657912));
#176382=CARTESIAN_POINT('Ctrl Pts',(-5.38610664811779,-6.0854799000411,
55.6862839906638));
#176383=CARTESIAN_POINT('Ctrl Pts',(-5.26936004560861,-6.18494399911944,
55.6922803155364));
#176384=CARTESIAN_POINT('Ctrl Pts',(-5.12202005641906,-6.31047261381124,
55.6998479742341));
#176385=CARTESIAN_POINT('Ctrl Pts',(-4.97008702844688,-6.43082209503759,
55.7074156329318));
#176386=CARTESIAN_POINT('Ctrl Pts',(-4.81398030021903,-6.54563069777108,
55.7149832916295));
#176387=CARTESIAN_POINT('Ctrl Pts',(-4.65791679505825,-6.66040751212495,
55.7225488549825));
#176388=CARTESIAN_POINT('Ctrl Pts',(-4.49768218492731,-6.76964628300164,
55.7301144183354));
#176389=CARTESIAN_POINT('Ctrl Pts',(-4.33372824331128,-6.87302604939237,
55.7376799816883));
#176390=CARTESIAN_POINT('Ctrl Pts',(-4.16978866553457,-6.97639675878613,
55.7452448822299));
#176391=CARTESIAN_POINT('Ctrl Pts',(-4.00213071628905,-7.0739092899868,
55.7528097827714));
#176392=CARTESIAN_POINT('Ctrl Pts',(-3.83123438527392,-7.16528650143138,
55.760374683313));
#176393=CARTESIAN_POINT('Ctrl Pts',(-3.66025417929713,-7.25670856029932,
55.7679432966654));
#176394=CARTESIAN_POINT('Ctrl Pts',(-3.48603273945837,-7.34198910719033,
55.7755119100177));
#176395=CARTESIAN_POINT('Ctrl Pts',(-3.30907435617335,-7.42089714709858,
55.7830805233701));
#176396=CARTESIAN_POINT('Ctrl Pts',(-3.13207662038864,-7.49982273479723,
55.7906508198518));
#176397=CARTESIAN_POINT('Ctrl Pts',(-2.95234106915857,-7.57237285329657,
55.7982211163335));
#176398=CARTESIAN_POINT('Ctrl Pts',(-2.77039087292521,-7.63836513749589,
55.8057914128153));
#176399=CARTESIAN_POINT('Ctrl Pts',(-2.58825630921775,-7.70442429071213,
55.8133693801678));
#176400=CARTESIAN_POINT('Ctrl Pts',(-2.40390296661676,-7.76391221895912,
55.8209473475203));
#176401=CARTESIAN_POINT('Ctrl Pts',(-2.21786891603798,-7.81669655505269,
55.8285253148728));
#176402=CARTESIAN_POINT('Ctrl Pts',(-2.03438338178489,-7.86875778834944,
55.8359994701895));
#176403=CARTESIAN_POINT('Ctrl Pts',(-1.84926323846872,-7.91429791085689,
55.8434736255062));
#176404=CARTESIAN_POINT('Ctrl Pts',(-1.66303227187805,-7.95323903986245,
55.850947780823));
#176405=CARTESIAN_POINT('Ctrl Pts',(-1.46183445975847,-7.99530975506528,
55.8590226124404));
#176406=CARTESIAN_POINT('Ctrl Pts',(-1.2589105843238,-8.0297684172589,55.8670974440578));
#176407=CARTESIAN_POINT('Ctrl Pts',(-1.05486315500429,-8.05648504539755,
55.8751722756752));
#176408=CARTESIAN_POINT('Ctrl Pts',(-0.850950723195874,-8.08318399785014,
55.8832417649946));
#176409=CARTESIAN_POINT('Ctrl Pts',(-0.645916532928484,-8.10215108926084,
55.8913112543141));
#176410=CARTESIAN_POINT('Ctrl Pts',(-0.440372350046428,-8.11330757187317,
55.8993807436335));
#176411=CARTESIAN_POINT('Ctrl Pts',(-0.234936153408985,-8.12445819323153,
55.907445993505));
#176412=CARTESIAN_POINT('Ctrl Pts',(-0.0289908141246323,-8.12780637205476,
55.9155112433766));
#176413=CARTESIAN_POINT('Ctrl Pts',(0.176847097141084,-8.12332522226783,
55.9235764932482));
#176414=CARTESIAN_POINT('Ctrl Pts',(0.382604879940012,-8.11884581690038,
55.9316386034838));
#176415=CARTESIAN_POINT('Ctrl Pts',(0.588255001873923,-8.10654316857554,
55.9397007137194));
#176416=CARTESIAN_POINT('Ctrl Pts',(0.793180577158063,-8.086442489409,55.947762823955));
#176417=CARTESIAN_POINT('Ctrl Pts',(0.998054245006541,-8.06634690172364,
55.9558228920664));
#176418=CARTESIAN_POINT('Ctrl Pts',(1.20220341731265,-8.03845725418866,
55.9638829601779));
#176419=CARTESIAN_POINT('Ctrl Pts',(1.40501538642423,-8.00285069999504,
55.9719430282893));
#176420=CARTESIAN_POINT('Ctrl Pts',(1.61086578575788,-7.96671070573456,
55.9801238484187));
#176421=CARTESIAN_POINT('Ctrl Pts',(1.81533826366942,-7.92262077005964,
55.9883046685482));
#176422=CARTESIAN_POINT('Ctrl Pts',(2.0178010609234,-7.87071575150802,55.9964854886776));
#176423=CARTESIAN_POINT('Ctrl Pts',(2.21729479539547,-7.81957190617372,
56.0045463392674));
#176424=CARTESIAN_POINT('Ctrl Pts',(2.41483707918783,-7.76084071773865,
56.0126071898573));
#176425=CARTESIAN_POINT('Ctrl Pts',(2.60983676881351,-7.69470204768508,
56.0206680404471));
#176426=CARTESIAN_POINT('Ctrl Pts',(2.80486879734938,-7.62855240913965,
56.0287302278551));
#176427=CARTESIAN_POINT('Ctrl Pts',(2.99735709055459,-7.55499294051914,
56.0367924152631));
#176428=CARTESIAN_POINT('Ctrl Pts',(3.18672790230071,-7.47425266091521,
56.0448546026711));
#176429=CARTESIAN_POINT('Ctrl Pts',(3.37615357913105,-7.39348898899332,
56.0529191258804));
#176430=CARTESIAN_POINT('Ctrl Pts',(3.56245968161549,-7.30554048087805,
56.0609836490897));
#176431=CARTESIAN_POINT('Ctrl Pts',(3.74509404969466,-7.2106836098557,56.069048172299));
#176432=CARTESIAN_POINT('Ctrl Pts',(3.93237147111605,-7.11341522386678,
56.0773177172237));
#176433=CARTESIAN_POINT('Ctrl Pts',(4.11578768127097,-7.00888273012241,
56.0855872621484));
#176434=CARTESIAN_POINT('Ctrl Pts',(4.29477602916872,-6.89743332129987,
56.0938568070732));
#176435=CARTESIAN_POINT('Ctrl Pts',(4.46956267802646,-6.78860015470516,
56.101932226853));
#176436=CARTESIAN_POINT('Ctrl Pts',(4.64012677096593,-6.67317137814245,
56.1100076466328));
#176437=CARTESIAN_POINT('Ctrl Pts',(4.80597140041664,-6.55151329548199,
56.1180830664126));
#176438=CARTESIAN_POINT('Ctrl Pts',(4.97779614240671,-6.42546840193691,
56.1264496739098));
#176439=CARTESIAN_POINT('Ctrl Pts',(5.14455444401536,-6.29273684981324,
56.134816281407));
#176440=CARTESIAN_POINT('Ctrl Pts',(5.30573229981658,-6.15377057788012,
56.1431828889042));
#176441=CARTESIAN_POINT('Ctrl Pts',(5.46691015561774,-6.01480430594705,
56.1515494964014));
#176442=CARTESIAN_POINT('Ctrl Pts',(5.62250731674663,-5.86960359742682,
56.1599161038986));
#176443=CARTESIAN_POINT('Ctrl Pts',(5.77205298320038,-5.71866172470689,
56.1682827113957));
#176444=CARTESIAN_POINT('Ctrl Pts',(5.91643912919243,-5.57292754338514,
56.1763606600264));
#176445=CARTESIAN_POINT('Ctrl Pts',(6.05546510078527,-5.42155839124349,
56.184438608657));
#176446=CARTESIAN_POINT('Ctrl Pts',(6.18867972450313,-5.26497206355587,
56.1925165572876));
#176447=CARTESIAN_POINT('Ctrl Pts',(6.32173132057101,-5.10857736573825,
56.2005846201494));
#176448=CARTESIAN_POINT('Ctrl Pts',(6.44898554226959,-4.94697845792061,
56.2086526830111));
#176449=CARTESIAN_POINT('Ctrl Pts',(6.57002744988545,-4.78063038419115,
56.2167207458728));
#176450=CARTESIAN_POINT('Ctrl Pts',(6.69093612857618,-4.61446540717174,
56.2247799283446));
#176451=CARTESIAN_POINT('Ctrl Pts',(6.80564593991808,-4.44356193885165,
56.2328391108164));
#176452=CARTESIAN_POINT('Ctrl Pts',(6.91378130758381,-4.2684090236767,56.2408982932882));
#176453=CARTESIAN_POINT('Ctrl Pts',(7.02177777914472,-4.09348108630681,
56.2489471240214));
#176454=CARTESIAN_POINT('Ctrl Pts',(7.12321648869526,-3.91431485850987,
56.2569959547546));
#176455=CARTESIAN_POINT('Ctrl Pts',(7.21776435450075,-3.73142938904092,
56.2650447854878));
#176456=CARTESIAN_POINT('Ctrl Pts',(7.31224070472476,-3.54868225332053,
56.2730875281216));
#176457=CARTESIAN_POINT('Ctrl Pts',(7.39983645606923,-3.36222176263079,
56.2811302707554));
#176458=CARTESIAN_POINT('Ctrl Pts',(7.48026309217137,-3.17259383382097,
56.2891730133891));
#176459=CARTESIAN_POINT('Ctrl Pts',(7.56062421774698,-2.98312036410657,
56.2972092049059));
#176460=CARTESIAN_POINT('Ctrl Pts',(7.63382775364498,-2.79048489256754,
56.3052453964226));
#176461=CARTESIAN_POINT('Ctrl Pts',(7.69963207399846,-2.59525595800378,
56.3132815879393));
#176462=CARTESIAN_POINT('Ctrl Pts',(7.73694046776287,-2.48456903158642,
56.317837784187));
#176463=CARTESIAN_POINT('Ctrl Pts',(7.77187128670256,-2.37304886704202,
56.3223939804346));
#176464=CARTESIAN_POINT('Ctrl Pts',(7.80438735588229,-2.26080197316009,
56.3269501766823));
#176465=CARTESIAN_POINT('Ctrl Pts',(7.85866325892142,-2.07343918047128,
56.3345553907196));
#176466=CARTESIAN_POINT('Ctrl Pts',(7.90618641271472,-1.88412563235468,
56.3421606047569));
#176467=CARTESIAN_POINT('Ctrl Pts',(7.94682714905332,-1.69340657420746,
56.3497658187942));
#176468=CARTESIAN_POINT('Ctrl Pts',(7.9874729292636,-1.50266384615311,56.3573719767053));
#176469=CARTESIAN_POINT('Ctrl Pts',(8.02123452283479,-1.31051561809717,
56.3649781346163));
#176470=CARTESIAN_POINT('Ctrl Pts',(8.04803359127215,-1.11751638746601,
56.3725842925274));
#176471=CARTESIAN_POINT('Ctrl Pts',(8.07485448690262,-0.924359963629182,
56.3801966454701));
#176472=CARTESIAN_POINT('Ctrl Pts',(8.09470148545109,-0.730351513950841,
56.3878089984128));
#176473=CARTESIAN_POINT('Ctrl Pts',(8.10754817391848,-0.53605052941974,
56.3954213513555));
#176474=CARTESIAN_POINT('Ctrl Pts',(8.11951963742666,-0.354986969590803,
56.4025150864995));
#176475=CARTESIAN_POINT('Ctrl Pts',(8.12541265295082,-0.173669645053181,
56.4096088216436));
#176476=CARTESIAN_POINT('Ctrl Pts',(8.12524658453948,0.00745002882984703,
56.4167025567876));
#176477=CARTESIAN_POINT('',(8.12524979689129,-0.00180012532809755,52.4166320361364));
#176478=CARTESIAN_POINT('Ctrl Pts',(8.12524979923223,-0.00180626037467281,
52.41679142628));
#176479=CARTESIAN_POINT('Ctrl Pts',(8.12529142980181,0.185463959284471,
52.4241148867614));
#176480=CARTESIAN_POINT('Ctrl Pts',(8.11885447565195,0.372914385266139,
52.4314383472427));
#176481=CARTESIAN_POINT('Ctrl Pts',(8.10592778611965,0.560019900283289,
52.4387618077241));
#176482=CARTESIAN_POINT('Ctrl Pts',(8.09300372005407,0.747087442307473,
52.4460837819119));
#176483=CARTESIAN_POINT('Ctrl Pts',(8.07359255433145,0.933809827599829,
52.4534057560997));
#176484=CARTESIAN_POINT('Ctrl Pts',(8.04773524373084,1.11966289985534,52.4607277302875));
#176485=CARTESIAN_POINT('Ctrl Pts',(8.02188165943195,1.30548918879088,52.4680486493043));
#176486=CARTESIAN_POINT('Ctrl Pts',(7.98958383553074,1.49044603221675,52.4753695683211));
#176487=CARTESIAN_POINT('Ctrl Pts',(7.95093442865585,1.67401591202566,52.4826904873379));
#176488=CARTESIAN_POINT('Ctrl Pts',(7.91227199465363,1.85764766569988,52.4900138739358));
#176489=CARTESIAN_POINT('Ctrl Pts',(7.86725378425988,2.03989114479142,52.4973372605336));
#176490=CARTESIAN_POINT('Ctrl Pts',(7.8160232871797,2.22024042318949,52.5046606471314));
#176491=CARTESIAN_POINT('Ctrl Pts',(7.78274734470621,2.33738338597818,52.5094174346902));
#176492=CARTESIAN_POINT('Ctrl Pts',(7.74685150652963,2.4537274576232,52.514174222249));
#176493=CARTESIAN_POINT('Ctrl Pts',(7.70838622756085,2.56913785719065,52.5189310098078));
#176494=CARTESIAN_POINT('Ctrl Pts',(7.63379529391426,2.79293889768875,52.5281552565747));
#176495=CARTESIAN_POINT('Ctrl Pts',(7.54954791469676,3.01320771803129,52.5373795033417));
#176496=CARTESIAN_POINT('Ctrl Pts',(7.4559985125789,3.22920636425132,52.5466037501086));
#176497=CARTESIAN_POINT('Ctrl Pts',(7.36202586583066,3.44618225100003,52.5558697300436));
#176498=CARTESIAN_POINT('Ctrl Pts',(7.25866691095433,3.65884919165463,52.5651357099785));
#176499=CARTESIAN_POINT('Ctrl Pts',(7.1463242493121,3.86648901281173,52.5744016899135));
#176500=CARTESIAN_POINT('Ctrl Pts',(7.03351765094578,4.07498631532998,52.5837059351727));
#176501=CARTESIAN_POINT('Ctrl Pts',(6.91165304755985,4.2784148422899,52.5930101804319));
#176502=CARTESIAN_POINT('Ctrl Pts',(6.7811806751285,4.47607821801225,52.6023144256911));
#176503=CARTESIAN_POINT('Ctrl Pts',(6.65058492372394,4.67392851073386,52.6116274693511));
#176504=CARTESIAN_POINT('Ctrl Pts',(6.51136516903268,4.86600269982851,52.6209405130112));
#176505=CARTESIAN_POINT('Ctrl Pts',(6.36401470585195,5.05163383334541,52.6302535566712));
#176506=CARTESIAN_POINT('Ctrl Pts',(6.21679692851287,5.23709781012148,52.6395582141408));
#176507=CARTESIAN_POINT('Ctrl Pts',(6.06146312303957,5.41613028144629,52.6488628716105));
#176508=CARTESIAN_POINT('Ctrl Pts',(5.89854619522163,5.58809809732581,52.6581675290801));
#176509=CARTESIAN_POINT('Ctrl Pts',(5.78513954772361,5.70780507767257,52.6646445110849));
#176510=CARTESIAN_POINT('Ctrl Pts',(5.66805929710808,5.82408949441311,52.6711214930897));
#176511=CARTESIAN_POINT('Ctrl Pts',(5.54749678423229,5.93674717260491,52.6775984750944));
#176512=CARTESIAN_POINT('Ctrl Pts',(5.40290965348903,6.07185426400015,52.6853661320685));
#176513=CARTESIAN_POINT('Ctrl Pts',(5.2532451898613,6.20180571678652,52.6931337890425));
#176514=CARTESIAN_POINT('Ctrl Pts',(5.09891321461151,6.3261972457678,52.7009014460165));
#176515=CARTESIAN_POINT('Ctrl Pts',(4.94467551481463,6.45051278876035,52.7086643580284));
#176516=CARTESIAN_POINT('Ctrl Pts',(4.78577625325051,6.56927495205543,52.7164272700403));
#176517=CARTESIAN_POINT('Ctrl Pts',(4.62266063250388,6.68211764631534,52.7241901820522));
#176518=CARTESIAN_POINT('Ctrl Pts',(4.4596160671024,6.79491118478899,52.7319497124358));
#176519=CARTESIAN_POINT('Ctrl Pts',(4.29235908890434,6.90179019128051,52.7397092428194));
#176520=CARTESIAN_POINT('Ctrl Pts',(4.1213665088273,7.00242998268577,52.747468773203));
#176521=CARTESIAN_POINT('Ctrl Pts',(3.95039498770512,7.10305737958349,52.7552273479452));
#176522=CARTESIAN_POINT('Ctrl Pts',(3.77568907959939,7.19744690792926,52.7629859226873));
#176523=CARTESIAN_POINT('Ctrl Pts',(3.59775334397401,7.28531800530518,52.7707444974295));
#176524=CARTESIAN_POINT('Ctrl Pts',(3.4198345896975,7.37318071667726,52.7785023317298));
#176525=CARTESIAN_POINT('Ctrl Pts',(3.2386869381476,7.45452608415542,52.7862601660301));
#176526=CARTESIAN_POINT('Ctrl Pts',(3.0548381577906,7.5291202269725,52.7940180003304));
#176527=CARTESIAN_POINT('Ctrl Pts',(2.87091998578194,7.60374252450873,52.8017787627379));
#176528=CARTESIAN_POINT('Ctrl Pts',(2.68429897349192,7.67160837433803,52.8095395251454));
#176529=CARTESIAN_POINT('Ctrl Pts',(2.4955220439955,7.73253239827888,52.8173002875529));
#176530=CARTESIAN_POINT('Ctrl Pts',(2.34174515461608,7.78216085083975,52.8236221718288));
#176531=CARTESIAN_POINT('Ctrl Pts',(2.18653809678768,7.82718383344977,52.8299440561048));
#176532=CARTESIAN_POINT('Ctrl Pts',(2.03020328100823,7.86752579914953,52.8362659403807));
#176533=CARTESIAN_POINT('Ctrl Pts',(1.8225771514488,7.92110341175808,52.8446619483792));
#176534=CARTESIAN_POINT('Ctrl Pts',(1.61286290931407,7.96644911872512,52.8530579563777));
#176535=CARTESIAN_POINT('Ctrl Pts',(1.40171550536911,8.00342934025832,52.8614539643762));
#176536=CARTESIAN_POINT('Ctrl Pts',(1.19051779013239,8.04041837327905,52.8698519729393));
#176537=CARTESIAN_POINT('Ctrl Pts',(0.977886494570286,8.06903789590412,
52.8782499815023));
#176538=CARTESIAN_POINT('Ctrl Pts',(0.764484866176533,8.0892057985866,52.8866479900654));
#176539=CARTESIAN_POINT('Ctrl Pts',(0.551036542337206,8.1093781143057,52.8950478362374));
#176540=CARTESIAN_POINT('Ctrl Pts',(0.336817815055019,8.12109509325748,
52.9034476824095));
#176541=CARTESIAN_POINT('Ctrl Pts',(0.122496212510106,8.12432657150245,
52.9118475285815));
#176542=CARTESIAN_POINT('Ctrl Pts',(-0.0919039381742978,8.12755923407322,
52.9202504532687));
#176543=CARTESIAN_POINT('Ctrl Pts',(-0.306406772346929,8.12230017603941,
52.9286533779558));
#176544=CARTESIAN_POINT('Ctrl Pts',(-0.520344185914271,8.10857135941253,
52.937056302643));
#176545=CARTESIAN_POINT('Ctrl Pts',(-0.734304306751976,8.09484108561206,
52.9454601192147));
#176546=CARTESIAN_POINT('Ctrl Pts',(-0.947698620842927,8.07263927854439,
52.9538639357865));
#176547=CARTESIAN_POINT('Ctrl Pts',(-1.15986297180958,8.04203988109516,
52.9622677523582));
#176548=CARTESIAN_POINT('Ctrl Pts',(-1.37207112322722,8.01143416652713,
52.970673303863));
#176549=CARTESIAN_POINT('Ctrl Pts',(-1.58304853993314,7.97242743636115,
52.9790788553679));
#176550=CARTESIAN_POINT('Ctrl Pts',(-1.79213879196529,7.92514517929061,
52.9874844068727));
#176551=CARTESIAN_POINT('Ctrl Pts',(-1.85390404454704,7.91117800233131,
52.9899674064709));
#176552=CARTESIAN_POINT('Ctrl Pts',(-1.91550468941563,7.89648903272553,
52.9924504060691));
#176553=CARTESIAN_POINT('Ctrl Pts',(-1.97692399346394,7.8810823550174,52.9949334056673));
#176554=CARTESIAN_POINT('Ctrl Pts',(-2.18546791597217,7.82877031645138,
53.0033642155539));
#176555=CARTESIAN_POINT('Ctrl Pts',(-2.39194333430613,7.76817430305625,
53.0117950254405));
#176556=CARTESIAN_POINT('Ctrl Pts',(-2.5957044001731,7.69948090649117,53.020225835327));
#176557=CARTESIAN_POINT('Ctrl Pts',(-2.79943222349145,7.63079871689325,
53.0286552697712));
#176558=CARTESIAN_POINT('Ctrl Pts',(-3.00044632993504,7.55402186671484,
53.0370847042154));
#176559=CARTESIAN_POINT('Ctrl Pts',(-3.1981173121605,7.46938640185118,53.0455141386595));
#176560=CARTESIAN_POINT('Ctrl Pts',(-3.39574895585102,7.3847677803054,53.0539418955606));
#176561=CARTESIAN_POINT('Ctrl Pts',(-3.59003856248263,7.29229377063194,
53.0623696524616));
#176562=CARTESIAN_POINT('Ctrl Pts',(-3.78037692044528,7.19224845940855,
53.0707974093626));
#176563=CARTESIAN_POINT('Ctrl Pts',(-3.97066168704092,7.09223131678475,
53.0792227933577));
#176564=CARTESIAN_POINT('Ctrl Pts',(-4.15699719452033,6.98464725259868,
53.0876481773528));
#176565=CARTESIAN_POINT('Ctrl Pts',(-4.33879814483341,6.86982665144399,
53.096073561348));
#176566=CARTESIAN_POINT('Ctrl Pts',(-4.52054763823719,6.75503854909224,
53.1044965606239));
#176567=CARTESIAN_POINT('Ctrl Pts',(-4.69776491502061,6.63301813953614,
53.1129195598998));
#176568=CARTESIAN_POINT('Ctrl Pts',(-4.86989202172793,6.50414016294319,
53.1213425591757));
#176569=CARTESIAN_POINT('Ctrl Pts',(-5.04195466287281,6.3753104541182,53.1297624038445));
#176570=CARTESIAN_POINT('Ctrl Pts',(-5.20893073079048,6.23962846456765,
53.1381822485134));
#176571=CARTESIAN_POINT('Ctrl Pts',(-5.37029303830708,6.09751098770724,
53.1466020931822));
#176572=CARTESIAN_POINT('Ctrl Pts',(-5.41500245102512,6.05813383064257,
53.148935019106));
#176573=CARTESIAN_POINT('Ctrl Pts',(-5.4592810817868,6.01826286209088,53.1512679450297));
#176574=CARTESIAN_POINT('Ctrl Pts',(-5.50311816005396,5.9779075000358,53.1536008709535));
#176575=CARTESIAN_POINT('Ctrl Pts',(-5.64845632790801,5.84411267118276,
53.1613354918019));
#176576=CARTESIAN_POINT('Ctrl Pts',(-5.78900199474849,5.70493168866682,
53.1690701126502));
#176577=CARTESIAN_POINT('Ctrl Pts',(-5.92433287199729,5.56075242968722,
53.1768047334986));
#176578=CARTESIAN_POINT('Ctrl Pts',(-6.05962189912813,5.41661775712514,
53.1845369624701));
#176579=CARTESIAN_POINT('Ctrl Pts',(-6.18969910655291,5.26748814351576,
53.1922691914416));
#176580=CARTESIAN_POINT('Ctrl Pts',(-6.31417889455817,5.11378846355773,
53.2000014204131));
#176581=CARTESIAN_POINT('Ctrl Pts',(-6.4386423110938,4.96010899804321,53.2077326324489));
#176582=CARTESIAN_POINT('Ctrl Pts',(-6.55750955281092,4.80186093838473,
53.2154638444846));
#176583=CARTESIAN_POINT('Ctrl Pts',(-6.67043508813259,4.63950248383483,
53.2231950565203));
#176584=CARTESIAN_POINT('Ctrl Pts',(-6.78340106456531,4.47708588516128,
53.2309290372726));
#176585=CARTESIAN_POINT('Ctrl Pts',(-6.89042087788212,4.31055623859291,
53.2386630180249));
#176586=CARTESIAN_POINT('Ctrl Pts',(-6.99119178996117,4.14040154073002,
53.2463969987773));
#176587=CARTESIAN_POINT('Ctrl Pts',(-7.09197973207841,3.97021808713849,
53.2541322865534));
#176588=CARTESIAN_POINT('Ctrl Pts',(-7.18651649518555,3.79640866959065,
53.2618675743296));
#176589=CARTESIAN_POINT('Ctrl Pts',(-7.27454510353943,3.6194863032025,53.2696028621058));
#176590=CARTESIAN_POINT('Ctrl Pts',(-7.36264578837941,3.44241907547074,
53.277344483418));
#176591=CARTESIAN_POINT('Ctrl Pts',(-7.44422752112627,3.26223412640846,
53.2850861047302));
#176592=CARTESIAN_POINT('Ctrl Pts',(-7.5190809496,3.07946573870573,53.2928277260425));
#176593=CARTESIAN_POINT('Ctrl Pts',(-7.58173777845746,2.92647758809798,
53.2993079294417));
#176594=CARTESIAN_POINT('Ctrl Pts',(-7.63968110812795,2.77167975125065,
53.3057881328409));
#176595=CARTESIAN_POINT('Ctrl Pts',(-7.69281501789776,2.61539378734957,
53.3122683362401));
#176596=CARTESIAN_POINT('Ctrl Pts',(-7.76986127328381,2.38877300336918,
53.321664885604));
#176597=CARTESIAN_POINT('Ctrl Pts',(-7.83683934975107,2.15889379270417,
53.3310614349679));
#176598=CARTESIAN_POINT('Ctrl Pts',(-7.8935407830906,1.92657765693091,53.3404579843318));
#176599=CARTESIAN_POINT('Ctrl Pts',(-7.95032228177454,1.69393347880798,
53.3498678021074));
#176600=CARTESIAN_POINT('Ctrl Pts',(-7.99679810175101,1.45884552910251,
53.359277619883));
#176601=CARTESIAN_POINT('Ctrl Pts',(-8.0328103301751,1.22214801146677,53.3686874376586));
#176602=CARTESIAN_POINT('Ctrl Pts',(-8.06876814688821,0.985808125598951,
53.3780830379223));
#176603=CARTESIAN_POINT('Ctrl Pts',(-8.09429396780832,0.747863569393553,
53.3874786381861));
#176604=CARTESIAN_POINT('Ctrl Pts',(-8.10928174435626,0.509153368986473,
53.3968742384498));
#176605=CARTESIAN_POINT('Ctrl Pts',(-8.12423175226499,0.271044709402109,
53.4062461621504));
#176606=CARTESIAN_POINT('Ctrl Pts',(-8.12869673648614,0.0321742965836574,
53.4156180858511));
#176607=CARTESIAN_POINT('Ctrl Pts',(-8.12262253898462,-0.206617162111417,
53.4249900095518));
#176608=CARTESIAN_POINT('Ctrl Pts',(-8.11658772510818,-0.443860354837681,
53.4343011679696));
#176609=CARTESIAN_POINT('Ctrl Pts',(-8.1001499332365,-0.681025568421049,
53.4436123263874));
#176610=CARTESIAN_POINT('Ctrl Pts',(-8.07330682219572,-0.91728104591125,
53.4529234848052));
#176611=CARTESIAN_POINT('Ctrl Pts',(-8.05599760400982,-1.06962544449004,
53.458927590379));
#176612=CARTESIAN_POINT('Ctrl Pts',(-8.03436283170225,-1.22159142398268,
53.4649316959528));
#176613=CARTESIAN_POINT('Ctrl Pts',(-8.00841329672666,-1.3729544898909,
53.4709358015266));
#176614=CARTESIAN_POINT('Ctrl Pts',(-7.97570399173204,-1.56374714541908,
53.4785039572033));
#176615=CARTESIAN_POINT('Ctrl Pts',(-7.93614904893175,-1.75350540783528,
53.4860721128799));
#176616=CARTESIAN_POINT('Ctrl Pts',(-7.88983874489199,-1.94168281191886,
53.4936402685566));
#176617=CARTESIAN_POINT('Ctrl Pts',(-7.84354123413481,-2.12980823174636,
53.5012063335203));
#176618=CARTESIAN_POINT('Ctrl Pts',(-7.79049216315058,-2.31635330559633,
53.508772398484));
#176619=CARTESIAN_POINT('Ctrl Pts',(-7.73083284066094,-2.50078210811303,
53.5163384634477));
#176620=CARTESIAN_POINT('Ctrl Pts',(-7.67117870900688,-2.68519486385699,
53.5239038701036));
#176621=CARTESIAN_POINT('Ctrl Pts',(-7.60491558457017,-2.86749136525201,
53.5314692767595));
#176622=CARTESIAN_POINT('Ctrl Pts',(-7.53223451333963,-3.04715125954641,
53.5390346834153));
#176623=CARTESIAN_POINT('Ctrl Pts',(-7.45951771598275,-3.22689946503346,
53.5466038088204));
#176624=CARTESIAN_POINT('Ctrl Pts',(-7.38037680440389,-3.40400813173496,
53.5541729342254));
#176625=CARTESIAN_POINT('Ctrl Pts',(-7.29505104634859,-3.57797677377431,
53.5617420596305));
#176626=CARTESIAN_POINT('Ctrl Pts',(-7.20970627224065,-3.75198418718738,
53.5693128719222));
#176627=CARTESIAN_POINT('Ctrl Pts',(-7.11817407806062,-3.9228498569337,
53.576883684214));
#176628=CARTESIAN_POINT('Ctrl Pts',(-7.02073938188642,-4.09009854332742,
53.5844544965058));
#176629=CARTESIAN_POINT('Ctrl Pts',(-6.9232059119717,-4.25751677690504,
53.5920329836554));
#176630=CARTESIAN_POINT('Ctrl Pts',(-6.81975818026263,-4.42131038948132,
53.5996114708051));
#176631=CARTESIAN_POINT('Ctrl Pts',(-6.71072457615695,-4.58103298672506,
53.6071899579548));
#176632=CARTESIAN_POINT('Ctrl Pts',(-6.60323593554964,-4.7384923772755,
53.6146610609075));
#176633=CARTESIAN_POINT('Ctrl Pts',(-6.49031892947357,-4.89199512838687,
53.6221321638602));
#176634=CARTESIAN_POINT('Ctrl Pts',(-6.37232536909627,-5.04114639272379,
53.6296032668129));
#176635=CARTESIAN_POINT('Ctrl Pts',(-6.24479984339853,-5.20234665935044,
53.6376779136711));
#176636=CARTESIAN_POINT('Ctrl Pts',(-6.11107242724856,-5.35880848322185,
53.6457525605292));
#176637=CARTESIAN_POINT('Ctrl Pts',(-5.97152241968435,-5.5100460573127,
53.6538272073874));
#176638=CARTESIAN_POINT('Ctrl Pts',(-5.83206481307636,-5.66118349169946,
53.6618965077386));
#176639=CARTESIAN_POINT('Ctrl Pts',(-5.68679251715282,-5.80710334209315,
53.6699658080898));
#176640=CARTESIAN_POINT('Ctrl Pts',(-5.53612476371952,-5.94735320651392,
53.678035108441));
#176641=CARTESIAN_POINT('Ctrl Pts',(-5.38553623836849,-6.08752932106094,
53.6861001655803));
#176642=CARTESIAN_POINT('Ctrl Pts',(-5.22955814501596,-6.22204118025769,
53.6941652227197));
#176643=CARTESIAN_POINT('Ctrl Pts',(-5.06864663283712,-6.3504731220539,
53.7022302798591));
#176644=CARTESIAN_POINT('Ctrl Pts',(-4.90779782796481,-6.47885501385036,
53.7102921940411));
#176645=CARTESIAN_POINT('Ctrl Pts',(-4.74201968601487,-6.60116151651033,
53.7183541082232));
#176646=CARTESIAN_POINT('Ctrl Pts',(-4.57180197775206,-6.71701676629754,
53.7264160224053));
#176647=CARTESIAN_POINT('Ctrl Pts',(-4.4016274473332,-6.83284262795619,
53.7344758915823));
#176648=CARTESIAN_POINT('Ctrl Pts',(-4.22701585865114,-6.94222032293446,
53.7425357607594));
#176649=CARTESIAN_POINT('Ctrl Pts',(-4.0484870533218,-7.04481654421077,
53.7505956299364));
#176650=CARTESIAN_POINT('Ctrl Pts',(-3.86727648178455,-7.14895391218758,
53.7587765702468));
#176651=CARTESIAN_POINT('Ctrl Pts',(-3.68203034285036,-7.24610425315686,
53.7669575105572));
#176652=CARTESIAN_POINT('Ctrl Pts',(-3.49332014501591,-7.3359663253675,
53.7751384508675));
#176653=CARTESIAN_POINT('Ctrl Pts',(-3.30738476615581,-7.42450705413245,
53.7831990975814));
#176654=CARTESIAN_POINT('Ctrl Pts',(-3.11808680048448,-7.50597225396094,
53.7912597442952));
#176655=CARTESIAN_POINT('Ctrl Pts',(-2.92599533830767,-7.58012129472225,
53.7993203910091));
#176656=CARTESIAN_POINT('Ctrl Pts',(-2.73387204916043,-7.65428262098184,
53.8073823732636));
#176657=CARTESIAN_POINT('Ctrl Pts',(-2.53895463601142,-7.72112525625011,
53.8154443555182));
#176658=CARTESIAN_POINT('Ctrl Pts',(-2.34183032616524,-7.78045745994108,
53.8235063377727));
#176659=CARTESIAN_POINT('Ctrl Pts',(-2.14464892525096,-7.83980684740246,
53.8315706549355));
#176660=CARTESIAN_POINT('Ctrl Pts',(-1.94525965622814,-7.8916413735799,
53.8396349720983));
#176661=CARTESIAN_POINT('Ctrl Pts',(-1.7442635756675,-7.93581956329021,
53.8476992892611));
#176662=CARTESIAN_POINT('Ctrl Pts',(-1.53814329739408,-7.98112403256795,
53.8559691982715));
#176663=CARTESIAN_POINT('Ctrl Pts',(-1.33033353834054,-8.01837652543524,
53.8642391072819));
#176664=CARTESIAN_POINT('Ctrl Pts',(-1.12149192529827,-8.04748056375353,
53.8725090162922));
#176665=CARTESIAN_POINT('Ctrl Pts',(-0.917566984062273,-8.07589941772295,
53.8805842302518));
#176666=CARTESIAN_POINT('Ctrl Pts',(-0.712658547025337,-8.09654916905283,
53.8886594442113));
#176667=CARTESIAN_POINT('Ctrl Pts',(-0.507382800075561,-8.10939271811937,
53.8967346581708));
#176668=CARTESIAN_POINT('Ctrl Pts',(-0.294683193115528,-8.12270075805598,
53.9051019147067));
#176669=CARTESIAN_POINT('Ctrl Pts',(-0.0815895931428846,-8.12762743478942,
53.9134691712425));
#176670=CARTESIAN_POINT('Ctrl Pts',(0.131213614354412,-8.12419045504893,
53.9218364277783));
#176671=CARTESIAN_POINT('Ctrl Pts',(0.344016821851631,-8.12075347530843,
53.9302036843141));
#176672=CARTESIAN_POINT('Ctrl Pts',(0.556529264119323,-8.10895289716088,
53.9385709408499));
#176673=CARTESIAN_POINT('Ctrl Pts',(0.768073252409577,-8.08886586867609,
53.9469381973857));
#176674=CARTESIAN_POINT('Ctrl Pts',(0.972307163530668,-8.06947296404473,
53.9550163164638));
#176675=CARTESIAN_POINT('Ctrl Pts',(1.17603556407372,-8.04231901093511,
53.9630944355419));
#176676=CARTESIAN_POINT('Ctrl Pts',(1.37864434331301,-8.00743575292059,
53.97117255462));
#176677=CARTESIAN_POINT('Ctrl Pts',(1.58100514933681,-7.97259518858248,
53.979240786875));
#176678=CARTESIAN_POINT('Ctrl Pts',(1.78224875691176,-7.93004422929355,
53.9873090191299));
#176679=CARTESIAN_POINT('Ctrl Pts',(1.98176501262701,-7.87986643270223,
53.9953772513849));
#176680=CARTESIAN_POINT('Ctrl Pts',(2.18106163449512,-7.82974387342714,
54.0034366018729));
#176681=CARTESIAN_POINT('Ctrl Pts',(2.37863439093669,-7.77201129082964,
54.0114959523609));
#176682=CARTESIAN_POINT('Ctrl Pts',(2.57388156976952,-7.70680356745264,
54.0195553028489));
#176683=CARTESIAN_POINT('Ctrl Pts',(2.76887789789266,-7.64167962200158,
54.0276042988017));
#176684=CARTESIAN_POINT('Ctrl Pts',(2.96155431105262,-7.56909979483945,
54.0356532947545));
#176685=CARTESIAN_POINT('Ctrl Pts',(3.15132250263827,-7.48924923118904,
54.0437022907072));
#176686=CARTESIAN_POINT('Ctrl Pts',(3.34094711543319,-7.40945908254956,
54.0517451967822));
#176687=CARTESIAN_POINT('Ctrl Pts',(3.52766760279783,-7.32240928431047,
54.0597881028571));
#176688=CARTESIAN_POINT('Ctrl Pts',(3.71091266240122,-7.22833416317551,
54.0678310089321));
#176689=CARTESIAN_POINT('Ctrl Pts',(3.89400838944722,-7.13433570701835,
54.0758673605725));
#176690=CARTESIAN_POINT('Ctrl Pts',(4.07363405838302,-7.0333234921172,54.083903712213));
#176691=CARTESIAN_POINT('Ctrl Pts',(4.24923987684056,-6.92557925603108,
54.0919400638535));
#176692=CARTESIAN_POINT('Ctrl Pts',(4.3487775266202,-6.86450720197548,54.0964952634598));
#176693=CARTESIAN_POINT('Ctrl Pts',(4.44702402957637,-6.80127308141812,
54.101050463066));
#176694=CARTESIAN_POINT('Ctrl Pts',(4.54388266994327,-6.73593481591748,
54.1056056626723));
#176695=CARTESIAN_POINT('Ctrl Pts',(4.71476441173592,-6.62066253280297,
54.1136421211646));
#176696=CARTESIAN_POINT('Ctrl Pts',(4.88118962102054,-6.49892972876899,
54.121678579657));
#176697=CARTESIAN_POINT('Ctrl Pts',(5.04267165464983,-6.37111843759721,
54.1297150381493));
#176698=CARTESIAN_POINT('Ctrl Pts',(5.2042512233777,-6.24322994844493,54.1377563506601));
#176699=CARTESIAN_POINT('Ctrl Pts',(5.3608814122162,-6.10925584351674,54.1457976631709));
#176700=CARTESIAN_POINT('Ctrl Pts',(5.51210984118968,-5.96961746355325,
54.1538389756816));
#176701=CARTESIAN_POINT('Ctrl Pts',(5.66344810492306,-5.82987766649482,
54.1618861284675));
#176702=CARTESIAN_POINT('Ctrl Pts',(5.80937654981052,-5.68446560085876,
54.1699332812534));
#176703=CARTESIAN_POINT('Ctrl Pts',(5.94948030747646,-5.53383877913423,
54.1779804340393));
#176704=CARTESIAN_POINT('Ctrl Pts',(6.08979055673919,-5.38298995641946,
54.1860394471026));
#176705=CARTESIAN_POINT('Ctrl Pts',(6.22425874553431,-5.22691124793029,
54.1940984601659));
#176706=CARTESIAN_POINT('Ctrl Pts',(6.35250978663326,-5.06609385752264,
54.2021574732292));
#176707=CARTESIAN_POINT('Ctrl Pts',(6.48086462185065,-4.90514631691017,
54.2102230084863));
#176708=CARTESIAN_POINT('Ctrl Pts',(6.60299208143421,-4.7394526949591,54.2182885437435));
#176709=CARTESIAN_POINT('Ctrl Pts',(6.71856045953086,-4.56953311774063,
54.2263540790006));
#176710=CARTESIAN_POINT('Ctrl Pts',(6.83431030468434,-4.39934673046492,
54.2344322788722));
#176711=CARTESIAN_POINT('Ctrl Pts',(6.94348031450639,-4.22492139177615,
54.2425104787438));
#176712=CARTESIAN_POINT('Ctrl Pts',(7.04578389662639,-4.04680328710703,
54.2505886786153));
#176713=CARTESIAN_POINT('Ctrl Pts',(7.10355122967148,-3.9462260867729,54.2551501617297));
#176714=CARTESIAN_POINT('Ctrl Pts',(7.15913007684663,-3.84447186092738,
54.2597116448442));
#176715=CARTESIAN_POINT('Ctrl Pts',(7.21247563134185,-3.74164172921459,
54.2642731279586));
#176716=CARTESIAN_POINT('Ctrl Pts',(7.31207324622793,-3.54965505002594,
54.2727895421723));
#176717=CARTESIAN_POINT('Ctrl Pts',(7.40405480498203,-3.35358662842629,
54.2813059563859));
#176718=CARTESIAN_POINT('Ctrl Pts',(7.48810513339414,-3.1540401192338,54.2898223705996));
#176719=CARTESIAN_POINT('Ctrl Pts',(7.57205211902636,-2.95473895936195,
54.2983283135881));
#176720=CARTESIAN_POINT('Ctrl Pts',(7.64808723974097,-2.75196847756056,
54.3068342565765));
#176721=CARTESIAN_POINT('Ctrl Pts',(7.71594230646601,-2.54635462687113,
54.315340199565));
#176722=CARTESIAN_POINT('Ctrl Pts',(7.7836627303163,-2.34114876988477,54.3238292644532));
#176723=CARTESIAN_POINT('Ctrl Pts',(7.84323542574184,-2.13311104534834,
54.3323183293414));
#176724=CARTESIAN_POINT('Ctrl Pts',(7.89444118896209,-1.92288477983439,
54.3408073942297));
#176725=CARTESIAN_POINT('Ctrl Pts',(7.94558245025501,-1.71292332824858,
54.3492857657699));
#176726=CARTESIAN_POINT('Ctrl Pts',(7.98837774946234,-1.50077907902443,
54.3577641373101));
#176727=CARTESIAN_POINT('Ctrl Pts',(8.02265754136298,-1.28711053779843,
54.3662425088503));
#176728=CARTESIAN_POINT('Ctrl Pts',(8.0568660294448,-1.07388643867972,54.3747032449198));
#176729=CARTESIAN_POINT('Ctrl Pts',(8.08259432589578,-0.859144623191298,
54.3831639809892));
#176730=CARTESIAN_POINT('Ctrl Pts',(8.09972385147236,-0.643553488367279,
54.3916247170586));
#176731=CARTESIAN_POINT('Ctrl Pts',(8.11664796987523,-0.430547595351899,
54.3999839969683));
#176732=CARTESIAN_POINT('Ctrl Pts',(8.12517833118536,-0.216712883417576,
54.4083432768779));
#176733=CARTESIAN_POINT('Ctrl Pts',(8.12524955008195,-0.0027039587645105,
54.4167025567876));
#176734=CARTESIAN_POINT('',(8.12524999842753,0.000155745727534607,50.4167086581892));
#176735=CARTESIAN_POINT('Ctrl Pts',(8.12524999842753,0.000155745727534607,
50.4167086581892));
#176736=CARTESIAN_POINT('Ctrl Pts',(8.12520464167094,2.24634946216138,50.5047042175299));
#176737=CARTESIAN_POINT('Ctrl Pts',(7.14394733579225,4.47538755847567,50.5926997768706));
#176738=CARTESIAN_POINT('Ctrl Pts',(3.83078204044946,7.50935546634353,50.7686929293524));
#176739=CARTESIAN_POINT('Ctrl Pts',(1.52412477697767,8.29110090552131,50.8566905224936));
#176740=CARTESIAN_POINT('Ctrl Pts',(-2.95101623932526,7.89663306204436,
51.032685708776));
#176741=CARTESIAN_POINT('Ctrl Pts',(-5.08535169588699,6.72342983085812,
51.1206833019172));
#176742=CARTESIAN_POINT('Ctrl Pts',(-7.81671694684382,3.15661951052992,
51.2966784881996));
#176743=CARTESIAN_POINT('Ctrl Pts',(-8.39290461146695,0.790229551554735,
51.3846760813408));
#176744=CARTESIAN_POINT('Ctrl Pts',(-7.60701611462514,-3.63299000730349,
51.5606712676232));
#176745=CARTESIAN_POINT('Ctrl Pts',(-6.25093680401409,-5.65606750609959,
51.6486688607644));
#176746=CARTESIAN_POINT('Ctrl Pts',(-2.45807268688641,-8.0636957548829,
51.8246640470468));
#176747=CARTESIAN_POINT('Ctrl Pts',(-0.0502299510463028,-8.42987470330084,
51.912661640188));
#176748=CARTESIAN_POINT('Ctrl Pts',(4.28689960880906,-7.25863639434614,
52.0886568264704));
#176749=CARTESIAN_POINT('Ctrl Pts',(6.18309125557085,-5.7301564626646,52.1766544196116));
#176750=CARTESIAN_POINT('Ctrl Pts',(7.81022974018296,-2.58694001339646,
52.3153120205474));
#176751=CARTESIAN_POINT('Ctrl Pts',(8.12495798447121,-1.29495785838389,
52.3659720283419));
#176752=CARTESIAN_POINT('Ctrl Pts',(8.12524979689129,-0.00180012532809755,
52.4166320361364));
#176753=CARTESIAN_POINT('',(8.12524962724961,0.00113542683362771,48.4167025567876));
#176754=CARTESIAN_POINT('Ctrl Pts',(8.12524824860312,0.00533489193623286,
48.4167025567876));
#176755=CARTESIAN_POINT('Ctrl Pts',(8.12509405526136,0.240177358298132,
48.4258982129203));
#176756=CARTESIAN_POINT('Ctrl Pts',(8.11475436208719,0.474765486234928,
48.4350938690529));
#176757=CARTESIAN_POINT('Ctrl Pts',(8.09431945547053,0.708293805769365,
48.4442895251855));
#176758=CARTESIAN_POINT('Ctrl Pts',(8.0737852173659,0.94295727683138,48.4535298802358));
#176759=CARTESIAN_POINT('Ctrl Pts',(8.04305742039561,1.17655052682022,48.462770235286));
#176760=CARTESIAN_POINT('Ctrl Pts',(8.00227883614591,1.40826879219532,48.4720105903362));
#176761=CARTESIAN_POINT('Ctrl Pts',(7.96144009132553,1.64032891110307,48.4812645776653));
#176762=CARTESIAN_POINT('Ctrl Pts',(7.91052092462163,1.87050843279415,48.4905185649944));
#176763=CARTESIAN_POINT('Ctrl Pts',(7.84971528909508,2.09801273653117,48.4997725523235));
#176764=CARTESIAN_POINT('Ctrl Pts',(7.78890031216287,2.32555199114029,48.5090279613177));
#176765=CARTESIAN_POINT('Ctrl Pts',(7.71819586053827,2.55041513008745,48.5182833703119));
#176766=CARTESIAN_POINT('Ctrl Pts',(7.63784592382679,2.77182200120833,48.5275387793061));
#176767=CARTESIAN_POINT('Ctrl Pts',(7.56635283748268,2.96882353228684,48.5357739787531));
#176768=CARTESIAN_POINT('Ctrl Pts',(7.48722417490742,3.1630889238551,48.5440091782001));
#176769=CARTESIAN_POINT('Ctrl Pts',(7.4006648329993,3.35407924654553,48.5522443776471));
#176770=CARTESIAN_POINT('Ctrl Pts',(7.31732883794868,3.53795736109197,48.5601729099721));
#176771=CARTESIAN_POINT('Ctrl Pts',(7.22706578225808,3.71888253593403,48.5681014422972));
#176772=CARTESIAN_POINT('Ctrl Pts',(7.13011092176217,3.89630668786067,48.5760299746223));
#176773=CARTESIAN_POINT('Ctrl Pts',(7.03322245478509,4.07360934186849,48.583953077584));
#176774=CARTESIAN_POINT('Ctrl Pts',(6.92965147418736,4.24741545864518,48.5918761805458));
#176775=CARTESIAN_POINT('Ctrl Pts',(6.81968041450227,4.41719895483033,48.5997992835076));
#176776=CARTESIAN_POINT('Ctrl Pts',(6.70976771037649,4.58689235630411,48.6077181821168));
#176777=CARTESIAN_POINT('Ctrl Pts',(6.59346187718006,4.75256711206116,48.6156370807261));
#176778=CARTESIAN_POINT('Ctrl Pts',(6.47109036267713,4.91372334188313,48.6235559793353));
#176779=CARTESIAN_POINT('Ctrl Pts',(6.3487604732,5.07482475394583,48.6314721843082));
#176780=CARTESIAN_POINT('Ctrl Pts',(6.22036921596723,5.23141043754099,48.6393883892811));
#176781=CARTESIAN_POINT('Ctrl Pts',(6.08628654583634,5.38301064874216,48.647304594254));
#176782=CARTESIAN_POINT('Ctrl Pts',(5.95223227009314,5.53457875590508,48.6552191228299));
#176783=CARTESIAN_POINT('Ctrl Pts',(5.81248920625189,5.68116324623945,48.6631336514057));
#176784=CARTESIAN_POINT('Ctrl Pts',(5.66746688746875,5.82232828359457,48.6710481799816));
#176785=CARTESIAN_POINT('Ctrl Pts',(5.52242962534958,5.96350786682515,48.6789635240833));
#176786=CARTESIAN_POINT('Ctrl Pts',(5.37211225842041,6.09926664600249,48.6868788681851));
#176787=CARTESIAN_POINT('Ctrl Pts',(5.2169608776247,6.22920594970445,48.6947942122868));
#176788=CARTESIAN_POINT('Ctrl Pts',(5.11165180460258,6.3174023134868,48.7001667558358));
#176789=CARTESIAN_POINT('Ctrl Pts',(5.00411644590343,6.40291840952884,48.7055392993848));
#176790=CARTESIAN_POINT('Ctrl Pts',(4.89450297224217,6.48564015477367,48.7109118429337));
#176791=CARTESIAN_POINT('Ctrl Pts',(4.72941840659802,6.6102241399986,48.71900322065));
#176792=CARTESIAN_POINT('Ctrl Pts',(4.55956536848283,6.72850849743512,48.7270945983663));
#176793=CARTESIAN_POINT('Ctrl Pts',(4.38545483821631,6.84013694486193,48.7351859760825));
#176794=CARTESIAN_POINT('Ctrl Pts',(4.21133698669297,6.95177008620663,48.743277694037));
#176795=CARTESIAN_POINT('Ctrl Pts',(4.0329615488586,7.05674659121316,48.7513694119915));
#176796=CARTESIAN_POINT('Ctrl Pts',(3.85086745973168,7.15475417957037,48.7594611299459));
#176797=CARTESIAN_POINT('Ctrl Pts',(3.66874498380537,7.25277704641225,48.7675541093251));
#176798=CARTESIAN_POINT('Ctrl Pts',(3.48290297530535,7.34382868226941,48.7756470887042));
#176799=CARTESIAN_POINT('Ctrl Pts',(3.29390445147555,7.42764303309264,48.7837400680833));
#176800=CARTESIAN_POINT('Ctrl Pts',(3.10479503248428,7.51150656210931,48.79183779603));
#176801=CARTESIAN_POINT('Ctrl Pts',(2.91252568231339,7.5881241929646,48.7999355239767));
#176802=CARTESIAN_POINT('Ctrl Pts',(2.71768000648576,7.65727777639335,48.8080332519233));
#176803=CARTESIAN_POINT('Ctrl Pts',(2.52277499100083,7.72645242033538,48.8161334460084));
#176804=CARTESIAN_POINT('Ctrl Pts',(2.32529238051981,7.78815838282438,48.8242336400934));
#176805=CARTESIAN_POINT('Ctrl Pts',(2.12583148881044,7.84222723744231,48.8323338341784));
#176806=CARTESIAN_POINT('Ctrl Pts',(1.92621631634278,7.89633791371168,48.8404402936726));
#176807=CARTESIAN_POINT('Ctrl Pts',(1.72462010761914,7.94279960123247,48.8485467531668));
#176808=CARTESIAN_POINT('Ctrl Pts',(1.52165420994225,7.98149459862406,48.8566532126609));
#176809=CARTESIAN_POINT('Ctrl Pts',(1.41377494853402,8.00206154009835,48.8609619111806));
#176810=CARTESIAN_POINT('Ctrl Pts',(1.30550889176043,8.02043520376885,48.8652706097003));
#176811=CARTESIAN_POINT('Ctrl Pts',(1.19694860265409,8.03660386015787,48.86957930822));
#176812=CARTESIAN_POINT('Ctrl Pts',(0.978053846880687,8.06920541382536,
48.8782671213967));
#176813=CARTESIAN_POINT('Ctrl Pts',(0.757838365444617,8.0928577768821,48.8869549345734));
#176814=CARTESIAN_POINT('Ctrl Pts',(0.537011557224253,8.1074845759895,48.8956427477501));
#176815=CARTESIAN_POINT('Ctrl Pts',(0.316234220785276,8.12210809825829,
48.904328614598));
#176816=CARTESIAN_POINT('Ctrl Pts',(0.0948460474159337,8.12771008307366,
48.9130144814458));
#176817=CARTESIAN_POINT('Ctrl Pts',(-0.126440066090956,8.12426614976312,
48.9217003482936));
#176818=CARTESIAN_POINT('Ctrl Pts',(-0.352643206937182,8.12074569147786,
48.9305792170614));
#176819=CARTESIAN_POINT('Ctrl Pts',(-0.578739470335517,8.10777262911778,
48.9394580858291));
#176820=CARTESIAN_POINT('Ctrl Pts',(-0.803966609970434,8.08537724862314,
48.9483369545969));
#176821=CARTESIAN_POINT('Ctrl Pts',(-1.02394625691664,8.06350365069696,
48.9570089575357));
#176822=CARTESIAN_POINT('Ctrl Pts',(-1.2430965929378,8.0326418826472,48.9656809604745));
#176823=CARTESIAN_POINT('Ctrl Pts',(-1.46071001826149,7.99287268790455,
48.9743529634133));
#176824=CARTESIAN_POINT('Ctrl Pts',(-1.68611001525814,7.95168048497764,
48.9833352650955));
#176825=CARTESIAN_POINT('Ctrl Pts',(-1.90986086182544,7.90093167741484,
48.9923175667777));
#176826=CARTESIAN_POINT('Ctrl Pts',(-2.13118291449833,7.84077463950153,
49.00129986846));
#176827=CARTESIAN_POINT('Ctrl Pts',(-2.35250496717114,7.78061760158825,
49.0102821701422));
#176828=CARTESIAN_POINT('Ctrl Pts',(-2.57139796323687,7.71105235475339,
49.0192644718244));
#176829=CARTESIAN_POINT('Ctrl Pts',(-2.7870929229118,7.63228672165525,49.0282467735066));
#176830=CARTESIAN_POINT('Ctrl Pts',(-2.97744349581197,7.56277613407511,
49.0361736452043));
#176831=CARTESIAN_POINT('Ctrl Pts',(-3.16523267751558,7.48612560747436,
49.0441005169019));
#176832=CARTESIAN_POINT('Ctrl Pts',(-3.34990292770109,7.4025561759084,49.0520273885996));
#176833=CARTESIAN_POINT('Ctrl Pts',(-3.53456242783743,7.31899160909731,
49.0599537988571));
#176834=CARTESIAN_POINT('Ctrl Pts',(-3.716103055548,7.22850907745022,49.0678802091146));
#176835=CARTESIAN_POINT('Ctrl Pts',(-3.89398852514512,7.13137721120809,
49.0758066193722));
#176836=CARTESIAN_POINT('Ctrl Pts',(-4.07189066434111,7.03423624276525,
49.0837337724114));
#176837=CARTESIAN_POINT('Ctrl Pts',(-4.24613667118519,6.93044485765078,
49.0916609254507));
#176838=CARTESIAN_POINT('Ctrl Pts',(-4.41621572419633,6.82031716563541,
49.09958807849));
#176839=CARTESIAN_POINT('Ctrl Pts',(-4.58639777019186,6.71012278475117,
49.107520031892));
#176840=CARTESIAN_POINT('Ctrl Pts',(-4.75240754060323,6.59358461043873,
49.115451985294));
#176841=CARTESIAN_POINT('Ctrl Pts',(-4.91376315920374,6.47106012781152,
49.1233839386961));
#176842=CARTESIAN_POINT('Ctrl Pts',(-5.07517035288604,6.34849648193565,
49.1313184274368));
#176843=CARTESIAN_POINT('Ctrl Pts',(-5.23192016811001,6.219942919279,49.1392529161775));
#176844=CARTESIAN_POINT('Ctrl Pts',(-5.38356408656067,6.08579701340705,
49.1471874049182));
#176845=CARTESIAN_POINT('Ctrl Pts',(-5.53534800335026,5.95152726343908,
49.1551292188142));
#176846=CARTESIAN_POINT('Ctrl Pts',(-5.68201636049718,5.81165508017606,
49.1630710327102));
#176847=CARTESIAN_POINT('Ctrl Pts',(-5.82315689846523,5.66661550648681,
49.1710128466061));
#176848=CARTESIAN_POINT('Ctrl Pts',(-5.91735582569032,5.56981431496942,
49.1763133106684));
#176849=CARTESIAN_POINT('Ctrl Pts',(-6.00909322572258,5.47071211191697,
49.1816137747306));
#176850=CARTESIAN_POINT('Ctrl Pts',(-6.09825655253652,5.3694463943637,49.1869142387928));
#176851=CARTESIAN_POINT('Ctrl Pts',(-6.23208145070166,5.2174570639581,49.1948696851484));
#176852=CARTESIAN_POINT('Ctrl Pts',(-6.36033685696158,5.06033019130039,
49.202825131504));
#176853=CARTESIAN_POINT('Ctrl Pts',(-6.48261644312577,4.8985070801026,49.2107805778595));
#176854=CARTESIAN_POINT('Ctrl Pts',(-6.60480242608076,4.7368078420958,49.218729934439));
#176855=CARTESIAN_POINT('Ctrl Pts',(-6.72102150762917,4.57041979332046,
49.2266792910184));
#176856=CARTESIAN_POINT('Ctrl Pts',(-6.83090671507786,4.39981829311214,
49.2346286475978));
#176857=CARTESIAN_POINT('Ctrl Pts',(-6.94072590306755,4.22931929094708,
49.242573228173));
#176858=CARTESIAN_POINT('Ctrl Pts',(-7.04421862370558,4.05461216063073,
49.2505178087481));
#176859=CARTESIAN_POINT('Ctrl Pts',(-7.14106017126255,3.87620267696462,
49.2584623893232));
#176860=CARTESIAN_POINT('Ctrl Pts',(-7.23785947669766,3.69787101521831,
49.2664035044856));
#176861=CARTESIAN_POINT('Ctrl Pts',(-7.32801323521957,3.51584050984272,
49.2743446196479));
#176862=CARTESIAN_POINT('Ctrl Pts',(-7.41124157611675,3.33064346079531,
49.2822857348102));
#176863=CARTESIAN_POINT('Ctrl Pts',(-7.49444730802118,3.14549672055728,
49.2902246927673));
#176864=CARTESIAN_POINT('Ctrl Pts',(-7.57073123781064,2.95718545319507,
49.2981636507244));
#176865=CARTESIAN_POINT('Ctrl Pts',(-7.63986053311785,2.76626437583399,
49.3061026086814));
#176866=CARTESIAN_POINT('Ctrl Pts',(-7.71175143377586,2.56771630522097,
49.3143587153766));
#176867=CARTESIAN_POINT('Ctrl Pts',(-7.77590415649592,2.36634596511415,
49.3226148220718));
#176868=CARTESIAN_POINT('Ctrl Pts',(-7.83211284222034,2.16279818504346,
49.330870928767));
#176869=CARTESIAN_POINT('Ctrl Pts',(-7.88617341184988,1.96702934975347,
49.3388115134847));
#176870=CARTESIAN_POINT('Ctrl Pts',(-7.93288578425423,1.76924675451631,
49.3467520982024));
#176871=CARTESIAN_POINT('Ctrl Pts',(-7.97211821269964,1.5700378228701,49.35469268292));
#176872=CARTESIAN_POINT('Ctrl Pts',(-8.01136013437536,1.37078068782833,
49.3626351890533));
#176873=CARTESIAN_POINT('Ctrl Pts',(-8.04311843908364,1.17009685298631,
49.3705776951866));
#176874=CARTESIAN_POINT('Ctrl Pts',(-8.06731275359214,0.968582726580205,
49.3785202013198));
#176875=CARTESIAN_POINT('Ctrl Pts',(-8.09151653536827,0.766989747426939,
49.3864658153664));
#176876=CARTESIAN_POINT('Ctrl Pts',(-8.10815038611567,0.564566157414711,
49.3944114294129));
#176877=CARTESIAN_POINT('Ctrl Pts',(-8.11718588958296,0.36191269175768,
49.4023570434594));
#176878=CARTESIAN_POINT('Ctrl Pts',(-8.12622627820231,0.159149659102155,
49.4103069533964));
#176879=CARTESIAN_POINT('Ctrl Pts',(-8.1276601137808,-0.0438431668199141,
49.4182568633334));
#176880=CARTESIAN_POINT('Ctrl Pts',(-8.12151108857014,-0.246465414880581,
49.4262067732703));
#176881=CARTESIAN_POINT('Ctrl Pts',(-8.11535469856938,-0.449330346988657,
49.4341662049471));
#176882=CARTESIAN_POINT('Ctrl Pts',(-8.1015973137944,-0.651823483752154,
49.4421256366238));
#176883=CARTESIAN_POINT('Ctrl Pts',(-8.08031458130745,-0.853348597942344,
49.4500850683006));
#176884=CARTESIAN_POINT('Ctrl Pts',(-8.05901692913426,-1.05501498588464,
49.4580500797224));
#176885=CARTESIAN_POINT('Ctrl Pts',(-8.0301834536962,-1.25571167114033,
49.4660150911443));
#176886=CARTESIAN_POINT('Ctrl Pts',(-7.99394096336068,-1.45485237629254,
49.4739801025662));
#176887=CARTESIAN_POINT('Ctrl Pts',(-7.95765074415915,-1.6542553360511,
49.4819556033601));
#176888=CARTESIAN_POINT('Ctrl Pts',(-7.9139320897016,-1.85209790024651,
49.489931104154));
#176889=CARTESIAN_POINT('Ctrl Pts',(-7.86296203991051,-2.04780749130046,
49.4979066049478));
#176890=CARTESIAN_POINT('Ctrl Pts',(-7.84945062821162,-2.09968722987224,
49.5000207930872));
#176891=CARTESIAN_POINT('Ctrl Pts',(-7.83542992459351,-2.15141718538454,
49.5021349812266));
#176892=CARTESIAN_POINT('Ctrl Pts',(-7.82090379551784,-2.20298692319193,
49.5042491693659));
#176893=CARTESIAN_POINT('Ctrl Pts',(-7.76804293468209,-2.39065018292006,
49.5119427403395));
#176894=CARTESIAN_POINT('Ctrl Pts',(-7.70832839993634,-2.5767471830493,
49.5196363113131));
#176895=CARTESIAN_POINT('Ctrl Pts',(-7.64186410911351,-2.76072463319737,
49.5273298822867));
#176896=CARTESIAN_POINT('Ctrl Pts',(-7.57548016190044,-2.94447968704398,
49.5350141530894));
#176897=CARTESIAN_POINT('Ctrl Pts',(-7.50236281859812,-3.12611995856152,
49.5426984238921));
#176898=CARTESIAN_POINT('Ctrl Pts',(-7.42266685376287,-3.30510277306924,
49.5503826946948));
#176899=CARTESIAN_POINT('Ctrl Pts',(-7.34305114840654,-3.48390533921112,
49.5580592268927));
#176900=CARTESIAN_POINT('Ctrl Pts',(-7.25687015394062,-3.66005545187811,
49.5657357590907));
#176901=CARTESIAN_POINT('Ctrl Pts',(-7.16432829059914,-3.83302592047339,
49.5734122912886));
#176902=CARTESIAN_POINT('Ctrl Pts',(-7.07186098524913,-4.00585703234666,
49.5810826387524));
#176903=CARTESIAN_POINT('Ctrl Pts',(-6.97304318171762,-4.17551328660332,
49.5887529862162));
#176904=CARTESIAN_POINT('Ctrl Pts',(-6.86812726052436,-4.34148770535426,
49.5964233336801));
#176905=CARTESIAN_POINT('Ctrl Pts',(-6.76327476256909,-4.50736179009542,
49.6040890443045));
#176906=CARTESIAN_POINT('Ctrl Pts',(-6.65233167795167,-4.669558169658,49.611754754929));
#176907=CARTESIAN_POINT('Ctrl Pts',(-6.53559620385363,-4.82759462078932,
49.6194204655534));
#176908=CARTESIAN_POINT('Ctrl Pts',(-6.41890783646469,-4.98556729887146,
49.6270830828045));
#176909=CARTESIAN_POINT('Ctrl Pts',(-6.29643194718965,-5.13938310428014,
49.6347457000557));
#176910=CARTESIAN_POINT('Ctrl Pts',(-6.16850996881306,-5.28858887862858,
49.6424083173068));
#176911=CARTESIAN_POINT('Ctrl Pts',(-6.04058987852066,-5.43779245075135,
49.6500708214604));
#176912=CARTESIAN_POINT('Ctrl Pts',(-5.90722408351136,-5.58238584811721,
49.6577333256139));
#176913=CARTESIAN_POINT('Ctrl Pts',(-5.76879447776803,-5.7219487795482,
49.6653958297675));
#176914=CARTESIAN_POINT('Ctrl Pts',(-5.63035960384037,-5.86151702229424,
49.6730586255312));
#176915=CARTESIAN_POINT('Ctrl Pts',(-5.48686078699429,-5.99605416267736,
49.680721421295));
#176916=CARTESIAN_POINT('Ctrl Pts',(-5.33871686536881,-6.12517671532231,
49.6883842170587));
#176917=CARTESIAN_POINT('Ctrl Pts',(-5.19054034300347,-6.25432768284047,
49.6960486991071));
#176918=CARTESIAN_POINT('Ctrl Pts',(-5.03771695023212,-6.37806145431482,
49.7037131811554));
#176919=CARTESIAN_POINT('Ctrl Pts',(-4.88069872336345,-6.49603475469908,
49.7113776632037));
#176920=CARTESIAN_POINT('Ctrl Pts',(-4.72361735401347,-6.61405549624393,
49.7190452274064));
#176921=CARTESIAN_POINT('Ctrl Pts',(-4.56233807763212,-6.72631093904359,
49.7267127916091));
#176922=CARTESIAN_POINT('Ctrl Pts',(-4.3973420624435,-6.83250103171343,
49.7343803558118));
#176923=CARTESIAN_POINT('Ctrl Pts',(-4.23215008656796,-6.93881724308669,
49.7420570265445));
#176924=CARTESIAN_POINT('Ctrl Pts',(-4.06323285690005,-7.03905352323911,
49.7497336972771));
#176925=CARTESIAN_POINT('Ctrl Pts',(-3.89109725091988,-7.13295519026888,
49.7574103680097));
#176926=CARTESIAN_POINT('Ctrl Pts',(-3.71885251649102,-7.22691638794133,
49.7650919055052));
#176927=CARTESIAN_POINT('Ctrl Pts',(-3.54338566076395,-7.31453481388569,
49.7727734430006));
#176928=CARTESIAN_POINT('Ctrl Pts',(-3.36522360387869,-7.39560394142342,
49.780454980496));
#176929=CARTESIAN_POINT('Ctrl Pts',(-3.18678481962152,-7.47679898828989,
49.788148449217));
#176930=CARTESIAN_POINT('Ctrl Pts',(-3.00564280229518,-7.55142428215892,
49.795841917938));
#176931=CARTESIAN_POINT('Ctrl Pts',(-2.82234092344189,-7.61932275693616,
49.803535386659));
#176932=CARTESIAN_POINT('Ctrl Pts',(-2.67900015934634,-7.6724188807532,
49.8095516244189));
#176933=CARTESIAN_POINT('Ctrl Pts',(-2.53433894520927,-7.72140246568362,
49.8155678621787));
#176934=CARTESIAN_POINT('Ctrl Pts',(-2.38862097292405,-7.76622027824394,
49.8215840999386));
#176935=CARTESIAN_POINT('Ctrl Pts',(-2.1962582923516,-7.82538439112784,
49.8295261513157));
#176936=CARTESIAN_POINT('Ctrl Pts',(-2.00145107000579,-7.87747278895808,
49.8374682026927));
#176937=CARTESIAN_POINT('Ctrl Pts',(-1.80475697291493,-7.92228122646596,
49.8454102540698));
#176938=CARTESIAN_POINT('Ctrl Pts',(-1.60828922623835,-7.96703809959776,
49.8533431659422));
#176939=CARTESIAN_POINT('Ctrl Pts',(-1.40993925436718,-8.00453163140133,
49.8612760778146));
#176940=CARTESIAN_POINT('Ctrl Pts',(-1.21028139561434,-8.03460680468745,
49.8692089896869));
#176941=CARTESIAN_POINT('Ctrl Pts',(-1.01081919040248,-8.0646525059849,
49.8771341277491));
#176942=CARTESIAN_POINT('Ctrl Pts',(-0.810051980740767,-8.08729428572821,
49.8850592658113));
#176943=CARTESIAN_POINT('Ctrl Pts',(-0.608566267360869,-8.10242770166636,
49.8929844038735));
#176944=CARTESIAN_POINT('Ctrl Pts',(-0.407243597863957,-8.11754887152088,
49.9009031288493));
#176945=CARTESIAN_POINT('Ctrl Pts',(-0.205203915256688,-8.12517376165031,
49.9088218538251));
#176946=CARTESIAN_POINT('Ctrl Pts',(-0.00304126880216057,-8.12524943082882,
49.916740578801));
#176947=CARTESIAN_POINT('Ctrl Pts',(0.198992286934878,-8.12532505168887,
49.9246542472844));
#176948=CARTESIAN_POINT('Ctrl Pts',(0.401148316694656,-8.11786105996389,
49.9325679157677));
#176949=CARTESIAN_POINT('Ctrl Pts',(0.602829902214262,-8.10285651307589,
49.9404815842511));
#176950=CARTESIAN_POINT('Ctrl Pts',(0.813547487829065,-8.0871797130084,
49.9487498111787));
#176951=CARTESIAN_POINT('Ctrl Pts',(1.0237467640609,-8.06327110342906,49.9570180381062));
#176952=CARTESIAN_POINT('Ctrl Pts',(1.23274817861052,-8.03119041553819,
49.9652862650337));
#176953=CARTESIAN_POINT('Ctrl Pts',(1.43264913325689,-8.00050660342659,
49.9731944720648));
#176954=CARTESIAN_POINT('Ctrl Pts',(1.63145396338488,-7.96234732507618,
49.9811026790958));
#176955=CARTESIAN_POINT('Ctrl Pts',(1.82857437159921,-7.91681775273566,
49.9890108861269));
#176956=CARTESIAN_POINT('Ctrl Pts',(2.02567888788894,-7.87129185100712,
49.9969184555952));
#176957=CARTESIAN_POINT('Ctrl Pts',(2.22109892714147,-7.81839691460787,
50.0048260250635));
#176958=CARTESIAN_POINT('Ctrl Pts',(2.4142575022211,-7.75828900437907,50.0127335945318));
#176959=CARTESIAN_POINT('Ctrl Pts',(2.60743037754448,-7.69817664413935,
50.0206417494268));
#176960=CARTESIAN_POINT('Ctrl Pts',(2.79834113580858,-7.63085034532393,
50.0285499043217));
#176961=CARTESIAN_POINT('Ctrl Pts',(2.98642867148884,-7.55651582097261,
50.0364580592166));
#176962=CARTESIAN_POINT('Ctrl Pts',(3.1745592206354,-7.48216429716651,50.0443680226161));
#176963=CARTESIAN_POINT('Ctrl Pts',(3.35986494964294,-7.40080147664705,
50.0522779860155));
#176964=CARTESIAN_POINT('Ctrl Pts',(3.54180507075917,-7.31268106806557,
50.0601879494149));
#176965=CARTESIAN_POINT('Ctrl Pts',(3.72388341191931,-7.22449371434484,
50.0681039220193));
#176966=CARTESIAN_POINT('Ctrl Pts',(3.90259073642823,-7.12953866306084,
50.0760198946238));
#176967=CARTESIAN_POINT('Ctrl Pts',(4.07741025868074,-7.02811590292199,
50.0839358672282));
#176968=CARTESIAN_POINT('Ctrl Pts',(4.25230714285979,-6.92664826072411,
50.0918553428447));
#176969=CARTESIAN_POINT('Ctrl Pts',(4.42331250995822,-6.81870737797382,
50.0997748184612));
#176970=CARTESIAN_POINT('Ctrl Pts',(4.58993838759777,-6.70463669116801,
50.1076942940777));
#176971=CARTESIAN_POINT('Ctrl Pts',(4.75672701053396,-6.5904545902888,50.1156215047316));
#176972=CARTESIAN_POINT('Ctrl Pts',(4.91912733013389,-6.47013092322236,
50.1235487153856));
#176973=CARTESIAN_POINT('Ctrl Pts',(5.07668346350215,-6.34405017113703,
50.1314759260395));
#176974=CARTESIAN_POINT('Ctrl Pts',(5.12599491373206,-6.30458979216928,
50.1339569608635));
#176975=CARTESIAN_POINT('Ctrl Pts',(5.17483211521669,-6.26456576137527,
50.1364379956876));
#176976=CARTESIAN_POINT('Ctrl Pts',(5.22318182438274,-6.22399061631183,
50.1389190305116));
#176977=CARTESIAN_POINT('Ctrl Pts',(5.381146124221,-6.09142675002737,50.1470248689046));
#176978=CARTESIAN_POINT('Ctrl Pts',(5.53418169031714,-5.95274456759449,
50.1551307072977));
#176979=CARTESIAN_POINT('Ctrl Pts',(5.68180697082179,-5.80833514088339,
50.1632365456907));
#176980=CARTESIAN_POINT('Ctrl Pts',(5.82930838711782,-5.66404688013585,
50.171335582923));
#176981=CARTESIAN_POINT('Ctrl Pts',(5.97140834685528,-5.51404117448959,
50.1794346201553));
#176982=CARTESIAN_POINT('Ctrl Pts',(6.10765932867919,-5.35874846277543,
50.1875336573877));
#176983=CARTESIAN_POINT('Ctrl Pts',(6.24381173869352,-5.20356809875523,
50.1956268353099));
#176984=CARTESIAN_POINT('Ctrl Pts',(6.37412340357326,-5.04310859039263,
50.2037200132321));
#176985=CARTESIAN_POINT('Ctrl Pts',(6.49818410722792,-4.87783669991836,
50.2118131911543));
#176986=CARTESIAN_POINT('Ctrl Pts',(6.62215384031421,-4.71268599913084,
50.2199004345543));
#176987=CARTESIAN_POINT('Ctrl Pts',(6.73988157087455,-4.54273020667023,
50.2279876779544));
#176988=CARTESIAN_POINT('Ctrl Pts',(6.85099752114733,-4.36846889970996,
50.2360749213544));
#176989=CARTESIAN_POINT('Ctrl Pts',(6.96206384269067,-4.19428542466521,
50.2441585526753));
#176990=CARTESIAN_POINT('Ctrl Pts',(7.06652410506711,-4.01580053289428,
50.2522421839961));
#176991=CARTESIAN_POINT('Ctrl Pts',(7.16405146167329,-3.83354329791602,
50.260325815317));
#176992=CARTESIAN_POINT('Ctrl Pts',(7.26154376603157,-3.65135156789968,
50.2684065413048));
#176993=CARTESIAN_POINT('Ctrl Pts',(7.35210798796967,-3.465390474538,50.2764872672926));
#176994=CARTESIAN_POINT('Ctrl Pts',(7.43546262163905,-3.27621476168894,
50.2845679932804));
#176995=CARTESIAN_POINT('Ctrl Pts',(7.48022561735247,-3.17462386925059,
50.2889074941195));
#176996=CARTESIAN_POINT('Ctrl Pts',(7.52291023104088,-3.07210634064467,
50.2932469949587));
#176997=CARTESIAN_POINT('Ctrl Pts',(7.56347845227602,-2.96875079190833,
50.2975864957978));
#176998=CARTESIAN_POINT('Ctrl Pts',(7.63905678384256,-2.77620007871927,
50.305670957558));
#176999=CARTESIAN_POINT('Ctrl Pts',(7.70726142573685,-2.58080430198568,
50.3137554193181));
#177000=CARTESIAN_POINT('Ctrl Pts',(7.76789915218257,-2.38315553920035,
50.3218398810783));
#177001=CARTESIAN_POINT('Ctrl Pts',(7.82858569751626,-2.18534765117446,
50.3299308515659));
#177002=CARTESIAN_POINT('Ctrl Pts',(7.88169305932133,-1.98528345031682,
50.3380218220535));
#177003=CARTESIAN_POINT('Ctrl Pts',(7.9270780998098,-1.78356955625953,50.3461127925411));
#177004=CARTESIAN_POINT('Ctrl Pts',(7.97248100561706,-1.58177625976075,
50.3542069479497));
#177005=CARTESIAN_POINT('Ctrl Pts',(8.01015546311294,-1.37833228028703,
50.3623011033582));
#177006=CARTESIAN_POINT('Ctrl Pts',(8.04000967540918,-1.17385347545031,
50.3703952587668));
#177007=CARTESIAN_POINT('Ctrl Pts',(8.06989506292854,-0.969161143882411,
50.3784978664868));
#177008=CARTESIAN_POINT('Ctrl Pts',(8.09194384218465,-0.763432136862623,
50.3866004742068));
#177009=CARTESIAN_POINT('Ctrl Pts',(8.10611605649862,-0.557288113165248,
50.3947030819268));
#177010=CARTESIAN_POINT('Ctrl Pts',(8.11887801713983,-0.37165714128154,
50.4019994125159));
#177011=CARTESIAN_POINT('Ctrl Pts',(8.12525366522605,-0.185689847070898,
50.409295743105));
#177012=CARTESIAN_POINT('Ctrl Pts',(8.12524999841854,0.000160310478422246,
50.416592073694));
#177013=CARTESIAN_POINT('',(8.12525,4.14113188185183E-13,46.4167025567876));
#177014=CARTESIAN_POINT('Ctrl Pts',(8.12525,4.14112967973255E-13,46.4167025567876));
#177015=CARTESIAN_POINT('Ctrl Pts',(8.12524999999989,2.24624642433447,46.5047001499288));
#177016=CARTESIAN_POINT('Ctrl Pts',(7.14398562317582,4.47535249753478,46.59269774307));
#177017=CARTESIAN_POINT('Ctrl Pts',(3.83078204044914,7.50935546634369,46.7686929293524));
#177018=CARTESIAN_POINT('Ctrl Pts',(1.52412477697731,8.29110090552138,46.8566905224936));
#177019=CARTESIAN_POINT('Ctrl Pts',(-2.9510162393256,7.89663306204424,47.032685708776));
#177020=CARTESIAN_POINT('Ctrl Pts',(-5.08535169588728,6.7234298308579,47.1206833019172));
#177021=CARTESIAN_POINT('Ctrl Pts',(-7.81671694684396,3.15661951052958,
47.2966784881996));
#177022=CARTESIAN_POINT('Ctrl Pts',(-8.39290461146698,0.790229551554374,
47.3846760813408));
#177023=CARTESIAN_POINT('Ctrl Pts',(-7.60701611462498,-3.63299000730381,
47.5606712676232));
#177024=CARTESIAN_POINT('Ctrl Pts',(-6.25093680401385,-5.65606750609986,
47.6486688607644));
#177025=CARTESIAN_POINT('Ctrl Pts',(-2.45807268688606,-8.06369575488301,
47.8246640470468));
#177026=CARTESIAN_POINT('Ctrl Pts',(-0.0502299510459392,-8.42987470330084,
47.912661640188));
#177027=CARTESIAN_POINT('Ctrl Pts',(4.28689960880937,-7.25863639434595,
48.0886568264704));
#177028=CARTESIAN_POINT('Ctrl Pts',(6.1830912555711,-5.73015646266433,48.1766544196116));
#177029=CARTESIAN_POINT('Ctrl Pts',(7.81050559202892,-2.58640713800313,
48.3153355274311));
#177030=CARTESIAN_POINT('Ctrl Pts',(8.12525000000004,-1.29375883538159,
48.3660190421093));
#177031=CARTESIAN_POINT('Ctrl Pts',(8.12525,2.38922734780257E-13,48.4167025567876));
#177032=CARTESIAN_POINT('',(8.12525,5.33559741527911E-13,42.4167025567876));
#177033=CARTESIAN_POINT('Ctrl Pts',(8.12524980845225,-0.00176429777071613,
46.4169402126099));
#177034=CARTESIAN_POINT('Ctrl Pts',(8.12524336551536,-0.0314364271678197,
46.4157867211515));
#177035=CARTESIAN_POINT('Ctrl Pts',(8.12507438574217,-0.0611082895719105,
46.4146319165874));
#177036=CARTESIAN_POINT('Ctrl Pts',(8.12437406859321,-0.123787156037501,
46.4121895060278));
#177037=CARTESIAN_POINT('Ctrl Pts',(8.1238041070432,-0.156793138196381,
46.4109016018563));
#177038=CARTESIAN_POINT('Ctrl Pts',(8.1222235994471,-0.224437375940562,
46.4082582697045));
#177039=CARTESIAN_POINT('Ctrl Pts',(8.12119256875095,-0.259074480346016,
46.406902695888));
#177040=CARTESIAN_POINT('Ctrl Pts',(8.11826360209412,-0.340050718864486,
46.4037285183971));
#177041=CARTESIAN_POINT('Ctrl Pts',(8.11619043274539,-0.386382246215232,
46.4019084990561));
#177042=CARTESIAN_POINT('Ctrl Pts',(8.10816968998069,-0.536784525350514,
46.3959872082714));
#177043=CARTESIAN_POINT('Ctrl Pts',(8.10061612005149,-0.640758594942385,
46.3918732211905));
#177044=CARTESIAN_POINT('Ctrl Pts',(8.08072228816024,-0.85694361806308,
46.3832762487718));
#177045=CARTESIAN_POINT('Ctrl Pts',(8.06803990408777,-0.969101100063071,
46.3787917803781));
#177046=CARTESIAN_POINT('Ctrl Pts',(8.03316353031277,-1.22892661807609,
46.3683533355293));
#177047=CARTESIAN_POINT('Ctrl Pts',(8.00922716218528,-1.37632012200615,
46.36239396653));
#177048=CARTESIAN_POINT('Ctrl Pts',(7.95287798781533,-1.67162239496777,
46.3504093054814));
#177049=CARTESIAN_POINT('Ctrl Pts',(7.92036464764697,-1.8194543570788,46.3443865170123));
#177050=CARTESIAN_POINT('Ctrl Pts',(7.87759736522188,-1.99092740557492,
46.3374041968547));
#177051=CARTESIAN_POINT('Ctrl Pts',(7.87133774666267,-2.01553324614104,
46.3364023665107));
#177052=CARTESIAN_POINT('Ctrl Pts',(7.86023131383483,-2.05835040207013,
46.3346595165833));
#177053=CARTESIAN_POINT('Ctrl Pts',(7.85543628679765,-2.0765749279254,46.3339178415516));
#177054=CARTESIAN_POINT('Ctrl Pts',(7.84594759615601,-2.11213551717461,
46.3324710580468));
#177055=CARTESIAN_POINT('Ctrl Pts',(7.84125976796006,-2.12947302831123,
46.3317658714593));
#177056=CARTESIAN_POINT('Ctrl Pts',(7.83182091250608,-2.16392798625774,
46.330364943579));
#177057=CARTESIAN_POINT('Ctrl Pts',(7.8270711730163,-2.18104561840115,46.3296692059075));
#177058=CARTESIAN_POINT('Ctrl Pts',(7.81311361609309,-2.23071458181794,
46.327651138887));
#177059=CARTESIAN_POINT('Ctrl Pts',(7.80375859356496,-2.26322419412593,
46.326331103278));
#177060=CARTESIAN_POINT('Ctrl Pts',(7.7571464083772,-2.42148039431153,46.3199074389535));
#177061=CARTESIAN_POINT('Ctrl Pts',(7.71705112061419,-2.54637201197463,
46.3148448902823));
#177062=CARTESIAN_POINT('Ctrl Pts',(7.65788772160375,-2.71640056833077,
46.3079325100559));
#177063=CARTESIAN_POINT('Ctrl Pts',(7.64140921612542,-2.76241590314978,
46.3060597455096));
#177064=CARTESIAN_POINT('Ctrl Pts',(7.50902671784351,-3.12183611318082,
46.2914073490015));
#177065=CARTESIAN_POINT('Ctrl Pts',(7.3743039082081,-3.4279713168692,46.2787735834716));
#177066=CARTESIAN_POINT('Ctrl Pts',(7.09796167809606,-3.96368421756942,
46.2558516907867));
#177067=CARTESIAN_POINT('Ctrl Pts',(6.96304550455104,-4.19617055669198,
46.2456047079432));
#177068=CARTESIAN_POINT('Ctrl Pts',(6.75747299275486,-4.51310954346834,
46.2310572037499));
#177069=CARTESIAN_POINT('Ctrl Pts',(6.6962436596425,-4.60346821379332,46.2268402812932));
#177070=CARTESIAN_POINT('Ctrl Pts',(6.59800694296685,-4.74233150138394,
46.2202427902082));
#177071=CARTESIAN_POINT('Ctrl Pts',(6.56224193997055,-4.79169952766249,
46.2178735694056));
#177072=CARTESIAN_POINT('Ctrl Pts',(6.50107200302626,-4.87416563644041,
46.2138746312995));
#177073=CARTESIAN_POINT('Ctrl Pts',(6.47596148784595,-4.90747905070353,
46.2122476227983));
#177074=CARTESIAN_POINT('Ctrl Pts',(6.42926783382067,-4.96844371676085,
46.2092484063285));
#177075=CARTESIAN_POINT('Ctrl Pts',(6.40776002280285,-4.99615145157797,
46.2078769008142));
#177076=CARTESIAN_POINT('Ctrl Pts',(6.36285554445283,-5.05323332654042,
46.2050337632221));
#177077=CARTESIAN_POINT('Ctrl Pts',(6.33943328737875,-5.08258628224926,
46.2035619339907));
#177078=CARTESIAN_POINT('Ctrl Pts',(6.2861213898629,-5.14845531641048,46.2002366431198));
#177079=CARTESIAN_POINT('Ctrl Pts',(6.25611544707481,-5.18487548223448,
46.1983822276097));
#177080=CARTESIAN_POINT('Ctrl Pts',(6.16331715168767,-5.29553235236255,
46.1926988024806));
#177081=CARTESIAN_POINT('Ctrl Pts',(6.09950832993655,-5.36890484046775,
46.1888617021973));
#177082=CARTESIAN_POINT('Ctrl Pts',(5.81876339123752,-5.68026144051294,
46.1722764913487));
#177083=CARTESIAN_POINT('Ctrl Pts',(5.58910503477557,-5.9063759593944,46.1594931154483));
#177084=CARTESIAN_POINT('Ctrl Pts',(5.05323131775854,-6.37466652749516,
46.1307515848629));
#177085=CARTESIAN_POINT('Ctrl Pts',(4.74177109018703,-6.60962220355473,
46.1146780262004));
#177086=CARTESIAN_POINT('Ctrl Pts',(4.22328341220484,-6.94518070483189,
46.0887254352519));
#177087=CARTESIAN_POINT('Ctrl Pts',(4.02677134496226,-7.06093255776235,
46.0790649838876));
#177088=CARTESIAN_POINT('Ctrl Pts',(3.58504144300756,-7.29668077770954,
46.0578742679747));
#177089=CARTESIAN_POINT('Ctrl Pts',(3.33810983977917,-7.41290098746993,
46.0463600053154));
#177090=CARTESIAN_POINT('Ctrl Pts',(2.96889379203362,-7.56447798537479,
46.0299487237922));
#177091=CARTESIAN_POINT('Ctrl Pts',(2.85088241532768,-7.6097390692465,46.0248204765168));
#177092=CARTESIAN_POINT('Ctrl Pts',(2.71176121135175,-7.65940560144486,
46.0189464140556));
#177093=CARTESIAN_POINT('Ctrl Pts',(2.69163353955806,-7.66650193594872,
46.0181007308151));
#177094=CARTESIAN_POINT('Ctrl Pts',(2.66232836974136,-7.67670431091013,
46.0168757190071));
#177095=CARTESIAN_POINT('Ctrl Pts',(2.6531729943345,-7.67987333805801,46.016493894785));
#177096=CARTESIAN_POINT('Ctrl Pts',(2.63713778230002,-7.68539164455165,
46.0158267272965));
#177097=CARTESIAN_POINT('Ctrl Pts',(2.63026042928107,-7.68774807649121,
46.0155410932482));
#177098=CARTESIAN_POINT('Ctrl Pts',(2.61693347656547,-7.69229439987594,
46.0149885866469));
#177099=CARTESIAN_POINT('Ctrl Pts',(2.6104842696778,-7.69448541705252,46.0147216675835));
#177100=CARTESIAN_POINT('Ctrl Pts',(2.59337811418094,-7.70027298377651,
46.0140148896106));
#177101=CARTESIAN_POINT('Ctrl Pts',(2.58271641696357,-7.70385552687754,
46.0135756220414));
#177102=CARTESIAN_POINT('Ctrl Pts',(2.54499834494907,-7.7164424516538,46.0120260971338));
#177103=CARTESIAN_POINT('Ctrl Pts',(2.51790183900885,-7.72532659781437,
46.0109210629608));
#177104=CARTESIAN_POINT('Ctrl Pts',(2.06627088260679,-7.87077448163264,
45.9926448166083));
#177105=CARTESIAN_POINT('Ctrl Pts',(1.6312345633962,-7.97230598977856,45.977250272847));
#177106=CARTESIAN_POINT('Ctrl Pts',(0.951560163103997,-8.07293937603262,
45.9541233936049));
#177107=CARTESIAN_POINT('Ctrl Pts',(0.711605282612934,-8.0976191636857,
45.9461308768391));
#177108=CARTESIAN_POINT('Ctrl Pts',(0.0869932142115497,-8.13388017662535,
45.9252111373475));
#177109=CARTESIAN_POINT('Ctrl Pts',(-0.298005582694259,-8.12888357574144,
45.9121859310117));
#177110=CARTESIAN_POINT('Ctrl Pts',(-0.806047737852952,-8.08614091774465,
45.8939740572312));
#177111=CARTESIAN_POINT('Ctrl Pts',(-0.93064487404062,-8.07274963355612,
45.8894277785557));
#177112=CARTESIAN_POINT('Ctrl Pts',(-1.21033957582965,-8.03612765574105,
45.8790098018641));
#177113=CARTESIAN_POINT('Ctrl Pts',(-1.36517191603069,-8.01127780957283,
45.8730940842373));
#177114=CARTESIAN_POINT('Ctrl Pts',(-1.54198906310983,-7.97762472193629,
45.866145295766));
#177115=CARTESIAN_POINT('Ctrl Pts',(-1.56477535075435,-7.97318660046487,
45.8652461221294));
#177116=CARTESIAN_POINT('Ctrl Pts',(-1.59922863863991,-7.966322697293,45.8638809043011));
#177117=CARTESIAN_POINT('Ctrl Pts',(-1.6109099166797,-7.96396878415137,
45.863417046909));
#177118=CARTESIAN_POINT('Ctrl Pts',(-1.63109493542001,-7.95985504166606,
45.8626137985644));
#177119=CARTESIAN_POINT('Ctrl Pts',(-1.63960112481182,-7.95810725761027,
45.8622747747221));
#177120=CARTESIAN_POINT('Ctrl Pts',(-1.65721164054363,-7.95445935561626,
45.8615717937013));
#177121=CARTESIAN_POINT('Ctrl Pts',(-1.66631553719116,-7.95255723598064,
45.861207775972));
#177122=CARTESIAN_POINT('Ctrl Pts',(-1.69105450889051,-7.94734406133373,
45.8602169383449));
#177123=CARTESIAN_POINT('Ctrl Pts',(-1.7066830758271,-7.94400250858541,
45.8595891903008));
#177124=CARTESIAN_POINT('Ctrl Pts',(-1.76535837372883,-7.93127596754589,
45.8572256012656));
#177125=CARTESIAN_POINT('Ctrl Pts',(-1.8083380212938,-7.92158710028727,
45.8554805117701));
#177126=CARTESIAN_POINT('Ctrl Pts',(-2.52960066047031,-7.75281767647352,
45.8259606724177));
#177127=CARTESIAN_POINT('Ctrl Pts',(-3.18463676915089,-7.50752101775611,
45.7953227894909));
#177128=CARTESIAN_POINT('Ctrl Pts',(-4.17441324213938,-6.98377828490047,
45.745028943772));
#177129=CARTESIAN_POINT('Ctrl Pts',(-4.53254600500595,-6.75684391358903,
45.7259416974196));
#177130=CARTESIAN_POINT('Ctrl Pts',(-4.96828512188053,-6.43043485913772,
45.7027486366266));
#177131=CARTESIAN_POINT('Ctrl Pts',(-5.06356531824567,-6.35567918774564,
45.6976813709935));
#177132=CARTESIAN_POINT('Ctrl Pts',(-5.2078560671055,-6.23716519663319,
45.6900550319017));
#177133=CARTESIAN_POINT('Ctrl Pts',(-5.25806279163667,-6.19489872400199,
45.6874118741333));
#177134=CARTESIAN_POINT('Ctrl Pts',(-5.31861179395697,-6.14265918378931,
45.6842314930712));
#177135=CARTESIAN_POINT('Ctrl Pts',(-5.32944625192273,-6.13326144188078,
45.6836626784716));
#177136=CARTESIAN_POINT('Ctrl Pts',(-5.3469881773048,-6.11796410471686,
45.6827420695414));
#177137=CARTESIAN_POINT('Ctrl Pts',(-5.35371086910122,-6.11208207452541,
45.6823893434816));
#177138=CARTESIAN_POINT('Ctrl Pts',(-5.36599298429608,-6.10130000671119,
45.681745054542));
#177139=CARTESIAN_POINT('Ctrl Pts',(-5.37155542465681,-6.09640343150863,
45.6814533114156));
#177140=CARTESIAN_POINT('Ctrl Pts',(-5.38371780423885,-6.08566740996543,
45.6808154987705));
#177141=CARTESIAN_POINT('Ctrl Pts',(-5.3903149628298,-6.07982481841757,
45.6804695919525));
#177142=CARTESIAN_POINT('Ctrl Pts',(-5.40840198695145,-6.06375396461244,
45.6795213627768));
#177143=CARTESIAN_POINT('Ctrl Pts',(-5.41987236313527,-6.053503759563,45.6789201534425));
#177144=CARTESIAN_POINT('Ctrl Pts',(-5.47654511129033,-6.00256942036892,
45.6759500318758));
#177145=CARTESIAN_POINT('Ctrl Pts',(-5.52131947526164,-5.9614106947656,
45.6736045147556));
#177146=CARTESIAN_POINT('Ctrl Pts',(-6.00117080475262,-5.51026446347943,
45.6484327917287));
#177147=CARTESIAN_POINT('Ctrl Pts',(-6.39022140888337,-5.05393303340372,
45.6275606749244));
#177148=CARTESIAN_POINT('Ctrl Pts',(-6.97133207312041,-4.19664947714925,
45.5901382393326));
#177149=CARTESIAN_POINT('Ctrl Pts',(-7.18726695421699,-3.8150367556271,
45.5740219014664));
#177150=CARTESIAN_POINT('Ctrl Pts',(-7.39631084374373,-3.36419061593246,
45.5550296700606));
#177151=CARTESIAN_POINT('Ctrl Pts',(-7.4206268995964,-3.31020980121936,
45.552757459196));
#177152=CARTESIAN_POINT('Ctrl Pts',(-7.45810354760932,-3.22452429177211,
45.5491531704004));
#177153=CARTESIAN_POINT('Ctrl Pts',(-7.4716569826887,-3.19299347819154,
45.547827379621));
#177154=CARTESIAN_POINT('Ctrl Pts',(-7.4943258370972,-3.13932175199636,
45.5455715045057));
#177155=CARTESIAN_POINT('Ctrl Pts',(-7.50354392024658,-3.11722463846776,
45.5446429947826));
#177156=CARTESIAN_POINT('Ctrl Pts',(-7.52155028395054,-3.07351802965036,
45.5428069768942));
#177157=CARTESIAN_POINT('Ctrl Pts',(-7.53034343937526,-3.05191078388361,
45.541899550129));
#177158=CARTESIAN_POINT('Ctrl Pts',(-7.53906851689393,-3.03020353517938,
45.5409881811403));
#177159=CARTESIAN_POINT('Ctrl Pts',(-7.53909363080346,-3.03014105166963,
45.5409855578006));
#177160=CARTESIAN_POINT('Ctrl Pts',(-7.53914408064139,-3.03001552775656,
45.5409802877447));
#177161=CARTESIAN_POINT('Ctrl Pts',(-7.53916941659177,-3.02995248725839,
45.5409776410244));
#177162=CARTESIAN_POINT('Ctrl Pts',(-7.53922031114152,-3.0298258476799,
45.5409723241366));
#177163=CARTESIAN_POINT('Ctrl Pts',(-7.53924586976819,-3.02976224849103,
45.5409696539645));
#177164=CARTESIAN_POINT('Ctrl Pts',(-7.53929721060149,-3.02963448909234,
45.5409642900706));
#177165=CARTESIAN_POINT('Ctrl Pts',(-7.53932299267492,-3.02957032917286,
45.5409615963611));
#177166=CARTESIAN_POINT('Ctrl Pts',(-7.53937478087994,-3.02944144699925,
45.5409561853373));
#177167=CARTESIAN_POINT('Ctrl Pts',(-7.53940078701182,-3.02937672470275,
45.5409534680213));
#177168=CARTESIAN_POINT('Ctrl Pts',(-7.53945302395908,-3.02924671609373,
45.5409480097142));
#177169=CARTESIAN_POINT('Ctrl Pts',(-7.53947925478269,-3.02918142971857,
45.5409452687204));
#177170=CARTESIAN_POINT('Ctrl Pts',(-7.53953193019778,-3.02905031999472,
45.5409397641933));
#177171=CARTESIAN_POINT('Ctrl Pts',(-7.5395583748154,-3.02898449654486,
45.5409370006561));
#177172=CARTESIAN_POINT('Ctrl Pts',(-7.53961153635078,-3.02885216683859,
45.5409314449186));
#177173=CARTESIAN_POINT('Ctrl Pts',(-7.53963821879948,-3.02878574634356,
45.5409286563194));
#177174=CARTESIAN_POINT('Ctrl Pts',(-7.53969180895005,-3.02865233953581,
45.5409230553705));
#177175=CARTESIAN_POINT('Ctrl Pts',(-7.53971871790345,-3.02858535006354,
45.5409202428882));
#177176=CARTESIAN_POINT('Ctrl Pts',(-7.53977276148186,-3.02845080412888,
45.5409145941242));
#177177=CARTESIAN_POINT('Ctrl Pts',(-7.53979989743318,-3.02838324432005,
45.540911757702));
#177178=CARTESIAN_POINT('Ctrl Pts',(-7.53985439568391,-3.02824755589569,
45.5409060609818));
#177179=CARTESIAN_POINT('Ctrl Pts',(-7.53988175919209,-3.02817942422567,
45.5409032005557));
#177180=CARTESIAN_POINT('Ctrl Pts',(-7.53993671313527,-3.02804259050424,
45.5408974557618));
#177181=CARTESIAN_POINT('Ctrl Pts',(-7.53996430472478,-3.02797388553272,
45.5408945712714));
#177182=CARTESIAN_POINT('Ctrl Pts',(-7.54001972393283,-3.02783588240704,
45.540888777392));
#177183=CARTESIAN_POINT('Ctrl Pts',(-7.54004755267668,-3.02776658139969,
45.5408858678827));
#177184=CARTESIAN_POINT('Ctrl Pts',(-7.54010885584952,-3.02761391404568,
45.5408794583566));
#177185=CARTESIAN_POINT('Ctrl Pts',(-7.54014235661827,-3.02753048085637,
45.5408759555342));
#177186=CARTESIAN_POINT('Ctrl Pts',(-7.54021050534136,-3.02736074928107,
45.540868829606));
#177187=CARTESIAN_POINT('Ctrl Pts',(-7.54024515321194,-3.02727445082401,
45.5408652064975));
#177188=CARTESIAN_POINT('Ctrl Pts',(-7.54031562566087,-3.02709891433387,
45.5408578368753));
#177189=CARTESIAN_POINT('Ctrl Pts',(-7.5403514501167,-3.02700967630925,
45.5408540903622));
#177190=CARTESIAN_POINT('Ctrl Pts',(-7.54042430538776,-3.02682818592322,
45.5408464707928));
#177191=CARTESIAN_POINT('Ctrl Pts',(-7.54046133604598,-3.02673593363831,
45.5408425977401));
#177192=CARTESIAN_POINT('Ctrl Pts',(-7.54053663329123,-3.02654834011407,
45.5408347219597));
#177193=CARTESIAN_POINT('Ctrl Pts',(-7.54057489978158,-3.02645299878228,
45.5408307192285));
#177194=CARTESIAN_POINT('Ctrl Pts',(-7.540652698301,-3.02625915238135,45.5408225809526));
#177195=CARTESIAN_POINT('Ctrl Pts',(-7.5406922302526,-3.02616064715243,
45.5408184454014));
#177196=CARTESIAN_POINT('Ctrl Pts',(-7.54077258936141,-3.02596039796529,
45.5408100383383));
#177197=CARTESIAN_POINT('Ctrl Pts',(-7.54081341638606,-3.02585865396432,
45.5408057668248));
#177198=CARTESIAN_POINT('Ctrl Pts',(-7.54089639528232,-3.02565185223482,
45.5407970846893));
#177199=CARTESIAN_POINT('Ctrl Pts',(-7.54093854695903,-3.02554679459784,
45.5407926740715));
#177200=CARTESIAN_POINT('Ctrl Pts',(-7.5491502900155,-3.0050788427179,45.5399333725441));
#177201=CARTESIAN_POINT('Ctrl Pts',(-7.55723736107177,-2.98468296767218,
45.5390773367234));
#177202=CARTESIAN_POINT('Ctrl Pts',(-7.57535143104456,-2.93845302631693,
45.5371374191445));
#177203=CARTESIAN_POINT('Ctrl Pts',(-7.58532906588683,-2.91259994601593,
45.5360528387105));
#177204=CARTESIAN_POINT('Ctrl Pts',(-7.61444622904872,-2.83598990586738,
45.5328393192778));
#177205=CARTESIAN_POINT('Ctrl Pts',(-7.63320985289154,-2.7850919906294,
45.53070484145));
#177206=CARTESIAN_POINT('Ctrl Pts',(-7.80497507508968,-2.30438600085963,
45.5105417701189));
#177207=CARTESIAN_POINT('Ctrl Pts',(-7.92202125832042,-1.86262356676084,
45.4919151453754));
#177208=CARTESIAN_POINT('Ctrl Pts',(-8.0440196866528,-1.17197978190414,
45.4624982583085));
#177209=CARTESIAN_POINT('Ctrl Pts',(-8.07571645024059,-0.928757313290472,
45.4520980391277));
#177210=CARTESIAN_POINT('Ctrl Pts',(-8.12970213534692,-0.290186252796987,
45.4249028951722));
#177211=CARTESIAN_POINT('Ctrl Pts',(-8.13418974339782,0.106027200574754,
45.4081196394064));
#177212=CARTESIAN_POINT('Ctrl Pts',(-8.10666456771426,0.551584987354708,
45.3901266501115));
#177213=CARTESIAN_POINT('Ctrl Pts',(-8.1030661332201,0.602142656589539,
45.3880983345551));
#177214=CARTESIAN_POINT('Ctrl Pts',(-8.09787649840437,0.66654153460252,
45.3855341621121));
#177215=CARTESIAN_POINT('Ctrl Pts',(-8.09672249047119,0.680416281329202,
45.3849828626505));
#177216=CARTESIAN_POINT('Ctrl Pts',(-8.0948154706107,0.702652501605304,
45.3841012392303));
#177217=CARTESIAN_POINT('Ctrl Pts',(-8.09408515436585,0.711015861822725,
45.383770081619));
#177218=CARTESIAN_POINT('Ctrl Pts',(-8.09267600877235,0.72686941246166,
45.3831431795118));
#177219=CARTESIAN_POINT('Ctrl Pts',(-8.09199973945508,0.734359818384843,
45.3828473391157));
#177220=CARTESIAN_POINT('Ctrl Pts',(-8.09044330900325,0.751335727411188,
45.3821776798022));
#177221=CARTESIAN_POINT('Ctrl Pts',(-8.08955686338025,0.760820653363481,
45.3818041022267));
#177222=CARTESIAN_POINT('Ctrl Pts',(-8.08689442566711,0.788777844420601,
45.3807047171814));
#177223=CARTESIAN_POINT('Ctrl Pts',(-8.08507182116498,0.807245683606145,
45.3799807425165));
#177224=CARTESIAN_POINT('Ctrl Pts',(-8.07085962259609,0.946374713739244,
45.3745443357744));
#177225=CARTESIAN_POINT('Ctrl Pts',(-8.05583420975066,1.06674096627667,
45.3699504409275));
#177226=CARTESIAN_POINT('Ctrl Pts',(-8.03641889366127,1.19824630978568,
45.3650373395693));
#177227=CARTESIAN_POINT('Ctrl Pts',(-8.03469534084682,1.20974941000309,
45.3646084182519));
#177228=CARTESIAN_POINT('Ctrl Pts',(-8.0277410386084,1.25549237527572,45.3629060046652));
#177229=CARTESIAN_POINT('Ctrl Pts',(-8.02231603376223,1.28970259457657,
45.3616399963894));
#177230=CARTESIAN_POINT('Ctrl Pts',(-8.00039206781983,1.42246206109011,
45.3567519599135));
#177231=CARTESIAN_POINT('Ctrl Pts',(-7.98229427654372,1.52074009796005,
45.3531869732088));
#177232=CARTESIAN_POINT('Ctrl Pts',(-7.83294448115052,2.2554096044385,45.3268019615254));
#177233=CARTESIAN_POINT('Ctrl Pts',(-7.62758768314559,2.87434716211447,
45.3059136198857));
#177234=CARTESIAN_POINT('Ctrl Pts',(-7.18360442274106,3.81697195364983,
45.2697024173584));
#177235=CARTESIAN_POINT('Ctrl Pts',(-6.991072983905,4.15912352909268,45.255540693643));
#177236=CARTESIAN_POINT('Ctrl Pts',(-6.7535741850353,4.51778422284777,45.2390338878057));
#177237=CARTESIAN_POINT('Ctrl Pts',(-6.73232038208992,4.54939565037014,
45.2375643656091));
#177238=CARTESIAN_POINT('Ctrl Pts',(-6.70262734549773,4.59289524179344,
45.2355215356989));
#177239=CARTESIAN_POINT('Ctrl Pts',(-6.6943770870959,4.60491209990383,45.2349550010346));
#177240=CARTESIAN_POINT('Ctrl Pts',(-6.68039415329947,4.62516185252005,
45.233996589977));
#177241=CARTESIAN_POINT('Ctrl Pts',(-6.67467847251796,4.63340646750193,
45.233605325962));
#177242=CARTESIAN_POINT('Ctrl Pts',(-6.66333719892671,4.64970121488785,
45.2328299396103));
#177243=CARTESIAN_POINT('Ctrl Pts',(-6.65771225028756,4.65775177589896,
45.2324458408619));
#177244=CARTESIAN_POINT('Ctrl Pts',(-6.64528126898984,4.67547476695927,
45.2315980217185));
#177245=CARTESIAN_POINT('Ctrl Pts',(-6.63846869124513,4.68514256713675,
45.2311340644658));
#177246=CARTESIAN_POINT('Ctrl Pts',(-6.61459166362652,4.71887007143144,
45.2295103000987));
#177247=CARTESIAN_POINT('Ctrl Pts',(-6.59741742187913,4.74285156492032,
45.2283465016564));
#177248=CARTESIAN_POINT('Ctrl Pts',(-6.41718535115487,4.9916479521449,45.2161753308082));
#177249=CARTESIAN_POINT('Ctrl Pts',(-6.242845461206,5.20803985701046,45.2047491767878));
#177250=CARTESIAN_POINT('Ctrl Pts',(-5.97721703900751,5.50519544344796,
45.1878086820734));
#177251=CARTESIAN_POINT('Ctrl Pts',(-5.89465495528056,5.59350892050967,
45.182602900367));
#177252=CARTESIAN_POINT('Ctrl Pts',(-5.42941418854369,6.06941506633686,
45.153622969414));
#177253=CARTESIAN_POINT('Ctrl Pts',(-5.01048674582911,6.41960287061624,
45.1287035164661));
#177254=CARTESIAN_POINT('Ctrl Pts',(-4.24805436883545,6.93653458664437,
45.0875440716594));
#177255=CARTESIAN_POINT('Ctrl Pts',(-3.92204468498437,7.12594497405542,
45.0710824623263));
#177256=CARTESIAN_POINT('Ctrl Pts',(-3.54042037364813,7.31351313601746,
45.0538769648425));
#177257=CARTESIAN_POINT('Ctrl Pts',(-3.49660021335185,7.33456459657802,
45.051931136617));
#177258=CARTESIAN_POINT('Ctrl Pts',(-3.44052797024926,7.36088530685993,
45.049475902821));
#177259=CARTESIAN_POINT('Ctrl Pts',(-3.42844852594054,7.36651925421631,
45.0489490146779));
#177260=CARTESIAN_POINT('Ctrl Pts',(-3.4090694708078,7.37549980594561,45.0481069013155));
#177261=CARTESIAN_POINT('Ctrl Pts',(-3.40177869902302,7.37886534148689,
45.0477908001003));
#177262=CARTESIAN_POINT('Ctrl Pts',(-3.38795125511701,7.38522345894802,
45.0471926312692));
#177263=CARTESIAN_POINT('Ctrl Pts',(-3.38141558069347,7.38821818280482,
45.0469104667181));
#177264=CARTESIAN_POINT('Ctrl Pts',(-3.36659825835626,7.39498387657562,
45.0462720215924));
#177265=CARTESIAN_POINT('Ctrl Pts',(-3.35831422474455,7.39874961981613,
45.0459159736402));
#177266=CARTESIAN_POINT('Ctrl Pts',(-3.33698435895785,7.40840251348089,
45.0450014683825));
#177267=CARTESIAN_POINT('Ctrl Pts',(-3.32392923518722,7.41426913838569,
45.0444439022422));
#177268=CARTESIAN_POINT('Ctrl Pts',(-3.2468858711594,7.44864598547684,45.0411658633859));
#177269=CARTESIAN_POINT('Ctrl Pts',(-3.18254548809281,7.4763627140695,45.0384785198737));
#177270=CARTESIAN_POINT('Ctrl Pts',(-2.44331803344873,7.7835369077003,45.0080920308414));
#177271=CARTESIAN_POINT('Ctrl Pts',(-1.73401533819079,7.97161566454119,
44.9831039707371));
#177272=CARTESIAN_POINT('Ctrl Pts',(-0.712458494096431,8.09947202621859,
44.9453992624519));
#177273=CARTESIAN_POINT('Ctrl Pts',(-0.414033940448249,8.12019772104746,
44.9342518477751));
#177274=CARTESIAN_POINT('Ctrl Pts',(0.0822609033961705,8.12723205720843,
44.9154013165454));
#177275=CARTESIAN_POINT('Ctrl Pts',(0.279709784340779,8.12283374114866,
44.9078264745174));
#177276=CARTESIAN_POINT('Ctrl Pts',(0.609571087942919,8.10344372815655,
44.8950799401636));
#177277=CARTESIAN_POINT('Ctrl Pts',(0.742131558063892,8.09238020800831,
44.8899287518685));
#177278=CARTESIAN_POINT('Ctrl Pts',(0.927038347820043,8.07236613493958,
44.8826877445129));
#177279=CARTESIAN_POINT('Ctrl Pts',(0.979659804493552,8.06614912752745,
44.8806207634749));
#177280=CARTESIAN_POINT('Ctrl Pts',(1.07025126604122,8.05454655223554,44.8770504252935));
#177281=CARTESIAN_POINT('Ctrl Pts',(1.10825096604494,8.04940604747869,44.8755491880151));
#177282=CARTESIAN_POINT('Ctrl Pts',(1.18116793908095,8.03901589347521,44.8726611590434));
#177283=CARTESIAN_POINT('Ctrl Pts',(1.21609019998089,8.03380724504245,44.8712747511448));
#177284=CARTESIAN_POINT('Ctrl Pts',(1.3079946995373,8.01948672563891,44.8676172489392));
#177285=CARTESIAN_POINT('Ctrl Pts',(1.3649156022477,8.00999518273489,44.8653429331886));
#177286=CARTESIAN_POINT('Ctrl Pts',(1.57085445535829,7.97339602694035,44.8570797287275));
#177287=CARTESIAN_POINT('Ctrl Pts',(1.71920691171149,7.94272967368668,44.8510605860194));
#177288=CARTESIAN_POINT('Ctrl Pts',(2.35131172397897,7.79352565555383,44.8251008319314));
#177289=CARTESIAN_POINT('Ctrl Pts',(2.82445890418429,7.63479694414776,44.8048301902614));
#177290=CARTESIAN_POINT('Ctrl Pts',(3.30695751754261,7.42189886193524,44.7834265270393));
#177291=CARTESIAN_POINT('Ctrl Pts',(3.33377254799363,7.40989280225078,44.7822346758421));
#177292=CARTESIAN_POINT('Ctrl Pts',(3.5218987488572,7.32443398875131,44.7738572087877));
#177293=CARTESIAN_POINT('Ctrl Pts',(3.68083531292024,7.2458647991905,44.7666970574187));
#177294=CARTESIAN_POINT('Ctrl Pts',(3.8952686160866,7.13098368279333,44.7569561587073));
#177295=CARTESIAN_POINT('Ctrl Pts',(3.95307928976165,7.09909924649732,44.7543218199998));
#177296=CARTESIAN_POINT('Ctrl Pts',(4.05248077617866,7.04268540303238,44.7497805730705));
#177297=CARTESIAN_POINT('Ctrl Pts',(4.09425328211408,7.01848332897948,44.7478685277292));
#177298=CARTESIAN_POINT('Ctrl Pts',(4.15512191629435,6.98248901915033,44.7450779768425));
#177299=CARTESIAN_POINT('Ctrl Pts',(4.17438867873645,6.97098774985198,44.744194030144));
#177300=CARTESIAN_POINT('Ctrl Pts',(4.20946027062326,6.94985426818393,44.7425838799892));
#177301=CARTESIAN_POINT('Ctrl Pts',(4.22528025939768,6.94024760736314,44.7418571582128));
#177302=CARTESIAN_POINT('Ctrl Pts',(4.26077861781979,6.91852492661886,44.7402253075828));
#177303=CARTESIAN_POINT('Ctrl Pts',(4.2804384178785,6.90637883021331,44.7393207420655));
#177304=CARTESIAN_POINT('Ctrl Pts',(4.33108051684267,6.8747921377427,44.7369880785158));
#177305=CARTESIAN_POINT('Ctrl Pts',(4.36198390488628,6.85522587610914,44.7355621098359));
#177306=CARTESIAN_POINT('Ctrl Pts',(4.58181546129759,6.71395269309282,44.7253954249804));
#177307=CARTESIAN_POINT('Ctrl Pts',(4.765756592046,6.58466096047464,44.7167626730908));
#177308=CARTESIAN_POINT('Ctrl Pts',(5.12668048785489,6.3079131543629,44.6992800782621));
#177309=CARTESIAN_POINT('Ctrl Pts',(5.30322850355997,6.16022626206441,44.6904374838974));
#177310=CARTESIAN_POINT('Ctrl Pts',(5.52648635794501,5.95674579546528,44.6787315525291));
#177311=CARTESIAN_POINT('Ctrl Pts',(5.5790551078985,5.90753890917359,44.6759350755949));
#177312=CARTESIAN_POINT('Ctrl Pts',(5.65994973397002,5.82977472070196,44.6715653994652));
#177313=CARTESIAN_POINT('Ctrl Pts',(5.6887294563797,5.80169470438309,44.6699973698012));
#177314=CARTESIAN_POINT('Ctrl Pts',(5.74224262745843,5.74870154523371,44.6670559263607));
#177315=CARTESIAN_POINT('Ctrl Pts',(5.76702536670895,5.72383946827723,44.66568310852));
#177316=CARTESIAN_POINT('Ctrl Pts',(5.82263150179234,5.66732755997899,44.6625784607601));
#177317=CARTESIAN_POINT('Ctrl Pts',(5.85335941919497,5.63558539706276,44.6608456116069));
#177318=CARTESIAN_POINT('Ctrl Pts',(5.94787501936967,5.53634312551023,44.6554610279046));
#177319=CARTESIAN_POINT('Ctrl Pts',(6.01076511112856,5.46799918161962,44.6517997115051));
#177320=CARTESIAN_POINT('Ctrl Pts',(6.19955859871954,5.25563963057183,44.6405614512073));
#177321=CARTESIAN_POINT('Ctrl Pts',(6.32155909416401,5.10824473013339,44.632948244177));
#177322=CARTESIAN_POINT('Ctrl Pts',(6.56778108748063,4.78842662361782,44.6168372472003));
#177323=CARTESIAN_POINT('Ctrl Pts',(6.6906733655091,4.61515634978962,44.608340014486));
#177324=CARTESIAN_POINT('Ctrl Pts',(6.86061903507362,4.35446494656249,44.5959635610578));
#177325=CARTESIAN_POINT('Ctrl Pts',(6.91308570474049,4.27067966809851,44.5920451139746));
#177326=CARTESIAN_POINT('Ctrl Pts',(6.97896116666159,4.1610852830678,44.5870060102031));
#177327=CARTESIAN_POINT('Ctrl Pts',(6.99377813402844,4.13613311204955,44.5858644220904));
#177328=CARTESIAN_POINT('Ctrl Pts',(7.01850027108073,4.09398768829716,44.5839461880536));
#177329=CARTESIAN_POINT('Ctrl Pts',(7.02847668828978,4.07683660354645,44.5831683248027));
#177330=CARTESIAN_POINT('Ctrl Pts',(7.04788451219962,4.04318841533717,44.5816474740091));
#177331=CARTESIAN_POINT('Ctrl Pts',(7.05732106851708,4.02669442567495,44.5809044070354));
#177332=CARTESIAN_POINT('Ctrl Pts',(7.08007106588813,3.98660447898564,44.5791040313858));
#177333=CARTESIAN_POINT('Ctrl Pts',(7.09332453617936,3.96297471622389,44.578047629301));
#177334=CARTESIAN_POINT('Ctrl Pts',(7.14408116358562,3.87140975788872,44.573971594418));
#177335=CARTESIAN_POINT('Ctrl Pts',(7.18072874295299,3.80300460682597,44.5709635611151));
#177336=CARTESIAN_POINT('Ctrl Pts',(7.41007777652969,3.35977086776508,44.5516760744117));
#177337=CARTESIAN_POINT('Ctrl Pts',(7.57434875249141,2.97095255935598,44.5356505910524));
#177338=CARTESIAN_POINT('Ctrl Pts',(7.77141585486654,2.38019025982771,44.5116677081881));
#177339=CARTESIAN_POINT('Ctrl Pts',(7.82799672897575,2.18693301614099,44.5038827246096));
#177340=CARTESIAN_POINT('Ctrl Pts',(7.8954304854544,1.92023697181414,44.4931762732301));
#177341=CARTESIAN_POINT('Ctrl Pts',(7.91254358578328,1.84845516938181,44.4902984279291));
#177342=CARTESIAN_POINT('Ctrl Pts',(7.9407035610943,1.7227712067595,44.4852647755205));
#177343=CARTESIAN_POINT('Ctrl Pts',(7.95218513525367,1.66897130712437,44.4831117497081));
#177344=CARTESIAN_POINT('Ctrl Pts',(7.97553790769001,1.55382944139232,44.4785070305282));
#177345=CARTESIAN_POINT('Ctrl Pts',(7.987249697207,1.49245873970389,44.4760546117448));
#177346=CARTESIAN_POINT('Ctrl Pts',(8.0225000196189,1.2954293794884,44.4681870697772));
#177347=CARTESIAN_POINT('Ctrl Pts',(8.04329871172858,1.15930558064328,44.4627601131665));
#177348=CARTESIAN_POINT('Ctrl Pts',(8.0760634814595,0.901068015869555,44.4524869881328));
#177349=CARTESIAN_POINT('Ctrl Pts',(8.08874250723559,0.779082527618561,
44.4476435785835));
#177350=CARTESIAN_POINT('Ctrl Pts',(8.10413182001569,0.589341440954557,
44.4401333083677));
#177351=CARTESIAN_POINT('Ctrl Pts',(8.10876331086594,0.521759993070642,
44.4374629606468));
#177352=CARTESIAN_POINT('Ctrl Pts',(8.11550502768295,0.401325983249336,
44.4327149325259));
#177353=CARTESIAN_POINT('Ctrl Pts',(8.11794525130967,0.348495798446415,
44.4306357991851));
#177354=CARTESIAN_POINT('Ctrl Pts',(8.12132811894089,0.255585713392512,
44.4269871001163));
#177355=CARTESIAN_POINT('Ctrl Pts',(8.12249022303476,0.215515792835325,
44.42541620068));
#177356=CARTESIAN_POINT('Ctrl Pts',(8.12461687105055,0.117045429389527,
44.421561277003));
#177357=CARTESIAN_POINT('Ctrl Pts',(8.12524832282328,0.0586400636367198,
44.4192794311841));
#177358=CARTESIAN_POINT('Ctrl Pts',(8.12525491974489,-0.171553006934017,
44.410296314558));
#177359=CARTESIAN_POINT('Ctrl Pts',(8.11981193981901,-0.343296123938928,
44.4036160078732));
#177360=CARTESIAN_POINT('Ctrl Pts',(8.10033598238096,-0.650111030153366,
44.3916430139931));
#177361=CARTESIAN_POINT('Ctrl Pts',(8.08835417673415,-0.78524766315252,
44.3863561626108));
#177362=CARTESIAN_POINT('Ctrl Pts',(8.06596022829843,-0.981750063222547,
44.3786252009258));
#177363=CARTESIAN_POINT('Ctrl Pts',(8.05821758982036,-1.04339677695893,
44.3761936553276));
#177364=CARTESIAN_POINT('Ctrl Pts',(8.04227813131998,-1.15951889108442,
44.3715993920579));
#177365=CARTESIAN_POINT('Ctrl Pts',(8.03423284598387,-1.2140115943198,44.3694375866352));
#177366=CARTESIAN_POINT('Ctrl Pts',(8.01401510338441,-1.34193486943712,
44.3643472006735));
#177367=CARTESIAN_POINT('Ctrl Pts',(8.00138653255227,-1.4152882248396,44.3614162290669));
#177368=CARTESIAN_POINT('Ctrl Pts',(7.94969598499687,-1.69268363622646,
44.3502812531698));
#177369=CARTESIAN_POINT('Ctrl Pts',(7.90382202973324,-1.89537332521706,
44.3420377557613));
#177370=CARTESIAN_POINT('Ctrl Pts',(7.79383566644714,-2.30729384807574,
44.325038503748));
#177371=CARTESIAN_POINT('Ctrl Pts',(7.72893873707275,-2.51614478645766,
44.3162852211738));
#177372=CARTESIAN_POINT('Ctrl Pts',(7.64671444242232,-2.74739241303451,
44.3064612791299));
#177373=CARTESIAN_POINT('Ctrl Pts',(7.63760438971574,-2.77261717916063,
44.3053879175072));
#177374=CARTESIAN_POINT('Ctrl Pts',(7.62689254112645,-2.80182371496526,
44.3041431628281));
#177375=CARTESIAN_POINT('Ctrl Pts',(7.62541228004832,-2.80584987533635,
44.3039715283971));
#177376=CARTESIAN_POINT('Ctrl Pts',(7.55279043406486,-3.00289202582133,
44.2955695528571));
#177377=CARTESIAN_POINT('Ctrl Pts',(7.47434704800034,-3.19313975625692,
44.2873564015562));
#177378=CARTESIAN_POINT('Ctrl Pts',(7.37020801602888,-3.42077648508081,
44.2774576128583));
#177379=CARTESIAN_POINT('Ctrl Pts',(7.35131418261996,-3.46119311497737,
44.2756973656458));
#177380=CARTESIAN_POINT('Ctrl Pts',(7.32087766773431,-3.52492758916795,
44.2729181437735));
#177381=CARTESIAN_POINT('Ctrl Pts',(7.30955425994735,-3.54834903336843,
44.2718960850059));
#177382=CARTESIAN_POINT('Ctrl Pts',(7.28936547854264,-3.5896009498445,44.2700948542616));
#177383=CARTESIAN_POINT('Ctrl Pts',(7.28054668615404,-3.60745395161059,
44.2693149550847));
#177384=CARTESIAN_POINT('Ctrl Pts',(7.26187857555311,-3.64489889565543,
44.2676785468383));
#177385=CARTESIAN_POINT('Ctrl Pts',(7.25201542904595,-3.66448367805545,
44.2668223161907));
#177386=CARTESIAN_POINT('Ctrl Pts',(7.22231308479321,-3.72287262706274,
44.264268424304));
#177387=CARTESIAN_POINT('Ctrl Pts',(7.20224081943805,-3.76155740398518,
44.2625747104102));
#177388=CARTESIAN_POINT('Ctrl Pts',(7.09661686954593,-3.96117857944336,
44.2538199189667));
#177389=CARTESIAN_POINT('Ctrl Pts',(7.00597820713182,-4.11936614395862,
44.2468304139154));
#177390=CARTESIAN_POINT('Ctrl Pts',(6.73024944483812,-4.56511859569667,
44.2267619975062));
#177391=CARTESIAN_POINT('Ctrl Pts',(6.53223439153364,-4.84422097220849,
44.2137151685589));
#177392=CARTESIAN_POINT('Ctrl Pts',(6.27669275257601,-5.16013278170267,
44.1979691883851));
#177393=CARTESIAN_POINT('Ctrl Pts',(6.23556078490337,-5.20976236227084,
44.195465505402));
#177394=CARTESIAN_POINT('Ctrl Pts',(6.16877857623918,-5.288417353187,44.191447282888));
#177395=CARTESIAN_POINT('Ctrl Pts',(6.14350367106949,-5.31775797247312,
44.189936922008));
#177396=CARTESIAN_POINT('Ctrl Pts',(6.09472873888611,-5.37356696079795,
44.1870416611897));
#177397=CARTESIAN_POINT('Ctrl Pts',(6.07126360448104,-5.40006467711225,
44.1856571777615));
#177398=CARTESIAN_POINT('Ctrl Pts',(6.01634083454644,-5.46127503365843,
44.1824357568248));
#177399=CARTESIAN_POINT('Ctrl Pts',(5.98475467598516,-5.49587058385891,
44.1805974177579));
#177400=CARTESIAN_POINT('Ctrl Pts',(5.87763019720732,-5.61118273672971,
44.1744097361266));
#177401=CARTESIAN_POINT('Ctrl Pts',(5.80074461844093,-5.69063001950176,
44.1700457494245));
#177402=CARTESIAN_POINT('Ctrl Pts',(5.59812717404535,-5.89162396064811,
44.1587398292857));
#177403=CARTESIAN_POINT('Ctrl Pts',(5.47005007425579,-6.01072476703551,
44.1517769658818));
#177404=CARTESIAN_POINT('Ctrl Pts',(5.17240468109232,-6.27011160082396,
44.1360318594264));
#177405=CARTESIAN_POINT('Ctrl Pts',(5.0007775741833,-6.40783069546567,44.1272487564396));
#177406=CARTESIAN_POINT('Ctrl Pts',(4.79384480209525,-6.56049715136603,
44.1170763769369));
#177407=CARTESIAN_POINT('Ctrl Pts',(4.76376435824148,-6.58237191409718,
44.1156076896143));
#177408=CARTESIAN_POINT('Ctrl Pts',(4.71460758325386,-6.6176056982552,44.1132245446566));
#177409=CARTESIAN_POINT('Ctrl Pts',(4.69562219348293,-6.63109056359063,
44.1123081903321));
#177410=CARTESIAN_POINT('Ctrl Pts',(4.66143152540633,-6.65515490476045,
44.1106654326722));
#177411=CARTESIAN_POINT('Ctrl Pts',(4.64624755393757,-6.66576434796622,
44.1099385237624));
#177412=CARTESIAN_POINT('Ctrl Pts',(4.6127407961705,-6.68900629439616,44.1083403673681));
#177413=CARTESIAN_POINT('Ctrl Pts',(4.59440217029388,-6.701615593223,44.1074695761782));
#177414=CARTESIAN_POINT('Ctrl Pts',(4.53694925374254,-6.74077248604679,
44.1047533091371));
#177415=CARTESIAN_POINT('Ctrl Pts',(4.49765482980891,-6.76705425670424,
44.1029125610495));
#177416=CARTESIAN_POINT('Ctrl Pts',(4.42874355548889,-6.8122796369159,44.0997121020318));
#177417=CARTESIAN_POINT('Ctrl Pts',(4.3992290443109,-6.83137666671693,44.0983500860251));
#177418=CARTESIAN_POINT('Ctrl Pts',(4.2736831408696,-6.9114586745001,44.0925915281276));
#177419=CARTESIAN_POINT('Ctrl Pts',(4.17649989330501,-6.97061529791405,
44.08822014177));
#177420=CARTESIAN_POINT('Ctrl Pts',(3.64928677856101,-7.27655140765172,
44.0648878450016));
#177421=CARTESIAN_POINT('Ctrl Pts',(3.19859017648461,-7.48562086624576,
44.0462431902046));
#177422=CARTESIAN_POINT('Ctrl Pts',(2.70831348368903,-7.66063573743803,
44.0263297441983));
#177423=CARTESIAN_POINT('Ctrl Pts',(2.68493375579961,-7.66886122917032,
44.0253810849795));
#177424=CARTESIAN_POINT('Ctrl Pts',(2.43999692083465,-7.75377789297895,
44.0154515978058));
#177425=CARTESIAN_POINT('Ctrl Pts',(2.21525949889722,-7.82095131979762,
44.0064163569928));
#177426=CARTESIAN_POINT('Ctrl Pts',(1.92275573253107,-7.89475881853295,
43.9946886352603));
#177427=CARTESIAN_POINT('Ctrl Pts',(1.85737498222384,-7.91039597764122,
43.9920694442624));
#177428=CARTESIAN_POINT('Ctrl Pts',(1.75158962550293,-7.93431292189322,
43.9878339908805));
#177429=CARTESIAN_POINT('Ctrl Pts',(1.71130273932041,-7.9430995637086,43.9862215320902));
#177430=CARTESIAN_POINT('Ctrl Pts',(1.63389254221699,-7.95936660056042,
43.9831240453414));
#177431=CARTESIAN_POINT('Ctrl Pts',(1.59678036329107,-7.96689487707838,
43.9816393970757));
#177432=CARTESIAN_POINT('Ctrl Pts',(1.51060492211509,-7.98374939516942,
43.9781926407273));
#177433=CARTESIAN_POINT('Ctrl Pts',(1.46150563849806,-7.99288326456616,
43.9762292922099));
#177434=CARTESIAN_POINT('Ctrl Pts',(1.30096065853655,-8.02122044401922,
43.9698106284283));
#177435=CARTESIAN_POINT('Ctrl Pts',(1.18919822655473,-8.03854983126021,
43.9653439406352));
#177436=CARTESIAN_POINT('Ctrl Pts',(0.485852237943699,-8.13261799363731,
43.9372409537668));
#177437=CARTESIAN_POINT('Ctrl Pts',(-0.112287566390233,-8.14634140401478,
43.9133683576055));
#177438=CARTESIAN_POINT('Ctrl Pts',(-1.14061059040513,-8.05658535462587,
43.870329392652));
#177439=CARTESIAN_POINT('Ctrl Pts',(-1.5709495469569,-7.98383744375511,
43.8517450237294));
#177440=CARTESIAN_POINT('Ctrl Pts',(-2.26669337639057,-7.80777085755481,
43.8215563886968));
#177441=CARTESIAN_POINT('Ctrl Pts',(-2.53625593626694,-7.72441604295968,
43.8098408578113));
#177442=CARTESIAN_POINT('Ctrl Pts',(-2.82190011867859,-7.61951871943386,
43.7977349152253));
#177443=CARTESIAN_POINT('Ctrl Pts',(-2.84282141182087,-7.61173779290116,
43.7968501330194));
#177444=CARTESIAN_POINT('Ctrl Pts',(-2.87202511825347,-7.60073932069382,
43.7956179776585));
#177445=CARTESIAN_POINT('Ctrl Pts',(-2.88033461846911,-7.59759428947356,
43.7952677143421));
#177446=CARTESIAN_POINT('Ctrl Pts',(-2.89550816017897,-7.59182284233145,
43.7946287398531));
#177447=CARTESIAN_POINT('Ctrl Pts',(-2.90237382297885,-7.58920073309052,
43.7943398526833));
#177448=CARTESIAN_POINT('Ctrl Pts',(-2.916223484814,-7.58388977734259,43.7937575839575));
#177449=CARTESIAN_POINT('Ctrl Pts',(-2.92320734657849,-7.58120058946147,
43.7934642170405));
#177450=CARTESIAN_POINT('Ctrl Pts',(-2.94029193037083,-7.57459492577229,
43.7927471828576));
#177451=CARTESIAN_POINT('Ctrl Pts',(-2.95038857148898,-7.57066788361836,
43.7923239679799));
#177452=CARTESIAN_POINT('Ctrl Pts',(-2.98664546640152,-7.55648238351508,
43.7908062215602));
#177453=CARTESIAN_POINT('Ctrl Pts',(-3.01276051441887,-7.54610835226529,
43.789716791176));
#177454=CARTESIAN_POINT('Ctrl Pts',(-3.09035711888323,-7.51481658287512,
43.7864921238135));
#177455=CARTESIAN_POINT('Ctrl Pts',(-3.14167608255709,-7.49350698273366,
43.7843766759602));
#177456=CARTESIAN_POINT('Ctrl Pts',(-3.33172440629778,-7.41229601884797,
43.7766033458235));
#177457=CARTESIAN_POINT('Ctrl Pts',(-3.46899534253118,-7.34905399182183,
43.7711056209107));
#177458=CARTESIAN_POINT('Ctrl Pts',(-3.89962638709474,-7.13590176015911,
43.7540358132553));
#177459=CARTESIAN_POINT('Ctrl Pts',(-4.18567940677025,-6.97196420692852,
43.7429590886332));
#177460=CARTESIAN_POINT('Ctrl Pts',(-4.6924009418013,-6.63910484374846,
43.7227108822087));
#177461=CARTESIAN_POINT('Ctrl Pts',(-4.91588129332239,-6.47537251974482,
43.7135302269684));
#177462=CARTESIAN_POINT('Ctrl Pts',(-5.53930228835542,-5.96771844354783,
43.6862958692775));
#177463=CARTESIAN_POINT('Ctrl Pts',(-5.91463767426695,-5.595937654131,43.6677090831581));
#177464=CARTESIAN_POINT('Ctrl Pts',(-6.2721373199752,-5.16536966161726,
43.6461965781401));
#177465=CARTESIAN_POINT('Ctrl Pts',(-6.292810882002,-5.14016356508407,43.6449376498866));
#177466=CARTESIAN_POINT('Ctrl Pts',(-6.3213087555192,-5.10498812409495,
43.6431812435748));
#177467=CARTESIAN_POINT('Ctrl Pts',(-6.32926239133614,-5.09512371877596,
43.6426887351025));
#177468=CARTESIAN_POINT('Ctrl Pts',(-6.34291455475529,-5.07811048441957,
43.6418393729979));
#177469=CARTESIAN_POINT('Ctrl Pts',(-6.34862416229896,-5.07097055661881,
43.641482943747));
#177470=CARTESIAN_POINT('Ctrl Pts',(-6.36037715505396,-5.05622234641789,
43.6407467447852));
#177471=CARTESIAN_POINT('Ctrl Pts',(-6.36641896637513,-5.04861283074464,
43.6403669160241));
#177472=CARTESIAN_POINT('Ctrl Pts',(-6.38043982209358,-5.0308887097145,
43.6394822618939));
#177473=CARTESIAN_POINT('Ctrl Pts',(-6.38840847881102,-5.02076594145754,
43.6389770436812));
#177474=CARTESIAN_POINT('Ctrl Pts',(-6.41368302088845,-4.98850152015256,
43.6373668452527));
#177475=CARTESIAN_POINT('Ctrl Pts',(-6.43089803964644,-4.96628912704614,
43.636258439679));
#177476=CARTESIAN_POINT('Ctrl Pts',(-6.75962287167571,-4.53756299518346,
43.6148664524412));
#177477=CARTESIAN_POINT('Ctrl Pts',(-7.0320853861352,-4.10263838288007,
43.5930931606757));
#177478=CARTESIAN_POINT('Ctrl Pts',(-7.53545778628034,-3.09979480313859,
43.5434612772505));
#177479=CARTESIAN_POINT('Ctrl Pts',(-7.74685067876847,-2.52549925227883,
43.5153755186125));
#177480=CARTESIAN_POINT('Ctrl Pts',(-7.93918042723531,-1.74025005816425,
43.4807326997601));
#177481=CARTESIAN_POINT('Ctrl Pts',(-7.97931233656667,-1.54584935029852,
43.4724715200992));
#177482=CARTESIAN_POINT('Ctrl Pts',(-8.01573678266102,-1.32969227894562,
43.4637227558245));
#177483=CARTESIAN_POINT('Ctrl Pts',(-8.0191048387637,-1.30922699381565,
43.4628983384693));
#177484=CARTESIAN_POINT('Ctrl Pts',(-8.02393742399501,-1.27914440365713,
43.4616919651483));
#177485=CARTESIAN_POINT('Ctrl Pts',(-8.02546308471682,-1.26953710718351,
43.4613075107311));
#177486=CARTESIAN_POINT('Ctrl Pts',(-8.02814497463701,-1.25245083727079,
43.4606251926377));
#177487=CARTESIAN_POINT('Ctrl Pts',(-8.02930801338898,-1.24497295560636,
43.4603270569537));
#177488=CARTESIAN_POINT('Ctrl Pts',(-8.03171030010472,-1.2293838072931,
43.4597065239183));
#177489=CARTESIAN_POINT('Ctrl Pts',(-8.03294771233321,-1.22127226365777,
43.4593841989911));
#177490=CARTESIAN_POINT('Ctrl Pts',(-8.0361248147711,-1.2002318283528,43.4585495451517));
#177491=CARTESIAN_POINT('Ctrl Pts',(-8.03804559635771,-1.18730007734661,
43.4580379456097));
#177492=CARTESIAN_POINT('Ctrl Pts',(-8.04608915636332,-1.13223221305118,
43.4558651127093));
#177493=CARTESIAN_POINT('Ctrl Pts',(-8.05191194838266,-1.09005254432804,
43.4542150961298));
#177494=CARTESIAN_POINT('Ctrl Pts',(-8.0940406148127,-0.766099145188816,
43.4416406689747));
#177495=CARTESIAN_POINT('Ctrl Pts',(-8.1158786617702,-0.482627865515014,
43.4312005377163));
#177496=CARTESIAN_POINT('Ctrl Pts',(-8.135225930706,0.308743104068866,43.4025211807722));
#177497=CARTESIAN_POINT('Ctrl Pts',(-8.10007344109652,0.816113456656182,
43.3845960547325));
#177498=CARTESIAN_POINT('Ctrl Pts',(-7.96596000923648,1.63265612685865,
43.3541518463842));
#177499=CARTESIAN_POINT('Ctrl Pts',(-7.89549106150435,1.94506885710805,
43.3421312063749));
#177500=CARTESIAN_POINT('Ctrl Pts',(-7.79381481825625,2.29746112418802,
43.3280077892873));
#177501=CARTESIAN_POINT('Ctrl Pts',(-7.78045501164359,2.3423058742983,43.3262001139419));
#177502=CARTESIAN_POINT('Ctrl Pts',(-7.75837642384178,2.41414316938138,
43.323287689265));
#177503=CARTESIAN_POINT('Ctrl Pts',(-7.74990232284037,2.44120993645363,
43.3221865233557));
#177504=CARTESIAN_POINT('Ctrl Pts',(-7.73457284415657,2.48928884623968,
43.3202237203911));
#177505=CARTESIAN_POINT('Ctrl Pts',(-7.72777310736054,2.51031847338947,
43.3193628732917));
#177506=CARTESIAN_POINT('Ctrl Pts',(-7.72086420084677,2.53139162522534,
43.3184979200565));
#177507=CARTESIAN_POINT('Ctrl Pts',(-7.72084072433549,2.53146322857538,
43.3184949810506));
#177508=CARTESIAN_POINT('Ctrl Pts',(-7.72079409662351,2.53160543639102,
43.3184891439847));
#177509=CARTESIAN_POINT('Ctrl Pts',(-7.72077095418529,2.53167601423059,
43.3184862470185));
#177510=CARTESIAN_POINT('Ctrl Pts',(-7.72072500094861,2.53181615201227,
43.3184804948148));
#177511=CARTESIAN_POINT('Ctrl Pts',(-7.72070219094693,2.53188570961862,
43.318477639674));
#177512=CARTESIAN_POINT('Ctrl Pts',(-7.72065689865357,2.53202381919728,
43.31847197062));
#177513=CARTESIAN_POINT('Ctrl Pts',(-7.72063441699642,2.53209236932629,
43.3184691567832));
#177514=CARTESIAN_POINT('Ctrl Pts',(-7.72058977699565,2.532228477628,43.3184635697781));
#177515=CARTESIAN_POINT('Ctrl Pts',(-7.72056761945206,2.53229603345048,
43.318460796707));
#177516=CARTESIAN_POINT('Ctrl Pts',(-7.72052362358933,2.53243016587103,
43.3184552907126));
#177517=CARTESIAN_POINT('Ctrl Pts',(-7.72050178604294,2.53249674019989,
43.3184525578832));
#177518=CARTESIAN_POINT('Ctrl Pts',(-7.72045842606367,2.53262892242341,
43.3184471318493));
#177519=CARTESIAN_POINT('Ctrl Pts',(-7.72043690442406,2.53269452798417,
43.3184444387413));
#177520=CARTESIAN_POINT('Ctrl Pts',(-7.72039417215233,2.53282478543858,
43.3184390916282));
#177521=CARTESIAN_POINT('Ctrl Pts',(-7.72037296235442,2.53288943487141,
43.3184364377248));
#177522=CARTESIAN_POINT('Ctrl Pts',(-7.72033084971694,2.53301779265579,
43.3184311685061));
#177523=CARTESIAN_POINT('Ctrl Pts',(-7.72030994774276,2.53308149844944,
43.3184285532965));
#177524=CARTESIAN_POINT('Ctrl Pts',(-7.72026844669099,2.53320798157188,
43.3184233609494));
#177525=CARTESIAN_POINT('Ctrl Pts',(-7.72024784853508,2.53327075616923,
43.3184207839247));
#177526=CARTESIAN_POINT('Ctrl Pts',(-7.7202069511716,2.53339538916199,43.3184156674459));
#177527=CARTESIAN_POINT('Ctrl Pts',(-7.72018665289644,2.5334572447914,43.318413128106));
#177528=CARTESIAN_POINT('Ctrl Pts',(-7.72014635131495,2.53358005219907,
43.3184080864914));
#177529=CARTESIAN_POINT('Ctrl Pts',(-7.72012634900176,2.53364100102445,
43.3184055843386));
#177530=CARTESIAN_POINT('Ctrl Pts',(-7.72009318223559,2.53374205906787,
43.3184014355359));
#177531=CARTESIAN_POINT('Ctrl Pts',(-7.72008001920702,2.53378216532449,
43.3183997890185));
#177532=CARTESIAN_POINT('Ctrl Pts',(-7.72005377507706,2.53386212612016,
43.3183965063012));
#177533=CARTESIAN_POINT('Ctrl Pts',(-7.72004066806906,2.53390205959654,
43.3183948668604));
#177534=CARTESIAN_POINT('Ctrl Pts',(-7.72001450106194,2.53398178123842,
43.3183915939277));
#177535=CARTESIAN_POINT('Ctrl Pts',(-7.72000144123687,2.5340215688813,43.3183899604572));
#177536=CARTESIAN_POINT('Ctrl Pts',(-7.71997536851898,2.5341009991124,43.3183866994548));
#177537=CARTESIAN_POINT('Ctrl Pts',(-7.71996235576821,2.53414064127546,
43.3183850719403));
#177538=CARTESIAN_POINT('Ctrl Pts',(-7.71993637702291,2.53421978110579,
43.3183818228271));
#177539=CARTESIAN_POINT('Ctrl Pts',(-7.71992341121742,2.53425927820475,
43.3183802012517));
#177540=CARTESIAN_POINT('Ctrl Pts',(-7.7198975261035,2.53433812871883,43.3183769639835));
#177541=CARTESIAN_POINT('Ctrl Pts',(-7.71988460704875,2.53437748136872,
43.3183753483221));
#177542=CARTESIAN_POINT('Ctrl Pts',(-7.71985881545119,2.5344560429617,43.3183721228831));
#177543=CARTESIAN_POINT('Ctrl Pts',(-7.71984594304755,2.53449525148833,
43.3183705131226));
#177544=CARTESIAN_POINT('Ctrl Pts',(-7.71982024462464,2.53457352524555,
43.3183672994685));
#177545=CARTESIAN_POINT('Ctrl Pts',(-7.71980741873576,2.5346125900864,43.318365695591));
#177546=CARTESIAN_POINT('Ctrl Pts',(-7.71978181325614,2.53469057675676,
43.3183624936915));
#177547=CARTESIAN_POINT('Ctrl Pts',(-7.7197690337824,2.53472949823728,43.3183608956839));
#177548=CARTESIAN_POINT('Ctrl Pts',(-7.71974352086098,2.53480719903753,
43.3183577054894));
#177549=CARTESIAN_POINT('Ctrl Pts',(-7.71973078762226,2.53484597772815,
43.3183561133283));
#177550=CARTESIAN_POINT('Ctrl Pts',(-7.71970536708742,2.53492339322454,
43.3183529348159));
#177551=CARTESIAN_POINT('Ctrl Pts',(-7.71969267995611,2.53496202953565,
43.3183513484848));
#177552=CARTESIAN_POINT('Ctrl Pts',(-7.71966735153383,2.535039160606,43.3183481816187));
#177553=CARTESIAN_POINT('Ctrl Pts',(-7.71965471038453,2.53507765494102,
43.3183466011012));
#177554=CARTESIAN_POINT('Ctrl Pts',(-7.71962947381584,2.53515450241696,
43.3183434458477));
#177555=CARTESIAN_POINT('Ctrl Pts',(-7.71961687854283,2.53519285511932,
43.3183418711298));
#177556=CARTESIAN_POINT('Ctrl Pts',(-7.71959173348298,2.53526942009338,
43.3183387274443));
#177557=CARTESIAN_POINT('Ctrl Pts',(-7.7195791839334,2.5353076316498,43.3183371585062));
#177558=CARTESIAN_POINT('Ctrl Pts',(-7.71955413011865,2.53538391496745,
43.3183340263545));
#177559=CARTESIAN_POINT('Ctrl Pts',(-7.71954162612672,2.53542198590384,
43.3183324631747));
#177560=CARTESIAN_POINT('Ctrl Pts',(-7.71951666337221,2.53549798817011,
43.3183293425322));
#177561=CARTESIAN_POINT('Ctrl Pts',(-7.71950420482444,2.53553591885301,
43.3183277850959));
#177562=CARTESIAN_POINT('Ctrl Pts',(-7.71947933281627,2.53561164106546,
43.3183246759219));
#177563=CARTESIAN_POINT('Ctrl Pts',(-7.71946691957511,2.53564943193453,
43.3183231242113));
#177564=CARTESIAN_POINT('Ctrl Pts',(-7.71944213804101,2.53572487496364,
43.3183200264705));
#177565=CARTESIAN_POINT('Ctrl Pts',(-7.71942976996171,2.53576252648026,
43.3183184804667));
#177566=CARTESIAN_POINT('Ctrl Pts',(-7.71940507867793,2.53583769104856,
43.3183153941297));
#177567=CARTESIAN_POINT('Ctrl Pts',(-7.71939275564967,2.53587520357067,
43.3183138538182));
#177568=CARTESIAN_POINT('Ctrl Pts',(-7.7193681543073,2.53595009065952,43.318310778845));
#177569=CARTESIAN_POINT('Ctrl Pts',(-7.71935587620204,2.53598746459734,
43.3183092442092));
#177570=CARTESIAN_POINT('Ctrl Pts',(-7.71933136448927,2.53606207519662,
43.3183061805595));
#177571=CARTESIAN_POINT('Ctrl Pts',(-7.71931913114104,2.53609931107565,
43.3183046515779));
#177572=CARTESIAN_POINT('Ctrl Pts',(-7.7192947088611,2.53617364582477,43.3183015992259));
#177573=CARTESIAN_POINT('Ctrl Pts',(-7.71928252014296,2.53621074405155,
43.3183000758819));
#177574=CARTESIAN_POINT('Ctrl Pts',(-7.71925818702915,2.53628480380246,
43.3182970347928));
#177575=CARTESIAN_POINT('Ctrl Pts',(-7.71924604282186,2.53632176475996,
43.318295517071));
#177576=CARTESIAN_POINT('Ctrl Pts',(-7.71922179861044,2.5363955503553,43.3182924872105));
#177577=CARTESIAN_POINT('Ctrl Pts',(-7.71920969881315,2.53643237437031,
43.3182909750976));
#177578=CARTESIAN_POINT('Ctrl Pts',(-7.71918554310673,2.53650588705915,
43.3182879564148));
#177579=CARTESIAN_POINT('Ctrl Pts',(-7.71917348752128,2.53654257475454,
43.3182864498853));
#177580=CARTESIAN_POINT('Ctrl Pts',(-7.71914942016059,2.53661581506093,
43.318283442359));
#177581=CARTESIAN_POINT('Ctrl Pts',(-7.71913740863179,2.53665236692852,
43.3182819413929));
#177582=CARTESIAN_POINT('Ctrl Pts',(-7.71911342952066,2.53672533518425,
43.3182789450098));
#177583=CARTESIAN_POINT('Ctrl Pts',(-7.71910146204209,2.53676175126314,
43.3182774496056));
#177584=CARTESIAN_POINT('Ctrl Pts',(-7.71907757056455,2.53683444938142,
43.3182744642875));
#177585=CARTESIAN_POINT('Ctrl Pts',(-7.71906564690765,2.53687073038643,
43.318272974416));
#177586=CARTESIAN_POINT('Ctrl Pts',(-7.71904184298302,2.53694315865129,
43.3182700001514));
#177587=CARTESIAN_POINT('Ctrl Pts',(-7.71902996300926,2.53697930502313,
43.3182685157948));
#177588=CARTESIAN_POINT('Ctrl Pts',(-7.71900624643302,2.53705146409521,
43.318265552557));
#177589=CARTESIAN_POINT('Ctrl Pts',(-7.71899441006016,2.53708747610323,
43.3182640737043));
#177590=CARTESIAN_POINT('Ctrl Pts',(-7.71897078042849,2.53715936724918,
43.3182611214415));
#177591=CARTESIAN_POINT('Ctrl Pts',(-7.71895898748708,2.53719524542784,
43.3182596480709));
#177592=CARTESIAN_POINT('Ctrl Pts',(-7.71893544458174,2.53726686934943,
43.3182567067546));
#177593=CARTESIAN_POINT('Ctrl Pts',(-7.71892369491311,2.53730261420029,
43.3182552388457));
#177594=CARTESIAN_POINT('Ctrl Pts',(-7.71890023856532,2.53737397144851,
43.3182523084536));
#177595=CARTESIAN_POINT('Ctrl Pts',(-7.71888853208125,2.53740958325863,
43.3182508459947));
#177596=CARTESIAN_POINT('Ctrl Pts',(-7.7188651619421,2.5374806749322,43.318247926482));
#177597=CARTESIAN_POINT('Ctrl Pts',(-7.71885349851508,2.53751615410806,
43.3182464694566));
#177598=CARTESIAN_POINT('Ctrl Pts',(-7.71883021431867,2.53758698105279,
43.3182435607888));
#177599=CARTESIAN_POINT('Ctrl Pts',(-7.71881859382518,2.53762232798861,
43.3182421091808));
#177600=CARTESIAN_POINT('Ctrl Pts',(-7.71879539527648,2.5376928911387,43.31823921132));
#177601=CARTESIAN_POINT('Ctrl Pts',(-7.71878381757113,2.53772810629498,
43.3182377651107));
#177602=CARTESIAN_POINT('Ctrl Pts',(-7.71876070436158,2.53779840662545,
43.318234878017));
#177603=CARTESIAN_POINT('Ctrl Pts',(-7.71874916924161,2.53783349063708,
43.3182334371804));
#177604=CARTESIAN_POINT('Ctrl Pts',(-7.71872614136112,2.53790352821487,
43.3182305608513));
#177605=CARTESIAN_POINT('Ctrl Pts',(-7.71871464880682,2.53793848115988,
43.3182291253844));
#177606=CARTESIAN_POINT('Ctrl Pts',(-7.71869170572183,2.53800825764377,
43.3182262597522));
#177607=CARTESIAN_POINT('Ctrl Pts',(-7.71868025555603,2.53804308007896,
43.3182248296323));
#177608=CARTESIAN_POINT('Ctrl Pts',(-7.7186573969895,2.53811259634722,43.3182219746612));
#177609=CARTESIAN_POINT('Ctrl Pts',(-7.71864598897575,2.53814728900938,
43.3182205498581));
#177610=CARTESIAN_POINT('Ctrl Pts',(-7.71862321504526,2.53821654473994,
43.3182177055615));
#177611=CARTESIAN_POINT('Ctrl Pts',(-7.71861184922293,2.53825110752712,
43.3182162860796));
#177612=CARTESIAN_POINT('Ctrl Pts',(-7.71141079274784,2.56014859472355,
43.3173169597234));
#177613=CARTESIAN_POINT('Ctrl Pts',(-7.70412826127212,2.58198082307861,
43.3164177782825));
#177614=CARTESIAN_POINT('Ctrl Pts',(-7.68565837342603,2.63657762841191,
43.3141625901609));
#177615=CARTESIAN_POINT('Ctrl Pts',(-7.67435419912403,2.66930212477082,
43.3128049217041));
#177616=CARTESIAN_POINT('Ctrl Pts',(-7.64958810192927,2.73953970964014,
43.3098775430473));
#177617=CARTESIAN_POINT('Ctrl Pts',(-7.63605863938204,2.77702797589849,
43.308306840452));
#177618=CARTESIAN_POINT('Ctrl Pts',(-7.59694764146552,2.8829519267926,43.3038443211235));
#177619=CARTESIAN_POINT('Ctrl Pts',(-7.57071828992925,2.95114379165832,
43.3009423080302));
#177620=CARTESIAN_POINT('Ctrl Pts',(-7.48094835357156,3.17545393848171,
43.2912937299656));
#177621=CARTESIAN_POINT('Ctrl Pts',(-7.41347117972893,3.32994576680014,
43.2844811355807));
#177622=CARTESIAN_POINT('Ctrl Pts',(-7.1943775174643,3.79183991538978,43.2635658903136));
#177623=CARTESIAN_POINT('Ctrl Pts',(-7.02808095223314,4.09184314423419,
43.2492081026081));
#177624=CARTESIAN_POINT('Ctrl Pts',(-6.66461197122455,4.65967297660361,
43.2206645242936));
#177625=CARTESIAN_POINT('Ctrl Pts',(-6.46895192405148,4.92770412172795,
43.2065172092838));
#177626=CARTESIAN_POINT('Ctrl Pts',(-6.19097616872694,5.2633037017996,43.1882993655216));
#177627=CARTESIAN_POINT('Ctrl Pts',(-6.12294815635756,5.34228961493669,
43.1839734291377));
#177628=CARTESIAN_POINT('Ctrl Pts',(-5.999762065711,5.47987344974748,43.1763941295349));
#177629=CARTESIAN_POINT('Ctrl Pts',(-5.94521789091443,5.53900194349548,
43.1731218052866));
#177630=CARTESIAN_POINT('Ctrl Pts',(-5.85993637499657,5.62873991630223,
43.168143008614));
#177631=CARTESIAN_POINT('Ctrl Pts',(-5.829817479223,5.65992893978231,43.1664102191611));
#177632=CARTESIAN_POINT('Ctrl Pts',(-5.78985835986735,5.70065042615432,
43.1641462327998));
#177633=CARTESIAN_POINT('Ctrl Pts',(-5.78024191196769,5.71040090977648,
43.1636040150442));
#177634=CARTESIAN_POINT('Ctrl Pts',(-5.765312195909,5.7254623639638,43.1627663281378));
#177635=CARTESIAN_POINT('Ctrl Pts',(-5.76001615936766,5.73079033308376,
43.1624699722669));
#177636=CARTESIAN_POINT('Ctrl Pts',(-5.74942422089966,5.74141662040014,
43.1618788719523));
#177637=CARTESIAN_POINT('Ctrl Pts',(-5.7441283658279,5.74671497450538,43.1615841256178));
#177638=CARTESIAN_POINT('Ctrl Pts',(-5.73232278041858,5.75849350719814,
43.1609288603418));
#177639=CARTESIAN_POINT('Ctrl Pts',(-5.72580936789303,5.76496999252924,
43.1605685405306));
#177640=CARTESIAN_POINT('Ctrl Pts',(-5.70732064493873,5.78329165210559,
43.1595491930477));
#177641=CARTESIAN_POINT('Ctrl Pts',(-5.69531942288969,5.79511069386634,
43.1588916021998));
#177642=CARTESIAN_POINT('Ctrl Pts',(-5.61000194549167,5.87861202412645,
43.1542460794458));
#177643=CARTESIAN_POINT('Ctrl Pts',(-5.53537483730188,5.94893501386298,
43.1503402883846));
#177644=CARTESIAN_POINT('Ctrl Pts',(-5.39356506901399,6.0775860160203,43.1432026924547));
#177645=CARTESIAN_POINT('Ctrl Pts',(-5.3267232241019,6.13625425928232,43.1399475758287));
#177646=CARTESIAN_POINT('Ctrl Pts',(-4.93736629972774,6.46684228061812,
43.1215289968502));
#177647=CARTESIAN_POINT('Ctrl Pts',(-4.59501171187625,6.71442759288274,
43.1074102534538));
#177648=CARTESIAN_POINT('Ctrl Pts',(-3.64554784453508,7.29428987859576,
43.0700097649961));
#177649=CARTESIAN_POINT('Ctrl Pts',(-3.01270579241394,7.57761180737288,
43.0465535127301));
#177650=CARTESIAN_POINT('Ctrl Pts',(-2.30997551292859,7.79009619240129,
43.0184483907628));
#177651=CARTESIAN_POINT('Ctrl Pts',(-2.26817382354244,7.80236970377461,
43.0167703832019));
#177652=CARTESIAN_POINT('Ctrl Pts',(-2.21097676559589,7.81866499880751,
43.0144654916384));
#177653=CARTESIAN_POINT('Ctrl Pts',(-2.19566499349843,7.82297870727617,
43.0138476024746));
#177654=CARTESIAN_POINT('Ctrl Pts',(-2.17139543113407,7.82973918282014,
43.0128668405602));
#177655=CARTESIAN_POINT('Ctrl Pts',(-2.16244591177299,7.83221561675182,
43.0125048807498));
#177656=CARTESIAN_POINT('Ctrl Pts',(-2.14511448355381,7.83697945024005,
43.0118033340963));
#177657=CARTESIAN_POINT('Ctrl Pts',(-2.1367331095607,7.83926875856409,43.0114638064462));
#177658=CARTESIAN_POINT('Ctrl Pts',(-2.11681478141822,7.84467498116884,
43.0106562876363));
#177659=CARTESIAN_POINT('Ctrl Pts',(-2.10527460572266,7.84777989064726,
43.0101879287998));
#177660=CARTESIAN_POINT('Ctrl Pts',(-2.07113658515394,7.85688408099155,
43.0088009338999));
#177661=CARTESIAN_POINT('Ctrl Pts',(-2.04851973565767,7.86281127193661,
43.0078800906289));
#177662=CARTESIAN_POINT('Ctrl Pts',(-1.86945097426594,7.90891471323045,
43.0005737026299));
#177663=CARTESIAN_POINT('Ctrl Pts',(-1.71186424149105,7.94451358068654,
42.9940487045344));
#177664=CARTESIAN_POINT('Ctrl Pts',(-1.34718749593792,8.01553981971223,
42.9787213989851));
#177665=CARTESIAN_POINT('Ctrl Pts',(-1.1395794686277,8.04767940722128,42.9698282733234));
#177666=CARTESIAN_POINT('Ctrl Pts',(-0.659246859878672,8.10307939567049,
42.9489161580937));
#177667=CARTESIAN_POINT('Ctrl Pts',(-0.386128024018008,8.12067704402824,
42.9367758549409));
#177668=CARTESIAN_POINT('Ctrl Pts',(0.15911113577437,8.12823727385243,42.9122975236471));
#177669=CARTESIAN_POINT('Ctrl Pts',(0.430891913528653,8.11836738840273,
42.8999773817311));
#177670=CARTESIAN_POINT('Ctrl Pts',(1.13116826917909,8.05766742681217,42.868457823685));
#177671=CARTESIAN_POINT('Ctrl Pts',(1.55709080156417,7.98630833263183,42.8495032297364));
#177672=CARTESIAN_POINT('Ctrl Pts',(2.00690392570419,7.87356842741467,42.8308946782213));
#177673=CARTESIAN_POINT('Ctrl Pts',(2.03837159261542,7.86548056025775,42.829599978799));
#177674=CARTESIAN_POINT('Ctrl Pts',(2.08127639483327,7.85417832863333,42.8278433961798));
#177675=CARTESIAN_POINT('Ctrl Pts',(2.09275595372134,7.85112738209627,42.8273742583536));
#177676=CARTESIAN_POINT('Ctrl Pts',(2.11092626501703,7.84625553665721,42.8266329794712));
#177677=CARTESIAN_POINT('Ctrl Pts',(2.11762141972482,7.84445123421721,42.8263601209435));
#177678=CARTESIAN_POINT('Ctrl Pts',(2.13057891356626,7.84094147285557,42.8258325676889));
#177679=CARTESIAN_POINT('Ctrl Pts',(2.1368415324452,7.83923707724237,42.8255778279998));
#177680=CARTESIAN_POINT('Ctrl Pts',(2.15171885206167,7.83516900544632,42.8249732253256));
#177681=CARTESIAN_POINT('Ctrl Pts',(2.16033172097101,7.8327986198037,42.8246236440325));
#177682=CARTESIAN_POINT('Ctrl Pts',(2.18580009454235,7.82574415353778,42.8235911813598));
#177683=CARTESIAN_POINT('Ctrl Pts',(2.20264446128824,7.82101981796767,42.8229099538309));
#177684=CARTESIAN_POINT('Ctrl Pts',(2.33028326768221,7.78477593201482,42.8177594111088));
#177685=CARTESIAN_POINT('Ctrl Pts',(2.44041450187959,7.75095703001012,42.8133808375343));
#177686=CARTESIAN_POINT('Ctrl Pts',(2.80946250071686,7.62898435703066,42.7988259573468));
#177687=CARTESIAN_POINT('Ctrl Pts',(3.06464376725408,7.53010294695429,42.788952647525));
#177688=CARTESIAN_POINT('Ctrl Pts',(3.78596785004583,7.20783908608765,42.7605983443867));
#177689=CARTESIAN_POINT('Ctrl Pts',(4.23639902806167,6.95265530020107,42.7422317071644));
#177690=CARTESIAN_POINT('Ctrl Pts',(5.00240361006941,6.41644662906668,42.7075275221651));
#177691=CARTESIAN_POINT('Ctrl Pts',(5.32618550505402,6.15032931690788,42.6915642532777));
#177692=CARTESIAN_POINT('Ctrl Pts',(5.70842868503499,5.78324824074013,42.6710815152664));
#177693=CARTESIAN_POINT('Ctrl Pts',(5.78724640700374,5.70437525018435,42.6667569547309));
#177694=CARTESIAN_POINT('Ctrl Pts',(5.8984332466823,5.58843343788272,42.6604987736079));
#177695=CARTESIAN_POINT('Ctrl Pts',(5.9321282397313,5.5526532013677,42.6585805493182));
#177696=CARTESIAN_POINT('Ctrl Pts',(5.99121129525999,5.48876209068082,42.6551774196928));
#177697=CARTESIAN_POINT('Ctrl Pts',(6.01673134874103,5.46077521387005,42.6536940813364));
#177698=CARTESIAN_POINT('Ctrl Pts',(6.06540148505567,5.40664514131769,42.6508388318612));
#177699=CARTESIAN_POINT('Ctrl Pts',(6.08858056437309,5.38052911521294,42.649467290668));
#177700=CARTESIAN_POINT('Ctrl Pts',(6.13810761446642,5.32399678521263,42.6465109754763));
#177701=CARTESIAN_POINT('Ctrl Pts',(6.16439941714729,5.29353253180919,42.6449256039618));
#177702=CARTESIAN_POINT('Ctrl Pts',(6.26465236088444,5.17560985699768,42.6388177138522));
#177703=CARTESIAN_POINT('Ctrl Pts',(6.33698691704785,5.08678710342411,42.6342773421413));
#177704=CARTESIAN_POINT('Ctrl Pts',(6.50770199983884,4.86786373601786,42.6232225498849));
#177705=CARTESIAN_POINT('Ctrl Pts',(6.60408954305541,4.7362731146837,42.6166892592864));
#177706=CARTESIAN_POINT('Ctrl Pts',(7.01237905660326,4.14214742259587,42.5876595647853));
#177707=CARTESIAN_POINT('Ctrl Pts',(7.28012406102139,3.65111381113903,42.56481333148));
#177708=CARTESIAN_POINT('Ctrl Pts',(7.54380157565832,3.02099870177545,42.5373708478235));
#177709=CARTESIAN_POINT('Ctrl Pts',(7.5894739181055,2.90435220511297,42.5323676853423));
#177710=CARTESIAN_POINT('Ctrl Pts',(7.6438398765672,2.75545021810583,42.5260906180345));
#177711=CARTESIAN_POINT('Ctrl Pts',(7.65505593485097,2.72413520487855,42.5247765736869));
#177712=CARTESIAN_POINT('Ctrl Pts',(7.67193533832621,2.67608070758901,42.5227696872137));
#177713=CARTESIAN_POINT('Ctrl Pts',(7.67773685304264,2.65939026993549,42.5220744229651));
#177714=CARTESIAN_POINT('Ctrl Pts',(7.68931090816715,2.62573919064727,42.5206761850738));
#177715=CARTESIAN_POINT('Ctrl Pts',(7.69508187228439,2.60877816636048,42.5199732275087));
#177716=CARTESIAN_POINT('Ctrl Pts',(7.70682845157251,2.57387652143945,42.5185302093478));
#177717=CARTESIAN_POINT('Ctrl Pts',(7.71279763185633,2.55593384548913,42.5177902574539));
#177718=CARTESIAN_POINT('Ctrl Pts',(7.72171367713446,2.52881756630794,42.516674689839));
#177719=CARTESIAN_POINT('Ctrl Pts',(7.72470694055985,2.51965931787174,42.5162983823247));
#177720=CARTESIAN_POINT('Ctrl Pts',(7.74835368152359,2.446871089066,42.5133111330687));
#177721=CARTESIAN_POINT('Ctrl Pts',(7.76823701919188,2.38299320471857,42.5107112547795));
#177722=CARTESIAN_POINT('Ctrl Pts',(7.82714155320064,2.18517803078143,42.5027136546651));
#177723=CARTESIAN_POINT('Ctrl Pts',(7.86350425565667,2.05047536182246,42.4973425384259));
#177724=CARTESIAN_POINT('Ctrl Pts',(7.96321135834686,1.63931856032761,42.4810720365312));
#177725=CARTESIAN_POINT('Ctrl Pts',(8.01556850876955,1.36042668233816,42.4701953982874));
#177726=CARTESIAN_POINT('Ctrl Pts',(8.06217324061677,1.01270633249905,42.4565928005351));
#177727=CARTESIAN_POINT('Ctrl Pts',(8.07028003231253,0.945934255082753,
42.4539793868732));
#177728=CARTESIAN_POINT('Ctrl Pts',(8.08180445319509,0.840039136813365,
42.449830204852));
#177729=CARTESIAN_POINT('Ctrl Pts',(8.0857691160484,0.800978626131609,42.4482987727469));
#177730=CARTESIAN_POINT('Ctrl Pts',(8.09265244415706,0.727894232208515,
42.4454311311958));
#177731=CARTESIAN_POINT('Ctrl Pts',(8.09564002075744,0.693877684027413,
42.4440955026879));
#177732=CARTESIAN_POINT('Ctrl Pts',(8.10118006138048,0.625883461946875,
42.4414237038685));
#177733=CARTESIAN_POINT('Ctrl Pts',(8.10373340690565,0.591906542886768,
42.4400875677428));
#177734=CARTESIAN_POINT('Ctrl Pts',(8.10909802289794,0.513962775514821,
42.4370198522718));
#177735=CARTESIAN_POINT('Ctrl Pts',(8.11176556218601,0.469987153224875,
42.4352871662012));
#177736=CARTESIAN_POINT('Ctrl Pts',(8.12151370489216,0.284309626197095,
42.427962665018));
#177737=CARTESIAN_POINT('Ctrl Pts',(8.12523976146772,0.142458731127623,
42.4223452556673));
#177738=CARTESIAN_POINT('Ctrl Pts',(8.12524997892878,0.000585164857848444,
42.4167054960774));
#177739=CARTESIAN_POINT('',(8.12525,7.08749465366809E-13,40.4167025567876));
#177740=CARTESIAN_POINT('Ctrl Pts',(8.12525,7.08750173002854E-13,40.4167025567876));
#177741=CARTESIAN_POINT('Ctrl Pts',(8.1252499999998,2.24624642433485,40.5047001499288));
#177742=CARTESIAN_POINT('Ctrl Pts',(7.14398562317558,4.47535249753519,40.59269774307));
#177743=CARTESIAN_POINT('Ctrl Pts',(3.83078204044859,7.50935546634399,40.7686929293524));
#177744=CARTESIAN_POINT('Ctrl Pts',(1.52412477697662,8.29110090552153,40.8566905224937));
#177745=CARTESIAN_POINT('Ctrl Pts',(-2.95101623932641,7.89663306204396,
41.032685708776));
#177746=CARTESIAN_POINT('Ctrl Pts',(-5.08535169588805,6.72342983085734,
41.1206833019173));
#177747=CARTESIAN_POINT('Ctrl Pts',(-7.81671694684439,3.15661951052857,
41.2966784881996));
#177748=CARTESIAN_POINT('Ctrl Pts',(-8.39290461146711,0.79022955155319,
41.3846760813409));
#177749=CARTESIAN_POINT('Ctrl Pts',(-7.60701611462442,-3.63299000730503,
41.5606712676232));
#177750=CARTESIAN_POINT('Ctrl Pts',(-6.2509368040129,-5.65606750610093,
41.6486688607645));
#177751=CARTESIAN_POINT('Ctrl Pts',(-2.45807268688456,-8.06369575488349,
41.8246640470469));
#177752=CARTESIAN_POINT('Ctrl Pts',(-0.05022995104427,-8.42987470330087,
41.9126616401881));
#177753=CARTESIAN_POINT('Ctrl Pts',(4.28689960881094,-7.25863639434505,
42.0886568264705));
#177754=CARTESIAN_POINT('Ctrl Pts',(6.18309125557241,-5.73015646266294,
42.1766544196117));
#177755=CARTESIAN_POINT('Ctrl Pts',(7.81050559202928,-2.58640713800177,
42.3153355274311));
#177756=CARTESIAN_POINT('Ctrl Pts',(8.12525000000008,-1.29375883538076,
42.3660190421094));
#177757=CARTESIAN_POINT('Ctrl Pts',(8.12525,5.33559939809858E-13,42.4167025567876));
#177758=CARTESIAN_POINT('',(8.11892105081991,0.00515126165398824,36.4167025567876));
#177759=CARTESIAN_POINT('Ctrl Pts',(8.1252485711882,-0.00481859980626085,
40.4188459864349));
#177760=CARTESIAN_POINT('Ctrl Pts',(8.1251819769692,-0.117111507396714,
40.4144052047108));
#177761=CARTESIAN_POINT('Ctrl Pts',(8.12278751819628,-0.22939079092564,
40.4099448085709));
#177762=CARTESIAN_POINT('Ctrl Pts',(8.09547973049322,-0.878385878674702,
40.3840313152647));
#177763=CARTESIAN_POINT('Ctrl Pts',(8.01970496545542,-1.41161764218638,
40.3621556303063));
#177764=CARTESIAN_POINT('Ctrl Pts',(7.8469380395891,-2.11681216089531,40.3327010699118));
#177765=CARTESIAN_POINT('Ctrl Pts',(7.79563605181829,-2.29856265439132,
40.3250679245549));
#177766=CARTESIAN_POINT('Ctrl Pts',(7.7170919871729,-2.54379630369786,40.3147517221167));
#177767=CARTESIAN_POINT('Ctrl Pts',(7.69530536892766,-2.60896220197726,
40.3120088286049));
#177768=CARTESIAN_POINT('Ctrl Pts',(7.66125444458475,-2.70667258326552,
40.307896309049));
#177769=CARTESIAN_POINT('Ctrl Pts',(7.64960356275784,-2.73942721905045,
40.3065177399438));
#177770=CARTESIAN_POINT('Ctrl Pts',(7.63028340929652,-2.79265835540521,
40.3042778008842));
#177771=CARTESIAN_POINT('Ctrl Pts',(7.62274109165079,-2.81318038005924,
40.3034143517969));
#177772=CARTESIAN_POINT('Ctrl Pts',(7.60916018908447,-2.84967724958447,
40.3018790702057));
#177773=CARTESIAN_POINT('Ctrl Pts',(7.6031539028261,-2.86566396210636,40.3012066760006));
#177774=CARTESIAN_POINT('Ctrl Pts',(7.59052060888832,-2.89897021809782,
40.2998060900536));
#177775=CARTESIAN_POINT('Ctrl Pts',(7.58388462978731,-2.91628622814618,
40.2990780542807));
#177776=CARTESIAN_POINT('Ctrl Pts',(7.56870242196635,-2.95550059683324,
40.2974294016943));
#177777=CARTESIAN_POINT('Ctrl Pts',(7.56012031828319,-2.9773849111008,40.2965093965113));
#177778=CARTESIAN_POINT('Ctrl Pts',(7.53743130477847,-3.03451114060876,
40.2941074784629));
#177779=CARTESIAN_POINT('Ctrl Pts',(7.52317215334946,-3.06969205429657,
40.2926279063032));
#177780=CARTESIAN_POINT('Ctrl Pts',(7.43791680690272,-3.27587596353569,
40.2839498226564));
#177781=CARTESIAN_POINT('Ctrl Pts',(7.36133807237399,-3.44451344136854,
40.276822830029));
#177782=CARTESIAN_POINT('Ctrl Pts',(7.18896156513465,-3.79204936111791,
40.2619058705827));
#177783=CARTESIAN_POINT('Ctrl Pts',(7.09208997161504,-3.97027281562581,
40.2541220989433));
#177784=CARTESIAN_POINT('Ctrl Pts',(6.93023358092275,-4.24319057357566,
40.2418710136692));
#177785=CARTESIAN_POINT('Ctrl Pts',(6.86973823107639,-4.34044929648943,
40.2374366352345));
#177786=CARTESIAN_POINT('Ctrl Pts',(6.78131951340159,-4.47611900089402,
40.2311401753544));
#177787=CARTESIAN_POINT('Ctrl Pts',(6.75508426352783,-4.51561426856414,
40.2292936188642));
#177788=CARTESIAN_POINT('Ctrl Pts',(6.70963802069234,-4.58274785551292,
40.2261307267005));
#177789=CARTESIAN_POINT('Ctrl Pts',(6.69059820030894,-4.6105006224167,40.2248160463785));
#177790=CARTESIAN_POINT('Ctrl Pts',(6.65025131904567,-4.66853465648938,
40.2220515368519));
#177791=CARTESIAN_POINT('Ctrl Pts',(6.62890859924075,-4.69879018647623,
40.2206013874757));
#177792=CARTESIAN_POINT('Ctrl Pts',(6.57387199283709,-4.77568899243237,
40.2168924205391));
#177793=CARTESIAN_POINT('Ctrl Pts',(6.53988815231436,-4.822122068366,40.2146308123889));
#177794=CARTESIAN_POINT('Ctrl Pts',(6.36557719683538,-5.05505564789734,
40.2031711204747));
#177795=CARTESIAN_POINT('Ctrl Pts',(6.21775544279945,-5.23580705588439,
40.1938993689842));
#177796=CARTESIAN_POINT('Ctrl Pts',(5.94837388922065,-5.53767498081775,
40.1777566921731));
#177797=CARTESIAN_POINT('Ctrl Pts',(5.8303790990267,-5.6617731878283,40.1709096303088));
#177798=CARTESIAN_POINT('Ctrl Pts',(5.63621283063207,-5.85347130840994,
40.1600262849563));
#177799=CARTESIAN_POINT('Ctrl Pts',(5.56253882696945,-5.92352795451505,
40.1559792936496));
#177800=CARTESIAN_POINT('Ctrl Pts',(5.45512319602477,-6.02189788605954,
40.1502062101591));
#177801=CARTESIAN_POINT('Ctrl Pts',(5.42243604516287,-6.05134783309196,
40.1484658181077));
#177802=CARTESIAN_POINT('Ctrl Pts',(5.37051791042152,-6.09736575027585,
40.1457283196326));
#177803=CARTESIAN_POINT('Ctrl Pts',(5.35144579075298,-6.11411151956304,
40.1447283216727));
#177804=CARTESIAN_POINT('Ctrl Pts',(5.31831846615572,-6.1429243358456,40.1430013238426));
#177805=CARTESIAN_POINT('Ctrl Pts',(5.30429988785251,-6.15503317679096,
40.1422735611404));
#177806=CARTESIAN_POINT('Ctrl Pts',(5.27676631023246,-6.17865195614285,
40.1408502386042));
#177807=CARTESIAN_POINT('Ctrl Pts',(5.26325478457163,-6.19016572984544,
40.1401545903957));
#177808=CARTESIAN_POINT('Ctrl Pts',(5.23268152857093,-6.21604609681591,
40.1385866999178));
#177809=CARTESIAN_POINT('Ctrl Pts',(5.2155981426956,-6.23038691217221,40.1377149301721));
#177810=CARTESIAN_POINT('Ctrl Pts',(5.16907263965613,-6.26911774497663,
40.1353520502838));
#177811=CARTESIAN_POINT('Ctrl Pts',(5.13951701783502,-6.29337064671277,
40.1338632365727));
#177812=CARTESIAN_POINT('Ctrl Pts',(4.97315107578598,-6.42793444380456,
40.125547264049));
#177813=CARTESIAN_POINT('Ctrl Pts',(4.83295985692925,-6.53399364949683,
40.1187807203424));
#177814=CARTESIAN_POINT('Ctrl Pts',(4.68016225860993,-6.6419799630296,40.1115959796777));
#177815=CARTESIAN_POINT('Ctrl Pts',(4.67087203141289,-6.6485164557599,40.1111598739999));
#177816=CARTESIAN_POINT('Ctrl Pts',(4.64096565903866,-6.66946459874231,
40.1097583047798));
#177817=CARTESIAN_POINT('Ctrl Pts',(4.62029628046534,-6.68380000929254,
40.1087931448782));
#177818=CARTESIAN_POINT('Ctrl Pts',(4.58336915500097,-6.70915796078588,
40.1070748082565));
#177819=CARTESIAN_POINT('Ctrl Pts',(4.56713738390945,-6.72021796303621,
40.1063215337671));
#177820=CARTESIAN_POINT('Ctrl Pts',(4.31249044281815,-6.89238054166912,
40.0945348456375));
#177821=CARTESIAN_POINT('Ctrl Pts',(4.06572372624255,-7.04076507792674,
40.0835270349664));
#177822=CARTESIAN_POINT('Ctrl Pts',(3.65930398638107,-7.25664683608995,
40.0657745856703));
#177823=CARTESIAN_POINT('Ctrl Pts',(3.50446420412401,-7.33267746359716,
40.0590951308392));
#177824=CARTESIAN_POINT('Ctrl Pts',(3.28305051318219,-7.43278160218562,
40.0496334060862));
#177825=CARTESIAN_POINT('Ctrl Pts',(3.21840185453257,-7.4610021083678,40.0468813884373));
#177826=CARTESIAN_POINT('Ctrl Pts',(3.10487426610065,-7.50880915987454,
40.0420659194891));
#177827=CARTESIAN_POINT('Ctrl Pts',(3.0561570490982,-7.52876904119957,40.0400049796456));
#177828=CARTESIAN_POINT('Ctrl Pts',(2.95302932740019,-7.56985546714256,
40.0356534523509));
#177829=CARTESIAN_POINT('Ctrl Pts',(2.89857819416075,-7.59087204647968,
40.0333623599727));
#177830=CARTESIAN_POINT('Ctrl Pts',(2.72695079120161,-7.65499934472716,
40.0261611326993));
#177831=CARTESIAN_POINT('Ctrl Pts',(2.6090047966837,-7.69599697012235,40.0212413762091));
#177832=CARTESIAN_POINT('Ctrl Pts',(2.34541753594677,-7.78086285281284,
40.0103154403997));
#177833=CARTESIAN_POINT('Ctrl Pts',(2.19939393744849,-7.82339290015442,
40.0043081043583));
#177834=CARTESIAN_POINT('Ctrl Pts',(1.99353865432809,-7.87712985526717,
39.9959176202091));
#177835=CARTESIAN_POINT('Ctrl Pts',(1.93464415275881,-7.89180100807817,
39.9935260622607));
#177836=CARTESIAN_POINT('Ctrl Pts',(1.87427880792064,-7.90612220565004,
39.9910849200648));
#177837=CARTESIAN_POINT('Ctrl Pts',(1.8729668150793,-7.90643312057372,39.9910318686688));
#177838=CARTESIAN_POINT('Ctrl Pts',(1.87034324980781,-7.9070541611145,39.9909257926807));
#177839=CARTESIAN_POINT('Ctrl Pts',(1.86903167747601,-7.90736428701065,
39.9908727680883));
#177840=CARTESIAN_POINT('Ctrl Pts',(1.86640865832378,-7.90798382005548,
39.9907667337977));
#177841=CARTESIAN_POINT('Ctrl Pts',(1.86509721158565,-7.90829322733173,
39.9907137241008));
#177842=CARTESIAN_POINT('Ctrl Pts',(1.86247413720249,-7.90891139578969,
39.9906077072349));
#177843=CARTESIAN_POINT('Ctrl Pts',(1.86116250958926,-7.90922015694973,
39.9905547000674));
#177844=CARTESIAN_POINT('Ctrl Pts',(1.85853875577263,-7.90983710783268,
39.9904486754479));
#177845=CARTESIAN_POINT('Ctrl Pts',(1.85722662956809,-7.91014529737471,
39.9903956579986));
#177846=CARTESIAN_POINT('Ctrl Pts',(1.85550300436084,-7.91054968645628,
39.9903260201186));
#177847=CARTESIAN_POINT('Ctrl Pts',(1.85509157451694,-7.91064618038513,
39.9903093980224));
#177848=CARTESIAN_POINT('Ctrl Pts',(1.85423286767628,-7.91084750491217,
39.9902747065918));
#177849=CARTESIAN_POINT('Ctrl Pts',(1.85378558932523,-7.91095232967285,
39.9902566372911));
#177850=CARTESIAN_POINT('Ctrl Pts',(1.85285235375731,-7.9111709605331,39.9902189373286));
#177851=CARTESIAN_POINT('Ctrl Pts',(1.85236639493926,-7.91128475979129,
39.990199306706));
#177852=CARTESIAN_POINT('Ctrl Pts',(1.85135278869658,-7.91152202221167,
39.9901583628404));
#177853=CARTESIAN_POINT('Ctrl Pts',(1.85082513940203,-7.91164547736515,
39.9901370496435));
#177854=CARTESIAN_POINT('Ctrl Pts',(1.84972495949717,-7.91190277255842,
39.9900926120434));
#177855=CARTESIAN_POINT('Ctrl Pts',(1.84915242669486,-7.91203660324274,
39.9900694876938));
#177856=CARTESIAN_POINT('Ctrl Pts',(1.84795909969006,-7.91231540920709,
39.9900212917084));
#177857=CARTESIAN_POINT('Ctrl Pts',(1.8473383029026,-7.9124603735837,39.989996220134));
#177858=CARTESIAN_POINT('Ctrl Pts',(1.84604487648848,-7.912762245483,39.9899439859762));
#177859=CARTESIAN_POINT('Ctrl Pts',(1.84537224392627,-7.91291914029817,
39.9899168234676));
#177860=CARTESIAN_POINT('Ctrl Pts',(1.8439713798153,-7.91324571032853,39.9898602559539));
#177861=CARTESIAN_POINT('Ctrl Pts',(1.84324314483148,-7.91341537078919,
39.9898308510351));
#177862=CARTESIAN_POINT('Ctrl Pts',(1.84172711196871,-7.91376834774494,
39.9897696393416));
#177863=CARTESIAN_POINT('Ctrl Pts',(1.84093931010477,-7.9139516471382,39.989737832667));
#177864=CARTESIAN_POINT('Ctrl Pts',(1.83929997896678,-7.91433281547642,
39.9896716501324));
#177865=CARTESIAN_POINT('Ctrl Pts',(1.83844844510834,-7.91453066463407,
39.9896372743897));
#177866=CARTESIAN_POINT('Ctrl Pts',(1.83667728213165,-7.91494188323866,
39.9895657783293));
#177867=CARTESIAN_POINT('Ctrl Pts',(1.83575764772262,-7.91515522984686,
39.9895286581475));
#177868=CARTESIAN_POINT('Ctrl Pts',(1.83384570951133,-7.91559843054879,
39.9894514896615));
#177869=CARTESIAN_POINT('Ctrl Pts',(1.83285339960373,-7.91582825834169,
39.9894114415142));
#177870=CARTESIAN_POINT('Ctrl Pts',(1.83079132645743,-7.91630544427434,
39.9893282252746));
#177871=CARTESIAN_POINT('Ctrl Pts',(1.82972155624718,-7.91655277217829,
39.9892850573654));
#177872=CARTESIAN_POINT('Ctrl Pts',(1.82749956446088,-7.91706601606434,
39.9891954013589));
#177873=CARTESIAN_POINT('Ctrl Pts',(1.82634733488476,-7.9173318973746,39.9891489134723));
#177874=CARTESIAN_POINT('Ctrl Pts',(1.82395520666374,-7.91788333997653,
39.9890524086529));
#177875=CARTESIAN_POINT('Ctrl Pts',(1.82271529889148,-7.91816886158542,
39.9890023919636));
#177876=CARTESIAN_POINT('Ctrl Pts',(1.82014236976715,-7.91876071030438,
39.9888986118119));
#177877=CARTESIAN_POINT('Ctrl Pts',(1.81880933801753,-7.91906699209084,
39.9888448486304));
#177878=CARTESIAN_POINT('Ctrl Pts',(1.81604448062742,-7.91970151992816,
39.9887333485743));
#177879=CARTESIAN_POINT('Ctrl Pts',(1.81461264317271,-7.92002971431345,
39.9886756120234));
#177880=CARTESIAN_POINT('Ctrl Pts',(1.81164424725919,-7.92070925917188,
39.9885559287147));
#177881=CARTESIAN_POINT('Ctrl Pts',(1.81010767539403,-7.92106055086305,
39.9884939823291));
#177882=CARTESIAN_POINT('Ctrl Pts',(1.80692362382067,-7.92178751516963,
39.9883656327704));
#177883=CARTESIAN_POINT('Ctrl Pts',(1.80527612891062,-7.92216312102983,
39.9882992300239));
#177884=CARTESIAN_POINT('Ctrl Pts',(1.76803700737578,-7.93064090172793,
39.9867984781306));
#177885=CARTESIAN_POINT('Ctrl Pts',(1.73239121354811,-7.93850367946046,
39.9853656918028));
#177886=CARTESIAN_POINT('Ctrl Pts',(1.65057425568284,-7.95597361443739,
39.9820861760189));
#177887=CARTESIAN_POINT('Ctrl Pts',(1.60436999730531,-7.96541954065471,
39.9802406517647));
#177888=CARTESIAN_POINT('Ctrl Pts',(1.39331777883707,-8.00665586283508,
39.9718353305307));
#177889=CARTESIAN_POINT('Ctrl Pts',(1.22759079173065,-8.03373473305531,
39.9653028489402));
#177890=CARTESIAN_POINT('Ctrl Pts',(0.903846226043641,-8.07638046380758,
39.9525894849163));
#177891=CARTESIAN_POINT('Ctrl Pts',(0.745976017161152,-8.09248904478588,
39.9464118006412));
#177892=CARTESIAN_POINT('Ctrl Pts',(0.532732046101728,-8.10795445732032,
39.9380593152625));
#177893=CARTESIAN_POINT('Ctrl Pts',(0.477688964854494,-8.11138349153013,
39.9359027156763));
#177894=CARTESIAN_POINT('Ctrl Pts',(0.382351215999723,-8.11634897647779,
39.932164683451));
#177895=CARTESIAN_POINT('Ctrl Pts',(0.34207209574314,-8.11814632980938,
39.9305845830816));
#177896=CARTESIAN_POINT('Ctrl Pts',(0.274014037820888,-8.12067583130098,
39.9279128300663));
#177897=CARTESIAN_POINT('Ctrl Pts',(0.246241666479283,-8.1215654087346,
39.9268220323059));
#177898=CARTESIAN_POINT('Ctrl Pts',(0.209379042880324,-8.122556900316,39.9253733660159));
#177899=CARTESIAN_POINT('Ctrl Pts',(0.200292375896853,-8.12278604584081,
39.9250162012173));
#177900=CARTESIAN_POINT('Ctrl Pts',(0.119515140179965,-8.12468744181302,
39.9218405076695));
#177901=CARTESIAN_POINT('Ctrl Pts',(0.0478059584587918,-8.12542579961906,
39.9190169058176));
#177902=CARTESIAN_POINT('Ctrl Pts',(-0.205672567958882,-8.12468009736984,
39.9090159528562));
#177903=CARTESIAN_POINT('Ctrl Pts',(-0.387371165912396,-8.11804597769241,
39.9018094927786));
#177904=CARTESIAN_POINT('Ctrl Pts',(-0.725351555175829,-8.09433230679333,
39.888317085699));
#177905=CARTESIAN_POINT('Ctrl Pts',(-0.881658147361512,-8.07880120349797,
39.882042347435));
#177906=CARTESIAN_POINT('Ctrl Pts',(-1.06783522663328,-8.05483433608878,
39.8745308909834));
#177907=CARTESIAN_POINT('Ctrl Pts',(-1.09823246219525,-8.0507461586496,
39.8733033137494));
#177908=CARTESIAN_POINT('Ctrl Pts',(-1.3453650205405,-8.01608317129101,
39.8633139249273));
#177909=CARTESIAN_POINT('Ctrl Pts',(-1.5608080161246,-7.97693396640702,
39.854546195635));
#177910=CARTESIAN_POINT('Ctrl Pts',(-1.84579645032834,-7.91315832151464,
39.8429235172893));
#177911=CARTESIAN_POINT('Ctrl Pts',(-1.91696667652322,-7.89621922300006,
39.8400191463585));
#177912=CARTESIAN_POINT('Ctrl Pts',(-2.02403149014228,-7.86920407591601,
39.8356505863755));
#177913=CARTESIAN_POINT('Ctrl Pts',(-2.06010120358055,-7.85983837680962,
39.8341789491582));
#177914=CARTESIAN_POINT('Ctrl Pts',(-2.11928562700564,-7.84403541740643,
39.8317649678267));
#177915=CARTESIAN_POINT('Ctrl Pts',(-2.14243846378034,-7.83774333800429,
39.8308208080423));
#177916=CARTESIAN_POINT('Ctrl Pts',(-2.16563225108831,-7.83132967769123,
39.8298752577217));
#177917=CARTESIAN_POINT('Ctrl Pts',(-2.1657013597474,-7.83131056643966,
39.8298724403441));
#177918=CARTESIAN_POINT('Ctrl Pts',(-2.16583972556701,-7.83127230089845,
39.8298667995399));
#177919=CARTESIAN_POINT('Ctrl Pts',(-2.16590898294062,-7.83125314654562,
39.8298639761046));
#177920=CARTESIAN_POINT('Ctrl Pts',(-2.16604764546928,-7.83121479498823,
39.8298583232143));
#177921=CARTESIAN_POINT('Ctrl Pts',(-2.16611705050937,-7.83119559781124,
39.8298554937641));
#177922=CARTESIAN_POINT('Ctrl Pts',(-2.16625600772886,-7.83115716077045,
39.8298498288703));
#177923=CARTESIAN_POINT('Ctrl Pts',(-2.1663255596686,-7.83113792096871,
39.8298469934364));
#177924=CARTESIAN_POINT('Ctrl Pts',(-2.16646480963405,-7.83109939895714,
39.8298413166183));
#177925=CARTESIAN_POINT('Ctrl Pts',(-2.16653450781359,-7.83108011670054,
39.8298384752278));
#177926=CARTESIAN_POINT('Ctrl Pts',(-2.16667404941672,-7.83104150999953,
39.8298327865306));
#177927=CARTESIAN_POINT('Ctrl Pts',(-2.16674389281416,-7.83102218555816,
39.8298299392251));
#177928=CARTESIAN_POINT('Ctrl Pts',(-2.16688372403984,-7.83098349470005,
39.8298242387311));
#177929=CARTESIAN_POINT('Ctrl Pts',(-2.16695371191143,-7.83096412826713,
39.829821385541));
#177930=CARTESIAN_POINT('Ctrl Pts',(-2.16709383120357,-7.83092535365741,
39.8298156733138));
#177931=CARTESIAN_POINT('Ctrl Pts',(-2.16716396271781,-7.83090594545052,
39.8298128142729));
#177932=CARTESIAN_POINT('Ctrl Pts',(-2.16730436858667,-7.83086708747645,
39.8298070903732));
#177933=CARTESIAN_POINT('Ctrl Pts',(-2.16737464284022,-7.8308476377331,
39.8298042255185));
#177934=CARTESIAN_POINT('Ctrl Pts',(-2.16751533335053,-7.83080869690536,
39.8297984900253));
#177935=CARTESIAN_POINT('Ctrl Pts',(-2.16758574963143,-7.83078920581017,
39.8297956193858));
#177936=CARTESIAN_POINT('Ctrl Pts',(-2.16772672343646,-7.83075018247673,
39.829789872354));
#177937=CARTESIAN_POINT('Ctrl Pts',(-2.16779728083816,-7.83073065026824,
39.8297869959668));
#177938=CARTESIAN_POINT('Ctrl Pts',(-2.16793853602321,-7.83069154493438,
39.8297812374746));
#177939=CARTESIAN_POINT('Ctrl Pts',(-2.16800923383181,-7.8306719717979,
39.8297783553687));
#177940=CARTESIAN_POINT('Ctrl Pts',(-2.16815076902445,-7.83063278481895,
39.8297725854722));
#177941=CARTESIAN_POINT('Ctrl Pts',(-2.16822160635381,-7.83061317098751,
39.8297696976838));
#177942=CARTESIAN_POINT('Ctrl Pts',(-2.16836341965642,-7.83057390286432,
39.8297639164604));
#177943=CARTESIAN_POINT('Ctrl Pts',(-2.16843439580468,-7.83055424852003,
39.8297610230182));
#177944=CARTESIAN_POINT('Ctrl Pts',(-2.16857648597554,-7.830514899572,39.8297552305184));
#177945=CARTESIAN_POINT('Ctrl Pts',(-2.16864760000675,-7.83049520496182,
39.8297523314606));
#177946=CARTESIAN_POINT('Ctrl Pts',(-2.16878996522908,-7.83045577566771,
39.8297465277587));
#177947=CARTESIAN_POINT('Ctrl Pts',(-2.16886121638479,-7.83043604098955,
39.8297436231162));
#177948=CARTESIAN_POINT('Ctrl Pts',(-2.16900385509695,-7.83039653175762,
39.829737808276));
#177949=CARTESIAN_POINT('Ctrl Pts',(-2.16907524258471,-7.83037675721885,
39.8297348980811));
#177950=CARTESIAN_POINT('Ctrl Pts',(-2.16921815312932,-7.83033716848402,
39.8297290721702));
#177951=CARTESIAN_POINT('Ctrl Pts',(-2.16928967619349,-7.83031735428191,
39.8297261564538));
#177952=CARTESIAN_POINT('Ctrl Pts',(-2.16943285704856,-7.83027768644172,
39.8297203195342));
#177953=CARTESIAN_POINT('Ctrl Pts',(-2.16950451488789,-7.83025783278623,
39.829717398329));
#177954=CARTESIAN_POINT('Ctrl Pts',(-2.16964796454732,-7.83021808623396,
39.8297115504623));
#177955=CARTESIAN_POINT('Ctrl Pts',(-2.16971975633641,-7.8301981933418,
39.829708623802));
#177956=CARTESIAN_POINT('Ctrl Pts',(-2.16986347300943,-7.83015836854977,
39.8297027650612));
#177957=CARTESIAN_POINT('Ctrl Pts',(-2.16993539805907,-7.8301384366,39.829699832974));
#177958=CARTESIAN_POINT('Ctrl Pts',(-2.17007938066475,-7.83009853384393,
39.8296939634032));
#177959=CARTESIAN_POINT('Ctrl Pts',(-2.17015143800203,-7.83007856309429,
39.8296910259287));
#177960=CARTESIAN_POINT('Ctrl Pts',(-2.17029568439011,-7.8300385829464,
39.8296851456157));
#177961=CARTESIAN_POINT('Ctrl Pts',(-2.170367873445,-7.83001857354307,39.8296822027772));
#177962=CARTESIAN_POINT('Ctrl Pts',(-2.17051238243866,-7.82997851630594,
39.8296763117701));
#177963=CARTESIAN_POINT('Ctrl Pts',(-2.17058470235686,-7.82995846847392,
39.8296733636023));
#177964=CARTESIAN_POINT('Ctrl Pts',(-2.17072947229866,-7.82991833458347,
39.8296674619687));
#177965=CARTESIAN_POINT('Ctrl Pts',(-2.17080192233333,-7.82989824851807,
39.8296645085023));
#177966=CARTESIAN_POINT('Ctrl Pts',(-2.17094695165827,-7.82985803838475,
39.8296585963061));
#177967=CARTESIAN_POINT('Ctrl Pts',(-2.17101953107432,-7.82983791427808,
39.829655637571));
#177968=CARTESIAN_POINT('Ctrl Pts',(-2.17116481847131,-7.82979762824209,
39.8296497148656));
#177969=CARTESIAN_POINT('Ctrl Pts',(-2.17123752641904,-7.8297774663181,
39.8296467508966));
#177970=CARTESIAN_POINT('Ctrl Pts',(-2.17138307014348,-7.82973710483994,
39.8296408177533));
#177971=CARTESIAN_POINT('Ctrl Pts',(-2.17145590593814,-7.82971690527694,
39.8296378485782));
#177972=CARTESIAN_POINT('Ctrl Pts',(-2.17160170465256,-7.82967646870439,
39.8296319050515));
#177973=CARTESIAN_POINT('Ctrl Pts',(-2.17167466749546,-7.82965623171232,
39.829628930703));
#177974=CARTESIAN_POINT('Ctrl Pts',(-2.17182071953564,-7.82961572048391,
39.8296229768609));
#177975=CARTESIAN_POINT('Ctrl Pts',(-2.17189380874019,-7.82959544624172,
39.829619997367));
#177976=CARTESIAN_POINT('Ctrl Pts',(-2.17204011275934,-7.82955486070807,
39.8296140332644));
#177977=CARTESIAN_POINT('Ctrl Pts',(-2.17211332754264,-7.82953454942148,
39.829611048657));
#177978=CARTESIAN_POINT('Ctrl Pts',(-2.17225988202463,-7.82949388998032,
39.8296050743558));
#177979=CARTESIAN_POINT('Ctrl Pts',(-2.17233322164535,-7.82947354184358,
39.8296020846652));
#177980=CARTESIAN_POINT('Ctrl Pts',(-2.17248002498705,-7.82943280891692,
39.8295961002309));
#177981=CARTESIAN_POINT('Ctrl Pts',(-2.17255348877729,-7.829412424104,39.8295931054844));
#177982=CARTESIAN_POINT('Ctrl Pts',(-2.17270053972405,-7.8293716180173,
39.8295871109681));
#177983=CARTESIAN_POINT('Ctrl Pts',(-2.17277412688221,-7.82935119673931,
39.8295841111983));
#177984=CARTESIAN_POINT('Ctrl Pts',(-2.17292142379105,-7.82931031792593,
39.8295781066672));
#177985=CARTESIAN_POINT('Ctrl Pts',(-2.17299513365084,-7.82928986035652,
39.8295751019014));
#177986=CARTESIAN_POINT('Ctrl Pts',(-2.17314267522118,-7.82924890915493,
39.8295690874084));
#177987=CARTESIAN_POINT('Ctrl Pts',(-2.1732165070184,-7.82922841549497,
39.8295660776777));
#177988=CARTESIAN_POINT('Ctrl Pts',(-2.1733642919015,-7.82918739225713,
39.829560053278));
#177989=CARTESIAN_POINT('Ctrl Pts',(-2.17343824485432,-7.82916686271247,
39.8295570386144));
#177990=CARTESIAN_POINT('Ctrl Pts',(-2.17356513994918,-7.82913163434596,
39.8295518657899));
#177991=CARTESIAN_POINT('Ctrl Pts',(-2.17361808209445,-7.82911693607337,
39.8295497076274));
#177992=CARTESIAN_POINT('Ctrl Pts',(-2.17372457475787,-7.82908736946283,
39.8295453665055));
#177993=CARTESIAN_POINT('Ctrl Pts',(-2.1737781252814,-7.82907250111,39.8295431835458));
#177994=CARTESIAN_POINT('Ctrl Pts',(-2.17388583901435,-7.8290425931012,
39.8295387926538));
#177995=CARTESIAN_POINT('Ctrl Pts',(-2.17394000228027,-7.82902755341591,
39.8295365847192));
#177996=CARTESIAN_POINT('Ctrl Pts',(-2.17404894592648,-7.82899730147151,
39.8295321436969));
#177997=CARTESIAN_POINT('Ctrl Pts',(-2.17410372625624,-7.82898208921256,
39.8295299106112));
#177998=CARTESIAN_POINT('Ctrl Pts',(-2.17421390831106,-7.82895149089026,
39.8295254191125));
#177999=CARTESIAN_POINT('Ctrl Pts',(-2.17426931014589,-7.8289361047823,
39.829523160695));
#178000=CARTESIAN_POINT('Ctrl Pts',(-2.17438073957824,-7.82890515750653,
39.8295186183544));
#178001=CARTESIAN_POINT('Ctrl Pts',(-2.17443676714711,-7.8288895963323,
39.8295163344327));
#178002=CARTESIAN_POINT('Ctrl Pts',(-2.17454945247657,-7.82885829765053,
39.8295117409033));
#178003=CARTESIAN_POINT('Ctrl Pts',(-2.17460611008935,-7.8288425601694,
39.8295094313017));
#178004=CARTESIAN_POINT('Ctrl Pts',(-2.17472005965025,-7.82881090767879,
39.829504786244));
#178005=CARTESIAN_POINT('Ctrl Pts',(-2.17477735171328,-7.82879499262247,
39.8295024507831));
#178006=CARTESIAN_POINT('Ctrl Pts',(-2.17489257446465,-7.82876298374484,
39.8294977538321));
#178007=CARTESIAN_POINT('Ctrl Pts',(-2.1749505050794,-7.8287468899288,39.8294953923449));
#178008=CARTESIAN_POINT('Ctrl Pts',(-2.17506700910107,-7.82871452232841,
39.8294906431713));
#178009=CARTESIAN_POINT('Ctrl Pts',(-2.17512558261446,-7.82869824849903,
39.8294882554807));
#178010=CARTESIAN_POINT('Ctrl Pts',(-2.17524337663283,-7.82866551965869,
39.8294834537293));
#178011=CARTESIAN_POINT('Ctrl Pts',(-2.17530259714821,-7.8286490646291,
39.8294810396681));
#178012=CARTESIAN_POINT('Ctrl Pts',(-2.17542168936825,-7.82861597217462,
39.8294761850045));
#178013=CARTESIAN_POINT('Ctrl Pts',(-2.17548156108439,-7.82859933473053,
39.8294737444018));
#178014=CARTESIAN_POINT('Ctrl Pts',(-2.175601959962,-7.82856587621615,39.8294688364816));
#178015=CARTESIAN_POINT('Ctrl Pts',(-2.17566248695237,-7.82854905517712,
39.8294663691713));
#178016=CARTESIAN_POINT('Ctrl Pts',(-2.17578420035632,-7.82851522831838,
39.8294614076742));
#178017=CARTESIAN_POINT('Ctrl Pts',(-2.17584538688022,-7.82849822245142,
39.8294589134828));
#178018=CARTESIAN_POINT('Ctrl Pts',(-2.17596842337759,-7.82846402476786,
39.8294538980597));
#178019=CARTESIAN_POINT('Ctrl Pts',(-2.17603027338683,-7.82844683292446,
39.8294513768264));
#178020=CARTESIAN_POINT('Ctrl Pts',(-2.17615464106193,-7.8284122620679,
39.8294463071479));
#178021=CARTESIAN_POINT('Ctrl Pts',(-2.17621715854566,-7.82839488308822,
39.8294437587102));
#178022=CARTESIAN_POINT('Ctrl Pts',(-2.17634286507707,-7.82835993682135,
39.8294386344637));
#178023=CARTESIAN_POINT('Ctrl Pts',(-2.17640605419629,-7.82834236949683,
39.8294360586521));
#178024=CARTESIAN_POINT('Ctrl Pts',(-2.17653310785606,-7.8283070454154,
39.8294308795007));
#178025=CARTESIAN_POINT('Ctrl Pts',(-2.17659697250595,-7.82828928861037,
39.8294282761566));
#178026=CARTESIAN_POINT('Ctrl Pts',(-2.17672538122505,-7.82825358440302,
39.8294230417773));
#178027=CARTESIAN_POINT('Ctrl Pts',(-2.17678992528318,-7.82823563698575,
39.8294204107426));
#178028=CARTESIAN_POINT('Ctrl Pts',(-2.17691969669401,-7.82819955042213,
39.8294151208246));
#178029=CARTESIAN_POINT('Ctrl Pts',(-2.17698492412455,-7.82818141123582,
39.8294124619381));
#178030=CARTESIAN_POINT('Ctrl Pts',(-2.1771160662694,-7.82814493996965,
39.8294071161538));
#178031=CARTESIAN_POINT('Ctrl Pts',(-2.17718198081471,-7.82812660791818,
39.8294044292629));
#178032=CARTESIAN_POINT('Ctrl Pts',(-2.17731450095326,-7.8280897498188,
39.8293990273167));
#178033=CARTESIAN_POINT('Ctrl Pts',(-2.17738110658052,-7.82807122374252,
39.82939631226));
#178034=CARTESIAN_POINT('Ctrl Pts',(-2.17751501257517,-7.82803397650965,
39.8293908538317));
#178035=CARTESIAN_POINT('Ctrl Pts',(-2.17758231299994,-7.82801525531789,
39.8293881104578));
#178036=CARTESIAN_POINT('Ctrl Pts',(-2.17771761244208,-7.8279776167246,
39.8293825952384));
#178037=CARTESIAN_POINT('Ctrl Pts',(-2.17778561133009,-7.82795869933952,
39.829379823398));
#178038=CARTESIAN_POINT('Ctrl Pts',(-2.1779223113467,-7.82792066728601,
39.8293742510972));
#178039=CARTESIAN_POINT('Ctrl Pts',(-2.17799101250686,-7.82790155258895,
39.8293714506353));
#178040=CARTESIAN_POINT('Ctrl Pts',(-2.17812912067033,-7.82786312484948,
39.8293658209447));
#178041=CARTESIAN_POINT('Ctrl Pts',(-2.17819852769838,-7.82784381178003,
39.8293629917149));
#178042=CARTESIAN_POINT('Ctrl Pts',(-2.17833805122705,-7.82780498622528,
39.8293573043406));
#178043=CARTESIAN_POINT('Ctrl Pts',(-2.178408167723,-7.82778547372082,39.8293544461963));
#178044=CARTESIAN_POINT('Ctrl Pts',(-2.17854911369094,-7.82774624825957,
39.8293487008504));
#178045=CARTESIAN_POINT('Ctrl Pts',(-2.17861994326358,-7.827726535254,39.8293458136447));
#178046=CARTESIAN_POINT('Ctrl Pts',(-2.17876231903963,-7.82768690771089,
39.829340010027));
#178047=CARTESIAN_POINT('Ctrl Pts',(-2.17883386508615,-7.82766699319594,
39.8293370936215));
#178048=CARTESIAN_POINT('Ctrl Pts',(-2.17897767725032,-7.82762696161307,
39.8293312314643));
#178049=CARTESIAN_POINT('Ctrl Pts',(-2.17904994339091,-7.82760684451737,
39.8293282857117));
#178050=CARTESIAN_POINT('Ctrl Pts',(-2.17919519912821,-7.82756640676634,
39.8293223647224));
#178051=CARTESIAN_POINT('Ctrl Pts',(-2.17926818871999,-7.82754608609068,
39.8293193894859));
#178052=CARTESIAN_POINT('Ctrl Pts',(-2.17941489469947,-7.82750524018461,
39.8293134093931));
#178053=CARTESIAN_POINT('Ctrl Pts',(-2.17948861115696,-7.82748471491273,
39.8293104045338));
#178054=CARTESIAN_POINT('Ctrl Pts',(-2.17963677435974,-7.82744345877572,
39.8293043650532));
#178055=CARTESIAN_POINT('Ctrl Pts',(-2.17971122089749,-7.827422727946,39.8293013304403));
#178056=CARTESIAN_POINT('Ctrl Pts',(-2.17986084748517,-7.82738105972819,
39.8292952313211));
#178057=CARTESIAN_POINT('Ctrl Pts',(-2.1799360275581,-7.82736012231101,
39.8292921668139));
#178058=CARTESIAN_POINT('Ctrl Pts',(-2.18008712435711,-7.8273180399753,
39.8292860077783));
#178059=CARTESIAN_POINT('Ctrl Pts',(-2.18016304113141,-7.82729689502034,
39.8292829132479));
#178060=CARTESIAN_POINT('Ctrl Pts',(-2.18031561457832,-7.82725439663604,
39.8292766940339));
#178061=CARTESIAN_POINT('Ctrl Pts',(-2.1803922711972,-7.82723304319832,
39.8292735693524));
#178062=CARTESIAN_POINT('Ctrl Pts',(-2.18054632750404,-7.82719012689511,
39.8292672897072));
#178063=CARTESIAN_POINT('Ctrl Pts',(-2.18062372713733,-7.82716856402118,
39.8292641347456));
#178064=CARTESIAN_POINT('Ctrl Pts',(-2.18077927237866,-7.82712522796489,
39.8292577944219));
#178065=CARTESIAN_POINT('Ctrl Pts',(-2.18085741820314,-7.82710345469824,
39.8292546090509));
#178066=CARTESIAN_POINT('Ctrl Pts',(-2.18101445892962,-7.82705969691989,
39.8292482077822));
#178067=CARTESIAN_POINT('Ctrl Pts',(-2.18109335380842,-7.82703771239033,
39.8292449918853));
#178068=CARTESIAN_POINT('Ctrl Pts',(-2.18125189566308,-7.82699353117163,
39.8292385294419));
#178069=CARTESIAN_POINT('Ctrl Pts',(-2.18133154268146,-7.82697133444599,
39.8292352828936));
#178070=CARTESIAN_POINT('Ctrl Pts',(-2.18149159181669,-7.82692672792455,
39.8292287590251));
#178071=CARTESIAN_POINT('Ctrl Pts',(-2.18157199383644,-7.82690431813084,
39.829225481709));
#178072=CARTESIAN_POINT('Ctrl Pts',(-2.18173355587189,-7.82685928459056,
39.8292188961868));
#178073=CARTESIAN_POINT('Ctrl Pts',(-2.181814715832,-7.82683666083416,39.8292155879832));
#178074=CARTESIAN_POINT('Ctrl Pts',(-2.1819777965221,-7.82679119851917,
39.8292089405733));
#178075=CARTESIAN_POINT('Ctrl Pts',(-2.18205971725393,-7.8267683599344,
39.829205601367));
#178076=CARTESIAN_POINT('Ctrl Pts',(-2.18222432225902,-7.82672246711287,
39.8291988918389));
#178077=CARTESIAN_POINT('Ctrl Pts',(-2.18230700650684,-7.82669941285721,
39.8291955215183));
#178078=CARTESIAN_POINT('Ctrl Pts',(-2.18247314122627,-7.82665308786786,
39.8291887496526));
#178079=CARTESIAN_POINT('Ctrl Pts',(-2.18255659173976,-7.82662981709617,
39.8291853481058));
#178080=CARTESIAN_POINT('Ctrl Pts',(-2.1827242616678,-7.82658305824907,
39.8291785136788));
#178081=CARTESIAN_POINT('Ctrl Pts',(-2.18280848107302,-7.8265595701496,
39.8291750807991));
#178082=CARTESIAN_POINT('Ctrl Pts',(-2.18297769139592,-7.8265123758385,
39.8291681836));
#178083=CARTESIAN_POINT('Ctrl Pts',(-2.18306268232895,-7.82648866959559,
39.82916471928));
#178084=CARTESIAN_POINT('Ctrl Pts',(-2.18323343819188,-7.8264410382235,
39.8291577590994));
#178085=CARTESIAN_POINT('Ctrl Pts',(-2.18331920323313,-7.82641711303592,
39.8291542632344));
#178086=CARTESIAN_POINT('Ctrl Pts',(-2.18349151003716,-7.82636904293224,
39.8291472398527));
#178087=CARTESIAN_POINT('Ctrl Pts',(-2.1835780515284,-7.82634489806422,
39.8291437123472));
#178088=CARTESIAN_POINT('Ctrl Pts',(-2.18375191356705,-7.82629638786513,
39.8291366255899));
#178089=CARTESIAN_POINT('Ctrl Pts',(-2.18383923420451,-7.82627202248092,
39.8291330663345));
#178090=CARTESIAN_POINT('Ctrl Pts',(-2.18401465689354,-7.8262230705073,
39.8291259159812));
#178091=CARTESIAN_POINT('Ctrl Pts',(-2.18410275890438,-7.8261984839009,
39.8291223248852));
#178092=CARTESIAN_POINT('Ctrl Pts',(-2.18427974664506,-7.82614908875446,
39.8291151107572));
#178093=CARTESIAN_POINT('Ctrl Pts',(-2.18436863244871,-7.82612428016514,
39.8291114877222));
#178094=CARTESIAN_POINT('Ctrl Pts',(-2.18454719004913,-7.82607444033188,
39.8291042096239));
#178095=CARTESIAN_POINT('Ctrl Pts',(-2.18463686187345,-7.82604940905124,
39.8291005545595));
#178096=CARTESIAN_POINT('Ctrl Pts',(-2.18481699381708,-7.82599912310556,
39.8290932123086));
#178097=CARTESIAN_POINT('Ctrl Pts',(-2.18490745387324,-7.82597386842877,
39.8290895251248));
#178098=CARTESIAN_POINT('Ctrl Pts',(-2.18508916441082,-7.82592313500779,
39.8290821185486));
#178099=CARTESIAN_POINT('Ctrl Pts',(-2.18518041493717,-7.82589765622135,
39.8290783991545));
#178100=CARTESIAN_POINT('Ctrl Pts',(-2.18536370855264,-7.82584647389493,
39.8290709280708));
#178101=CARTESIAN_POINT('Ctrl Pts',(-2.18545575159851,-7.82582077033697,
39.8290671763831));
#178102=CARTESIAN_POINT('Ctrl Pts',(-2.18564063231989,-7.82576913780003,
39.8290596406282));
#178103=CARTESIAN_POINT('Ctrl Pts',(-2.18573346998756,-7.82574320879284,
39.8290558565614));
#178104=CARTESIAN_POINT('Ctrl Pts',(-2.18591994196658,-7.82569112470357,
39.8290482559666));
#178105=CARTESIAN_POINT('Ctrl Pts',(-2.1860135762373,-7.82566496960211,
39.8290444394403));
#178106=CARTESIAN_POINT('Ctrl Pts',(-2.18620164333323,-7.8256124326982,
39.8290367738488));
#178107=CARTESIAN_POINT('Ctrl Pts',(-2.18629607619411,-7.82558605085471,
39.8290329247823));
#178108=CARTESIAN_POINT('Ctrl Pts',(-2.18648574237248,-7.82553305984195,
39.8290251940331));
#178109=CARTESIAN_POINT('Ctrl Pts',(-2.18658097567478,-7.82550645064551,
39.8290213123511));
#178110=CARTESIAN_POINT('Ctrl Pts',(-2.18677224462759,-7.82545300430393,
39.8290135162943));
#178111=CARTESIAN_POINT('Ctrl Pts',(-2.18686828021034,-7.82542616714597,
39.8290096019222));
#178112=CARTESIAN_POINT('Ctrl Pts',(-2.18706115544613,-7.82537226430469,
39.8290017404152));
#178113=CARTESIAN_POINT('Ctrl Pts',(-2.18715799515145,-7.82534519857466,
39.8289977932782));
#178114=CARTESIAN_POINT('Ctrl Pts',(-2.18735248031133,-7.82529083802356,
39.8289898661732));
#178115=CARTESIAN_POINT('Ctrl Pts',(-2.18745012583376,-7.82526354315109,
39.8289858862025));
#178116=CARTESIAN_POINT('Ctrl Pts',(-2.1876462243892,-7.82520872372528,
39.8289778933587));
#178117=CARTESIAN_POINT('Ctrl Pts',(-2.18774467735244,-7.82518119915869,
39.8289738804884));
#178118=CARTESIAN_POINT('Ctrl Pts',(-2.1879423924795,-7.82512591977371,
39.8289658217768));
#178119=CARTESIAN_POINT('Ctrl Pts',(-2.18804165453847,-7.82509816495153,
39.8289617759398));
#178120=CARTESIAN_POINT('Ctrl Pts',(-2.18824098937266,-7.82504242453209,
39.8289536512331));
#178121=CARTESIAN_POINT('Ctrl Pts',(-2.18834106213754,-7.82501443890428,
39.8289495723641));
#178122=CARTESIAN_POINT('Ctrl Pts',(-2.18854201987731,-7.82495823635534,
39.8289413815327));
#178123=CARTESIAN_POINT('Ctrl Pts',(-2.18864290482272,-7.82493001940868,
39.8289372695717));
#178124=CARTESIAN_POINT('Ctrl Pts',(-2.18884548831427,-7.82487335373156,
39.8289290125002));
#178125=CARTESIAN_POINT('Ctrl Pts',(-2.18894718694298,-7.82484490494389,
39.8289248673864));
#178126=CARTESIAN_POINT('Ctrl Pts',(-2.18915139921468,-7.82478777508681,
39.8289165439519));
#178127=CARTESIAN_POINT('Ctrl Pts',(-2.1892539128725,-7.82475909397881,
39.8289123656308));
#178128=CARTESIAN_POINT('Ctrl Pts',(-2.1894597565891,-7.82470149898959,
39.8289039757253));
#178129=CARTESIAN_POINT('Ctrl Pts',(-2.1895630866467,-7.82467258507391,
39.8288997641412));
#178130=CARTESIAN_POINT('Ctrl Pts',(-2.1897705644194,-7.82461452401322,
39.828891307659));
#178131=CARTESIAN_POINT('Ctrl Pts',(-2.18987471220733,-7.8245853768127,
39.828887062758));
#178132=CARTESIAN_POINT('Ctrl Pts',(-2.190083826865,-7.82452684867818,39.8288785395843));
#178133=CARTESIAN_POINT('Ctrl Pts',(-2.19018879350566,-7.82449746777283,
39.8288742613211));
#178134=CARTESIAN_POINT('Ctrl Pts',(-2.19039954697668,-7.82443847181203,
39.828865671378));
#178135=CARTESIAN_POINT('Ctrl Pts',(-2.19050533386394,-7.82440885670487,
39.828861359696));
#178136=CARTESIAN_POINT('Ctrl Pts',(-2.19071772889649,-7.8243493919338,
39.8288527028721));
#178137=CARTESIAN_POINT('Ctrl Pts',(-2.19082433707031,-7.82431954222581,
39.8288483577293));
#178138=CARTESIAN_POINT('Ctrl Pts',(-2.21080074354796,-7.81872581693615,
39.8280341593126));
#178139=CARTESIAN_POINT('Ctrl Pts',(-2.23064931950368,-7.81308626249394,
39.8272254034176));
#178140=CARTESIAN_POINT('Ctrl Pts',(-2.26783679034714,-7.8023669668516,
39.8257107047351));
#178141=CARTESIAN_POINT('Ctrl Pts',(-2.28518064861989,-7.79730488056071,
39.825004493789));
#178142=CARTESIAN_POINT('Ctrl Pts',(-2.33265394550703,-7.78327702770808,
39.8230721870066));
#178143=CARTESIAN_POINT('Ctrl Pts',(-2.36274850212809,-7.77419418642854,
39.8218479991728));
#178144=CARTESIAN_POINT('Ctrl Pts',(-2.50354086373117,-7.73080857813394,
39.8161222314859));
#178145=CARTESIAN_POINT('Ctrl Pts',(-2.61355021155178,-7.6943143865977,
39.8116521764866));
#178146=CARTESIAN_POINT('Ctrl Pts',(-3.02176321312957,-7.54912965435448,
39.7950005510652));
#178147=CARTESIAN_POINT('Ctrl Pts',(-3.31429661051441,-7.42535188935789,
39.7829240683185));
#178148=CARTESIAN_POINT('Ctrl Pts',(-3.68355772473503,-7.24292887832528,
39.767079830347));
#178149=CARTESIAN_POINT('Ctrl Pts',(-3.76753836991228,-7.19960212234876,
39.7634354675164));
#178150=CARTESIAN_POINT('Ctrl Pts',(-3.91598720521225,-7.11970655789409,
39.7569106956654));
#178151=CARTESIAN_POINT('Ctrl Pts',(-3.9807469209437,-7.08370179507006,
39.7540355427547));
#178152=CARTESIAN_POINT('Ctrl Pts',(-4.08028154438181,-7.02656705409377,
39.7495687932789));
#178153=CARTESIAN_POINT('Ctrl Pts',(-4.11540557468927,-7.00605302483863,
39.7479832149848));
#178154=CARTESIAN_POINT('Ctrl Pts',(-4.17862274511229,-6.96849188993833,
39.7451120882393));
#178155=CARTESIAN_POINT('Ctrl Pts',(-4.20676935586562,-6.95153643765855,
39.7438274632443));
#178156=CARTESIAN_POINT('Ctrl Pts',(-4.27005236105911,-6.91288980170372,
39.7409247364454));
#178157=CARTESIAN_POINT('Ctrl Pts',(-4.30512778280207,-6.89110058942634,
39.7393057048506));
#178158=CARTESIAN_POINT('Ctrl Pts',(-4.40567795364597,-6.82757046108686,
39.7346346850221));
#178159=CARTESIAN_POINT('Ctrl Pts',(-4.47072221078912,-6.785157289266,39.7315763171149));
#178160=CARTESIAN_POINT('Ctrl Pts',(-4.64483531312543,-6.66803329234237,
39.7232884877699));
#178161=CARTESIAN_POINT('Ctrl Pts',(-4.75270461248176,-6.59158262676681,
39.7180441076068));
#178162=CARTESIAN_POINT('Ctrl Pts',(-5.04186857747583,-6.37585258856342,
39.7036902037643));
#178163=CARTESIAN_POINT('Ctrl Pts',(-5.21922735953489,-6.23150065531565,
39.6945538642326));
#178164=CARTESIAN_POINT('Ctrl Pts',(-5.44162917706752,-6.03432446338089,
39.6827292205568));
#178165=CARTESIAN_POINT('Ctrl Pts',(-5.49241576650423,-5.98813568194523,
39.6800029015519));
#178166=CARTESIAN_POINT('Ctrl Pts',(-5.56791879952114,-5.9176993575639,
39.6759139053764));
#178167=CARTESIAN_POINT('Ctrl Pts',(-5.59307544350426,-5.89392844716465,
39.6745453805691));
#178168=CARTESIAN_POINT('Ctrl Pts',(-5.63686501069081,-5.85201816168369,
39.6721530789692));
#178169=CARTESIAN_POINT('Ctrl Pts',(-5.65556414987715,-5.83394873703186,
39.6711282232715));
#178170=CARTESIAN_POINT('Ctrl Pts',(-5.68856969444956,-5.80174687219388,
39.6693137029558));
#178171=CARTESIAN_POINT('Ctrl Pts',(-5.70291096838506,-5.78765051014218,
39.6685233886861));
#178172=CARTESIAN_POINT('Ctrl Pts',(-5.73045188577533,-5.76037816248689,
39.6670021805882));
#178173=CARTESIAN_POINT('Ctrl Pts',(-5.74365877919381,-5.7472096901385,
39.6662711493347));
#178174=CARTESIAN_POINT('Ctrl Pts',(-5.77682943181101,-5.71390700000489,
39.6644312369548));
#178175=CARTESIAN_POINT('Ctrl Pts',(-5.79673336005715,-5.69371353783658,
39.6633236240303));
#178176=CARTESIAN_POINT('Ctrl Pts',(-5.8731262452021,-5.61539360085841,
39.6590577573738));
#178177=CARTESIAN_POINT('Ctrl Pts',(-5.92885029447873,-5.55652693334649,
39.655914627342));
#178178=CARTESIAN_POINT('Ctrl Pts',(-6.2672918596412,-5.18810997591716,
39.6365957456872));
#178179=CARTESIAN_POINT('Ctrl Pts',(-6.52658519441173,-4.85789336847288,
39.620770287007));
#178180=CARTESIAN_POINT('Ctrl Pts',(-6.99462319292796,-4.15630089341364,
39.5887171053279));
#178181=CARTESIAN_POINT('Ctrl Pts',(-7.20201354171842,-3.78557541896965,
39.5725300128041));
#178182=CARTESIAN_POINT('Ctrl Pts',(-7.4018062149867,-3.35198302043742,
39.5539859670726));
#178183=CARTESIAN_POINT('Ctrl Pts',(-7.4236235778997,-3.3033828655158,39.5519130455387));
#178184=CARTESIAN_POINT('Ctrl Pts',(-7.46045253399993,-3.21913517609428,
39.5483286639629));
#178185=CARTESIAN_POINT('Ctrl Pts',(-7.47569045822439,-3.1835884556694,
39.546819039659));
#178186=CARTESIAN_POINT('Ctrl Pts',(-7.50549377912414,-3.11266989951469,
39.5438124010645));
#178187=CARTESIAN_POINT('Ctrl Pts',(-7.52006433329674,-3.07730128257048,
39.5423154668215));
#178188=CARTESIAN_POINT('Ctrl Pts',(-7.54844025853394,-3.00701627285619,
39.539345562679));
#178189=CARTESIAN_POINT('Ctrl Pts',(-7.56225445162001,-2.97210443971392,
39.5378726966557));
#178190=CARTESIAN_POINT('Ctrl Pts',(-7.59288346851263,-2.89310125603126,
39.5345447924184));
#178191=CARTESIAN_POINT('Ctrl Pts',(-7.60955715573164,-2.84895667188855,
39.5326888154104));
#178192=CARTESIAN_POINT('Ctrl Pts',(-7.66694852514242,-2.6929105804216,
39.5261402518591));
#178193=CARTESIAN_POINT('Ctrl Pts',(-7.70558977749548,-2.58026219475194,
39.5214345800578));
#178194=CARTESIAN_POINT('Ctrl Pts',(-7.93100723669749,-1.87281958140106,
39.4920136738859));
#178195=CARTESIAN_POINT('Ctrl Pts',(-8.05127663399291,-1.25905660289138,
39.4669951067845));
#178196=CARTESIAN_POINT('Ctrl Pts',(-8.14033006716474,-0.127718535303896,
39.4195089625374));
#178197=CARTESIAN_POINT('Ctrl Pts',(-8.13223161532385,0.384803107321045,
39.3975519182653));
#178198=CARTESIAN_POINT('Ctrl Pts',(-8.05880298280382,1.04875732503032,
39.3698639516156));
#178199=CARTESIAN_POINT('Ctrl Pts',(-8.0370995506624,1.20384018408007,39.3634622230776));
#178200=CARTESIAN_POINT('Ctrl Pts',(-8.00591166621803,1.38779199831945,
39.3560140780603));
#178201=CARTESIAN_POINT('Ctrl Pts',(-8.00073110030372,1.41735321167889,
39.3548216879439));
#178202=CARTESIAN_POINT('Ctrl Pts',(-7.99340680751234,1.45782674158068,
39.353195959149));
#178203=CARTESIAN_POINT('Ctrl Pts',(-7.99140431983574,1.46876417347065,
39.3527573118923));
#178204=CARTESIAN_POINT('Ctrl Pts',(-7.98800569133949,1.48711450017874,
39.3520225568526));
#178205=CARTESIAN_POINT('Ctrl Pts',(-7.98662167113063,1.4945296063384,39.3517259784986));
#178206=CARTESIAN_POINT('Ctrl Pts',(-7.98387773655974,1.50911800574823,
39.3511431488239));
#178207=CARTESIAN_POINT('Ctrl Pts',(-7.98251847571596,1.51629141424244,
39.3508568718564));
#178208=CARTESIAN_POINT('Ctrl Pts',(-7.97952028349018,1.53199840587013,
39.3502307340822));
#178209=CARTESIAN_POINT('Ctrl Pts',(-7.97787732642742,1.54053121859241,
39.349891036781));
#178210=CARTESIAN_POINT('Ctrl Pts',(-7.97218250784277,1.56985422008605,
39.3487252589104));
#178211=CARTESIAN_POINT('Ctrl Pts',(-7.96806301912931,1.59063130400415,
39.347901987745));
#178212=CARTESIAN_POINT('Ctrl Pts',(-7.90966495723687,1.879247652144,39.3365064246268));
#178213=CARTESIAN_POINT('Ctrl Pts',(-7.84198957560371,2.14419451368648,
39.3265982952413));
#178214=CARTESIAN_POINT('Ctrl Pts',(-7.62116266974008,2.85674971452128,
39.3005436146682));
#178215=CARTESIAN_POINT('Ctrl Pts',(-7.44209265334162,3.29521284361814,
39.2851093655004));
#178216=CARTESIAN_POINT('Ctrl Pts',(-6.94639615476124,4.25921113486542,
39.2487269731623));
#178217=CARTESIAN_POINT('Ctrl Pts',(-6.60647419115726,4.76945478166142,
39.2274971347593));
#178218=CARTESIAN_POINT('Ctrl Pts',(-6.1942304959262,5.25851755566576,39.2028609958781));
#178219=CARTESIAN_POINT('Ctrl Pts',(-6.17576484996748,5.28019193005629,
39.2017598645026));
#178220=CARTESIAN_POINT('Ctrl Pts',(-6.14873421471051,5.31158383965963,
39.2001513385859));
#178221=CARTESIAN_POINT('Ctrl Pts',(-6.14025922797868,5.32137876308843,
39.1996474865322));
#178222=CARTESIAN_POINT('Ctrl Pts',(-6.12537852284956,5.33849418249886,
39.1987636185115));
#178223=CARTESIAN_POINT('Ctrl Pts',(-6.11898300182386,5.34582352938619,
39.1983840059675));
#178224=CARTESIAN_POINT('Ctrl Pts',(-6.10656431222097,5.36000401864025,
39.1976473830777));
#178225=CARTESIAN_POINT('Ctrl Pts',(-6.10054273522479,5.36685653937149,
39.1972904360502));
#178226=CARTESIAN_POINT('Ctrl Pts',(-6.08617890577347,5.38314708687933,
39.1964395110524));
#178227=CARTESIAN_POINT('Ctrl Pts',(-6.07782623232217,5.39257587058624,
39.1959451187171));
#178228=CARTESIAN_POINT('Ctrl Pts',(-6.04807675668433,5.42600117620617,
39.1941857499752));
#178229=CARTESIAN_POINT('Ctrl Pts',(-6.02655962286843,5.44988993486056,
39.1929159693117));
#178230=CARTESIAN_POINT('Ctrl Pts',(-5.67630873194198,5.83413481687002,
39.172289487356));
#178231=CARTESIAN_POINT('Ctrl Pts',(-5.31596416505834,6.1642548336654,39.1515908810326));
#178232=CARTESIAN_POINT('Ctrl Pts',(-4.80596876738529,6.553319860956,39.1232821619198));
#178233=CARTESIAN_POINT('Ctrl Pts',(-4.68108033619358,6.64310337415656,
39.1164264849211));
#178234=CARTESIAN_POINT('Ctrl Pts',(-4.47782224747682,6.78064850313609,
39.1054333653861));
#178235=CARTESIAN_POINT('Ctrl Pts',(-4.40105982948991,6.830721665907,39.1013177998181));
#178236=CARTESIAN_POINT('Ctrl Pts',(-4.02643373674881,7.06615840036962,
39.0814404921693));
#178237=CARTESIAN_POINT('Ctrl Pts',(-3.7176128548317,7.23340398818993,39.065665669073));
#178238=CARTESIAN_POINT('Ctrl Pts',(-3.21207764323464,7.4662285892181,39.0416262750269));
#178239=CARTESIAN_POINT('Ctrl Pts',(-3.02199307797236,7.54516986998229,
39.0329685035316));
#178240=CARTESIAN_POINT('Ctrl Pts',(-2.79364619224551,7.62998417493303,
39.0231550531384));
#178241=CARTESIAN_POINT('Ctrl Pts',(-2.75810527558184,7.64290343483283,
39.0216433411657));
#178242=CARTESIAN_POINT('Ctrl Pts',(-2.71069127494805,7.65976480006877,
39.0196460350253));
#178243=CARTESIAN_POINT('Ctrl Pts',(-2.69889779933894,7.66392814759418,
39.0191508293896));
#178244=CARTESIAN_POINT('Ctrl Pts',(-2.67946956959745,7.67073631868657,
39.0183375982761));
#178245=CARTESIAN_POINT('Ctrl Pts',(-2.67184042521701,7.67339700445627,
39.0180189035023));
#178246=CARTESIAN_POINT('Ctrl Pts',(-2.6570130716723,7.6785432922786,39.0174007530652));
#178247=CARTESIAN_POINT('Ctrl Pts',(-2.64981531387917,7.68103016250182,
39.0171012451035));
#178248=CARTESIAN_POINT('Ctrl Pts',(-2.63313331164547,7.68676765894157,
39.0164083754198));
#178249=CARTESIAN_POINT('Ctrl Pts',(-2.62364651481158,7.69001086123238,
39.0160153157868));
#178250=CARTESIAN_POINT('Ctrl Pts',(-2.5937980755633,7.70015332965275,39.0147815971318));
#178251=CARTESIAN_POINT('Ctrl Pts',(-2.57341494957766,7.70698937749371,
39.0139434468122));
#178252=CARTESIAN_POINT('Ctrl Pts',(-2.37318488798664,7.77325917847878,
39.0057506887219));
#178253=CARTESIAN_POINT('Ctrl Pts',(-2.19133161432705,7.82647020614236,
38.9986300272372));
#178254=CARTESIAN_POINT('Ctrl Pts',(-1.59997415219955,7.97727334479463,
38.9761003291139));
#178255=CARTESIAN_POINT('Ctrl Pts',(-1.1846960634733,8.04942993408061,38.9611945069414));
#178256=CARTESIAN_POINT('Ctrl Pts',(-0.466645763163058,8.11739846189286,
38.9352016274706));
#178257=CARTESIAN_POINT('Ctrl Pts',(-0.166270535428642,8.12909976743459,
38.9242725170387));
#178258=CARTESIAN_POINT('Ctrl Pts',(0.372946335110583,8.12020209798196,
38.9041827851706));
#178259=CARTESIAN_POINT('Ctrl Pts',(0.611538127078164,8.10572554099386,
38.8951304917143));
#178260=CARTESIAN_POINT('Ctrl Pts',(0.894796380222606,8.07596028686548,
38.8841469783617));
#178261=CARTESIAN_POINT('Ctrl Pts',(0.940411408907324,8.07077576570451,
38.8823710529108));
#178262=CARTESIAN_POINT('Ctrl Pts',(1.01140198766865,8.06209709233737,38.8795960123034));
#178263=CARTESIAN_POINT('Ctrl Pts',(1.03680923264027,8.05886903452129,38.8786006036997));
#178264=CARTESIAN_POINT('Ctrl Pts',(1.08376294110711,8.05267772003594,38.8767569378992));
#178265=CARTESIAN_POINT('Ctrl Pts',(1.10531363264755,8.04974796776937,38.8759091437725));
#178266=CARTESIAN_POINT('Ctrl Pts',(1.15122654221731,8.0433183928796,38.8740995060946));
#178267=CARTESIAN_POINT('Ctrl Pts',(1.1755851650669,8.03979432788134,38.8731373350038));
#178268=CARTESIAN_POINT('Ctrl Pts',(1.24076640661903,8.03006172458242,38.8705568025145));
#178269=CARTESIAN_POINT('Ctrl Pts',(1.28155821572863,8.02365260260789,38.8689356848157));
#178270=CARTESIAN_POINT('Ctrl Pts',(1.46536826638818,7.99333528642364,38.8616010472481));
#178271=CARTESIAN_POINT('Ctrl Pts',(1.60777737506264,7.96591260974251,38.8558362765378));
#178272=CARTESIAN_POINT('Ctrl Pts',(1.88024380044932,7.90584152130384,38.8446220005729));
#178273=CARTESIAN_POINT('Ctrl Pts',(2.01037725672817,7.87375571543561,38.8391835136085));
#178274=CARTESIAN_POINT('Ctrl Pts',(2.36067167923866,7.77813632074388,38.8243078955258));
#178275=CARTESIAN_POINT('Ctrl Pts',(2.5790313095104,7.70848675196743,38.8147756178591));
#178276=CARTESIAN_POINT('Ctrl Pts',(3.04706937102918,7.53708184172281,38.7938161458616));
#178277=CARTESIAN_POINT('Ctrl Pts',(3.29522364002373,7.43194003210416,38.7823610311762));
#178278=CARTESIAN_POINT('Ctrl Pts',(3.78529660430662,7.19491936498721,38.7592837995907));
#178279=CARTESIAN_POINT('Ctrl Pts',(4.02666577315459,7.0626698419597,38.7476782488455));
#178280=CARTESIAN_POINT('Ctrl Pts',(4.35602448774592,6.85982708395537,38.7318200207872));
#178281=CARTESIAN_POINT('Ctrl Pts',(4.44996492774435,6.79926395421352,38.7272953178517));
#178282=CARTESIAN_POINT('Ctrl Pts',(4.55729241029078,6.72689276440429,38.7221465314803));
#178283=CARTESIAN_POINT('Ctrl Pts',(4.57192437164105,6.7169567456133,38.7214450553498));
#178284=CARTESIAN_POINT('Ctrl Pts',(4.59413157391607,6.70177048157487,38.7203812348059));
#178285=CARTESIAN_POINT('Ctrl Pts',(4.60173046936383,6.69655502436361,38.7200173622722));
#178286=CARTESIAN_POINT('Ctrl Pts',(4.61549132842539,6.68707585631193,38.7193587130828));
#178287=CARTESIAN_POINT('Ctrl Pts',(4.62165629382854,6.68281653294731,38.7190637387434));
#178288=CARTESIAN_POINT('Ctrl Pts',(4.63397042472076,6.67428361255352,38.718474769448));
#178289=CARTESIAN_POINT('Ctrl Pts',(4.6401195918153,6.67001003088353,38.7181807742692));
#178290=CARTESIAN_POINT('Ctrl Pts',(4.65742011509124,6.65795091606179,38.7173539591712));
#178291=CARTESIAN_POINT('Ctrl Pts',(4.66855787503468,6.65014585550233,38.7168220608693));
#178292=CARTESIAN_POINT('Ctrl Pts',(4.71436446408398,6.61787396437697,38.7146362753966));
#178293=CARTESIAN_POINT('Ctrl Pts',(4.74886137634211,6.59316341589212,38.7129943441616));
#178294=CARTESIAN_POINT('Ctrl Pts',(5.42577333761911,6.10021423977058,38.6808821688189));
#178295=CARTESIAN_POINT('Ctrl Pts',(5.99628020856969,5.54043843477751,38.6557683994322));
#178296=CARTESIAN_POINT('Ctrl Pts',(6.69034224076001,4.62433826554945,38.616440448427));
#178297=CARTESIAN_POINT('Ctrl Pts',(6.88556393405946,4.32829877959735,38.6039893486984));
#178298=CARTESIAN_POINT('Ctrl Pts',(7.13490096290407,3.89040867536051,38.5853271585033));
#178299=CARTESIAN_POINT('Ctrl Pts',(7.20535340390675,3.75832024706725,38.579671258999));
#178300=CARTESIAN_POINT('Ctrl Pts',(7.2823530659317,3.60382409685525,38.5730055821192));
#178301=CARTESIAN_POINT('Ctrl Pts',(7.29250338161553,3.58323997478331,38.57211649349));
#178302=CARTESIAN_POINT('Ctrl Pts',(7.30776695201863,3.55195304356195,38.5707635452649));
#178303=CARTESIAN_POINT('Ctrl Pts',(7.31294424068456,3.54128151661286,38.5703017973906));
#178304=CARTESIAN_POINT('Ctrl Pts',(7.32226615092641,3.52195939609975,38.5694652358078));
#178305=CARTESIAN_POINT('Ctrl Pts',(7.32641886046876,3.51331271778877,38.5690906890524));
#178306=CARTESIAN_POINT('Ctrl Pts',(7.33467399100099,3.49604578728306,38.5683423673731));
#178307=CARTESIAN_POINT('Ctrl Pts',(7.33877655070547,3.48742561772021,38.5679685977979));
#178308=CARTESIAN_POINT('Ctrl Pts',(7.35023305430371,3.46324383408953,38.5669195529469));
#178309=CARTESIAN_POINT('Ctrl Pts',(7.357552738207,3.44766609564364,38.5662431565377));
#178310=CARTESIAN_POINT('Ctrl Pts',(7.38714904733828,3.38415577281091,38.5634829593133));
#178311=CARTESIAN_POINT('Ctrl Pts',(7.4090069631374,3.33603013089226,38.5613855175646));
#178312=CARTESIAN_POINT('Ctrl Pts',(7.81088301153502,2.42776552140212,38.5216849519242));
#178313=CARTESIAN_POINT('Ctrl Pts',(8.03915329819708,1.50839263913174,38.4785037434441));
#178314=CARTESIAN_POINT('Ctrl Pts',(8.11850364623492,0.381530010391947,
38.4281981582461));
#178315=CARTESIAN_POINT('Ctrl Pts',(8.1251981936157,0.191901387828279,38.4198586473823));
#178316=CARTESIAN_POINT('Ctrl Pts',(8.12530306403275,-0.194326991398393,
38.4033160972334));
#178317=CARTESIAN_POINT('Ctrl Pts',(8.11822602146989,-0.390818134096953,
38.3951409940692));
#178318=CARTESIAN_POINT('Ctrl Pts',(8.10272852959197,-0.604814845761113,
38.3865972702528));
#178319=CARTESIAN_POINT('Ctrl Pts',(8.10137078755534,-0.622737498371618,
38.3858842035754));
#178320=CARTESIAN_POINT('Ctrl Pts',(8.09922980642979,-0.649806406752644,
38.3848108126932));
#178321=CARTESIAN_POINT('Ctrl Pts',(8.09849052636613,-0.658956006821622,
38.3844486102723));
#178322=CARTESIAN_POINT('Ctrl Pts',(8.09718030352606,-0.67483651734461,
38.3838209935984));
#178323=CARTESIAN_POINT('Ctrl Pts',(8.0966164701167,-0.68156799307307,38.3835552822289));
#178324=CARTESIAN_POINT('Ctrl Pts',(8.09542535404545,-0.69557837460763,
38.3830029125989));
#178325=CARTESIAN_POINT('Ctrl Pts',(8.09479664715481,-0.702857154612624,
38.3827163132664));
#178326=CARTESIAN_POINT('Ctrl Pts',(8.09329245903785,-0.720001972001027,
38.3820420988152));
#178327=CARTESIAN_POINT('Ctrl Pts',(8.09240875190378,-0.729867289602332,
38.3816548167233));
#178328=CARTESIAN_POINT('Ctrl Pts',(8.0894560857593,-0.762164866655926,
38.3803890337384));
#178329=CARTESIAN_POINT('Ctrl Pts',(8.08731186458667,-0.784590252826219,
38.3795135051035));
#178330=CARTESIAN_POINT('Ctrl Pts',(8.04959315081964,-1.16247888389211,
38.3648124580738));
#178331=CARTESIAN_POINT('Ctrl Pts',(7.99070460628798,-1.51524869881281,
38.3518484376183));
#178332=CARTESIAN_POINT('Ctrl Pts',(7.76002544546271,-2.49451799077964,
38.3156875430688));
#178333=CARTESIAN_POINT('Ctrl Pts',(7.53617333959681,-3.10591474188473,
38.2926583529603));
#178334=CARTESIAN_POINT('Ctrl Pts',(7.09240338266829,-3.97823448761708,
38.2558383317433));
#178335=CARTESIAN_POINT('Ctrl Pts',(6.92504051766862,-4.26290253188216,
38.2431887587551));
#178336=CARTESIAN_POINT('Ctrl Pts',(6.68596845706459,-4.61813526113775,
38.2266177051951));
#178337=CARTESIAN_POINT('Ctrl Pts',(6.629618049335,-4.69867128156877,38.222801620362));
#178338=CARTESIAN_POINT('Ctrl Pts',(6.5439579866085,-4.81648693133922,38.2171240403336));
#178339=CARTESIAN_POINT('Ctrl Pts',(6.51576054539933,-4.85456455103081,
38.2152739764911));
#178340=CARTESIAN_POINT('Ctrl Pts',(6.46461056187599,-4.92238857501888,
38.2119506819065));
#178341=CARTESIAN_POINT('Ctrl Pts',(6.44178165851802,-4.95222657511283,
38.2104787902989));
#178342=CARTESIAN_POINT('Ctrl Pts',(6.39261892962319,-5.01556842865307,
38.2073326169962));
#178343=CARTESIAN_POINT('Ctrl Pts',(6.36622681929078,-5.04902559985828,
38.2056577436812));
#178344=CARTESIAN_POINT('Ctrl Pts',(6.29347563904454,-5.13977463228924,
38.201078300959));
#178345=CARTESIAN_POINT('Ctrl Pts',(6.24659849945455,-5.1966456466147,38.1981681408436));
#178346=CARTESIAN_POINT('Ctrl Pts',(5.92853419942872,-5.57199584455395,
38.1786822707243));
#178347=CARTESIAN_POINT('Ctrl Pts',(5.63388052916184,-5.86975559237063,
38.1618398356592));
#178348=CARTESIAN_POINT('Ctrl Pts',(4.98793605025122,-6.42886540178347,
38.1271601353612));
#178349=CARTESIAN_POINT('Ctrl Pts',(4.635808550968,-6.6872343296369,38.1093687099196));
#178350=CARTESIAN_POINT('Ctrl Pts',(4.2027030661909,-6.95429876935298,38.08906144608));
#178351=CARTESIAN_POINT('Ctrl Pts',(4.14024314918993,-6.99166441277781,
38.0861691646487));
#178352=CARTESIAN_POINT('Ctrl Pts',(4.05608685828283,-7.04048633233219,
38.0823231776387));
#178353=CARTESIAN_POINT('Ctrl Pts',(4.03482888471358,-7.05269056997144,
38.0813559692687));
#178354=CARTESIAN_POINT('Ctrl Pts',(3.99862959878405,-7.07325540452159,
38.0797163663507));
#178355=CARTESIAN_POINT('Ctrl Pts',(3.9837165839922,-7.08166526080852,38.0790430386715));
#178356=CARTESIAN_POINT('Ctrl Pts',(3.9518331056948,-7.09951263980306,38.0776079672001));
#178357=CARTESIAN_POINT('Ctrl Pts',(3.93485520347087,-7.10893656949247,
38.0768464742973));
#178358=CARTESIAN_POINT('Ctrl Pts',(3.89265383398506,-7.13216379752461,
38.074960018663));
#178359=CARTESIAN_POINT('Ctrl Pts',(3.86739053135358,-7.14589426130388,
38.0738363263668));
#178360=CARTESIAN_POINT('Ctrl Pts',(3.76718489166121,-7.19966841833148,
38.0693999879081));
#178361=CARTESIAN_POINT('Ctrl Pts',(3.69168882356309,-7.23866984759135,
38.0661031788969));
#178362=CARTESIAN_POINT('Ctrl Pts',(3.53881857215696,-7.31462921584078,
38.0595012597281));
#178363=CARTESIAN_POINT('Ctrl Pts',(3.46144338978405,-7.35156086953082,
38.0561967567631));
#178364=CARTESIAN_POINT('Ctrl Pts',(3.12042697096105,-7.50775250016901,
38.0417594496031));
#178365=CARTESIAN_POINT('Ctrl Pts',(2.85110864840801,-7.61410474270099,
38.0306748309688));
#178366=CARTESIAN_POINT('Ctrl Pts',(2.49958217425814,-7.73164842399371,
38.0163262144808));
#178367=CARTESIAN_POINT('Ctrl Pts',(2.4220894585606,-7.75627365082814,38.0131711528636));
#178368=CARTESIAN_POINT('Ctrl Pts',(2.30355733940408,-7.7919905384352,38.0083529839391));
#178369=CARTESIAN_POINT('Ctrl Pts',(2.26277870120508,-7.80393013163419,
38.0066967918507));
#178370=CARTESIAN_POINT('Ctrl Pts',(2.18822927863056,-7.82512403381542,
38.0036710009939));
#178371=CARTESIAN_POINT('Ctrl Pts',(2.15448870355277,-7.83448096155193,
38.0023022828169));
#178372=CARTESIAN_POINT('Ctrl Pts',(2.0805848968681,-7.85446242204418,37.9993055923255));
#178373=CARTESIAN_POINT('Ctrl Pts',(2.0403985538727,-7.86499759549781,37.9976769210452));
#178374=CARTESIAN_POINT('Ctrl Pts',(1.92401868187338,-7.89455551698002,
37.9929621209266));
#178375=CARTESIAN_POINT('Ctrl Pts',(1.84762818350918,-7.91278236053515,
37.9898696026554));
#178376=CARTESIAN_POINT('Ctrl Pts',(1.71673107361407,-7.94201563689225,
37.9845731132626));
#178377=CARTESIAN_POINT('Ctrl Pts',(1.66235356184399,-7.95357520588922,
37.9823736185903));
#178378=CARTESIAN_POINT('Ctrl Pts',(1.43070741043288,-8.00033915452698,
37.9730071196873));
#178379=CARTESIAN_POINT('Ctrl Pts',(1.25241025727234,-8.03018169061828,
37.9658042810544));
#178380=CARTESIAN_POINT('Ctrl Pts',(0.806402868076624,-8.0896157855723,
37.9478358823616));
#178381=CARTESIAN_POINT('Ctrl Pts',(0.537933932950174,-8.11189237201577,
37.9370595542143));
#178382=CARTESIAN_POINT('Ctrl Pts',(0.229100257388967,-8.12211688850682,
37.924854738887));
#178383=CARTESIAN_POINT('Ctrl Pts',(0.189336934210476,-8.12314109366498,
37.9232871390134));
#178384=CARTESIAN_POINT('Ctrl Pts',(0.128256249534165,-8.12426564204894,
37.9208858886481));
#178385=CARTESIAN_POINT('Ctrl Pts',(0.106943524038269,-8.12457414109394,
37.9200493183069));
#178386=CARTESIAN_POINT('Ctrl Pts',(0.0655187816009979,-8.12501072899457,
37.9184257591139));
#178387=CARTESIAN_POINT('Ctrl Pts',(0.0454070909787996,-8.12514801442794,
37.917638624657));
#178388=CARTESIAN_POINT('Ctrl Pts',(-0.00238489442532232,-8.12529679839415,
37.915770527126));
#178389=CARTESIAN_POINT('Ctrl Pts',(-0.0300651776680895,-8.12524152518288,
37.9146904645797));
#178390=CARTESIAN_POINT('Ctrl Pts',(-0.124701342575879,-8.12456894581731,
37.9110035177865));
#178391=CARTESIAN_POINT('Ctrl Pts',(-0.19164988562061,-8.12326543896288,
37.9084049675273));
#178392=CARTESIAN_POINT('Ctrl Pts',(-0.687696142308071,-8.1074714453238,
37.8891985523274));
#178393=CARTESIAN_POINT('Ctrl Pts',(-1.11506257674444,-8.0598176923586,
37.8728801079191));
#178394=CARTESIAN_POINT('Ctrl Pts',(-1.73677604599634,-7.94007733791922,
37.8485063210257));
#178395=CARTESIAN_POINT('Ctrl Pts',(-1.93536873457752,-7.89402088552531,
37.8406283630125));
#178396=CARTESIAN_POINT('Ctrl Pts',(-2.19815186944007,-7.82256435002126,
37.8300330313126));
#178397=CARTESIAN_POINT('Ctrl Pts',(-2.26405537785717,-7.80374511643277,
37.8273614133427));
#178398=CARTESIAN_POINT('Ctrl Pts',(-2.37809651167119,-7.76961358315815,
37.8227120533384));
#178399=CARTESIAN_POINT('Ctrl Pts',(-2.42634414940916,-7.75468195982484,
37.8207367841108));
#178400=CARTESIAN_POINT('Ctrl Pts',(-2.52929458623334,-7.72176611601376,
37.8165039011953));
#178401=CARTESIAN_POINT('Ctrl Pts',(-2.58395176566452,-7.70364824604006,
37.8142456209746));
#178402=CARTESIAN_POINT('Ctrl Pts',(-2.72960265991232,-7.65364311095802,
37.8081979401269));
#178403=CARTESIAN_POINT('Ctrl Pts',(-2.82022894836474,-7.6207146728734,
37.8044035581415));
#178404=CARTESIAN_POINT('Ctrl Pts',(-3.04507782880851,-7.53445706123394,
37.7949119447178));
#178405=CARTESIAN_POINT('Ctrl Pts',(-3.1785050998285,-7.479147504975,37.7892091446805));
#178406=CARTESIAN_POINT('Ctrl Pts',(-3.42461792422765,-7.36935040389043,
37.7785706455184));
#178407=CARTESIAN_POINT('Ctrl Pts',(-3.53765710650911,-7.31575803791595,
37.773635939523));
#178408=CARTESIAN_POINT('Ctrl Pts',(-3.69004523030179,-7.23915201102149,
37.7669279919342));
#178409=CARTESIAN_POINT('Ctrl Pts',(-3.7305041767151,-7.21838584766392,
37.7651416289053));
#178410=CARTESIAN_POINT('Ctrl Pts',(-3.80914010237132,-7.17718705299606,
37.7616600405768));
#178411=CARTESIAN_POINT('Ctrl Pts',(-3.84733230485705,-7.15678674141199,
37.7599646592506));
#178412=CARTESIAN_POINT('Ctrl Pts',(-3.98262712480989,-7.08312320570872,
37.753940008585));
#178413=CARTESIAN_POINT('Ctrl Pts',(-4.07880194526745,-7.02818098858735,
37.7496224809905));
#178414=CARTESIAN_POINT('Ctrl Pts',(-4.38345385296372,-6.8457809721673,
37.73579129896));
#178415=CARTESIAN_POINT('Ctrl Pts',(-4.58731545109521,-6.71088081352194,
37.7262952494593));
#178416=CARTESIAN_POINT('Ctrl Pts',(-4.83447285745584,-6.53079925521143,
37.7143402980482));
#178417=CARTESIAN_POINT('Ctrl Pts',(-4.88374560459725,-6.49403538330858,
37.7119341361101));
#178418=CARTESIAN_POINT('Ctrl Pts',(-4.97649313243812,-6.42318108006872,
37.7073589339506));
#178419=CARTESIAN_POINT('Ctrl Pts',(-5.02004674185723,-6.38919946223021,
37.7051907140946));
#178420=CARTESIAN_POINT('Ctrl Pts',(-5.12248485360041,-6.30758057132354,
37.7000421754501));
#178421=CARTESIAN_POINT('Ctrl Pts',(-5.18105638535243,-6.25955896199597,
37.6970592819009));
#178422=CARTESIAN_POINT('Ctrl Pts',(-5.4086378096875,-6.06758667695662,
37.6853080290312));
#178423=CARTESIAN_POINT('Ctrl Pts',(-5.57238863410537,-5.91755475100201,
37.6764937704057));
#178424=CARTESIAN_POINT('Ctrl Pts',(-5.87594308056476,-5.61564527162143,
37.6594122447874));
#178425=CARTESIAN_POINT('Ctrl Pts',(-6.0165124841956,-5.46477409508698,
37.6511574605115));
#178426=CARTESIAN_POINT('Ctrl Pts',(-6.30171123252783,-5.13431560608808,
37.6336860043781));
#178427=CARTESIAN_POINT('Ctrl Pts',(-6.444746455658,-4.95358517693716,37.6244778103));
#178428=CARTESIAN_POINT('Ctrl Pts',(-6.60909871605692,-4.72673005949495,
37.6133986925933));
#178429=CARTESIAN_POINT('Ctrl Pts',(-6.63791768817087,-4.6861723934592,
37.6114358750152));
#178430=CARTESIAN_POINT('Ctrl Pts',(-6.6806488929502,-4.62485052324696,
37.6084961248085));
#178431=CARTESIAN_POINT('Ctrl Pts',(-6.69484071648923,-4.60428276502318,
37.6075147802132));
#178432=CARTESIAN_POINT('Ctrl Pts',(-6.72006386873803,-4.56736446673624,
37.6057618232111));
#178433=CARTESIAN_POINT('Ctrl Pts',(-6.73113096112512,-4.55103862424891,
37.6049895946091));
#178434=CARTESIAN_POINT('Ctrl Pts',(-6.75497548820163,-4.51558664827104,
37.6033191874099));
#178435=CARTESIAN_POINT('Ctrl Pts',(-6.76773130968638,-4.49644632427089,
37.6024214589137));
#178436=CARTESIAN_POINT('Ctrl Pts',(-6.80811223630881,-4.43529294964012,
37.5995659454713));
#178437=CARTESIAN_POINT('Ctrl Pts',(-6.83542876999993,-4.39307743500752,
37.5976136567261));
#178438=CARTESIAN_POINT('Ctrl Pts',(-6.90115011089745,-4.28941315114365,
37.5928611064934));
#178439=CARTESIAN_POINT('Ctrl Pts',(-6.93912824112716,-4.22769882934905,
37.5900668407345));
#178440=CARTESIAN_POINT('Ctrl Pts',(-7.1046934159661,-3.95041335404007,
37.5776442808977));
#178441=CARTESIAN_POINT('Ctrl Pts',(-7.22309701559356,-3.72951804601877,
37.5680944432444));
#178442=CARTESIAN_POINT('Ctrl Pts',(-7.41925984880203,-3.31904611005962,
37.550655796394));
#178443=CARTESIAN_POINT('Ctrl Pts',(-7.50041820856906,-3.1313270518481,
37.5427918180161));
#178444=CARTESIAN_POINT('Ctrl Pts',(-7.59524941694852,-2.88707278317949,
37.5326279248495));
#178445=CARTESIAN_POINT('Ctrl Pts',(-7.61551777827767,-2.83317699507591,
37.5303895952474));
#178446=CARTESIAN_POINT('Ctrl Pts',(-7.64670015806661,-2.74750660141824,
37.5268373426887));
#178447=CARTESIAN_POINT('Ctrl Pts',(-7.65799295421377,-2.71587181883277,
37.5255268564697));
#178448=CARTESIAN_POINT('Ctrl Pts',(-7.68082991192148,-2.65062304618199,
37.5228261671469));
#178449=CARTESIAN_POINT('Ctrl Pts',(-7.692350339879,-2.61700151061444,37.5214357831341));
#178450=CARTESIAN_POINT('Ctrl Pts',(-7.71887350205123,-2.53790705239747,
37.5181675486405));
#178451=CARTESIAN_POINT('Ctrl Pts',(-7.73369556827182,-2.49237500759929,
37.5162881645062));
#178452=CARTESIAN_POINT('Ctrl Pts',(-7.78362248806716,-2.33426933516128,
37.5097685944556));
#178453=CARTESIAN_POINT('Ctrl Pts',(-7.81667845274167,-2.22106505550809,
37.5051114846297));
#178454=CARTESIAN_POINT('Ctrl Pts',(-7.87422443180798,-2.00676076768006,
37.4963159468717));
#178455=CARTESIAN_POINT('Ctrl Pts',(-7.89925983462117,-1.90583133551186,
37.4921821412222));
#178456=CARTESIAN_POINT('Ctrl Pts',(-7.95395165523837,-1.66570947667068,
37.482373756228));
#178457=CARTESIAN_POINT('Ctrl Pts',(-7.98190207549247,-1.52616321537475,
37.476694091203));
#178458=CARTESIAN_POINT('Ctrl Pts',(-8.03202753252847,-1.23660619738642,
37.4649792258475));
#178459=CARTESIAN_POINT('Ctrl Pts',(-8.05369761241732,-1.08656179414735,
37.4589471566957));
#178460=CARTESIAN_POINT('Ctrl Pts',(-8.07505458824178,-0.902399591329861,
37.4516226785151));
#178461=CARTESIAN_POINT('Ctrl Pts',(-8.07874116122626,-0.868776662209606,
37.4502886834988));
#178462=CARTESIAN_POINT('Ctrl Pts',(-8.08411540477477,-0.81676592974232,
37.4482307325988));
#178463=CARTESIAN_POINT('Ctrl Pts',(-8.08595051860162,-0.798393809419776,
37.4475048638575));
#178464=CARTESIAN_POINT('Ctrl Pts',(-8.08932561298056,-0.763398573696936,
37.4461243938638));
#178465=CARTESIAN_POINT('Ctrl Pts',(-8.09087701609042,-0.746776651994654,
37.4454696323381));
#178466=CARTESIAN_POINT('Ctrl Pts',(-8.09454642366884,-0.706107982780919,
37.4438700224355));
#178467=CARTESIAN_POINT('Ctrl Pts',(-8.0966085163781,-0.682056322335849,
37.442926040087));
#178468=CARTESIAN_POINT('Ctrl Pts',(-8.10326462236594,-0.600133460629295,
37.4397171739875));
#178469=CARTESIAN_POINT('Ctrl Pts',(-8.10734561813163,-0.542222107185787,
37.4374597754607));
#178470=CARTESIAN_POINT('Ctrl Pts',(-8.11582498784977,-0.400205711281178,
37.4319460653837));
#178471=CARTESIAN_POINT('Ctrl Pts',(-8.11953706568488,-0.316066234122284,
37.4286983690644));
#178472=CARTESIAN_POINT('Ctrl Pts',(-8.13341522268754,0.170028859495288,
37.4100122569928));
#178473=CARTESIAN_POINT('Ctrl Pts',(-8.11504142195906,0.572242905391769,
37.3948386913516));
#178474=CARTESIAN_POINT('Ctrl Pts',(-8.02040776561461,1.35809115875314,
37.3647320158234));
#178475=CARTESIAN_POINT('Ctrl Pts',(-7.94610990120337,1.74088513977439,
37.3498428923332));
#178476=CARTESIAN_POINT('Ctrl Pts',(-7.82579951276028,2.18672945908209,
37.3319055269939));
#178477=CARTESIAN_POINT('Ctrl Pts',(-7.80601487142752,2.25633674140283,
37.3290880041147));
#178478=CARTESIAN_POINT('Ctrl Pts',(-7.77322970878715,2.36608679634183,
37.3246170148992));
#178479=CARTESIAN_POINT('Ctrl Pts',(-7.76084171098822,2.40640868416693,
37.3229682280847));
#178480=CARTESIAN_POINT('Ctrl Pts',(-7.73707727742894,2.48166730563065,
37.3198790379777));
#178481=CARTESIAN_POINT('Ctrl Pts',(-7.72577674844785,2.51662691635659,
37.318439224322));
#178482=CARTESIAN_POINT('Ctrl Pts',(-7.69980642164302,2.5951456876696,37.3151944131068));
#178483=CARTESIAN_POINT('Ctrl Pts',(-7.68500335385168,2.63865941416542,
37.3133885219715));
#178484=CARTESIAN_POINT('Ctrl Pts',(-7.63989872617744,2.76764490848981,
37.3080121925767));
#178485=CARTESIAN_POINT('Ctrl Pts',(-7.60853473568339,2.85273727055215,
37.3044348722191));
#178486=CARTESIAN_POINT('Ctrl Pts',(-7.44440862655155,3.27604596334917,
37.2864829278164));
#178487=CARTESIAN_POINT('Ctrl Pts',(-7.29049172156961,3.60560945604558,
37.2720616140364));
#178488=CARTESIAN_POINT('Ctrl Pts',(-6.98398079870945,4.16141277402086,
37.2463444282087));
#178489=CARTESIAN_POINT('Ctrl Pts',(-6.84109986260679,4.39234441302397,
37.2351863685049));
#178490=CARTESIAN_POINT('Ctrl Pts',(-6.43369110442789,4.98257404325643,
37.2052698070201));
#178491=CARTESIAN_POINT('Ctrl Pts',(-6.15069180496686,5.32798251608046,
37.1862400322237));
#178492=CARTESIAN_POINT('Ctrl Pts',(-5.71326178205887,5.78031016722106,
37.1598078433099));
#178493=CARTESIAN_POINT('Ctrl Pts',(-5.58129108446918,5.90783707758814,
37.1521707301604));
#178494=CARTESIAN_POINT('Ctrl Pts',(-5.37732554496077,6.09199465435793,
37.1409756237096));
#178495=CARTESIAN_POINT('Ctrl Pts',(-5.30850856854674,6.15205383290401,
37.1372963428697));
#178496=CARTESIAN_POINT('Ctrl Pts',(-5.22675544019093,6.22100948333098,
37.1330522728761));
#178497=CARTESIAN_POINT('Ctrl Pts',(-5.21478948634788,6.23104341506426,
37.132434205476));
#178498=CARTESIAN_POINT('Ctrl Pts',(-5.19557971513977,6.24705748470578,
37.1314470711861));
#178499=CARTESIAN_POINT('Ctrl Pts',(-5.18835435632236,6.25305964050697,
37.1310769285995));
#178500=CARTESIAN_POINT('Ctrl Pts',(-5.17553471412573,6.26367148962491,
37.1304222554507));
#178501=CARTESIAN_POINT('Ctrl Pts',(-5.16994464690103,6.26828624549559,
37.13013747176));
#178502=CARTESIAN_POINT('Ctrl Pts',(-5.15832444728088,6.27785292458736,
37.1295469293536));
#178503=CARTESIAN_POINT('Ctrl Pts',(-5.15229333989172,6.28280365652295,
37.1292412313205));
#178504=CARTESIAN_POINT('Ctrl Pts',(-5.13672792651202,6.29554329195237,
37.1284543621582));
#178505=CARTESIAN_POINT('Ctrl Pts',(-5.12718301125246,6.30331924490339,
37.1279738626732));
#178506=CARTESIAN_POINT('Ctrl Pts',(-5.08728165438416,6.33567507135007,
37.1259737356764));
#178507=CARTESIAN_POINT('Ctrl Pts',(-5.05676550222269,6.36005785902611,
37.1244646255642));
#178508=CARTESIAN_POINT('Ctrl Pts',(-4.843991490142,6.5275674400667,37.1140913687883));
#178509=CARTESIAN_POINT('Ctrl Pts',(-4.65585324261567,6.66306446823743,
37.1056859838987));
#178510=CARTESIAN_POINT('Ctrl Pts',(-3.99321458678843,7.09850809267342,
37.077854293084));
#178511=CARTESIAN_POINT('Ctrl Pts',(-3.49357627801123,7.35727921880065,
37.0597437380901));
#178512=CARTESIAN_POINT('Ctrl Pts',(-2.47487979833628,7.75751686430239,
37.0227001854279));
#178513=CARTESIAN_POINT('Ctrl Pts',(-1.96057718935779,7.90317386145941,
37.0039182551235));
#178514=CARTESIAN_POINT('Ctrl Pts',(-1.40362232001673,8.00316166898179,
36.9821668922066));
#178515=CARTESIAN_POINT('Ctrl Pts',(-1.37147098397941,8.00873395911033,
36.980906780968));
#178516=CARTESIAN_POINT('Ctrl Pts',(-1.32678424706177,8.01620183211323,
36.9791489961083));
#178517=CARTESIAN_POINT('Ctrl Pts',(-1.31427648243856,8.01826200478602,
36.9786563025079));
#178518=CARTESIAN_POINT('Ctrl Pts',(-1.29273869721206,8.02175777650204,
36.9778067059103));
#178519=CARTESIAN_POINT('Ctrl Pts',(-1.28371096440708,8.02320742118287,
36.9774502278366));
#178520=CARTESIAN_POINT('Ctrl Pts',(-1.2650854019114,8.02616601395783,36.9767140071667));
#178521=CARTESIAN_POINT('Ctrl Pts',(-1.25548727579643,8.02767299142703,
36.976334205721));
#178522=CARTESIAN_POINT('Ctrl Pts',(-1.23316018731623,8.03113748937763,
36.9754497502369));
#178523=CARTESIAN_POINT('Ctrl Pts',(-1.22042924411967,8.03308196641377,
36.9749447038983));
#178524=CARTESIAN_POINT('Ctrl Pts',(-1.1799263826769,8.03916971708846,36.9733355908616));
#178525=CARTESIAN_POINT('Ctrl Pts',(-1.15213772341481,8.04319927987422,
36.9722281053273));
#178526=CARTESIAN_POINT('Ctrl Pts',(-0.850959933323492,8.08527947499498,
36.960186727106));
#178527=CARTESIAN_POINT('Ctrl Pts',(-0.575841607544147,8.10951696116799,
36.9488375274159));
#178528=CARTESIAN_POINT('Ctrl Pts',(0.108004096137983,8.13478632827817,
36.9197876448925));
#178529=CARTESIAN_POINT('Ctrl Pts',(0.516575916144777,8.11908378719154,
36.9016721629172));
#178530=CARTESIAN_POINT('Ctrl Pts',(1.53296812704108,8.00297396181324,36.8557705926273));
#178531=CARTESIAN_POINT('Ctrl Pts',(2.13392119096461,7.8641062988252,36.8278357264556));
#178532=CARTESIAN_POINT('Ctrl Pts',(2.74694008390008,7.64691212990139,36.8016568879921));
#178533=CARTESIAN_POINT('Ctrl Pts',(2.78028635316732,7.63485119681187,36.8002398167166));
#178534=CARTESIAN_POINT('Ctrl Pts',(2.82541572252063,7.61819358214124,36.7983303093581));
#178535=CARTESIAN_POINT('Ctrl Pts',(2.83726828853964,7.61378723903433,36.7978295847397));
#178536=CARTESIAN_POINT('Ctrl Pts',(2.85594416764985,7.60679457581252,36.7970417699991));
#178537=CARTESIAN_POINT('Ctrl Pts',(2.86277433597345,7.60422671342119,36.7967538961836));
#178538=CARTESIAN_POINT('Ctrl Pts',(2.8759408279522,7.59925640026952,36.7961994246806));
#178539=CARTESIAN_POINT('Ctrl Pts',(2.88227762066764,7.59685521782957,36.7959327742801));
#178540=CARTESIAN_POINT('Ctrl Pts',(2.89725171354938,7.59115969573271,36.7953031433129));
#178541=CARTESIAN_POINT('Ctrl Pts',(2.90588642051966,7.58785853384698,36.7949404446646));
#178542=CARTESIAN_POINT('Ctrl Pts',(2.93114843639161,7.5781510880231,36.7938803703278));
#178543=CARTESIAN_POINT('Ctrl Pts',(2.9477603858686,7.57170481348814,36.7931846138128));
#178544=CARTESIAN_POINT('Ctrl Pts',(3.07158038497103,7.52318715932068,36.7880078309173));
#178545=CARTESIAN_POINT('Ctrl Pts',(3.17790712970326,7.47889421805786,36.783613597906));
#178546=CARTESIAN_POINT('Ctrl Pts',(3.53446288756006,7.32138494224311,36.7689569950812));
#178547=CARTESIAN_POINT('Ctrl Pts',(3.77988831775344,7.19774683603318,36.7589969941373));
#178548=CARTESIAN_POINT('Ctrl Pts',(4.33586462258877,6.88136813430985,36.7359634571538));
#178549=CARTESIAN_POINT('Ctrl Pts',(4.64061076973154,6.67964670464074,36.7229576760477));
#178550=CARTESIAN_POINT('Ctrl Pts',(5.00087770235044,6.40458369834443,36.7064221848967));
#178551=CARTESIAN_POINT('Ctrl Pts',(5.07011888369741,6.34991058396381,36.7031882560278));
#178552=CARTESIAN_POINT('Ctrl Pts',(5.37332611482754,6.10237533113688,36.6887542385641));
#178553=CARTESIAN_POINT('Ctrl Pts',(5.59727087153957,5.89764070327418,36.6773458144166));
#178554=CARTESIAN_POINT('Ctrl Pts',(5.84451849769205,5.64480614569987,36.6637264080394));
#178555=CARTESIAN_POINT('Ctrl Pts',(5.87945526296628,5.60840785351286,36.6617766270597));
#178556=CARTESIAN_POINT('Ctrl Pts',(5.93226733494533,5.55235063404496,36.6587902128289));
#178557=CARTESIAN_POINT('Ctrl Pts',(5.95038908197754,5.53292536208915,36.6577583077418));
#178558=CARTESIAN_POINT('Ctrl Pts',(5.98295131327453,5.49767587784272,36.6558911460154));
#178559=CARTESIAN_POINT('Ctrl Pts',(5.99742512976749,5.48188273161136,36.6550565069261));
#178560=CARTESIAN_POINT('Ctrl Pts',(6.0255434587052,5.45095668299506,36.6534258568991));
#178561=CARTESIAN_POINT('Ctrl Pts',(6.03919386736983,5.43582929843389,36.6526299448002));
#178562=CARTESIAN_POINT('Ctrl Pts',(6.07494585337241,5.39590804671453,36.6505338727248));
#178563=CARTESIAN_POINT('Ctrl Pts',(6.09695250358661,5.37102978248296,36.6492320085259));
#178564=CARTESIAN_POINT('Ctrl Pts',(6.17728191408485,5.27908842896727,36.6444359053918));
#178565=CARTESIAN_POINT('Ctrl Pts',(6.2346552404826,5.21120525557357,36.6409240257727));
#178566=CARTESIAN_POINT('Ctrl Pts',(6.56839075168565,4.80293292186313,36.6199515541404));
#178567=CARTESIAN_POINT('Ctrl Pts',(6.81793057208248,4.44158822725121,36.601937187932));
#178568=CARTESIAN_POINT('Ctrl Pts',(7.34050343706632,3.53624976299989,36.5579718189738));
#178569=CARTESIAN_POINT('Ctrl Pts',(7.58405867599734,2.9782708836275,36.5316849932689));
#178570=CARTESIAN_POINT('Ctrl Pts',(7.77870714222655,2.34822476958046,36.5050808676723));
#178571=CARTESIAN_POINT('Ctrl Pts',(7.79371911470639,2.29790923968159,36.5029780492243));
#178572=CARTESIAN_POINT('Ctrl Pts',(7.81227328950041,2.23344710535848,36.5003144284647));
#178573=CARTESIAN_POINT('Ctrl Pts',(7.81626640876989,2.2194322140264,36.4997371528914));
#178574=CARTESIAN_POINT('Ctrl Pts',(7.82256266058574,2.19710613331562,36.498820521354));
#178575=CARTESIAN_POINT('Ctrl Pts',(7.82489029215667,2.18880192257014,36.4984802351187));
#178576=CARTESIAN_POINT('Ctrl Pts',(7.8292150485915,2.17327757172662,36.4978453282286));
#178577=CARTESIAN_POINT('Ctrl Pts',(7.83121541708501,2.16605834929088,36.4975505818709));
#178578=CARTESIAN_POINT('Ctrl Pts',(7.83564627788241,2.14998124163357,36.4968953163169));
#178579=CARTESIAN_POINT('Ctrl Pts',(7.83807174189637,2.14112197252275,36.496534996252));
#178580=CARTESIAN_POINT('Ctrl Pts',(7.84508416622161,2.1153367378781,36.4954885245381));
#178581=CARTESIAN_POINT('Ctrl Pts',(7.84963137678619,2.09839994864755,36.4948039813032));
#178582=CARTESIAN_POINT('Ctrl Pts',(7.88364621727185,1.97004857797567,36.4896383087437));
#178583=CARTESIAN_POINT('Ctrl Pts',(7.91079350474151,1.85804100352943,36.4852629932323));
#178584=CARTESIAN_POINT('Ctrl Pts',(7.95695899968721,1.64815694583263,36.4772948993053));
#178585=CARTESIAN_POINT('Ctrl Pts',(7.97657444123336,1.55044476404425,36.4736732144773));
#178586=CARTESIAN_POINT('Ctrl Pts',(8.08115054270371,0.974828388749765,
36.4527439956508));
#178587=CARTESIAN_POINT('Ctrl Pts',(8.12494782763725,0.490438023465154,
36.4367273681874));
#178588=CARTESIAN_POINT('Ctrl Pts',(8.12524844182851,0.00503200391154854,
36.4203543227145));
#178589=CARTESIAN_POINT('',(8.120871211716,-0.00172117854340554,34.4167025567877));
#178590=CARTESIAN_POINT('Ctrl Pts',(8.120871211716,-0.00172117854340554,
34.4167025567877));
#178591=CARTESIAN_POINT('Ctrl Pts',(8.12076539718447,0.119070448189721,
34.4214150269101));
#178592=CARTESIAN_POINT('Ctrl Pts',(8.08738294886854,1.59563522457119,34.479016652128));
#178593=CARTESIAN_POINT('Ctrl Pts',(6.87712117603644,5.73415005919172,34.6423965875369));
#178594=CARTESIAN_POINT('Ctrl Pts',(1.64131973131669,8.81124817329271,34.8539532079189));
#178595=CARTESIAN_POINT('Ctrl Pts',(-3.82482145636865,7.54243940143105,
35.0655098283007));
#178596=CARTESIAN_POINT('Ctrl Pts',(-6.96195299981451,4.82582851322905,
35.2241772935872));
#178597=CARTESIAN_POINT('Ctrl Pts',(-8.42537801125605,0.894369939753666,
35.3828447588736));
#178598=CARTESIAN_POINT('Ctrl Pts',(-7.82264342903586,-3.23476629007719,
35.54151222416));
#178599=CARTESIAN_POINT('Ctrl Pts',(-5.33310408397497,-6.58368385109594,
35.7001796894465));
#178600=CARTESIAN_POINT('Ctrl Pts',(-1.52043507705952,-8.3334079215629,
35.8588471547329));
#178601=CARTESIAN_POINT('Ctrl Pts',(2.61913853473312,-8.04100520042323,
36.0175146200193));
#178602=CARTESIAN_POINT('Ctrl Pts',(6.80819671928331,-5.43726497504425,
36.2034664207042));
#178603=CARTESIAN_POINT('Ctrl Pts',(8.10078544928885,-2.03703630869931,
36.3365290662937));
#178604=CARTESIAN_POINT('Ctrl Pts',(8.11892105081991,0.00515126165398824,
36.4167025567876));
#178605=CARTESIAN_POINT('',(8.12588319212562,-0.00333877610576572,32.4167025567876));
#178606=CARTESIAN_POINT('Ctrl Pts',(8.12524931413266,-0.00333851565694556,
32.4167025567876));
#178607=CARTESIAN_POINT('Ctrl Pts',(8.12533264120618,0.199462164817699,
32.4246762945215));
#178608=CARTESIAN_POINT('Ctrl Pts',(8.11781906538481,0.402445848508343,
32.4326500322554));
#178609=CARTESIAN_POINT('Ctrl Pts',(8.10269393801063,0.605011164711699,
32.4406237699892));
#178610=CARTESIAN_POINT('Ctrl Pts',(8.08758128338672,0.807409437918437,
32.4485909322784));
#178611=CARTESIAN_POINT('Ctrl Pts',(8.06486961318257,1.00938970431921,32.4565580945675));
#178612=CARTESIAN_POINT('Ctrl Pts',(8.03459632854458,1.21035094077627,32.4645252568566));
#178613=CARTESIAN_POINT('Ctrl Pts',(8.00434310015103,1.41117903913057,32.4724871408498));
#178614=CARTESIAN_POINT('Ctrl Pts',(7.96653829317832,1.61098912868181,32.4804490248431));
#178615=CARTESIAN_POINT('Ctrl Pts',(7.92127114606062,1.80918517379715,32.4884109088363));
#178616=CARTESIAN_POINT('Ctrl Pts',(7.87458221998924,2.01360628462991,32.4966228646766));
#178617=CARTESIAN_POINT('Ctrl Pts',(7.8199545913438,2.21630995564091,32.5048348205169));
#178618=CARTESIAN_POINT('Ctrl Pts',(7.75754347982598,2.4166519652423,32.5130467763573));
#178619=CARTESIAN_POINT('Ctrl Pts',(7.69708101937612,2.61073873180324,32.5210023317566));
#178620=CARTESIAN_POINT('Ctrl Pts',(7.62931389273452,2.80260874993346,32.5289578871559));
#178621=CARTESIAN_POINT('Ctrl Pts',(7.55443431239011,2.99169012136667,32.5369134425552));
#178622=CARTESIAN_POINT('Ctrl Pts',(7.47956462708131,3.18074650645654,32.5448679466598));
#178623=CARTESIAN_POINT('Ctrl Pts',(7.39758448288845,3.3670146732867,32.5528224507644));
#178624=CARTESIAN_POINT('Ctrl Pts',(7.30873478426675,3.54994132567698,32.5607769548691));
#178625=CARTESIAN_POINT('Ctrl Pts',(7.21988377005464,3.73287068664765,32.5687315767554));
#178626=CARTESIAN_POINT('Ctrl Pts',(7.12416314297998,3.91245813848594,32.5766861986417));
#178627=CARTESIAN_POINT('Ctrl Pts',(7.02186064015138,4.08817327333284,32.5846408205281));
#178628=CARTESIAN_POINT('Ctrl Pts',(6.91954158903092,4.2639168315834,32.5925967291415));
#178629=CARTESIAN_POINT('Ctrl Pts',(6.81063870605211,4.43578653992892,32.600552637755));
#178630=CARTESIAN_POINT('Ctrl Pts',(6.69548431629431,4.60327897620347,32.6085085463684));
#178631=CARTESIAN_POINT('Ctrl Pts',(6.58025746384561,4.77087680969878,32.6164694613611));
#178632=CARTESIAN_POINT('Ctrl Pts',(6.4587714325685,4.9340915968601,32.6244303763538));
#178633=CARTESIAN_POINT('Ctrl Pts',(6.33140089099655,5.09245032572612,32.6323912913465));
#178634=CARTESIAN_POINT('Ctrl Pts',(6.20398294524252,5.25086799181519,32.6403551691959));
#178635=CARTESIAN_POINT('Ctrl Pts',(6.07067633399234,5.40442574385364,32.6483190470453));
#178636=CARTESIAN_POINT('Ctrl Pts',(5.93189469190031,5.55268519967636,32.6562829248947));
#178637=CARTESIAN_POINT('Ctrl Pts',(5.79299791080893,5.70106765768533,32.6642534099071));
#178638=CARTESIAN_POINT('Ctrl Pts',(5.64861725715567,5.84414280526376,32.6722238949195));
#178639=CARTESIAN_POINT('Ctrl Pts',(5.49920245619378,5.98150983517475,32.6801943799319));
#178640=CARTESIAN_POINT('Ctrl Pts',(5.4660628260617,6.01197731586801,32.681962202956));
#178641=CARTESIAN_POINT('Ctrl Pts',(5.43267567652258,6.04216415184208,32.6837300259801));
#178642=CARTESIAN_POINT('Ctrl Pts',(5.39904612847492,6.072066243471,32.6854978490042));
#178643=CARTESIAN_POINT('Ctrl Pts',(5.25488410256312,6.2002495334193,32.6930760938337));
#178644=CARTESIAN_POINT('Ctrl Pts',(5.10595192852175,6.32347549322777,32.7006543386631));
#178645=CARTESIAN_POINT('Ctrl Pts',(4.95264020853747,6.44135409112695,32.7082325834926));
#178646=CARTESIAN_POINT('Ctrl Pts',(4.79944257183473,6.5591449724623,32.7158051891509));
#178647=CARTESIAN_POINT('Ctrl Pts',(4.64187216176423,6.67159618525623,32.7233777948091));
#178648=CARTESIAN_POINT('Ctrl Pts',(4.48035529049402,6.77835555525396,32.7309504004674));
#178649=CARTESIAN_POINT('Ctrl Pts',(4.31892793655416,6.88505575611526,32.7385188091681));
#178650=CARTESIAN_POINT('Ctrl Pts',(4.15355877926477,6.98607018940402,32.7460872178689));
#178651=CARTESIAN_POINT('Ctrl Pts',(3.98470591506945,7.08108793427327,32.7536556265696));
#178652=CARTESIAN_POINT('Ctrl Pts',(3.81589384707356,7.17608272209712,32.7612222066825));
#178653=CARTESIAN_POINT('Ctrl Pts',(3.64360006343698,7.26508351828062,32.7687887867953));
#178654=CARTESIAN_POINT('Ctrl Pts',(3.46831037012406,7.3478235375511,32.7763553669081));
#178655=CARTESIAN_POINT('Ctrl Pts',(3.29305177240959,7.43054887911654,32.7839206047438));
#178656=CARTESIAN_POINT('Ctrl Pts',(3.11479865672792,7.50701550028967,32.7914858425796));
#178657=CARTESIAN_POINT('Ctrl Pts',(2.93405982546309,7.57700339864669,32.7990510804153));
#178658=CARTESIAN_POINT('Ctrl Pts',(2.75325814263375,7.64701563515439,32.8066189490473));
#178659=CARTESIAN_POINT('Ctrl Pts',(2.56996935946642,7.71054451188793,32.8141868176793));
#178660=CARTESIAN_POINT('Ctrl Pts',(2.38472103070679,7.76741869401957,32.8217546863112));
#178661=CARTESIAN_POINT('Ctrl Pts',(2.20186323275607,7.82355894518661,32.8292248956377));
#178662=CARTESIAN_POINT('Ctrl Pts',(2.01709650532465,7.87321516599391,32.8366951049643));
#178663=CARTESIAN_POINT('Ctrl Pts',(1.83094063365424,7.91627083660822,32.8441653142908));
#178664=CARTESIAN_POINT('Ctrl Pts',(1.59904123836584,7.96990644793545,32.853471155734));
#178665=CARTESIAN_POINT('Ctrl Pts',(1.36510048989128,8.01327489456442,32.8627769971773));
#178666=CARTESIAN_POINT('Ctrl Pts',(1.12994981778146,8.04629734547485,32.8720828386205));
#178667=CARTESIAN_POINT('Ctrl Pts',(0.893536669155535,8.07949708726183,
32.881438641249));
#178668=CARTESIAN_POINT('Ctrl Pts',(0.655900623007412,8.10223949089091,
32.8907944438775));
#178669=CARTESIAN_POINT('Ctrl Pts',(0.417882586364596,8.11449700884246,
32.900150246506));
#178670=CARTESIAN_POINT('Ctrl Pts',(0.178709101831053,8.12681403036552,
32.909551466459));
#178671=CARTESIAN_POINT('Ctrl Pts',(-0.0608500475701027,8.12854414403122,
32.918952686412));
#178672=CARTESIAN_POINT('Ctrl Pts',(-0.299946381647792,8.11971180095922,
32.928353906365));
#178673=CARTESIAN_POINT('Ctrl Pts',(-0.539301488910411,8.11086989867103,
32.9377653012278));
#178674=CARTESIAN_POINT('Ctrl Pts',(-0.778192742263481,8.0914426860629,
32.9471766960906));
#178675=CARTESIAN_POINT('Ctrl Pts',(-1.01577422354322,8.06150670093905,
32.9565880909534));
#178676=CARTESIAN_POINT('Ctrl Pts',(-1.25307701775994,8.03160583122793,
32.9659884460921));
#178677=CARTESIAN_POINT('Ctrl Pts',(-1.48907307527489,7.99122083726528,
32.9753888012308));
#178678=CARTESIAN_POINT('Ctrl Pts',(-1.72292528536935,7.9404795839757,32.9847891563696));
#178679=CARTESIAN_POINT('Ctrl Pts',(-1.87254875182174,7.90801428374929,
32.9908036974388));
#178680=CARTESIAN_POINT('Ctrl Pts',(-2.02129470894103,7.8713104735582,32.996818238508));
#178681=CARTESIAN_POINT('Ctrl Pts',(-2.16894526312187,7.83041276102871,
33.0028327795772));
#178682=CARTESIAN_POINT('Ctrl Pts',(-2.35901041586562,7.77776663300085,
33.0105750780965));
#178683=CARTESIAN_POINT('Ctrl Pts',(-2.54734889156301,7.71814326754754,
33.0183173766158));
#178684=CARTESIAN_POINT('Ctrl Pts',(-2.73340470777657,7.65167865673964,
33.0260596751351));
#178685=CARTESIAN_POINT('Ctrl Pts',(-2.91934462806418,7.58525544736582,
33.0337971509035));
#178686=CARTESIAN_POINT('Ctrl Pts',(-3.10300438871746,7.51199959605789,
33.0415346266719));
#178687=CARTESIAN_POINT('Ctrl Pts',(-3.28384194403098,7.43209725778147,
33.0492721024402));
#178688=CARTESIAN_POINT('Ctrl Pts',(-3.46459899395702,7.35223049048305,
33.0570061336338));
#178689=CARTESIAN_POINT('Ctrl Pts',(-3.64253601833489,7.2657232716565,33.0647401648274));
#178690=CARTESIAN_POINT('Ctrl Pts',(-3.81712965369039,7.17281038153229,
33.072474196021));
#178691=CARTESIAN_POINT('Ctrl Pts',(-3.99170094655791,7.07990938133252,
33.0802072375021));
#178692=CARTESIAN_POINT('Ctrl Pts',(-4.16292938732278,6.98060450167136,
33.0879402789832));
#178693=CARTESIAN_POINT('Ctrl Pts',(-4.33031465918097,6.87517727153144,
33.0956733204643));
#178694=CARTESIAN_POINT('Ctrl Pts',(-4.49768320937557,6.76976057349303,
33.1034055894204));
#178695=CARTESIAN_POINT('Ctrl Pts',(-4.66120905830741,6.65822293464464,
33.1111378583764));
#178696=CARTESIAN_POINT('Ctrl Pts',(-4.82041952696814,6.54089008824673,
33.1188701273325));
#178697=CARTESIAN_POINT('Ctrl Pts',(-4.97969123665482,6.42351210923942,
33.1266053705407));
#178698=CARTESIAN_POINT('Ctrl Pts',(-5.13464396491998,6.30033467881232,
33.1343406137489));
#178699=CARTESIAN_POINT('Ctrl Pts',(-5.28483636192333,6.17172521991971,
33.1420758569572));
#178700=CARTESIAN_POINT('Ctrl Pts',(-5.41055511445368,6.06407249542646,
33.1485506529259));
#178701=CARTESIAN_POINT('Ctrl Pts',(-5.53293900276645,5.95261459081656,
33.1550254488947));
#178702=CARTESIAN_POINT('Ctrl Pts',(-5.6517484076503,5.83758747250286,33.1615002448635));
#178703=CARTESIAN_POINT('Ctrl Pts',(-5.80614264483297,5.68810836178156,
33.1699143193679));
#178704=CARTESIAN_POINT('Ctrl Pts',(-5.95457441705346,5.53252925030719,
33.1783283938722));
#178705=CARTESIAN_POINT('Ctrl Pts',(-6.09658687204909,5.37134211106113,
33.1867424683766));
#178706=CARTESIAN_POINT('Ctrl Pts',(-6.23863898721543,5.21010995668271,
33.1951588927004));
#178707=CARTESIAN_POINT('Ctrl Pts',(-6.37426803170842,5.04326684605947,
33.2035753170243));
#178708=CARTESIAN_POINT('Ctrl Pts',(-6.50305678842,4.87133862188665,33.2119917413481));
#178709=CARTESIAN_POINT('Ctrl Pts',(-6.63187748384527,4.69936776071301,
33.2204102528865));
#178710=CARTESIAN_POINT('Ctrl Pts',(-6.75385434666259,4.52230947963071,
33.2288287644249));
#178711=CARTESIAN_POINT('Ctrl Pts',(-6.86861227674034,4.34072032666375,
33.2372472759632));
#178712=CARTESIAN_POINT('Ctrl Pts',(-6.98341428486049,4.15906142606036,
33.2456690210168));
#178713=CARTESIAN_POINT('Ctrl Pts',(-7.0909916771743,3.97286839841154,33.2540907660704));
#178714=CARTESIAN_POINT('Ctrl Pts',(-7.1910135405162,3.78272544901326,33.2625125111239));
#178715=CARTESIAN_POINT('Ctrl Pts',(-7.29104624595438,3.59256188863962,
33.2709351690716));
#178716=CARTESIAN_POINT('Ctrl Pts',(-7.38352166699777,3.39844778665161,
33.2793578270193));
#178717=CARTESIAN_POINT('Ctrl Pts',(-7.46815530497601,3.2009910814088,33.287780484967));
#178718=CARTESIAN_POINT('Ctrl Pts',(-7.55280503783703,3.00349682558206,
33.2962047446618));
#178719=CARTESIAN_POINT('Ctrl Pts',(-7.62960990449206,2.80265893920064,
33.3046290043567));
#178720=CARTESIAN_POINT('Ctrl Pts',(-7.69833341527587,2.59910565190163,
33.3130532640516));
#178721=CARTESIAN_POINT('Ctrl Pts',(-7.71767951534411,2.54180412262302,
33.3154247460844));
#178722=CARTESIAN_POINT('Ctrl Pts',(-7.73638549978518,2.48428751806916,
33.3177962281173));
#178723=CARTESIAN_POINT('Ctrl Pts',(-7.75444679713097,2.42657009644585,
33.3201677101501));
#178724=CARTESIAN_POINT('Ctrl Pts',(-7.81860677837113,2.22153783227988,
33.3285920353703));
#178725=CARTESIAN_POINT('Ctrl Pts',(-7.87463413800463,2.01394911798742,
33.3370163605904));
#178726=CARTESIAN_POINT('Ctrl Pts',(-7.92235089313825,1.80445113219825,
33.3454406858106));
#178727=CARTESIAN_POINT('Ctrl Pts',(-7.97005940223307,1.59498935022292,
33.3538635552043));
#178728=CARTESIAN_POINT('Ctrl Pts',(-8.00946011672307,1.38361921295956,
33.362286424598));
#178729=CARTESIAN_POINT('Ctrl Pts',(-8.04042581154511,1.17099971457691,
33.3707092939918));
#178730=CARTESIAN_POINT('Ctrl Pts',(-8.07138517847581,0.958423665343055,
33.3791304421581));
#178731=CARTESIAN_POINT('Ctrl Pts',(-8.09391292985907,0.744599025845439,
33.3875515903245));
#178732=CARTESIAN_POINT('Ctrl Pts',(-8.10793335615874,0.530192657991854,
33.3959727384908));
#178733=CARTESIAN_POINT('Ctrl Pts',(-8.12194984879967,0.315846445333534,
33.404391523967));
#178734=CARTESIAN_POINT('Ctrl Pts',(-8.12746376636122,0.100919093475446,
33.4128103094432));
#178735=CARTESIAN_POINT('Ctrl Pts',(-8.12445137104079,-0.11391875215882,
33.4212290949194));
#178736=CARTESIAN_POINT('Ctrl Pts',(-8.1214398172128,-0.328696584281594,
33.4296455286643));
#178737=CARTESIAN_POINT('Ctrl Pts',(-8.10990670965498,-0.543384696404741,
33.4380619624092));
#178738=CARTESIAN_POINT('Ctrl Pts',(-8.08988041762325,-0.757312611182398,
33.4464783961542));
#178739=CARTESIAN_POINT('Ctrl Pts',(-8.0698613939715,-0.971162882561556,
33.4548917752228));
#178740=CARTESIAN_POINT('Ctrl Pts',(-8.041355366176,-1.18425324501899,33.4633051542915));
#178741=CARTESIAN_POINT('Ctrl Pts',(-8.00444263315897,-1.39591751008687,
33.4717185333602));
#178742=CARTESIAN_POINT('Ctrl Pts',(-7.99403481695767,-1.45559780431469,
33.4740907473856));
#178743=CARTESIAN_POINT('Ctrl Pts',(-7.98295898412734,-1.51516475896524,
33.476462961411));
#178744=CARTESIAN_POINT('Ctrl Pts',(-7.97121767767481,-1.57460353664807,
33.4788351754364));
#178745=CARTESIAN_POINT('Ctrl Pts',(-7.93293227191862,-1.76841823098716,
33.486570360347));
#178746=CARTESIAN_POINT('Ctrl Pts',(-7.88755027022448,-1.96095538472589,
33.4943055452577));
#178747=CARTESIAN_POINT('Ctrl Pts',(-7.83518219328127,-2.15165228617173,
33.5020407301683));
#178748=CARTESIAN_POINT('Ctrl Pts',(-7.78283030984125,-2.34229021942431,
33.5097735231687));
#178749=CARTESIAN_POINT('Ctrl Pts',(-7.72349674658826,-2.53108869332655,
33.517506316169));
#178750=CARTESIAN_POINT('Ctrl Pts',(-7.657342730468,-2.71749698631828,33.5252391091694));
#178751=CARTESIAN_POINT('Ctrl Pts',(-7.59119741715084,-2.90388075661636,
33.5329708848925));
#178752=CARTESIAN_POINT('Ctrl Pts',(-7.51823355702077,-3.08787463971037,
33.5407026606156));
#178753=CARTESIAN_POINT('Ctrl Pts',(-7.43866171381144,-3.26894470280179,
33.5484344363387));
#178754=CARTESIAN_POINT('Ctrl Pts',(-7.35906139762417,-3.45007955770527,
33.5561689787023));
#178755=CARTESIAN_POINT('Ctrl Pts',(-7.27284851266753,-3.6282881768599,
33.5639035210659));
#178756=CARTESIAN_POINT('Ctrl Pts',(-7.18028137304695,-3.80305758125945,
33.5716380634294));
#178757=CARTESIAN_POINT('Ctrl Pts',(-7.08769859986825,-3.9778565022634,
33.579373912071));
#178758=CARTESIAN_POINT('Ctrl Pts',(-6.98875960585026,-4.14921474241172,
33.5871097607126));
#178759=CARTESIAN_POINT('Ctrl Pts',(-6.88376792891641,-4.316645302005,33.5948456093541));
#178760=CARTESIAN_POINT('Ctrl Pts',(-6.77869034303867,-4.48421286086308,
33.6025877878173));
#178761=CARTESIAN_POINT('Ctrl Pts',(-6.6675503734878,-4.64784602265518,
33.6103299662805));
#178762=CARTESIAN_POINT('Ctrl Pts',(-6.55069455383339,-4.80708731196735,
33.6180721447437));
#178763=CARTESIAN_POINT('Ctrl Pts',(-6.45293711838823,-4.94030292849529,
33.6245489767368));
#178764=CARTESIAN_POINT('Ctrl Pts',(-6.35118031518691,-5.07044540173571,
33.6310258087299));
#178765=CARTESIAN_POINT('Ctrl Pts',(-6.2456480000629,-5.19726549464334,
33.637502640723));
#178766=CARTESIAN_POINT('Ctrl Pts',(-6.09251824414858,-5.38128429352174,
33.6469006691946));
#178767=CARTESIAN_POINT('Ctrl Pts',(-5.93135238108043,-5.55841258206398,
33.6562986976661));
#178768=CARTESIAN_POINT('Ctrl Pts',(-5.76274268177044,-5.72804367530497,
33.6656967261376));
#178769=CARTESIAN_POINT('Ctrl Pts',(-5.59389306497075,-5.89791613939373,
33.6751081272171));
#178770=CARTESIAN_POINT('Ctrl Pts',(-5.41757845098032,-6.06027004263627,
33.6845195282966));
#178771=CARTESIAN_POINT('Ctrl Pts',(-5.23442833419645,-6.21453518588972,
33.693930929376));
#178772=CARTESIAN_POINT('Ctrl Pts',(-5.05155398082456,-6.36856805693391,
33.7033281600028));
#178773=CARTESIAN_POINT('Ctrl Pts',(-4.86186472487565,-6.51453648871021,
33.7127253906295));
#178774=CARTESIAN_POINT('Ctrl Pts',(-4.66602124068028,-6.65191200663542,
33.7221226212562));
#178775=CARTESIAN_POINT('Ctrl Pts',(-4.47067174680851,-6.78894101225855,
33.7314961485618));
#178776=CARTESIAN_POINT('Ctrl Pts',(-4.26919905109153,-6.9174203594827,
33.7408696758674));
#178777=CARTESIAN_POINT('Ctrl Pts',(-4.06229233142146,-7.03686496790825,
33.750243203173));
#178778=CARTESIAN_POINT('Ctrl Pts',(-3.85672925183439,-7.15553391006335,
33.7595558593429));
#178779=CARTESIAN_POINT('Ctrl Pts',(-3.64580252352251,-7.26528503378603,
33.7688685155128));
#178780=CARTESIAN_POINT('Ctrl Pts',(-3.43022070587989,-7.3656821456979,
33.7781811716827));
#178781=CARTESIAN_POINT('Ctrl Pts',(-3.29141007051721,-7.43032668318932,
33.7841774831249));
#178782=CARTESIAN_POINT('Ctrl Pts',(-3.15067013035487,-7.49109391630273,
33.7901737945671));
#178783=CARTESIAN_POINT('Ctrl Pts',(-3.00819722507071,-7.54787632500539,
33.7961701060093));
#178784=CARTESIAN_POINT('Ctrl Pts',(-2.82838897756056,-7.61953869040649,
33.8037377642233));
#178785=CARTESIAN_POINT('Ctrl Pts',(-2.64589067218342,-7.68482273278492,
33.8113054224373));
#178786=CARTESIAN_POINT('Ctrl Pts',(-2.4612154913732,-7.74352025034639,
33.8188730806513));
#178787=CARTESIAN_POINT('Ctrl Pts',(-2.27659144380121,-7.80220151562026,
33.8264386435167));
#178788=CARTESIAN_POINT('Ctrl Pts',(-2.08979207012664,-7.85429977352598,
33.8340042063822));
#178789=CARTESIAN_POINT('Ctrl Pts',(-1.90134819948848,-7.89965585242812,
33.8415697692476));
#178790=CARTESIAN_POINT('Ctrl Pts',(-1.71292083831543,-7.94500795770884,
33.8491346692982));
#178791=CARTESIAN_POINT('Ctrl Pts',(-1.52284962459433,-7.98361897446067,
33.8566995693488));
#178792=CARTESIAN_POINT('Ctrl Pts',(-1.33167806492943,-8.01538028379726,
33.8642644693994));
#178793=CARTESIAN_POINT('Ctrl Pts',(-1.14041267944472,-8.04715718138815,
33.8718330822562));
#178794=CARTESIAN_POINT('Ctrl Pts',(-0.948046231811912,-8.07207759181744,
33.879401695113));
#178795=CARTESIAN_POINT('Ctrl Pts',(-0.755130451195359,-8.0900843978402,
33.8869703079698));
#178796=CARTESIAN_POINT('Ctrl Pts',(-0.562171769501025,-8.10809520826003,
33.894540603953));
#178797=CARTESIAN_POINT('Ctrl Pts',(-0.36866387859067,-8.11918932886303,
33.9021108999362));
#178798=CARTESIAN_POINT('Ctrl Pts',(-0.17516079945972,-8.12336175833827,
33.9096811959194));
#178799=CARTESIAN_POINT('Ctrl Pts',(0.0185383534548096,-8.12753841567405,
33.9172591627707));
#178800=CARTESIAN_POINT('Ctrl Pts',(0.212232316991425,-8.12477937273059,
33.9248371296218));
#178801=CARTESIAN_POINT('Ctrl Pts',(0.405368986399675,-8.11513176401747,
33.9324150964731));
#178802=CARTESIAN_POINT('Ctrl Pts',(0.595859927315845,-8.10561631536143,
33.9398892547473));
#178803=CARTESIAN_POINT('Ctrl Pts',(0.785808414656637,-8.08939992281175,
33.9473634130216));
#178804=CARTESIAN_POINT('Ctrl Pts',(0.974693342529583,-8.06657674918726,
33.9548375712958));
#178805=CARTESIAN_POINT('Ctrl Pts',(1.17875832895955,-8.04191935238796,
33.9629124030147));
#178806=CARTESIAN_POINT('Ctrl Pts',(1.38201771513442,-8.00949834448808,
33.9709872347336));
#178807=CARTESIAN_POINT('Ctrl Pts',(1.58385912450158,-7.96938378020742,
33.9790620664525));
#178808=CARTESIAN_POINT('Ctrl Pts',(1.78556699591701,-7.92929575565795,
33.9871315558757));
#178809=CARTESIAN_POINT('Ctrl Pts',(1.98585845150732,-7.88152438633841,
33.9952010452989));
#178810=CARTESIAN_POINT('Ctrl Pts',(2.18412877315489,-7.82619122337149,
34.0032705347222));
#178811=CARTESIAN_POINT('Ctrl Pts',(2.38229493006097,-7.77088713063841,
34.0113357846996));
#178812=CARTESIAN_POINT('Ctrl Pts',(2.57844176615795,-7.70802925192821,
34.019401034677));
#178813=CARTESIAN_POINT('Ctrl Pts',(2.77197663982588,-7.6377898027348,34.0274662846545));
#178814=CARTESIAN_POINT('Ctrl Pts',(2.96543617439079,-7.56757769629878,
34.0355283949977));
#178815=CARTESIAN_POINT('Ctrl Pts',(3.15628547712697,-7.48998985841786,
34.043590505341));
#178816=CARTESIAN_POINT('Ctrl Pts',(3.34394831142824,-7.40524795351217,
34.0516526156843));
#178817=CARTESIAN_POINT('Ctrl Pts',(3.53156361096603,-7.32052751362603,
34.059712683905));
#178818=CARTESIAN_POINT('Ctrl Pts',(3.71599376363942,-7.2286567516874,34.0677727521257));
#178819=CARTESIAN_POINT('Ctrl Pts',(3.8966831435325,-7.12990519161438,34.0758328203465));
#178820=CARTESIAN_POINT('Ctrl Pts',(4.08007951981587,-7.02967418589374,
34.0840136404099));
#178821=CARTESIAN_POINT('Ctrl Pts',(4.25962184019905,-6.92235470453889,
34.0921944604733));
#178822=CARTESIAN_POINT('Ctrl Pts',(4.43475493420291,-6.80827703872742,
34.1003752805367));
#178823=CARTESIAN_POINT('Ctrl Pts',(4.60731975200248,-6.69587228891284,
34.1084361312384));
#178824=CARTESIAN_POINT('Ctrl Pts',(4.77560351615612,-6.57690640215509,
34.1164969819402));
#178825=CARTESIAN_POINT('Ctrl Pts',(4.93910395641602,-6.45173927481695,
34.1245578326419));
#178826=CARTESIAN_POINT('Ctrl Pts',(5.10263151173733,-6.32655138964882,
34.1326200201624));
#178827=CARTESIAN_POINT('Ctrl Pts',(5.26137390929089,-6.19516040529427,
34.1406822076829));
#178828=CARTESIAN_POINT('Ctrl Pts',(5.41486111847034,-6.05796720279816,
34.1487443952034));
#178829=CARTESIAN_POINT('Ctrl Pts',(5.56839279643728,-5.92073425226441,
34.1568089185258));
#178830=CARTESIAN_POINT('Ctrl Pts',(5.716666013082,-5.77769594188403,34.1648734418481));
#178831=CARTESIAN_POINT('Ctrl Pts',(5.85924639888388,-5.62929118092733,
34.1729379651705));
#178832=CARTESIAN_POINT('Ctrl Pts',(6.00545155325516,-5.47711358045951,
34.1812075098953));
#178833=CARTESIAN_POINT('Ctrl Pts',(6.14567034559919,-5.31929331423924,
34.1894770546201));
#178834=CARTESIAN_POINT('Ctrl Pts',(6.27947735424209,-5.15634092356787,
34.197746599345));
#178835=CARTESIAN_POINT('Ctrl Pts',(6.41014328753384,-4.99721378646835,
34.2058220192376));
#178836=CARTESIAN_POINT('Ctrl Pts',(6.53469492018589,-4.83319304331193,
34.2138974391303));
#178837=CARTESIAN_POINT('Ctrl Pts',(6.65277901944452,-4.66478497692431,
34.2219728590229));
#178838=CARTESIAN_POINT('Ctrl Pts',(6.77512105010348,-4.49030437411188,
34.2303394661638));
#178839=CARTESIAN_POINT('Ctrl Pts',(6.89052025400354,-4.31111448626926,
34.2387060733048));
#178840=CARTESIAN_POINT('Ctrl Pts',(6.99863465908814,-4.12780819214147,
34.2470726804457));
#178841=CARTESIAN_POINT('Ctrl Pts',(7.10674906417275,-3.94450189801367,
34.2554392875867));
#178842=CARTESIAN_POINT('Ctrl Pts',(7.20757852552032,-3.75707954566137,
34.2638058947276));
#178843=CARTESIAN_POINT('Ctrl Pts',(7.30083524784917,-3.56615931307942,
34.2721725018686));
#178844=CARTESIAN_POINT('Ctrl Pts',(7.39190886085651,-3.37970846060229,
34.280343249477));
#178845=CARTESIAN_POINT('Ctrl Pts',(7.4759325855816,-3.18956949062817,34.2885139970854));
#178846=CARTESIAN_POINT('Ctrl Pts',(7.55260879493786,-2.99629570522125,
34.2966847446939));
#178847=CARTESIAN_POINT('Ctrl Pts',(7.62918229596141,-2.80328081143694,
34.3048445475273));
#178848=CARTESIAN_POINT('Ctrl Pts',(7.69842779444841,-2.60713975455653,
34.3130043503606));
#178849=CARTESIAN_POINT('Ctrl Pts',(7.76009405630176,-2.4084492520811,34.321164153194));
#178850=CARTESIAN_POINT('Ctrl Pts',(7.82165318383096,-2.2101039395371,34.3293097797998));
#178851=CARTESIAN_POINT('Ctrl Pts',(7.87565925711571,-2.00921830639751,
34.3374554064056));
#178852=CARTESIAN_POINT('Ctrl Pts',(7.92190957329863,-1.80638763142893,
34.3456010330114));
#178853=CARTESIAN_POINT('Ctrl Pts',(7.9681129779998,-1.60376268667573,34.3537383975458));
#178854=CARTESIAN_POINT('Ctrl Pts',(8.00657624106007,-1.39919692676357,
34.3618757620802));
#178855=CARTESIAN_POINT('Ctrl Pts',(8.03714624980014,-1.19330118655077,
34.3700131266146));
#178856=CARTESIAN_POINT('Ctrl Pts',(8.06767649776054,-0.987673243944254,
34.378139907313));
#178857=CARTESIAN_POINT('Ctrl Pts',(8.09033393005807,-0.780719070800755,
34.3862666880114));
#178858=CARTESIAN_POINT('Ctrl Pts',(8.10501632571067,-0.573060138609772,
34.3943934687099));
#178859=CARTESIAN_POINT('Ctrl Pts',(8.1184513582358,-0.383043156767717,
34.4018298275706));
#178860=CARTESIAN_POINT('Ctrl Pts',(8.12520938963273,-0.192436394347444,
34.4092661864313));
#178861=CARTESIAN_POINT('Ctrl Pts',(8.12524981744152,-0.00172240138687737,
34.416702545292));
#178862=CARTESIAN_POINT('',(8.12804752138608,0.000138485945550895,30.4167025567876));
#178863=CARTESIAN_POINT('Ctrl Pts',(8.12804752138608,0.000138485945550895,
30.4167025567876));
#178864=CARTESIAN_POINT('Ctrl Pts',(8.13188959766799,0.403006519365657,
30.4325194828565));
#178865=CARTESIAN_POINT('Ctrl Pts',(8.01567158785024,2.15330402273085,30.5012255640209));
#178866=CARTESIAN_POINT('Ctrl Pts',(6.73558121933894,5.11366765981583,30.6228208002808));
#178867=CARTESIAN_POINT('Ctrl Pts',(3.50109731423418,7.71360667956193,30.7814882655671));
#178868=CARTESIAN_POINT('Ctrl Pts',(-0.62887488263501,8.44934367887132,
30.9401557308536));
#178869=CARTESIAN_POINT('Ctrl Pts',(-4.5833286137765,7.11692082205467,31.09882319614));
#178870=CARTESIAN_POINT('Ctrl Pts',(-7.43229334537612,4.06791197667428,
31.2574906614265));
#178871=CARTESIAN_POINT('Ctrl Pts',(-8.47097384492051,0.00353968824748415,
31.4161581267129));
#178872=CARTESIAN_POINT('Ctrl Pts',(-7.44199729007049,-4.01675585914069,
31.5748255919993));
#178873=CARTESIAN_POINT('Ctrl Pts',(-3.67416070295655,-8.17511883464782,
31.7863822123813));
#178874=CARTESIAN_POINT('Ctrl Pts',(2.38173522129231,-8.63148943733773,
31.9979388327631));
#178875=CARTESIAN_POINT('Ctrl Pts',(6.72405806064641,-5.12185486701296,
32.2094954531451));
#178876=CARTESIAN_POINT('Ctrl Pts',(8.00961219341287,-2.17106617787569,
32.3314536427881));
#178877=CARTESIAN_POINT('Ctrl Pts',(8.12957810661569,-0.414884693015649,
32.4005226773356));
#178878=CARTESIAN_POINT('Ctrl Pts',(8.12588319212562,-0.00333877610576572,
32.4167025567876));
#178879=CARTESIAN_POINT('',(8.12524926709318,0.00223483220777574,28.4167025567876));
#178880=CARTESIAN_POINT('Ctrl Pts',(8.1252482522699,0.00532930435881126,
28.4167025567876));
#178881=CARTESIAN_POINT('Ctrl Pts',(8.12509106864763,0.244977083153327,
28.4260839083502));
#178882=CARTESIAN_POINT('Ctrl Pts',(8.11432752923275,0.484323489608783,
28.4354652599127));
#178883=CARTESIAN_POINT('Ctrl Pts',(8.09306141022359,0.722526520516521,
28.4448466114753));
#178884=CARTESIAN_POINT('Ctrl Pts',(8.07128129778416,0.966486821610978,
28.4544547064821));
#178885=CARTESIAN_POINT('Ctrl Pts',(8.03848466495988,1.20924773715741,28.464062801489));
#178886=CARTESIAN_POINT('Ctrl Pts',(7.99483706199556,1.44991996835765,28.4736708964958));
#178887=CARTESIAN_POINT('Ctrl Pts',(7.95184974422027,1.6869513968819,28.4831336437081));
#178888=CARTESIAN_POINT('Ctrl Pts',(7.89833745508182,1.92195688380524,28.4925963909204));
#178889=CARTESIAN_POINT('Ctrl Pts',(7.8345091458018,2.15410167049931,28.5020591381326));
#178890=CARTESIAN_POINT('Ctrl Pts',(7.76921023230268,2.39159507298165,28.5117399070367));
#178891=CARTESIAN_POINT('Ctrl Pts',(7.6931142730173,2.62609435745481,28.5214206759408));
#178892=CARTESIAN_POINT('Ctrl Pts',(7.60649905761435,2.85672183612825,28.5311014448449));
#178893=CARTESIAN_POINT('Ctrl Pts',(7.51988384221139,3.08734931480173,28.540782213749));
#178894=CARTESIAN_POINT('Ctrl Pts',(7.42274934721133,3.31410495540211,28.5504629826531));
#178895=CARTESIAN_POINT('Ctrl Pts',(7.31542809573566,3.53612773222649,28.5601437515572));
#178896=CARTESIAN_POINT('Ctrl Pts',(7.22959677648631,3.71369282372714,28.5678860500765));
#178897=CARTESIAN_POINT('Ctrl Pts',(7.13721021316495,3.88830969019066,28.5756283485958));
#178898=CARTESIAN_POINT('Ctrl Pts',(7.03850176295656,4.05945568954231,28.583370647115));
#178899=CARTESIAN_POINT('Ctrl Pts',(6.93985479917425,4.23049508043424,28.5911081228834));
#178900=CARTESIAN_POINT('Ctrl Pts',(6.83489396518796,4.39806760432478,28.5988455986518));
#178901=CARTESIAN_POINT('Ctrl Pts',(6.72389947446002,4.56167331358311,28.6065830744202));
#178902=CARTESIAN_POINT('Ctrl Pts',(6.61295439633667,4.72520618873798,28.6143171056137));
#178903=CARTESIAN_POINT('Ctrl Pts',(6.49598120900059,4.884775474622,28.6220511368073));
#178904=CARTESIAN_POINT('Ctrl Pts',(6.37330461960953,5.03990831148383,28.6297851680008));
#178905=CARTESIAN_POINT('Ctrl Pts',(6.25064372895854,5.19502129622804,28.6375182094819));
#178906=CARTESIAN_POINT('Ctrl Pts',(6.12228110297427,5.34569868106632,28.645251250963));
#178907=CARTESIAN_POINT('Ctrl Pts',(5.98858331476219,5.49149865197579,28.6529842924441));
#178908=CARTESIAN_POINT('Ctrl Pts',(5.8548988828592,5.63728405757716,28.6607165614002));
#178909=CARTESIAN_POINT('Ctrl Pts',(5.71588059186604,5.77819276177285,28.6684488303562));
#178910=CARTESIAN_POINT('Ctrl Pts',(5.57193355532975,5.91381805752344,28.6761810993123));
#178911=CARTESIAN_POINT('Ctrl Pts',(5.42793114891565,6.04949552215667,28.6839163425205));
#178912=CARTESIAN_POINT('Ctrl Pts',(5.27899646657123,6.17988527542889,28.6916515857287));
#178913=CARTESIAN_POINT('Ctrl Pts',(5.12557002731086,6.30461889868313,28.699386828937));
#178914=CARTESIAN_POINT('Ctrl Pts',(4.99714421525889,6.40902734962442,28.7058616249058));
#178915=CARTESIAN_POINT('Ctrl Pts',(4.86557192918227,6.50947342548462,28.7123364208746));
#178916=CARTESIAN_POINT('Ctrl Pts',(4.73112823130852,6.60576363650831,28.7188112168435));
#178917=CARTESIAN_POINT('Ctrl Pts',(4.55641704411399,6.73089391296767,28.7272252913479));
#178918=CARTESIAN_POINT('Ctrl Pts',(4.3767721993223,6.84906573986351,28.7356393658523));
#178919=CARTESIAN_POINT('Ctrl Pts',(4.19275952876206,6.95991775069756,28.7440534403567));
#178920=CARTESIAN_POINT('Ctrl Pts',(4.00869546852586,7.07080071944825,28.7524698646806));
#178921=CARTESIAN_POINT('Ctrl Pts',(3.82026137354079,7.17435965494173,28.7608862890045));
#178922=CARTESIAN_POINT('Ctrl Pts',(3.62804930012442,7.27027825040876,28.7693027133284));
#178923=CARTESIAN_POINT('Ctrl Pts',(3.43578955945314,7.36622063301913,28.7777212248669));
#178924=CARTESIAN_POINT('Ctrl Pts',(3.23975020606864,7.45451877506325,28.7861397364054));
#178925=CARTESIAN_POINT('Ctrl Pts',(3.04054596310806,7.53490330453731,28.7945582479439));
#178926=CARTESIAN_POINT('Ctrl Pts',(2.84126520662993,7.61531870937334,28.8029799929975));
#178927=CARTESIAN_POINT('Ctrl Pts',(2.63881737573806,7.6878143275157,28.8114017380511));
#178928=CARTESIAN_POINT('Ctrl Pts',(2.43383649091729,7.75216921241916,28.8198234831048));
#178929=CARTESIAN_POINT('Ctrl Pts',(2.22883338672855,7.81653107321633,28.8282461410525));
#178930=CARTESIAN_POINT('Ctrl Pts',(2.02129693312102,7.87275036272454,28.8366687990003));
#178931=CARTESIAN_POINT('Ctrl Pts',(1.81187618825483,7.92065604864491,28.8450914569481));
#178932=CARTESIAN_POINT('Ctrl Pts',(1.60241561758895,7.96857084484827,28.853515716643));
#178933=CARTESIAN_POINT('Ctrl Pts',(1.39107029708886,8.0081688201962,28.861939976338));
#178934=CARTESIAN_POINT('Ctrl Pts',(1.1785006509006,8.03932980902804,28.8703642360329));
#178935=CARTESIAN_POINT('Ctrl Pts',(1.11866095995868,8.04810182316354,28.8727357180653));
#178936=CARTESIAN_POINT('Ctrl Pts',(1.05872430008753,8.05620555411314,28.8751072000976));
#178937=CARTESIAN_POINT('Ctrl Pts',(0.998705517653771,8.06363905761586,
28.87747868213));
#178938=CARTESIAN_POINT('Ctrl Pts',(0.78549802308374,8.09004543564329,28.8859030073501));
#178939=CARTESIAN_POINT('Ctrl Pts',(0.571231764690501,8.10799285447874,
28.8943273325702));
#178940=CARTESIAN_POINT('Ctrl Pts',(0.356575332115341,8.11742210280005,
28.9027516577903));
#178941=CARTESIAN_POINT('Ctrl Pts',(0.141955994797125,8.12684972163193,
28.911174527184));
#178942=CARTESIAN_POINT('Ctrl Pts',(-0.0730531184909462,8.12776209849467,
28.9195973965777));
#178943=CARTESIAN_POINT('Ctrl Pts',(-0.287780883101245,8.12015207528908,
28.9280202659714));
#178944=CARTESIAN_POINT('Ctrl Pts',(-0.502464767732327,8.1125436072045,
28.9364414141376));
#178945=CARTESIAN_POINT('Ctrl Pts',(-0.716867154888951,8.09641622618733,
28.9448625623037));
#178946=CARTESIAN_POINT('Ctrl Pts',(-0.930318404587091,8.07181486585183,
28.9532837104699));
#178947=CARTESIAN_POINT('Ctrl Pts',(-1.14370976706711,8.0472204078279,28.9617024959461));
#178948=CARTESIAN_POINT('Ctrl Pts',(-1.35615026307032,8.01415674921051,
28.9701212814222));
#178949=CARTESIAN_POINT('Ctrl Pts',(-1.56697583717458,7.97272063277091,
28.9785400668984));
#178950=CARTESIAN_POINT('Ctrl Pts',(-1.77774251856639,7.93129609123299,
28.9869565006432));
#178951=CARTESIAN_POINT('Ctrl Pts',(-1.9868949199916,7.88150381237641,28.995372934388));
#178952=CARTESIAN_POINT('Ctrl Pts',(-2.19377848254012,7.82349177362921,
29.0037893681328));
#178953=CARTESIAN_POINT('Ctrl Pts',(-2.40058695838251,7.76550078987958,
29.0122027472015));
#178954=CARTESIAN_POINT('Ctrl Pts',(-2.60512798586169,7.69929607501525,
29.0206161262701));
#178955=CARTESIAN_POINT('Ctrl Pts',(-2.80676052500101,7.62507592865776,
29.0290295053387));
#178956=CARTESIAN_POINT('Ctrl Pts',(-2.86361230043232,7.60414901323426,
29.0314017193647));
#178957=CARTESIAN_POINT('Ctrl Pts',(-2.92023294230354,7.58258517603043,
29.0337739333906));
#178958=CARTESIAN_POINT('Ctrl Pts',(-2.9766083084613,7.56038957597419,29.0361461474165));
#178959=CARTESIAN_POINT('Ctrl Pts',(-3.16043399909156,7.48801538512858,
29.0438813323272));
#178960=CARTESIAN_POINT('Ctrl Pts',(-3.34173196659764,7.40888809131464,
29.0516165172379));
#178961=CARTESIAN_POINT('Ctrl Pts',(-3.51996838710042,7.32321719712816,
29.0593517021486));
#178962=CARTESIAN_POINT('Ctrl Pts',(-3.69814969249814,7.23757279449892,
29.067084495149));
#178963=CARTESIAN_POINT('Ctrl Pts',(-3.87327101813675,7.14538897388429,
29.0748172881494));
#178964=CARTESIAN_POINT('Ctrl Pts',(-4.04481941675133,7.04692297732645,
29.0825500811498));
#178965=CARTESIAN_POINT('Ctrl Pts',(-4.21634524754578,6.94846993433108,
29.090281856873));
#178966=CARTESIAN_POINT('Ctrl Pts',(-4.3842987816045,6.84373653803983,29.0980136325962));
#178967=CARTESIAN_POINT('Ctrl Pts',(-4.54819242409716,6.73302556328767,
29.1057454083193));
#178968=CARTESIAN_POINT('Ctrl Pts',(-4.71214471220984,6.62227497312603,
29.1134799506829));
#178969=CARTESIAN_POINT('Ctrl Pts',(-4.87203391087088,6.50554272554384,
29.1212144930466));
#178970=CARTESIAN_POINT('Ctrl Pts',(-5.02740159129819,6.38317482153767,
29.1289490354102));
#178971=CARTESIAN_POINT('Ctrl Pts',(-5.18279551159434,6.26078625095693,
29.1366848840517));
#178972=CARTESIAN_POINT('Ctrl Pts',(-5.33366611915968,6.13276035210405,
29.1444207326933));
#178973=CARTESIAN_POINT('Ctrl Pts',(-5.47958864309167,5.9994829664731,29.1521565813349));
#178974=CARTESIAN_POINT('Ctrl Pts',(-5.62563056744023,5.8660965272503,29.1598987597981));
#178975=CARTESIAN_POINT('Ctrl Pts',(-5.76671606303793,5.72745026007294,
29.1676409382614));
#178976=CARTESIAN_POINT('Ctrl Pts',(-5.90245710552311,5.58396701995631,
29.1753831167246));
#178977=CARTESIAN_POINT('Ctrl Pts',(-6.01601324878065,5.46393402867057,
29.1818599487173));
#178978=CARTESIAN_POINT('Ctrl Pts',(-6.12582973275853,5.34051664665965,
29.1883367807101));
#178979=CARTESIAN_POINT('Ctrl Pts',(-6.23170143661774,5.21397974366572,
29.1948136127028));
#178980=CARTESIAN_POINT('Ctrl Pts',(-6.3853236532053,5.03037185969414,29.2042116411742));
#178981=CARTESIAN_POINT('Ctrl Pts',(-6.53072766535562,4.8400916997463,29.2136096696457));
#178982=CARTESIAN_POINT('Ctrl Pts',(-6.66742265689711,4.64383060380061,
29.2230076981171));
#178983=CARTESIAN_POINT('Ctrl Pts',(-6.8043121539704,4.44729024474212,29.2324190991965));
#178984=CARTESIAN_POINT('Ctrl Pts',(-6.93246782083146,4.24475195686816,
29.2418305002759));
#178985=CARTESIAN_POINT('Ctrl Pts',(-7.05144140319556,4.03693716817582,
29.2512419013552));
#178986=CARTESIAN_POINT('Ctrl Pts',(-7.17023585075172,3.82943527972167,
29.2606391319819));
#178987=CARTESIAN_POINT('Ctrl Pts',(-7.27987583040652,3.61667280239571,
29.2700363626085));
#178988=CARTESIAN_POINT('Ctrl Pts',(-7.37995972155779,3.39939436821982,
29.2794335932351));
#178989=CARTESIAN_POINT('Ctrl Pts',(-7.47979116380052,3.18266399130795,
29.2888071205406));
#178990=CARTESIAN_POINT('Ctrl Pts',(-7.57011462987414,2.96144043637393,
29.2981806478461));
#178991=CARTESIAN_POINT('Ctrl Pts',(-7.65057629621841,2.73648860736546,
29.3075541751515));
#178992=CARTESIAN_POINT('Ctrl Pts',(-7.73051544922783,2.51299760232069,
29.3168668313213));
#178993=CARTESIAN_POINT('Ctrl Pts',(-7.80072043542531,2.28582662313103,
29.3261794874911));
#178994=CARTESIAN_POINT('Ctrl Pts',(-7.86088899879242,2.05575088742881,
29.3354921436608));
#178995=CARTESIAN_POINT('Ctrl Pts',(-7.89963083983558,1.90760778608734,
29.3414884551037));
#178996=CARTESIAN_POINT('Ctrl Pts',(-7.93421255934564,1.75826090109098,
29.3474847665466));
#178997=CARTESIAN_POINT('Ctrl Pts',(-7.9645635351637,1.60792265263002,29.3534810779894));
#178998=CARTESIAN_POINT('Ctrl Pts',(-8.00286805180554,1.41818793126225,
29.3610487362034));
#178999=CARTESIAN_POINT('Ctrl Pts',(-8.03441562384965,1.22694884437615,
29.3686163944174));
#179000=CARTESIAN_POINT('Ctrl Pts',(-8.05909331398302,1.03474756294192,
29.3761840526314));
#179001=CARTESIAN_POINT('Ctrl Pts',(-8.08376417130756,0.842599498587761,
29.3837496154969));
#179002=CARTESIAN_POINT('Ctrl Pts',(-8.10156888475985,0.649490134078745,
29.3913151783624));
#179003=CARTESIAN_POINT('Ctrl Pts',(-8.11244591473116,0.455970221683052,
29.3988807412279));
#179004=CARTESIAN_POINT('Ctrl Pts',(-8.12332199177175,0.262467263462304,
29.4064456412785));
#179005=CARTESIAN_POINT('Ctrl Pts',(-8.12727157357842,0.0685541960751146,
29.4140105413291));
#179006=CARTESIAN_POINT('Ctrl Pts',(-8.12428512635025,-0.12521480848541,
29.4215754413797));
#179007=CARTESIAN_POINT('Ctrl Pts',(-8.12129721339224,-0.3190789136761,
29.4291440542365));
#179008=CARTESIAN_POINT('Ctrl Pts',(-8.11136647299121,-0.51279844657361,
29.4367126670933));
#179009=CARTESIAN_POINT('Ctrl Pts',(-8.09453551293872,-0.705820368276455,
29.4442812799501));
#179010=CARTESIAN_POINT('Ctrl Pts',(-8.07770080997662,-0.898885214661145,
29.4518515759333));
#179011=CARTESIAN_POINT('Ctrl Pts',(-8.05396287399185,-1.09125177555957,
29.4594218719166));
#179012=CARTESIAN_POINT('Ctrl Pts',(-8.02341599667671,-1.28237409002689,
29.4669921678998));
#179013=CARTESIAN_POINT('Ctrl Pts',(-7.99283816666645,-1.47369006588444,
29.474570134751));
#179014=CARTESIAN_POINT('Ctrl Pts',(-7.95543768024925,-1.66375891510597,
29.4821481016022));
#179015=CARTESIAN_POINT('Ctrl Pts',(-7.91135977901552,-1.85204589831771,
29.4897260684535));
#179016=CARTESIAN_POINT('Ctrl Pts',(-7.8678856893714,-2.03775358760998,
29.4972002267276));
#179017=CARTESIAN_POINT('Ctrl Pts',(-7.81791611631227,-2.22172761022478,
29.5046743850016));
#179018=CARTESIAN_POINT('Ctrl Pts',(-7.76163701836414,-2.40347214622084,
29.5121485432757));
#179019=CARTESIAN_POINT('Ctrl Pts',(-7.70083495496687,-2.59982289103774,
29.5202233749946));
#179020=CARTESIAN_POINT('Ctrl Pts',(-7.63253904220119,-2.79399077746816,
29.5282982067135));
#179021=CARTESIAN_POINT('Ctrl Pts',(-7.55692786463111,-2.98538587309277,
29.5363730384324));
#179022=CARTESIAN_POINT('Ctrl Pts',(-7.48136671129449,-3.17665434202997,
29.5444425278556));
#179023=CARTESIAN_POINT('Ctrl Pts',(-7.39850006015966,-3.3651533845707,
29.5525120172788));
#179024=CARTESIAN_POINT('Ctrl Pts',(-7.30855578831577,-3.55030982473024,
29.5605815067021));
#179025=CARTESIAN_POINT('Ctrl Pts',(-7.21865877025028,-3.73536898975248,
29.5686467566795));
#179026=CARTESIAN_POINT('Ctrl Pts',(-7.12169168501351,-3.91708877020396,
29.5767120066569));
#179027=CARTESIAN_POINT('Ctrl Pts',(-7.01793009246643,-4.09491694418265,
29.5847772566343));
#179028=CARTESIAN_POINT('Ctrl Pts',(-6.91420889215014,-4.27267589335023,
29.5928393669776));
#179029=CARTESIAN_POINT('Ctrl Pts',(-6.80369861926473,-4.44654598430514,
29.6009014773209));
#179030=CARTESIAN_POINT('Ctrl Pts',(-6.6867205455098,-4.61599999011667,
29.6089635876641));
#179031=CARTESIAN_POINT('Ctrl Pts',(-6.56977210215631,-4.78541107343805,
29.6170236558848));
#179032=CARTESIAN_POINT('Ctrl Pts',(-6.44635930570642,-4.95040804246024,
29.6250837241055));
#179033=CARTESIAN_POINT('Ctrl Pts',(-6.31684682282501,-5.11049251828682,
29.6331437923262));
#179034=CARTESIAN_POINT('Ctrl Pts',(-6.18539404979508,-5.27297529831132,
29.6413246123897));
#179035=CARTESIAN_POINT('Ctrl Pts',(-6.04765755625816,-5.43039694305914,
29.6495054324531));
#179036=CARTESIAN_POINT('Ctrl Pts',(-5.90406171228676,-5.58227040369862,
29.6576862525165));
#179037=CARTESIAN_POINT('Ctrl Pts',(-5.76257165986339,-5.73191668393412,
29.6657471032182));
#179038=CARTESIAN_POINT('Ctrl Pts',(-5.61539316654647,-5.87617616748634,
29.67380795392));
#179039=CARTESIAN_POINT('Ctrl Pts',(-5.46297025584037,-6.01461915222431,
29.6818688046217));
#179040=CARTESIAN_POINT('Ctrl Pts',(-5.31052206718053,-6.1530850964724,
29.6899309921422));
#179041=CARTESIAN_POINT('Ctrl Pts',(-5.15282796097336,-6.28573240484384,
29.6979931796627));
#179042=CARTESIAN_POINT('Ctrl Pts',(-4.99036650953078,-6.41217043309467,
29.7060553671832));
#179043=CARTESIAN_POINT('Ctrl Pts',(-4.82785798925588,-6.53864509336066,
29.7141198905055));
#179044=CARTESIAN_POINT('Ctrl Pts',(-4.66057961893391,-6.65890669085907,
29.7221844138278));
#179045=CARTESIAN_POINT('Ctrl Pts',(-4.48904099831805,-6.77260647593817,
29.7302489371502));
#179046=CARTESIAN_POINT('Ctrl Pts',(-4.31314141460697,-6.88919680872534,
29.738518481875));
#179047=CARTESIAN_POINT('Ctrl Pts',(-4.13276239494973,-6.99888707914173,
29.7467880265999));
#179048=CARTESIAN_POINT('Ctrl Pts',(-3.94848241085994,-7.1013501683574,
29.7550575713248));
#179049=CARTESIAN_POINT('Ctrl Pts',(-3.76852833855681,-7.20140797038181,
29.7631329912174));
#179050=CARTESIAN_POINT('Ctrl Pts',(-3.58485469236599,-7.29457397854348,
29.77120841111));
#179051=CARTESIAN_POINT('Ctrl Pts',(-3.39802282682166,-7.38059133341624,
29.7792838310027));
#179052=CARTESIAN_POINT('Ctrl Pts',(-3.20445409092812,-7.46971034209882,
29.7876504381436));
#179053=CARTESIAN_POINT('Ctrl Pts',(-3.00749549223416,-7.55115543137243,
29.7960170452846));
#179054=CARTESIAN_POINT('Ctrl Pts',(-2.80779156485647,-7.62469632777731,
29.8043836524256));
#179055=CARTESIAN_POINT('Ctrl Pts',(-2.60808763747882,-7.69823722418218,
29.8127502595666));
#179056=CARTESIAN_POINT('Ctrl Pts',(-2.4056387498038,-7.7638738474689,29.8211168667075));
#179057=CARTESIAN_POINT('Ctrl Pts',(-2.20110462445034,-7.82143375569488,
29.8294834738485));
#179058=CARTESIAN_POINT('Ctrl Pts',(-2.00362718461449,-7.87700777442652,
29.8375614224816));
#179059=CARTESIAN_POINT('Ctrl Pts',(-1.80382204229118,-7.92516113503516,
29.8456393711146));
#179060=CARTESIAN_POINT('Ctrl Pts',(-1.60227339677148,-7.96570194800799,
29.8537173197477));
#179061=CARTESIAN_POINT('Ctrl Pts',(-1.40097140586131,-8.0061931472592,
29.8617853826122));
#179062=CARTESIAN_POINT('Ctrl Pts',(-1.19793047197389,-8.03909030748399,
29.8698534454767));
#179063=CARTESIAN_POINT('Ctrl Pts',(-0.993749792458142,-8.0642512927419,
29.8779215083412));
#179064=CARTESIAN_POINT('Ctrl Pts',(-0.789793851398478,-8.08938458369987,
29.885980690816));
#179065=CARTESIAN_POINT('Ctrl Pts',(-0.584700977059645,-8.10679863641572,
29.8940398732909));
#179066=CARTESIAN_POINT('Ctrl Pts',(-0.379081006085367,-8.11640222964124,
29.9020990557657));
#179067=CARTESIAN_POINT('Ctrl Pts',(-0.173725146775017,-8.12599348738702,
29.9101478865024));
#179068=CARTESIAN_POINT('Ctrl Pts',(0.0321561446039651,-8.12779428496848,
29.9181967172391));
#179069=CARTESIAN_POINT('Ctrl Pts',(0.237947405400235,-8.12176511570996,
29.9262455479758));
#179070=CARTESIAN_POINT('Ctrl Pts',(0.443583006615233,-8.11574050688788,
29.9342882906133));
#179071=CARTESIAN_POINT('Ctrl Pts',(0.649128398758211,-8.10189774556756,
29.9423310332508));
#179072=CARTESIAN_POINT('Ctrl Pts',(0.853966240181079,-8.08024932926769,
29.9503737758882));
#179073=CARTESIAN_POINT('Ctrl Pts',(1.05863723347137,-8.05861854641782,
29.9584099674091));
#179074=CARTESIAN_POINT('Ctrl Pts',(1.26260151263647,-8.02919482440692,
29.9664461589299));
#179075=CARTESIAN_POINT('Ctrl Pts',(1.46524469802764,-7.9920426386126,29.9744823504507));
#179076=CARTESIAN_POINT('Ctrl Pts',(1.58013520487318,-7.97097884883803,
29.9790385466788));
#179077=CARTESIAN_POINT('Ctrl Pts',(1.69460110762108,-7.94743174291968,
29.983594742907));
#179078=CARTESIAN_POINT('Ctrl Pts',(1.80853123421068,-7.92142047472449,
29.9881509391351));
#179079=CARTESIAN_POINT('Ctrl Pts',(2.00948858316323,-7.8755401122965,29.9961874536438));
#179080=CARTESIAN_POINT('Ctrl Pts',(2.20861949664047,-7.82202660687131,
30.0042239681525));
#179081=CARTESIAN_POINT('Ctrl Pts',(2.40533228911578,-7.76106076135454,
30.0122604826611));
#179082=CARTESIAN_POINT('Ctrl Pts',(2.60216391569675,-7.70005808639909,
30.0203018520245));
#179083=CARTESIAN_POINT('Ctrl Pts',(2.79657420525973,-7.63159418320123,
30.0283432213878));
#179084=CARTESIAN_POINT('Ctrl Pts',(2.98798925228111,-7.55589887377753,
30.0363845907511));
#179085=CARTESIAN_POINT('Ctrl Pts',(3.17954333713474,-7.48014858167667,
30.0444318011107));
#179086=CARTESIAN_POINT('Ctrl Pts',(3.36809754543241,-7.39715651978964,
30.0524790114702));
#179087=CARTESIAN_POINT('Ctrl Pts',(3.55309991214548,-7.30719977671418,
30.0605262218297));
#179088=CARTESIAN_POINT('Ctrl Pts',(3.7383749591358,-7.21711044382337,30.0685852932027));
#179089=CARTESIAN_POINT('Ctrl Pts',(3.92008741688246,-7.12003605088192,
30.0766443645756));
#179090=CARTESIAN_POINT('Ctrl Pts',(4.09771027214318,-7.0162994582666,30.0847034359486));
#179091=CARTESIAN_POINT('Ctrl Pts',(4.27547688629555,-6.91247890653715,
30.0927690299234));
#179092=CARTESIAN_POINT('Ctrl Pts',(4.44914702680273,-6.80198556403027,
30.1008346238982));
#179093=CARTESIAN_POINT('Ctrl Pts',(4.61822371020947,-6.6851849132959,30.108900217873));
#179094=CARTESIAN_POINT('Ctrl Pts',(4.78756588263793,-6.56820085885455,
30.1169784766731));
#179095=CARTESIAN_POINT('Ctrl Pts',(4.95229992811656,-6.44488988889585,
30.1250567354732));
#179096=CARTESIAN_POINT('Ctrl Pts',(5.11196154100573,-6.31565806276577,
30.1331349942733));
#179097=CARTESIAN_POINT('Ctrl Pts',(5.20210948782359,-6.24269134535427,
30.1376961309893));
#179098=CARTESIAN_POINT('Ctrl Pts',(5.29064102548129,-6.16783777771843,
30.1422572677054));
#179099=CARTESIAN_POINT('Ctrl Pts',(5.37747790963913,-6.09117549360082,
30.1468184044214));
#179100=CARTESIAN_POINT('Ctrl Pts',(5.52883585597059,-5.95755202244966,
30.1547685317547));
#179101=CARTESIAN_POINT('Ctrl Pts',(5.6753673482983,-5.81814516238551,30.1627186590879));
#179102=CARTESIAN_POINT('Ctrl Pts',(5.81661134720278,-5.6733341165572,30.1706687864212));
#179103=CARTESIAN_POINT('Ctrl Pts',(5.95772227539224,-5.52865950207861,
30.1786114236725));
#179104=CARTESIAN_POINT('Ctrl Pts',(6.09355540705588,-5.37859108581603,
30.1865540609238));
#179105=CARTESIAN_POINT('Ctrl Pts',(6.22368390162456,-5.2235472865821,30.194496698175));
#179106=CARTESIAN_POINT('Ctrl Pts',(6.35371169464857,-5.06862346990947,
30.2024331889183));
#179107=CARTESIAN_POINT('Ctrl Pts',(6.4780434366407,-4.90873219855639,30.2103696796615));
#179108=CARTESIAN_POINT('Ctrl Pts',(6.59628989787571,-4.7443278918813,30.2183061704047));
#179109=CARTESIAN_POINT('Ctrl Pts',(6.71945343540229,-4.57308711407514,
30.226572686504));
#179110=CARTESIAN_POINT('Ctrl Pts',(6.83601451609805,-4.39695019710985,
30.2348392026033));
#179111=CARTESIAN_POINT('Ctrl Pts',(6.94557959981183,-4.21646908979275,
30.2431057187026));
#179112=CARTESIAN_POINT('Ctrl Pts',(7.05066059802903,-4.04337439325814,
30.2510339174868));
#179113=CARTESIAN_POINT('Ctrl Pts',(7.1493066296484,-3.86628431438256,30.258962116271));
#179114=CARTESIAN_POINT('Ctrl Pts',(7.2412145404669,-3.68571560777968,30.2668903150552));
#179115=CARTESIAN_POINT('Ctrl Pts',(7.33310268708142,-3.50518573131358,
30.2748168089314));
#179116=CARTESIAN_POINT('Ctrl Pts',(7.41825544997759,-3.32117901450807,
30.2827433028075));
#179117=CARTESIAN_POINT('Ctrl Pts',(7.49641562669018,-3.13423679935248,
30.2906697966837));
#179118=CARTESIAN_POINT('Ctrl Pts',(7.57457091042752,-2.94730628713398,
30.2985957943463));
#179119=CARTESIAN_POINT('Ctrl Pts',(7.64573435264783,-2.75744095010262,
30.3065217920089));
#179120=CARTESIAN_POINT('Ctrl Pts',(7.70969674304275,-2.56520246624238,
30.3144477896715));
#179121=CARTESIAN_POINT('Ctrl Pts',(7.773664879282,-2.37294671329017,30.3223744993392));
#179122=CARTESIAN_POINT('Ctrl Pts',(7.8304305701621,-2.17831770466007,30.3303012090069));
#179123=CARTESIAN_POINT('Ctrl Pts',(7.87983423502881,-1.98189303217099,
30.3382279186747));
#179124=CARTESIAN_POINT('Ctrl Pts',(7.92926493333466,-1.7853608770803,30.3461589657984));
#179125=CARTESIAN_POINT('Ctrl Pts',(7.97132547621662,-1.5870314181205,30.3540900129221));
#179126=CARTESIAN_POINT('Ctrl Pts',(8.0059070414091,-1.38749414658807,30.3620210600459));
#179127=CARTESIAN_POINT('Ctrl Pts',(8.04049966217458,-1.18789308387503,
30.3699546426902));
#179128=CARTESIAN_POINT('Ctrl Pts',(8.06760848826027,-0.987083767686729,
30.3778882253345));
#179129=CARTESIAN_POINT('Ctrl Pts',(8.08717641414289,-0.785662274155305,
30.3858218079788));
#179130=CARTESIAN_POINT('Ctrl Pts',(8.10675980185596,-0.584081625024089,
30.3937616594382));
#179131=CARTESIAN_POINT('Ctrl Pts',(8.1187903637721,-0.381888164136896,
30.4017015108977));
#179132=CARTESIAN_POINT('Ctrl Pts',(8.12326304575953,-0.17968041601016,
30.4096413623571));
#179133=CARTESIAN_POINT('Ctrl Pts',(8.12458895121676,-0.119736883809696,
30.4119950938339));
#179134=CARTESIAN_POINT('Ctrl Pts',(8.12525101991889,-0.0597920845778729,
30.4143488253108));
#179135=CARTESIAN_POINT('Ctrl Pts',(8.12524999882064,0.000138438281265886,
30.4167025567876));
#179136=CARTESIAN_POINT('',(8.12479782686936,-0.00219746833155191,26.4167025567876));
#179137=CARTESIAN_POINT('Ctrl Pts',(8.12525,8.95881079881578E-13,26.4167025567876));
#179138=CARTESIAN_POINT('Ctrl Pts',(8.12524999999975,2.24624642433496,26.5047001499288));
#179139=CARTESIAN_POINT('Ctrl Pts',(7.14398562317555,4.4753524975352,26.59269774307));
#179140=CARTESIAN_POINT('Ctrl Pts',(3.83078204044869,7.50935546634392,26.7686929293524));
#179141=CARTESIAN_POINT('Ctrl Pts',(1.52412477697682,8.29110090552147,26.8566905224936));
#179142=CARTESIAN_POINT('Ctrl Pts',(-2.95101623932607,7.89663306204406,
27.032685708776));
#179143=CARTESIAN_POINT('Ctrl Pts',(-5.08535169588768,6.7234298308576,27.1206833019172));
#179144=CARTESIAN_POINT('Ctrl Pts',(-7.81671694684414,3.15661951052912,
27.2966784881996));
#179145=CARTESIAN_POINT('Ctrl Pts',(-8.39290461146703,0.790229551553876,
27.3846760813408));
#179146=CARTESIAN_POINT('Ctrl Pts',(-7.60701611462477,-3.63299000730427,
27.5606712676232));
#179147=CARTESIAN_POINT('Ctrl Pts',(-6.25093680401351,-5.65606750610023,
27.6486688607644));
#179148=CARTESIAN_POINT('Ctrl Pts',(-2.45807268688558,-8.06369575488316,
27.8246640470468));
#179149=CARTESIAN_POINT('Ctrl Pts',(-0.050229951045439,-8.42987470330085,
27.912661640188));
#179150=CARTESIAN_POINT('Ctrl Pts',(4.2868996088098,-7.2586363943457,28.0886568264704));
#179151=CARTESIAN_POINT('Ctrl Pts',(6.18309125557144,-5.73015646266396,
28.1766544196116));
#179152=CARTESIAN_POINT('Ctrl Pts',(7.8105055920291,-2.5864071380026,28.3153355274311));
#179153=CARTESIAN_POINT('Ctrl Pts',(8.12525000000015,-1.29375883538096,
28.3660190421094));
#179154=CARTESIAN_POINT('Ctrl Pts',(8.12525,9.51624341237972E-13,28.4167025567876));
#179155=CARTESIAN_POINT('',(8.12465437257904,0.000424865304964707,24.4167025657623));
#179156=CARTESIAN_POINT('Ctrl Pts',(8.12465437257904,0.000424865304964707,
24.4167025657623));
#179157=CARTESIAN_POINT('Ctrl Pts',(8.12471506055511,0.154179418475467,
24.4227315952114));
#179158=CARTESIAN_POINT('Ctrl Pts',(8.08253234226184,1.65664906305814,24.4816497797562));
#179159=CARTESIAN_POINT('Ctrl Pts',(7.20239531903253,4.46233054468966,24.5934571193965));
#179160=CARTESIAN_POINT('Ctrl Pts',(4.17773714921789,7.36911953511172,24.7521245846828));
#179161=CARTESIAN_POINT('Ctrl Pts',(0.172450800896666,8.45505245510799,
24.9107920499693));
#179162=CARTESIAN_POINT('Ctrl Pts',(-5.30273476857889,7.22585834388332,
25.1223486703512));
#179163=CARTESIAN_POINT('Ctrl Pts',(-8.68429813962363,2.18133867002514,
25.3339052907331));
#179164=CARTESIAN_POINT('Ctrl Pts',(-7.77043274392747,-3.32666936346071,
25.545461911115));
#179165=CARTESIAN_POINT('Ctrl Pts',(-4.41553899415244,-7.78962694628804,
25.757018531497));
#179166=CARTESIAN_POINT('Ctrl Pts',(1.56871213603083,-8.82446412344869,
25.9685751518788));
#179167=CARTESIAN_POINT('Ctrl Pts',(6.23719048967391,-5.71096367462437,
26.1801317722608));
#179168=CARTESIAN_POINT('Ctrl Pts',(7.88015377287066,-2.68210296929991,
26.3118778555319));
#179169=CARTESIAN_POINT('Ctrl Pts',(8.12460569558809,-0.666438545426924,
26.3907347837075));
#179170=CARTESIAN_POINT('Ctrl Pts',(8.12479782686936,-0.00219746833155191,
26.4167025567876));
#179171=CARTESIAN_POINT('',(8.12525,8.99861782310829E-13,22.4167025567876));
#179172=CARTESIAN_POINT('Ctrl Pts',(8.12524999843797,0.000159322666138746,
22.4167025567876));
#179173=CARTESIAN_POINT('Ctrl Pts',(8.12524613254614,0.19731480844615,22.4244104961116));
#179174=CARTESIAN_POINT('Ctrl Pts',(8.11806209000327,0.39450754566343,22.4321184354356));
#179175=CARTESIAN_POINT('Ctrl Pts',(8.10371576501125,0.591166949691999,
22.4398263747596));
#179176=CARTESIAN_POINT('Ctrl Pts',(8.08936474420554,0.787890723928413,
22.4475368370327));
#179177=CARTESIAN_POINT('Ctrl Pts',(8.06784677763421,0.984080460747862,
22.4552472993057));
#179178=CARTESIAN_POINT('Ctrl Pts',(8.03923178276477,1.17916915897796,22.4629577615788));
#179179=CARTESIAN_POINT('Ctrl Pts',(8.01061268339087,1.37428584052358,22.4706693298323));
#179180=CARTESIAN_POINT('Ctrl Pts',(7.97489458651551,1.56830081786643,22.4783808980859));
#179181=CARTESIAN_POINT('Ctrl Pts',(7.93219875068048,1.76065628167539,22.4860924663395));
#179182=CARTESIAN_POINT('Ctrl Pts',(7.88946783566493,1.95316978600304,22.4938103704684));
#179183=CARTESIAN_POINT('Ctrl Pts',(7.83974781083228,2.14402070647978,22.5015282745973));
#179184=CARTESIAN_POINT('Ctrl Pts',(7.78321038226485,2.33266450821901,22.5092461787263));
#179185=CARTESIAN_POINT('Ctrl Pts',(7.73062827977641,2.50811089777367,22.5164241427085));
#179186=CARTESIAN_POINT('Ctrl Pts',(7.67214987165433,2.68164812048831,22.5236021066907));
#179187=CARTESIAN_POINT('Ctrl Pts',(7.60795081508275,2.85285330113233,22.5307800706729));
#179188=CARTESIAN_POINT('Ctrl Pts',(7.52389570377249,3.07701034150697,22.5401780991444));
#179189=CARTESIAN_POINT('Ctrl Pts',(7.42998474518825,3.29730468523387,22.549576127616));
#179190=CARTESIAN_POINT('Ctrl Pts',(7.32657761269766,3.51296855203934,22.5589741560875));
#179191=CARTESIAN_POINT('Ctrl Pts',(7.2230233405123,3.72893929047707,22.568385557167));
#179192=CARTESIAN_POINT('Ctrl Pts',(7.10994588178427,3.94026633875174,22.5777969582464));
#179193=CARTESIAN_POINT('Ctrl Pts',(6.98775206573189,4.14620412309376,22.5872083593259));
#179194=CARTESIAN_POINT('Ctrl Pts',(6.86574223309334,4.35183183334347,22.5966055899526));
#179195=CARTESIAN_POINT('Ctrl Pts',(6.73464349860567,4.55208646802926,22.6060028205793));
#179196=CARTESIAN_POINT('Ctrl Pts',(6.59490586401416,4.74625159544789,22.615400051206));
#179197=CARTESIAN_POINT('Ctrl Pts',(6.45552069986431,4.93992696598452,22.6247735785116));
#179198=CARTESIAN_POINT('Ctrl Pts',(6.30754016686787,5.12754346748758,22.6341471058171));
#179199=CARTESIAN_POINT('Ctrl Pts',(6.15145546131005,5.30841626759043,22.6435206331227));
#179200=CARTESIAN_POINT('Ctrl Pts',(5.99638436066216,5.48811449035336,22.6528332892925));
#179201=CARTESIAN_POINT('Ctrl Pts',(5.83331401469013,5.66115626605527,22.6621459454623));
#179202=CARTESIAN_POINT('Ctrl Pts',(5.66277000741065,5.82689655010885,22.6714586016321));
#179203=CARTESIAN_POINT('Ctrl Pts',(5.55295869647669,5.93361479929755,22.6774549130745));
#179204=CARTESIAN_POINT('Ctrl Pts',(5.44004974799199,6.03730644182918,22.6834512245169));
#179205=CARTESIAN_POINT('Ctrl Pts',(5.32419319158091,6.1378053424024,22.6894475359593));
#179206=CARTESIAN_POINT('Ctrl Pts',(5.17797616646616,6.2646402037544,22.6970151941733));
#179207=CARTESIAN_POINT('Ctrl Pts',(5.02712019411757,6.3863370125112,22.7045828523873));
#179208=CARTESIAN_POINT('Ctrl Pts',(4.87204137709522,6.50253030614792,22.7121505106013));
#179209=CARTESIAN_POINT('Ctrl Pts',(4.71700549860974,6.61869142795021,22.7197160734668));
#179210=CARTESIAN_POINT('Ctrl Pts',(4.55774939586706,6.72935184644465,22.7272816363322));
#179211=CARTESIAN_POINT('Ctrl Pts',(4.39472196805478,6.83418659285775,22.7348471991977));
#179212=CARTESIAN_POINT('Ctrl Pts',(4.23170882298712,6.93901215475553,22.7424120992483));
#179213=CARTESIAN_POINT('Ctrl Pts',(4.06492532018506,7.03801286229386,22.7499769992989));
#179214=CARTESIAN_POINT('Ctrl Pts',(3.89484896389969,7.13090731330239,22.7575418993495));
#179215=CARTESIAN_POINT('Ctrl Pts',(3.7246891351898,7.22384735633334,22.7651105122063));
#179216=CARTESIAN_POINT('Ctrl Pts',(3.55123354591468,7.31067497624838,22.7726791250631));
#179217=CARTESIAN_POINT('Ctrl Pts',(3.37498441075564,7.39115469934545,22.7802477379199));
#179218=CARTESIAN_POINT('Ctrl Pts',(3.19869608088749,7.47165231971807,22.7878180339031));
#179219=CARTESIAN_POINT('Ctrl Pts',(3.01961330681129,7.54579908893877,22.7953883298864));
#179220=CARTESIAN_POINT('Ctrl Pts',(2.83825761526305,7.61340799326434,22.8029586258696));
#179221=CARTESIAN_POINT('Ctrl Pts',(2.656718158698,7.68108540468407,22.8105365927208));
#179222=CARTESIAN_POINT('Ctrl Pts',(2.47290153176808,7.74221159786422,22.818114559572));
#179223=CARTESIAN_POINT('Ctrl Pts',(2.28734460604277,7.79664942239338,22.8256925264233));
#179224=CARTESIAN_POINT('Ctrl Pts',(2.1043295758947,7.85034151746586,22.8331666846974));
#179225=CARTESIAN_POINT('Ctrl Pts',(1.91962196643571,7.89752730173872,22.8406408429716));
#179226=CARTESIAN_POINT('Ctrl Pts',(1.73374485027924,7.93812423413934,22.8481150012457));
#179227=CARTESIAN_POINT('Ctrl Pts',(1.53292940346886,7.98198380807579,22.8561898329646));
#179228=CARTESIAN_POINT('Ctrl Pts',(1.33032021960521,8.01824699099574,22.8642646646835));
#179229=CARTESIAN_POINT('Ctrl Pts',(1.12651862753549,8.04677844508692,22.8723394964024));
#179230=CARTESIAN_POINT('Ctrl Pts',(0.922851870271271,8.07529102281397,
22.8804089858256));
#179231=CARTESIAN_POINT('Ctrl Pts',(0.717994590687884,8.09608202834019,
22.8884784752488));
#179232=CARTESIAN_POINT('Ctrl Pts',(0.512557829620091,8.10906727273828,
22.8965479646721));
#179233=CARTESIAN_POINT('Ctrl Pts',(0.307228998306923,8.12204569511371,
22.9046132146495));
#179234=CARTESIAN_POINT('Ctrl Pts',(0.101321608117274,8.12722651473287,
22.9126784646269));
#179235=CARTESIAN_POINT('Ctrl Pts',(-0.104548033950805,8.12457735953674,
22.9207437146043));
#179236=CARTESIAN_POINT('Ctrl Pts',(-0.310337535247146,8.12192923560166,
22.9288058249476));
#179237=CARTESIAN_POINT('Ctrl Pts',(-0.516089001426615,8.11145722018747,
22.9368679352909));
#179238=CARTESIAN_POINT('Ctrl Pts',(-0.721185346747057,8.0931810345585,
22.9449300456341));
#179239=CARTESIAN_POINT('Ctrl Pts',(-0.926229741416818,8.07490947826475,
22.9529901138548));
#179240=CARTESIAN_POINT('Ctrl Pts',(-1.1306190309936,8.04883772304286,22.9610501820755));
#179241=CARTESIAN_POINT('Ctrl Pts',(-1.33373984546315,8.01503746635809,
22.9691102502962));
#179242=CARTESIAN_POINT('Ctrl Pts',(-1.53990371266804,7.98073083141845,
22.9772910703597));
#179243=CARTESIAN_POINT('Ctrl Pts',(-1.74476046205535,7.93846230746238,
22.9854718904231));
#179244=CARTESIAN_POINT('Ctrl Pts',(-1.9476771592851,7.88836112546194,22.9936527104865));
#179245=CARTESIAN_POINT('Ctrl Pts',(-2.14761814179938,7.83899466281469,
23.0017135611882));
#179246=CARTESIAN_POINT('Ctrl Pts',(-2.34567527301639,7.78202379074947,
23.00977441189));
#179247=CARTESIAN_POINT('Ctrl Pts',(-2.54125583220034,7.71762310286061,
23.0178352625917));
#179248=CARTESIAN_POINT('Ctrl Pts',(-2.73686882664154,7.65321173470327,
23.0258974501122));
#179249=CARTESIAN_POINT('Ctrl Pts',(-2.93000412883017,7.58136819220191,
23.0339596376327));
#179250=CARTESIAN_POINT('Ctrl Pts',(-3.12008597723112,7.50231637943814,
23.0420218251532));
#179251=CARTESIAN_POINT('Ctrl Pts',(-3.31022289673115,7.42324166353947,
23.0500863484755));
#179252=CARTESIAN_POINT('Ctrl Pts',(-3.49730430546083,7.33695463370158,
23.0581508717979));
#179253=CARTESIAN_POINT('Ctrl Pts',(-3.68077560478952,7.24372683842277,
23.0662153951202));
#179254=CARTESIAN_POINT('Ctrl Pts',(-3.86891122730385,7.14812894728343,
23.0744849398451));
#179255=CARTESIAN_POINT('Ctrl Pts',(-4.05325043723003,7.04523287427622,
23.0827544845699));
#179256=CARTESIAN_POINT('Ctrl Pts',(-4.23322351628943,6.93538075549094,
23.0910240292948));
#179257=CARTESIAN_POINT('Ctrl Pts',(-4.40897178673598,6.82810737892651,
23.0990994491874));
#179258=CARTESIAN_POINT('Ctrl Pts',(-4.58055636480016,6.71420107553466,
23.1071748690801));
#179259=CARTESIAN_POINT('Ctrl Pts',(-4.74747710272014,6.5940237125482,23.1152502889727));
#179260=CARTESIAN_POINT('Ctrl Pts',(-4.9204167462837,6.46951293828328,23.1236168961137));
#179261=CARTESIAN_POINT('Ctrl Pts',(-5.08834965723348,6.33827068294546,
23.1319835032547));
#179262=CARTESIAN_POINT('Ctrl Pts',(-5.25075782862163,6.20074429304004,
23.1403501103956));
#179263=CARTESIAN_POINT('Ctrl Pts',(-5.41316600000977,6.06321790313462,
23.1487167175366));
#179264=CARTESIAN_POINT('Ctrl Pts',(-5.57004918046089,5.91940765965785,
23.1570833246776));
#179265=CARTESIAN_POINT('Ctrl Pts',(-5.72093219888789,5.76980262558675,
23.1654499318186));
#179266=CARTESIAN_POINT('Ctrl Pts',(-5.86660956271246,5.62535915404454,
23.1735278804516));
#179267=CARTESIAN_POINT('Ctrl Pts',(-6.0069771118089,5.47523323290718,23.1816058290847));
#179268=CARTESIAN_POINT('Ctrl Pts',(-6.14157997247383,5.31983862576755,
23.1896837777177));
#179269=CARTESIAN_POINT('Ctrl Pts',(-6.27601810657397,5.16463419006776,
23.1977518405822));
#179270=CARTESIAN_POINT('Ctrl Pts',(-6.40470540980992,5.00417415775252,
23.2058199034467));
#179271=CARTESIAN_POINT('Ctrl Pts',(-6.52722290931678,4.83890986220969,
23.2138879663112));
#179272=CARTESIAN_POINT('Ctrl Pts',(-6.6496055557427,4.67382747047254,23.221947148786));
#179273=CARTESIAN_POINT('Ctrl Pts',(-6.76583174964362,4.50395160936267,
23.2300063312609));
#179274=CARTESIAN_POINT('Ctrl Pts',(-6.87552157740191,4.32976796158649,
23.2380655137357));
#179275=CARTESIAN_POINT('Ctrl Pts',(-6.98507051241126,4.1558080466163,23.2461143444724));
#179276=CARTESIAN_POINT('Ctrl Pts',(-7.0880996629979,3.97755164942091,23.2541631752091));
#179277=CARTESIAN_POINT('Ctrl Pts',(-7.18427134143612,3.79551483400074,
23.2622120059459));
#179278=CARTESIAN_POINT('Ctrl Pts',(-7.28037027605087,3.61361571040607,
23.2702547485833));
#179279=CARTESIAN_POINT('Ctrl Pts',(-7.36962193058903,3.42794214622832,
23.2782974912208));
#179280=CARTESIAN_POINT('Ctrl Pts',(-7.45173294182424,3.23903746909964,
23.2863402338582));
#179281=CARTESIAN_POINT('Ctrl Pts',(-7.53377707054975,3.05028666194177,
23.2943764253791));
#179282=CARTESIAN_POINT('Ctrl Pts',(-7.60869203270067,2.85831028048253,
23.3024126168999));
#179283=CARTESIAN_POINT('Ctrl Pts',(-7.67623115236972,2.66367469070243,
23.3104488084207));
#179284=CARTESIAN_POINT('Ctrl Pts',(-7.71452310714555,2.55332416735911,
23.3150050046488));
#179285=CARTESIAN_POINT('Ctrl Pts',(-7.75044499652292,2.44211928009065,
23.3195612008769));
#179286=CARTESIAN_POINT('Ctrl Pts',(-7.78395869918349,2.33016620263571,
23.324117397105));
#179287=CARTESIAN_POINT('Ctrl Pts',(-7.84307234227238,2.13269610121472,
23.3321539116137));
#179288=CARTESIAN_POINT('Ctrl Pts',(-7.89464404251992,1.93305348126937,
23.3401904261224));
#179289=CARTESIAN_POINT('Ctrl Pts',(-7.93853952839887,1.73184229032226,
23.348226940631));
#179290=CARTESIAN_POINT('Ctrl Pts',(-7.9824615315202,1.5305095477893,23.3562683099943));
#179291=CARTESIAN_POINT('Ctrl Pts',(-8.01869800149608,1.32760665236261,
23.3643096793576));
#179292=CARTESIAN_POINT('Ctrl Pts',(-8.04716608221183,1.1237462381692,23.3723510487209));
#179293=CARTESIAN_POINT('Ctrl Pts',(-8.07565484124043,0.919737746222929,
23.3803982590804));
#179294=CARTESIAN_POINT('Ctrl Pts',(-8.09636390961471,0.714770660353516,
23.38844546944));
#179295=CARTESIAN_POINT('Ctrl Pts',(-8.10926237207028,0.509461817435902,
23.3964926797995));
#179296=CARTESIAN_POINT('Ctrl Pts',(-8.12217984593844,0.303850363944689,
23.4045517511724));
#179297=CARTESIAN_POINT('Ctrl Pts',(-8.12726368494022,0.0978964621942852,
23.4126108225453));
#179298=CARTESIAN_POINT('Ctrl Pts',(-8.12453509800826,-0.107782205079918,
23.4206698939183));
#179299=CARTESIAN_POINT('Ctrl Pts',(-8.12180430269702,-0.313627338190728,
23.4287354878931));
#179300=CARTESIAN_POINT('Ctrl Pts',(-8.11124847955766,-0.5191964775084,
23.4368010818679));
#179301=CARTESIAN_POINT('Ctrl Pts',(-8.09294072368294,-0.723877065152807,
23.4448666758427));
#179302=CARTESIAN_POINT('Ctrl Pts',(-8.07460422044872,-0.928879048083216,
23.4529449346428));
#179303=CARTESIAN_POINT('Ctrl Pts',(-8.04849149397113,-1.13298937748313,
23.4610231934428));
#179304=CARTESIAN_POINT('Ctrl Pts',(-8.01472705075418,-1.33560393246244,
23.4691014522429));
#179305=CARTESIAN_POINT('Ctrl Pts',(-7.99566301165002,-1.45000391751123,
23.4736625889591));
#179306=CARTESIAN_POINT('Ctrl Pts',(-7.97416056690779,-1.56392728920816,
23.4782237256753));
#179307=CARTESIAN_POINT('Ctrl Pts',(-7.95024914288382,-1.67726745886728,
23.4827848623915));
#179308=CARTESIAN_POINT('Ctrl Pts',(-7.90785786651976,-1.87820214390952,
23.4908710561237));
#179309=CARTESIAN_POINT('Ctrl Pts',(-7.85780988190975,-2.07769396799896,
23.4989572498559));
#179310=CARTESIAN_POINT('Ctrl Pts',(-7.80022011101215,-2.27513818970665,
23.507043443588));
#179311=CARTESIAN_POINT('Ctrl Pts',(-7.74268170745739,-2.47240630053786,
23.5151224248191));
#179312=CARTESIAN_POINT('Ctrl Pts',(-7.67761501873223,-2.66763014792167,
23.5232014060502));
#179313=CARTESIAN_POINT('Ctrl Pts',(-7.60518575397833,-2.86021628727358,
23.5312803872813));
#179314=CARTESIAN_POINT('Ctrl Pts',(-7.53281120208989,-3.05265694759065,
23.5393532656724));
#179315=CARTESIAN_POINT('Ctrl Pts',(-7.45308527572228,-3.242463577664,23.5474261440635));
#179316=CARTESIAN_POINT('Ctrl Pts',(-7.3662233330471,-3.42905837952235,
23.5554990224546));
#179317=CARTESIAN_POINT('Ctrl Pts',(-7.27941516179569,-3.61553767086075,
23.5635669033732));
#179318=CARTESIAN_POINT('Ctrl Pts',(-7.18547991732006,-3.79880881266836,
23.5716347842919));
#179319=CARTESIAN_POINT('Ctrl Pts',(-7.08468109217274,-3.97831388715244,
23.5797026652105));
#179320=CARTESIAN_POINT('Ctrl Pts',(-6.98393093876615,-4.15773228578064,
23.5877666504706));
#179321=CARTESIAN_POINT('Ctrl Pts',(-6.87632396956717,-4.33338796830507,
23.5958306357307));
#179322=CARTESIAN_POINT('Ctrl Pts',(-6.76216993216977,-4.50474698190244,
23.6038946209907));
#179323=CARTESIAN_POINT('Ctrl Pts',(-6.64642951920311,-4.67848733705319,
23.612070669823));
#179324=CARTESIAN_POINT('Ctrl Pts',(-6.52395887079913,-4.84781042206556,
23.6202467186552));
#179325=CARTESIAN_POINT('Ctrl Pts',(-6.39512741719872,-5.01218843224127,
23.6284227674874));
#179326=CARTESIAN_POINT('Ctrl Pts',(-6.26812197128787,-5.17423661144646,
23.6364829321344));
#179327=CARTESIAN_POINT('Ctrl Pts',(-6.13493504605435,-5.33147871664951,
23.6445430967814));
#179328=CARTESIAN_POINT('Ctrl Pts',(-5.9959625525229,-5.48344058336033,
23.6526032614283));
#179329=CARTESIAN_POINT('Ctrl Pts',(-5.85699677344482,-5.63539510803646,
23.6606630366486));
#179330=CARTESIAN_POINT('Ctrl Pts',(-5.7122461974415,-5.78206966938098,
23.6687228118688));
#179331=CARTESIAN_POINT('Ctrl Pts',(-5.56214532607138,-5.92302515055966,
23.6767825870891));
#179332=CARTESIAN_POINT('Ctrl Pts',(-5.41203312189491,-6.06399127405612,
23.6848429708326));
#179333=CARTESIAN_POINT('Ctrl Pts',(-5.25657004797934,-6.19923723975241,
23.6929033545761));
#179334=CARTESIAN_POINT('Ctrl Pts',(-5.09622601367504,-6.32836218780514,
23.7009637383197));
#179335=CARTESIAN_POINT('Ctrl Pts',(-4.93185127324367,-6.46073306091851,
23.7092267428734));
#179336=CARTESIAN_POINT('Ctrl Pts',(-4.7623472301346,-6.58667091871485,
23.7174897474271));
#179337=CARTESIAN_POINT('Ctrl Pts',(-4.58825462489004,-6.70578907062213,
23.7257527519808));
#179338=CARTESIAN_POINT('Ctrl Pts',(-4.41829137045866,-6.82208182602993,
23.7338197640366));
#179339=CARTESIAN_POINT('Ctrl Pts',(-4.24395504270791,-6.93187456709233,
23.7418867760924));
#179340=CARTESIAN_POINT('Ctrl Pts',(-4.06577688249518,-7.03485223045003,
23.7499537881482));
#179341=CARTESIAN_POINT('Ctrl Pts',(-3.88110531757662,-7.14158274232207,
23.7583147889509));
#179342=CARTESIAN_POINT('Ctrl Pts',(-3.69230696823037,-7.2409919342672,
23.7666757897536));
#179343=CARTESIAN_POINT('Ctrl Pts',(-3.49999990501188,-7.3327817523377,
23.7750367905563));
#179344=CARTESIAN_POINT('Ctrl Pts',(-3.30769284179336,-7.42457157040823,
23.783397791359));
#179345=CARTESIAN_POINT('Ctrl Pts',(-3.11187742065025,-7.50874188779212,
23.7917587921616));
#179346=CARTESIAN_POINT('Ctrl Pts',(-2.91319360868107,-7.5850504652797,
23.8001197929643));
#179347=CARTESIAN_POINT('Ctrl Pts',(-2.73311055328088,-7.65421504215694,
23.8076980377938));
#179348=CARTESIAN_POINT('Ctrl Pts',(-2.55031007436823,-7.71705940980132,
23.8152762826232));
#179349=CARTESIAN_POINT('Ctrl Pts',(-2.36529515513901,-7.77335618581677,
23.8228545274527));
#179350=CARTESIAN_POINT('Ctrl Pts',(-2.18041791037555,-7.82961106992106,
23.8304271331109));
#179351=CARTESIAN_POINT('Ctrl Pts',(-1.99332985263676,-7.87932794874501,
23.8379997387692));
#179352=CARTESIAN_POINT('Ctrl Pts',(-1.80455404516674,-7.92232745224359,
23.8455723444274));
#179353=CARTESIAN_POINT('Ctrl Pts',(-1.61588286271852,-7.96530312417152,
23.8531407531282));
#179354=CARTESIAN_POINT('Ctrl Pts',(-1.42552614896208,-8.00156874760897,
23.8607091618289));
#179355=CARTESIAN_POINT('Ctrl Pts',(-1.23402217667708,-8.03099475967761,
23.8682775705297));
#179356=CARTESIAN_POINT('Ctrl Pts',(-1.04256447328066,-8.0604136621868,
23.8758441506425));
#179357=CARTESIAN_POINT('Ctrl Pts',(-0.84996042466078,-8.08299617879292,
23.8834107307554));
#179358=CARTESIAN_POINT('Ctrl Pts',(-0.656758684149105,-8.09866381530279,
23.8909773108682));
#179359=CARTESIAN_POINT('Ctrl Pts',(-0.463591216752003,-8.11432867244483,
23.8985425487039));
#179360=CARTESIAN_POINT('Ctrl Pts',(-0.269826635269474,-8.12308106450025,
23.9061077865396));
#179361=CARTESIAN_POINT('Ctrl Pts',(-0.0760186299643247,-8.12489438272267,
23.9136730243754));
#179362=CARTESIAN_POINT('Ctrl Pts',(0.117856771684291,-8.12670833152284,
23.9212408930073));
#179363=CARTESIAN_POINT('Ctrl Pts',(0.311775259201533,-8.12157837899451,
23.9288087616393));
#179364=CARTESIAN_POINT('Ctrl Pts',(0.505182741367443,-8.10953007025219,
23.9363766302713));
#179365=CARTESIAN_POINT('Ctrl Pts',(0.696094403204386,-8.09763723850358,
23.9438468395978));
#179366=CARTESIAN_POINT('Ctrl Pts',(0.88650782579579,-8.07900360419725,
23.9513170489243));
#179367=CARTESIAN_POINT('Ctrl Pts',(1.07589550392165,-8.0537032740933,23.9587872582508));
#179368=CARTESIAN_POINT('Ctrl Pts',(1.31182084776506,-8.02218596980935,
23.968093099694));
#179369=CARTESIAN_POINT('Ctrl Pts',(1.5460388441147,-7.98034070549909,23.9773989411372));
#179370=CARTESIAN_POINT('Ctrl Pts',(1.77774361147715,-7.9283866715967,23.9867047825804));
#179371=CARTESIAN_POINT('Ctrl Pts',(2.01069235499054,-7.8761537069677,23.9960605852089));
#179372=CARTESIAN_POINT('Ctrl Pts',(2.24110077828056,-7.81370319993051,
24.0054163878374));
#179373=CARTESIAN_POINT('Ctrl Pts',(2.46817220066963,-7.74130567477745,
24.0147721904659));
#179374=CARTESIAN_POINT('Ctrl Pts',(2.69634593110011,-7.66855669908379,
24.0241734104189));
#179375=CARTESIAN_POINT('Ctrl Pts',(2.92115015044056,-7.58576393175628,
24.0335746303719));
#179376=CARTESIAN_POINT('Ctrl Pts',(3.14179941299455,-7.49324922920672,
24.0429758503249));
#179377=CARTESIAN_POINT('Ctrl Pts',(3.36268748352705,-7.40063439829578,
24.0523872451877));
#179378=CARTESIAN_POINT('Ctrl Pts',(3.57941157252882,-7.29827661029634,
24.0617986400504));
#179379=CARTESIAN_POINT('Ctrl Pts',(3.79120698546053,-7.186545564866,24.0712100349132));
#179380=CARTESIAN_POINT('Ctrl Pts',(4.00275395882051,-7.07494558182599,
24.0806103900519));
#179381=CARTESIAN_POINT('Ctrl Pts',(4.2093837819533,-6.95399433920389,24.0900107451906));
#179382=CARTESIAN_POINT('Ctrl Pts',(4.4103580886906,-6.82410646839727,24.0994111003293));
#179383=CARTESIAN_POINT('Ctrl Pts',(4.53894559457774,-6.74100153014341,
24.1054256413986));
#179384=CARTESIAN_POINT('Ctrl Pts',(4.6652183752779,-6.65423912874416,24.1114401824679));
#179385=CARTESIAN_POINT('Ctrl Pts',(4.7889882302884,-6.56393778860367,24.1174547235371));
#179386=CARTESIAN_POINT('Ctrl Pts',(4.94831263328778,-6.44769617947591,
24.1251970220564));
#179387=CARTESIAN_POINT('Ctrl Pts',(5.10356257850886,-6.32553324874517,
24.1329393205757));
#179388=CARTESIAN_POINT('Ctrl Pts',(5.25426566110439,-6.1977721743413,24.140681619095));
#179389=CARTESIAN_POINT('Ctrl Pts',(5.40487486932615,-6.07009068351757,
24.1484190948633));
#179390=CARTESIAN_POINT('Ctrl Pts',(5.55094258597142,-5.93681821978935,
24.1561565706317));
#179391=CARTESIAN_POINT('Ctrl Pts',(5.69202712464408,-5.79831999589674,
24.1638940464001));
#179392=CARTESIAN_POINT('Ctrl Pts',(5.83304885520387,-5.6598834287396,24.1716280775937));
#179393=CARTESIAN_POINT('Ctrl Pts',(5.96909157444715,-5.51622598168545,
24.1793621087872));
#179394=CARTESIAN_POINT('Ctrl Pts',(6.09974821376229,-5.36775179113228,
24.1870961399808));
#179395=CARTESIAN_POINT('Ctrl Pts',(6.23038813314207,-5.21929660059993,
24.1948291814619));
#179396=CARTESIAN_POINT('Ctrl Pts',(6.3556431064549,-5.06602615429118,24.202562222943));
#179397=CARTESIAN_POINT('Ctrl Pts',(6.47514410617666,-4.90838021823347,
24.2102952644241));
#179398=CARTESIAN_POINT('Ctrl Pts',(6.5946331678376,-4.75075003088729,24.2180275333802));
#179399=CARTESIAN_POINT('Ctrl Pts',(6.70836919027415,-4.58874550826861,
24.2257598023362));
#179400=CARTESIAN_POINT('Ctrl Pts',(6.816024587135,-4.42283804700909,24.2334920712922));
#179401=CARTESIAN_POINT('Ctrl Pts',(6.92372139413071,-4.2568667686949,24.2412273145005));
#179402=CARTESIAN_POINT('Ctrl Pts',(7.0253327099813,-4.0869898489721,24.2489625577087));
#179403=CARTESIAN_POINT('Ctrl Pts',(7.12057495808006,-3.91370666106481,
24.2566978009169));
#179404=CARTESIAN_POINT('Ctrl Pts',(7.20029761287676,-3.76865973023976,
24.2631725968858));
#179405=CARTESIAN_POINT('Ctrl Pts',(7.27555848415153,-3.62122675606321,
24.2696473928547));
#179406=CARTESIAN_POINT('Ctrl Pts',(7.34621646707183,-3.47171300389629,
24.2761221888236));
#179407=CARTESIAN_POINT('Ctrl Pts',(7.43804233416082,-3.27740757134609,
24.2845367193479));
#179408=CARTESIAN_POINT('Ctrl Pts',(7.5221378580496,-3.07949401598327,24.2929512498722));
#179409=CARTESIAN_POINT('Ctrl Pts',(7.59824883961314,-2.87859377714494,
24.3013657803965));
#179410=CARTESIAN_POINT('Ctrl Pts',(7.67438162949918,-2.67763597371988,
24.309782721963));
#179411=CARTESIAN_POINT('Ctrl Pts',(7.74252521601516,-2.47369002499559,
24.3181996635296));
#179412=CARTESIAN_POINT('Ctrl Pts',(7.80247441353559,-2.26739511083146,
24.3266166050962));
#179413=CARTESIAN_POINT('Ctrl Pts',(7.86245134216148,-2.06100476943464,
24.3350374401443));
#179414=CARTESIAN_POINT('Ctrl Pts',(7.91422623132519,-1.85226354414678,
24.3434582751925));
#179415=CARTESIAN_POINT('Ctrl Pts',(7.95764402696705,-1.64182493055002,
24.3518791102406));
#179416=CARTESIAN_POINT('Ctrl Pts',(8.00106769685982,-1.43135784546596,
24.3603010845934));
#179417=CARTESIAN_POINT('Ctrl Pts',(8.03613196578301,-1.21919317265353,
24.3687230589462));
#179418=CARTESIAN_POINT('Ctrl Pts',(8.06273298342256,-1.00599423483932,
24.3771450332991));
#179419=CARTESIAN_POINT('Ctrl Pts',(8.08934101921505,-0.792739048697539,
24.3855692296234));
#179420=CARTESIAN_POINT('Ctrl Pts',(8.10748130955641,-0.578449314158817,
24.3939934259478));
#179421=CARTESIAN_POINT('Ctrl Pts',(8.11710176759307,-0.363794525848674,
24.4024176222721));
#179422=CARTESIAN_POINT('Ctrl Pts',(8.12253958060108,-0.242464273624073,
24.4071792671106));
#179423=CARTESIAN_POINT('Ctrl Pts',(8.12525633609621,-0.121017470923162,
24.4119409119492));
#179424=CARTESIAN_POINT('Ctrl Pts',(8.12524998890234,0.000424667562427413,
24.4167025567877));
#179425=CARTESIAN_POINT('',(8.12179382505447,-0.00475747993537114,20.4167025567876));
#179426=CARTESIAN_POINT('Ctrl Pts',(8.12525,8.44118043087094E-13,20.4167025567876));
#179427=CARTESIAN_POINT('Ctrl Pts',(8.12524999999977,2.24624642433502,20.5047001499288));
#179428=CARTESIAN_POINT('Ctrl Pts',(7.14398562317547,4.47535249753539,20.5926977430701));
#179429=CARTESIAN_POINT('Ctrl Pts',(3.83078204044833,7.50935546634414,20.7686929293525));
#179430=CARTESIAN_POINT('Ctrl Pts',(1.52412477697628,8.2911009055216,20.8566905224937));
#179431=CARTESIAN_POINT('Ctrl Pts',(-2.95101623932681,7.89663306204382,
21.0326857087761));
#179432=CARTESIAN_POINT('Ctrl Pts',(-5.08535169588843,6.72342983085707,
21.1206833019173));
#179433=CARTESIAN_POINT('Ctrl Pts',(-7.8167169468446,3.15661951052808,21.2966784881997));
#179434=CARTESIAN_POINT('Ctrl Pts',(-8.39290461146718,0.790229551552612,
21.3846760813409));
#179435=CARTESIAN_POINT('Ctrl Pts',(-7.60701611462415,-3.63299000730563,
21.5606712676233));
#179436=CARTESIAN_POINT('Ctrl Pts',(-6.25093680401244,-5.65606750610146,
21.6486688607645));
#179437=CARTESIAN_POINT('Ctrl Pts',(-2.45807268688382,-8.06369575488373,
21.8246640470469));
#179438=CARTESIAN_POINT('Ctrl Pts',(-0.0502299510434481,-8.42987470330089,
21.9126616401881));
#179439=CARTESIAN_POINT('Ctrl Pts',(4.28689960881172,-7.2586363943446,22.0886568264705));
#179440=CARTESIAN_POINT('Ctrl Pts',(6.18309125557306,-5.73015646266226,
22.1766544196117));
#179441=CARTESIAN_POINT('Ctrl Pts',(7.81050559202949,-2.58640713800104,
22.3153355274312));
#179442=CARTESIAN_POINT('Ctrl Pts',(8.12525000000014,-1.2937588353802,22.3660190421094));
#179443=CARTESIAN_POINT('Ctrl Pts',(8.12525,8.99861304443488E-13,22.4167025567876));
#179444=CARTESIAN_POINT('',(8.13495457859621,0.00273215638295254,18.4167025567877));
#179445=CARTESIAN_POINT('Ctrl Pts',(8.13495457859621,0.00273215638295254,
18.4167025567877));
#179446=CARTESIAN_POINT('Ctrl Pts',(8.12219365949143,2.60157214278194,18.5187220057913));
#179447=CARTESIAN_POINT('Ctrl Pts',(6.08468278693466,6.5155798553575,18.6736306098904));
#179448=CARTESIAN_POINT('Ctrl Pts',(0.934776268559737,8.40074683640842,
18.881428369085));
#179449=CARTESIAN_POINT('Ctrl Pts',(-4.60194067302227,7.68097745167893,
19.0929849894669));
#179450=CARTESIAN_POINT('Ctrl Pts',(-8.4515383039797,2.98387753236073,19.3045416098488));
#179451=CARTESIAN_POINT('Ctrl Pts',(-8.04309746149275,-2.61270635975162,
19.5160982302307));
#179452=CARTESIAN_POINT('Ctrl Pts',(-5.84417858547815,-6.13212745071067,
19.6747656955172));
#179453=CARTESIAN_POINT('Ctrl Pts',(-2.18625041274964,-8.18579265278837,
19.8334331608036));
#179454=CARTESIAN_POINT('Ctrl Pts',(1.98642421298176,-8.22870475927635,
19.99210062609));
#179455=CARTESIAN_POINT('Ctrl Pts',(5.67997759279721,-6.28687098380536,
20.1507680913764));
#179456=CARTESIAN_POINT('Ctrl Pts',(7.7478105945485,-3.16811172828057,20.2923020682757));
#179457=CARTESIAN_POINT('Ctrl Pts',(8.12198112487852,-0.915751868132923,
20.3809468900794));
#179458=CARTESIAN_POINT('Ctrl Pts',(8.12170811034813,-0.00487546759574239,
20.4167025567876));
#179459=CARTESIAN_POINT('',(8.11704416097361,0.0053549714669613,16.4167025567876));
#179460=CARTESIAN_POINT('Ctrl Pts',(8.11704416097361,0.0053549714669613,
16.4167025567876));
#179461=CARTESIAN_POINT('Ctrl Pts',(8.12312230185039,0.724943922503215,
16.4449405011213));
#179462=CARTESIAN_POINT('Ctrl Pts',(7.87111371571117,2.78990206214897,16.5260676005504));
#179463=CARTESIAN_POINT('Ctrl Pts',(6.09986490165294,5.85132482975188,16.660083855075));
#179464=CARTESIAN_POINT('Ctrl Pts',(1.38755966192534,8.84590022303072,16.8716404754569));
#179465=CARTESIAN_POINT('Ctrl Pts',(-4.5775196263014,7.70573415727464,17.0831970958388));
#179466=CARTESIAN_POINT('Ctrl Pts',(-7.84949254946182,3.14692199034251,
17.2947537162207));
#179467=CARTESIAN_POINT('Ctrl Pts',(-8.41592959045643,-0.964126308737623,
17.4534211815072));
#179468=CARTESIAN_POINT('Ctrl Pts',(-6.9230488953515,-4.88449446864917,
17.6120886467936));
#179469=CARTESIAN_POINT('Ctrl Pts',(-3.74670372206902,-7.5907624378775,
17.77075611208));
#179470=CARTESIAN_POINT('Ctrl Pts',(0.333338327069147,-8.46615484038642,
17.9294235773664));
#179471=CARTESIAN_POINT('Ctrl Pts',(4.35323706612459,-7.26682444103609,
18.0880910426529));
#179472=CARTESIAN_POINT('Ctrl Pts',(7.27202321558427,-4.31686572056175,
18.2467585079393));
#179473=CARTESIAN_POINT('Ctrl Pts',(8.11531900160381,-1.53650348273241,
18.3562956793176));
#179474=CARTESIAN_POINT('Ctrl Pts',(8.13542474898045,-0.0930209461116091,
18.4129436956003));
#179475=CARTESIAN_POINT('Ctrl Pts',(8.13495457859621,0.00273215638295254,
18.4167025567877));
#179476=CARTESIAN_POINT('',(8.12115743020385,-0.00265292485854291,14.4167025567876));
#179477=CARTESIAN_POINT('Ctrl Pts',(8.12115743020385,-0.00265292485854291,
14.4167025567876));
#179478=CARTESIAN_POINT('Ctrl Pts',(8.1208903862547,0.185607932901776,14.4240481515468));
#179479=CARTESIAN_POINT('Ctrl Pts',(8.06645284195536,1.72963063830796,14.4842829014014));
#179480=CARTESIAN_POINT('Ctrl Pts',(6.7327160091308,5.90303377185082,14.6502959614469));
#179481=CARTESIAN_POINT('Ctrl Pts',(1.4221714321135,8.84926286475003,14.8618525818288));
#179482=CARTESIAN_POINT('Ctrl Pts',(-4.01080233417677,7.44520758162725,
15.0734092022108));
#179483=CARTESIAN_POINT('Ctrl Pts',(-7.07955773652492,4.65158818748291,
15.2320766674971));
#179484=CARTESIAN_POINT('Ctrl Pts',(-8.44497665565605,0.685026647011867,
15.3907441327836));
#179485=CARTESIAN_POINT('Ctrl Pts',(-7.73996699874801,-3.42788185729165,
15.54941159807));
#179486=CARTESIAN_POINT('Ctrl Pts',(-5.16809395608709,-6.71399263350416,
15.7080790633565));
#179487=CARTESIAN_POINT('Ctrl Pts',(-1.31318116064738,-8.36857010785243,
15.8667465286429));
#179488=CARTESIAN_POINT('Ctrl Pts',(2.81786210763198,-7.97353776185511,
16.0254139939293));
#179489=CARTESIAN_POINT('Ctrl Pts',(6.88263605041008,-5.30498188964788,
16.2087326699775));
#179490=CARTESIAN_POINT('Ctrl Pts',(8.10035380767631,-1.97061005881078,
16.3391621909303));
#179491=CARTESIAN_POINT('Ctrl Pts',(8.11704416097361,0.0053549714669613,
16.4167025567876));
#179492=CARTESIAN_POINT('',(8.12771990326935,-0.00255226564017053,12.4167025567876));
#179493=CARTESIAN_POINT('Ctrl Pts',(8.12771990326935,-0.00255226564017053,
12.4167025567876));
#179494=CARTESIAN_POINT('Ctrl Pts',(8.10769023119547,2.34268520044713,12.5089341121632));
#179495=CARTESIAN_POINT('Ctrl Pts',(6.43672742380787,6.03729498712112,12.6540548226342));
#179496=CARTESIAN_POINT('Ctrl Pts',(1.69039256538473,8.28614652732196,12.8520646882007));
#179497=CARTESIAN_POINT('Ctrl Pts',(-2.45563682176706,8.10723493000556,
13.0107321534872));
#179498=CARTESIAN_POINT('Ctrl Pts',(-6.04529291051789,5.93644050317478,
13.1693996187736));
#179499=CARTESIAN_POINT('Ctrl Pts',(-8.13900558166093,2.32681140425045,
13.32806708406));
#179500=CARTESIAN_POINT('Ctrl Pts',(-8.26960761947707,-1.84403959870139,
13.4867345493464));
#179501=CARTESIAN_POINT('Ctrl Pts',(-6.36979470017056,-5.58418533793423,
13.6454020146329));
#179502=CARTESIAN_POINT('Ctrl Pts',(-2.94483553187357,-7.92752136468722,
13.8040694799193));
#179503=CARTESIAN_POINT('Ctrl Pts',(2.62992883968321,-8.56828449165679,
14.0156261003012));
#179504=CARTESIAN_POINT('Ctrl Pts',(7.31450585013114,-5.04406336557082,
14.219837125924));
#179505=CARTESIAN_POINT('Ctrl Pts',(8.12281313441969,-1.16989261279938,
14.3711589964513));
#179506=CARTESIAN_POINT('Ctrl Pts',(8.12115743020385,-0.00265292485854291,
14.4167025567876));
#179507=CARTESIAN_POINT('',(8.12607929659709,0.000602397285608403,10.4167025567876));
#179508=CARTESIAN_POINT('Ctrl Pts',(8.12607929659709,0.000602397285608403,
10.4167025567876));
#179509=CARTESIAN_POINT('Ctrl Pts',(8.13073112681322,0.470635535523587,
10.4351526074932));
#179510=CARTESIAN_POINT('Ctrl Pts',(7.98907354300784,2.28814380995213,10.5064918132942));
#179511=CARTESIAN_POINT('Ctrl Pts',(6.60661632725948,5.27923024708584,10.6307201741907));
#179512=CARTESIAN_POINT('Ctrl Pts',(3.30861330952928,7.79810799993987,10.7893876394771));
#179513=CARTESIAN_POINT('Ctrl Pts',(-0.838343829035709,8.43113704348409,
10.9480551047636));
#179514=CARTESIAN_POINT('Ctrl Pts',(-4.75851708790317,7.00099837833084,
11.10672257005));
#179515=CARTESIAN_POINT('Ctrl Pts',(-7.53094626422831,3.88223396860591,
11.2653900353364));
#179516=CARTESIAN_POINT('Ctrl Pts',(-8.46845332731798,-0.206660721371117,
11.4240575006229));
#179517=CARTESIAN_POINT('Ctrl Pts',(-7.3400337247469,-4.20018525983505,
11.5827249659093));
#179518=CARTESIAN_POINT('Ctrl Pts',(-3.47017141527117,-8.26377245453908,
11.7942815862912));
#179519=CARTESIAN_POINT('Ctrl Pts',(2.5951842104773,-8.56973112092244,12.0058382066731));
#179520=CARTESIAN_POINT('Ctrl Pts',(6.84908166713351,-4.95342653106151,
12.217394827055));
#179521=CARTESIAN_POINT('Ctrl Pts',(8.03485269117871,-2.03602439612437,
12.3367198920614));
#179522=CARTESIAN_POINT('Ctrl Pts',(8.13066181458715,-0.347015251302779,
12.4031558019722));
#179523=CARTESIAN_POINT('Ctrl Pts',(8.12771990326935,-0.00255226564017053,
12.4167025567876));
#179524=CARTESIAN_POINT('',(8.12524838875447,0.00511698572321418,8.41670255678763));
#179525=CARTESIAN_POINT('Ctrl Pts',(8.12524838875447,0.00511698572321418,
8.41670255678763));
#179526=CARTESIAN_POINT('Ctrl Pts',(8.125098058661,0.2438257521285,8.42604123424159));
#179527=CARTESIAN_POINT('Ctrl Pts',(8.11442430814408,0.48221832798838,8.43537991169555));
#179528=CARTESIAN_POINT('Ctrl Pts',(8.09333451737573,0.719460876180585,
8.4447185891495));
#179529=CARTESIAN_POINT('Ctrl Pts',(8.072136057386,0.957925862436575,8.45410538594323));
#179530=CARTESIAN_POINT('Ctrl Pts',(8.04041399138175,1.19522890544064,8.46349218273696));
#179531=CARTESIAN_POINT('Ctrl Pts',(7.99832782015985,1.43053823568509,8.47287897953069));
#179532=CARTESIAN_POINT('Ctrl Pts',(7.95606163645599,1.66685403944175,8.48230592586855));
#179533=CARTESIAN_POINT('Ctrl Pts',(7.90334252502713,1.90115900887101,8.4917328722064));
#179534=CARTESIAN_POINT('Ctrl Pts',(7.84038219011455,2.13262623903827,8.50115981854426));
#179535=CARTESIAN_POINT('Ctrl Pts',(7.77737494260372,2.36426593857363,8.5105937890275));
#179536=CARTESIAN_POINT('Ctrl Pts',(7.70411122610931,2.5930636433074,8.52002775951075));
#179537=CARTESIAN_POINT('Ctrl Pts',(7.62085292578376,2.8182065655436,8.529461729994));
#179538=CARTESIAN_POINT('Ctrl Pts',(7.5377264010515,3.04299314682599,8.53888076902834));
#179539=CARTESIAN_POINT('Ctrl Pts',(7.44463691312889,3.26413647656692,8.54829980806267));
#179540=CARTESIAN_POINT('Ctrl Pts',(7.34189438505438,3.48084392083399,8.55771884709701));
#179541=CARTESIAN_POINT('Ctrl Pts',(7.30435543667455,3.56002213180782,8.56116027322039));
#179542=CARTESIAN_POINT('Ctrl Pts',(7.26552833483325,3.6386083356071,8.56460169934378));
#179543=CARTESIAN_POINT('Ctrl Pts',(7.22542984209052,3.7165644296215,8.56804312546716));
#179544=CARTESIAN_POINT('Ctrl Pts',(7.13521883948435,3.89194502174051,8.57578542398638));
#179545=CARTESIAN_POINT('Ctrl Pts',(7.03852776872942,4.06421563435813,8.58352772250561));
#179546=CARTESIAN_POINT('Ctrl Pts',(6.93560288403208,4.23285957687069,8.59127002102483));
#179547=CARTESIAN_POINT('Ctrl Pts',(6.83274211221766,4.40139846947843,8.59900749679318));
#179548=CARTESIAN_POINT('Ctrl Pts',(6.72365544141641,4.5663148897864,8.60674497256152));
#179549=CARTESIAN_POINT('Ctrl Pts',(6.60863540454276,4.72711599734172,8.61448244832986));
#179550=CARTESIAN_POINT('Ctrl Pts',(6.49366657236876,4.88784551934864,8.62221647952338));
#179551=CARTESIAN_POINT('Ctrl Pts',(6.37276983990874,5.04446309062786,8.6299505107169));
#179552=CARTESIAN_POINT('Ctrl Pts',(6.24628154791172,5.19650405433476,8.63768454191043));
#179553=CARTESIAN_POINT('Ctrl Pts',(6.11980944243305,5.34852556158596,8.6454175833915));
#179554=CARTESIAN_POINT('Ctrl Pts',(5.9877474225559,5.49597135147781,8.65315062487257));
#179555=CARTESIAN_POINT('Ctrl Pts',(5.85047291171498,5.63840884219912,8.66088366635364));
#179556=CARTESIAN_POINT('Ctrl Pts',(5.71321211449538,5.78083210352127,8.66861593530963));
#179557=CARTESIAN_POINT('Ctrl Pts',(5.57074011136782,5.91824781031278,8.67634820426562));
#179558=CARTESIAN_POINT('Ctrl Pts',(5.42347198319433,6.05025943328104,8.68408047322161));
#179559=CARTESIAN_POINT('Ctrl Pts',(5.27614720766975,6.1823218351167,8.6918157164298));
#179560=CARTESIAN_POINT('Ctrl Pts',(5.12402288457192,6.30897576393484,8.69955095963798));
#179561=CARTESIAN_POINT('Ctrl Pts',(4.96754853923773,6.42986384558935,8.70728620284617));
#179562=CARTESIAN_POINT('Ctrl Pts',(4.83657147320705,6.53105338064936,8.7137609988153));
#179563=CARTESIAN_POINT('Ctrl Pts',(4.70254722464643,6.62820368388824,8.72023579478444));
#179564=CARTESIAN_POINT('Ctrl Pts',(4.56575557235517,6.72112815054197,8.72671059075357));
#179565=CARTESIAN_POINT('Ctrl Pts',(4.38799319042858,6.84188460208664,8.73512466525799));
#179566=CARTESIAN_POINT('Ctrl Pts',(4.2054713374984,6.95556232257409,8.74353873976241));
#179567=CARTESIAN_POINT('Ctrl Pts',(4.01876463813715,7.06181409736608,8.75195281426683));
#179568=CARTESIAN_POINT('Ctrl Pts',(3.83200579673226,7.16809554535512,8.76036923859074));
#179569=CARTESIAN_POINT('Ctrl Pts',(3.64106000524196,7.26694677693808,8.76878566291464));
#179570=CARTESIAN_POINT('Ctrl Pts',(3.4465269865376,7.3580662740674,8.77720208723855));
#179571=CARTESIAN_POINT('Ctrl Pts',(3.25194572499939,7.44920836819741,8.78562059877707));
#179572=CARTESIAN_POINT('Ctrl Pts',(3.05377569925666,7.53261478798179,8.7940391103156));
#179573=CARTESIAN_POINT('Ctrl Pts',(2.85263812737841,7.60803149814241,8.80245762185412));
#179574=CARTESIAN_POINT('Ctrl Pts',(2.65142329939928,7.68347717554625,8.81087936690775));
#179575=CARTESIAN_POINT('Ctrl Pts',(2.44723889432485,7.75092691688914,8.81930111196138));
#179576=CARTESIAN_POINT('Ctrl Pts',(2.24072421999721,7.81017557628623,8.827722857015));
#179577=CARTESIAN_POINT('Ctrl Pts',(2.03418716004291,7.86943065807617,8.83614551496279));
#179578=CARTESIAN_POINT('Ctrl Pts',(1.82531958104599,7.92048281310389,8.84456817291058));
#179579=CARTESIAN_POINT('Ctrl Pts',(1.61477458531803,7.96317716750739,8.85299083085837));
#179580=CARTESIAN_POINT('Ctrl Pts',(1.40418954999055,8.00587964114851,8.86141509055333));
#179581=CARTESIAN_POINT('Ctrl Pts',(1.19192671933118,8.04022108650938,8.86983935024829));
#179582=CARTESIAN_POINT('Ctrl Pts',(0.978649295929383,8.06609776273986,
8.87826360994325));
#179583=CARTESIAN_POINT('Ctrl Pts',(0.918610361257806,8.07338220967727,
8.8806350919755));
#179584=CARTESIAN_POINT('Ctrl Pts',(0.858491070339641,8.0799961730106,8.88300657400776));
#179585=CARTESIAN_POINT('Ctrl Pts',(0.7983063132151,8.08593807747629,8.88537805604001));
#179586=CARTESIAN_POINT('Ctrl Pts',(0.584509219070929,8.10704577931211,
8.89380238126012));
#179587=CARTESIAN_POINT('Ctrl Pts',(0.369863588301559,8.11967085437079,
8.90222670648022));
#179588=CARTESIAN_POINT('Ctrl Pts',(0.15503927395233,8.123770699991,8.91065103170033));
#179589=CARTESIAN_POINT('Ctrl Pts',(-0.0597479161277014,8.12786983710775,
8.919073901094));
#179590=CARTESIAN_POINT('Ctrl Pts',(-0.274713464367256,8.12344668231059,
8.92749677048766));
#179591=CARTESIAN_POINT('Ctrl Pts',(-0.489186275147421,8.11051073303694,
8.93591963988132));
#179592=CARTESIAN_POINT('Ctrl Pts',(-0.703615258049017,8.09757742724622,
8.9443407880475));
#179593=CARTESIAN_POINT('Ctrl Pts',(-0.917551441270378,8.07613481673323,
8.95276193621368));
#179594=CARTESIAN_POINT('Ctrl Pts',(-1.13032650600636,8.04624443776843,
8.96118308437986));
#179595=CARTESIAN_POINT('Ctrl Pts',(-1.34304187323866,8.01636244503541,
8.96960186985601));
#179596=CARTESIAN_POINT('Ctrl Pts',(-1.5545965114634,7.97803745437985,8.97802065533217));
#179597=CARTESIAN_POINT('Ctrl Pts',(-1.76432897031372,7.93138265670064,
8.98643944080832));
#179598=CARTESIAN_POINT('Ctrl Pts',(-1.97400284180562,7.88474089172686,
8.99485587455311));
#179599=CARTESIAN_POINT('Ctrl Pts',(-2.18185529279267,7.82977402285051,
9.00327230829789));
#179600=CARTESIAN_POINT('Ctrl Pts',(-2.38723563783614,7.76664622420418,
9.01168874204267));
#179601=CARTESIAN_POINT('Ctrl Pts',(-2.59254144175425,7.70354133727879,
9.0201021211113));
#179602=CARTESIAN_POINT('Ctrl Pts',(-2.79537667941255,7.63228151299868,
9.02851550017993));
#179603=CARTESIAN_POINT('Ctrl Pts',(-2.99510542884134,7.55308089673513,
9.03692887924856));
#179604=CARTESIAN_POINT('Ctrl Pts',(-3.05142041678122,7.53074970123889,
9.03930109327452));
#179605=CARTESIAN_POINT('Ctrl Pts',(-3.10748853771055,7.50778751544481,
9.04167330730049));
#179606=CARTESIAN_POINT('Ctrl Pts',(-3.16329578184452,7.48419984761662,
9.04404552132645));
#179607=CARTESIAN_POINT('Ctrl Pts',(-3.34526897145014,7.40728647881186,
9.05178070623714));
#179608=CARTESIAN_POINT('Ctrl Pts',(-3.52454764430374,7.32368480952295,
9.05951589114782));
#179609=CARTESIAN_POINT('Ctrl Pts',(-3.70060333951096,7.23361752417837,
9.0672510760585));
#179610=CARTESIAN_POINT('Ctrl Pts',(-3.87660459394719,7.14357808986381,
9.07498386905889));
#179611=CARTESIAN_POINT('Ctrl Pts',(-4.0493845412807,7.04707718170321,9.08271666205927));
#179612=CARTESIAN_POINT('Ctrl Pts',(-4.2184367754129,6.94438469083792,9.09044945505966));
#179613=CARTESIAN_POINT('Ctrl Pts',(-4.38746677010459,6.84170570954588,
9.09818123078281));
#179614=CARTESIAN_POINT('Ctrl Pts',(-4.55276972691651,6.73283695199524,
9.10591300650596));
#179615=CARTESIAN_POINT('Ctrl Pts',(-4.71386571423205,6.61809319900283,
9.11364478222911));
#179616=CARTESIAN_POINT('Ctrl Pts',(-4.87501934609027,6.50330838756275,
9.12137932459271));
#179617=CARTESIAN_POINT('Ctrl Pts',(-5.03196271033564,6.38264458232978,
9.12911386695631));
#179618=CARTESIAN_POINT('Ctrl Pts',(-5.184246105036,6.25645905324402,9.13684840931992));
#179619=CARTESIAN_POINT('Ctrl Pts',(-5.33655521870373,6.1302522128294,9.14458425796148));
#179620=CARTESIAN_POINT('Ctrl Pts',(-5.48420252739657,5.99852202175738,
9.15232010660305));
#179621=CARTESIAN_POINT('Ctrl Pts',(-5.62677296530292,5.86166474300912,
9.16005595524462));
#179622=CARTESIAN_POINT('Ctrl Pts',(-5.76946006079732,5.72469548143833,
9.16779813370783));
#179623=CARTESIAN_POINT('Ctrl Pts',(-5.90706173597879,5.5825910006595,9.17554031217104));
#179624=CARTESIAN_POINT('Ctrl Pts',(-6.03920057871778,5.43578365394677,
9.18328249063426));
#179625=CARTESIAN_POINT('Ctrl Pts',(-6.14974324939096,5.31296983294089,
9.18975932262712));
#179626=CARTESIAN_POINT('Ctrl Pts',(-6.25646343178564,5.18686545947815,
9.19623615461998));
#179627=CARTESIAN_POINT('Ctrl Pts',(-6.35916264071861,5.0577404116254,9.20271298661285));
#179628=CARTESIAN_POINT('Ctrl Pts',(-6.50818149601939,4.87037707142447,
9.21211101508435));
#179629=CARTESIAN_POINT('Ctrl Pts',(-6.6488191110939,4.6765474368328,9.22150904355584));
#179630=CARTESIAN_POINT('Ctrl Pts',(-6.78060197585802,4.47695481409968,
9.23090707202734));
#179631=CARTESIAN_POINT('Ctrl Pts',(-6.91257235660879,4.27707818776984,
9.24031847310676));
#179632=CARTESIAN_POINT('Ctrl Pts',(-7.0356627634241,4.07142220134046,9.24972987418617));
#179633=CARTESIAN_POINT('Ctrl Pts',(-7.14944298160735,3.86071918368138,
9.25914127526559));
#179634=CARTESIAN_POINT('Ctrl Pts',(-7.26305188446895,3.65033341497663,
9.26853850589229));
#179635=CARTESIAN_POINT('Ctrl Pts',(-7.3673786016306,3.43491583680912,9.27793573651898));
#179636=CARTESIAN_POINT('Ctrl Pts',(-7.46204011350519,3.21522081775722,
9.28733296714567));
#179637=CARTESIAN_POINT('Ctrl Pts',(-7.55646285373454,2.99607995149786,
9.2967064944512));
#179638=CARTESIAN_POINT('Ctrl Pts',(-7.64126905143205,2.77268322230516,
9.30608002175674));
#179639=CARTESIAN_POINT('Ctrl Pts',(-7.71612397236401,2.54580407840224,
9.31545354906227));
#179640=CARTESIAN_POINT('Ctrl Pts',(-7.79049278983644,2.32039827433284,
9.32476620523208));
#179641=CARTESIAN_POINT('Ctrl Pts',(-7.8550391226782,2.09155517351854,9.3340788614019));
#179642=CARTESIAN_POINT('Ctrl Pts',(-7.90948004424336,1.86005725509084,
9.34339151757171));
#179643=CARTESIAN_POINT('Ctrl Pts',(-7.94453392306917,1.710998426774,9.34938782901424));
#179644=CARTESIAN_POINT('Ctrl Pts',(-7.97539909056265,1.56083941500507,
9.35538414045678));
#179645=CARTESIAN_POINT('Ctrl Pts',(-8.00201021731963,1.40979432698968,
9.36138045189931));
#179646=CARTESIAN_POINT('Ctrl Pts',(-8.03559484912476,1.2191675371774,9.36894811011331));
#179647=CARTESIAN_POINT('Ctrl Pts',(-8.06238728747812,1.02720451234722,
9.37651576832731));
#179648=CARTESIAN_POINT('Ctrl Pts',(-8.08228808330916,0.834450058960203,
9.38408342654131));
#179649=CARTESIAN_POINT('Ctrl Pts',(-8.10218336896755,0.641748975816641,
9.39164898940678));
#179650=CARTESIAN_POINT('Ctrl Pts',(-8.11519077118466,0.448257265478159,
9.39921455227225));
#179651=CARTESIAN_POINT('Ctrl Pts',(-8.12126243570495,0.254527037675314,
9.40678011513772));
#179652=CARTESIAN_POINT('Ctrl Pts',(-8.12733356828999,0.060813782473072,
9.41434501518831));
#179653=CARTESIAN_POINT('Ctrl Pts',(-8.12647016194583,-0.13313758109363,
9.4219099152389));
#179654=CARTESIAN_POINT('Ctrl Pts',(-8.1186764370686,-0.326772815097942,
9.4294748152895));
#179655=CARTESIAN_POINT('Ctrl Pts',(-8.11087888707936,-0.520503084078696,
9.43704342814629));
#179656=CARTESIAN_POINT('Ctrl Pts',(-8.09614423488416,-0.713916545491256,
9.44461204100309));
#179657=CARTESIAN_POINT('Ctrl Pts',(-8.07452879829972,-0.906461387996509,
9.45218065385988));
#179658=CARTESIAN_POINT('Ctrl Pts',(-8.0529085548222,-1.0990490490896,9.45975094984312));
#179659=CARTESIAN_POINT('Ctrl Pts',(-8.02440453124403,-1.29076734241741,
9.46732124582635));
#179660=CARTESIAN_POINT('Ctrl Pts',(-7.98912453773546,-1.48107281490588,
9.47489154180958));
#179661=CARTESIAN_POINT('Ctrl Pts',(-7.95380879553575,-1.67157112109072,
9.4824695086608));
#179662=CARTESIAN_POINT('Ctrl Pts',(-7.91170344402178,-1.86065338679133,
9.49004747551202));
#179663=CARTESIAN_POINT('Ctrl Pts',(-7.8629669491208,-2.04778864132361,
9.49762544236324));
#179664=CARTESIAN_POINT('Ctrl Pts',(-7.81489808265974,-2.23236037916696,
9.5050996006374));
#179665=CARTESIAN_POINT('Ctrl Pts',(-7.76037875217189,-2.41503780479106,
9.51257375891156));
#179666=CARTESIAN_POINT('Ctrl Pts',(-7.69960716223324,-2.59532986531318,
9.52004791718572));
#179667=CARTESIAN_POINT('Ctrl Pts',(-7.6339515600846,-2.79011140399185,
9.52812274890461));
#179668=CARTESIAN_POINT('Ctrl Pts',(-7.56085858164267,-2.98252480353528,
9.5361975806235));
#179669=CARTESIAN_POINT('Ctrl Pts',(-7.48052139510541,-3.17198474458347,
9.54427241234239));
#179670=CARTESIAN_POINT('Ctrl Pts',(-7.40023735952158,-3.36131933923931,
9.55234190176561));
#179671=CARTESIAN_POINT('Ctrl Pts',(-7.31271879635653,-3.54770408113246,
9.56041139118882));
#179672=CARTESIAN_POINT('Ctrl Pts',(-7.2182077353601,-3.73057162532603,
9.56848088061203));
#179673=CARTESIAN_POINT('Ctrl Pts',(-7.12374632738373,-3.91334309689331,
9.57654613058944));
#179674=CARTESIAN_POINT('Ctrl Pts',(-7.02229989294093,-4.09260077501462,
9.58461138056686));
#179675=CARTESIAN_POINT('Ctrl Pts',(-6.91415760991501,-4.2677994455872,
9.59267663054428));
#179676=CARTESIAN_POINT('Ctrl Pts',(-6.80605742443153,-4.4429299149598,
9.60073874088756));
#179677=CARTESIAN_POINT('Ctrl Pts',(-6.69126675523716,-4.61400425905557,
9.60880085123083));
#179678=CARTESIAN_POINT('Ctrl Pts',(-6.57011985775149,-4.78050338534338,
9.61686296157411));
#179679=CARTESIAN_POINT('Ctrl Pts',(-6.4490036466253,-4.94696033760817,
9.6249230297948));
#179680=CARTESIAN_POINT('Ctrl Pts',(-6.32153460501466,-5.10884412785562,
9.63298309801549));
#179681=CARTESIAN_POINT('Ctrl Pts',(-6.18808965410538,-5.26566557951167,
9.64104316623618));
#179682=CARTESIAN_POINT('Ctrl Pts',(-6.05264549881148,-5.42483645039727,
9.64922398629962));
#179683=CARTESIAN_POINT('Ctrl Pts',(-5.91104514522524,-5.5787918197457,
9.65740480636305));
#179684=CARTESIAN_POINT('Ctrl Pts',(-5.76372491841141,-5.7270553190434,
9.66558562642648));
#179685=CARTESIAN_POINT('Ctrl Pts',(-5.61856510014355,-5.8731445769768,
9.67364647712821));
#179686=CARTESIAN_POINT('Ctrl Pts',(-5.46785226088467,-6.01370754355162,
9.68170732782993));
#179687=CARTESIAN_POINT('Ctrl Pts',(-5.31204095007485,-6.14832566697861,
9.68976817853165));
#179688=CARTESIAN_POINT('Ctrl Pts',(-5.15620379937592,-6.28296611559727,
9.69783036605216));
#179689=CARTESIAN_POINT('Ctrl Pts',(-4.99526673045904,-6.4116595474387,
9.70589255357267));
#179690=CARTESIAN_POINT('Ctrl Pts',(-4.82971786174866,-6.53402731387052,
9.71395474109319));
#179691=CARTESIAN_POINT('Ctrl Pts',(-4.66412102970979,-6.65643053306877,
9.72201926441551));
#179692=CARTESIAN_POINT('Ctrl Pts',(-4.49390998769988,-6.77250424322061,
9.73008378773784));
#179693=CARTESIAN_POINT('Ctrl Pts',(-4.31960283245551,-6.88191244730288,
9.73814831106017));
#179694=CARTESIAN_POINT('Ctrl Pts',(-4.14086433068113,-6.994102095812,9.74641785578504));
#179695=CARTESIAN_POINT('Ctrl Pts',(-3.95781899086813,-7.09928265356517,
9.75468740050991));
#179696=CARTESIAN_POINT('Ctrl Pts',(-3.77105322355808,-7.19714145668905,
9.76295694523478));
#179697=CARTESIAN_POINT('Ctrl Pts',(-3.58867172097493,-7.29270305671768,
9.77103236512742));
#179698=CARTESIAN_POINT('Ctrl Pts',(-3.40274280326232,-7.38128268722101,
9.77910778502006));
#179699=CARTESIAN_POINT('Ctrl Pts',(-3.21383402583139,-7.46263749735363,
9.7871832049127));
#179700=CARTESIAN_POINT('Ctrl Pts',(-3.01811348779624,-7.546925837088,9.79554981205368));
#179701=CARTESIAN_POINT('Ctrl Pts',(-2.81919455191184,-7.62345850405344,
9.80391641919466));
#179702=CARTESIAN_POINT('Ctrl Pts',(-2.6177272678535,-7.69202128920847,
9.81228302633563));
#179703=CARTESIAN_POINT('Ctrl Pts',(-2.41625998379515,-7.76058407436349,
9.82064963347661));
#179704=CARTESIAN_POINT('Ctrl Pts',(-2.21224472182711,-7.82117690662455,
9.82901624061759));
#179705=CARTESIAN_POINT('Ctrl Pts',(-2.00634528041495,-7.87364376754858,
9.83738284775857));
#179706=CARTESIAN_POINT('Ctrl Pts',(-1.80754962964786,-7.9243004555394,
9.84546079639163));
#179707=CARTESIAN_POINT('Ctrl Pts',(-1.60661112984514,-7.96748101058202,
9.8535387450247));
#179708=CARTESIAN_POINT('Ctrl Pts',(-1.40411856197274,-8.0030080986104,
9.86161669365776));
#179709=CARTESIAN_POINT('Ctrl Pts',(-1.20187380387928,-8.03849170869821,
9.86968475652224));
#179710=CARTESIAN_POINT('Ctrl Pts',(-0.998079077257228,-8.06634046783967,
9.87775281938672));
#179711=CARTESIAN_POINT('Ctrl Pts',(-0.793336921923672,-8.08642715238397,
9.88582088225121));
#179712=CARTESIAN_POINT('Ctrl Pts',(-0.588820123053253,-8.1064917278312,
9.89388006472607));
#179713=CARTESIAN_POINT('Ctrl Pts',(-0.383358286685486,-8.11881122997671,
9.90193924720093));
#179714=CARTESIAN_POINT('Ctrl Pts',(-0.177563325255657,-8.12330959818867,
9.90999842967579));
#179715=CARTESIAN_POINT('Ctrl Pts',(0.0279672997404689,-8.12780218840391,
9.9180472604125));
#179716=CARTESIAN_POINT('Ctrl Pts',(0.233829882009029,-8.1244936791582,
9.92609609114921));
#179717=CARTESIAN_POINT('Ctrl Pts',(0.439408168088388,-8.11335984807264,
9.93414492188592));
#179718=CARTESIAN_POINT('Ctrl Pts',(0.64483095568013,-8.10223443856664,
9.94218766452339));
#179719=CARTESIAN_POINT('Ctrl Pts',(0.849969561810193,-8.0832955223537,
9.95023040716086));
#179720=CARTESIAN_POINT('Ctrl Pts',(1.05420714503438,-8.05657091186185,
9.95827314979833));
#179721=CARTESIAN_POINT('Ctrl Pts',(1.25827836905849,-8.02986806957129,
9.96630934131915));
#179722=CARTESIAN_POINT('Ctrl Pts',(1.46144972204523,-7.99539222414565,
9.97434553283997));
#179723=CARTESIAN_POINT('Ctrl Pts',(1.6631086134198,-7.95322307636777,9.98238172436079));
#179724=CARTESIAN_POINT('Ctrl Pts',(1.77744106528548,-7.92931487164808,
9.98693792058886));
#179725=CARTESIAN_POINT('Ctrl Pts',(1.89128742262083,-7.90293465159328,
9.99149411681694));
#179726=CARTESIAN_POINT('Ctrl Pts',(2.00453702288224,-7.87410432280361,
9.99605031304501));
#179727=CARTESIAN_POINT('Ctrl Pts',(2.20429401534752,-7.82325151840061,
10.0040868275537));
#179728=CARTESIAN_POINT('Ctrl Pts',(2.40203572539872,-7.76481324266406,
10.0121233420623));
#179729=CARTESIAN_POINT('Ctrl Pts',(2.59717513615446,-7.69898492495219,
10.020159856571));
#179730=CARTESIAN_POINT('Ctrl Pts',(2.79243243053666,-7.63311684038448,
10.0282012259343));
#179731=CARTESIAN_POINT('Ctrl Pts',(2.98508399004642,-7.55984990822988,
10.0362425952976));
#179732=CARTESIAN_POINT('Ctrl Pts',(3.17456178869415,-7.47942812066959,
10.0442839646609));
#179733=CARTESIAN_POINT('Ctrl Pts',(3.36417721801751,-7.3989479172683,10.0523311750204));
#179734=CARTESIAN_POINT('Ctrl Pts',(3.55061399672931,-7.3113026130809,10.0603783853799));
#179735=CARTESIAN_POINT('Ctrl Pts',(3.73332720545528,-7.21678290788267,
10.0684255957394));
#179736=CARTESIAN_POINT('Ctrl Pts',(3.91630972040398,-7.12212388738831,
10.0764846671123));
#179737=CARTESIAN_POINT('Ctrl Pts',(4.09555741533467,-7.02057035998896,
10.0845437384853));
#179738=CARTESIAN_POINT('Ctrl Pts',(4.27055145076036,-6.91245816398975,
10.0926028098582));
#179739=CARTESIAN_POINT('Ctrl Pts',(4.44568711744493,-6.80425846748584,
10.100668403833));
#179740=CARTESIAN_POINT('Ctrl Pts',(4.61656199277263,-6.68948968504108,
10.1087339978078));
#179741=CARTESIAN_POINT('Ctrl Pts',(4.78268831542635,-6.56852951884851,
10.1167995917826));
#179742=CARTESIAN_POINT('Ctrl Pts',(4.94907549436119,-6.44737941755949,
10.1248778505827));
#179743=CARTESIAN_POINT('Ctrl Pts',(5.11069896875312,-6.32001869528888,
10.1329561093828));
#179744=CARTESIAN_POINT('Ctrl Pts',(5.26710465191401,-6.18686480766194,
10.1410343681829));
#179745=CARTESIAN_POINT('Ctrl Pts',(5.35541423962851,-6.11168362062782,
10.1455955048991));
#179746=CARTESIAN_POINT('Ctrl Pts',(5.44206109547213,-6.03465627404792,
10.1501566416153));
#179747=CARTESIAN_POINT('Ctrl Pts',(5.52696893801387,-5.95586281916649,
10.1547177783315));
#179748=CARTESIAN_POINT('Ctrl Pts',(5.67489187501032,-5.81859211585745,
10.1626640023657));
#179749=CARTESIAN_POINT('Ctrl Pts',(5.81785214234309,-5.67566425775407,
10.1706102264));
#179750=CARTESIAN_POINT('Ctrl Pts',(5.95539848735943,-5.52746925991063,
10.1785564504342));
#179751=CARTESIAN_POINT('Ctrl Pts',(6.09281483459454,-5.37941432410161,
10.1864951643344));
#179752=CARTESIAN_POINT('Ctrl Pts',(6.22482723158983,-5.22610241249131,
10.1944338782345));
#179753=CARTESIAN_POINT('Ctrl Pts',(6.35101957562125,-5.06796190914806,
10.2023725921347));
#179754=CARTESIAN_POINT('Ctrl Pts',(6.47711398298939,-4.90994413712695,
10.2103051448755));
#179755=CARTESIAN_POINT('Ctrl Pts',(6.59739713336566,-4.74710550222358,
10.2182376976162));
#179756=CARTESIAN_POINT('Ctrl Pts',(6.71149140988143,-4.57990945517352,
10.2261702503569));
#179757=CARTESIAN_POINT('Ctrl Pts',(6.82567620409571,-4.4125807616679,10.2341090964582));
#179758=CARTESIAN_POINT('Ctrl Pts',(6.93366208037581,-4.24088799197895,
10.2420479425595));
#179759=CARTESIAN_POINT('Ctrl Pts',(7.03511154143971,-4.06532817396108,
10.2499867886608));
#179760=CARTESIAN_POINT('Ctrl Pts',(7.13637486580226,-3.89009046830412,
10.257911068784));
#179761=CARTESIAN_POINT('Ctrl Pts',(7.23112556563233,-3.7110001773017,10.2658353489072));
#179762=CARTESIAN_POINT('Ctrl Pts',(7.31907177064689,-3.52857988128649,
10.2737596290304));
#179763=CARTESIAN_POINT('Ctrl Pts',(7.40699841233518,-3.34620016402927,
10.2816821464251));
#179764=CARTESIAN_POINT('Ctrl Pts',(7.48812343151978,-3.16049221822206,
10.2896046638199));
#179765=CARTESIAN_POINT('Ctrl Pts',(7.5622014199931,-2.97200222845715,10.2975271812146));
#179766=CARTESIAN_POINT('Ctrl Pts',(7.63627427329671,-2.78352530503093,
10.3054491494115));
#179767=CARTESIAN_POINT('Ctrl Pts',(7.70330094841308,-2.59226703245282,
10.3133711176084));
#179768=CARTESIAN_POINT('Ctrl Pts',(7.76308445035316,-2.39879290043657,
10.3212930858053));
#179769=CARTESIAN_POINT('Ctrl Pts',(7.82308545170148,-2.20461488678313,
10.3292438750539));
#179770=CARTESIAN_POINT('Ctrl Pts',(7.87579035692534,-2.00820517647219,
10.3371946643024));
#179771=CARTESIAN_POINT('Ctrl Pts',(7.9210506457439,-1.81015033355248,10.3451454535509));
#179772=CARTESIAN_POINT('Ctrl Pts',(7.96617330192918,-1.6126977583221,10.3530720651353));
#179773=CARTESIAN_POINT('Ctrl Pts',(8.00389651687895,-1.41361037583155,
10.3609986767197));
#179774=CARTESIAN_POINT('Ctrl Pts',(8.03412444581144,-1.21347927535452,
10.3689252883041));
#179775=CARTESIAN_POINT('Ctrl Pts',(8.06449067609217,-1.01243251833082,
10.3768881663847));
#179776=CARTESIAN_POINT('Ctrl Pts',(8.08729281276306,-0.810332804847844,
10.3848510444653));
#179777=CARTESIAN_POINT('Ctrl Pts',(8.10248639470418,-0.607784325343876,
10.3928139225459));
#179778=CARTESIAN_POINT('Ctrl Pts',(8.1176799766453,-0.405235845839927,
10.4007768006264));
#179779=CARTESIAN_POINT('Ctrl Pts',(8.12526501457307,-0.202238940266611,
10.408739678707));
#179780=CARTESIAN_POINT('Ctrl Pts',(8.12524997767401,0.00060233580707081,
10.4167025567876));
#179781=CARTESIAN_POINT('',(8.12456022843635,0.000454668290610622,4.4166972245402));
#179782=CARTESIAN_POINT('Ctrl Pts',(8.12524944607656,0.00300025542302204,
8.41865443786164));
#179783=CARTESIAN_POINT('Ctrl Pts',(8.12534260691395,-0.249296611252544,
8.40866000239997));
#179784=CARTESIAN_POINT('Ctrl Pts',(8.11368452319427,-0.501462439799894,
8.39863635441595));
#179785=CARTESIAN_POINT('Ctrl Pts',(8.0377516071859,-1.31764703565447,8.36566170274765));
#179786=CARTESIAN_POINT('Ctrl Pts',(7.92615719088016,-1.87552917470942,
8.34208384265915));
#179787=CARTESIAN_POINT('Ctrl Pts',(7.64656162715796,-2.77282008568974,
8.30231745151355));
#179788=CARTESIAN_POINT('Ctrl Pts',(7.51142444228261,-3.12040800446353,
8.28647102020751));
#179789=CARTESIAN_POINT('Ctrl Pts',(7.30041202776761,-3.5691590430266,8.26611919427734));
#179790=CARTESIAN_POINT('Ctrl Pts',(7.24536934550857,-3.67961094765436,
8.2611223662416));
#179791=CARTESIAN_POINT('Ctrl Pts',(7.17966997329027,-3.80425195867326,
8.25553074496127));
#179792=CARTESIAN_POINT('Ctrl Pts',(7.17145871633034,-3.81970859833049,
8.25483817907225));
#179793=CARTESIAN_POINT('Ctrl Pts',(7.15898032954345,-3.84301548696492,
8.25379528236128));
#179794=CARTESIAN_POINT('Ctrl Pts',(7.15475011581351,-3.85088537519616,
8.25344337872774));
#179795=CARTESIAN_POINT('Ctrl Pts',(7.14713155394543,-3.86500305670066,
8.25281256485714));
#179796=CARTESIAN_POINT('Ctrl Pts',(7.1437479759943,-3.87125340601894,8.25253344602394));
#179797=CARTESIAN_POINT('Ctrl Pts',(7.13697882924859,-3.88371868709492,
8.25197712692639));
#179798=CARTESIAN_POINT('Ctrl Pts',(7.13359333311571,-3.88993365081527,
8.25169992380246));
#179799=CARTESIAN_POINT('Ctrl Pts',(7.12415972589869,-3.90719777146968,
8.25093038305258));
#179800=CARTESIAN_POINT('Ctrl Pts',(7.11809401932202,-3.91823732817893,
8.25043885005597));
#179801=CARTESIAN_POINT('Ctrl Pts',(7.09387332162766,-3.96207701920554,
8.24848922888969));
#179802=CARTESIAN_POINT('Ctrl Pts',(7.07551689672411,-3.99476579024089,
8.24704069771003));
#179803=CARTESIAN_POINT('Ctrl Pts',(6.76188044598456,-4.54433926815202,
8.22279112250198));
#179804=CARTESIAN_POINT('Ctrl Pts',(6.4108794613095,-5.02740199910961,8.20309811404289));
#179805=CARTESIAN_POINT('Ctrl Pts',(5.88158080035,-5.60921083806592,8.17687225117711));
#179806=CARTESIAN_POINT('Ctrl Pts',(5.74797533568672,-5.74604363652688,
8.17049518475249));
#179807=CARTESIAN_POINT('Ctrl Pts',(5.5653126300551,-5.92036674148974,8.1619582002572));
#179808=CARTESIAN_POINT('Ctrl Pts',(5.52047853553056,-5.96219453576103,
8.15987661446729));
#179809=CARTESIAN_POINT('Ctrl Pts',(5.11529906270398,-6.33171644982272,
8.14116181751614));
#179810=CARTESIAN_POINT('Ctrl Pts',(4.7266803899364,-6.62686534366664,8.12381544392025));
#179811=CARTESIAN_POINT('Ctrl Pts',(4.2902568765596,-6.90030203766106,8.103975392903));
#179812=CARTESIAN_POINT('Ctrl Pts',(4.26644192529054,-6.91505210083696,
8.10289194788854));
#179813=CARTESIAN_POINT('Ctrl Pts',(4.23157834451104,-6.93639660154787,
8.10130457156946));
#179814=CARTESIAN_POINT('Ctrl Pts',(4.22058946460535,-6.94308848201863,
8.10080405154524));
#179815=CARTESIAN_POINT('Ctrl Pts',(4.20127629922086,-6.95478679598479,
8.0999240430966));
#179816=CARTESIAN_POINT('Ctrl Pts',(4.19295883117123,-6.95980446271971,
8.09954494727588));
#179817=CARTESIAN_POINT('Ctrl Pts',(4.1767916233789,-6.96951813026772,8.09880785797876));
#179818=CARTESIAN_POINT('Ctrl Pts',(4.16894290974978,-6.97421581598019,
8.09844992386518));
#179819=CARTESIAN_POINT('Ctrl Pts',(4.148031421311,-6.98668404236181,8.0974960051728));
#179820=CARTESIAN_POINT('Ctrl Pts',(4.13495477586364,-6.99443118334179,
8.09689921099505));
#179821=CARTESIAN_POINT('Ctrl Pts',(4.08820580666027,-7.02195027038946,
8.09476465377508));
#179822=CARTESIAN_POINT('Ctrl Pts',(4.05441303839648,-7.04151597170442,
8.09321979085663));
#179823=CARTESIAN_POINT('Ctrl Pts',(3.44455844645803,-7.38877064412927,
8.06530385254013));
#179824=CARTESIAN_POINT('Ctrl Pts',(2.83076068569412,-7.64496356562687,
8.03635968125928));
#179825=CARTESIAN_POINT('Ctrl Pts',(1.76624123764915,-7.94331856062741,
7.98676579225785));
#179826=CARTESIAN_POINT('Ctrl Pts',(1.33062448440572,-8.02778799728385,
7.96670764408717));
#179827=CARTESIAN_POINT('Ctrl Pts',(0.775496644500221,-8.08898196579719,
7.94277600558132));
#179828=CARTESIAN_POINT('Ctrl Pts',(0.660446611907645,-8.09918738663522,
7.93790535856544));
#179829=CARTESIAN_POINT('Ctrl Pts',(0.455676824548966,-8.11295873628207,
7.92943506002988));
#179830=CARTESIAN_POINT('Ctrl Pts',(0.36605036596667,-8.11749644997351,
7.92579858182746));
#179831=CARTESIAN_POINT('Ctrl Pts',(0.259815004791978,-8.1211118533455,
7.92156732655496));
#179832=CARTESIAN_POINT('Ctrl Pts',(0.243269607749017,-8.12162431257731,
7.92091051794962));
#179833=CARTESIAN_POINT('Ctrl Pts',(0.217750631279871,-8.12233665797232,
7.91990070580214));
#179834=CARTESIAN_POINT('Ctrl Pts',(0.208778151374865,-8.12257224081205,
7.91954627008097));
#179835=CARTESIAN_POINT('Ctrl Pts',(0.192395847720523,-8.12297521436143,
7.91890022384888));
#179836=CARTESIAN_POINT('Ctrl Pts',(0.184986157592064,-8.12314733445795,
7.91860842759105));
#179837=CARTESIAN_POINT('Ctrl Pts',(0.168805544615237,-8.12350104402242,
7.91797210607642));
#179838=CARTESIAN_POINT('Ctrl Pts',(0.160034536221588,-8.12367856774821,
7.91762773846986));
#179839=CARTESIAN_POINT('Ctrl Pts',(0.136054314233893,-8.12412507151278,
7.91668772858946));
#179840=CARTESIAN_POINT('Ctrl Pts',(0.120844564410304,-8.12436554747737,
7.91609316786816));
#179841=CARTESIAN_POINT('Ctrl Pts',(0.0466763598827749,-8.12532986964952,
7.91320160250645));
#179842=CARTESIAN_POINT('Ctrl Pts',(-0.0122889087893892,-8.12545465525289,
7.91092654445423));
#179843=CARTESIAN_POINT('Ctrl Pts',(-0.221388313676638,-8.12362097148719,
7.90292955103741));
#179844=CARTESIAN_POINT('Ctrl Pts',(-0.37146443918913,-8.11814307850608,
7.89731873305295));
#179845=CARTESIAN_POINT('Ctrl Pts',(-1.34457009813896,-8.05558092027543,
7.86138567143121));
#179846=CARTESIAN_POINT('Ctrl Pts',(-2.15498582732562,-7.87758984720788,
7.83291006186798));
#179847=CARTESIAN_POINT('Ctrl Pts',(-3.00975943467444,-7.54780382010189,
7.79821889491473));
#179848=CARTESIAN_POINT('Ctrl Pts',(-3.09423291042571,-7.51356884163044,
7.79474483606738));
#179849=CARTESIAN_POINT('Ctrl Pts',(-3.22114261913608,-7.45963228960563,
7.78945382780329));
#179850=CARTESIAN_POINT('Ctrl Pts',(-3.26401458009064,-7.44097321912761,
7.78765390572753));
#179851=CARTESIAN_POINT('Ctrl Pts',(-3.33336314464183,-7.41007613233208,
7.78472186493577));
#179852=CARTESIAN_POINT('Ctrl Pts',(-3.35993921279015,-7.39806370731183,
7.78359329768125));
#179853=CARTESIAN_POINT('Ctrl Pts',(-3.41107049969226,-7.37461993674546,
7.78141244117141));
#179854=CARTESIAN_POINT('Ctrl Pts',(-3.43563438110046,-7.36320837386806,
7.78036046433375));
#179855=CARTESIAN_POINT('Ctrl Pts',(-3.47949209787296,-7.3425662908357,
7.77847456083947));
#179856=CARTESIAN_POINT('Ctrl Pts',(-3.49880745423363,-7.33338198842546,
7.77764132398668));
#179857=CARTESIAN_POINT('Ctrl Pts',(-3.53658784984703,-7.31523446189932,
7.77600629816258));
#179858=CARTESIAN_POINT('Ctrl Pts',(-3.55505567025594,-7.30627730313551,
7.77520459026061));
#179859=CARTESIAN_POINT('Ctrl Pts',(-3.60303835966907,-7.28278001013083,
7.77311500387701));
#179860=CARTESIAN_POINT('Ctrl Pts',(-3.63249913769739,-7.26813044032397,
7.77182548892977));
#179861=CARTESIAN_POINT('Ctrl Pts',(-3.73370930349587,-7.21703392552023,
7.76737209568682));
#179862=CARTESIAN_POINT('Ctrl Pts',(-3.80500512558346,-7.17970052405029,
7.76419423100621));
#179863=CARTESIAN_POINT('Ctrl Pts',(-4.53486090853337,-6.78359321615267,
7.73121007958053));
#179864=CARTESIAN_POINT('Ctrl Pts',(-5.14125102299569,-6.33635816074945,
7.69947678387429));
#179865=CARTESIAN_POINT('Ctrl Pts',(-5.82529055125906,-5.66818198326413,
7.65900168320172));
#179866=CARTESIAN_POINT('Ctrl Pts',(-5.96740705251279,-5.51836510735763,
7.6503131271698));
#179867=CARTESIAN_POINT('Ctrl Pts',(-6.19879604448457,-5.25503430559901,
7.63583922995285));
#179868=CARTESIAN_POINT('Ctrl Pts',(-6.29103179474673,-5.14425693088022,
7.62997231297557));
#179869=CARTESIAN_POINT('Ctrl Pts',(-6.39189037085557,-5.01635096240967,
7.62348980335229));
#179870=CARTESIAN_POINT('Ctrl Pts',(-6.40345525169489,-5.00157978417776,
7.62274545896565));
#179871=CARTESIAN_POINT('Ctrl Pts',(-6.4207619423157,-4.97931649282912,
7.6216301462768));
#179872=CARTESIAN_POINT('Ctrl Pts',(-6.42654198222926,-4.97185426246654,
7.62125741857805));
#179873=CARTESIAN_POINT('Ctrl Pts',(-6.43646502730784,-4.95899705427772,
7.62061713785193));
#179874=CARTESIAN_POINT('Ctrl Pts',(-6.44061427861283,-4.9536069228976,
7.62034929099859));
#179875=CARTESIAN_POINT('Ctrl Pts',(-6.44915072201265,-4.94248870362179,
7.61979800370699));
#179876=CARTESIAN_POINT('Ctrl Pts',(-6.45353706358665,-4.93675996884284,
7.61951460398038));
#179877=CARTESIAN_POINT('Ctrl Pts',(-6.46408547284372,-4.92294524812819,
7.61883278074699));
#179878=CARTESIAN_POINT('Ctrl Pts',(-6.47024001582722,-4.91485351308372,
7.61843472280437));
#179879=CARTESIAN_POINT('Ctrl Pts',(-6.49275756970491,-4.88513277842739,
7.61697751651493));
#179880=CARTESIAN_POINT('Ctrl Pts',(-6.50902756029763,-4.86343328981747,
7.61592298916242));
#179881=CARTESIAN_POINT('Ctrl Pts',(-6.77406394104908,-4.50623863859396,
7.59872303054515));
#179882=CARTESIAN_POINT('Ctrl Pts',(-6.99670818662388,-4.15213277211256,
7.5841195827693));
#179883=CARTESIAN_POINT('Ctrl Pts',(-7.41618764208672,-3.35463143982238,
7.55346737421054));
#179884=CARTESIAN_POINT('Ctrl Pts',(-7.60259977251472,-2.90755416900889,
7.53755568600385));
#179885=CARTESIAN_POINT('Ctrl Pts',(-7.86953076971025,-2.06219278068322,
7.50676350167311));
#179886=CARTESIAN_POINT('Ctrl Pts',(-7.96211877441408,-1.66936444718148,
7.49220103349142));
#179887=CARTESIAN_POINT('Ctrl Pts',(-8.03021801509914,-1.23948548241302,
7.47546118782563));
#179888=CARTESIAN_POINT('Ctrl Pts',(-8.03506977776106,-1.20763374810521,
7.47421639424351));
#179889=CARTESIAN_POINT('Ctrl Pts',(-8.04170330318605,-1.16227412645094,
7.47243717475473));
#179890=CARTESIAN_POINT('Ctrl Pts',(-8.043640759158,-1.14878914381878,7.47190741067092));
#179891=CARTESIAN_POINT('Ctrl Pts',(-8.04691974277996,-1.1255519183334,
7.47099309931554));
#179892=CARTESIAN_POINT('Ctrl Pts',(-8.04827748155222,-1.11580197468481,
7.47060903788999));
#179893=CARTESIAN_POINT('Ctrl Pts',(-8.0508375941445,-1.09716996491519,
7.4698742706666));
#179894=CARTESIAN_POINT('Ctrl Pts',(-8.05204299659385,-1.08828832558782,
7.46952365605336));
#179895=CARTESIAN_POINT('Ctrl Pts',(-8.05482410754143,-1.06753898490405,
7.46870370087325));
#179896=CARTESIAN_POINT('Ctrl Pts',(-8.05638828600611,-1.05566977381634,
7.46823401631452));
#179897=CARTESIAN_POINT('Ctrl Pts',(-8.06167364626418,-1.0148677445927,
7.46661717166501));
#179898=CARTESIAN_POINT('Ctrl Pts',(-8.06526522551564,-0.985918525290401,
7.46546614354029));
#179899=CARTESIAN_POINT('Ctrl Pts',(-8.10168630555391,-0.67882770478392,
7.45321446269102));
#179900=CARTESIAN_POINT('Ctrl Pts',(-8.12026749782283,-0.399205255910186,
7.44168764108077));
#179901=CARTESIAN_POINT('Ctrl Pts',(-8.12566580845965,-0.0312605098491741,
7.42603884627491));
#179902=CARTESIAN_POINT('Ctrl Pts',(-8.12552815692169,0.0566895633651244,
7.4222630430183));
#179903=CARTESIAN_POINT('Ctrl Pts',(-8.11591258082036,0.596845258737921,
7.39887079871206));
#179904=CARTESIAN_POINT('Ctrl Pts',(-8.07011624145231,1.04758863163167,
7.37842566821632));
#179905=CARTESIAN_POINT('Ctrl Pts',(-7.92731785978853,1.8119497849267,7.34337567173789));
#179906=CARTESIAN_POINT('Ctrl Pts',(-7.84841626461965,2.1278886018736,7.3287895323074));
#179907=CARTESIAN_POINT('Ctrl Pts',(-7.70980537876419,2.56850799508236,
7.30892515066826));
#179908=CARTESIAN_POINT('Ctrl Pts',(-7.66555168973068,2.69771246994982,
7.30316198463242));
#179909=CARTESIAN_POINT('Ctrl Pts',(-7.59614441358077,2.88483085741031,
7.29496020799337));
#179910=CARTESIAN_POINT('Ctrl Pts',(-7.57354118326881,2.94365989215785,
7.29240365041295));
#179911=CARTESIAN_POINT('Ctrl Pts',(-7.53987257898884,3.02833262489012,
7.28875750915561));
#179912=CARTESIAN_POINT('Ctrl Pts',(-7.5293555430975,3.05438735736778,7.28763990774156));
#179913=CARTESIAN_POINT('Ctrl Pts',(-7.5145965565082,3.09041154358981,7.28610004706287));
#179914=CARTESIAN_POINT('Ctrl Pts',(-7.51046957890354,3.10042765143268,
7.28567248450194));
#179915=CARTESIAN_POINT('Ctrl Pts',(-7.50345776048527,3.11734906667848,
7.28495108287856));
#179916=CARTESIAN_POINT('Ctrl Pts',(-7.50058339563923,3.12425867886637,
7.28465677213816));
#179917=CARTESIAN_POINT('Ctrl Pts',(-7.49486730198034,3.13794609607371,
7.28407426865178));
#179918=CARTESIAN_POINT('Ctrl Pts',(-7.4920259153668,3.14472403560261,7.28378606113987));
#179919=CARTESIAN_POINT('Ctrl Pts',(-7.48572913914173,3.15968760508366,
7.28315031236115));
#179920=CARTESIAN_POINT('Ctrl Pts',(-7.48226950847464,3.16787144778167,
7.2828029564108));
#179921=CARTESIAN_POINT('Ctrl Pts',(-7.47007070796946,3.19659654872677,
7.2815849097379));
#179922=CARTESIAN_POINT('Ctrl Pts',(-7.46126027198687,3.2171075585464,7.28071726426838));
#179923=CARTESIAN_POINT('Ctrl Pts',(-7.33987764428502,3.49650979661669,
7.26892356072496));
#179924=CARTESIAN_POINT('Ctrl Pts',(-7.21396527920489,3.74941410588792,
7.2585382690809));
#179925=CARTESIAN_POINT('Ctrl Pts',(-6.86103050427722,4.37442016803562,
7.2325510889286));
#179926=CARTESIAN_POINT('Ctrl Pts',(-6.61679079851957,4.7357555489666,7.21717627980339));
#179927=CARTESIAN_POINT('Ctrl Pts',(-5.97215748615665,5.54155253418819,
7.17968465351304));
#179928=CARTESIAN_POINT('Ctrl Pts',(-5.549408455108,5.96485191978368,7.15719195527464));
#179929=CARTESIAN_POINT('Ctrl Pts',(-4.99597346967715,6.40880054611747,
7.12977449297168));
#179930=CARTESIAN_POINT('Ctrl Pts',(-4.9062968159236,6.47770998082798,7.12538876577189));
#179931=CARTESIAN_POINT('Ctrl Pts',(-4.77498594283834,6.57432056041182,
7.11903810587708));
#179932=CARTESIAN_POINT('Ctrl Pts',(-4.73448824508579,6.60354470062865,
7.11708899843027));
#179933=CARTESIAN_POINT('Ctrl Pts',(-4.66281366740475,6.65426857140178,
7.11365513904391));
#179934=CARTESIAN_POINT('Ctrl Pts',(-4.63175103283471,6.6759271920774,7.1121720778364));
#179935=CARTESIAN_POINT('Ctrl Pts',(-4.56655066807166,6.7207144542792,7.10906938499359));
#179936=CARTESIAN_POINT('Ctrl Pts',(-4.53238599631842,6.7438019649925,7.10744937750362));
#179937=CARTESIAN_POINT('Ctrl Pts',(-4.44206404910055,6.8038425577854,7.10318109711383));
#179938=CARTESIAN_POINT('Ctrl Pts',(-4.38562150698715,6.84036040635741,
7.10052847164612));
#179939=CARTESIAN_POINT('Ctrl Pts',(-4.13030844277705,7.00108671385293,
7.08859114512913));
#179940=CARTESIAN_POINT('Ctrl Pts',(-3.92657334985303,7.11735075261285,
7.0792288084521));
#179941=CARTESIAN_POINT('Ctrl Pts',(-3.69550106896186,7.23627012680759,
7.06876990993719));
#179942=CARTESIAN_POINT('Ctrl Pts',(-3.67284842843474,7.24779400351911,
7.06774627856101));
#179943=CARTESIAN_POINT('Ctrl Pts',(-3.20770173738158,7.4816832564008,7.04676157098265));
#179944=CARTESIAN_POINT('Ctrl Pts',(-2.74585191758023,7.66323864455631,
7.02651657541934));
#179945=CARTESIAN_POINT('Ctrl Pts',(-2.16117722389955,7.83338563846384,
7.00195916229492));
#179946=CARTESIAN_POINT('Ctrl Pts',(-2.05134039133282,7.86286338396046,
6.99739262479145));
#179947=CARTESIAN_POINT('Ctrl Pts',(-1.90679551975368,7.89842094187259,
6.99145350898929));
#179948=CARTESIAN_POINT('Ctrl Pts',(-1.87261656037477,7.90659406850063,
6.99005426983802));
#179949=CARTESIAN_POINT('Ctrl Pts',(-1.79235027644293,7.92523826995822,
6.98678081330815));
#179950=CARTESIAN_POINT('Ctrl Pts',(-1.74622235047893,7.93552951596186,
6.98490925483222));
#179951=CARTESIAN_POINT('Ctrl Pts',(-1.67824647164587,7.95007368156257,
6.98216629364125));
#179952=CARTESIAN_POINT('Ctrl Pts',(-1.65646679806028,7.95464018776109,
6.98128970645587));
#179953=CARTESIAN_POINT('Ctrl Pts',(-1.61652387749098,7.96284379054159,
6.97968633436949));
#179954=CARTESIAN_POINT('Ctrl Pts',(-1.59836647930091,7.96650834932912,
6.97895905787417));
#179955=CARTESIAN_POINT('Ctrl Pts',(-1.55735235247661,7.97464002883764,
6.97731964527661));
#179956=CARTESIAN_POINT('Ctrl Pts',(-1.53448860954826,7.97907103940914,
6.97640809438307));
#179957=CARTESIAN_POINT('Ctrl Pts',(-1.47505548828391,7.99032431816325,
6.97404418834783));
#179958=CARTESIAN_POINT('Ctrl Pts',(-1.43845767320748,7.99699386923838,
6.9725940568141));
#179959=CARTESIAN_POINT('Ctrl Pts',(-1.1850270053247,8.04138280916626,6.96258521506639));
#179960=CARTESIAN_POINT('Ctrl Pts',(-0.96678317271843,8.07053026927719,
6.95412927206227));
#179961=CARTESIAN_POINT('Ctrl Pts',(-0.573608558143245,8.10686133038639,
6.9389515139325));
#179962=CARTESIAN_POINT('Ctrl Pts',(-0.399120584786872,8.11732282281341,
6.93223603027996));
#179963=CARTESIAN_POINT('Ctrl Pts',(-0.113961355100009,8.1252023604628,
6.92121873631451));
#179964=CARTESIAN_POINT('Ctrl Pts',(-0.00344080132436661,8.12600076934443,
6.91693867788918));
#179965=CARTESIAN_POINT('Ctrl Pts',(0.153896966162853,8.12392745351893,
6.91081993913141));
#179966=CARTESIAN_POINT('Ctrl Pts',(0.200726542749659,8.12290529175856,
6.90899557764855));
#179967=CARTESIAN_POINT('Ctrl Pts',(0.282921203010633,8.12039997945412,
6.90578708406969));
#179968=CARTESIAN_POINT('Ctrl Pts',(0.318290368681357,8.11909055649516,
6.90440435854074));
#179969=CARTESIAN_POINT('Ctrl Pts',(0.392340890805987,8.11586446605905,
6.9015047369219));
#179970=CARTESIAN_POINT('Ctrl Pts',(0.431019368450027,8.11390224840457,
6.89998751152092));
#179971=CARTESIAN_POINT('Ctrl Pts',(0.534042672797172,8.10793698406128,
6.89593868383245));
#179972=CARTESIAN_POINT('Ctrl Pts',(0.59835621223947,8.10344454513105,6.89340325719327));
#179973=CARTESIAN_POINT('Ctrl Pts',(1.00324152840568,8.07031605083843,6.87738872789994));
#179974=CARTESIAN_POINT('Ctrl Pts',(1.34177188564481,8.02098101831701,6.86374158095071));
#179975=CARTESIAN_POINT('Ctrl Pts',(1.85459408217703,7.91286383608297,6.84280958408104));
#179976=CARTESIAN_POINT('Ctrl Pts',(2.03169094336306,7.86925448640611,6.83553700447935));
#179977=CARTESIAN_POINT('Ctrl Pts',(2.24912107997073,7.80788331740689,6.82660761787461));
#179978=CARTESIAN_POINT('Ctrl Pts',(2.29097489695784,7.79570532939139,6.82488883832693));
#179979=CARTESIAN_POINT('Ctrl Pts',(2.35373497259993,7.77689527612172,6.82231276765226));
#179980=CARTESIAN_POINT('Ctrl Pts',(2.37471550717156,7.77051444384044,6.82145183272699));
#179981=CARTESIAN_POINT('Ctrl Pts',(2.41469682568755,7.7581778329147,6.81981165584626));
#179982=CARTESIAN_POINT('Ctrl Pts',(2.43370197224416,7.75223701653842,6.81903216819185));
#179983=CARTESIAN_POINT('Ctrl Pts',(2.47748460362841,7.73837413629093,6.81723662437312));
#179984=CARTESIAN_POINT('Ctrl Pts',(2.50224629014142,7.73040281902605,6.81622127160013));
#179985=CARTESIAN_POINT('Ctrl Pts',(2.56936410481981,7.70843988313111,6.81346891702132));
#179986=CARTESIAN_POINT('Ctrl Pts',(2.61164407699267,7.69421812652251,6.81173490079762));
#179987=CARTESIAN_POINT('Ctrl Pts',(2.84790229169533,7.61257595434493,6.8020385380735));
#179988=CARTESIAN_POINT('Ctrl Pts',(3.03938889924414,7.5381679986173,6.79415245964485));
#179989=CARTESIAN_POINT('Ctrl Pts',(3.23201800181182,7.45478153987207,6.78610264548836));
#179990=CARTESIAN_POINT('Ctrl Pts',(3.23618258423733,7.45297460432817,6.78592855508331));
#179991=CARTESIAN_POINT('Ctrl Pts',(3.31091498706415,7.42047514374496,6.78280352748804));
#179992=CARTESIAN_POINT('Ctrl Pts',(3.38104480385011,7.38878511343108,6.7798546212425));
#179993=CARTESIAN_POINT('Ctrl Pts',(3.66554315654899,7.25532826509284,6.76780905966538));
#179994=CARTESIAN_POINT('Ctrl Pts',(3.87585341173315,7.14519097639767,6.75870773653853));
#179995=CARTESIAN_POINT('Ctrl Pts',(4.14474530550063,6.98900575353771,6.74669834615255));
#179996=CARTESIAN_POINT('Ctrl Pts',(4.20794370920409,6.95113837776932,6.74384794559773));
#179997=CARTESIAN_POINT('Ctrl Pts',(4.36176045991743,6.85610756234524,6.73683765943862));
#179998=CARTESIAN_POINT('Ctrl Pts',(4.45177966673619,6.79800138311449,6.73267166060439));
#179999=CARTESIAN_POINT('Ctrl Pts',(4.59084941709583,6.70428649628685,6.72612996389287));
#180000=CARTESIAN_POINT('Ctrl Pts',(4.64069558631785,6.66988007635293,6.72376342215126));
#180001=CARTESIAN_POINT('Ctrl Pts',(4.73543647177023,6.60290877862507,6.71922262612382));
#180002=CARTESIAN_POINT('Ctrl Pts',(4.78039165042046,6.5704351879868,6.71704911487873));
#180003=CARTESIAN_POINT('Ctrl Pts',(4.88912097587145,6.49018741059794,6.71174561180416));
#180004=CARTESIAN_POINT('Ctrl Pts',(4.95253152735596,6.44193045193084,6.70861281418788));
#180005=CARTESIAN_POINT('Ctrl Pts',(5.17186400146934,6.2698603368207,6.69763640265128));
#180006=CARTESIAN_POINT('Ctrl Pts',(5.32393619346197,6.14125629959123,6.68977121629631));
#180007=CARTESIAN_POINT('Ctrl Pts',(5.55119565259601,5.93427689029336,6.6776403218635));
#180008=CARTESIAN_POINT('Ctrl Pts',(5.62979524603987,5.85976287954128,6.67337050000588));
#180009=CARTESIAN_POINT('Ctrl Pts',(5.73758103940436,5.75340867349887,6.6674173026549));
#180010=CARTESIAN_POINT('Ctrl Pts',(5.76803843152039,5.72287342338029,6.66572379276338));
#180011=CARTESIAN_POINT('Ctrl Pts',(5.8257065919205,5.66412978541909,6.6624963737859));
#180012=CARTESIAN_POINT('Ctrl Pts',(5.85295918608722,5.63596418538932,6.66096199776645));
#180013=CARTESIAN_POINT('Ctrl Pts',(5.94161647773084,5.54300012504445,6.65593806446214));
#180014=CARTESIAN_POINT('Ctrl Pts',(6.00215730512554,5.47738665123967,6.65245576057196));
#180015=CARTESIAN_POINT('Ctrl Pts',(6.17649973924291,5.28207410494277,6.64225332444279));
#180016=CARTESIAN_POINT('Ctrl Pts',(6.28726577251524,5.14973251800901,6.63554457889934));
#180017=CARTESIAN_POINT('Ctrl Pts',(6.44104691979512,4.95363306853353,6.62583134624681));
#180018=CARTESIAN_POINT('Ctrl Pts',(6.48750297118287,4.89263437812307,6.62284042754036));
#180019=CARTESIAN_POINT('Ctrl Pts',(6.57266211790494,4.7774711202026,6.61724465829791));
#180020=CARTESIAN_POINT('Ctrl Pts',(6.61157640712332,4.72347065147373,6.61464113603285));
#180021=CARTESIAN_POINT('Ctrl Pts',(6.68119531416642,4.6243158944227,6.60989444328971));
#180022=CARTESIAN_POINT('Ctrl Pts',(6.71211666789849,4.57931852238201,6.60775275845275));
#180023=CARTESIAN_POINT('Ctrl Pts',(6.7806606895358,4.47738593186195,6.60292728369555));
#180024=CARTESIAN_POINT('Ctrl Pts',(6.81802428594229,4.42028154687014,6.60024195024954));
#180025=CARTESIAN_POINT('Ctrl Pts',(6.93068741383284,4.24326605037025,6.59196911941288));
#180026=CARTESIAN_POINT('Ctrl Pts',(7.00357515034894,4.12185267120524,6.5863657564496));
#180027=CARTESIAN_POINT('Ctrl Pts',(7.13877674625197,3.88269005900418,6.57545219426951));
#180028=CARTESIAN_POINT('Ctrl Pts',(7.20144151866026,3.76518993752006,6.5701461306324));
#180029=CARTESIAN_POINT('Ctrl Pts',(7.39781159943072,3.37413100157306,6.55266714804397));
#180030=CARTESIAN_POINT('Ctrl Pts',(7.51903306928777,3.09459498170755,6.54044844891182));
#180031=CARTESIAN_POINT('Ctrl Pts',(7.64656428269432,2.74843534593787,6.52574662935895));
#180032=CARTESIAN_POINT('Ctrl Pts',(7.66812658004269,2.68768989865309,6.52318263928415));
#180033=CARTESIAN_POINT('Ctrl Pts',(7.71296085907612,2.55644920807708,6.51768042639647));
#180034=CARTESIAN_POINT('Ctrl Pts',(7.73599424129968,2.48587831419442,6.51474465795376));
#180035=CARTESIAN_POINT('Ctrl Pts',(7.76661079117959,2.38752435064765,6.51068827575413));
#180036=CARTESIAN_POINT('Ctrl Pts',(7.77501807843115,2.36000203302036,6.50955697749339));
#180037=CARTESIAN_POINT('Ctrl Pts',(7.78910994264862,2.31297783533513,6.50763080211099));
#180038=CARTESIAN_POINT('Ctrl Pts',(7.79486791673719,2.29349827328752,6.5068348590345));
#180039=CARTESIAN_POINT('Ctrl Pts',(7.80568970057907,2.2563760230479,6.50532188057857));
#180040=CARTESIAN_POINT('Ctrl Pts',(7.81076689172109,2.23873737331282,6.50460464626402));
#180041=CARTESIAN_POINT('Ctrl Pts',(7.82503322855306,2.18853543035179,6.50256806908899));
#180042=CARTESIAN_POINT('Ctrl Pts',(7.8340788150833,2.15593169951779,6.50125103362099));
#180043=CARTESIAN_POINT('Ctrl Pts',(7.8886509379055,1.95435377673246,6.49313938982417));
#180044=CARTESIAN_POINT('Ctrl Pts',(7.92891277239194,1.78399997108743,6.48641778450668));
#180045=CARTESIAN_POINT('Ctrl Pts',(8.01352897698686,1.36610069993303,6.47008156455319));
#180046=CARTESIAN_POINT('Ctrl Pts',(8.05195484632911,1.11754224131128,6.4604901689047));
#180047=CARTESIAN_POINT('Ctrl Pts',(8.08901348025839,0.772466144738703,
6.44714064034087));
#180048=CARTESIAN_POINT('Ctrl Pts',(8.09754913961777,0.677156404271413,
6.44345074189368));
#180049=CARTESIAN_POINT('Ctrl Pts',(8.10975373398638,0.507124178290068,
6.43685352159689));
#180050=CARTESIAN_POINT('Ctrl Pts',(8.11407783103944,0.432459727183408,
6.43395163544928));
#180051=CARTESIAN_POINT('Ctrl Pts',(8.11916750736217,0.31697352879727,6.42945271224466));
#180052=CARTESIAN_POINT('Ctrl Pts',(8.12065721446378,0.276187652715635,
6.42786183699706));
#180053=CARTESIAN_POINT('Ctrl Pts',(8.12285490345266,0.200359892209235,
6.42489998955969));
#180054=CARTESIAN_POINT('Ctrl Pts',(8.12364356278413,0.165321273295582,
6.42352973111424));
#180055=CARTESIAN_POINT('Ctrl Pts',(8.1249006836545,0.0869269813255745,
6.42046003758502));
#180056=CARTESIAN_POINT('Ctrl Pts',(8.12524885851972,0.0435704858206847,
6.41875963865154));
#180057=CARTESIAN_POINT('Ctrl Pts',(8.12525232991186,-0.0886077110125687,
6.4135671185659));
#180058=CARTESIAN_POINT('Ctrl Pts',(8.12379824240537,-0.177422407388084,
6.41006615265063));
#180059=CARTESIAN_POINT('Ctrl Pts',(8.11682034707346,-0.390299132962066,
6.40164541196985));
#180060=CARTESIAN_POINT('Ctrl Pts',(8.10990803241573,-0.514293045013356,
6.39671642998146));
#180061=CARTESIAN_POINT('Ctrl Pts',(8.08878601781311,-0.782428510927059,
6.38601217876998));
#180062=CARTESIAN_POINT('Ctrl Pts',(8.07355855089664,-0.926447934362717,
6.38023404808976));
#180063=CARTESIAN_POINT('Ctrl Pts',(8.03214735229637,-1.23817823809826,
6.36769357498648));
#180064=CARTESIAN_POINT('Ctrl Pts',(8.00454069269799,-1.40563347901672,
6.36093538142092));
#180065=CARTESIAN_POINT('Ctrl Pts',(7.96508484775443,-1.60570354945919,
6.35287829542204));
#180066=CARTESIAN_POINT('Ctrl Pts',(7.95824592922307,-1.63926271979714,
6.35152746725958));
#180067=CARTESIAN_POINT('Ctrl Pts',(7.94737705343012,-1.69092562092554,
6.34944949725413));
#180068=CARTESIAN_POINT('Ctrl Pts',(7.94349696303247,-1.70906041019681,
6.34872038492125));
#180069=CARTESIAN_POINT('Ctrl Pts',(7.93600915400054,-1.74348056829766,
6.34733720531024));
#180070=CARTESIAN_POINT('Ctrl Pts',(7.93241330782144,-1.75976842238526,
6.34668296887366));
#180071=CARTESIAN_POINT('Ctrl Pts',(7.92353739585709,-1.79939300175523,
6.34509219263836));
#180072=CARTESIAN_POINT('Ctrl Pts',(7.91820434942849,-1.82271773045062,
6.34415649319395));
#180073=CARTESIAN_POINT('Ctrl Pts',(7.89986991021914,-1.90130641229966,
6.34100571826802));
#180074=CARTESIAN_POINT('Ctrl Pts',(7.88639230614848,-1.95645780314268,
6.33879776999435));
#180075=CARTESIAN_POINT('Ctrl Pts',(7.85210127511134,-2.09066384317768,
6.33342832649012));
#180076=CARTESIAN_POINT('Ctrl Pts',(7.83067064544867,-2.16955459697653,
6.33027487996843));
#180077=CARTESIAN_POINT('Ctrl Pts',(7.69761994025812,-2.63166163046686,
6.31178984219167));
#180078=CARTESIAN_POINT('Ctrl Pts',(7.55907402456714,-3.00655981756993,
6.29672429453929));
#180079=CARTESIAN_POINT('Ctrl Pts',(7.22927055340681,-3.73017709404831,
6.26648240530952));
#180080=CARTESIAN_POINT('Ctrl Pts',(7.0388702101042,-4.0780964977272,6.25134483720988));
#180081=CARTESIAN_POINT('Ctrl Pts',(6.78407955916589,-4.47228386014423,
6.23311409154311));
#180082=CARTESIAN_POINT('Ctrl Pts',(6.74346606891664,-4.53329060259494,
6.23026059779853));
#180083=CARTESIAN_POINT('Ctrl Pts',(6.67775340821961,-4.62916204609271,
6.22572361506056));
#180084=CARTESIAN_POINT('Ctrl Pts',(6.65319340791715,-4.66439163137536,
6.22404490304277));
#180085=CARTESIAN_POINT('Ctrl Pts',(6.60665046153806,-4.73003864165022,
6.22089478824505));
#180086=CARTESIAN_POINT('Ctrl Pts',(6.58473380664365,-4.76050171281416,
6.21942398551053));
#180087=CARTESIAN_POINT('Ctrl Pts',(6.53496280221221,-4.82867962352841,
6.21611169725738));
#180088=CARTESIAN_POINT('Ctrl Pts',(6.50699148376161,-4.86630738279328,
6.21426928946835));
#180089=CARTESIAN_POINT('Ctrl Pts',(6.42101029709143,-4.97990467058126,
6.20866289566927));
#180090=CARTESIAN_POINT('Ctrl Pts',(6.36198435342906,-5.05509433177263,
6.20489113107061));
#180091=CARTESIAN_POINT('Ctrl Pts',(6.05011725604874,-5.4382469709654,6.18534947580899));
#180092=CARTESIAN_POINT('Ctrl Pts',(5.77620356263925,-5.72834277345652,
6.16952276348681));
#180093=CARTESIAN_POINT('Ctrl Pts',(5.0645170486095,-6.37890855708647,6.13027338027674));
#180094=CARTESIAN_POINT('Ctrl Pts',(4.60819705605136,-6.71597053437957,
6.10639126153788));
#180095=CARTESIAN_POINT('Ctrl Pts',(3.84816781490912,-7.16318486787771,
6.06909059857595));
#180096=CARTESIAN_POINT('Ctrl Pts',(3.5665918704455,-7.30746514284052,6.05577989717409));
#180097=CARTESIAN_POINT('Ctrl Pts',(3.21325917657124,-7.4632134002591,6.04014392924312));
#180098=CARTESIAN_POINT('Ctrl Pts',(3.14883451750185,-7.49062282482243,
6.03733543806319));
#180099=CARTESIAN_POINT('Ctrl Pts',(3.07082393472642,-7.52262804402004,
6.03399211057144));
#180100=CARTESIAN_POINT('Ctrl Pts',(3.05757083009318,-7.52802450506658,
6.03342609993361));
#180101=CARTESIAN_POINT('Ctrl Pts',(3.03586744692814,-7.53679502147722,
6.03250251552035));
#180102=CARTESIAN_POINT('Ctrl Pts',(3.0274256636631,-7.54018993148782,6.03214409601736));
#180103=CARTESIAN_POINT('Ctrl Pts',(3.01230382465039,-7.54624177404082,
6.03150354448433));
#180104=CARTESIAN_POINT('Ctrl Pts',(3.00562591907132,-7.54890403166635,
6.03122119132868));
#180105=CARTESIAN_POINT('Ctrl Pts',(2.99148086956729,-7.55452144482498,
6.03062422551331));
#180106=CARTESIAN_POINT('Ctrl Pts',(2.98401285609766,-7.55747440144834,
6.03030970612527));
#180107=CARTESIAN_POINT('Ctrl Pts',(2.96413606855629,-7.56529990471083,
6.02947434770399));
#180108=CARTESIAN_POINT('Ctrl Pts',(2.95171962795997,-7.57015300518029,
6.02895434948083));
#180109=CARTESIAN_POINT('Ctrl Pts',(2.89394677691967,-7.59257040239105,
6.02654349991929));
#180110=CARTESIAN_POINT('Ctrl Pts',(2.84844414513394,-7.60975817291452,
6.02466949191959));
#180111=CARTESIAN_POINT('Ctrl Pts',(2.44874655658326,-7.75664894937057,
6.00844180996087));
#180112=CARTESIAN_POINT('Ctrl Pts',(2.08604493589621,-7.86196049688276,
5.99529705772231));
#180113=CARTESIAN_POINT('Ctrl Pts',(1.03945584850741,-8.08827540521311,
5.95902652866962));
#180114=CARTESIAN_POINT('Ctrl Pts',(0.345643442502322,-8.14746666044795,
5.93670786753447));
#180115=CARTESIAN_POINT('Ctrl Pts',(-0.597646219634858,-8.10711503305624,
5.90278417019366));
#180116=CARTESIAN_POINT('Ctrl Pts',(-0.847387615950354,-8.08482637934851,
5.89348793007021));
#180117=CARTESIAN_POINT('Ctrl Pts',(-1.12417482889773,-8.04715756974659,
5.88273011742332));
#180118=CARTESIAN_POINT('Ctrl Pts',(-1.15263909094815,-8.0431298077382,
5.88161847649228));
#180119=CARTESIAN_POINT('Ctrl Pts',(-1.19380699916249,-8.03708142628259,
5.88000287080551));
#180120=CARTESIAN_POINT('Ctrl Pts',(-1.20652829804827,-8.03518154543719,
5.87950254765853));
#180121=CARTESIAN_POINT('Ctrl Pts',(-1.22888439551128,-8.03178845360035,
5.87862137284333));
#180122=CARTESIAN_POINT('Ctrl Pts',(-1.23852113231481,-8.03030809028723,
5.87824090939046));
#180123=CARTESIAN_POINT('Ctrl Pts',(-1.25835564662612,-8.02722462583741,
5.87745653449831));
#180124=CARTESIAN_POINT('Ctrl Pts',(-1.26855307788293,-8.02561942872277,
5.87705256042104));
#180125=CARTESIAN_POINT('Ctrl Pts',(-1.29448170544511,-8.0214873017863,
5.87602358451191));
#180126=CARTESIAN_POINT('Ctrl Pts',(-1.31020854664372,-8.01893353129054,
5.87539777364794));
#180127=CARTESIAN_POINT('Ctrl Pts',(-1.3730919341761,-8.00853241381991,
5.87288867097006));
#180128=CARTESIAN_POINT('Ctrl Pts',(-1.4201858728081,-8.00031529844626,
5.87099423424373));
#180129=CARTESIAN_POINT('Ctrl Pts',(-1.72303468425219,-7.94471486958922,
5.85871123342657));
#180130=CARTESIAN_POINT('Ctrl Pts',(-1.97644567524322,-7.88549239591398,
5.84796478218518));
#180131=CARTESIAN_POINT('Ctrl Pts',(-2.59163390453521,-7.71020201346001,
5.82074546388056));
#180132=CARTESIAN_POINT('Ctrl Pts',(-2.9489396503776,-7.58073237732512,
5.80392948868379));
#180133=CARTESIAN_POINT('Ctrl Pts',(-3.68546763559995,-7.25387480309033,
5.76780109843996));
#180134=CARTESIAN_POINT('Ctrl Pts',(-4.06086922836336,-7.0505836638282,
5.74849142393269));
#180135=CARTESIAN_POINT('Ctrl Pts',(-4.60862968298228,-6.69563276166751,
5.72031328829264));
#180136=CARTESIAN_POINT('Ctrl Pts',(-4.7934564059013,-6.56458450353027,
5.71082429191021));
#180137=CARTESIAN_POINT('Ctrl Pts',(-4.98768420393661,-6.41428545528504,
5.70101965103718));
#180138=CARTESIAN_POINT('Ctrl Pts',(-5.00273301871611,-6.40255526895245,
5.70026075932994));
#180139=CARTESIAN_POINT('Ctrl Pts',(-5.02534892617591,-6.38479829813846,
5.69912123422882));
#180140=CARTESIAN_POINT('Ctrl Pts',(-5.03294673870893,-6.37881088166991,
5.6987385759128));
#180141=CARTESIAN_POINT('Ctrl Pts',(-5.04609027587779,-6.36841508369905,
5.6980768670434));
#180142=CARTESIAN_POINT('Ctrl Pts',(-5.05164095092335,-6.3640129991996,
5.69779749869067));
#180143=CARTESIAN_POINT('Ctrl Pts',(-5.06315734618847,-6.35485510907926,
5.69721802314798));
#180144=CARTESIAN_POINT('Ctrl Pts',(-5.06912214064605,-6.35009814832334,
5.69691797413697));
#180145=CARTESIAN_POINT('Ctrl Pts',(-5.08311297686504,-6.33890809433681,
5.69621436626992));
#180146=CARTESIAN_POINT('Ctrl Pts',(-5.09113353112616,-6.33246813915875,
5.69581114534354));
#180147=CARTESIAN_POINT('Ctrl Pts',(-5.11716616851667,-6.311484288515,5.69450277521781));
#180148=CARTESIAN_POINT('Ctrl Pts',(-5.13512841444604,-6.29687856803288,
5.69360060702961));
#180149=CARTESIAN_POINT('Ctrl Pts',(-5.17727803395046,-6.26230496239157,
5.6914844527172));
#180150=CARTESIAN_POINT('Ctrl Pts',(-5.20141277987012,-6.24227333638913,
5.69027340893791));
#180151=CARTESIAN_POINT('Ctrl Pts',(-5.48949761964464,-6.00033461408997,
5.67581873829444));
#180152=CARTESIAN_POINT('Ctrl Pts',(-5.7391931963483,-5.76196887449449,
5.66328538900836));
#180153=CARTESIAN_POINT('Ctrl Pts',(-6.15587418725555,-5.31014766605553,
5.64114682175235));
#180154=CARTESIAN_POINT('Ctrl Pts',(-6.32876330481973,-5.1028629732481,
5.63151489822027));
#180155=CARTESIAN_POINT('Ctrl Pts',(-6.78351995582515,-4.49889000133021,
5.60419711140439));
#180156=CARTESIAN_POINT('Ctrl Pts',(-7.04053775527606,-4.08496589091026,
5.58624595265662));
#180157=CARTESIAN_POINT('Ctrl Pts',(-7.2834664003618,-3.60191204589582,
5.56543942619082));
#180158=CARTESIAN_POINT('Ctrl Pts',(-7.30744357641358,-3.55301583217703,
5.56333594000879));
#180159=CARTESIAN_POINT('Ctrl Pts',(-7.34289665984757,-3.47883983662502,
5.56014883509978));
#180160=CARTESIAN_POINT('Ctrl Pts',(-7.3547376163541,-3.45373602818275,
5.55907087582187));
#180161=CARTESIAN_POINT('Ctrl Pts',(-7.37571027162546,-3.40867528428791,
5.55713718840274));
#180162=CARTESIAN_POINT('Ctrl Pts',(-7.38489020297537,-3.3887410479115,
5.55628218241575));
#180163=CARTESIAN_POINT('Ctrl Pts',(-7.40367061626517,-3.34752060961314,
5.5545150699663));
#180164=CARTESIAN_POINT('Ctrl Pts',(-7.41326033961299,-3.32622969113096,
5.55360280443975));
#180165=CARTESIAN_POINT('Ctrl Pts',(-7.43718893031105,-3.27248638254035,
5.55130099919129));
#180166=CARTESIAN_POINT('Ctrl Pts',(-7.45140723759167,-3.23998093676556,
5.54990968780126));
#180167=CARTESIAN_POINT('Ctrl Pts',(-7.5072290452423,-3.11005172897094,
5.54435080000825));
#180168=CARTESIAN_POINT('Ctrl Pts',(-7.54713794642953,-3.01191268001567,
5.54015719238398));
#180169=CARTESIAN_POINT('Ctrl Pts',(-7.87903707971608,-2.14769227750029,
5.50322087029232));
#180170=CARTESIAN_POINT('Ctrl Pts',(-8.05541768030784,-1.34230376443491,
5.4680569872185));
#180171=CARTESIAN_POINT('Ctrl Pts',(-8.12089080699165,-0.32985724350419,
5.4254761944709));
#180172=CARTESIAN_POINT('Ctrl Pts',(-8.12646672181003,-0.134968312819105,
5.41739007952805));
#180173=CARTESIAN_POINT('Ctrl Pts',(-8.12458564705031,0.12002795536611,
5.40707588049529));
#180174=CARTESIAN_POINT('Ctrl Pts',(-8.12347574967377,0.180112734732693,
5.40466501000413));
#180175=CARTESIAN_POINT('Ctrl Pts',(-8.12128124929383,0.254319730730189,
5.40171538954389));
#180176=CARTESIAN_POINT('Ctrl Pts',(-8.1208261899965,0.268457911773179,
5.40115466960329));
#180177=CARTESIAN_POINT('Ctrl Pts',(-8.12001203901789,0.291852454346871,
5.40022898440858));
#180178=CARTESIAN_POINT('Ctrl Pts',(-8.11967403561938,0.301109490127723,
5.39986325316387));
#180179=CARTESIAN_POINT('Ctrl Pts',(-8.11903385230963,0.317856988594379,
5.39920261111447));
#180180=CARTESIAN_POINT('Ctrl Pts',(-8.11873713531192,0.325347642247356,
5.39890749711187));
#180181=CARTESIAN_POINT('Ctrl Pts',(-8.1180791467036,0.341397000374113,
5.39827599979355));
#180182=CARTESIAN_POINT('Ctrl Pts',(-8.11771470568656,0.349955571162441,
5.39793973723901));
#180183=CARTESIAN_POINT('Ctrl Pts',(-8.11668863042323,0.373187602312117,
5.39702832568894));
#180184=CARTESIAN_POINT('Ctrl Pts',(-8.11600073939201,0.387859912290294,
5.39645419731952));
#180185=CARTESIAN_POINT('Ctrl Pts',(-8.11441020355196,0.419926147981283,
5.39520278108484));
#180186=CARTESIAN_POINT('Ctrl Pts',(-8.11349140746026,0.437319229577799,
5.39452614623912));
#180187=CARTESIAN_POINT('Ctrl Pts',(-8.08954533061119,0.864543708153112,
5.37796079832828));
#180188=CARTESIAN_POINT('Ctrl Pts',(-8.03555058516449,1.27204805710462,
5.36356684083488));
#180189=CARTESIAN_POINT('Ctrl Pts',(-7.87146529600756,2.05153295490933,
5.33643141259876));
#180190=CARTESIAN_POINT('Ctrl Pts',(-7.76510698738187,2.42319439503791,
5.32365072200401));
#180191=CARTESIAN_POINT('Ctrl Pts',(-7.45808207833201,3.26437629369158,
5.29309941169533));
#180192=CARTESIAN_POINT('Ctrl Pts',(-7.23885078118004,3.72533384370265,
5.27505788615528));
#180193=CARTESIAN_POINT('Ctrl Pts',(-6.96138661896661,4.1904446429482,5.25423394023942));
#180194=CARTESIAN_POINT('Ctrl Pts',(-6.94468076830957,4.21807289675835,
5.25298690382023));
#180195=CARTESIAN_POINT('Ctrl Pts',(-6.92121703811957,4.25636012545102,
5.25124453064633));
#180196=CARTESIAN_POINT('Ctrl Pts',(-6.91459823148122,4.26710418220342,
5.25075402213369));
#180197=CARTESIAN_POINT('Ctrl Pts',(-6.90314850834073,4.28559348986726,
5.24990719318394));
#180198=CARTESIAN_POINT('Ctrl Pts',(-6.89832951125912,4.29334611253515,
5.24955128842167));
#180199=CARTESIAN_POINT('Ctrl Pts',(-6.88835007369052,4.309340481012,5.24881530979452));
#180200=CARTESIAN_POINT('Ctrl Pts',(-6.8831878828718,4.31758111531482,5.24843517505561));
#180201=CARTESIAN_POINT('Ctrl Pts',(-6.8711264303219,4.33675873880178,5.24754831809148));
#180202=CARTESIAN_POINT('Ctrl Pts',(-6.86421583651924,4.34768855000711,
5.24704119918948));
#180203=CARTESIAN_POINT('Ctrl Pts',(-6.84206604716215,4.38253625971744,
5.2454189604195));
#180204=CARTESIAN_POINT('Ctrl Pts',(-6.82672778400444,4.4063907685154,5.24430035863782));
#180205=CARTESIAN_POINT('Ctrl Pts',(-6.49992156421237,4.90884702246101,
5.22056537378684));
#180206=CARTESIAN_POINT('Ctrl Pts',(-6.1390299566808,5.35330865290066,5.19607918780533));
#180207=CARTESIAN_POINT('Ctrl Pts',(-5.4704259057323,6.0193995109578,5.1539656341846));
#180208=CARTESIAN_POINT('Ctrl Pts',(-5.18846286744886,6.26407037739234,
5.13699553120796));
#180209=CARTESIAN_POINT('Ctrl Pts',(-4.56780363947828,6.73189070104351,
5.10226249786165));
#180210=CARTESIAN_POINT('Ctrl Pts',(-4.22713812340037,6.95086991935527,
5.08461539831018));
#180211=CARTESIAN_POINT('Ctrl Pts',(-3.84785604988537,7.15642482874979,
5.0673592963047));
#180212=CARTESIAN_POINT('Ctrl Pts',(-3.82412029836396,7.1691363830802,5.06628841617375));
#180213=CARTESIAN_POINT('Ctrl Pts',(-3.79159301836404,7.18634868814052,
5.06483260021745));
#180214=CARTESIAN_POINT('Ctrl Pts',(-3.78285600005353,7.19095164553996,
5.0644427089687));
#180215=CARTESIAN_POINT('Ctrl Pts',(-3.76796439187685,7.19876239864356,
5.06378008768861));
#180216=CARTESIAN_POINT('Ctrl Pts',(-3.76181405757817,7.20197825095378,
5.06350697697769));
#180217=CARTESIAN_POINT('Ctrl Pts',(-3.74990588199596,7.20818531521317,
5.06297924628006));
#180218=CARTESIAN_POINT('Ctrl Pts',(-3.74414856567166,7.21117751693691,
5.06272458046948));
#180219=CARTESIAN_POINT('Ctrl Pts',(-3.73046953443604,7.21826600701172,
5.06212063346116));
#180220=CARTESIAN_POINT('Ctrl Pts',(-3.72254463770475,7.22235616100697,
5.06177163217249));
#180221=CARTESIAN_POINT('Ctrl Pts',(-3.69911827548553,7.23439804480659,
5.06074255917797));
#180222=CARTESIAN_POINT('Ctrl Pts',(-3.68359789515752,7.24231300341309,
5.06006412501378));
#180223=CARTESIAN_POINT('Ctrl Pts',(-3.5601255894997,7.3047808282414,5.05469247676947));
#180224=CARTESIAN_POINT('Ctrl Pts',(-3.45099010739142,7.35696853685853,
5.05009958089078));
#180225=CARTESIAN_POINT('Ctrl Pts',(-3.02101973879993,7.55090288573556,
5.03246266239784));
#180226=CARTESIAN_POINT('Ctrl Pts',(-2.69229794003966,7.67425863066218,
5.01993542762059));
#180227=CARTESIAN_POINT('Ctrl Pts',(-1.61270406842232,8.00144487814768,
4.97954131372518));
#180228=CARTESIAN_POINT('Ctrl Pts',(-0.84031410007732,8.11897324172928,
4.95118425324574));
#180229=CARTESIAN_POINT('Ctrl Pts',(0.10236826241514,8.12628913446624,4.91491667432805));
#180230=CARTESIAN_POINT('Ctrl Pts',(0.267791726187582,8.12252061476756,
4.90852397459318));
#180231=CARTESIAN_POINT('Ctrl Pts',(0.491608188638076,8.11057677420916,
4.89980637060434));
#180232=CARTESIAN_POINT('Ctrl Pts',(0.550197193736433,8.1068130126858,4.89751802596582));
#180233=CARTESIAN_POINT('Ctrl Pts',(0.644141471555606,8.09975491367764,
4.89383735157487));
#180234=CARTESIAN_POINT('Ctrl Pts',(0.679525000258183,8.09686319881122,
4.89244844177727));
#180235=CARTESIAN_POINT('Ctrl Pts',(0.75038111184046,8.09060475567301,4.88966157928532));
#180236=CARTESIAN_POINT('Ctrl Pts',(0.785852776565953,8.08723639619641,
4.88826364236603));
#180237=CARTESIAN_POINT('Ctrl Pts',(0.868243654216268,8.07886544471657,
4.88500978743938));
#180238=CARTESIAN_POINT('Ctrl Pts',(0.915143674549388,8.07368725835118,
4.88315240841811));
#180239=CARTESIAN_POINT('Ctrl Pts',(1.05558306582045,8.05694204098354,4.87757419875539));
#180240=CARTESIAN_POINT('Ctrl Pts',(1.14896853074906,8.04415575231379,4.87384306263687));
#180241=CARTESIAN_POINT('Ctrl Pts',(1.37076988736651,8.00984562814346,4.86492447764506));
#180242=CARTESIAN_POINT('Ctrl Pts',(1.49893199230972,7.98685416410106,4.85972544058036));
#180243=CARTESIAN_POINT('Ctrl Pts',(1.97290890052978,7.89001501689279,4.84031823128928));
#180244=CARTESIAN_POINT('Ctrl Pts',(2.31433922519872,7.7967002249336,4.82596878109188));
#180245=CARTESIAN_POINT('Ctrl Pts',(2.98289097917001,7.56618044286883,4.79722650145095));
#180246=CARTESIAN_POINT('Ctrl Pts',(3.30930773043352,7.42921361795735,4.78286617568901));
#180247=CARTESIAN_POINT('Ctrl Pts',(3.67411639125232,7.24730814750974,4.76664647285415));
#180248=CARTESIAN_POINT('Ctrl Pts',(3.72222598233871,7.22271697120772,4.76450413228667));
#180249=CARTESIAN_POINT('Ctrl Pts',(3.78957621870951,7.18743929959827,4.76150149796102));
#180250=CARTESIAN_POINT('Ctrl Pts',(3.8090239551273,7.17715181093442,4.76063405742896));
#180251=CARTESIAN_POINT('Ctrl Pts',(3.84482723829831,7.15802603207816,4.7590364468075));
#180252=CARTESIAN_POINT('Ctrl Pts',(3.86119465249933,7.1492103777332,4.75830586496622));
#180253=CARTESIAN_POINT('Ctrl Pts',(3.89306109876846,7.13190543436495,4.75688282963261));
#180254=CARTESIAN_POINT('Ctrl Pts',(3.90856298256548,7.12342159760816,4.75619027692029));
#180255=CARTESIAN_POINT('Ctrl Pts',(3.94650682583049,7.10249462525842,4.75449418663749));
#180256=CARTESIAN_POINT('Ctrl Pts',(3.96891778323162,7.08999560401707,4.75349161142473));
#180257=CARTESIAN_POINT('Ctrl Pts',(4.0211739101204,7.06052594744116,4.75115141356499));
#180258=CARTESIAN_POINT('Ctrl Pts',(4.0509715119971,7.0434718777822,4.74981508304263));
#180259=CARTESIAN_POINT('Ctrl Pts',(4.13928601414858,6.99218099983484,4.74584706432741));
#180260=CARTESIAN_POINT('Ctrl Pts',(4.1974836481589,6.95740001342429,4.74322247336926));
#180261=CARTESIAN_POINT('Ctrl Pts',(4.44449831574806,6.80554757911282,4.73202276886598));
#180262=CARTESIAN_POINT('Ctrl Pts',(4.62890654610473,6.68148697339444,4.7235068423513));
#180263=CARTESIAN_POINT('Ctrl Pts',(4.95638727298149,6.44110207872386,4.70787586103235));
#180264=CARTESIAN_POINT('Ctrl Pts',(5.10102979365904,6.3271687958893,4.70077625663744));
#180265=CARTESIAN_POINT('Ctrl Pts',(5.28315293130661,6.17340498692566,4.69152043902881));
#180266=CARTESIAN_POINT('Ctrl Pts',(5.32427670190291,6.13797292236906,4.68940874404883));
#180267=CARTESIAN_POINT('Ctrl Pts',(5.39231515997852,6.07815297300311,4.68587719103964));
#180268=CARTESIAN_POINT('Ctrl Pts',(5.41942697564301,6.05399187253007,4.68445972415975));
#180269=CARTESIAN_POINT('Ctrl Pts',(5.4707946460436,6.00759321835222,4.681754163444));
#180270=CARTESIAN_POINT('Ctrl Pts',(5.49507918200014,5.98538846790477,4.68046644303451));
#180271=CARTESIAN_POINT('Ctrl Pts',(5.54504320464867,5.93914309908232,4.67779882725267));
#180272=CARTESIAN_POINT('Ctrl Pts',(5.5707028042295,5.91508200701462,4.67641873018814));
#180273=CARTESIAN_POINT('Ctrl Pts',(5.66201748323369,5.82833472129175,4.67147058462562));
#180274=CARTESIAN_POINT('Ctrl Pts',(5.72677697876963,5.76471620053082,4.66789244235388));
#180275=CARTESIAN_POINT('Ctrl Pts',(5.83823466527357,5.6514902503089,4.66160992866191));
#180276=CARTESIAN_POINT('Ctrl Pts',(5.88540043062122,5.6023555550965,4.65891076108105));
#180277=CARTESIAN_POINT('Ctrl Pts',(6.14874366581022,5.32102294302209,4.64360852361233));
#180278=CARTESIAN_POINT('Ctrl Pts',(6.35179329391646,5.07691375995268,4.63089333341676));
#180279=CARTESIAN_POINT('Ctrl Pts',(6.60865141920152,4.72850714447214,4.6136562108051));
#180280=CARTESIAN_POINT('Ctrl Pts',(6.67526202607647,4.63399726782813,4.60906702635525));
#180281=CARTESIAN_POINT('Ctrl Pts',(6.75737873598373,4.51204022588916,4.60326967860078));
#180282=CARTESIAN_POINT('Ctrl Pts',(6.77477263137045,4.48588120519447,4.60203333108536));
#180283=CARTESIAN_POINT('Ctrl Pts',(6.80192954443494,4.44452116390416,4.6000902187715));
#180284=CARTESIAN_POINT('Ctrl Pts',(6.81179426605689,4.4293874048048,4.59938168554052));
#180285=CARTESIAN_POINT('Ctrl Pts',(6.8318076396895,4.39845931960947,4.59793856714897));
#180286=CARTESIAN_POINT('Ctrl Pts',(6.84195219379009,4.38266245477478,4.5972040513849));
#180287=CARTESIAN_POINT('Ctrl Pts',(6.86312212308146,4.34944448544432,4.59566472019088));
#180288=CARTESIAN_POINT('Ctrl Pts',(6.87413612886836,4.33201628497644,4.59486008754088));
#180289=CARTESIAN_POINT('Ctrl Pts',(6.90026625551849,4.29031824866774,4.59294184532809));
#180290=CARTESIAN_POINT('Ctrl Pts',(6.91532085340261,4.26601014698498,4.59182913438244));
#180291=CARTESIAN_POINT('Ctrl Pts',(6.95585665404035,4.19978004988552,4.58881170286466));
#180292=CARTESIAN_POINT('Ctrl Pts',(6.98108705254511,4.15770584059715,4.58691022677691));
#180293=CARTESIAN_POINT('Ctrl Pts',(7.06230916243994,4.01943591635763,4.58070721442079));
#180294=CARTESIAN_POINT('Ctrl Pts',(7.1167057915507,3.92231751934114,4.57642206672313));
#180295=CARTESIAN_POINT('Ctrl Pts',(7.2915260128715,3.59458078179143,4.56215110718107));
#180296=CARTESIAN_POINT('Ctrl Pts',(7.40286786778409,3.35930204235497,4.55220930235642));
#180297=CARTESIAN_POINT('Ctrl Pts',(7.59796583798547,2.89000862147893,4.53268231613359));
#180298=CARTESIAN_POINT('Ctrl Pts',(7.68265787026303,2.65668978895327,4.52311229968511));
#180299=CARTESIAN_POINT('Ctrl Pts',(7.78026824986612,2.34381319174337,4.51036639596665));
#180300=CARTESIAN_POINT('Ctrl Pts',(7.80287468792881,2.26741721694004,4.50726132353649));
#180301=CARTESIAN_POINT('Ctrl Pts',(7.83924221422636,2.13752621834267,4.50199211535184));
#180302=CARTESIAN_POINT('Ctrl Pts',(7.85358797868169,2.08420072479798,4.49983177053173));
#180303=CARTESIAN_POINT('Ctrl Pts',(7.87962932393522,1.98331234279912,4.49574956977132));
#180304=CARTESIAN_POINT('Ctrl Pts',(7.89144061056077,1.93578180702159,4.49382845729737));
#180305=CARTESIAN_POINT('Ctrl Pts',(7.92462991764106,1.79686831131078,4.48821972597953));
#180306=CARTESIAN_POINT('Ctrl Pts',(7.94485526131314,1.70521841400727,4.48452669359542));
#180307=CARTESIAN_POINT('Ctrl Pts',(7.99103232689364,1.47727294633488,4.47536113521955));
#180308=CARTESIAN_POINT('Ctrl Pts',(8.01508953984548,1.3406239431761,4.46988345684139));
#180309=CARTESIAN_POINT('Ctrl Pts',(8.05473324783536,1.07591111125145,4.45931645733786));
#180310=CARTESIAN_POINT('Ctrl Pts',(8.07079218089952,0.947958941933727,
4.4542285512639));
#180311=CARTESIAN_POINT('Ctrl Pts',(8.08859149756639,0.772419289995171,
4.44728749952557));
#180312=CARTESIAN_POINT('Ctrl Pts',(8.09296897744624,0.725118696483148,
4.44542108391337));
#180313=CARTESIAN_POINT('Ctrl Pts',(8.09998902213617,0.641255755700322,
4.44211989343702));
#180314=CARTESIAN_POINT('Ctrl Pts',(8.10279940678399,0.604708923499361,
4.44068400515952));
#180315=CARTESIAN_POINT('Ctrl Pts',(8.1089410853851,0.517089391751259,4.43724695953343));
#180316=CARTESIAN_POINT('Ctrl Pts',(8.11203731028862,0.46600178376016,4.43524734198575));
#180317=CARTESIAN_POINT('Ctrl Pts',(8.12170829110583,0.276850531843856,
4.42785506884705));
#180318=CARTESIAN_POINT('Ctrl Pts',(8.12524251661006,0.138655883878553,
4.42247614954586));
#180319=CARTESIAN_POINT('Ctrl Pts',(8.12524998812855,0.000439223138430957,
4.41709488796514));
#180320=CARTESIAN_POINT('',(8.12571492871015,-5.96162441064372E-5,2.41670257632164));
#180321=CARTESIAN_POINT('Ctrl Pts',(8.12571492871015,-5.96162441064372E-5,
2.41670257632164));
#180322=CARTESIAN_POINT('Ctrl Pts',(8.12424960426803,1.03977077379999,2.45736153240871));
#180323=CARTESIAN_POINT('Ctrl Pts',(7.66272101425109,3.43456748704045,2.55090964359126));
#180324=CARTESIAN_POINT('Ctrl Pts',(5.3892250497751,6.51729066085763,2.69734690986928));
#180325=CARTESIAN_POINT('Ctrl Pts',(0.335793904015849,8.95641601104349,
2.90890353025119));
#180326=CARTESIAN_POINT('Ctrl Pts',(-5.44841867805424,7.1057006866787,3.12046015063309));
#180327=CARTESIAN_POINT('Ctrl Pts',(-8.15520229705821,2.22234120788701,
3.332016771015));
#180328=CARTESIAN_POINT('Ctrl Pts',(-8.30012585283045,-3.35904394789357,
3.5435733913969));
#180329=CARTESIAN_POINT('Ctrl Pts',(-4.25467436631767,-7.88859242601576,
3.75513001177881));
#180330=CARTESIAN_POINT('Ctrl Pts',(1.33775837807641,-8.35032807926611,
3.96668663216071));
#180331=CARTESIAN_POINT('Ctrl Pts',(5.15483525499161,-6.72198816743905,
4.12535409744715));
#180332=CARTESIAN_POINT('Ctrl Pts',(7.60768009450967,-3.60555357023,4.2753576282403));
#180333=CARTESIAN_POINT('Ctrl Pts',(8.1240908003074,-1.12746725914049,4.37247200393799));
#180334=CARTESIAN_POINT('Ctrl Pts',(8.12456022843635,0.000454668290610622,
4.4166972245402));
#180335=CARTESIAN_POINT('Ctrl Pts',(8.12525,4.45452207025868E-13,0.416702556787629));
#180336=CARTESIAN_POINT('Ctrl Pts',(8.12524999999988,2.24624642433457,0.50470014992883));
#180337=CARTESIAN_POINT('Ctrl Pts',(7.14398562317574,4.47535249753493,0.59269774307003));
#180338=CARTESIAN_POINT('Ctrl Pts',(3.83078204044889,7.50935546634383,0.768692929352432));
#180339=CARTESIAN_POINT('Ctrl Pts',(1.52412477697697,8.29110090552146,0.856690522493633));
#180340=CARTESIAN_POINT('Ctrl Pts',(-2.95101623932604,7.89663306204409,
1.03268570877603));
#180341=CARTESIAN_POINT('Ctrl Pts',(-5.08535169588772,6.72342983085759,
1.12068330191723));
#180342=CARTESIAN_POINT('Ctrl Pts',(-7.81671694684421,3.15661951052899,
1.29667848819964));
#180343=CARTESIAN_POINT('Ctrl Pts',(-8.39290461146706,0.790229551553667,
1.38467608134084));
#180344=CARTESIAN_POINT('Ctrl Pts',(-7.60701611462464,-3.63299000730456,
1.56067126762324));
#180345=CARTESIAN_POINT('Ctrl Pts',(-6.25093680401326,-5.65606750610053,
1.64866886076444));
#180346=CARTESIAN_POINT('Ctrl Pts',(-2.45807268688511,-8.06369575488332,
1.82466404704684));
#180347=CARTESIAN_POINT('Ctrl Pts',(-0.0502299510448689,-8.42987470330086,
1.91266164018804));
#180348=CARTESIAN_POINT('Ctrl Pts',(4.28689960881039,-7.25863639434537,
2.08865682647044));
#180349=CARTESIAN_POINT('Ctrl Pts',(6.18309125557196,-5.73015646266342,
2.17665441961164));
#180350=CARTESIAN_POINT('Ctrl Pts',(7.8104963945153,-2.5864249052526,2.31533474365933));
#180351=CARTESIAN_POINT('Ctrl Pts',(8.1252402654945,-1.29379881447011,2.36601747456583));
#180352=CARTESIAN_POINT('Ctrl Pts',(8.1252499997742,-6.00202038690051E-5,
2.41670020547233));
#180353=CARTESIAN_POINT('Origin',(7.,0.,120.));
#180354=CARTESIAN_POINT('',(-7.,-8.57252759403147E-16,120.));
#180355=CARTESIAN_POINT('Origin',(0.,0.,120.));
#180356=CARTESIAN_POINT('',(-4.,-4.89858719658941E-16,120.));
#180357=CARTESIAN_POINT('Origin',(0.,0.,120.));
#180358=CARTESIAN_POINT('Origin',(0.,0.,140.));
#180359=CARTESIAN_POINT('',(-10.,-1.22464679914735E-15,160.));
#180360=CARTESIAN_POINT('',(-8.5,-1.04094977927525E-15,140.));
#180361=CARTESIAN_POINT('Origin',(0.,0.,160.));
#180362=CARTESIAN_POINT('Origin',(4.,16.,160.));
#180363=CARTESIAN_POINT('',(4.,16.,160.));
#180364=CARTESIAN_POINT('',(-4.,16.,160.));
#180365=CARTESIAN_POINT('',(2.,16.,160.));
#180366=CARTESIAN_POINT('',(4.,16.,0.));
#180367=CARTESIAN_POINT('',(4.,16.,160.));
#180368=CARTESIAN_POINT('',(-4.,16.,0.));
#180369=CARTESIAN_POINT('',(2.,16.,0.));
#180370=CARTESIAN_POINT('',(-4.,16.,160.));
#180371=CARTESIAN_POINT('Origin',(4.,24.,160.));
#180372=CARTESIAN_POINT('',(4.,19.5959179422654,0.));
#180373=CARTESIAN_POINT('',(4.,19.5959179422654,160.));
#180374=CARTESIAN_POINT('',(4.,19.5959179422654,0.));
#180375=CARTESIAN_POINT('',(4.,12.,0.));
#180376=CARTESIAN_POINT('',(4.,12.,160.));
#180377=CARTESIAN_POINT('Origin',(-4.,16.,160.));
#180378=CARTESIAN_POINT('',(-4.,19.5959179422654,160.));
#180379=CARTESIAN_POINT('',(-4.,19.5959179422654,0.));
#180380=CARTESIAN_POINT('',(-4.,19.5959179422654,0.));
#180381=CARTESIAN_POINT('',(-4.,8.,160.));
#180382=CARTESIAN_POINT('',(-4.,8.,0.));
#180383=CARTESIAN_POINT('Origin',(0.,0.,160.));
#180384=CARTESIAN_POINT('Origin',(0.,0.,160.));
#180385=CARTESIAN_POINT('Origin',(1.01053986535715E-15,-4.14056453134834E-16,
99.));
#180386=CARTESIAN_POINT('Ctrl Pts',(-5.31037376991249,-4.5779424402591,
99.));
#180387=CARTESIAN_POINT('Ctrl Pts',(-5.4441239624656,-4.44540070235016,
99.));
#180388=CARTESIAN_POINT('Ctrl Pts',(-5.5722612323594,-4.307542198691,98.9999999999999));
#180389=CARTESIAN_POINT('Ctrl Pts',(-5.69462771650504,-4.16482393050322,
99.));
#180390=CARTESIAN_POINT('Ctrl Pts',(-5.81894587851274,-4.01982938473437,
99.));
#180391=CARTESIAN_POINT('Ctrl Pts',(-5.93730819124591,-3.86981839507266,
99.));
#180392=CARTESIAN_POINT('Ctrl Pts',(-6.04951933541627,-3.71522500998853,
99.));
#180393=CARTESIAN_POINT('Ctrl Pts',(-6.14969329868596,-3.57721525887465,
99.));
#180394=CARTESIAN_POINT('Ctrl Pts',(-6.24496481579415,-3.43555263050148,
99.));
#180395=CARTESIAN_POINT('Ctrl Pts',(-6.33517059446557,-3.29052067230091,
99.));
#180396=CARTESIAN_POINT('Ctrl Pts',(-6.35035764256056,-3.26610308667676,
99.));
#180397=CARTESIAN_POINT('Ctrl Pts',(-6.36539986619513,-3.24159175654722,
99.));
#180398=CARTESIAN_POINT('Ctrl Pts',(-6.380290705594,-3.21699782006883,99.));
#180399=CARTESIAN_POINT('Ctrl Pts',(-6.48066943276825,-3.05121078995038,
99.));
#180400=CARTESIAN_POINT('Ctrl Pts',(-6.57424835379599,-2.88155110031512,
99.));
#180401=CARTESIAN_POINT('Ctrl Pts',(-6.66083506361849,-2.70846730956609,
99.));
#180402=CARTESIAN_POINT('Ctrl Pts',(-6.74771904956312,-2.53478927429357,
99.));
#180403=CARTESIAN_POINT('Ctrl Pts',(-6.82756318108919,-2.35766302336224,
99.));
#180404=CARTESIAN_POINT('Ctrl Pts',(-6.90013458560465,-2.17750647052253,
99.));
#180405=CARTESIAN_POINT('Ctrl Pts',(-6.94218771559863,-2.07311071042365,
99.));
#180406=CARTESIAN_POINT('Ctrl Pts',(-6.98179799933791,-1.96769679885147,
99.0000000000001));
#180407=CARTESIAN_POINT('Ctrl Pts',(-7.01891332167098,-1.86134180381851,
99.0000000000001));
#180408=CARTESIAN_POINT('Ctrl Pts',(-7.0309690691284,-1.82679572202925,
99.0000000000001));
#180409=CARTESIAN_POINT('Ctrl Pts',(-7.04276153851497,-1.79215032813677,
99.));
#180410=CARTESIAN_POINT('Ctrl Pts',(-7.05428882037421,-1.75740820588289,
99.));
#180411=CARTESIAN_POINT('Ctrl Pts',(-7.0624020809098,-1.73295561655203,
99.));
#180412=CARTESIAN_POINT('Ctrl Pts',(-7.07038375930567,-1.70845559507833,
99.));
#180413=CARTESIAN_POINT('Ctrl Pts',(-7.07822921067514,-1.68392195839963,
99.));
#180414=CARTESIAN_POINT('Ctrl Pts',(-7.09344804866636,-1.63633088627839,
99.));
#180415=CARTESIAN_POINT('Ctrl Pts',(-7.1081584504933,-1.58860089826392,
99.0000000000001));
#180416=CARTESIAN_POINT('Ctrl Pts',(-7.12235757386568,-1.54073952803008,
99.0000000000001));
#180417=CARTESIAN_POINT('Ctrl Pts',(-7.17672926898223,-1.35746738073137,
99.0000000000001));
#180418=CARTESIAN_POINT('Ctrl Pts',(-7.2236074452293,-1.17227121702206,
98.9999999999999));
#180419=CARTESIAN_POINT('Ctrl Pts',(-7.26310819089592,-0.985637740964515,
98.9999999999999));
#180420=CARTESIAN_POINT('Ctrl Pts',(-7.30356248337767,-0.794498938395065,
98.9999999999999));
#180421=CARTESIAN_POINT('Ctrl Pts',(-7.33627911130937,-0.601852048356352,
98.9999999999999));
#180422=CARTESIAN_POINT('Ctrl Pts',(-7.36133604383713,-0.40819153426746,
99.));
#180423=CARTESIAN_POINT('Ctrl Pts',(-7.38658963276242,-0.213011098336481,
99.));
#180424=CARTESIAN_POINT('Ctrl Pts',(-7.40406296219896,-0.0168003880434584,
99.));
#180425=CARTESIAN_POINT('Ctrl Pts',(-7.41378618299848,0.179953433725718,
98.9999999999999));
#180426=CARTESIAN_POINT('Ctrl Pts',(-7.42351220200831,0.376763878561074,
98.9999999999999));
#180427=CARTESIAN_POINT('Ctrl Pts',(-7.42548374008242,0.574118468878499,
98.9999999999999));
#180428=CARTESIAN_POINT('Ctrl Pts',(-7.41967984053872,0.771538034948267,
99.));
#180429=CARTESIAN_POINT('Ctrl Pts',(-7.41706251960698,0.860566171758501,
99.));
#180430=CARTESIAN_POINT('Ctrl Pts',(-7.41286325582366,0.949607569888835,
99.));
#180431=CARTESIAN_POINT('Ctrl Pts',(-7.4070766488981,1.0386182379253,99.));
#180432=CARTESIAN_POINT('Ctrl Pts',(-7.4048233678607,1.07327862750993,99.));
#180433=CARTESIAN_POINT('Ctrl Pts',(-7.40232878885474,1.1079408443067,99.));
#180434=CARTESIAN_POINT('Ctrl Pts',(-7.39959553385162,1.14256672634978,
99.));
#180435=CARTESIAN_POINT('Ctrl Pts',(-7.38373855400664,1.34344879298543,
99.));
#180436=CARTESIAN_POINT('Ctrl Pts',(-7.35984388220669,1.54328450280515,
99.0000000000001));
#180437=CARTESIAN_POINT('Ctrl Pts',(-7.32799719857053,1.74156168524455,
99.0000000000001));
#180438=CARTESIAN_POINT('Ctrl Pts',(-7.30708081276114,1.8717869260415,99.));
#180439=CARTESIAN_POINT('Ctrl Pts',(-7.28273319238425,2.00134031869882,
99.));
#180440=CARTESIAN_POINT('Ctrl Pts',(-7.25496680053308,2.13007981682335,
99.));
#180441=CARTESIAN_POINT('Ctrl Pts',(-7.21294541865853,2.32491289567739,
99.));
#180442=CARTESIAN_POINT('Ctrl Pts',(-7.16309648166436,2.51788222848557,
99.));
#180443=CARTESIAN_POINT('Ctrl Pts',(-7.10569000657273,2.70861680076425,
99.));
#180444=CARTESIAN_POINT('Ctrl Pts',(-7.04776212324125,2.90108376607787,
99.));
#180445=CARTESIAN_POINT('Ctrl Pts',(-6.98213864267679,3.09127581520037,
99.0000000000001));
#180446=CARTESIAN_POINT('Ctrl Pts',(-6.90904422969321,3.27880510883622,
99.0000000000001));
#180447=CARTESIAN_POINT('Ctrl Pts',(-6.83602882644324,3.46613169697206,
99.0000000000001));
#180448=CARTESIAN_POINT('Ctrl Pts',(-6.75555839763656,3.65080191536816,
99.0000000000001));
#180449=CARTESIAN_POINT('Ctrl Pts',(-6.66780748293597,3.8324131713319,99.0000000000001));
#180450=CARTESIAN_POINT('Ctrl Pts',(-6.65631659233788,3.85619497555336,
99.0000000000001));
#180451=CARTESIAN_POINT('Ctrl Pts',(-6.64470079214548,3.8799242953817,99.0000000000001));
#180452=CARTESIAN_POINT('Ctrl Pts',(-6.63296041476652,3.9036001974702,99.0000000000001));
#180453=CARTESIAN_POINT('Ctrl Pts',(-6.62357084759944,3.92253540421238,
99.0000000000001));
#180454=CARTESIAN_POINT('Ctrl Pts',(-6.61410251488555,3.94143453716387,
99.0000000000001));
#180455=CARTESIAN_POINT('Ctrl Pts',(-6.60455977814979,3.96028910061425,
99.0000000000001));
#180456=CARTESIAN_POINT('Ctrl Pts',(-6.5121376073237,4.14289706018757,99.0000000000001));
#180457=CARTESIAN_POINT('Ctrl Pts',(-6.4126341111438,4.32154027408393,99.0000000000001));
#180458=CARTESIAN_POINT('Ctrl Pts',(-6.30635263066292,4.4958407175706,99.0000000000001));
#180459=CARTESIAN_POINT('Ctrl Pts',(-6.19486933451546,4.67867208077645,
99.0000000000001));
#180460=CARTESIAN_POINT('Ctrl Pts',(-6.07592850174037,4.85672597420854,
99.));
#180461=CARTESIAN_POINT('Ctrl Pts',(-5.94982020079738,5.0295555387748,99.));
#180462=CARTESIAN_POINT('Ctrl Pts',(-5.8237118998544,5.20238510334106,99.));
#180463=CARTESIAN_POINT('Ctrl Pts',(-5.69043581377082,5.36999112631312,
99.));
#180464=CARTESIAN_POINT('Ctrl Pts',(-5.55022529123391,5.53190436285328,
99.));
#180465=CARTESIAN_POINT('Ctrl Pts',(-5.41582967601333,5.68710262218101,
99.));
#180466=CARTESIAN_POINT('Ctrl Pts',(-5.27506221971937,5.83707093675673,
99.));
#180467=CARTESIAN_POINT('Ctrl Pts',(-5.12835296435508,5.9815326016203,99.));
#180468=CARTESIAN_POINT('Ctrl Pts',(-5.02818687131797,6.08016414689722,
99.));
#180469=CARTESIAN_POINT('Ctrl Pts',(-4.92525007450858,6.17622815003104,
99.));
#180470=CARTESIAN_POINT('Ctrl Pts',(-4.81966940361318,6.26962688161364,
99.));
#180471=CARTESIAN_POINT('Ctrl Pts',(-4.79262515876311,6.29355075086131,
98.9999999999999));
#180472=CARTESIAN_POINT('Ctrl Pts',(-4.76540395473991,6.31730253980657,
99.));
#180473=CARTESIAN_POINT('Ctrl Pts',(-4.73803536116702,6.34085724026832,
99.));
#180474=CARTESIAN_POINT('Ctrl Pts',(-4.58135254906828,6.47570584681658,
99.));
#180475=CARTESIAN_POINT('Ctrl Pts',(-4.41966754978226,6.60425479419713,
99.));
#180476=CARTESIAN_POINT('Ctrl Pts',(-4.2534808509546,6.72628759081721,99.));
#180477=CARTESIAN_POINT('Ctrl Pts',(-4.08406266016045,6.85069330900507,
98.9999999999999));
#180478=CARTESIAN_POINT('Ctrl Pts',(-3.90996557742534,6.96832754417173,
98.9999999999999));
#180479=CARTESIAN_POINT('Ctrl Pts',(-3.73167391547189,7.07893251890552,
98.9999999999999));
#180480=CARTESIAN_POINT('Ctrl Pts',(-3.55289453959222,7.18984005173932,
99.));
#180481=CARTESIAN_POINT('Ctrl Pts',(-3.36989703671833,7.29368031139852,
98.9999999999999));
#180482=CARTESIAN_POINT('Ctrl Pts',(-3.18313162493484,7.39015734245661,
98.9999999999999));
#180483=CARTESIAN_POINT('Ctrl Pts',(-2.99809644729706,7.48574058996121,
98.9999999999999));
#180484=CARTESIAN_POINT('Ctrl Pts',(-2.80936223503177,7.57409682111926,
99.));
#180485=CARTESIAN_POINT('Ctrl Pts',(-2.61733841546728,7.65489620503951,
99.));
#180486=CARTESIAN_POINT('Ctrl Pts',(-2.51411760901224,7.69832924156714,
99.));
#180487=CARTESIAN_POINT('Ctrl Pts',(-2.40994583401986,7.73957796042281,
99.));
#180488=CARTESIAN_POINT('Ctrl Pts',(-2.30488418583278,7.77858539180664,
99.));
#180489=CARTESIAN_POINT('Ctrl Pts',(-2.23787782486739,7.80346360448216,
99.));
#180490=CARTESIAN_POINT('Ctrl Pts',(-2.17050946251637,7.82743005065559,
99.));
#180491=CARTESIAN_POINT('Ctrl Pts',(-2.10279483963357,7.85048474619616,
98.9999999999999));
#180492=CARTESIAN_POINT('Ctrl Pts',(2.10208451021631,7.8486258844723,99.));
#180493=CARTESIAN_POINT('Ctrl Pts',(2.30190062853963,7.78030966332679,99.));
#180494=CARTESIAN_POINT('Ctrl Pts',(2.49875490991879,7.70414622796948,99.));
#180495=CARTESIAN_POINT('Ctrl Pts',(2.69224761706191,7.62041821762084,99.));
#180496=CARTESIAN_POINT('Ctrl Pts',(2.88624622343728,7.53647129495876,99.));
#180497=CARTESIAN_POINT('Ctrl Pts',(3.07686623436583,7.44491978320085,99.));
#180498=CARTESIAN_POINT('Ctrl Pts',(3.2636773692486,7.34600421877401,99.));
#180499=CARTESIAN_POINT('Ctrl Pts',(3.36420325946888,7.29277626115312,99.));
#180500=CARTESIAN_POINT('Ctrl Pts',(3.46362570021794,7.23741518831547,99.));
#180501=CARTESIAN_POINT('Ctrl Pts',(3.56187347705617,7.1799538143239,99.));
#180502=CARTESIAN_POINT('Ctrl Pts',(3.60872217996291,7.1525537964774,99.));
#180503=CARTESIAN_POINT('Ctrl Pts',(3.65530374284034,7.12467617000491,99.));
#180504=CARTESIAN_POINT('Ctrl Pts',(3.70161017699924,7.09632425594086,99.));
#180505=CARTESIAN_POINT('Ctrl Pts',(3.73919757890556,7.07331071995833,99.));
#180506=CARTESIAN_POINT('Ctrl Pts',(3.7766037026839,7.04998468560165,99.));
#180507=CARTESIAN_POINT('Ctrl Pts',(3.81382418637943,7.02634785912935,99.));
#180508=CARTESIAN_POINT('Ctrl Pts',(3.83950955773068,7.01003639282833,99.));
#180509=CARTESIAN_POINT('Ctrl Pts',(3.86509847400006,6.99358202542449,99.));
#180510=CARTESIAN_POINT('Ctrl Pts',(3.89058870562973,6.97698620639156,99.));
#180511=CARTESIAN_POINT('Ctrl Pts',(4.06559275533802,6.86304704800397,99.));
#180512=CARTESIAN_POINT('Ctrl Pts',(4.23596366333074,6.74243376712933,99.0000000000001));
#180513=CARTESIAN_POINT('Ctrl Pts',(4.40128720552182,6.61538533541099,99.));
#180514=CARTESIAN_POINT('Ctrl Pts',(4.56468155565826,6.48981945615782,99.));
#180515=CARTESIAN_POINT('Ctrl Pts',(4.72314610040225,6.35796726953965,99.));
#180516=CARTESIAN_POINT('Ctrl Pts',(4.87624397923126,6.2200250828707,99.));
#180517=CARTESIAN_POINT('Ctrl Pts',(4.9694927706806,6.13600731400844,99.));
#180518=CARTESIAN_POINT('Ctrl Pts',(5.06074989929111,6.04972965074367,99.));
#180519=CARTESIAN_POINT('Ctrl Pts',(5.14990873179672,5.96123116898666,99.));
#180520=CARTESIAN_POINT('Ctrl Pts',(5.18053035147137,5.93083634691477,98.9999999999999));
#180521=CARTESIAN_POINT('Ctrl Pts',(5.21090440419704,5.90017952976678,98.9999999999999));
#180522=CARTESIAN_POINT('Ctrl Pts',(5.24102638922979,5.86926220478056,99.));
#180523=CARTESIAN_POINT('Ctrl Pts',(5.26128721225004,5.84846641562109,99.));
#180524=CARTESIAN_POINT('Ctrl Pts',(5.28143496446116,5.82755166573488,99.));
#180525=CARTESIAN_POINT('Ctrl Pts',(5.30145552672904,5.80653198951449,99.));
#180526=CARTESIAN_POINT('Ctrl Pts',(5.33795501899862,5.76821101233864,99.));
#180527=CARTESIAN_POINT('Ctrl Pts',(5.37404154619558,5.72953138765668,98.9999999999999));
#180528=CARTESIAN_POINT('Ctrl Pts',(5.40970872589704,5.6904972373425,98.9999999999999));
#180529=CARTESIAN_POINT('Ctrl Pts',(5.54691998828725,5.54033327468093,98.9999999999999));
#180530=CARTESIAN_POINT('Ctrl Pts',(5.6779283030564,5.38492524438802,99.));
#180531=CARTESIAN_POINT('Ctrl Pts',(5.80255536908089,5.22473368313874,98.9999999999999));
#180532=CARTESIAN_POINT('Ctrl Pts',(5.92854010608881,5.06279701593907,98.9999999999999));
#180533=CARTESIAN_POINT('Ctrl Pts',(6.04800416329334,4.89597139565613,98.9999999999999));
#180534=CARTESIAN_POINT('Ctrl Pts',(6.1607195382386,4.72470292325923,98.9999999999999));
#180535=CARTESIAN_POINT('Ctrl Pts',(6.27313238497297,4.55389413566188,98.9999999999999));
#180536=CARTESIAN_POINT('Ctrl Pts',(6.37883299157331,4.37866563188071,98.9999999999999));
#180537=CARTESIAN_POINT('Ctrl Pts',(6.47754731264676,4.19944056913079,98.9999999999999));
#180538=CARTESIAN_POINT('Ctrl Pts',(6.57481450704896,4.02284289991042,98.9999999999999));
#180539=CARTESIAN_POINT('Ctrl Pts',(6.66529890074785,3.84236434123862,98.9999999999999));
#180540=CARTESIAN_POINT('Ctrl Pts',(6.7486888561583,3.65840077965049,98.9999999999999));
#180541=CARTESIAN_POINT('Ctrl Pts',(6.78704586559754,3.57378276980052,98.9999999999999));
#180542=CARTESIAN_POINT('Ctrl Pts',(6.82390116975331,3.48842735837073,98.9999999999999));
#180543=CARTESIAN_POINT('Ctrl Pts',(6.85922070921012,3.40237299082903,98.9999999999999));
#180544=CARTESIAN_POINT('Ctrl Pts',(6.86883102667818,3.37895791225478,98.9999999999999));
#180545=CARTESIAN_POINT('Ctrl Pts',(6.87832762775247,3.35549108616156,98.9999999999999));
#180546=CARTESIAN_POINT('Ctrl Pts',(6.88770979494492,3.33197328910791,98.9999999999999));
#180547=CARTESIAN_POINT('Ctrl Pts',(6.89678219080322,3.30923197996156,98.9999999999999));
#180548=CARTESIAN_POINT('Ctrl Pts',(6.9057443663046,3.28645104029557,98.9999999999999));
#180549=CARTESIAN_POINT('Ctrl Pts',(6.91459439792578,3.26363522828114,98.9999999999999));
#180550=CARTESIAN_POINT('Ctrl Pts',(6.98724898062089,3.07632817993211,98.9999999999999));
#180551=CARTESIAN_POINT('Ctrl Pts',(7.05238393900141,2.88658602815681,98.9999999999999));
#180552=CARTESIAN_POINT('Ctrl Pts',(7.10978797891896,2.69482691931312,98.9999999999999));
#180553=CARTESIAN_POINT('Ctrl Pts',(7.14635429773413,2.57267654941297,98.9999999999999));
#180554=CARTESIAN_POINT('Ctrl Pts',(7.17978269938958,2.44970735410828,99.));
#180555=CARTESIAN_POINT('Ctrl Pts',(7.21000787802527,2.32602464360164,99.));
#180556=CARTESIAN_POINT('Ctrl Pts',(7.25759404308455,2.13130004170314,99.));
#180557=CARTESIAN_POINT('Ctrl Pts',(7.29724296889094,1.93480668573839,98.9999999999999));
#180558=CARTESIAN_POINT('Ctrl Pts',(7.3289508054908,1.73700590882653,98.9999999999999));
#180559=CARTESIAN_POINT('Ctrl Pts',(7.36047806932643,1.54033158634623,99.));
#180560=CARTESIAN_POINT('Ctrl Pts',(7.38415432922803,1.34236400852322,99.));
#180561=CARTESIAN_POINT('Ctrl Pts',(7.39992496655846,1.14356149378338,99.));
#180562=CARTESIAN_POINT('Ctrl Pts',(7.41563864782707,0.945476959432181,
99.0000000000001));
#180563=CARTESIAN_POINT('Ctrl Pts',(7.42350362986571,0.746562848109662,
99.0000000000001));
#180564=CARTESIAN_POINT('Ctrl Pts',(7.42341659129658,0.547287345855029,
99.0000000000001));
#180565=CARTESIAN_POINT('Ctrl Pts',(7.42340550747857,0.521910855612056,
99.0000000000001));
#180566=CARTESIAN_POINT('Ctrl Pts',(7.42326540537986,0.496528532433158,
99.0000000000001));
#180567=CARTESIAN_POINT('Ctrl Pts',(7.42299601492983,0.471141368953221,
99.0000000000001));
#180568=CARTESIAN_POINT('Ctrl Pts',(7.42274491984217,0.44747834734576,99.0000000000001));
#180569=CARTESIAN_POINT('Ctrl Pts',(7.42238158447833,0.423819981672156,
99.0000000000001));
#180570=CARTESIAN_POINT('Ctrl Pts',(7.42190613018156,0.400170373528206,
99.0000000000001));
#180571=CARTESIAN_POINT('Ctrl Pts',(7.41795192148876,0.203483779803561,
99.0000000000001));
#180572=CARTESIAN_POINT('Ctrl Pts',(7.4062462526585,0.00732774803814901,
99.0000000000001));
#180573=CARTESIAN_POINT('Ctrl Pts',(7.38680961699137,-0.187863192996554,
99.0000000000001));
#180574=CARTESIAN_POINT('Ctrl Pts',(7.36725247120289,-0.384264347794748,
99.0000000000001));
#180575=CARTESIAN_POINT('Ctrl Pts',(7.3398681641559,-0.579689108817622,
99.0000000000001));
#180576=CARTESIAN_POINT('Ctrl Pts',(7.30462493342045,-0.77368649553837,
99.0000000000001));
#180577=CARTESIAN_POINT('Ctrl Pts',(7.2693817026849,-0.967683882260041,
99.0000000000001));
#180578=CARTESIAN_POINT('Ctrl Pts',(7.22627947325658,-1.16025458134264,
99.0000000000001));
#180579=CARTESIAN_POINT('Ctrl Pts',(7.17523488235393,-1.35092889850015,
99.0000000000001));
#180580=CARTESIAN_POINT('Ctrl Pts',(7.1298757765253,-1.52036539270661,99.0000000000001));
#180581=CARTESIAN_POINT('Ctrl Pts',(7.07824390585094,-1.68830450180102,
99.0000000000001));
#180582=CARTESIAN_POINT('Ctrl Pts',(7.02047627612835,-1.85438726839183,
99.));
#180583=CARTESIAN_POINT('Ctrl Pts',(6.99159246126706,-1.93742865168724,
99.));
#180584=CARTESIAN_POINT('Ctrl Pts',(6.96117429436383,-2.02000562832631,
99.));
#180585=CARTESIAN_POINT('Ctrl Pts',(6.92923657396901,-2.10207115808548,
99.));
#180586=CARTESIAN_POINT('Ctrl Pts',(6.9132677137716,-2.14310392296506,99.));
#180587=CARTESIAN_POINT('Ctrl Pts',(6.8969189421459,-2.18400880153455,99.));
#180588=CARTESIAN_POINT('Ctrl Pts',(6.88019197511766,-2.22477975857366,
99.));
#180589=CARTESIAN_POINT('Ctrl Pts',(6.86909426420502,-2.25182974881326,
99.));
#180590=CARTESIAN_POINT('Ctrl Pts',(6.85782907052836,-2.27882315355165,
99.));
#180591=CARTESIAN_POINT('Ctrl Pts',(6.84640004100657,-2.30575073479,99.));
#180592=CARTESIAN_POINT('Ctrl Pts',(6.84060272525045,-2.31940961026055,
99.));
#180593=CARTESIAN_POINT('Ctrl Pts',(6.83476365407463,-2.33305061289471,
99.));
#180594=CARTESIAN_POINT('Ctrl Pts',(6.82888422386179,-2.34667057652511,
99.));
#180595=CARTESIAN_POINT('Ctrl Pts',(6.75258519374973,-2.52342069984376,
99.));
#180596=CARTESIAN_POINT('Ctrl Pts',(6.66941539803663,-2.69681260533179,
99.));
#180597=CARTESIAN_POINT('Ctrl Pts',(6.57963636685594,-2.86641735240571,
99.));
#180598=CARTESIAN_POINT('Ctrl Pts',(6.48992260889698,-3.03589878952498,
98.9999999999999));
#180599=CARTESIAN_POINT('Ctrl Pts',(6.39360879097073,-3.20159920820404,
99.));
#180600=CARTESIAN_POINT('Ctrl Pts',(6.29091200366129,-3.36306354964613,
99.));
#180601=CARTESIAN_POINT('Ctrl Pts',(6.18918516724972,-3.52300289223437,
98.9999999999999));
#180602=CARTESIAN_POINT('Ctrl Pts',(6.08119490995241,-3.67878634959697,
98.9999999999999));
#180603=CARTESIAN_POINT('Ctrl Pts',(5.96711584560785,-3.82993631724309,
98.9999999999999));
#180604=CARTESIAN_POINT('Ctrl Pts',(5.85555853856988,-3.97774506240029,
98.9999999999998));
#180605=CARTESIAN_POINT('Ctrl Pts',(5.73817818216436,-4.12112330181221,
98.9999999999999));
#180606=CARTESIAN_POINT('Ctrl Pts',(5.61510989546301,-4.25958363995518,
98.9999999999999));
#180607=CARTESIAN_POINT('Ctrl Pts',(5.55868785672443,-4.32306233761039,
98.9999999999999));
#180608=CARTESIAN_POINT('Ctrl Pts',(5.50106993712163,-4.38550675014418,
98.9999999999999));
#180609=CARTESIAN_POINT('Ctrl Pts',(5.44226749982611,-4.44686660289124,
98.9999999999999));
#180610=CARTESIAN_POINT('Ctrl Pts',(5.39901359961217,-4.49200168691037,
98.9999999999999));
#180611=CARTESIAN_POINT('Ctrl Pts',(5.35511875420783,-4.5365498853096,98.9999999999999));
#180612=CARTESIAN_POINT('Ctrl Pts',(5.3105951928988,-4.58050191706119,98.9999999999999));
#180613=CARTESIAN_POINT('Ctrl Pts',(-5.30378086654373,4.57361536730093,
0.00446747043563128));
#180614=CARTESIAN_POINT('Ctrl Pts',(-6.0639413951417,3.69210156778049,0.057372191261254));
#180615=CARTESIAN_POINT('Ctrl Pts',(-7.13636830945187,1.54513735705448,
0.163166067182353));
#180616=CARTESIAN_POINT('Ctrl Pts',(-7.00278762888421,-2.05811838864947,
0.321849098198928));
#180617=CARTESIAN_POINT('Ctrl Pts',(-5.17287422036016,-5.15049374409531,
0.480516563485356));
#180618=CARTESIAN_POINT('Ctrl Pts',(-2.06992536476629,-7.00586681229451,
0.639184028771785));
#180619=CARTESIAN_POINT('Ctrl Pts',(1.51099084548779,-7.1268219767527,0.797851494058213));
#180620=CARTESIAN_POINT('Ctrl Pts',(5.8549714641742,-5.04026049610657,1.00940811444012));
#180621=CARTESIAN_POINT('Ctrl Pts',(8.19966432523108,1.11131240077932,1.2738538899175));
#180622=CARTESIAN_POINT('Ctrl Pts',(4.30252989486095,6.41644447484682,1.53829966539488));
#180623=CARTESIAN_POINT('Ctrl Pts',(-0.440438479635278,7.27223127969325,
1.74985628577678));
#180624=CARTESIAN_POINT('Ctrl Pts',(-3.85933553388024,6.20169133701892,
1.90852375106322));
#180625=CARTESIAN_POINT('Ctrl Pts',(-6.35800508006661,3.58921836875176,
2.06719121634964));
#180626=CARTESIAN_POINT('Ctrl Pts',(-7.2961685757795,0.117923577904027,
2.22585868163607));
#180627=CARTESIAN_POINT('Ctrl Pts',(-6.47127337767897,-3.38407271816467,
2.3845261469225));
#180628=CARTESIAN_POINT('Ctrl Pts',(-4.05427435445179,-6.07236054551186,
2.54319361220892));
#180629=CARTESIAN_POINT('Ctrl Pts',(-0.679028220406368,-7.25757857856526,
2.70186107749536));
#180630=CARTESIAN_POINT('Ctrl Pts',(4.10468304959755,-6.54456291005896,
2.91341769787726));
#180631=CARTESIAN_POINT('Ctrl Pts',(7.32848383063627,-2.42047858723412,
3.12497431825917));
#180632=CARTESIAN_POINT('Ctrl Pts',(6.88866860112692,2.3718685787921,3.33653093864107));
#180633=CARTESIAN_POINT('Ctrl Pts',(4.28490662509515,6.4190526417461,3.54808755902298));
#180634=CARTESIAN_POINT('Ctrl Pts',(-0.794465437437627,7.68440215608013,
3.75964417940489));
#180635=CARTESIAN_POINT('Ctrl Pts',(-5.00317805612076,5.30101957579333,
3.97120079978678));
#180636=CARTESIAN_POINT('Ctrl Pts',(-6.93319317044858,2.28946327644455,
4.12986826507322));
#180637=CARTESIAN_POINT('Ctrl Pts',(-7.18305822535648,-1.31770430691025,
4.28853573035964));
#180638=CARTESIAN_POINT('Ctrl Pts',(-5.67670789282273,-4.58383194552348,
4.44720319564608));
#180639=CARTESIAN_POINT('Ctrl Pts',(-2.80114571582052,-6.74435065760599,
4.6058706609325));
#180640=CARTESIAN_POINT('Ctrl Pts',(0.777722768978429,-7.25988463091362,
4.76453812621893));
#180641=CARTESIAN_POINT('Ctrl Pts',(4.12824572376459,-6.00751555059738,
4.92320559150536));
#180642=CARTESIAN_POINT('Ctrl Pts',(7.34465462839528,-2.39523911495696,
5.13476221188726));
#180643=CARTESIAN_POINT('Ctrl Pts',(7.17759831039412,2.83667934145036,5.34631883226917));
#180644=CARTESIAN_POINT('Ctrl Pts',(3.76964374075252,6.23453863249777,5.55787545265107));
#180645=CARTESIAN_POINT('Ctrl Pts',(-0.822518600318629,7.67386017329656,
5.76943207303298));
#180646=CARTESIAN_POINT('Ctrl Pts',(-5.53318091736508,5.39119949546253,
5.98098869341488));
#180647=CARTESIAN_POINT('Ctrl Pts',(-7.23773325362757,0.86479597768524,
6.1925453137968));
#180648=CARTESIAN_POINT('Ctrl Pts',(-6.79019730453254,-2.6840267763159,
6.35121277908321));
#180649=CARTESIAN_POINT('Ctrl Pts',(-4.6710360787768,-5.61374242815181,
6.50988024436965));
#180650=CARTESIAN_POINT('Ctrl Pts',(-1.42191810959925,-7.15644284387903,
6.66854770965607));
#180651=CARTESIAN_POINT('Ctrl Pts',(2.17016344940662,-6.97302464538298,
6.8272151749425));
#180652=CARTESIAN_POINT('Ctrl Pts',(5.24835772874372,-5.07597481362461,
6.98588264022893));
#180653=CARTESIAN_POINT('Ctrl Pts',(7.01857685474314,-1.96779920245025,
7.14455010551536));
#180654=CARTESIAN_POINT('Ctrl Pts',(7.17389309592126,2.86642300166595,7.35610672589728));
#180655=CARTESIAN_POINT('Ctrl Pts',(3.6936765813652,6.77653452959824,7.56766334627916));
#180656=CARTESIAN_POINT('Ctrl Pts',(-1.09991472711457,7.20207424796267,
7.77921996666108));
#180657=CARTESIAN_POINT('Ctrl Pts',(-5.54797533933759,5.36513155035279,
7.99077658704298));
#180658=CARTESIAN_POINT('Ctrl Pts',(-7.70244879166337,0.594479258170977,
8.20233320742488));
#180659=CARTESIAN_POINT('Ctrl Pts',(-6.1112839041896,-3.97301696557823,
8.4138898278068));
#180660=CARTESIAN_POINT('Ctrl Pts',(-3.4940250724007,-6.41112844610217,
8.57255729309321));
#180661=CARTESIAN_POINT('Ctrl Pts',(0.0100858356750476,-7.30291588173751,
8.73122475837966));
#180662=CARTESIAN_POINT('Ctrl Pts',(3.49317025910466,-6.40580102964345,
8.88989222366607));
#180663=CARTESIAN_POINT('Ctrl Pts',(6.13370953241007,-3.96362075277578,
9.04855968895252));
#180664=CARTESIAN_POINT('Ctrl Pts',(7.28180167568219,-0.534923840390513,
9.20722715423893));
#180665=CARTESIAN_POINT('Ctrl Pts',(6.6496768096039,2.985708139488,9.36589461952537));
#180666=CARTESIAN_POINT('Ctrl Pts',(3.67177574156317,6.79699829926491,9.57745123990726));
#180667=CARTESIAN_POINT('Ctrl Pts',(-1.50548545536504,7.56955616019083,
9.78900786028918));
#180668=CARTESIAN_POINT('Ctrl Pts',(-5.45870349896653,4.82516756086003,
10.0005644806711));
#180669=CARTESIAN_POINT('Ctrl Pts',(-7.69710713562264,0.564985540828748,
10.212121101053));
#180670=CARTESIAN_POINT('Ctrl Pts',(-6.29491438534592,-4.47830055464201,
10.4236777214349));
#180671=CARTESIAN_POINT('Ctrl Pts',(-2.14692484031353,-6.96587169681106,
10.6352343418168));
#180672=CARTESIAN_POINT('Ctrl Pts',(1.42467490292068,-7.16108096448956,
10.7939018071032));
#180673=CARTESIAN_POINT('Ctrl Pts',(4.68652417010474,-5.60081898500879,
10.9525692723897));
#180674=CARTESIAN_POINT('Ctrl Pts',(6.78612783456425,-2.68048396813529,
11.1112367376761));
#180675=CARTESIAN_POINT('Ctrl Pts',(7.24893206726443,0.88637801416566,11.2699042029625));
#180676=CARTESIAN_POINT('Ctrl Pts',(5.93378011989064,4.25453083756337,11.428571668249));
#180677=CARTESIAN_POINT('Ctrl Pts',(3.19285241050036,6.55273593632083,11.5872391335354));
#180678=CARTESIAN_POINT('Ctrl Pts',(-1.53541180788721,7.57123725402545,
11.7987957539173));
#180679=CARTESIAN_POINT('Ctrl Pts',(-6.00554205653118,4.8474871351901,12.0103523742992));
#180680=CARTESIAN_POINT('Ctrl Pts',(-7.28262268868039,0.207587702725835,
12.2219089946811));
#180681=CARTESIAN_POINT('Ctrl Pts',(-6.27191716258512,-4.49752398818159,
12.433465615063));
#180682=CARTESIAN_POINT('Ctrl Pts',(-1.96419739535735,-7.47148255492932,
12.6450222354449));
#180683=CARTESIAN_POINT('Ctrl Pts',(2.81440621039056,-6.72396999170161,
12.8565788558268));
#180684=CARTESIAN_POINT('Ctrl Pts',(5.68179560826575,-4.58562730985399,
13.0152463211133));
#180685=CARTESIAN_POINT('Ctrl Pts',(7.18667145538097,-1.29785804008884,
13.1739137863997));
#180686=CARTESIAN_POINT('Ctrl Pts',(6.92779700763258,2.28957505042202,13.3325812516861));
#180687=CARTESIAN_POINT('Ctrl Pts',(4.9979528284151,5.32476756532605,13.4912487169725));
#180688=CARTESIAN_POINT('Ctrl Pts',(1.83027665600578,7.06830011540733,13.649916182259));
#180689=CARTESIAN_POINT('Ctrl Pts',(-1.74664355286525,7.07685601560628,
13.8085836475454));
#180690=CARTESIAN_POINT('Ctrl Pts',(-6.02959695876137,4.82960490013808,
14.0201402679273));
#180691=CARTESIAN_POINT('Ctrl Pts',(-7.7167925087142,-0.125619648347784,
14.2316968883092));
#180692=CARTESIAN_POINT('Ctrl Pts',(-5.72469512022718,-4.50639009190866,
14.4432535086911));
#180693=CARTESIAN_POINT('Ctrl Pts',(-1.93422387439583,-7.47150887855429,
14.654810129073));
#180694=CARTESIAN_POINT('Ctrl Pts',(3.27863805495107,-6.99511654521699,
14.8663667494549));
#180695=CARTESIAN_POINT('Ctrl Pts',(6.46880555178497,-3.35964425193866,
15.0779233698368));
#180696=CARTESIAN_POINT('Ctrl Pts',(7.30044898119669,0.119263707518536,
15.2365908351232));
#180697=CARTESIAN_POINT('Ctrl Pts',(6.34952905775644,3.60779196247754,15.3952583004097));
#180698=CARTESIAN_POINT('Ctrl Pts',(3.85239056755433,6.19641930517106,15.5539257656961));
#180699=CARTESIAN_POINT('Ctrl Pts',(0.426063761775362,7.29048364449936,
15.7125932309825));
#180700=CARTESIAN_POINT('Ctrl Pts',(-3.12315621384476,6.59974805753294,
15.871260696269));
#180701=CARTESIAN_POINT('Ctrl Pts',(-5.87504698961792,4.31468163786968,
16.0299281615554));
#180702=CARTESIAN_POINT('Ctrl Pts',(-7.72380553529842,-0.154761201324391,
16.2414847819373));
#180703=CARTESIAN_POINT('Ctrl Pts',(-5.84457985362868,-5.04039217255527,
16.4530414023192));
#180704=CARTESIAN_POINT('Ctrl Pts',(-1.50837888309736,-7.12772607673944,
16.6645980227011));
#180705=CARTESIAN_POINT('Ctrl Pts',(3.30166900737697,-6.97593353497041,
16.876154643083));
#180706=CARTESIAN_POINT('Ctrl Pts',(6.99896548152602,-3.2704136076266,17.0877112634649));
#180707=CARTESIAN_POINT('Ctrl Pts',(7.11927210416913,1.56480652899573,17.2992678838468));
#180708=CARTESIAN_POINT('Ctrl Pts',(5.52897756315104,4.76877198712199,17.4579353491332));
#180709=CARTESIAN_POINT('Ctrl Pts',(2.5638425465892,6.83808405155348,17.6166028144197));
#180710=CARTESIAN_POINT('Ctrl Pts',(-1.01195855279308,7.22581934301619,
17.7752702797061));
#180711=CARTESIAN_POINT('Ctrl Pts',(-4.34367742670664,5.87070255697988,
17.9339377449926));
#180712=CARTESIAN_POINT('Ctrl Pts',(-6.62628248831759,3.06645716487327,
18.092605210279));
#180713=CARTESIAN_POINT('Ctrl Pts',(-7.27524254505321,-0.451110493156939,
18.2512726755654));
#180714=CARTESIAN_POINT('Ctrl Pts',(-5.83129435071667,-5.06726051943665,
18.4628292959473));
#180715=CARTESIAN_POINT('Ctrl Pts',(-1.25830740500688,-7.61454722180532,
18.6743859163292));
#180716=CARTESIAN_POINT('Ctrl Pts',(3.40838641667838,-6.43914496766518,
18.8859425367111));
#180717=CARTESIAN_POINT('Ctrl Pts',(7.0043589337785,-3.24092931817342,19.097499157093));
#180718=CARTESIAN_POINT('Ctrl Pts',(7.46916864160391,1.97297814985943,19.3090557774749));
#180719=CARTESIAN_POINT('Ctrl Pts',(4.46374735160538,5.76260482311814,19.5206123978568));
#180720=CARTESIAN_POINT('Ctrl Pts',(1.1900032485206,7.20379562643869,19.6792798631432));
#180721=CARTESIAN_POINT('Ctrl Pts',(-2.41242090028973,6.89296072088447,
19.8379473284297));
#180722=CARTESIAN_POINT('Ctrl Pts',(-5.40638235949189,4.89975051134777,
19.9966147937161));
#180723=CARTESIAN_POINT('Ctrl Pts',(-7.09633602667786,1.7247310214306,20.1552822590025));
#180724=CARTESIAN_POINT('Ctrl Pts',(-7.05234807878063,-1.89081086698428,
20.313949724289));
#180725=CARTESIAN_POINT('Ctrl Pts',(-5.29701847508217,-5.00741949920584,
20.4726171895754));
#180726=CARTESIAN_POINT('Ctrl Pts',(-1.23089278942476,-7.62666545204941,
20.6841738099573));
#180727=CARTESIAN_POINT('Ctrl Pts',(3.91228788997283,-6.65271902191656,
20.8957304303392));
#180728=CARTESIAN_POINT('Ctrl Pts',(6.7423921741068,-2.76040461718001,21.1072870507211));
#180729=CARTESIAN_POINT('Ctrl Pts',(7.45442002495894,1.99907203724366,21.318843671103));
#180730=CARTESIAN_POINT('Ctrl Pts',(4.47089830846171,6.30017390965807,21.5304002914849));
#180731=CARTESIAN_POINT('Ctrl Pts',(-0.264617112092554,7.28441024039534,
21.7419569118668));
#180732=CARTESIAN_POINT('Ctrl Pts',(-3.70157536819359,6.29357759565806,
21.9006243771533));
#180733=CARTESIAN_POINT('Ctrl Pts',(-6.26842339864247,3.74693877654311,
22.0592918424397));
#180734=CARTESIAN_POINT('Ctrl Pts',(-7.29023306121876,0.298374267641664,
22.2179593077261));
#180735=CARTESIAN_POINT('Ctrl Pts',(-6.55365419606674,-3.22215747259312,
22.3766267730125));
#180736=CARTESIAN_POINT('Ctrl Pts',(-4.2035000142001,-5.97003909447894,
22.535294238299));
#180737=CARTESIAN_POINT('Ctrl Pts',(-0.859006836306873,-7.23842261971257,
22.6939617035854));
#180738=CARTESIAN_POINT('Ctrl Pts',(3.94110103574177,-6.64445976755199,
22.9055183239673));
#180739=CARTESIAN_POINT('Ctrl Pts',(7.26612585956124,-2.60155374951473,
23.1170749443492));
#180740=CARTESIAN_POINT('Ctrl Pts',(6.94541914943577,2.20019060961913,23.3286315647311));
#180741=CARTESIAN_POINT('Ctrl Pts',(4.44285646893537,6.31076012181081,23.540188185113));
#180742=CARTESIAN_POINT('Ctrl Pts',(-0.603532440634358,7.70174470945665,
23.7517448054949));
#180743=CARTESIAN_POINT('Ctrl Pts',(-4.87010077296144,5.42353881036995,
23.9633014258768));
#180744=CARTESIAN_POINT('Ctrl Pts',(-6.87424567478842,2.46079774903175,
24.1219688911633));
#180745=CARTESIAN_POINT('Ctrl Pts',(-7.21354498832649,-1.13905697890876,
24.2806363564497));
#180746=CARTESIAN_POINT('Ctrl Pts',(-5.78870296013593,-4.44155865995165,
24.4393038217361));
#180747=CARTESIAN_POINT('Ctrl Pts',(-2.96763823370584,-6.67276594926407,
24.5979712870226));
#180748=CARTESIAN_POINT('Ctrl Pts',(0.597336160113703,-7.27694775787263,
24.7566387523089));
#180749=CARTESIAN_POINT('Ctrl Pts',(3.97790360703269,-6.10810426069701,
24.9153062175955));
#180750=CARTESIAN_POINT('Ctrl Pts',(7.28295751464038,-2.57675237779755,
25.1268628379772));
#180751=CARTESIAN_POINT('Ctrl Pts',(7.24577773808857,2.65770048892243,25.3384194583593));
#180752=CARTESIAN_POINT('Ctrl Pts',(3.92318728070308,6.13907871268442,25.549976078741));
#180753=CARTESIAN_POINT('Ctrl Pts',(-0.631845655261499,7.69190730485788,
25.7615326991231));
#180754=CARTESIAN_POINT('Ctrl Pts',(-5.39769956561323,5.52684018005954,
25.9730893195048));
#180755=CARTESIAN_POINT('Ctrl Pts',(-7.21404553293603,1.0441272983282,26.1846459398869));
#180756=CARTESIAN_POINT('Ctrl Pts',(-6.85470811288257,-2.51470790474136,
26.3433134051732));
#180757=CARTESIAN_POINT('Ctrl Pts',(-4.80889757630427,-5.49610645825077,
26.5019808704597));
#180758=CARTESIAN_POINT('Ctrl Pts',(-1.59906073563414,-7.11895568564879,
26.6606483357461));
#180759=CARTESIAN_POINT('Ctrl Pts',(1.99646611371862,-7.02472811976266,
26.8193158010326));
#180760=CARTESIAN_POINT('Ctrl Pts',(5.1207860900796,-5.20464494260984,26.977983266319));
#180761=CARTESIAN_POINT('Ctrl Pts',(6.96758661695681,-2.14135272703788,
27.1366507316054));
#180762=CARTESIAN_POINT('Ctrl Pts',(7.24281175153932,2.68752691303849,27.3482073519873));
#180763=CARTESIAN_POINT('Ctrl Pts',(3.8606926253612,6.68279278229395,27.5597639723692));
#180764=CARTESIAN_POINT('Ctrl Pts',(-0.92086328633324,7.22714996993207,
27.7713205927511));
#180765=CARTESIAN_POINT('Ctrl Pts',(-5.41313628853642,5.50114737489633,
27.9828772131331));
#180766=CARTESIAN_POINT('Ctrl Pts',(-7.68532563280776,0.785425295142589,
28.1944338335149));
#180767=CARTESIAN_POINT('Ctrl Pts',(-6.20798885225515,-3.82014779513366,
28.4059904538969));
#180768=CARTESIAN_POINT('Ctrl Pts',(-3.65203538103778,-6.32245337939593,
28.5646579191832));
#180769=CARTESIAN_POINT('Ctrl Pts',(-0.171132320066336,-7.3009174648697,
28.7233253844697));
#180770=CARTESIAN_POINT('Ctrl Pts',(3.33314067339357,-6.49050834232939,
28.8819928497561));
#180771=CARTESIAN_POINT('Ctrl Pts',(6.03346730846092,-4.11460257346248,
29.0406603150426));
#180772=CARTESIAN_POINT('Ctrl Pts',(7.26628585314741,-0.715450249379295,
29.199327780329));
#180773=CARTESIAN_POINT('Ctrl Pts',(6.72171682947609,2.81978325953014,29.3579952456154));
#180774=CARTESIAN_POINT('Ctrl Pts',(3.83930631857236,6.70379369974286,29.5695518659973));
#180775=CARTESIAN_POINT('Ctrl Pts',(-1.31719041161547,7.60458258802853,
29.7811084863792));
#180776=CARTESIAN_POINT('Ctrl Pts',(-5.33729063949059,4.95913445165702,
29.9926651067611));
#180777=CARTESIAN_POINT('Ctrl Pts',(-7.6807174806566,0.755808111186173,
30.2042217271431));
#180778=CARTESIAN_POINT('Ctrl Pts',(-6.40410093183508,-4.32071917988325,
30.4157783475249));
#180779=CARTESIAN_POINT('Ctrl Pts',(-2.31911537984777,-6.91045285211773,
30.6273349679068));
#180780=CARTESIAN_POINT('Ctrl Pts',(1.2465406732832,-7.19422793000318,30.7860024331933));
#180781=CARTESIAN_POINT('Ctrl Pts',(4.54610201023657,-5.71538612976707,
30.9446698984797));
#180782=CARTESIAN_POINT('Ctrl Pts',(6.71752456355529,-2.84805003967788,
31.1033373637662));
#180783=CARTESIAN_POINT('Ctrl Pts',(7.26869464646612,0.70622959173733,31.2620048290525));
#180784=CARTESIAN_POINT('Ctrl Pts',(6.03752522859731,4.1059795753313,31.420672294339));
#180785=CARTESIAN_POINT('Ctrl Pts',(3.35446931300588,6.47149058521222,31.5793397596254));
#180786=CARTESIAN_POINT('Ctrl Pts',(-1.34706583454684,7.60700575876862,
31.7908963800074));
#180787=CARTESIAN_POINT('Ctrl Pts',(-5.88340697707029,4.99501644249136,
32.0024530003892));
#180788=CARTESIAN_POINT('Ctrl Pts',(-7.27522915446992,0.388235276547886,
32.2140096207711));
#180789=CARTESIAN_POINT('Ctrl Pts',(-6.38158780188008,-4.34050734885841,
32.425566241153));
#180790=CARTESIAN_POINT('Ctrl Pts',(-2.14899046180226,-7.42044223558306,
32.6371228615349));
#180791=CARTESIAN_POINT('Ctrl Pts',(2.64669056104301,-6.79173643779515,
32.8486794819169));
#180792=CARTESIAN_POINT('Ctrl Pts',(5.5662580231132,-4.72520378175531,33.0073469472032));
#180793=CARTESIAN_POINT('Ctrl Pts',(7.15225342400828,-1.47578896139418,
33.1660144124897));
#180794=CARTESIAN_POINT('Ctrl Pts',(6.98247749603769,2.11696322778769,33.3246818777761));
#180795=CARTESIAN_POINT('Ctrl Pts',(5.12854302045249,5.19910844156755,33.4833493430626));
#180796=CARTESIAN_POINT('Ctrl Pts',(2.00510636243318,7.0207070608534,33.642016808349));
#180797=CARTESIAN_POINT('Ctrl Pts',(-1.57050014739987,7.11801826728517,
33.8006842736354));
#180798=CARTESIAN_POINT('Ctrl Pts',(-5.90789820339567,4.97773661364845,
34.0122408940173));
#180799=CARTESIAN_POINT('Ctrl Pts',(-7.71753351631667,0.0659040448482104,
34.2237975143992));
#180800=CARTESIAN_POINT('Ctrl Pts',(-5.83475426225609,-4.36294952745157,
34.4353541347811));
#180801=CARTESIAN_POINT('Ctrl Pts',(-2.11902682337525,-7.42121231608519,
34.646910755163));
#180802=CARTESIAN_POINT('Ctrl Pts',(3.10405121203628,-7.07431898132942,
34.8584673755449));
#180803=CARTESIAN_POINT('Ctrl Pts',(6.38344726014795,-3.51912714224682,
35.0700239959268));
#180804=CARTESIAN_POINT('Ctrl Pts',(7.30116047104728,-0.0619268520409932,
35.2286914612133));
#180805=CARTESIAN_POINT('Ctrl Pts',(6.43709792822838,3.44912341939353,35.3873589264997));
#180806=CARTESIAN_POINT('Ctrl Pts',(4.00496272239371,6.09891784521768,35.5460263917862));
#180807=CARTESIAN_POINT('Ctrl Pts',(0.606839125529545,7.27766641002028,
35.7046938570725));
#180808=CARTESIAN_POINT('Ctrl Pts',(-2.95842794681358,6.67521409712822,
35.8633613223591));
#180809=CARTESIAN_POINT('Ctrl Pts',(-5.76617316348475,4.45913689127132,
36.0220287876453));
#180810=CARTESIAN_POINT('Ctrl Pts',(-7.72526750394771,0.0369454867507112,
36.2335854080274));
#180811=CARTESIAN_POINT('Ctrl Pts',(-5.96785284504142,-4.89381235219836,
36.4451420284092));
#180812=CARTESIAN_POINT('Ctrl Pts',(-1.68478230696053,-7.08810231713384,
36.6566986487911));
#180813=CARTESIAN_POINT('Ctrl Pts',(3.12755108137221,-7.05571336946209,
36.868255269173));
#180814=CARTESIAN_POINT('Ctrl Pts',(6.9156581202202,-3.44307939797708,37.0798118895549));
#180815=CARTESIAN_POINT('Ctrl Pts',(7.15590917899246,1.38766659843061,37.2913685099369));
#180816=CARTESIAN_POINT('Ctrl Pts',(5.64560773197196,4.63010717971896,37.4500359752233));
#180817=CARTESIAN_POINT('Ctrl Pts',(2.73273377903033,6.77235913052149,37.6087034405097));
#180818=CARTESIAN_POINT('Ctrl Pts',(-0.83234498276647,7.24870520300981,
37.7673709057962));
#180819=CARTESIAN_POINT('Ctrl Pts',(-4.19666392570441,5.97667917781288,
37.9260383710825));
#180820=CARTESIAN_POINT('Ctrl Pts',(-6.54815087122052,3.22993797567709,
38.084705836369));
#180821=CARTESIAN_POINT('Ctrl Pts',(-7.28419626503113,-0.270443226750539,
38.2433733016553));
#180822=CARTESIAN_POINT('Ctrl Pts',(-5.9552381459358,-4.92100209324613,
38.4549299220374));
#180823=CARTESIAN_POINT('Ctrl Pts',(-1.44686784289757,-7.58097885261444,
38.6664865424192));
#180824=CARTESIAN_POINT('Ctrl Pts',(3.2475555385614,-6.52173818118793,38.8780431628012));
#180825=CARTESIAN_POINT('Ctrl Pts',(6.9217815368992,-3.41373802070984,39.089599783183));
#180826=CARTESIAN_POINT('Ctrl Pts',(7.51582637584137,1.78703018014509,39.3011564035649));
#180827=CARTESIAN_POINT('Ctrl Pts',(4.60536655768288,5.65006669303687,39.5127130239469));
#180828=CARTESIAN_POINT('Ctrl Pts',(1.36839230042613,7.17204863836835,39.6713804892333));
#180829=CARTESIAN_POINT('Ctrl Pts',(-2.24063568138784,6.9507002412061,39.8300479545197));
#180830=CARTESIAN_POINT('Ctrl Pts',(-5.2831349041589,5.03239613652743,39.9887154198062));
#180831=CARTESIAN_POINT('Ctrl Pts',(-7.05135335594436,1.9002889120929,40.1473828850925));
#180832=CARTESIAN_POINT('Ctrl Pts',(-7.09709525436831,-1.71523121164749,
40.306050350379));
#180833=CARTESIAN_POINT('Ctrl Pts',(-5.41964188346313,-4.87443705687134,
40.4647178156654));
#180834=CARTESIAN_POINT('Ctrl Pts',(-1.41976237131237,-7.59377361958779,
40.6762744360474));
#180835=CARTESIAN_POINT('Ctrl Pts',(3.7460022112624,-6.74775031783296,40.8878310564292));
#180836=CARTESIAN_POINT('Ctrl Pts',(6.67181921361694,-2.92686082019938,
41.0993876768112));
#180837=CARTESIAN_POINT('Ctrl Pts',(7.50172979602892,1.81348200596779,41.310944297193));
#180838=CARTESIAN_POINT('Ctrl Pts',(4.62585458842672,6.18729280891685,41.5225009175749));
#180839=CARTESIAN_POINT('Ctrl Pts',(-0.0837797822404395,7.28873347807959,
41.7340575379569));
#180840=CARTESIAN_POINT('Ctrl Pts',(-3.54426633103808,6.38349084229388,
41.8927250032432));
#180841=CARTESIAN_POINT('Ctrl Pts',(-6.17351645534622,3.90133011617787,
42.0513924685297));
#180842=CARTESIAN_POINT('Ctrl Pts',(-7.28058439966683,0.479182731092116,
42.2100599338161));
#180843=CARTESIAN_POINT('Ctrl Pts',(-6.63159105267217,-3.05854249765599,
42.3687273991026));
#180844=CARTESIAN_POINT('Ctrl Pts',(-4.35034664277355,-5.86389488707565,
42.5273948643889));
#180845=CARTESIAN_POINT('Ctrl Pts',(-1.03835704400452,-7.21487833684687,
42.6860623296755));
#180846=CARTESIAN_POINT('Ctrl Pts',(3.77501143071734,-6.74020857799426,
42.8976189500573));
#180847=CARTESIAN_POINT('Ctrl Pts',(7.1993333690414,-2.78105482849902,43.1091755704392));
#180848=CARTESIAN_POINT('Ctrl Pts',(6.99787622017836,2.02716903286916,43.3207321908211));
#180849=CARTESIAN_POINT('Ctrl Pts',(4.59808407027556,6.19857159357774,43.532288811203));
#180850=CARTESIAN_POINT('Ctrl Pts',(-0.412234987062465,7.71434931083846,
43.743845431585));
#180851=CARTESIAN_POINT('Ctrl Pts',(-4.73402112950856,5.54271582504479,
43.9554020519668));
#180852=CARTESIAN_POINT('Ctrl Pts',(-6.81106657879855,2.63061802727325,
44.1140695172533));
#180853=CARTESIAN_POINT('Ctrl Pts',(-7.23958845831873,-0.959708849175259,
44.2727369825396));
#180854=CARTESIAN_POINT('Ctrl Pts',(-5.89713365859142,-4.29654976458308,
44.4314044478262));
#180855=CARTESIAN_POINT('Ctrl Pts',(-3.13230292181754,-6.59707211633677,
44.5900719131126));
#180856=CARTESIAN_POINT('Ctrl Pts',(0.416581565586644,-7.28952941102346,
44.748739378399));
#180857=CARTESIAN_POINT('Ctrl Pts',(3.82511181316626,-6.20493143702771,
44.9074068436854));
#180858=CARTESIAN_POINT('Ctrl Pts',(7.21677530648096,-2.75667877403707,
45.1189634640673));
#180859=CARTESIAN_POINT('Ctrl Pts',(7.30949492399773,2.47708495470907,45.3305200844492));
#180860=CARTESIAN_POINT('Ctrl Pts',(4.07431487762509,6.03983811237955,45.5420767048312));
#180861=CARTESIAN_POINT('Ctrl Pts',(-0.440783824531858,7.70521760537255,
45.7536333252129));
#180862=CARTESIAN_POINT('Ctrl Pts',(-5.25889366826367,5.65907705053069,
45.9651899455951));
#180863=CARTESIAN_POINT('Ctrl Pts',(-7.18591574462435,1.22281586655384,
46.1767465659768));
#180864=CARTESIAN_POINT('Ctrl Pts',(-6.9149963450596,-2.34384093444894,
46.3354140312633));
#180865=CARTESIAN_POINT('Ctrl Pts',(-4.94379997775315,-5.37508475202271,
46.4940814965496));
#180866=CARTESIAN_POINT('Ctrl Pts',(-1.77521407621494,-7.07708644730382,
46.6527489618362));
#180867=CARTESIAN_POINT('Ctrl Pts',(1.82153073585822,-7.07210174974048,
46.8114164271225));
#180868=CARTESIAN_POINT('Ctrl Pts',(4.99007686623289,-5.33011694781774,
46.9700838924091));
#180869=CARTESIAN_POINT('Ctrl Pts',(6.91227697700186,-2.31357490358806,
47.1287513576954));
#180870=CARTESIAN_POINT('Ctrl Pts',(7.30733455477124,2.50694719739402,47.3403079780773));
#180871=CARTESIAN_POINT('Ctrl Pts',(4.02520767790373,6.58499020741276,47.5518645984592));
#180872=CARTESIAN_POINT('Ctrl Pts',(-0.741099433620822,7.24771064107016,
47.7634212188411));
#180873=CARTESIAN_POINT('Ctrl Pts',(-5.27532288542961,5.63393445682585,
47.9749778392231));
#180874=CARTESIAN_POINT('Ctrl Pts',(-7.66274994821465,0.975569028180616,
48.1865344596049));
#180875=CARTESIAN_POINT('Ctrl Pts',(-6.30175893983736,-3.66453279862005,
48.3980910799869));
#180876=CARTESIAN_POINT('Ctrl Pts',(-3.80592445995426,-6.23071373925649,
48.5567585452732));
#180877=CARTESIAN_POINT('Ctrl Pts',(-0.355881681196406,-7.29281176210305,
48.7154260105597));
#180878=CARTESIAN_POINT('Ctrl Pts',(3.17791768866892,-6.5742646074729,48.8740934758461));
#180879=CARTESIAN_POINT('Ctrl Pts',(5.91706485393949,-4.25746597045867,
49.0327609411326));
#180880=CARTESIAN_POINT('Ctrl Pts',(7.71518712742009,0.212958204582113,
49.2443175615145));
#180881=CARTESIAN_POINT('Ctrl Pts',(5.3332736079391,6.33388915228324,49.5087633369919));
#180882=CARTESIAN_POINT('Ctrl Pts',(-2.45101487628526,7.91115770243905,
49.8260982675646));
#180883=CARTESIAN_POINT('Ctrl Pts',(-7.02573858895822,3.19290517876247,
50.0905440430422));
#180884=CARTESIAN_POINT('Ctrl Pts',(-7.10655132029403,-1.61882067803289,
50.3021006634239));
#180885=CARTESIAN_POINT('Ctrl Pts',(-5.48414662636755,-4.82881078130398,
50.4607681287105));
#180886=CARTESIAN_POINT('Ctrl Pts',(-2.50656909549661,-6.84409312782312,
50.6194355939968));
#180887=CARTESIAN_POINT('Ctrl Pts',(2.27895306528776,-7.37372428966872,
50.8309922143788));
#180888=CARTESIAN_POINT('Ctrl Pts',(7.53371292847594,-3.43308380079491,
51.0954379898561));
#180889=CARTESIAN_POINT('Ctrl Pts',(6.96415171352099,4.48792878509655,51.412772920429));
#180890=CARTESIAN_POINT('Ctrl Pts',(1.17864575368756,7.62636082207304,51.6772186959064));
#180891=CARTESIAN_POINT('Ctrl Pts',(-3.46063736178883,6.40824902510984,
51.8887753162883));
#180892=CARTESIAN_POINT('Ctrl Pts',(-7.03711701014562,3.17872162429317,
52.1003319366701));
#180893=CARTESIAN_POINT('Ctrl Pts',(-7.44912142538699,-2.03950264176283,
52.3118885570521));
#180894=CARTESIAN_POINT('Ctrl Pts',(-4.4132576416278,-5.8020426150045,52.523445177434));
#180895=CARTESIAN_POINT('Ctrl Pts',(-1.12530437433415,-7.2141332047132,
52.6821126427204));
#180896=CARTESIAN_POINT('Ctrl Pts',(2.47337717630653,-6.87120137135288,
52.8407801080068));
#180897=CARTESIAN_POINT('Ctrl Pts',(5.44992684100399,-4.85145260601411,
52.9994475732933));
#180898=CARTESIAN_POINT('Ctrl Pts',(7.11132296817816,-1.6615052764948,53.1581150385797));
#180899=CARTESIAN_POINT('Ctrl Pts',(7.03528347837356,1.95349460782157,53.3167825038662));
#180900=CARTESIAN_POINT('Ctrl Pts',(5.2522263462681,5.05436226548548,53.4754499691526));
#180901=CARTESIAN_POINT('Ctrl Pts',(1.16298787833305,7.63731658881341,53.6870065895345));
#180902=CARTESIAN_POINT('Ctrl Pts',(-3.9713456319968,6.61763934552863,53.8985632099163));
#180903=CARTESIAN_POINT('Ctrl Pts',(-6.76668767926396,2.70029239264587,
54.1101198302983));
#180904=CARTESIAN_POINT('Ctrl Pts',(-7.43633718779138,-2.06533199412456,
54.3216764506802));
#180905=CARTESIAN_POINT('Ctrl Pts',(-4.41465255275869,-6.3397124742808,
54.5332330710621));
#180906=CARTESIAN_POINT('Ctrl Pts',(0.329432312156239,-7.2817668285877,
54.7447896914439));
#180907=CARTESIAN_POINT('Ctrl Pts',(3.75743771505433,-6.26038688161627,
54.9034571567305));
#180908=CARTESIAN_POINT('Ctrl Pts',(6.30152019550041,-3.69100566880029,
55.0621246220168));
#180909=CARTESIAN_POINT('Ctrl Pts',(7.29259979915511,-0.233484326409,55.2207920873034));
#180910=CARTESIAN_POINT('Ctrl Pts',(6.52471960310607,3.2803529583477,55.3794595525896));
#180911=CARTESIAN_POINT('Ctrl Pts',(4.15020428334716,6.00721098109562,55.5381270178762));
#180912=CARTESIAN_POINT('Ctrl Pts',(0.794555753034778,7.24578055922568,
55.6967944831625));
#180913=CARTESIAN_POINT('Ctrl Pts',(-4.00007614591683,6.60912352067989,
55.9083511035445));
#180914=CARTESIAN_POINT('Ctrl Pts',(-7.28899019261408,2.53678713496527,
56.1199077239264));
#180915=CARTESIAN_POINT('Ctrl Pts',(-6.92556390568595,-2.26191300443743,
56.3314643443083));
#180916=CARTESIAN_POINT('Ctrl Pts',(-4.38651904809834,-6.35004862765727,
56.5430209646902));
#180917=CARTESIAN_POINT('Ctrl Pts',(0.672048848250074,-7.69606869279577,
56.7545775850721));
#180918=CARTESIAN_POINT('Ctrl Pts',(4.91817373622454,-5.37998344443186,
56.966134205454));
#180919=CARTESIAN_POINT('Ctrl Pts',(6.89587288824271,-2.39952417604946,
57.1248016707404));
#180920=CARTESIAN_POINT('Ctrl Pts',(7.20312249874772,1.20320753242157,57.2834691360269));
#180921=CARTESIAN_POINT('Ctrl Pts',(5.7489468681493,4.49289830715034,57.4421366013132));
#180922=CARTESIAN_POINT('Ctrl Pts',(2.90813762287981,6.6989116777301,57.6008040665998));
#180923=CARTESIAN_POINT('Ctrl Pts',(-0.662072407274711,7.27134370570345,
57.7594715318861));
#180924=CARTESIAN_POINT('Ctrl Pts',(-4.03210406990081,6.07246173606323,
57.9181389971726));
#180925=CARTESIAN_POINT('Ctrl Pts',(-7.30560046055249,2.51183695474357,
58.1296956175544));
#180926=CARTESIAN_POINT('Ctrl Pts',(-7.22183907457384,-2.72207775414384,
58.3412522379364));
#180927=CARTESIAN_POINT('Ctrl Pts',(-3.86839828499165,-6.1737493137209,
58.5528088583183));
#180928=CARTESIAN_POINT('Ctrl Pts',(0.700273394512465,-7.68597970928456,
58.7643654787002));
#180929=CARTESIAN_POINT('Ctrl Pts',(5.44667094866594,-5.47858545187604,
58.9759220990821));
#180930=CARTESIAN_POINT('Ctrl Pts',(7.22305188360823,-0.979885836762679,
59.187478719464));
#180931=CARTESIAN_POINT('Ctrl Pts',(6.83205747267965,2.57561057790011,59.3461461847504));
#180932=CARTESIAN_POINT('Ctrl Pts',(4.75979552384035,5.53868474197977,59.5048136500368));
#180933=CARTESIAN_POINT('Ctrl Pts',(1.5356435340166,7.13290433322296,59.6634811153233));
#180934=CARTESIAN_POINT('Ctrl Pts',(-2.0589023719168,7.00668274740098,59.8221485806097));
#180935=CARTESIAN_POINT('Ctrl Pts',(-5.16690111965939,5.1588673154724,59.9808160458961));
#180936=CARTESIAN_POINT('Ctrl Pts',(-6.98636728977782,2.07926113288135,
60.1394835111826));
#180937=CARTESIAN_POINT('Ctrl Pts',(-7.2186077705201,-2.7518766018717,60.3510401315645));
#180938=CARTESIAN_POINT('Ctrl Pts',(-3.80106741782251,-6.71688569232549,
60.5625967519464));
#180939=CARTESIAN_POINT('Ctrl Pts',(0.985143555366984,-7.21866871766008,
60.7741533723283));
#180940=CARTESIAN_POINT('Ctrl Pts',(5.46187841175089,-5.45275628777296,
60.9857099927101));
#180941=CARTESIAN_POINT('Ctrl Pts',(7.692011048468,-0.717000004733705,61.1972666130922));
#180942=CARTESIAN_POINT('Ctrl Pts',(6.17374629198927,3.8752434102308,61.408823233474));
#180943=CARTESIAN_POINT('Ctrl Pts',(3.59562521266291,6.35470365076531,61.5674906987604));
#180944=CARTESIAN_POINT('Ctrl Pts',(0.106152327585856,7.30215131198737,
61.7261581640469));
#180945=CARTESIAN_POINT('Ctrl Pts',(-3.39076980577516,6.46058862757269,
61.8848256293334));
#180946=CARTESIAN_POINT('Ctrl Pts',(-6.06984555801569,4.06074586765145,
62.0434930946197));
#180947=CARTESIAN_POINT('Ctrl Pts',(-7.27236513221156,0.650756899909928,
62.2021605599062));
#180948=CARTESIAN_POINT('Ctrl Pts',(-6.6963564918669,-2.8794903195219,62.3608280251925));
#180949=CARTESIAN_POINT('Ctrl Pts',(-3.77949506399865,-6.73769545451199,
62.5723846455745));
#180950=CARTESIAN_POINT('Ctrl Pts',(1.38481388060952,-7.5925593467993,62.7839412659564));
#180951=CARTESIAN_POINT('Ctrl Pts',(5.38121221862196,-4.91143980296606,
62.9954978863382));
#180952=CARTESIAN_POINT('Ctrl Pts',(7.68713950594068,-0.687425003040209,
63.2070545067203));
#180953=CARTESIAN_POINT('Ctrl Pts',(6.36539585962448,4.37754023703006,63.418611127102));
#180954=CARTESIAN_POINT('Ctrl Pts',(2.25752519810707,6.93081775451498,63.6301677474841));
#180955=CARTESIAN_POINT('Ctrl Pts',(-1.31051506173819,7.18284967348925,
63.7888352127705));
#180956=CARTESIAN_POINT('Ctrl Pts',(-4.59678504746447,5.67470257610194,
63.9475026780568));
#180957=CARTESIAN_POINT('Ctrl Pts',(-6.74260426573885,2.78815584322654,
64.1061701433434));
#180958=CARTESIAN_POINT('Ctrl Pts',(-7.26212184340347,-0.770888079667159,
64.2648376086296));
#180959=CARTESIAN_POINT('Ctrl Pts',(-6.00074570958805,-4.15954686087889,
64.4235050739162));
#180960=CARTESIAN_POINT('Ctrl Pts',(-3.29674459808297,-6.50108681847883,
64.5821725392026));
#180961=CARTESIAN_POINT('Ctrl Pts',(1.41470968505832,-7.5947165505728,64.7937291595845));
#180962=CARTESIAN_POINT('Ctrl Pts',(5.92762625552272,-4.94246030772492,
65.0052857799664));
#180963=CARTESIAN_POINT('Ctrl Pts',(7.27839608796312,-0.323475295391354,
65.2168424003483));
#180964=CARTESIAN_POINT('Ctrl Pts',(6.3427075198956,4.39712727080518,65.4283990207302));
#180965=CARTESIAN_POINT('Ctrl Pts',(2.08286845720701,7.43927294609588,65.6399556411121));
#180966=CARTESIAN_POINT('Ctrl Pts',(-2.70702760250574,6.767913735093,65.8515122614941));
#180967=CARTESIAN_POINT('Ctrl Pts',(-5.60808871082759,4.67548074217773,
66.0101797267804));
#180968=CARTESIAN_POINT('Ctrl Pts',(-7.16510371778334,1.41208031401127,
66.1688471920669));
#180969=CARTESIAN_POINT('Ctrl Pts',(-6.96336145416755,-2.17901871242343,
66.3275146573532));
#180970=CARTESIAN_POINT('Ctrl Pts',(-5.08207139110363,-5.24454311408888,
66.4861821226398));
#180971=CARTESIAN_POINT('Ctrl Pts',(-1.9425474276618,-7.03827312984311,
66.6448495879261));
#180972=CARTESIAN_POINT('Ctrl Pts',(1.63378349280974,-7.10376000896784,
66.8035170532126));
#180973=CARTESIAN_POINT('Ctrl Pts',(5.95196273324006,-4.92496320784874,
67.0150736735945));
#180974=CARTESIAN_POINT('Ctrl Pts',(7.71781440523415,0.00277938102636093,
67.2266302939764));
#180975=CARTESIAN_POINT('Ctrl Pts',(5.79569591456879,4.41470211292405,67.4381869143583));
#180976=CARTESIAN_POINT('Ctrl Pts',(2.05289915213827,7.43977634003525,67.6497435347402));
#180977=CARTESIAN_POINT('Ctrl Pts',(-3.16688493518823,7.04641488870896,
67.8613001551221));
#180978=CARTESIAN_POINT('Ctrl Pts',(-6.41451232295659,3.46217943281784,
68.072856775504));
#180979=CARTESIAN_POINT('Ctrl Pts',(-7.30142245391383,-0.0030509785204721,
68.2315242407905));
#180980=CARTESIAN_POINT('Ctrl Pts',(-6.40614816070338,-3.50627264241207,
68.3901917060768));
#180981=CARTESIAN_POINT('Ctrl Pts',(-3.95052789288941,-6.13431778260475,
68.5488591713634));
#180982=CARTESIAN_POINT('Ctrl Pts',(-0.542048797793145,-7.28277867304929,
68.7075266366497));
#180983=CARTESIAN_POINT('Ctrl Pts',(3.01771567371951,-6.64862175729487,
68.8661941019362));
#180984=CARTESIAN_POINT('Ctrl Pts',(5.80562811966774,-4.40764527866205,
69.0248615672226));
#180985=CARTESIAN_POINT('Ctrl Pts',(7.72529037506696,0.0318056196186821,
69.2364181876045));
#180986=CARTESIAN_POINT('Ctrl Pts',(5.92406490744874,4.9467284027863,69.4479748079864));
#180987=CARTESIAN_POINT('Ctrl Pts',(1.62163628485237,7.10281505036246,69.6595314283683));
#180988=CARTESIAN_POINT('Ctrl Pts',(-3.19021829660345,7.02760088071422,
69.8710880487503));
#180989=CARTESIAN_POINT('Ctrl Pts',(-6.94602533424518,3.38139838418462,
70.082644669132));
#180990=CARTESIAN_POINT('Ctrl Pts',(-7.14327651483587,-1.45129438742892,
70.2942012895141));
#180991=CARTESIAN_POINT('Ctrl Pts',(-5.60417935245795,-4.68016590993002,
70.4528687548005));
#180992=CARTESIAN_POINT('Ctrl Pts',(-2.67235615860385,-6.79641042473032,
70.6115362200868));
#180993=CARTESIAN_POINT('Ctrl Pts',(0.896820584063685,-7.24101085004557,
70.7702036853734));
#180994=CARTESIAN_POINT('Ctrl Pts',(4.24968613157379,-5.93909503905437,
70.9288711506597));
#180995=CARTESIAN_POINT('Ctrl Pts',(6.57663582428436,-3.17153596759146,
71.0875386159461));
#180996=CARTESIAN_POINT('Ctrl Pts',(7.28150105130947,0.335256925607207,
71.2462060812327));
#180997=CARTESIAN_POINT('Ctrl Pts',(5.91120873762049,4.97380480485727,71.4577627016144));
#180998=CARTESIAN_POINT('Ctrl Pts',(1.37934497512927,7.59355479062239,71.6693193219963));
#180999=CARTESIAN_POINT('Ctrl Pts',(-3.30546598448607,6.49257887941386,
71.8808759423784));
#181000=CARTESIAN_POINT('Ctrl Pts',(-6.95188739007309,3.35200367457157,
72.0924325627602));
#181001=CARTESIAN_POINT('Ctrl Pts',(-7.49962539393021,-1.85384517348655,
72.3039891831422));
#181002=CARTESIAN_POINT('Ctrl Pts',(-4.55490242328635,-5.69082759189985,
72.515545803524));
#181003=CARTESIAN_POINT('Ctrl Pts',(-1.30451174193676,-7.18394239078625,
72.6742132688105));
#181004=CARTESIAN_POINT('Ctrl Pts',(2.30240347260119,-6.93048485671565,
72.8328807340969));
#181005=CARTESIAN_POINT('Ctrl Pts',(5.32771060717041,-4.98518053602091,
72.9915481993833));
#181006=CARTESIAN_POINT('Ctrl Pts',(7.06798540710278,-1.83746139681714,
73.1502156646698));
#181007=CARTESIAN_POINT('Ctrl Pts',(7.08154981624765,1.77832262511333,73.3088831299561));
#181008=CARTESIAN_POINT('Ctrl Pts',(5.37604808188036,4.92247516882501,73.4675505952426));
#181009=CARTESIAN_POINT('Ctrl Pts',(1.35212671216226,7.60610783060554,73.6791072156245));
#181010=CARTESIAN_POINT('Ctrl Pts',(-3.80590427361156,6.71414622857621,
73.8906638360064));
#181011=CARTESIAN_POINT('Ctrl Pts',(-6.69760208823675,2.8673702494886,74.1022204563883));
#181012=CARTESIAN_POINT('Ctrl Pts',(-7.48529396902241,-1.88017050182019,
74.3137770767701));
#181013=CARTESIAN_POINT('Ctrl Pts',(-4.57060869449738,-6.22821476334324,
74.5253336971522));
#181014=CARTESIAN_POINT('Ctrl Pts',(0.14864125104275,-7.28769926279049,
74.736890317534));
#181015=CARTESIAN_POINT('Ctrl Pts',(3.60093471970022,-6.35169649018624,
74.8955577828204));
#181016=CARTESIAN_POINT('Ctrl Pts',(6.20799117870964,-3.84623551344357,
75.054225248107));
#181017=CARTESIAN_POINT('Ctrl Pts',(7.28456049178201,-0.414371490388394,
75.2128927133932));
#181018=CARTESIAN_POINT('Ctrl Pts',(6.60410948866829,3.11743804453148,75.3715601786798));
#181019=CARTESIAN_POINT('Ctrl Pts',(4.29798968114953,5.90237781404404,75.5302276439661));
#181020=CARTESIAN_POINT('Ctrl Pts',(0.974108399537163,7.22383330319435,
75.6888951092526));
#181021=CARTESIAN_POINT('Ctrl Pts',(-3.83484522790941,6.70634662499054,
75.9004517296344));
#181022=CARTESIAN_POINT('Ctrl Pts',(-7.22379777981015,2.71687551334403,
76.1120083500165));
#181023=CARTESIAN_POINT('Ctrl Pts',(-6.97955867591795,-2.08936511156467,
76.3235649703983));
#181024=CARTESIAN_POINT('Ctrl Pts',(-4.54273890266891,-6.23924596251639,
76.5351215907802));
#181025=CARTESIAN_POINT('Ctrl Pts',(0.480871141788821,-7.71037521275954,
76.7466782111622));
#181026=CARTESIAN_POINT('Ctrl Pts',(4.78316007615798,-5.50036675615697,
76.958234831544));
#181027=CARTESIAN_POINT('Ctrl Pts',(6.83420758004432,-2.56989998090428,
77.1169022968304));
#181028=CARTESIAN_POINT('Ctrl Pts',(7.23076101275103,1.02409827472298,77.2755697621169));
#181029=CARTESIAN_POINT('Ctrl Pts',(5.85866375653961,4.34886011252226,77.4342372274033));
#181030=CARTESIAN_POINT('Ctrl Pts',(3.07346940853301,6.62468624876852,77.5929046926898));
#181031=CARTESIAN_POINT('Ctrl Pts',(-0.481436928319852,7.2855334494488,
77.7515721579762));
#181032=CARTESIAN_POINT('Ctrl Pts',(-3.88018004147505,6.17064482952365,
77.9102396232625));
#181033=CARTESIAN_POINT('Ctrl Pts',(-7.2410220538478,2.69234518444999,78.1217962436445));
#181034=CARTESIAN_POINT('Ctrl Pts',(-7.28716117403719,-2.54203637704176,
78.3333528640264));
#181035=CARTESIAN_POINT('Ctrl Pts',(-4.02040297608787,-6.07585761764288,
78.5449094844083));
#181036=CARTESIAN_POINT('Ctrl Pts',(0.509337346907534,-7.70098970169701,
78.7564661047903));
#181037=CARTESIAN_POINT('Ctrl Pts',(5.30904783833082,-5.61205256807673,
78.968022725172));
#181038=CARTESIAN_POINT('Ctrl Pts',(7.19651283393159,-1.15881741333442,
79.1795793455541));
#181039=CARTESIAN_POINT('Ctrl Pts',(6.89386514584086,2.40528636755536,79.3382468108404));
#181040=CARTESIAN_POINT('Ctrl Pts',(4.89576720374896,5.41886940113037,79.4969142761268));
#181041=CARTESIAN_POINT('Ctrl Pts',(1.71216705625423,7.09260243224975,79.6555817414134));
#181042=CARTESIAN_POINT('Ctrl Pts',(-1.88440410108198,7.05561501809986,
79.8142492066997));
#181043=CARTESIAN_POINT('Ctrl Pts',(-5.03729766256781,5.2854906506091,79.9729166719862));
#181044=CARTESIAN_POINT('Ctrl Pts',(-6.93262114598237,2.25198108621416,
80.1315841372726));
#181045=CARTESIAN_POINT('Ctrl Pts',(-7.28467029558747,-2.57190623101369,
80.3431407576545));
#181046=CARTESIAN_POINT('Ctrl Pts',(-3.96657026414199,-6.62049750836168,
80.5546973780365));
#181047=CARTESIAN_POINT('Ctrl Pts',(0.805715678220276,-7.2408913902831,
80.7662539984183));
#181048=CARTESIAN_POINT('Ctrl Pts',(5.32489154541992,-5.5866087162172,80.9778106188002));
#181049=CARTESIAN_POINT('Ctrl Pts',(7.67185086545011,-0.907649312693826,
81.1893672391822));
#181050=CARTESIAN_POINT('Ctrl Pts',(6.26800584722486,3.72085439993874,81.400923859564));
#181051=CARTESIAN_POINT('Ctrl Pts',(3.7522041082529,6.26352484540433,81.5595913248505));
#181052=CARTESIAN_POINT('Ctrl Pts',(0.287315719605677,7.29726878887425,
81.7182587901368));
#181053=CARTESIAN_POINT('Ctrl Pts',(-3.22941224766972,6.54273809846297,
81.8769262554235));
#181054=CARTESIAN_POINT('Ctrl Pts',(-5.96721292964122,4.21011305693017,
82.0355937207096));
#181055=CARTESIAN_POINT('Ctrl Pts',(-7.25397792594564,0.831013482971333,
82.1942611859963));
#181056=CARTESIAN_POINT('Ctrl Pts',(-6.76574644210904,-2.71243983296907,
82.3529286512825));
#181057=CARTESIAN_POINT('Ctrl Pts',(-3.94552092764993,-6.64183616073285,
82.5644852716646));
#181058=CARTESIAN_POINT('Ctrl Pts',(1.19598519098252,-7.62458433893602,
82.7760418920463));
#181059=CARTESIAN_POINT('Ctrl Pts',(5.25768245471263,-5.04345725523793,
82.9875985124284));
#181060=CARTESIAN_POINT('Ctrl Pts',(7.6677146990491,-0.877962534841406,
83.1991551328101));
#181061=CARTESIAN_POINT('Ctrl Pts',(6.47206043035542,4.21824095594002,83.4107117531922));
#181062=CARTESIAN_POINT('Ctrl Pts',(2.42881185107603,6.87266525872325,83.622268373574));
#181063=CARTESIAN_POINT('Ctrl Pts',(-1.13187581356494,7.21315716601639,
83.7809358388604));
#181064=CARTESIAN_POINT('Ctrl Pts',(-4.45455716730101,5.78702017821416,
83.9396033041469));
#181065=CARTESIAN_POINT('Ctrl Pts',(-6.67134261913675,2.95460876404444,
84.0982707694333));
#181066=CARTESIAN_POINT('Ctrl Pts',(-7.27901458618699,-0.59044792648265,
84.2569382347199));
#181067=CARTESIAN_POINT('Ctrl Pts',(-6.10211325965054,-4.0093631570841,
84.415605700006));
#181068=CARTESIAN_POINT('Ctrl Pts',(-3.45704788576693,-6.41727938318902,
84.5742731652928));
#181069=CARTESIAN_POINT('Ctrl Pts',(1.22581826102235,-7.62748271499098,
84.7858297856743));
#181070=CARTESIAN_POINT('Ctrl Pts',(5.80315849686724,-5.08802696325753,
84.9973864060566));
#181071=CARTESIAN_POINT('Ctrl Pts',(7.26812821260561,-0.503982306367513,
85.2089430264381));
#181072=CARTESIAN_POINT('Ctrl Pts',(6.44986511072318,4.23838494854769,85.4204996468203));
#181073=CARTESIAN_POINT('Ctrl Pts',(2.26682573146811,7.38529783283633,85.6320562672021));
#181074=CARTESIAN_POINT('Ctrl Pts',(-2.53825459376176,6.83300215012667,
85.843612887584));
#181075=CARTESIAN_POINT('Ctrl Pts',(-5.49034419207115,4.8132005787809,86.0022803528705));
#181076=CARTESIAN_POINT('Ctrl Pts',(-7.12785800821615,1.58944088110241,
86.1609478181568));
#181077=CARTESIAN_POINT('Ctrl Pts',(-7.01528763922505,-2.00555843330848,
86.3196152834433));
#181078=CARTESIAN_POINT('Ctrl Pts',(-5.21064498668112,-5.11682136903231,
86.4782827487299));
#181079=CARTESIAN_POINT('Ctrl Pts',(-2.11659747242173,-6.98790342654534,
86.636950214016));
#181080=CARTESIAN_POINT('Ctrl Pts',(1.45700724128982,-7.14211345927923,
86.7956176793028));
#181081=CARTESIAN_POINT('Ctrl Pts',(5.82792165520774,-5.07113913803433,
87.0071742996843));
#181082=CARTESIAN_POINT('Ctrl Pts',(7.71550693145075,-0.188731845047518,
87.2187309200666));
#181083=CARTESIAN_POINT('Ctrl Pts',(5.90345804255837,4.26952796217078,87.4302875404482));
#181084=CARTESIAN_POINT('Ctrl Pts',(2.23687814569083,7.38654473214158,87.6418441608304));
#181085=CARTESIAN_POINT('Ctrl Pts',(-2.99105958231513,7.12282847972511,
87.853400781212));
#181086=CARTESIAN_POINT('Ctrl Pts',(-6.32662643415989,3.62028351499959,
88.0649574015941));
#181087=CARTESIAN_POINT('Ctrl Pts',(-7.29924993347449,0.178127953053212,
88.2236248668804));
#181088=CARTESIAN_POINT('Ctrl Pts',(-6.4911804899301,-3.34623040852862,
88.3822923321669));
#181089=CARTESIAN_POINT('Ctrl Pts',(-4.10152883824385,-6.03440025847909,
88.5409597974534));
#181090=CARTESIAN_POINT('Ctrl Pts',(-0.722597256169509,-7.2670857505046,
88.6996272627396));
#181091=CARTESIAN_POINT('Ctrl Pts',(2.85180711825703,-6.72145633916083,
88.8582947280263));
#181092=CARTESIAN_POINT('Ctrl Pts',(5.69446886265268,-4.55034934248657,
89.0169621933125));
#181093=CARTESIAN_POINT('Ctrl Pts',(7.72370085836359,-0.159900053332423,
89.2285188136947));
#181094=CARTESIAN_POINT('Ctrl Pts',(6.04498924497306,4.79820507552133,89.4400754340764));
#181095=CARTESIAN_POINT('Ctrl Pts',(1.79738669100653,7.06038858441927,89.6516320544583));
#181096=CARTESIAN_POINT('Ctrl Pts',(-3.0148526110767,7.10459926048484,89.8631886748402));
#181097=CARTESIAN_POINT('Ctrl Pts',(-6.85998029030325,3.55271634009713,
90.0747452952221));
#181098=CARTESIAN_POINT('Ctrl Pts',(-7.17708950032582,-1.27359376203776,
90.286301915604));
#181099=CARTESIAN_POINT('Ctrl Pts',(-5.71858768820459,-4.53966232348847,
90.4449693808904));
#181100=CARTESIAN_POINT('Ctrl Pts',(-2.84017988572216,-6.72800567156068,
90.603636846177));
#181101=CARTESIAN_POINT('Ctrl Pts',(0.716865503818649,-7.2610349909575,
90.7623043114633));
#181102=CARTESIAN_POINT('Ctrl Pts',(4.10100447634138,-6.04271829434759,
90.9209717767497));
#181103=CARTESIAN_POINT('Ctrl Pts',(6.49591206166963,-3.3337524872193,91.0796392420362));
#181104=CARTESIAN_POINT('Ctrl Pts',(7.28757804590501,0.154470033412751,
91.2383067073226));
#181105=CARTESIAN_POINT('Ctrl Pts',(6.03280890944947,4.82559215419812,91.4498633277045));
#181106=CARTESIAN_POINT('Ctrl Pts',(1.5673472359543,7.55698945086174,91.6614199480865));
#181107=CARTESIAN_POINT('Ctrl Pts',(-3.14334088454258,6.57260176518045,
91.8729765684682));
#181108=CARTESIAN_POINT('Ctrl Pts',(-6.86656994343417,3.52347614302835,
92.0845331888503));
#181109=CARTESIAN_POINT('Ctrl Pts',(-7.54331757626141,-1.6671781308104,
92.2960898092321));
#181110=CARTESIAN_POINT('Ctrl Pts',(-4.69471247615664,-5.57604963511976,
92.5076464296141));
#181111=CARTESIAN_POINT('Ctrl Pts',(-1.48237289522515,-7.14936009422644,
92.6663138949004));
#181112=CARTESIAN_POINT('Ctrl Pts',(2.12972100334073,-6.98548284302441,
92.8249813601869));
#181113=CARTESIAN_POINT('Ctrl Pts',(5.20236750987503,-5.11584768931891,
92.9836488254733));
#181114=CARTESIAN_POINT('Ctrl Pts',(7.02021416653538,-2.01228108246395,
93.1423162907598));
#181115=CARTESIAN_POINT('Ctrl Pts',(7.1234967097829,1.60205299418413,93.3009837560462));
#181116=CARTESIAN_POINT('Ctrl Pts',(5.4965393404678,4.78755783384145,93.4596512213326));
#181117=CARTESIAN_POINT('Ctrl Pts',(1.54044884797169,7.57021402675984,93.6712078417144));
#181118=CARTESIAN_POINT('Ctrl Pts',(-3.63812709720397,6.8065187894964,93.8827644620965));
#181119=CARTESIAN_POINT('Ctrl Pts',(-6.62438866228044,3.03268210390607,
94.0943210824783));
#181120=CARTESIAN_POINT('Ctrl Pts',(-7.52964381413117,-1.6938510040437,
94.3058777028602));
#181121=CARTESIAN_POINT('Ctrl Pts',(-4.72374865002601,-6.11288153979815,
94.5174343232423));
#181122=CARTESIAN_POINT('Ctrl Pts',(-0.0322420101528263,-7.2891437288087,
94.7289909436239));
#181123=CARTESIAN_POINT('Ctrl Pts',(3.44221456469878,-6.43909438121071,
94.8876584089105));
#181124=CARTESIAN_POINT('Ctrl Pts',(6.11063877182138,-3.99909701236707,
95.0463258741969));
#181125=CARTESIAN_POINT('Ctrl Pts',(7.27203543413222,-0.59500289912095,
95.2049933394833));
#181126=CARTESIAN_POINT('Ctrl Pts',(6.67943187871136,2.95260222294936,95.3636608047698));
#181127=CARTESIAN_POINT('Ctrl Pts',(4.44312903876971,5.79391180272748,95.522328270056));
#181128=CARTESIAN_POINT('Ctrl Pts',(1.15305975893871,7.1974337368613,95.6809957353428));
#181129=CARTESIAN_POINT('Ctrl Pts',(-3.66724954191073,6.79944796472536,
95.8925523557242));
#181130=CARTESIAN_POINT('Ctrl Pts',(-7.15416271867079,2.89527501251126,
96.1041089761066));
#181131=CARTESIAN_POINT('Ctrl Pts',(-7.02924814289869,-1.9155119933763,
96.3156655964883));
#181132=CARTESIAN_POINT('Ctrl Pts',(-4.69617864516543,-6.12464676367938,
96.5272222168702));
#181133=CARTESIAN_POINT('Ctrl Pts',(0.289432265469185,-7.71984168134798,
96.7387788372523));
#181134=CARTESIAN_POINT('Ctrl Pts',(4.64515762980606,-5.61747601173444,
96.950335457634));
#181135=CARTESIAN_POINT('Ctrl Pts',(6.76842455697748,-2.73845433636555,
97.1090029229205));
#181136=CARTESIAN_POINT('Ctrl Pts',(7.25376943663278,0.843893506703,97.2676703882068));
#181137=CARTESIAN_POINT('Ctrl Pts',(5.96510980865853,4.20302829244156,97.4263378534934));
#181138=CARTESIAN_POINT('Ctrl Pts',(3.23627226523146,6.54471228718507,97.5850053187797));
#181139=CARTESIAN_POINT('Ctrl Pts',(-0.299318307035372,7.29834602864233,
97.7436727840662));
#181140=CARTESIAN_POINT('Ctrl Pts',(-3.72798211249406,6.25951141932153,
97.9023402493526));
#181141=CARTESIAN_POINT('Ctrl Pts',(-7.16726359359828,2.88320234719056,
98.1138968697345));
#181142=CARTESIAN_POINT('Ctrl Pts',(-7.40368502527283,-3.69526160713197,
98.3783426452119));
#181143=CARTESIAN_POINT('Ctrl Pts',(-2.00393381935232,-7.46117725044532,
98.6427884206892));
#181144=CARTESIAN_POINT('Ctrl Pts',(2.76117551751445,-6.74170561393421,
98.8543450410712));
#181145=CARTESIAN_POINT('Ctrl Pts',(5.65332152640388,-4.62673929743301,
99.0130125063575));
#181146=CARTESIAN_POINT('Ctrl Pts',(7.17439520364235,-1.34694727795331,
99.1716799716442));
#181147=CARTESIAN_POINT('Ctrl Pts',(6.94703914831595,2.23909199201735,99.3303474369303));
#181148=CARTESIAN_POINT('Ctrl Pts',(5.03003528944799,5.29274464953559,99.4890207192591));
#181149=CARTESIAN_POINT('Ctrl Pts',(2.93567476420474,6.46407674877753,99.5948048464922));
#181150=CARTESIAN_POINT('Ctrl Pts',(1.81148773798651,6.7650987574823,99.6476998186297));
#181151=CARTESIAN_POINT('Ctrl Pts',(-5.59319257183209,4.82318409121508,
-0.216170757716313));
#181152=CARTESIAN_POINT('Ctrl Pts',(-6.39483282223799,3.89356867920839,
-0.16326603689069));
#181153=CARTESIAN_POINT('Ctrl Pts',(-7.52577891557862,1.62945095308381,
-0.057472160969592));
#181154=CARTESIAN_POINT('Ctrl Pts',(-7.38490913059102,-2.17042384913742,
0.101210870046983));
#181155=CARTESIAN_POINT('Ctrl Pts',(-5.45514273541142,-5.43154102245448,
0.259878335333412));
#181156=CARTESIAN_POINT('Ctrl Pts',(-2.18287509717614,-7.38815633597361,
0.41854580061984));
#181157=CARTESIAN_POINT('Ctrl Pts',(1.59344116692286,-7.51571166761254,
0.577213265906269));
#181158=CARTESIAN_POINT('Ctrl Pts',(6.17446001743441,-5.31529267069683,
0.788769886288175));
#181159=CARTESIAN_POINT('Ctrl Pts',(8.64709586414073,1.1719534463109,1.05321566176556));
#181160=CARTESIAN_POINT('Ctrl Pts',(4.53730628273561,6.7665709570828,1.31766143724294));
#181161=CARTESIAN_POINT('Ctrl Pts',(-0.464471910629743,7.66905552806737,
1.52921805762484));
#181162=CARTESIAN_POINT('Ctrl Pts',(-4.0699281104299,6.54009937284872,1.68788552291128));
#181163=CARTESIAN_POINT('Ctrl Pts',(-6.70494269659998,3.7850714469408,1.8465529881977));
#181164=CARTESIAN_POINT('Ctrl Pts',(-7.69429901191945,0.124358320332814,
2.00522045348413));
#181165=CARTESIAN_POINT('Ctrl Pts',(-6.82439171170274,-3.5687316022377,
2.16388791877056));
#181166=CARTESIAN_POINT('Ctrl Pts',(-4.27550416845679,-6.40371138085426,
2.32255538405699));
#181167=CARTESIAN_POINT('Ctrl Pts',(-0.716080791044483,-7.65360327218264,
2.48122284934342));
#181168=CARTESIAN_POINT('Ctrl Pts',(4.32866351767188,-6.90168043806902,
2.69277946972532));
#181169=CARTESIAN_POINT('Ctrl Pts',(7.72837761508381,-2.55255697681545,
2.90433609010723));
#181170=CARTESIAN_POINT('Ctrl Pts',(7.26456296350423,2.50129446334141,3.11589271048913));
#181171=CARTESIAN_POINT('Ctrl Pts',(4.51872136302912,6.76932144397021,3.32744933087104));
#181172=CARTESIAN_POINT('Ctrl Pts',(-0.837817077112605,8.10371735557139,
3.53900595125293));
#181173=CARTESIAN_POINT('Ctrl Pts',(-5.27618675114756,5.59028060557585,
3.75056257163485));
#181174=CARTESIAN_POINT('Ctrl Pts',(-7.3115171074744,2.41439254628121,3.90923003692127));
#181175=CARTESIAN_POINT('Ctrl Pts',(-7.57501656271908,-1.38960755105337,
4.0678975022077));
#181176=CARTESIAN_POINT('Ctrl Pts',(-5.98646912787849,-4.83395815802925,
4.22656496749413));
#181177=CARTESIAN_POINT('Ctrl Pts',(-2.953995989762,-7.11237001473912,4.38523243278056));
#181178=CARTESIAN_POINT('Ctrl Pts',(0.820160810533175,-7.65603515901766,
4.54389989806699));
#181179=CARTESIAN_POINT('Ctrl Pts',(4.35351193758964,-6.33532798549869,
4.70256736335343));
#181180=CARTESIAN_POINT('Ctrl Pts',(7.74543080566278,-2.52594026085192,
4.91412398373532));
#181181=CARTESIAN_POINT('Ctrl Pts',(7.56925871627352,2.99146858071628,5.12568060411723));
#181182=CARTESIAN_POINT('Ctrl Pts',(3.9753421002422,6.57473904852535,5.33723722449913));
#181183=CARTESIAN_POINT('Ctrl Pts',(-0.867401018491525,8.09260012782741,
5.54879384488104));
#181184=CARTESIAN_POINT('Ctrl Pts',(-5.83511030797489,5.68538137793315,
5.76035046526294));
#181185=CARTESIAN_POINT('Ctrl Pts',(-7.63267504629624,0.911985347858353,
5.97190708564485));
#181186=CARTESIAN_POINT('Ctrl Pts',(-7.1607183781963,-2.83048621457686,
6.13057455093128));
#181187=CARTESIAN_POINT('Ctrl Pts',(-4.92592076406795,-5.92006782319774,
6.28924201621771));
#181188=CARTESIAN_POINT('Ctrl Pts',(-1.49950799410512,-7.54694885824143,
6.44790948150413));
#181189=CARTESIAN_POINT('Ctrl Pts',(2.28858287895152,-7.3535220687151,6.60657694679056));
#181190=CARTESIAN_POINT('Ctrl Pts',(5.53474515659174,-5.35295581336359,
6.765244412077));
#181191=CARTESIAN_POINT('Ctrl Pts',(7.40155992801486,-2.07517621088562,
6.92391187736342));
#181192=CARTESIAN_POINT('Ctrl Pts',(7.56535131915662,3.02283526489178,7.13546849774533));
#181193=CARTESIAN_POINT('Ctrl Pts',(3.89522963664692,7.14631006586288,7.34702511812723));
#181194=CARTESIAN_POINT('Ctrl Pts',(-1.1599338351539,7.59507023368757,7.55858173850914));
#181195=CARTESIAN_POINT('Ctrl Pts',(-5.85071201799335,5.65789098181395,
7.77013835889103));
#181196=CARTESIAN_POINT('Ctrl Pts',(-8.12274874292138,0.626918240888216,
7.98169497927295));
#181197=CARTESIAN_POINT('Ctrl Pts',(-6.44475867260803,-4.1898128031289,
8.19325159965485));
#181198=CARTESIAN_POINT('Ctrl Pts',(-3.68468373269764,-6.76096484830223,
8.35191906494128));
#181199=CARTESIAN_POINT('Ctrl Pts',(0.0106361900308246,-7.70141449849661,
8.51058653022771));
#181200=CARTESIAN_POINT('Ctrl Pts',(3.68378227475696,-6.75534673041355,
8.66925399551413));
#181201=CARTESIAN_POINT('Ctrl Pts',(6.46840800132986,-4.17990386666028,
8.82792146080057));
#181202=CARTESIAN_POINT('Ctrl Pts',(7.6791481523861,-0.564113059316087,
8.98658892608699));
#181203=CARTESIAN_POINT('Ctrl Pts',(7.01253009361185,3.14862944145831,9.14525639137342));
#181204=CARTESIAN_POINT('Ctrl Pts',(3.87213373250231,7.16789048318619,9.35681301175533));
#181205=CARTESIAN_POINT('Ctrl Pts',(-1.58763536387134,7.98260455184212,
9.56836963213724));
#181206=CARTESIAN_POINT('Ctrl Pts',(-5.75656887614772,5.08846274729946,
9.77992625251913));
#181207=CARTESIAN_POINT('Ctrl Pts',(-8.11711560843863,0.595815138232739,
9.99148287290104));
#181208=CARTESIAN_POINT('Ctrl Pts',(-6.63840932843439,-4.72266822987694,
10.2030394932829));
#181209=CARTESIAN_POINT('Ctrl Pts',(-2.26407620738462,-7.34597880480092,
10.4145961136648));
#181210=CARTESIAN_POINT('Ctrl Pts',(1.5024152175209,-7.5518400674371,10.5732635789513));
#181211=CARTESIAN_POINT('Ctrl Pts',(4.94225399493611,-5.90643918581452,
10.7319310442377));
#181212=CARTESIAN_POINT('Ctrl Pts',(7.15642684923409,-2.82675008578538,
10.8905985095241));
#181213=CARTESIAN_POINT('Ctrl Pts',(7.64448494621918,0.934745052522767,
11.0492659748105));
#181214=CARTESIAN_POINT('Ctrl Pts',(6.25756902944692,4.48668805821105,11.207933440097));
#181215=CARTESIAN_POINT('Ctrl Pts',(3.36707696541851,6.91029944230909,11.3666009053834));
#181216=CARTESIAN_POINT('Ctrl Pts',(-1.61919470933465,7.98437737801743,
11.5781575257653));
#181217=CARTESIAN_POINT('Ctrl Pts',(-6.33324680367213,5.11200023508237,
11.7897141461472));
#181218=CARTESIAN_POINT('Ctrl Pts',(-7.68001396564619,0.218915152436606,
12.0012707665291));
#181219=CARTESIAN_POINT('Ctrl Pts',(-6.61415721494119,-4.74294062958273,
12.212827386911));
#181220=CARTESIAN_POINT('Ctrl Pts',(-2.0713778637849,-7.87917935871215,
12.4243840072929));
#181221=CARTESIAN_POINT('Ctrl Pts',(2.96798007047616,-7.0908772359057,12.6359406276748));
#181222=CARTESIAN_POINT('Ctrl Pts',(5.99183446497284,-4.83585149010497,
12.7946080929613));
#181223=CARTESIAN_POINT('Ctrl Pts',(7.57882695606709,-1.3686783318874,12.9532755582477));
#181224=CARTESIAN_POINT('Ctrl Pts',(7.30582649194216,2.4145104194355,13.1119430235341));
#181225=CARTESIAN_POINT('Ctrl Pts',(5.27067639815129,5.61532445297314,13.2706104888206));
#181226=CARTESIAN_POINT('Ctrl Pts',(1.93014946400685,7.45399644060694,13.429277954107));
#181227=CARTESIAN_POINT('Ctrl Pts',(-1.84195274867956,7.46301921108751,
13.5879454193934));
#181228=CARTESIAN_POINT('Ctrl Pts',(-6.35861431108908,5.09314221911649,
13.7995020397753));
#181229=CARTESIAN_POINT('Ctrl Pts',(-8.13787515437763,-0.132474342680147,
14.0110586601572));
#181230=CARTESIAN_POINT('Ctrl Pts',(-6.03707487698749,-4.75229053048462,
14.2226152805391));
#181231=CARTESIAN_POINT('Ctrl Pts',(-2.03976877603939,-7.87920711873978,
14.434171900921));
#181232=CARTESIAN_POINT('Ctrl Pts',(3.45754367989726,-7.37681945847504,
14.6457285213029));
#181233=CARTESIAN_POINT('Ctrl Pts',(6.82178922381607,-3.54297014653757,
14.8572851416848));
#181234=CARTESIAN_POINT('Ctrl Pts',(7.69881298645689,0.125771576874462,
15.0159526069713));
#181235=CARTESIAN_POINT('Ctrl Pts',(6.69600416270939,3.8046585469876,15.1746200722577));
#181236=CARTESIAN_POINT('Ctrl Pts',(4.06260417774054,6.53453966174601,15.3332875375441));
#181237=CARTESIAN_POINT('Ctrl Pts',(0.449312806741529,7.6883038706782,15.4919550028306));
#181238=CARTESIAN_POINT('Ctrl Pts',(-3.29357765252681,6.95987687655195,
15.650622468117));
#181239=CARTESIAN_POINT('Ctrl Pts',(-6.19563100519067,4.55012111058039,
15.8092899334034));
#181240=CARTESIAN_POINT('Ctrl Pts',(-8.14527086117322,-0.163206064397509,
16.0208465537853));
#181241=CARTESIAN_POINT('Ctrl Pts',(-6.16350136729878,-5.31543153234161,
16.2324031741672));
#181242=CARTESIAN_POINT('Ctrl Pts',(-1.59068667743553,-7.5166651016735,
16.4439597945491));
#181243=CARTESIAN_POINT('Ctrl Pts',(3.48183136358408,-7.35658968784228,
16.655516414931));
#181244=CARTESIAN_POINT('Ctrl Pts',(7.38087841990553,-3.44887044869859,
16.867073035313));
#181245=CARTESIAN_POINT('Ctrl Pts',(7.50774982071213,1.65019341382345,17.0786296556948));
#181246=CARTESIAN_POINT('Ctrl Pts',(5.83067758909786,5.02898983315523,17.2372971209813));
#181247=CARTESIAN_POINT('Ctrl Pts',(2.70374388530774,7.21121816400311,17.3959645862677));
#181248=CARTESIAN_POINT('Ctrl Pts',(-1.06717815138028,7.62011102866245,
17.5546320515542));
#181249=CARTESIAN_POINT('Ctrl Pts',(-4.58069911423817,6.19104950965544,
17.7132995168405));
#181250=CARTESIAN_POINT('Ctrl Pts',(-6.98785921309585,3.23378470339919,
17.871966982127));
#181251=CARTESIAN_POINT('Ctrl Pts',(-7.67223110931155,-0.475726264506312,
18.0306344474134));
#181252=CARTESIAN_POINT('Ctrl Pts',(-6.1494909136111,-5.34376600580041,
18.2421910677953));
#181253=CARTESIAN_POINT('Ctrl Pts',(-1.326969535103,-8.03005064321598,18.4537476881773));
#181254=CARTESIAN_POINT('Ctrl Pts',(3.59437202768935,-6.7905101489543,18.6653043085591));
#181255=CARTESIAN_POINT('Ctrl Pts',(7.38656617696681,-3.4177772883843,18.8768609289411));
#181256=CARTESIAN_POINT('Ctrl Pts',(7.87673918194969,2.08063775820587,19.0884175493229));
#181257=CARTESIAN_POINT('Ctrl Pts',(4.70732090140145,6.07705320074283,19.2999741697049));
#181258=CARTESIAN_POINT('Ctrl Pts',(1.25493822191392,7.59688554271855,19.4586416349913));
#181259=CARTESIAN_POINT('Ctrl Pts',(-2.54405960561978,7.26908929159913,
19.6173091002777));
#181260=CARTESIAN_POINT('Ctrl Pts',(-5.70139272614777,5.16711546979122,
19.7759765655641));
#181261=CARTESIAN_POINT('Ctrl Pts',(-7.48356218900576,1.81884451492439,
19.9346440308506));
#181262=CARTESIAN_POINT('Ctrl Pts',(-7.43717394831114,-1.99398684863986,
20.093311496137));
#181263=CARTESIAN_POINT('Ctrl Pts',(-5.58606117657983,-5.28065963729316,
20.2519789614235));
#181264=CARTESIAN_POINT('Ctrl Pts',(-1.29805898466894,-8.04283012960326,
20.4635355818053));
#181265=CARTESIAN_POINT('Ctrl Pts',(4.12576992068009,-7.01573831049282,
20.6750922021873));
#181266=CARTESIAN_POINT('Ctrl Pts',(7.11030466256198,-2.91103176932789,
20.8866488225691));
#181267=CARTESIAN_POINT('Ctrl Pts',(7.86118577672066,2.10815551219311,21.098205442951));
#181268=CARTESIAN_POINT('Ctrl Pts',(4.71486206491794,6.64395584950197,21.3097620633329));
#181269=CARTESIAN_POINT('Ctrl Pts',(-0.279056488753504,7.68189905879491,
21.5213186837149));
#181270=CARTESIAN_POINT('Ctrl Pts',(-3.90355943701511,6.63699959406936,
21.6799861490013));
#181271=CARTESIAN_POINT('Ctrl Pts',(-6.61047280658732,3.951398192989,21.8386536142877));
#181272=CARTESIAN_POINT('Ctrl Pts',(-7.68803961380581,0.314655672885429,
21.9973210795742));
#181273=CARTESIAN_POINT('Ctrl Pts',(-6.9112678087856,-3.39798111846303,
22.1559885448605));
#181274=CARTESIAN_POINT('Ctrl Pts',(-4.4328726330734,-6.29580654951658,
22.314656010147));
#181275=CARTESIAN_POINT('Ctrl Pts',(-0.905880310080676,-7.63340202905871,
22.4733234754334));
#181276=CARTESIAN_POINT('Ctrl Pts',(4.15615531497542,-7.00702837293636,
22.6848800958154));
#181277=CARTESIAN_POINT('Ctrl Pts',(7.66261695313574,-2.743512877539,22.8964367161972));
#181278=CARTESIAN_POINT('Ctrl Pts',(7.32441022213643,2.32024853288402,23.1079933365791));
#181279=CARTESIAN_POINT('Ctrl Pts',(4.68529006477581,6.65511972008154,23.319549956961));
#181280=CARTESIAN_POINT('Ctrl Pts',(-0.63646542886217,8.12200624102177,
23.5311065773429));
#181281=CARTESIAN_POINT('Ctrl Pts',(-5.13584783248266,5.71948535403429,
23.7426631977248));
#181282=CARTESIAN_POINT('Ctrl Pts',(-7.24935302054271,2.59507623655552,
23.9013306630113));
#181283=CARTESIAN_POINT('Ctrl Pts',(-7.60716689857828,-1.20121196437697,
24.0599981282977));
#181284=CARTESIAN_POINT('Ctrl Pts',(-6.1045754362536,-4.68392143817716,
24.2186655935842));
#181285=CARTESIAN_POINT('Ctrl Pts',(-3.12957351412315,-7.03687913963897,
24.3773330588706));
#181286=CARTESIAN_POINT('Ctrl Pts',(0.629931035558008,-7.67402937057367,
24.536000524157));
#181287=CARTESIAN_POINT('Ctrl Pts',(4.19496609421918,-6.44140552533228,
24.6946679894434));
#181288=CARTESIAN_POINT('Ctrl Pts',(7.68036706207295,-2.71735816799305,
24.9062246098253));
#181289=CARTESIAN_POINT('Ctrl Pts',(7.6411584945879,2.80272337919616,25.1177812302072));
#181290=CARTESIAN_POINT('Ctrl Pts',(4.13726405907001,6.47407016196261,25.3293378505891));
#181291=CARTESIAN_POINT('Ctrl Pts',(-0.666323612245312,8.11163203821956,
25.540894470971));
#181292=CARTESIAN_POINT('Ctrl Pts',(-5.69223613777299,5.82842357530445,
25.7524510913529));
#181293=CARTESIAN_POINT('Ctrl Pts',(-7.60769475643336,1.10110225064071,
25.9640077117349));
#181294=CARTESIAN_POINT('Ctrl Pts',(-7.22874935141058,-2.65192811072765,
26.1226751770213));
#181295=CARTESIAN_POINT('Ctrl Pts',(-5.0713049575923,-5.7960128047898,26.2813426423077));
#181296=CARTESIAN_POINT('Ctrl Pts',(-1.68631677165908,-7.50741613616482,
26.4400101075941));
#181297=CARTESIAN_POINT('Ctrl Pts',(2.10540739109427,-7.40804684945452,
26.5986775728806));
#181298=CARTESIAN_POINT('Ctrl Pts',(5.40021230923117,-5.48864709242768,
26.757345038167));
#181299=CARTESIAN_POINT('Ctrl Pts',(7.3477873030896,-2.2582000402942,26.9160125034534));
#181300=CARTESIAN_POINT('Ctrl Pts',(7.63803066288575,2.83417734345448,27.1275691238354));
#181301=CARTESIAN_POINT('Ctrl Pts',(4.07135925439712,7.04745310742402,27.3391257442172));
#181302=CARTESIAN_POINT('Ctrl Pts',(-0.971112084453145,7.62151426397118,
27.5506823645992));
#181303=CARTESIAN_POINT('Ctrl Pts',(-5.70851519721377,5.80132878941409,
27.7622389849811));
#181304=CARTESIAN_POINT('Ctrl Pts',(-8.10469122370494,0.828283640870579,
27.9737956053629));
#181305=CARTESIAN_POINT('Ctrl Pts',(-6.54674052494879,-4.02860201216538,
28.1853522257449));
#181306=CARTESIAN_POINT('Ctrl Pts',(-3.85131619862713,-6.66745104430312,
28.3440196910312));
#181307=CARTESIAN_POINT('Ctrl Pts',(-0.180470506885619,-7.69930703390452,
28.5026871563177));
#181308=CARTESIAN_POINT('Ctrl Pts',(3.51502034574916,-6.84467627173819,
28.6613546216041));
#181309=CARTESIAN_POINT('Ctrl Pts',(6.36269585437578,-4.33912432074682,
28.8200220868905));
#181310=CARTESIAN_POINT('Ctrl Pts',(7.66278567710082,-0.754490262896438,
28.978689552177));
#181311=CARTESIAN_POINT('Ctrl Pts',(7.08850112525183,2.97365052935496,29.1373570174634));
#181312=CARTESIAN_POINT('Ctrl Pts',(4.04880595981722,7.06959998310242,29.3489136378453));
#181313=CARTESIAN_POINT('Ctrl Pts',(-1.38906561400548,8.01954226871414,
29.5604702582273));
#181314=CARTESIAN_POINT('Ctrl Pts',(-5.62853087442155,5.22973981687144,
29.7720268786091));
#181315=CARTESIAN_POINT('Ctrl Pts',(-8.09983161825924,0.797050334391309,
29.9835834989911));
#181316=CARTESIAN_POINT('Ctrl Pts',(-6.75355386327359,-4.55648810348452,
30.1951401193729));
#181317=CARTESIAN_POINT('Ctrl Pts',(-2.44566267765865,-7.28753591692948,
30.4066967397549));
#181318=CARTESIAN_POINT('Ctrl Pts',(1.31456072747546,-7.58679576525994,
30.5653642050413));
#181319=CARTESIAN_POINT('Ctrl Pts',(4.79416941126681,-6.02725792232762,
30.7240316703277));
#181320=CARTESIAN_POINT('Ctrl Pts',(7.08408009972356,-3.00345974446586,
30.8826991356141));
#181321=CARTESIAN_POINT('Ctrl Pts',(7.66532591117842,0.744766461116509,
31.0413666009006));
#181322=CARTESIAN_POINT('Ctrl Pts',(6.36697520326575,4.33003079099741,31.200034066187));
#181323=CARTESIAN_POINT('Ctrl Pts',(3.53751282642449,6.82462077161154,31.3587015314734));
#181324=CARTESIAN_POINT('Ctrl Pts',(-1.42057125080021,8.02209766474667,
31.5702581518554));
#181325=CARTESIAN_POINT('Ctrl Pts',(-6.20444717254293,5.26757978229367,
31.7818147722372));
#181326=CARTESIAN_POINT('Ctrl Pts',(-7.6722169880436,0.409420132458434,
31.9933713926192));
#181327=CARTESIAN_POINT('Ctrl Pts',(-6.72981225810521,-4.57735605457585,
32.204928013001));
#181328=CARTESIAN_POINT('Ctrl Pts',(-2.26625454375591,-7.82535391942366,
32.416484633383));
#181329=CARTESIAN_POINT('Ctrl Pts',(2.7911126719703,-7.16234149742921,32.6280412537649));
#181330=CARTESIAN_POINT('Ctrl Pts',(5.86999233399055,-4.98304423910511,
32.7867087190513));
#181331=CARTESIAN_POINT('Ctrl Pts',(7.54253083406379,-1.55631841966368,
32.9453761843377));
#181332=CARTESIAN_POINT('Ctrl Pts',(7.3634907335968,2.23247967788305,33.1040436496241));
#181333=CARTESIAN_POINT('Ctrl Pts',(5.4083925124548,5.48280848082534,33.2627111149106));
#181334=CARTESIAN_POINT('Ctrl Pts',(2.11451911274058,7.4038063732003,33.421378580197));
#181335=CARTESIAN_POINT('Ctrl Pts',(-1.65619771621946,7.50642756564124,
33.5800460454834));
#181336=CARTESIAN_POINT('Ctrl Pts',(-6.23027481297625,5.24935704407002,
33.7916026658653));
#181337=CARTESIAN_POINT('Ctrl Pts',(-8.13865659658314,0.0695002345258844,
34.0031592862473));
#181338=CARTESIAN_POINT('Ctrl Pts',(-6.15313962233573,-4.60102283677544,
34.2147159066291));
#181339=CARTESIAN_POINT('Ctrl Pts',(-2.23465587780572,-7.82616602095135,
34.4262725270111));
#181340=CARTESIAN_POINT('Ctrl Pts',(3.27343014702295,-7.46034373832027,
34.6378291473929));
#181341=CARTESIAN_POINT('Ctrl Pts',(6.73177318153571,-3.71115554858403,
34.8493857677749));
#181342=CARTESIAN_POINT('Ctrl Pts',(7.6995633002137,-0.0653060180177375,
35.0080532330613));
#181343=CARTESIAN_POINT('Ctrl Pts',(6.78835140860278,3.63733192869553,35.1667206983477));
#181344=CARTESIAN_POINT('Ctrl Pts',(4.22350174583183,6.43171783420898,35.3253881636342));
#181345=CARTESIAN_POINT('Ctrl Pts',(0.639952549815799,7.67478723745301,
35.4840556289205));
#181346=CARTESIAN_POINT('Ctrl Pts',(-3.1198606489942,7.03946087572367,35.6427230942071));
#181347=CARTESIAN_POINT('Ctrl Pts',(-6.08081625493652,4.70245886182211,
35.8013905594934));
#181348=CARTESIAN_POINT('Ctrl Pts',(-8.14681260514703,0.0389614931793878,
36.0129471798754));
#181349=CARTESIAN_POINT('Ctrl Pts',(-6.29350100288451,-5.16085328278152,
36.2245038002573));
#181350=CARTESIAN_POINT('Ctrl Pts',(-1.77671591673179,-7.47487919017552,
36.4360604206391));
#181351=CARTESIAN_POINT('Ctrl Pts',(3.29821233503487,-7.44072287299623,
36.6476170410211));
#181352=CARTESIAN_POINT('Ctrl Pts',(7.29302522118576,-3.63095810282656,
36.859173661403));
#181353=CARTESIAN_POINT('Ctrl Pts',(7.54638607283336,1.46338747882308,37.0707302817849));
#181354=CARTESIAN_POINT('Ctrl Pts',(5.95367192282226,4.88275849550071,37.2293977470713));
#181355=CARTESIAN_POINT('Ctrl Pts',(2.88185101501516,7.14190682755269,37.3880652123578));
#181356=CARTESIAN_POINT('Ctrl Pts',(-0.877763597696466,7.64424570265017,
37.5467326776441));
#181357=CARTESIAN_POINT('Ctrl Pts',(-4.42566351935687,6.30280896264681,
37.7054001429306));
#181358=CARTESIAN_POINT('Ctrl Pts',(-6.90546418370667,3.40618618069116,
37.864067608217));
#181359=CARTESIAN_POINT('Ctrl Pts',(-7.68167340742512,-0.285200517333806,
38.0227350735034));
#181360=CARTESIAN_POINT('Ctrl Pts',(-6.28019795679177,-5.18952668794002,
38.2342916938854));
#181361=CARTESIAN_POINT('Ctrl Pts',(-1.52581916088684,-7.994650546958,38.4458483142672));
#181362=CARTESIAN_POINT('Ctrl Pts',(3.42476508210843,-6.87761023094924,
38.6574049346492));
#181363=CARTESIAN_POINT('Ctrl Pts',(7.29948277468298,-3.60001565299542,
38.8689615550311));
#181364=CARTESIAN_POINT('Ctrl Pts',(7.92594289136418,1.88454315529457,39.0805181754129));
#181365=CARTESIAN_POINT('Ctrl Pts',(4.85666785056708,5.95837419626339,39.2920747957949));
#181366=CARTESIAN_POINT('Ctrl Pts',(1.44306143912829,7.56340621498592,39.4507422610813));
#181367=CARTESIAN_POINT('Ctrl Pts',(-2.36290057313157,7.32997948753485,
39.6094097263677));
#181368=CARTESIAN_POINT('Ctrl Pts',(-5.57142002007046,5.30699917617148,
39.7680771916542));
#181369=CARTESIAN_POINT('Ctrl Pts',(-7.43612494637858,2.00398208276263,
39.9267446569406));
#181370=CARTESIAN_POINT('Ctrl Pts',(-7.48436284551581,-1.80882632849291,
40.085412122227));
#181371=CARTESIAN_POINT('Ctrl Pts',(-5.71537578330039,-5.14042073463766,
40.2440795875134));
#181372=CARTESIAN_POINT('Ctrl Pts',(-1.49723462352733,-8.00814348669179,
40.4556362078954));
#181373=CARTESIAN_POINT('Ctrl Pts',(3.95041052209858,-7.11595518441463,
40.6671928282772));
#181374=CARTESIAN_POINT('Ctrl Pts',(7.03588074341516,-3.08657099722778,
40.8787494486592));
#181375=CARTESIAN_POINT('Ctrl Pts',(7.91107710269774,1.91243837936691,41.090306069041));
#181376=CARTESIAN_POINT('Ctrl Pts',(4.87827385282309,6.52491515946354,41.301862689423));
#181377=CARTESIAN_POINT('Ctrl Pts',(-0.0883513982737931,7.68645820283012,
41.5134193098049));
#181378=CARTESIAN_POINT('Ctrl Pts',(-3.7376665088871,6.73181914183104,41.6720867750913));
#181379=CARTESIAN_POINT('Ctrl Pts',(-6.51038707084204,4.11421421343349,
41.8307542403778));
#181380=CARTESIAN_POINT('Ctrl Pts',(-7.67786445320275,0.505330321808945,
41.9894217056641));
#181381=CARTESIAN_POINT('Ctrl Pts',(-6.99345745017656,-3.22543815609603,
42.1480891709506));
#181382=CARTESIAN_POINT('Ctrl Pts',(-4.58773224978883,-6.18387036524922,
42.306756636237));
#181383=CARTESIAN_POINT('Ctrl Pts',(-1.09501713052869,-7.60857300400148,
42.4654241015234));
#181384=CARTESIAN_POINT('Ctrl Pts',(3.98100268924364,-7.108001914039,42.6769807219053));
#181385=CARTESIAN_POINT('Ctrl Pts',(7.59217979307386,-2.93280880187554,
42.8885373422872));
#181386=CARTESIAN_POINT('Ctrl Pts',(7.37972972077339,2.13778567814032,43.1000939626691));
#181387=CARTESIAN_POINT('Ctrl Pts',(4.8489879792647,6.53680939419379,43.311650583051));
#181388=CARTESIAN_POINT('Ctrl Pts',(-0.43472943651037,8.13529863838765,
43.523207203433));
#181389=CARTESIAN_POINT('Ctrl Pts',(-4.99234272356322,5.84516550749184,
43.7347638238148));
#181390=CARTESIAN_POINT('Ctrl Pts',(-7.18272642731095,2.77416310735713,
43.8934312891013));
#181391=CARTESIAN_POINT('Ctrl Pts',(-7.63463148404488,-1.0120773352815,
44.0520987543877));
#181392=CARTESIAN_POINT('Ctrl Pts',(-6.21892287865747,-4.53099983435654,
44.2107662196742));
#181393=CARTESIAN_POINT('Ctrl Pts',(-3.30322346942185,-6.95705491712383,
44.3694336849606));
#181394=CARTESIAN_POINT('Ctrl Pts',(0.439313195026434,-7.6872975674912,
44.528101150247));
#181395=CARTESIAN_POINT('Ctrl Pts',(4.03383690204582,-6.54351627557473,
44.6867686155335));
#181396=CARTESIAN_POINT('Ctrl Pts',(7.61057348568299,-2.90710261789513,
44.8983252359153));
#181397=CARTESIAN_POINT('Ctrl Pts',(7.70835253972146,2.61225218709017,45.1098818562973));
#181398=CARTESIAN_POINT('Ctrl Pts',(4.29663824397178,6.36941429430586,45.3214384766791));
#181399=CARTESIAN_POINT('Ctrl Pts',(-0.464836099980491,8.12566864264212,
45.532995097061));
#181400=CARTESIAN_POINT('Ctrl Pts',(-5.54585601130899,5.96787622243531,
45.744551717443));
#181401=CARTESIAN_POINT('Ctrl Pts',(-7.57803000839963,1.28954132789886,
45.9561083378248));
#181402=CARTESIAN_POINT('Ctrl Pts',(-7.29232733490318,-2.4717374329718,
46.1147758031113));
#181403=CARTESIAN_POINT('Ctrl Pts',(-5.21356858587787,-5.66838730039252,
46.2734432683977));
#181404=CARTESIAN_POINT('Ctrl Pts',(-1.87208228136461,-7.4632622167643,
46.4321107336842));
#181405=CARTESIAN_POINT('Ctrl Pts',(1.92092630474857,-7.458005518932,46.5907781989705));
#181406=CARTESIAN_POINT('Ctrl Pts',(5.262370667903,-5.62096573551653,46.7494456642571));
#181407=CARTESIAN_POINT('Ctrl Pts',(7.28945957893753,-2.43981987392297,
46.9081131295434));
#181408=CARTESIAN_POINT('Ctrl Pts',(7.70607428550732,2.64374392443121,47.1196697499254));
#181409=CARTESIAN_POINT('Ctrl Pts',(4.24485140895422,6.94431373400415,47.3312263703072));
#181410=CARTESIAN_POINT('Ctrl Pts',(-0.781539047599859,7.64319687039387,
47.5427829906891));
#181411=CARTESIAN_POINT('Ctrl Pts',(-5.56318172248103,5.94136167142255,
47.754339611071));
#181412=CARTESIAN_POINT('Ctrl Pts',(-8.08088365047604,1.02880295755603,
47.965896231453));
#181413=CARTESIAN_POINT('Ctrl Pts',(-6.64562737011112,-3.86449556348911,
48.1774528518348));
#181414=CARTESIAN_POINT('Ctrl Pts',(-4.01360255146483,-6.57070544212201,
48.3361203171214));
#181415=CARTESIAN_POINT('Ctrl Pts',(-0.375301096671435,-7.69075902680454,
48.4947877824077));
#181416=CARTESIAN_POINT('Ctrl Pts',(3.35132729979093,-6.93300286965634,
48.6534552476943));
#181417=CARTESIAN_POINT('Ctrl Pts',(6.23994166064972,-4.48978335266614,
48.8121227129805));
#181418=CARTESIAN_POINT('Ctrl Pts',(8.13618217215324,0.224578706766124,
49.0236793333626));
#181419=CARTESIAN_POINT('Ctrl Pts',(5.62429464528615,6.67951083364511,49.2881251088398));
#181420=CARTESIAN_POINT('Ctrl Pts',(-2.5847595412482,8.34284628442979,49.6054600394127));
#181421=CARTESIAN_POINT('Ctrl Pts',(-7.40911245697885,3.36713261308933,
49.8699058148902));
#181422=CARTESIAN_POINT('Ctrl Pts',(-7.49433490111638,-1.70715495593281,
50.0814624352719));
#181423=CARTESIAN_POINT('Ctrl Pts',(-5.78340036009558,-5.09230476755583,
50.2401299005585));
#181424=CARTESIAN_POINT('Ctrl Pts',(-2.64334519062654,-7.2175551378715,
50.3987973658448));
#181425=CARTESIAN_POINT('Ctrl Pts',(2.40330882384813,-7.7760867127584,50.6103539862269));
#181426=CARTESIAN_POINT('Ctrl Pts',(7.94480546051037,-3.62041707533747,
50.8747997617041));
#181427=CARTESIAN_POINT('Ctrl Pts',(7.34416496708709,4.73282184451775,51.1921346922771));
#181428=CARTESIAN_POINT('Ctrl Pts',(1.24296098202915,8.04250887686602,51.4565804677543));
#181429=CARTESIAN_POINT('Ctrl Pts',(-3.64947415302537,6.75792830578459,
51.6681370881364));
#181430=CARTESIAN_POINT('Ctrl Pts',(-7.42111176510748,3.35217510381507,
51.8796937085182));
#181431=CARTESIAN_POINT('Ctrl Pts',(-7.8555980481714,-2.1507922957559,52.0912503289001));
#181432=CARTESIAN_POINT('Ctrl Pts',(-4.65407611661369,-6.1186429968107,
52.302806949282));
#181433=CARTESIAN_POINT('Ctrl Pts',(-1.18670892066426,-7.60778721220126,
52.4614744145685));
#181434=CARTESIAN_POINT('Ctrl Pts',(2.60834208613747,-7.24614259843243,
52.6201418798549));
#181435=CARTESIAN_POINT('Ctrl Pts',(5.74731330180241,-5.1161820899732,52.7788093451413));
#181436=CARTESIAN_POINT('Ctrl Pts',(7.49936692377579,-1.75216872725107,
52.9374768104277));
#181437=CARTESIAN_POINT('Ctrl Pts',(7.41917818290533,2.0600910566469,53.0961442757142));
#181438=CARTESIAN_POINT('Ctrl Pts',(5.53882487318358,5.33016393210911,53.2548117410006));
#181439=CARTESIAN_POINT('Ctrl Pts',(1.22644870252003,8.05406246753895,53.4663683613825));
#181440=CARTESIAN_POINT('Ctrl Pts',(-4.18805026979504,6.97874443945398,
53.6779249817644));
#181441=CARTESIAN_POINT('Ctrl Pts',(-7.13592590189922,2.84763939769702,
53.8894816021462));
#181442=CARTESIAN_POINT('Ctrl Pts',(-7.84211621237246,-2.17803107982334,
54.1010382225283));
#181443=CARTESIAN_POINT('Ctrl Pts',(-4.65554714393779,-6.68565191717772,
54.31259484291));
#181444=CARTESIAN_POINT('Ctrl Pts',(0.347408463441009,-7.67911140378827,
54.5241514632921));
#181445=CARTESIAN_POINT('Ctrl Pts',(3.96247002766141,-6.60199776048994,
54.6828189285784));
#181446=CARTESIAN_POINT('Ctrl Pts',(6.64537559819868,-3.89241298024765,
54.841486393865));
#181447=CARTESIAN_POINT('Ctrl Pts',(7.69053549766263,-0.246224878623426,
55.0001538591513));
#181448=CARTESIAN_POINT('Ctrl Pts',(6.88075434028287,3.45935216052283,55.1588213244378));
#181449=CARTESIAN_POINT('Ctrl Pts',(4.37666871111325,6.33500679653603,55.3174887897242));
#181450=CARTESIAN_POINT('Ctrl Pts',(0.837912320965971,7.64116146966611,
55.4761562550106));
#181451=CARTESIAN_POINT('Ctrl Pts',(-4.21834852326479,6.96976393111749,
55.6877128753925));
#181452=CARTESIAN_POINT('Ctrl Pts',(-7.6867289255209,2.67521213953418,55.8992694957745));
#181453=CARTESIAN_POINT('Ctrl Pts',(-7.3034715361975,-2.38533893705042,
56.1108261161562));
#181454=CARTESIAN_POINT('Ctrl Pts',(-4.62587847676516,-6.69655208400989,
56.3223827365383));
#181455=CARTESIAN_POINT('Ctrl Pts',(0.708720575099877,-8.1160205008443,
56.53393935692));
#181456=CARTESIAN_POINT('Ctrl Pts',(5.18654399580368,-5.67355330002261,
56.7454959773021));
#181457=CARTESIAN_POINT('Ctrl Pts',(7.27216036735544,-2.53045914511118,
56.9041634425884));
#181458=CARTESIAN_POINT('Ctrl Pts',(7.59617568443146,1.26886302470831,57.0628309078749));
#181459=CARTESIAN_POINT('Ctrl Pts',(6.06264997138618,4.73806253875762,57.2214983731613));
#181460=CARTESIAN_POINT('Ctrl Pts',(3.06682613015959,7.06445156352318,57.3801658384477));
#181461=CARTESIAN_POINT('Ctrl Pts',(-0.698199749115411,7.66811952177836,
57.5388333037342));
#181462=CARTESIAN_POINT('Ctrl Pts',(-4.25212411675666,6.40381809307606,
57.6975007690206));
#181463=CARTESIAN_POINT('Ctrl Pts',(-7.704245566873,2.64890050144179,57.9090573894025));
#181464=CARTESIAN_POINT('Ctrl Pts',(-7.6159135686908,-2.87061352222651,
58.1206140097845));
#181465=CARTESIAN_POINT('Ctrl Pts',(-4.07948538918484,-6.51063263561258,
58.3321706301662));
#181466=CARTESIAN_POINT('Ctrl Pts',(0.738485251746679,-8.10538099120919,
58.5437272505483));
#181467=CARTESIAN_POINT('Ctrl Pts',(5.74387974500619,-5.77753572868652,
58.7552838709301));
#181468=CARTESIAN_POINT('Ctrl Pts',(7.61719255714318,-1.03335532167188,
58.9668404913121));
#181469=CARTESIAN_POINT('Ctrl Pts',(7.20486273246497,2.71615406343716,59.1255079565984));
#181470=CARTESIAN_POINT('Ctrl Pts',(5.01952355070286,5.8409144600932,59.2841754218849));
#181471=CARTESIAN_POINT('Ctrl Pts',(1.61943908007662,7.52212592036633,59.4428428871712));
#181472=CARTESIAN_POINT('Ctrl Pts',(-2.17125061206326,7.38901679425637,
59.6015103524578));
#181473=CARTESIAN_POINT('Ctrl Pts',(-5.44884370019278,5.44037151496626,
59.7601778177441));
#181474=CARTESIAN_POINT('Ctrl Pts',(-7.3675927819281,2.19272029066876,59.9188452830306));
#181475=CARTESIAN_POINT('Ctrl Pts',(-7.61250594188919,-2.90203840533433,
60.1304019034125));
#181476=CARTESIAN_POINT('Ctrl Pts',(-4.00848047484515,-7.08340636717186,
60.3419585237944));
#181477=CARTESIAN_POINT('Ctrl Pts',(1.03889993849945,-7.61257021473515,
60.5535151441763));
#181478=CARTESIAN_POINT('Ctrl Pts',(5.75991703457443,-5.75029714315045,
60.7650717645582));
#181479=CARTESIAN_POINT('Ctrl Pts',(8.111741442813,-0.756124583837398,60.9766283849402));
#181480=CARTESIAN_POINT('Ctrl Pts',(6.51062944899396,4.08670403275333,61.188185005322));
#181481=CARTESIAN_POINT('Ctrl Pts',(3.79182789345968,6.70146111802254,61.3468524706085));
#181482=CARTESIAN_POINT('Ctrl Pts',(0.111944747544373,7.70060820842643,
61.5055199358949));
#181483=CARTESIAN_POINT('Ctrl Pts',(-3.57579413020001,6.81312392624366,
61.6641874011813));
#181484=CARTESIAN_POINT('Ctrl Pts',(-6.40105915789561,4.28232881307684,
61.8228548664678));
#181485=CARTESIAN_POINT('Ctrl Pts',(-7.66919668452351,0.686266787831419,
61.9815223317541));
#181486=CARTESIAN_POINT('Ctrl Pts',(-7.06175694869098,-3.03661562780735,
62.1401897970406));
#181487=CARTESIAN_POINT('Ctrl Pts',(-3.98573098119137,-7.10535165680803,
62.3517464174224));
#181488=CARTESIAN_POINT('Ctrl Pts',(1.46037909659013,-8.00686295461261,
62.5633030378044));
#181489=CARTESIAN_POINT('Ctrl Pts',(5.67484912480221,-5.17944261163483,
62.7748596581863));
#181490=CARTESIAN_POINT('Ctrl Pts',(8.1066040745539,-0.72493576138295,62.9864162785683));
#181491=CARTESIAN_POINT('Ctrl Pts',(6.71273676923672,4.61640971841437,63.1979728989501));
#181492=CARTESIAN_POINT('Ctrl Pts',(2.38071170104819,7.30901207208755,63.409529519332));
#181493=CARTESIAN_POINT('Ctrl Pts',(-1.38202600994047,7.5747966307905,63.5681969846185));
#181494=CARTESIAN_POINT('Ctrl Pts',(-4.8476180726037,5.98435438692876,63.7268644499048));
#181495=CARTESIAN_POINT('Ctrl Pts',(-7.11052832740991,2.9402972980683,63.8855319151914));
#181496=CARTESIAN_POINT('Ctrl Pts',(-7.65839444960578,-0.812953172350435,
64.0441993804778));
#181497=CARTESIAN_POINT('Ctrl Pts',(-6.32818873419878,-4.38652108559234,
64.2028668457641));
#181498=CARTESIAN_POINT('Ctrl Pts',(-3.47663824377446,-6.85583198418356,
64.3615343110507));
#181499=CARTESIAN_POINT('Ctrl Pts',(1.49190622706167,-8.00913787064428,
64.5730909314324));
#181500=CARTESIAN_POINT('Ctrl Pts',(6.25107936682005,-5.21215581400079,
64.7846475518145));
#181501=CARTESIAN_POINT('Ctrl Pts',(7.67555673177271,-0.341126389811259,
64.9962041721963));
#181502=CARTESIAN_POINT('Ctrl Pts',(6.68881039361302,4.63706555894997,65.2077607925782));
#181503=CARTESIAN_POINT('Ctrl Pts',(2.19652445606137,7.84521216636351,65.4193174129601));
#181504=CARTESIAN_POINT('Ctrl Pts',(-2.85474212812762,7.13721885998481,
65.630874033342));
#181505=CARTESIAN_POINT('Ctrl Pts',(-5.91410559916608,4.93060795966368,
65.7895414986284));
#181506=CARTESIAN_POINT('Ctrl Pts',(-7.55608233053341,1.48913337897857,
65.9482089639149));
#181507=CARTESIAN_POINT('Ctrl Pts',(-7.34333158560759,-2.29792134759746,
66.1068764292013));
#181508=CARTESIAN_POINT('Ctrl Pts',(-5.35938506312473,-5.53072238964705,
66.2655438944878));
#181509=CARTESIAN_POINT('Ctrl Pts',(-2.04854652109898,-7.42233097085277,
66.4242113597741));
#181510=CARTESIAN_POINT('Ctrl Pts',(1.72293424745511,-7.49139127614996,
66.5828788250607));
#181511=CARTESIAN_POINT('Ctrl Pts',(6.27674381446943,-5.19370394890329,
66.7944354454424));
#181512=CARTESIAN_POINT('Ctrl Pts',(8.1389528127818,0.00293104366527835,
67.0059920658245));
#181513=CARTESIAN_POINT('Ctrl Pts',(6.1119499756196,4.65559940845542,67.2175486862063));
#181514=CARTESIAN_POINT('Ctrl Pts',(2.16491981425747,7.84574302902793,67.4291053065882));
#181515=CARTESIAN_POINT('Ctrl Pts',(-3.33969252143794,7.43091700152713,
67.6406619269702));
#181516=CARTESIAN_POINT('Ctrl Pts',(-6.764533373353,3.65110037032991,67.852218547352));
#181517=CARTESIAN_POINT('Ctrl Pts',(-7.69983957871388,-0.00321746143493831,
68.0108860126386));
#181518=CARTESIAN_POINT('Ctrl Pts',(-6.75571280339331,-3.69759961654247,
68.1695534779248));
#181519=CARTESIAN_POINT('Ctrl Pts',(-4.16609656796089,-6.46904944194669,
68.3282209432115));
#181520=CARTESIAN_POINT('Ctrl Pts',(-0.571626804665265,-7.68017846162284,
68.4868884084976));
#181521=CARTESIAN_POINT('Ctrl Pts',(3.18238353258899,-7.01141747020483,
68.6455558737843));
#181522=CARTESIAN_POINT('Ctrl Pts',(6.12242415190615,-4.64815750352609,
68.8042233390705));
#181523=CARTESIAN_POINT('Ctrl Pts',(8.14683672427592,0.0335411586319285,
69.0157799594527));
#181524=CARTESIAN_POINT('Ctrl Pts',(6.24732368646782,5.21665680644255,69.2273365798343));
#181525=CARTESIAN_POINT('Ctrl Pts',(1.71012420212608,7.49039475393584,69.4388932002164));
#181526=CARTESIAN_POINT('Ctrl Pts',(-3.3642991156822,7.41107636851257,69.6504498205982));
#181527=CARTESIAN_POINT('Ctrl Pts',(-7.32504948466601,3.56591133772674,
69.8620064409801));
#181528=CARTESIAN_POINT('Ctrl Pts',(-7.53306408138971,-1.53048724891962,
70.073563061362));
#181529=CARTESIAN_POINT('Ctrl Pts',(-5.90998291862105,-4.93554878322507,
70.2322305266485));
#181530=CARTESIAN_POINT('Ctrl Pts',(-2.81817876561956,-7.16727053006921,
70.3908979919348));
#181531=CARTESIAN_POINT('Ctrl Pts',(0.945757442712733,-7.63613149150012,
70.5495654572214));
#181532=CARTESIAN_POINT('Ctrl Pts',(4.48157899088049,-6.26317396810003,
70.7082329225078));
#181533=CARTESIAN_POINT('Ctrl Pts',(6.93550347678732,-3.34459734698479,
70.8669003877941));
#181534=CARTESIAN_POINT('Ctrl Pts',(7.67883112382652,0.353550908897835,
71.0255678530808));
#181535=CARTESIAN_POINT('Ctrl Pts',(6.2337659933061,5.24521068805003,71.2371244734623));
#181536=CARTESIAN_POINT('Ctrl Pts',(1.45461176904061,8.00791271687411,71.4486810938446));
#181537=CARTESIAN_POINT('Ctrl Pts',(-3.48583553055409,6.84685979193482,
71.6602377142262));
#181538=CARTESIAN_POINT('Ctrl Pts',(-7.33123141562007,3.53491264536072,
71.8717943346083));
#181539=CARTESIAN_POINT('Ctrl Pts',(-7.90885786957273,-1.95500404609076,
72.0833509549901));
#181540=CARTESIAN_POINT('Ctrl Pts',(-4.80345003694453,-6.00135929735981,
72.2949075753721));
#181541=CARTESIAN_POINT('Ctrl Pts',(-1.37569510665384,-7.57594897445298,
72.4535750406583));
#181542=CARTESIAN_POINT('Ctrl Pts',(2.42803885084062,-7.30866100903549,
72.6122425059449));
#181543=CARTESIAN_POINT('Ctrl Pts',(5.61842808794537,-5.25720715936825,
72.7709099712313));
#181544=CARTESIAN_POINT('Ctrl Pts',(7.45366455959685,-1.93772625496934,
72.9295774365178));
#181545=CARTESIAN_POINT('Ctrl Pts',(7.46796913860933,1.8753604546235,73.0882449018041));
#181546=CARTESIAN_POINT('Ctrl Pts',(5.66940319632406,5.19108014491588,73.2469123670907));
#181547=CARTESIAN_POINT('Ctrl Pts',(1.42590828560569,8.02115073928762,73.4584689874725));
#181548=CARTESIAN_POINT('Ctrl Pts',(-4.01358126361283,7.08051741895192,
73.6700256078544));
#181549=CARTESIAN_POINT('Ctrl Pts',(-7.06307051358718,3.023834201239,73.8815822282364));
#181550=CARTESIAN_POINT('Ctrl Pts',(-7.89374442100557,-1.98276587007854,
74.0931388486181));
#181551=CARTESIAN_POINT('Ctrl Pts',(-4.82001335312958,-6.56807010445122,
74.3046954690001));
#181552=CARTESIAN_POINT('Ctrl Pts',(0.156752166448748,-7.68536755345788,
74.516252089382));
#181553=CARTESIAN_POINT('Ctrl Pts',(3.79742712466257,-6.69828986554504,
74.6749195546685));
#181554=CARTESIAN_POINT('Ctrl Pts',(6.54674297835105,-4.05611326045006,
74.8335870199548));
#181555=CARTESIAN_POINT('Ctrl Pts',(7.68205750895736,-0.436982522532017,
74.9922544852414));
#181556=CARTESIAN_POINT('Ctrl Pts',(6.96447629814245,3.28754745955083,75.1509219505277));
#181557=CARTESIAN_POINT('Ctrl Pts',(4.53251832293027,6.2244531922321,75.3095894158142));
#181558=CARTESIAN_POINT('Ctrl Pts',(1.02726262670822,7.61801661649528,75.4682568811006));
#181559=CARTESIAN_POINT('Ctrl Pts',(-4.04410144057219,7.07229221396395,
75.6798135014825));
#181560=CARTESIAN_POINT('Ctrl Pts',(-7.61797915470459,2.86512741046386,
75.8913701218644));
#181561=CARTESIAN_POINT('Ctrl Pts',(-7.36041264205738,-2.20337561371838,
76.1029267422464));
#181562=CARTESIAN_POINT('Ctrl Pts',(-4.7906227888216,-6.5797032436827,76.3144833626282));
#181563=CARTESIAN_POINT('Ctrl Pts',(0.507110864105959,-8.13110768547802,
76.5260399830101));
#181564=CARTESIAN_POINT('Ctrl Pts',(5.04416303784523,-5.8005055746086,76.7375966033921));
#181565=CARTESIAN_POINT('Ctrl Pts',(7.2071301648577,-2.71013185597771,76.8962640686785));
#181566=CARTESIAN_POINT('Ctrl Pts',(7.62532235076434,1.07998030219135,77.0549315339649));
#181567=CARTESIAN_POINT('Ctrl Pts',(6.17835378732253,4.58616460395872,77.2135989992513));
#181568=CARTESIAN_POINT('Ctrl Pts',(3.24117958454841,6.98617587145457,77.3722664645377));
#181569=CARTESIAN_POINT('Ctrl Pts',(-0.507707523942078,7.68308355805921,
77.5309339298242));
#181570=CARTESIAN_POINT('Ctrl Pts',(-4.09191004142901,6.50735874885361,
77.6896013951107));
#181571=CARTESIAN_POINT('Ctrl Pts',(-7.63614330666086,2.83925853374987,
77.9011580154925));
#181572=CARTESIAN_POINT('Ctrl Pts',(-7.68480010278568,-2.68074781729478,
78.1127146358744));
#181573=CARTESIAN_POINT('Ctrl Pts',(-4.23978452870737,-6.4073992779146,
78.3242712562563));
#181574=CARTESIAN_POINT('Ctrl Pts',(0.537130386221318,-8.12121003471172,
78.5358278766383));
#181575=CARTESIAN_POINT('Ctrl Pts',(5.59874694676139,-5.91828575243403,
78.74738449702));
#181576=CARTESIAN_POINT('Ctrl Pts',(7.58920534966798,-1.22205066752606,
78.9589411174022));
#181577=CARTESIAN_POINT('Ctrl Pts',(7.27004306836239,2.53653576244122,79.1176085826884));
#181578=CARTESIAN_POINT('Ctrl Pts',(5.1629148048253,5.71456114888126,79.2762760479749));
#181579=CARTESIAN_POINT('Ctrl Pts',(1.80559497116204,7.47962486332303,79.4349435132613));
#181580=CARTESIAN_POINT('Ctrl Pts',(-1.98723048438653,7.44061915488974,
79.5936109785478));
#181581=CARTESIAN_POINT('Ctrl Pts',(-5.3121681640557,5.57390431266812,79.7522784438342));
#181582=CARTESIAN_POINT('Ctrl Pts',(-7.31091386931737,2.37486506329353,
79.9109459091206));
#181583=CARTESIAN_POINT('Ctrl Pts',(-7.68217330443316,-2.71224758124834,
80.1225025295025));
#181584=CARTESIAN_POINT('Ctrl Pts',(-4.18301432417714,-6.98175856381715,
80.3340591498844));
#181585=CARTESIAN_POINT('Ctrl Pts',(0.849681210409256,-7.63600551317016,
80.5456157702664));
#181586=CARTESIAN_POINT('Ctrl Pts',(5.61545519829567,-5.8914535044961,80.7571723906482));
#181587=CARTESIAN_POINT('Ctrl Pts',(8.09048117796806,-0.957177063179817,
80.9687290110302));
#181588=CARTESIAN_POINT('Ctrl Pts',(6.61003247061829,3.92389046875689,81.1802856314119));
#181589=CARTESIAN_POINT('Ctrl Pts',(3.95695083834681,6.60530695372241,81.3389530966986));
#181590=CARTESIAN_POINT('Ctrl Pts',(0.302993692444209,7.69545926040326,
81.4976205619847));
#181591=CARTESIAN_POINT('Ctrl Pts',(-3.40563176525438,6.89975605187724,
81.6562880272715));
#181592=CARTESIAN_POINT('Ctrl Pts',(-6.2928261691851,4.43984653007363,81.8149554925576));
#181593=CARTESIAN_POINT('Ctrl Pts',(-7.64980614255145,0.876359441878015,
81.9736229578442));
#181594=CARTESIAN_POINT('Ctrl Pts',(-7.13493330420416,-2.86044968807139,
82.1322904231306));
#181595=CARTESIAN_POINT('Ctrl Pts',(-4.16081638737094,-7.00426160361813,
82.3438470435126));
#181596=CARTESIAN_POINT('Ctrl Pts',(1.26124658136258,-8.04063545627494,
82.5554036638944));
#181597=CARTESIAN_POINT('Ctrl Pts',(5.54457870540081,-5.31866386756137,
82.7669602842763));
#181598=CARTESIAN_POINT('Ctrl Pts',(8.08611931314516,-0.925870365270548,
82.9785169046583));
#181599=CARTESIAN_POINT('Ctrl Pts',(6.82522171152634,4.44841794460044,83.1900735250401));
#181600=CARTESIAN_POINT('Ctrl Pts',(2.56134496232852,7.24768636582629,83.4016301454221));
#181601=CARTESIAN_POINT('Ctrl Pts',(-1.19363894398475,7.60675791394662,
83.5602976107085));
#181602=CARTESIAN_POINT('Ctrl Pts',(-4.69762923579942,6.1028008298772,83.7189650759949));
#181603=CARTESIAN_POINT('Ctrl Pts',(-7.03537814257748,3.11583306466665,
83.8776325412813));
#181604=CARTESIAN_POINT('Ctrl Pts',(-7.67620897962355,-0.622666931299617,
84.0363000065679));
#181605=CARTESIAN_POINT('Ctrl Pts',(-6.43508761299876,-4.22814229928651,
84.194967471854));
#181606=CARTESIAN_POINT('Ctrl Pts',(-3.64568880986591,-6.76745142391492,
84.3536349371408));
#181607=CARTESIAN_POINT('Ctrl Pts',(1.29270755419318,-8.04369198817716,
84.5651915575224));
#181608=CARTESIAN_POINT('Ctrl Pts',(6.11981976906105,-5.36566561331532,
84.7767481779045));
#181609=CARTESIAN_POINT('Ctrl Pts',(7.66472856868996,-0.531483136886555,
84.9883047982863));
#181610=CARTESIAN_POINT('Ctrl Pts',(6.80181525865428,4.46966113557217,85.1998614186682));
#181611=CARTESIAN_POINT('Ctrl Pts',(2.39051973713001,7.7882917900992,85.4114180390501));
#181612=CARTESIAN_POINT('Ctrl Pts',(-2.67675967323638,7.20585895817874,
85.6229746594321));
#181613=CARTESIAN_POINT('Ctrl Pts',(-5.78993610871133,5.0758427622442,85.7816421247185));
#181614=CARTESIAN_POINT('Ctrl Pts',(-7.51680423226243,1.67617198999052,
85.9403095900049));
#181615=CARTESIAN_POINT('Ctrl Pts',(-7.39809122969079,-2.11499585179245,
86.0989770552914));
#181616=CARTESIAN_POINT('Ctrl Pts',(-5.49497454123724,-5.39603124503018,
86.2576445205777));
#181617=CARTESIAN_POINT('Ctrl Pts',(-2.23209396432371,-7.36921274115597,
86.4163119858643));
#181618=CARTESIAN_POINT('Ctrl Pts',(1.53651183639463,-7.53183756131588,
86.5749794511506));
#181619=CARTESIAN_POINT('Ctrl Pts',(6.14593418003887,-5.34785626919466,
86.7865360715324));
#181620=CARTESIAN_POINT('Ctrl Pts',(8.13651942694822,-0.199030386124499,
86.9980926919146));
#181621=CARTESIAN_POINT('Ctrl Pts',(6.22559236563579,4.50250353175033,87.2096493122962));
#181622=CARTESIAN_POINT('Ctrl Pts',(2.35893799977536,7.78960672902815,87.4212059326784));
#181623=CARTESIAN_POINT('Ctrl Pts',(-3.15427289676359,7.5115002572107,87.63276255306));
#181624=CARTESIAN_POINT('Ctrl Pts',(-6.67185181037829,3.8178317267503,87.8443191734422));
#181625=CARTESIAN_POINT('Ctrl Pts',(-7.697548510231,0.187847870966458,88.0029866387283));
#181626=CARTESIAN_POINT('Ctrl Pts',(-6.84538509645438,-3.52882434918875,
88.161654104015));
#181627=CARTESIAN_POINT('Ctrl Pts',(-4.32533719029197,-6.36367971272943,
88.3203215693013));
#181628=CARTESIAN_POINT('Ctrl Pts',(-0.762027260803349,-7.66362922250155,
88.4789890345877));
#181629=CARTESIAN_POINT('Ctrl Pts',(3.00742183576063,-7.08822642074706,
88.6376564998743));
#181630=CARTESIAN_POINT('Ctrl Pts',(6.00519926153617,-4.79864850793173,
88.7963239651606));
#181631=CARTESIAN_POINT('Ctrl Pts',(8.14516047232624,-0.168625328428629,
89.0078805855426));
#181632=CARTESIAN_POINT('Ctrl Pts',(6.37484650903789,5.06002899852491,89.2194372059244));
#181633=CARTESIAN_POINT('Ctrl Pts',(1.89546479045971,7.4456532006678,89.4309938263063));
#181634=CARTESIAN_POINT('Ctrl Pts',(-3.1793642410478,7.49227632315112,89.6425504466883));
#181635=CARTESIAN_POINT('Ctrl Pts',(-7.23430921602959,3.74657761006007,
89.8541070670701));
#181636=CARTESIAN_POINT('Ctrl Pts',(-7.56872214193795,-1.34309002362748,
90.0656636874521));
#181637=CARTESIAN_POINT('Ctrl Pts',(-6.03063418038231,-4.78737832977405,
90.2243311527385));
#181638=CARTESIAN_POINT('Ctrl Pts',(-2.99516013938188,-7.09513313093194,
90.3829986180249));
#181639=CARTESIAN_POINT('Ctrl Pts',(0.755982743603434,-7.65724829082198,
90.5416660833114));
#181640=CARTESIAN_POINT('Ctrl Pts',(4.32478421550443,-6.37245163932341,
90.7003335485977));
#181641=CARTESIAN_POINT('Ctrl Pts',(6.85037485613197,-3.51566554445393,
90.8590010138843));
#181642=CARTESIAN_POINT('Ctrl Pts',(7.68523972212387,0.162899008310248,
91.0176684791705));
#181643=CARTESIAN_POINT('Ctrl Pts',(6.36200152846888,5.08891050944583,91.2292250995527));
#181644=CARTESIAN_POINT('Ctrl Pts',(1.65287275967981,7.9693521141867,91.4407817199344));
#181645=CARTESIAN_POINT('Ctrl Pts',(-3.31486374127232,6.9312492909561,91.6523383403164));
#181646=CARTESIAN_POINT('Ctrl Pts',(-7.24125844712909,3.71574186153288,
91.8638949606982));
#181647=CARTESIAN_POINT('Ctrl Pts',(-7.95493420564528,-1.75815113252337,
92.0754515810801));
#181648=CARTESIAN_POINT('Ctrl Pts',(-4.95088911273936,-5.88031824543361,
92.2870082014621));
#181649=CARTESIAN_POINT('Ctrl Pts',(-1.56326161937788,-7.53947962379497,
92.4456756667484));
#181650=CARTESIAN_POINT('Ctrl Pts',(2.24593360768367,-7.36666007351953,
92.604343132035));
#181651=CARTESIAN_POINT('Ctrl Pts',(5.48624538689425,-5.39500443448174,
92.7630105973214));
#181652=CARTESIAN_POINT('Ctrl Pts',(7.40328658309064,-2.122085336118,92.9216780626076));
#181653=CARTESIAN_POINT('Ctrl Pts',(7.5122049506152,1.68947230894764,93.0803455278944));
#181654=CARTESIAN_POINT('Ctrl Pts',(5.79646930811482,5.0488007682166,93.2390129931805));
#181655=CARTESIAN_POINT('Ctrl Pts',(1.62450660586534,7.98329831625276,93.4505696135627));
#181656=CARTESIAN_POINT('Ctrl Pts',(-3.83664898069644,7.17793047853722,
93.6621262339443));
#181657=CARTESIAN_POINT('Ctrl Pts',(-6.98586204654806,3.19816663680324,
93.8736828543265));
#181658=CARTESIAN_POINT('Ctrl Pts',(-7.94051430657702,-1.78627946591266,
94.0852394747081));
#181659=CARTESIAN_POINT('Ctrl Pts',(-4.98150970512187,-6.44644348648762,
94.2967960950903));
#181660=CARTESIAN_POINT('Ctrl Pts',(-0.0340013617126023,-7.68689083973357,
94.5083527154719));
#181661=CARTESIAN_POINT('Ctrl Pts',(3.63004607814272,-6.79045680214596,
94.6670201807586));
#181662=CARTESIAN_POINT('Ctrl Pts',(6.44407833726602,-4.21731596128019,
94.8256876460449));
#181663=CARTESIAN_POINT('Ctrl Pts',(7.66884899579075,-0.627470455383009,
94.9843551113314));
#181664=CARTESIAN_POINT('Ctrl Pts',(7.04390880922885,3.11371703253214,95.1430225766178));
#181665=CARTESIAN_POINT('Ctrl Pts',(4.68557750794345,6.11006851004831,95.3016900419042));
#181666=CARTESIAN_POINT('Ctrl Pts',(1.21597883488297,7.59017650355904,95.4603575071907));
#181667=CARTESIAN_POINT('Ctrl Pts',(-3.86736055146191,7.17047381967795,
95.6719141275726));
#181668=CARTESIAN_POINT('Ctrl Pts',(-7.54454431331429,3.05326164501626,
95.8834707479544));
#181669=CARTESIAN_POINT('Ctrl Pts',(-7.41281351694419,-2.02003584276841,
96.0950273683364));
#181670=CARTESIAN_POINT('Ctrl Pts',(-4.95243528627397,-6.45885070399418,
96.3065839887182));
#181671=CARTESIAN_POINT('Ctrl Pts',(0.305225731983484,-8.14109071138399,
96.5181406091002));
#181672=CARTESIAN_POINT('Ctrl Pts',(4.8986302043341,-5.92400513744318,96.729697229482));
#181673=CARTESIAN_POINT('Ctrl Pts',(7.13775755591544,-2.8878837263204,96.8883646947684));
#181674=CARTESIAN_POINT('Ctrl Pts',(7.64958627659066,0.889942290580429,
97.047032160055));
#181675=CARTESIAN_POINT('Ctrl Pts',(6.29060828708289,4.43237517084745,97.2056996253414));
#181676=CARTESIAN_POINT('Ctrl Pts',(3.41286611377566,6.90183796626506,97.3643670906277));
#181677=CARTESIAN_POINT('Ctrl Pts',(-0.315651225729196,7.69659528197362,
97.5230345559143));
#181678=CARTESIAN_POINT('Ctrl Pts',(-3.93140711959932,6.60107452679552,
97.6817020212007));
#181679=CARTESIAN_POINT('Ctrl Pts',(-7.55836006441197,3.04053020989608,
97.8932586415825));
#181680=CARTESIAN_POINT('Ctrl Pts',(-7.80768231748721,-3.89690115260277,
98.1577044170599));
#181681=CARTESIAN_POINT('Ctrl Pts',(-2.11328258743627,-7.86831172410565,
98.4221501925374));
#181682=CARTESIAN_POINT('Ctrl Pts',(2.9118447354237,-7.10958063882229,98.6337068129191));
#181683=CARTESIAN_POINT('Ctrl Pts',(5.96180663630364,-4.87920683779491,
98.7923742782056));
#181684=CARTESIAN_POINT('Ctrl Pts',(7.56588082541761,-1.42044622492244,
98.9510417434921));
#181685=CARTESIAN_POINT('Ctrl Pts',(7.32611861958554,2.3612726491774,99.1097092087785));
#181686=CARTESIAN_POINT('Ctrl Pts',(5.30450950461827,5.58155414095716,99.268382491107));
#181687=CARTESIAN_POINT('Ctrl Pts',(3.0958658922055,6.81680238395213,99.3741666183402));
#181688=CARTESIAN_POINT('Ctrl Pts',(1.91033529005388,7.1342502773344,99.4270615904777));
#181689=CARTESIAN_POINT('Ctrl Pts',(-5.88260427712044,5.07275281512923,
-0.436808985868258));
#181690=CARTESIAN_POINT('Ctrl Pts',(-6.72572424933426,4.0950357906363,-0.383904265042635));
#181691=CARTESIAN_POINT('Ctrl Pts',(-7.91518952170536,1.71376454911315,
-0.278110389121537));
#181692=CARTESIAN_POINT('Ctrl Pts',(-7.76703063229785,-2.28272930962537,
-0.119427358104962));
#181693=CARTESIAN_POINT('Ctrl Pts',(-5.73741125046268,-5.71258830081366,
0.0392401071814675));
#181694=CARTESIAN_POINT('Ctrl Pts',(-2.295824829586,-7.77044585965269,0.197907572467895));
#181695=CARTESIAN_POINT('Ctrl Pts',(1.67589148835794,-7.90460135847237,
0.356575037754326));
#181696=CARTESIAN_POINT('Ctrl Pts',(6.49394857069463,-5.59032484528709,
0.568131658136229));
#181697=CARTESIAN_POINT('Ctrl Pts',(9.09452740305039,1.23259449184249,0.832577433613612));
#181698=CARTESIAN_POINT('Ctrl Pts',(4.77208267061024,7.11669743931879,1.09702320909099));
#181699=CARTESIAN_POINT('Ctrl Pts',(-0.488505341624206,8.0658797764415,
1.30857982947289));
#181700=CARTESIAN_POINT('Ctrl Pts',(-4.28052068697957,6.87850740867851,
1.46724729475932));
#181701=CARTESIAN_POINT('Ctrl Pts',(-7.05188031313337,3.98092452512984,
1.62591476004575));
#181702=CARTESIAN_POINT('Ctrl Pts',(-8.09242944805938,0.130793062761592,
1.78458222533218));
#181703=CARTESIAN_POINT('Ctrl Pts',(-7.17751004572653,-3.75339048631073,
1.94324969061861));
#181704=CARTESIAN_POINT('Ctrl Pts',(-4.49673398246179,-6.73506221619666,
2.10191715590504));
#181705=CARTESIAN_POINT('Ctrl Pts',(-0.753133361682607,-8.04962796580004,
2.26058462119146));
#181706=CARTESIAN_POINT('Ctrl Pts',(4.55264398574624,-7.25879796607905,
2.47214124157337));
#181707=CARTESIAN_POINT('Ctrl Pts',(8.12827139953132,-2.68463536639679,
2.68369786195528));
#181708=CARTESIAN_POINT('Ctrl Pts',(7.64045732588155,2.63072034789073,2.89525448233718));
#181709=CARTESIAN_POINT('Ctrl Pts',(4.75253610096309,7.11959024619432,3.1068111027191));
#181710=CARTESIAN_POINT('Ctrl Pts',(-0.881168716787595,8.52303255506265,
3.31836772310098));
#181711=CARTESIAN_POINT('Ctrl Pts',(-5.54919544617434,5.87954163535837,
3.52992434348291));
#181712=CARTESIAN_POINT('Ctrl Pts',(-7.68984104450024,2.53932181611785,
3.68859180876932));
#181713=CARTESIAN_POINT('Ctrl Pts',(-7.96697490008165,-1.46151079519648,
3.84725927405576));
#181714=CARTESIAN_POINT('Ctrl Pts',(-6.29623036293426,-5.08408437053503,
4.00592673934218));
#181715=CARTESIAN_POINT('Ctrl Pts',(-3.10684626370346,-7.48038937187224,
4.16459420462861));
#181716=CARTESIAN_POINT('Ctrl Pts',(0.862598852087911,-8.05218568712171,
4.32326166991504));
#181717=CARTESIAN_POINT('Ctrl Pts',(4.5787781514147,-6.6631404204,4.48192913520147));
#181718=CARTESIAN_POINT('Ctrl Pts',(8.14620698293027,-2.6566414067469,4.69348575558337));
#181719=CARTESIAN_POINT('Ctrl Pts',(7.96091912215295,3.14625781998219,4.90504237596528));
#181720=CARTESIAN_POINT('Ctrl Pts',(4.18104045973186,6.91493946455292,5.11659899634718));
#181721=CARTESIAN_POINT('Ctrl Pts',(-0.912283436664409,8.51134008235826,
5.32815561672909));
#181722=CARTESIAN_POINT('Ctrl Pts',(-6.13703969858474,5.97956326040377,
5.539712237111));
#181723=CARTESIAN_POINT('Ctrl Pts',(-8.02761683896492,0.959174718031465,
5.7512688574929));
#181724=CARTESIAN_POINT('Ctrl Pts',(-7.53123945186008,-2.97694565283782,
5.90993632277932));
#181725=CARTESIAN_POINT('Ctrl Pts',(-5.18080544935911,-6.22639321824364,
6.06860378806576));
#181726=CARTESIAN_POINT('Ctrl Pts',(-1.57709787861097,-7.93745487260388,
6.22727125335218));
#181727=CARTESIAN_POINT('Ctrl Pts',(2.40700230849641,-7.73401949204719,
6.38593871863862));
#181728=CARTESIAN_POINT('Ctrl Pts',(5.82113258443977,-5.6299368131026,6.54460618392504));
#181729=CARTESIAN_POINT('Ctrl Pts',(7.78454300128656,-2.18255321932097,
6.70327364921147));
#181730=CARTESIAN_POINT('Ctrl Pts',(7.95680954239199,3.17924752811758,6.91483026959338));
#181731=CARTESIAN_POINT('Ctrl Pts',(4.09678269192862,7.51608560212756,7.12638688997527));
#181732=CARTESIAN_POINT('Ctrl Pts',(-1.21995294319321,7.98806621941246,
7.33794351035719));
#181733=CARTESIAN_POINT('Ctrl Pts',(-6.15344869664912,5.95065041327512,
7.54950013073908));
#181734=CARTESIAN_POINT('Ctrl Pts',(-8.54304869417939,0.659357223605445,
7.76105675112099));
#181735=CARTESIAN_POINT('Ctrl Pts',(-6.77823344102648,-4.40660864067956,
7.9726133715029));
#181736=CARTESIAN_POINT('Ctrl Pts',(-3.87534239299458,-7.11080125050227,
8.13128083678932));
#181737=CARTESIAN_POINT('Ctrl Pts',(0.0111865443866004,-8.0999131152557,
8.28994830207576));
#181738=CARTESIAN_POINT('Ctrl Pts',(3.87439429040926,-7.10489243118364,
8.44861576736218));
#181739=CARTESIAN_POINT('Ctrl Pts',(6.80310647024964,-4.39618698054479,
8.60728323264862));
#181740=CARTESIAN_POINT('Ctrl Pts',(8.07649462909002,-0.593302278241658,
8.76595069793504));
#181741=CARTESIAN_POINT('Ctrl Pts',(7.37538337761979,3.31155074342861,8.92461816322147));
#181742=CARTESIAN_POINT('Ctrl Pts',(4.07249172344147,7.53878266710748,9.13617478360338));
#181743=CARTESIAN_POINT('Ctrl Pts',(-1.66978527237763,8.3956529434934,9.34773140398528));
#181744=CARTESIAN_POINT('Ctrl Pts',(-6.0544342533289,5.35175793373891,9.55928802436719));
#181745=CARTESIAN_POINT('Ctrl Pts',(-8.53712408125462,0.626644735636713,
9.77084464474909));
#181746=CARTESIAN_POINT('Ctrl Pts',(-6.98190427152286,-4.96703590511184,
9.98240126513099));
#181747=CARTESIAN_POINT('Ctrl Pts',(-2.3812275744557,-7.72608591279081,
10.1939578855129));
#181748=CARTESIAN_POINT('Ctrl Pts',(1.58015553212113,-7.94259917038461,
10.3526253507993));
#181749=CARTESIAN_POINT('Ctrl Pts',(5.19798381976746,-6.21205938662028,
10.5112928160857));
#181750=CARTESIAN_POINT('Ctrl Pts',(7.52672586390396,-2.97301620343546,
10.6699602813721));
#181751=CARTESIAN_POINT('Ctrl Pts',(8.04003782517391,0.983112090879871,
10.8286277466587));
#181752=CARTESIAN_POINT('Ctrl Pts',(6.5813579390032,4.7188452788587,10.987295211945));
#181753=CARTESIAN_POINT('Ctrl Pts',(3.54130152033665,7.26786294829738,11.1459626772314));
#181754=CARTESIAN_POINT('Ctrl Pts',(-1.70297761078211,8.3975175020094,11.3575192976133));
#181755=CARTESIAN_POINT('Ctrl Pts',(-6.66095155081305,5.37651333497463,
11.5690759179952));
#181756=CARTESIAN_POINT('Ctrl Pts',(-8.07740524261201,0.230242602147388,
11.7806325383771));
#181757=CARTESIAN_POINT('Ctrl Pts',(-6.95639726729727,-4.9883572709839,
11.9921891587591));
#181758=CARTESIAN_POINT('Ctrl Pts',(-2.17855833221247,-8.28687616249494,
12.2037457791409));
#181759=CARTESIAN_POINT('Ctrl Pts',(3.12155393056176,-7.45778448010983,
12.4153023995229));
#181760=CARTESIAN_POINT('Ctrl Pts',(6.30187332167991,-5.08607567035594,
12.5739698648093));
#181761=CARTESIAN_POINT('Ctrl Pts',(7.97098245675322,-1.43949862368597,
12.7326373300957));
#181762=CARTESIAN_POINT('Ctrl Pts',(7.68385597625173,2.53944578844899,12.8913047953821));
#181763=CARTESIAN_POINT('Ctrl Pts',(5.5433999678875,5.90588134062023,13.0499722606686));
#181764=CARTESIAN_POINT('Ctrl Pts',(2.03002227200793,7.83969276580654,13.208639725955));
#181765=CARTESIAN_POINT('Ctrl Pts',(-1.93726194449388,7.84918240656874,
13.3673071912414));
#181766=CARTESIAN_POINT('Ctrl Pts',(-6.68763166341679,5.3566795380949,13.5788638116233));
#181767=CARTESIAN_POINT('Ctrl Pts',(-8.55895780004107,-0.139329037012525,
13.7904204320052));
#181768=CARTESIAN_POINT('Ctrl Pts',(-6.34945463374779,-4.99819096906056,
14.0019770523871));
#181769=CARTESIAN_POINT('Ctrl Pts',(-2.14531367768294,-8.2869053589253,
14.2135336727691));
#181770=CARTESIAN_POINT('Ctrl Pts',(3.63644930484346,-7.75852237173309,
14.425090293151));
#181771=CARTESIAN_POINT('Ctrl Pts',(7.17477289584716,-3.7262960411365,14.6366469135329));
#181772=CARTESIAN_POINT('Ctrl Pts',(8.0971769917171,0.132279446230392,14.7953143788193));
#181773=CARTESIAN_POINT('Ctrl Pts',(7.04247926766235,4.00152513149765,14.9539818441057));
#181774=CARTESIAN_POINT('Ctrl Pts',(4.27281778792673,6.87266001832097,15.1126493093922));
#181775=CARTESIAN_POINT('Ctrl Pts',(0.4725618517077,8.08612409685704,15.2713167746785));
#181776=CARTESIAN_POINT('Ctrl Pts',(-3.46399909120887,7.32000569557098,
15.429984239965));
#181777=CARTESIAN_POINT('Ctrl Pts',(-6.51621502076343,4.78556058329111,
15.5886517052514));
#181778=CARTESIAN_POINT('Ctrl Pts',(-8.56673618704802,-0.171650927470619,
15.8002083256334));
#181779=CARTESIAN_POINT('Ctrl Pts',(-6.48242288096887,-5.59047089212797,
16.0117649460152));
#181780=CARTESIAN_POINT('Ctrl Pts',(-1.67299447177369,-7.90560412660755,
16.2233215663972));
#181781=CARTESIAN_POINT('Ctrl Pts',(3.66199371979118,-7.73724584071417,
16.4348781867791));
#181782=CARTESIAN_POINT('Ctrl Pts',(7.76279135828505,-3.62732728977057,
16.646434807161));
#181783=CARTESIAN_POINT('Ctrl Pts',(7.89622753725514,1.73558029865116,16.8579914275429));
#181784=CARTESIAN_POINT('Ctrl Pts',(6.1323776150447,5.28920767918846,17.0166588928293));
#181785=CARTESIAN_POINT('Ctrl Pts',(2.84364522402627,7.58435227645275,17.1753263581157));
#181786=CARTESIAN_POINT('Ctrl Pts',(-1.12239774996747,8.0144027143087,17.3339938234021));
#181787=CARTESIAN_POINT('Ctrl Pts',(-4.81772080176973,6.511396462331,17.4926612886886));
#181788=CARTESIAN_POINT('Ctrl Pts',(-7.34943593787407,3.40111224192512,
17.651328753975));
#181789=CARTESIAN_POINT('Ctrl Pts',(-8.06921967356995,-0.500342035855678,
17.8099962192614));
#181790=CARTESIAN_POINT('Ctrl Pts',(-6.46768747650548,-5.6202714921642,
18.0215528396434));
#181791=CARTESIAN_POINT('Ctrl Pts',(-1.39563166519913,-8.44555406462666,
18.2331094600252));
#181792=CARTESIAN_POINT('Ctrl Pts',(3.78035763870035,-7.14187533024342,
18.4446660804073));
#181793=CARTESIAN_POINT('Ctrl Pts',(7.76877342015511,-3.59462525859519,
18.6562227007891));
#181794=CARTESIAN_POINT('Ctrl Pts',(8.28430972229547,2.18829736655231,18.867779321171));
#181795=CARTESIAN_POINT('Ctrl Pts',(4.95089445119752,6.39150157836752,19.0793359415529));
#181796=CARTESIAN_POINT('Ctrl Pts',(1.31987319530725,7.98997545899841,19.2380034068393));
#181797=CARTESIAN_POINT('Ctrl Pts',(-2.67569831094984,7.64521786231378,
19.3966708721258));
#181798=CARTESIAN_POINT('Ctrl Pts',(-5.99640309280362,5.43448042823468,
19.5553383374121));
#181799=CARTESIAN_POINT('Ctrl Pts',(-7.87078835133371,1.91295800841818,
19.7140058026986));
#181800=CARTESIAN_POINT('Ctrl Pts',(-7.82199981784164,-2.09716283029542,
19.872673267985));
#181801=CARTESIAN_POINT('Ctrl Pts',(-5.8751038780775,-5.55389977538047,
20.0313407332714));
#181802=CARTESIAN_POINT('Ctrl Pts',(-1.3652251799131,-8.4589948071571,20.2428973536535));
#181803=CARTESIAN_POINT('Ctrl Pts',(4.33925195138733,-7.3787575990691,20.4544539740352));
#181804=CARTESIAN_POINT('Ctrl Pts',(7.47821715101717,-3.06165892147577,
20.6660105944172));
#181805=CARTESIAN_POINT('Ctrl Pts',(8.26795152848235,2.21723898714254,20.877567214799));
#181806=CARTESIAN_POINT('Ctrl Pts',(4.95882582137418,6.98773778934587,21.089123835181));
#181807=CARTESIAN_POINT('Ctrl Pts',(-0.293495865414464,8.0793878771945,
21.3006804555629));
#181808=CARTESIAN_POINT('Ctrl Pts',(-4.10554350583665,6.98042159248063,
21.4593479208493));
#181809=CARTESIAN_POINT('Ctrl Pts',(-6.95252221453218,4.15585760943489,
21.6180153861357));
#181810=CARTESIAN_POINT('Ctrl Pts',(-8.08584616639284,0.330937078129198,
21.7766828514222));
#181811=CARTESIAN_POINT('Ctrl Pts',(-7.26888142150446,-3.57380476433294,
21.9353503167086));
#181812=CARTESIAN_POINT('Ctrl Pts',(-4.66224525194671,-6.62157400455422,
22.094017781995));
#181813=CARTESIAN_POINT('Ctrl Pts',(-0.952753783854475,-8.02838143840485,
22.2526852472814));
#181814=CARTESIAN_POINT('Ctrl Pts',(4.37120959420905,-7.36959697832074,
22.4642418676634));
#181815=CARTESIAN_POINT('Ctrl Pts',(8.05910804671024,-2.88547200556326,
22.6757984880452));
#181816=CARTESIAN_POINT('Ctrl Pts',(7.70340129483707,2.44030645614891,22.8873551084271));
#181817=CARTESIAN_POINT('Ctrl Pts',(4.92772366061626,6.99947931835228,23.0989117288091));
#181818=CARTESIAN_POINT('Ctrl Pts',(-0.669398417089992,8.54226777258687,
23.3104683491909));
#181819=CARTESIAN_POINT('Ctrl Pts',(-5.40159489200389,6.01543189769863,
23.5220249695729));
#181820=CARTESIAN_POINT('Ctrl Pts',(-7.62446036629699,2.7293547240793,23.6806924348593));
#181821=CARTESIAN_POINT('Ctrl Pts',(-8.00078880883006,-1.26336694984519,
23.8393599001457));
#181822=CARTESIAN_POINT('Ctrl Pts',(-6.42044791237127,-4.92628421640267,
23.9980273654321));
#181823=CARTESIAN_POINT('Ctrl Pts',(-3.29150879454047,-7.40099233001387,
24.1566948307186));
#181824=CARTESIAN_POINT('Ctrl Pts',(0.662525911002324,-8.07111098327473,
24.315362296005));
#181825=CARTESIAN_POINT('Ctrl Pts',(4.41202858140564,-6.77470678996754,
24.4740297612914));
#181826=CARTESIAN_POINT('Ctrl Pts',(8.07777660950554,-2.85796395818857,
24.6855863816734));
#181827=CARTESIAN_POINT('Ctrl Pts',(8.03653925108718,2.9477462694699,24.8971430020552));
#181828=CARTESIAN_POINT('Ctrl Pts',(4.35134083743695,6.80906161124081,25.1086996224372));
#181829=CARTESIAN_POINT('Ctrl Pts',(-0.700801569229135,8.53135677158124,
25.320256242819));
#181830=CARTESIAN_POINT('Ctrl Pts',(-5.98677270993274,6.13000697054935,
25.531812863201));
#181831=CARTESIAN_POINT('Ctrl Pts',(-8.00134397993067,1.15807720295321,
25.7433694835829));
#181832=CARTESIAN_POINT('Ctrl Pts',(-7.60279058993861,-2.78914831671395,
25.9020369488693));
#181833=CARTESIAN_POINT('Ctrl Pts',(-5.33371233888031,-6.09591915132881,
26.0607044141557));
#181834=CARTESIAN_POINT('Ctrl Pts',(-1.77357280768402,-7.89587658668085,
26.2193718794422));
#181835=CARTESIAN_POINT('Ctrl Pts',(2.21434866846989,-7.79136557914638,
26.3780393447286));
#181836=CARTESIAN_POINT('Ctrl Pts',(5.67963852838276,-5.77264924224552,
26.536706810015));
#181837=CARTESIAN_POINT('Ctrl Pts',(7.72798798922236,-2.37504735355052,
26.6953742753014));
#181838=CARTESIAN_POINT('Ctrl Pts',(8.03324957423221,2.98082777387049,26.9069308956833));
#181839=CARTESIAN_POINT('Ctrl Pts',(4.28202588343303,7.41211343255407,27.1184875160653));
#181840=CARTESIAN_POINT('Ctrl Pts',(-1.02136088257305,8.0158785580103,27.3300441364471));
#181841=CARTESIAN_POINT('Ctrl Pts',(-6.00389410589115,6.10151020393185,
27.5416007568292));
#181842=CARTESIAN_POINT('Ctrl Pts',(-8.5240568146021,0.871141986598558,
27.7531573772109));
#181843=CARTESIAN_POINT('Ctrl Pts',(-6.88549219764244,-4.23705622919709,
27.9647139975929));
#181844=CARTESIAN_POINT('Ctrl Pts',(-4.05059701621648,-7.01244870921033,
28.1233814628793));
#181845=CARTESIAN_POINT('Ctrl Pts',(-0.189808693704911,-8.09769660293935,
28.2820489281657));
#181846=CARTESIAN_POINT('Ctrl Pts',(3.69690001810475,-7.19884420114699,
28.4407163934522));
#181847=CARTESIAN_POINT('Ctrl Pts',(6.69192440029062,-4.56364606803117,
28.5993838587386));
#181848=CARTESIAN_POINT('Ctrl Pts',(8.05928550105423,-0.793530276413581,
28.758051324025));
#181849=CARTESIAN_POINT('Ctrl Pts',(7.45528542102758,3.12751779917977,28.9167187893114));
#181850=CARTESIAN_POINT('Ctrl Pts',(4.25830560106211,7.43540626646198,29.1282754096933));
#181851=CARTESIAN_POINT('Ctrl Pts',(-1.4609408163955,8.43450194939975,29.3398320300753));
#181852=CARTESIAN_POINT('Ctrl Pts',(-5.91977110935251,5.50034518208584,
29.5513886504571));
#181853=CARTESIAN_POINT('Ctrl Pts',(-8.5189457558619,0.838292557596449,
29.7629452708391));
#181854=CARTESIAN_POINT('Ctrl Pts',(-7.10300679471207,-4.79225702708581,
29.9745018912209));
#181855=CARTESIAN_POINT('Ctrl Pts',(-2.57220997546955,-7.66461898174121,
30.1860585116029));
#181856=CARTESIAN_POINT('Ctrl Pts',(1.38258078166772,-7.9793636005167,30.3447259768893));
#181857=CARTESIAN_POINT('Ctrl Pts',(5.04223681229703,-6.33912971488816,
30.5033934421758));
#181858=CARTESIAN_POINT('Ctrl Pts',(7.45063563589183,-3.15886944925386,
30.6620609074621));
#181859=CARTESIAN_POINT('Ctrl Pts',(8.0619571758907,0.783303330495699,30.8207283727486));
#181860=CARTESIAN_POINT('Ctrl Pts',(6.6964251779342,4.5540820066635,30.979395838035));
#181861=CARTESIAN_POINT('Ctrl Pts',(3.72055633984306,7.17775095801089,31.1380633033215));
#181862=CARTESIAN_POINT('Ctrl Pts',(-1.49407666705354,8.4371895707247,31.3496199237034));
#181863=CARTESIAN_POINT('Ctrl Pts',(-6.5254873680156,5.540143122096,31.5611765440852));
#181864=CARTESIAN_POINT('Ctrl Pts',(-8.06920482161725,0.430604988368971,
31.7727331644672));
#181865=CARTESIAN_POINT('Ctrl Pts',(-7.07803671433036,-4.81420476029328,
31.984289784849));
#181866=CARTESIAN_POINT('Ctrl Pts',(-2.38351862570955,-8.23026560326427,
32.195846405231));
#181867=CARTESIAN_POINT('Ctrl Pts',(2.93553478289759,-7.53294655706325,
32.4074030256128));
#181868=CARTESIAN_POINT('Ctrl Pts',(6.17372664486792,-5.24088469645491,
32.5660704908993));
#181869=CARTESIAN_POINT('Ctrl Pts',(7.93280824411931,-1.63684787793316,
32.7247379561857));
#181870=CARTESIAN_POINT('Ctrl Pts',(7.74450397115589,2.3479961279784,32.8834054214723));
#181871=CARTESIAN_POINT('Ctrl Pts',(5.68824200445711,5.76650852008312,33.0420728867586));
#181872=CARTESIAN_POINT('Ctrl Pts',(2.223931863048,7.7869056855472,33.2007403520451));
#181873=CARTESIAN_POINT('Ctrl Pts',(-1.74189528503904,7.89483686399733,
33.3594078173314));
#181874=CARTESIAN_POINT('Ctrl Pts',(-6.55265142255683,5.52097747449158,
33.5709644377134));
#181875=CARTESIAN_POINT('Ctrl Pts',(-8.5597796768496,0.0730964242035642,
33.7825210580952));
#181876=CARTESIAN_POINT('Ctrl Pts',(-6.47152498241538,-4.83909614609933,
33.9940776784773));
#181877=CARTESIAN_POINT('Ctrl Pts',(-2.35028493223617,-8.23111972581751,
34.2056342988591));
#181878=CARTESIAN_POINT('Ctrl Pts',(3.4428090820096,-7.84636849531113,34.4171909192411));
#181879=CARTESIAN_POINT('Ctrl Pts',(7.08009910292349,-3.90318395492124,
34.6287475396229));
#181880=CARTESIAN_POINT('Ctrl Pts',(8.09796612938011,-0.0686851839944798,
34.7874150049093));
#181881=CARTESIAN_POINT('Ctrl Pts',(7.1396048889772,3.82554043799754,34.9460824701958));
#181882=CARTESIAN_POINT('Ctrl Pts',(4.44204076926994,6.76451782320029,35.1047499354821));
#181883=CARTESIAN_POINT('Ctrl Pts',(0.673065974102065,8.07190806488574,
35.2634174007686));
#181884=CARTESIAN_POINT('Ctrl Pts',(-3.28129335117483,7.40370765431913,
35.422084866055));
#181885=CARTESIAN_POINT('Ctrl Pts',(-6.39545934638827,4.94578083237291,
35.5807523313416));
#181886=CARTESIAN_POINT('Ctrl Pts',(-8.56835770634636,0.0409774996080618,
35.7923089517233));
#181887=CARTESIAN_POINT('Ctrl Pts',(-6.61914916072759,-5.42789421336466,
36.0038655721053));
#181888=CARTESIAN_POINT('Ctrl Pts',(-1.86864952650306,-7.8616560632172,
36.2154221924872));
#181889=CARTESIAN_POINT('Ctrl Pts',(3.46887358869753,-7.82573237653036,
36.4269788128691));
#181890=CARTESIAN_POINT('Ctrl Pts',(7.67039232215131,-3.81883680767606,
36.6385354332509));
#181891=CARTESIAN_POINT('Ctrl Pts',(7.93686296667427,1.53910835921557,36.8500920536329));
#181892=CARTESIAN_POINT('Ctrl Pts',(6.26173611367256,5.13540981128245,37.0087595189193));
#181893=CARTESIAN_POINT('Ctrl Pts',(3.030968251,7.51145452458389,37.1674269842058));
#181894=CARTESIAN_POINT('Ctrl Pts',(-0.923182212626471,8.03978620229051,
37.3260944494921));
#181895=CARTESIAN_POINT('Ctrl Pts',(-4.65466311300933,6.62893874748074,
37.4847619147786));
#181896=CARTESIAN_POINT('Ctrl Pts',(-7.26277749619282,3.58243438570523,
37.643429380065));
#181897=CARTESIAN_POINT('Ctrl Pts',(-8.07915054981909,-0.299957807917071,
37.8020968453515));
#181898=CARTESIAN_POINT('Ctrl Pts',(-6.60515776764774,-5.45805128263392,
38.0136534657333));
#181899=CARTESIAN_POINT('Ctrl Pts',(-1.60477047887609,-8.40832224130156,
38.2252100861153));
#181900=CARTESIAN_POINT('Ctrl Pts',(3.60197462565547,-7.23348228071057,
38.4367667064971));
#181901=CARTESIAN_POINT('Ctrl Pts',(7.67718401246675,-3.78629328528101,
38.6483233268791));
#181902=CARTESIAN_POINT('Ctrl Pts',(8.33605940688698,1.98205613044405,38.859879947261));
#181903=CARTESIAN_POINT('Ctrl Pts',(5.10796914345129,6.26668169948992,39.0714365676429));
#181904=CARTESIAN_POINT('Ctrl Pts',(1.51773057783043,7.9547637916035,39.2301040329293));
#181905=CARTESIAN_POINT('Ctrl Pts',(-2.48516546487529,7.70925873386361,
39.3887714982157));
#181906=CARTESIAN_POINT('Ctrl Pts',(-5.85970513598202,5.58160221581555,
39.5474389635022));
#181907=CARTESIAN_POINT('Ctrl Pts',(-7.82089653681279,2.10767525343236,
39.7061064287886));
#181908=CARTESIAN_POINT('Ctrl Pts',(-7.87163043666332,-1.90242144533834,
39.864773894075));
#181909=CARTESIAN_POINT('Ctrl Pts',(-6.01110968313766,-5.40640441240397,
40.0234413593615));
#181910=CARTESIAN_POINT('Ctrl Pts',(-1.57470687574229,-8.42251335379584,
40.2349979797433));
#181911=CARTESIAN_POINT('Ctrl Pts',(4.15481883293474,-7.48416005099628,
40.4465546001254));
#181912=CARTESIAN_POINT('Ctrl Pts',(7.39994227321339,-3.24628117425619,
40.6581112205073));
#181913=CARTESIAN_POINT('Ctrl Pts',(8.32042440936654,2.01139475276605,40.8696678408892));
#181914=CARTESIAN_POINT('Ctrl Pts',(5.13069311721947,6.86253751001021,41.081224461271));
#181915=CARTESIAN_POINT('Ctrl Pts',(-0.0929230143071497,8.08418292758069,
41.292781081653));
#181916=CARTESIAN_POINT('Ctrl Pts',(-3.93106668673612,7.08014744136818,
41.4514485469393));
#181917=CARTESIAN_POINT('Ctrl Pts',(-6.84725768633784,4.32709831068912,
41.6101160122258));
#181918=CARTESIAN_POINT('Ctrl Pts',(-8.07514450673869,0.531477912525767,
41.7687834775121));
#181919=CARTESIAN_POINT('Ctrl Pts',(-7.35532384768093,-3.39233381453608,
41.9274509427987));
#181920=CARTESIAN_POINT('Ctrl Pts',(-4.82511785680412,-6.5038458434228,
42.086118408085));
#181921=CARTESIAN_POINT('Ctrl Pts',(-1.15167721705284,-8.00226767115608,
42.2447858733715));
#181922=CARTESIAN_POINT('Ctrl Pts',(4.18699394776991,-7.47579525008377,
42.4563424937533));
#181923=CARTESIAN_POINT('Ctrl Pts',(7.98502621710635,-3.08456277525204,
42.6678991141353));
#181924=CARTESIAN_POINT('Ctrl Pts',(7.76158322136841,2.24840232341148,42.8794557345171));
#181925=CARTESIAN_POINT('Ctrl Pts',(5.09989188825386,6.87504719480985,43.0910123548991));
#181926=CARTESIAN_POINT('Ctrl Pts',(-0.457223885958288,8.55624796593684,
43.302568975281));
#181927=CARTESIAN_POINT('Ctrl Pts',(-5.25066431761787,6.1476151899389,43.5141255956629));
#181928=CARTESIAN_POINT('Ctrl Pts',(-7.55438627582335,2.91770818744103,
43.6727930609493));
#181929=CARTESIAN_POINT('Ctrl Pts',(-8.02967450977103,-1.06444582138774,
43.8314605262359));
#181930=CARTESIAN_POINT('Ctrl Pts',(-6.5407120987235,-4.76544990412998,
43.9901279915221));
#181931=CARTESIAN_POINT('Ctrl Pts',(-3.47414401702616,-7.31703771791091,
44.1487954568087));
#181932=CARTESIAN_POINT('Ctrl Pts',(0.462044824466225,-8.08506572395892,
44.3074629220949));
#181933=CARTESIAN_POINT('Ctrl Pts',(4.24256199092539,-6.88210111412175,
44.4661303873815));
#181934=CARTESIAN_POINT('Ctrl Pts',(8.00437166488504,-3.05752646175317,
44.6776870077635));
#181935=CARTESIAN_POINT('Ctrl Pts',(8.10721015544517,2.74741941947125,44.8892436281453));
#181936=CARTESIAN_POINT('Ctrl Pts',(4.51896161031848,6.69899047623219,45.1008002485272));
#181937=CARTESIAN_POINT('Ctrl Pts',(-0.488888375429131,8.54611967991167,
45.3123568689091));
#181938=CARTESIAN_POINT('Ctrl Pts',(-5.83281835435429,6.27667539433993,
45.523913489291));
#181939=CARTESIAN_POINT('Ctrl Pts',(-7.97014427217491,1.35626678924387,
45.7354701096728));
#181940=CARTESIAN_POINT('Ctrl Pts',(-7.66965832474677,-2.59963393149468,
45.8941375749593));
#181941=CARTESIAN_POINT('Ctrl Pts',(-5.4833371940026,-5.96168984876232,
46.0528050402458));
#181942=CARTESIAN_POINT('Ctrl Pts',(-1.96895048651429,-7.84943798622479,
46.2114725055322));
#181943=CARTESIAN_POINT('Ctrl Pts',(2.02032187363893,-7.84390928812353,
46.3701399708186));
#181944=CARTESIAN_POINT('Ctrl Pts',(5.53466446957311,-5.91181452321533,
46.5288074361051));
#181945=CARTESIAN_POINT('Ctrl Pts',(7.66664218087319,-2.56606484425791,
46.6874749013914));
#181946=CARTESIAN_POINT('Ctrl Pts',(8.10481401624341,2.78054065146841,46.8990315217734));
#181947=CARTESIAN_POINT('Ctrl Pts',(4.46449514000472,7.30363726059554,47.1105881421552));
#181948=CARTESIAN_POINT('Ctrl Pts',(-0.821978661578898,8.03868309971759,
47.3221447625372));
#181949=CARTESIAN_POINT('Ctrl Pts',(-5.85104055953245,6.24878888601925,
47.533701382919));
#181950=CARTESIAN_POINT('Ctrl Pts',(-8.49901735273743,1.08203688693143,
47.745258003301));
#181951=CARTESIAN_POINT('Ctrl Pts',(-6.9894958003849,-4.06445832835817,
47.9568146236829));
#181952=CARTESIAN_POINT('Ctrl Pts',(-4.22128064297539,-6.91069714498755,
48.1154820889693));
#181953=CARTESIAN_POINT('Ctrl Pts',(-0.394720512146466,-8.08870629150604,
48.2741495542558));
#181954=CARTESIAN_POINT('Ctrl Pts',(3.52473691091294,-7.29174113183975,
48.4328170195422));
#181955=CARTESIAN_POINT('Ctrl Pts',(6.56281846735994,-4.72210073487363,
48.5914844848286));
#181956=CARTESIAN_POINT('Ctrl Pts',(8.55717721688639,0.236199208950159,
48.8030411052105));
#181957=CARTESIAN_POINT('Ctrl Pts',(5.9153156826332,7.02513251500696,49.0674868806879));
#181958=CARTESIAN_POINT('Ctrl Pts',(-2.71850420621116,8.77453486642056,
49.3848218112606));
#181959=CARTESIAN_POINT('Ctrl Pts',(-7.79248632499947,3.54136004741615,
49.6492675867384));
#181960=CARTESIAN_POINT('Ctrl Pts',(-7.88211848193875,-1.79548923383272,
49.8608242071199));
#181961=CARTESIAN_POINT('Ctrl Pts',(-6.08265409382359,-5.3557987538077,
50.0194916724066));
#181962=CARTESIAN_POINT('Ctrl Pts',(-2.78012128575648,-7.59101714791989,
50.1781591376928));
#181963=CARTESIAN_POINT('Ctrl Pts',(2.52766458240851,-8.17844913584806,
50.3897157580749));
#181964=CARTESIAN_POINT('Ctrl Pts',(8.35589799254476,-3.80775034988006,
50.6541615335521));
#181965=CARTESIAN_POINT('Ctrl Pts',(7.72417822065321,4.97771490393895,50.9714964641252));
#181966=CARTESIAN_POINT('Ctrl Pts',(1.30727621037075,8.45865693165901,51.2359422396023));
#181967=CARTESIAN_POINT('Ctrl Pts',(-3.8383109442619,7.10760758645932,51.4474988599843));
#181968=CARTESIAN_POINT('Ctrl Pts',(-7.80510652006937,3.52562858333696,
51.6590554803662));
#181969=CARTESIAN_POINT('Ctrl Pts',(-8.2620746709558,-2.26208194974895,
51.8706121007481));
#181970=CARTESIAN_POINT('Ctrl Pts',(-4.89489459159957,-6.43524337861689,
52.08216872113));
#181971=CARTESIAN_POINT('Ctrl Pts',(-1.24811346699438,-8.00144121968931,
52.2408361864165));
#181972=CARTESIAN_POINT('Ctrl Pts',(2.74330699596842,-7.62108382551198,
52.3995036517029));
#181973=CARTESIAN_POINT('Ctrl Pts',(6.04469976260079,-5.38091157393227,
52.5581711169893));
#181974=CARTESIAN_POINT('Ctrl Pts',(7.88741087937344,-1.84283217800734,
52.7168385822757));
#181975=CARTESIAN_POINT('Ctrl Pts',(7.80307288743708,2.16668750547222,52.8755060475622));
#181976=CARTESIAN_POINT('Ctrl Pts',(5.82542340009905,5.60596559873273,53.0341735128486));
#181977=CARTESIAN_POINT('Ctrl Pts',(1.28990952670701,8.4708083462645,53.2457301332307));
#181978=CARTESIAN_POINT('Ctrl Pts',(-4.40475490759329,7.33984953337933,
53.4572867536124));
#181979=CARTESIAN_POINT('Ctrl Pts',(-7.50516412453447,2.99498640274816,
53.6688433739943));
#181980=CARTESIAN_POINT('Ctrl Pts',(-8.24789523695355,-2.29073016552212,
53.8803999943762));
#181981=CARTESIAN_POINT('Ctrl Pts',(-4.89644173511686,-7.03159136007465,
54.0919566147581));
#181982=CARTESIAN_POINT('Ctrl Pts',(0.365384614725759,-8.07645597898883,
54.30351323514));
#181983=CARTESIAN_POINT('Ctrl Pts',(4.1675023402685,-6.94360863936363,54.4621807004266));
#181984=CARTESIAN_POINT('Ctrl Pts',(6.98923100089694,-4.09382029169499,
54.6208481657129));
#181985=CARTESIAN_POINT('Ctrl Pts',(8.08847119617018,-0.25896543083787,
54.7795156309993));
#181986=CARTESIAN_POINT('Ctrl Pts',(7.23678907745967,3.63835136269798,54.9381830962858));
#181987=CARTESIAN_POINT('Ctrl Pts',(4.60313313887934,6.66280261197641,55.0968505615722));
#181988=CARTESIAN_POINT('Ctrl Pts',(0.88126888889716,8.03654238010657,55.2555180268586));
#181989=CARTESIAN_POINT('Ctrl Pts',(-4.43662090061271,7.33040434155508,
55.4670746472405));
#181990=CARTESIAN_POINT('Ctrl Pts',(-8.08446765842773,2.81363714410309,
55.6786312676224));
#181991=CARTESIAN_POINT('Ctrl Pts',(-7.68137916670904,-2.50876486966342,
55.8901878880043));
#181992=CARTESIAN_POINT('Ctrl Pts',(-4.865237905432,-7.04305554036251,56.1017445083862));
#181993=CARTESIAN_POINT('Ctrl Pts',(0.745392301949692,-8.53597230889284,
56.3133011287681));
#181994=CARTESIAN_POINT('Ctrl Pts',(5.4549142553828,-5.96712315561334,56.5248577491501));
#181995=CARTESIAN_POINT('Ctrl Pts',(7.64844784646817,-2.66139411417292,
56.6835252144364));
#181996=CARTESIAN_POINT('Ctrl Pts',(7.9892288701152,1.33451851699505,56.8421926797231));
#181997=CARTESIAN_POINT('Ctrl Pts',(6.37635307462309,4.98322677036489,57.0008601450092));
#181998=CARTESIAN_POINT('Ctrl Pts',(3.22551463743937,7.42999144931627,57.1595276102958));
#181999=CARTESIAN_POINT('Ctrl Pts',(-0.734327090956097,8.06489533785327,
57.3181950755822));
#182000=CARTESIAN_POINT('Ctrl Pts',(-4.47214416361251,6.73517445008891,
57.4768625408686));
#182001=CARTESIAN_POINT('Ctrl Pts',(-8.10289067319347,2.78596404814002,
57.6884191612504));
#182002=CARTESIAN_POINT('Ctrl Pts',(-8.00998806280779,-3.01914929030919,
57.8999757816326));
#182003=CARTESIAN_POINT('Ctrl Pts',(-4.29057249337804,-6.84751595750426,
58.1115324020142));
#182004=CARTESIAN_POINT('Ctrl Pts',(0.776697108980894,-8.52478227313381,
58.3230890223963));
#182005=CARTESIAN_POINT('Ctrl Pts',(6.04108854134644,-6.07648600549702,
58.5346456427781));
#182006=CARTESIAN_POINT('Ctrl Pts',(8.01133323067813,-1.08682480658109,
58.74620226316));
#182007=CARTESIAN_POINT('Ctrl Pts',(7.57766799225029,2.85669754897422,58.9048697284464));
#182008=CARTESIAN_POINT('Ctrl Pts',(5.27925157756536,6.14314417820664,59.0635371937329));
#182009=CARTESIAN_POINT('Ctrl Pts',(1.70323462613665,7.91134750750969,59.2222046590193));
#182010=CARTESIAN_POINT('Ctrl Pts',(-2.28359885220972,7.77135084111175,
59.3808721243058));
#182011=CARTESIAN_POINT('Ctrl Pts',(-5.73078628072618,5.72187571446011,
59.5395395895922));
#182012=CARTESIAN_POINT('Ctrl Pts',(-7.74881827407838,2.30617944845616,
59.6982070548786));
#182013=CARTESIAN_POINT('Ctrl Pts',(-8.0064041132583,-3.05220020879696,
59.9097636752605));
#182014=CARTESIAN_POINT('Ctrl Pts',(-4.21589353186778,-7.44992704201823,
60.1213202956424));
#182015=CARTESIAN_POINT('Ctrl Pts',(1.09265632163192,-8.00647171181022,
60.3328769160243));
#182016=CARTESIAN_POINT('Ctrl Pts',(6.05795565739796,-6.04783799852794,
60.5444335364063));
#182017=CARTESIAN_POINT('Ctrl Pts',(8.53147183715803,-0.795249162941086,
60.7559901567881));
#182018=CARTESIAN_POINT('Ctrl Pts',(6.84751260599863,4.29816465527584,60.9675467771701));
#182019=CARTESIAN_POINT('Ctrl Pts',(3.98803057425647,7.04821858527979,61.1262142424565));
#182020=CARTESIAN_POINT('Ctrl Pts',(0.117737167502885,8.09906510486547,
61.284881707743));
#182021=CARTESIAN_POINT('Ctrl Pts',(-3.76081845462485,7.16565922491463,
61.4435491730294));
#182022=CARTESIAN_POINT('Ctrl Pts',(-6.73227275777555,4.50391175850224,
61.6022166383157));
#182023=CARTESIAN_POINT('Ctrl Pts',(-8.06602823683544,0.72177667575291,
61.7608841036022));
#182024=CARTESIAN_POINT('Ctrl Pts',(-7.42715740551509,-3.1937409360928,
61.9195515688887));
#182025=CARTESIAN_POINT('Ctrl Pts',(-4.19196689838406,-7.47300785910407,
62.1311081892706));
#182026=CARTESIAN_POINT('Ctrl Pts',(1.53594431257073,-8.4211665624259,62.3426648096525));
#182027=CARTESIAN_POINT('Ctrl Pts',(5.96848603098247,-5.44744542030362,
62.5542214300343));
#182028=CARTESIAN_POINT('Ctrl Pts',(8.5260686431671,-0.762446519725676,
62.7657780504163));
#182029=CARTESIAN_POINT('Ctrl Pts',(7.06007767884898,4.85527919979866,62.9773346707981));
#182030=CARTESIAN_POINT('Ctrl Pts',(2.50389820398932,7.68720638966013,63.1888912911801));
#182031=CARTESIAN_POINT('Ctrl Pts',(-1.45353695814277,7.96674358809175,
63.3475587564665));
#182032=CARTESIAN_POINT('Ctrl Pts',(-5.09845109774291,6.29400619775557,
63.5062262217529));
#182033=CARTESIAN_POINT('Ctrl Pts',(-7.47845238908096,3.09243875291006,
63.6648936870394));
#182034=CARTESIAN_POINT('Ctrl Pts',(-8.05466705580809,-0.855018265033708,
63.8235611523257));
#182035=CARTESIAN_POINT('Ctrl Pts',(-6.65563175880953,-4.61349531030578,
63.9822286176123));
#182036=CARTESIAN_POINT('Ctrl Pts',(-3.65653188946597,-7.21057714988829,
64.1408960828986));
#182037=CARTESIAN_POINT('Ctrl Pts',(1.56910276906502,-8.42355919071576,
64.3524527032806));
#182038=CARTESIAN_POINT('Ctrl Pts',(6.57453247811738,-5.48185132027664,
64.5640093236623));
#182039=CARTESIAN_POINT('Ctrl Pts',(8.07271737558231,-0.35877748423116,
64.7755659440445));
#182040=CARTESIAN_POINT('Ctrl Pts',(7.03491326733044,4.87700384709477,64.9871225644261));
#182041=CARTESIAN_POINT('Ctrl Pts',(2.31018045491571,8.25115138663115,65.1986791848083));
#182042=CARTESIAN_POINT('Ctrl Pts',(-3.00245665374948,7.50652398487662,
65.41023580519));
#182043=CARTESIAN_POINT('Ctrl Pts',(-6.22012248750458,5.18573517714964,
65.5689032704766));
#182044=CARTESIAN_POINT('Ctrl Pts',(-7.94706094328348,1.56618644394587,
65.7275707357629));
#182045=CARTESIAN_POINT('Ctrl Pts',(-7.72330171704765,-2.4168239827715,
65.8862382010493));
#182046=CARTESIAN_POINT('Ctrl Pts',(-5.63669873514582,-5.81690166520522,
66.0449056663359));
#182047=CARTESIAN_POINT('Ctrl Pts',(-2.15454561453617,-7.80638881186242,
66.2035731316222));
#182048=CARTESIAN_POINT('Ctrl Pts',(1.81208500210048,-7.87902254333207,
66.3622405969087));
#182049=CARTESIAN_POINT('Ctrl Pts',(6.60152489569881,-5.46244468995782,
66.5737972172905));
#182050=CARTESIAN_POINT('Ctrl Pts',(8.56009122032943,0.00308270630419909,
66.7853538376725));
#182051=CARTESIAN_POINT('Ctrl Pts',(6.42820403667042,4.8964967039868,66.9969104580544));
#182052=CARTESIAN_POINT('Ctrl Pts',(2.27694047637668,8.25170971802063,67.2084670784361));
#182053=CARTESIAN_POINT('Ctrl Pts',(-3.51250010768767,7.81541911434526,
67.4200236988182));
#182054=CARTESIAN_POINT('Ctrl Pts',(-7.11455442374939,3.84002130784199,
67.6315803192001));
#182055=CARTESIAN_POINT('Ctrl Pts',(-8.09825670351394,-0.00338394434941844,
67.7902477844866));
#182056=CARTESIAN_POINT('Ctrl Pts',(-7.10527744608323,-3.88892659067283,
67.9489152497728));
#182057=CARTESIAN_POINT('Ctrl Pts',(-4.38166524303238,-6.80378110128866,
68.1075827150595));
#182058=CARTESIAN_POINT('Ctrl Pts',(-0.601204811537375,-8.07757825019637,
68.2662501803458));
#182059=CARTESIAN_POINT('Ctrl Pts',(3.34705139145844,-7.37421318311479,
68.4249176456322));
#182060=CARTESIAN_POINT('Ctrl Pts',(6.43922018414456,-4.88866972839014,
68.5835851109187));
#182061=CARTESIAN_POINT('Ctrl Pts',(8.56838307348488,0.0352766976451838,
68.7951417313005));
#182062=CARTESIAN_POINT('Ctrl Pts',(6.57058246548689,5.48658521009879,69.0066983516824));
#182063=CARTESIAN_POINT('Ctrl Pts',(1.79861211939978,7.87797445750923,69.2182549720644));
#182064=CARTESIAN_POINT('Ctrl Pts',(-3.53837993476094,7.79455185631092,
69.4298115924462));
#182065=CARTESIAN_POINT('Ctrl Pts',(-7.70407363508685,3.75042429126886,
69.6413682128281));
#182066=CARTESIAN_POINT('Ctrl Pts',(-7.92285164794354,-1.60968011041032,
69.8529248332102));
#182067=CARTESIAN_POINT('Ctrl Pts',(-6.21578648478412,-5.19093165652013,
70.0115922984965));
#182068=CARTESIAN_POINT('Ctrl Pts',(-2.96400137263525,-7.53813063540808,
70.1702597637831));
#182069=CARTESIAN_POINT('Ctrl Pts',(0.994694301361778,-8.03125213295468,
70.3289272290693));
#182070=CARTESIAN_POINT('Ctrl Pts',(4.7134718501872,-6.58725289714569,70.4875946943558));
#182071=CARTESIAN_POINT('Ctrl Pts',(7.29437112929025,-3.51765872637811,
70.6462621596422));
#182072=CARTESIAN_POINT('Ctrl Pts',(8.07616119634359,0.371844892188463,
70.8049296249286));
#182073=CARTESIAN_POINT('Ctrl Pts',(6.55632324899169,5.51661657124278,71.0164862453105));
#182074=CARTESIAN_POINT('Ctrl Pts',(1.52987856295196,8.42227064312582,71.2280428656924));
#182075=CARTESIAN_POINT('Ctrl Pts',(-3.66620507662212,7.20114070445578,
71.4395994860744));
#182076=CARTESIAN_POINT('Ctrl Pts',(-7.71057544116701,3.71782161614985,
71.6511561064562));
#182077=CARTESIAN_POINT('Ctrl Pts',(-8.31809034521527,-2.05616291869497,
71.8627127268381));
#182078=CARTESIAN_POINT('Ctrl Pts',(-5.05199765060271,-6.31189100281976,
72.0742693472201));
#182079=CARTESIAN_POINT('Ctrl Pts',(-1.44687847137091,-7.96795555811971,
72.2329368125064));
#182080=CARTESIAN_POINT('Ctrl Pts',(2.55367422908007,-7.68683716135536,
72.391604277793));
#182081=CARTESIAN_POINT('Ctrl Pts',(5.90914556872033,-5.52923378271561,
72.5502717430793));
#182082=CARTESIAN_POINT('Ctrl Pts',(7.8393437120909,-2.03799111312154,72.7089392083658));
#182083=CARTESIAN_POINT('Ctrl Pts',(7.85438846097099,1.97239828413365,72.8676066736522));
#182084=CARTESIAN_POINT('Ctrl Pts',(5.96275831076774,5.45968512100677,73.0262741389386));
#182085=CARTESIAN_POINT('Ctrl Pts',(1.49968985904912,8.43619364796968,73.2378307593206));
#182086=CARTESIAN_POINT('Ctrl Pts',(-4.2212582536141,7.44688860932765,73.4493873797026));
#182087=CARTESIAN_POINT('Ctrl Pts',(-7.42853893893759,3.18029815298939,
73.6609440000843));
#182088=CARTESIAN_POINT('Ctrl Pts',(-8.30219487298872,-2.08536123833689,
73.8725006204664));
#182089=CARTESIAN_POINT('Ctrl Pts',(-5.06941801176177,-6.90792544555923,
74.0840572408481));
#182090=CARTESIAN_POINT('Ctrl Pts',(0.164863081854742,-8.08303584412526,
74.2956138612302));
#182091=CARTESIAN_POINT('Ctrl Pts',(3.99391952962493,-7.04488324090387,
74.4542813265165));
#182092=CARTESIAN_POINT('Ctrl Pts',(6.88549477799248,-4.26599100745655,
74.6129487918029));
#182093=CARTESIAN_POINT('Ctrl Pts',(8.07955452613269,-0.459593554675651,
74.7716162570894));
#182094=CARTESIAN_POINT('Ctrl Pts',(7.32484310761663,3.45765687457021,74.9302837223757));
#182095=CARTESIAN_POINT('Ctrl Pts',(4.76704696471102,6.54652857042015,75.0889511876623));
#182096=CARTESIAN_POINT('Ctrl Pts',(1.08041685387929,8.01219992979621,75.2476186529485));
#182097=CARTESIAN_POINT('Ctrl Pts',(-4.25335765323495,7.43823780293737,
75.4591752733308));
#182098=CARTESIAN_POINT('Ctrl Pts',(-8.01216052959904,3.01337930758371,
75.6707318937123));
#182099=CARTESIAN_POINT('Ctrl Pts',(-7.74126660819681,-2.31738611587211,
75.8822885140946));
#182100=CARTESIAN_POINT('Ctrl Pts',(-5.03850667497429,-6.92016052484901,
76.0938451344761));
#182101=CARTESIAN_POINT('Ctrl Pts',(0.533350586423094,-8.55184015819647,
76.3054017548582));
#182102=CARTESIAN_POINT('Ctrl Pts',(5.30516599953248,-6.10064439306021,
76.51695837524));
#182103=CARTESIAN_POINT('Ctrl Pts',(7.58005274967108,-2.85036373105114,
76.6756258405266));
#182104=CARTESIAN_POINT('Ctrl Pts',(8.01988368877764,1.13586232965973,76.8342933058129));
#182105=CARTESIAN_POINT('Ctrl Pts',(6.49804381810543,4.82346909539517,76.9929607710994));
#182106=CARTESIAN_POINT('Ctrl Pts',(3.4088897605638,7.34766549414064,77.1516282363858));
#182107=CARTESIAN_POINT('Ctrl Pts',(-0.533978119564296,8.08063366666963,
77.3102957016723));
#182108=CARTESIAN_POINT('Ctrl Pts',(-4.30364004138297,6.84407266818358,
77.4689631669586));
#182109=CARTESIAN_POINT('Ctrl Pts',(-8.03126455947391,2.98617188304975,
77.6805197873407));
#182110=CARTESIAN_POINT('Ctrl Pts',(-8.08243903153417,-2.81945925754779,
77.8920764077226));
#182111=CARTESIAN_POINT('Ctrl Pts',(-4.45916608132687,-6.73894093818632,
78.1036330281042));
#182112=CARTESIAN_POINT('Ctrl Pts',(0.564923425535108,-8.54143036772646,
78.3151896484865));
#182113=CARTESIAN_POINT('Ctrl Pts',(5.88844605519194,-6.22451893679133,
78.526746268868));
#182114=CARTESIAN_POINT('Ctrl Pts',(7.98189786540439,-1.28528392171771,
78.7383028892501));
#182115=CARTESIAN_POINT('Ctrl Pts',(7.64622099088389,2.66778515732707,78.8969703545365));
#182116=CARTESIAN_POINT('Ctrl Pts',(5.43006240590164,6.01025289663214,79.0556378198229));
#182117=CARTESIAN_POINT('Ctrl Pts',(1.89902288606984,7.86664729439632,79.2143052851094));
#182118=CARTESIAN_POINT('Ctrl Pts',(-2.09005686769106,7.82562329167963,
79.3729727503958));
#182119=CARTESIAN_POINT('Ctrl Pts',(-5.5870386655436,5.86231797472716,79.5316402156822));
#182120=CARTESIAN_POINT('Ctrl Pts',(-7.68920659265237,2.49774904037289,
79.6903076809687));
#182121=CARTESIAN_POINT('Ctrl Pts',(-8.07967631327886,-2.85258893148296,
79.9018643013505));
#182122=CARTESIAN_POINT('Ctrl Pts',(-4.39945838421227,-7.34301961927268,
80.1134209217327));
#182123=CARTESIAN_POINT('Ctrl Pts',(0.893646742598228,-8.03111963605721,
80.3249775421143));
#182124=CARTESIAN_POINT('Ctrl Pts',(5.90601885117144,-6.19629829277502,
80.5365341624965));
#182125=CARTESIAN_POINT('Ctrl Pts',(8.50911149048599,-1.00670481366578,
80.7480907828781));
#182126=CARTESIAN_POINT('Ctrl Pts',(6.95205909401174,4.12692653757503,80.9596474032601));
#182127=CARTESIAN_POINT('Ctrl Pts',(4.16169756844071,6.94708906204051,81.1183148685464));
#182128=CARTESIAN_POINT('Ctrl Pts',(0.318671665282749,8.09364973193226,
81.276982333833));
#182129=CARTESIAN_POINT('Ctrl Pts',(-3.58185128283906,7.25677400529152,
81.4356497991193));
#182130=CARTESIAN_POINT('Ctrl Pts',(-6.618439408729,4.6695800032171,81.5943172644059));
#182131=CARTESIAN_POINT('Ctrl Pts',(-8.04563435915725,0.921705400784701,
81.7529847296922));
#182132=CARTESIAN_POINT('Ctrl Pts',(-7.50412016629928,-3.00845954317373,
81.9116521949786));
#182133=CARTESIAN_POINT('Ctrl Pts',(-4.37611184709195,-7.36668704650339,
82.1232088153607));
#182134=CARTESIAN_POINT('Ctrl Pts',(1.32650797174266,-8.45668657361387,
82.3347654357425));
#182135=CARTESIAN_POINT('Ctrl Pts',(5.83147495608897,-5.5938704798848,82.5463220561243));
#182136=CARTESIAN_POINT('Ctrl Pts',(8.50452392724124,-0.973778195699686,
82.7578786765063));
#182137=CARTESIAN_POINT('Ctrl Pts',(7.17838299269727,4.67859493326084,82.9694352968883));
#182138=CARTESIAN_POINT('Ctrl Pts',(2.69387807358101,7.62270747292933,83.18099191727));
#182139=CARTESIAN_POINT('Ctrl Pts',(-1.25540207440457,8.00035866187685,
83.3396593825567));
#182140=CARTESIAN_POINT('Ctrl Pts',(-4.94070130429781,6.41858148154023,
83.4983268478428));
#182141=CARTESIAN_POINT('Ctrl Pts',(-7.39941366601822,3.27705736528888,
83.6569943131295));
#182142=CARTESIAN_POINT('Ctrl Pts',(-8.07340337306009,-0.654885936116582,
83.8156617784157));
#182143=CARTESIAN_POINT('Ctrl Pts',(-6.76806196634699,-4.44692144148893,
83.9743292437024));
#182144=CARTESIAN_POINT('Ctrl Pts',(-3.8343297339649,-7.11762346464079,
84.1329967089886));
#182145=CARTESIAN_POINT('Ctrl Pts',(1.35959684736402,-8.45990126136336,
84.3445533293706));
#182146=CARTESIAN_POINT('Ctrl Pts',(6.43648104125485,-5.64330426337308,
84.5561099497524));
#182147=CARTESIAN_POINT('Ctrl Pts',(8.06132892477432,-0.558983967405612,
84.7676665701346));
#182148=CARTESIAN_POINT('Ctrl Pts',(7.15376540658539,4.70093732259667,84.9792231905161));
#182149=CARTESIAN_POINT('Ctrl Pts',(2.51421374279191,8.19128574736206,85.1907798108983));
#182150=CARTESIAN_POINT('Ctrl Pts',(-2.815264752711,7.57871576623082,85.40233643128));
#182151=CARTESIAN_POINT('Ctrl Pts',(-6.0895280253515,5.33848494570748,85.5610038965666));
#182152=CARTESIAN_POINT('Ctrl Pts',(-7.90575045630871,1.76290309887863,
85.7196713618529));
#182153=CARTESIAN_POINT('Ctrl Pts',(-7.78089482015652,-2.22443327027643,
85.8783388271395));
#182154=CARTESIAN_POINT('Ctrl Pts',(-5.77930409579335,-5.67524112102804,
86.0370062924257));
#182155=CARTESIAN_POINT('Ctrl Pts',(-2.34759045622567,-7.75052205576662,
86.1956737577123));
#182156=CARTESIAN_POINT('Ctrl Pts',(1.61601643149944,-7.92156166335252,
86.3543412229986));
#182157=CARTESIAN_POINT('Ctrl Pts',(6.46394670487,-5.624573400355,86.5658978433806));
#182158=CARTESIAN_POINT('Ctrl Pts',(8.55753192244567,-0.209328927201481,
86.7774544637624));
#182159=CARTESIAN_POINT('Ctrl Pts',(6.54772668871323,4.73547910132988,86.9890110841444));
#182160=CARTESIAN_POINT('Ctrl Pts',(2.48099785385986,8.1926687259147,87.2005677045262));
#182161=CARTESIAN_POINT('Ctrl Pts',(-3.31748621121201,7.9001720346963,87.4121243249083));
#182162=CARTESIAN_POINT('Ctrl Pts',(-7.01707718659673,4.01537993850101,
87.6236809452901));
#182163=CARTESIAN_POINT('Ctrl Pts',(-8.09584708698749,0.197567788879703,
87.7823484105764));
#182164=CARTESIAN_POINT('Ctrl Pts',(-7.19958970297868,-3.71141828984888,
87.941015875863));
#182165=CARTESIAN_POINT('Ctrl Pts',(-4.54914554234009,-6.69295916697977,
88.0996833411494));
#182166=CARTESIAN_POINT('Ctrl Pts',(-0.801457265437198,-8.0601726944985,
88.2583508064357));
#182167=CARTESIAN_POINT('Ctrl Pts',(3.16303655326425,-7.45499650233329,
88.4170182717223));
#182168=CARTESIAN_POINT('Ctrl Pts',(6.31592966041965,-5.04694767337688,
88.5756857370086));
#182169=CARTESIAN_POINT('Ctrl Pts',(8.56662008628893,-0.177350603524844,
88.7872423573906));
#182170=CARTESIAN_POINT('Ctrl Pts',(6.70470377310268,5.3218529215285,88.9987989777724));
#182171=CARTESIAN_POINT('Ctrl Pts',(1.99354288991289,7.83091781691632,89.2103555981544));
#182172=CARTESIAN_POINT('Ctrl Pts',(-3.34387587101894,7.87995338581739,
89.4219122185362));
#182173=CARTESIAN_POINT('Ctrl Pts',(-7.60863814175591,3.94043888002301,
89.6334688389183));
#182174=CARTESIAN_POINT('Ctrl Pts',(-7.96035478355009,-1.41258628521722,
89.8450254593));
#182175=CARTESIAN_POINT('Ctrl Pts',(-6.34268067256004,-5.03509433605964,
90.0036929245866));
#182176=CARTESIAN_POINT('Ctrl Pts',(-3.15014039304159,-7.46226059030319,
90.1623603898729));
#182177=CARTESIAN_POINT('Ctrl Pts',(0.795099983388211,-8.05346159068648,
90.3210278551594));
#182178=CARTESIAN_POINT('Ctrl Pts',(4.54856395466749,-6.70218498429923,
90.4796953204458));
#182179=CARTESIAN_POINT('Ctrl Pts',(7.20483765059431,-3.69757860168855,
90.6383627857322));
#182180=CARTESIAN_POINT('Ctrl Pts',(8.08290139834275,0.171327983207752,
90.7970302510186));
#182181=CARTESIAN_POINT('Ctrl Pts',(6.69119414748828,5.35222886469354,91.0085868714007));
#182182=CARTESIAN_POINT('Ctrl Pts',(1.73839828340533,8.38171477751168,91.2201434917824));
#182183=CARTESIAN_POINT('Ctrl Pts',(-3.48638659800205,7.28989681673174,
91.4317001121644));
#182184=CARTESIAN_POINT('Ctrl Pts',(-7.61594695082403,3.90800758003743,
91.6432567325462));
#182185=CARTESIAN_POINT('Ctrl Pts',(-8.36655083502915,-1.84912413423635,
91.8548133529282));
#182186=CARTESIAN_POINT('Ctrl Pts',(-5.20706574932211,-6.18458685574747,
92.0663699733101));
#182187=CARTESIAN_POINT('Ctrl Pts',(-1.64415034353059,-7.9295991533635,
92.2250374385965));
#182188=CARTESIAN_POINT('Ctrl Pts',(2.3621462120266,-7.74783730401467,92.383704903883));
#182189=CARTESIAN_POINT('Ctrl Pts',(5.7701232639135,-5.67416117964458,92.5423723691693));
#182190=CARTESIAN_POINT('Ctrl Pts',(7.78635899964589,-2.23188958977203,
92.7010398344559));
#182191=CARTESIAN_POINT('Ctrl Pts',(7.90091319144752,1.77689162371117,92.8597072997422));
#182192=CARTESIAN_POINT('Ctrl Pts',(6.09639927576183,5.31004370259175,93.0183747650287));
#182193=CARTESIAN_POINT('Ctrl Pts',(1.70856436375901,8.39638260574568,93.2299313854105));
#182194=CARTESIAN_POINT('Ctrl Pts',(-4.03517086418892,7.54934216757803,
93.4414880057924));
#182195=CARTESIAN_POINT('Ctrl Pts',(-7.34733543081567,3.36365116970041,
93.6530446261744));
#182196=CARTESIAN_POINT('Ctrl Pts',(-8.35138479902285,-1.87870792778163,
93.8646012465563));
#182197=CARTESIAN_POINT('Ctrl Pts',(-5.23927076021774,-6.78000543317708,
94.0761578669382));
#182198=CARTESIAN_POINT('Ctrl Pts',(-0.03576071327238,-8.08463795065846,
94.2877144873201));
#182199=CARTESIAN_POINT('Ctrl Pts',(3.81787759158665,-7.14181922308119,
94.4463819526065));
#182200=CARTESIAN_POINT('Ctrl Pts',(6.77751790271065,-4.43553491019332,
94.605049417893));
#182201=CARTESIAN_POINT('Ctrl Pts',(8.06566255744928,-0.659938011645058,
94.7637168831795));
#182202=CARTESIAN_POINT('Ctrl Pts',(7.40838573974634,3.27483184211492,94.9223843484658));
#182203=CARTESIAN_POINT('Ctrl Pts',(4.9280259771172,6.42622521736914,95.0810518137522));
#182204=CARTESIAN_POINT('Ctrl Pts',(1.27889791082725,7.98291927025678,95.2397192790387));
#182205=CARTESIAN_POINT('Ctrl Pts',(-4.0674715610131,7.54149967463055,95.4512758994206));
#182206=CARTESIAN_POINT('Ctrl Pts',(-7.93492590795773,3.21124827752124,
95.6628325198024));
#182207=CARTESIAN_POINT('Ctrl Pts',(-7.79637889098973,-2.1245596921605,
95.8743891401844));
#182208=CARTESIAN_POINT('Ctrl Pts',(-5.20869192738245,-6.79305464430902,
96.0859457605662));
#182209=CARTESIAN_POINT('Ctrl Pts',(0.32101919849777,-8.56233974141997,
96.2975023809482));
#182210=CARTESIAN_POINT('Ctrl Pts',(5.15210277886213,-6.23053426315196,
96.5090590013301));
#182211=CARTESIAN_POINT('Ctrl Pts',(7.50709055485341,-3.03731311627524,
96.6677264666165));
#182212=CARTESIAN_POINT('Ctrl Pts',(8.04540311654855,0.935991074457848,
96.826393931903));
#182213=CARTESIAN_POINT('Ctrl Pts',(6.61610676550725,4.66172204925334,96.9850613971894));
#182214=CARTESIAN_POINT('Ctrl Pts',(3.58945996231984,7.25896364534505,97.1437288624758));
#182215=CARTESIAN_POINT('Ctrl Pts',(-0.331984144423014,8.09484453530492,
97.3023963277622));
#182216=CARTESIAN_POINT('Ctrl Pts',(-4.13483212670458,6.9426376342695,97.4610637930487));
#182217=CARTESIAN_POINT('Ctrl Pts',(-7.94945653522564,3.19785807260161,
97.6726204134305));
#182218=CARTESIAN_POINT('Ctrl Pts',(-8.21167960970159,-4.09854069807359,
97.937066188908));
#182219=CARTESIAN_POINT('Ctrl Pts',(-2.22263135552021,-8.275446197766,98.2015119643853));
#182220=CARTESIAN_POINT('Ctrl Pts',(3.06251395333299,-7.47745566371039,
98.4130685847673));
#182221=CARTESIAN_POINT('Ctrl Pts',(6.27029174620337,-5.13167437815679,
98.5717360500536));
#182222=CARTESIAN_POINT('Ctrl Pts',(7.95736644719291,-1.49394517189156,
98.7304035153404));
#182223=CARTESIAN_POINT('Ctrl Pts',(7.7051980908551,2.48345330633745,98.8890709806263));
#182224=CARTESIAN_POINT('Ctrl Pts',(5.57898371978856,5.87036363237872,99.0477442629553));
#182225=CARTESIAN_POINT('Ctrl Pts',(3.25605702020626,7.16952801912672,99.1535283901882));
#182226=CARTESIAN_POINT('Ctrl Pts',(2.00918284212126,7.50340179718649,99.2064233623258));
#182227=CARTESIAN_POINT('Ctrl Pts',(-6.17201598240879,5.32232153904337,
-0.657447214020203));
#182228=CARTESIAN_POINT('Ctrl Pts',(-7.05661567643055,4.2965029020642,-0.60454249319458));
#182229=CARTESIAN_POINT('Ctrl Pts',(-8.30460012783212,1.79807814514246,
-0.498748617273481));
#182230=CARTESIAN_POINT('Ctrl Pts',(-8.14915213400464,-2.39503477011331,
-0.340065586256907));
#182231=CARTESIAN_POINT('Ctrl Pts',(-6.01967976551396,-5.99363557917286,
-0.181398120970476));
#182232=CARTESIAN_POINT('Ctrl Pts',(-2.40877456199585,-8.15273538333176,
-0.0227306556840495));
#182233=CARTESIAN_POINT('Ctrl Pts',(1.75834180979301,-8.29349104933222,
0.135936809602381));
#182234=CARTESIAN_POINT('Ctrl Pts',(6.81343712395487,-5.86535701987734,
0.347493429984283));
#182235=CARTESIAN_POINT('Ctrl Pts',(9.54195894196003,1.29323553737407,0.611939205461667));
#182236=CARTESIAN_POINT('Ctrl Pts',(5.0068590584849,7.46682392155477,0.876384980939047));
#182237=CARTESIAN_POINT('Ctrl Pts',(-0.512538772618678,8.46270402481564,
1.08794160132095));
#182238=CARTESIAN_POINT('Ctrl Pts',(-4.49111326352922,7.21691544450829,
1.24660906660738));
#182239=CARTESIAN_POINT('Ctrl Pts',(-7.39881792966678,4.17677760331887,
1.40527653189381));
#182240=CARTESIAN_POINT('Ctrl Pts',(-8.49055988419928,0.137227805190378,
1.56394399718024));
#182241=CARTESIAN_POINT('Ctrl Pts',(-7.53062837975034,-3.93804937038376,
1.72261146246667));
#182242=CARTESIAN_POINT('Ctrl Pts',(-4.71796379646677,-7.06641305153905,
1.88127892775309));
#182243=CARTESIAN_POINT('Ctrl Pts',(-0.79018593232073,-8.44565265941745,
2.03994639303953));
#182244=CARTESIAN_POINT('Ctrl Pts',(4.77662445382059,-7.61591549408909,
2.25150301342142));
#182245=CARTESIAN_POINT('Ctrl Pts',(8.52816518397885,-2.81671375597811,
2.46305963380334));
#182246=CARTESIAN_POINT('Ctrl Pts',(8.01635168825888,2.76014623244002,2.67461625418524));
#182247=CARTESIAN_POINT('Ctrl Pts',(4.98635083889706,7.46985904841845,2.88617287456715));
#182248=CARTESIAN_POINT('Ctrl Pts',(-0.924520356462571,8.94234775455389,
3.09772949494905));
#182249=CARTESIAN_POINT('Ctrl Pts',(-5.82220414120115,6.16880266514092,
3.30928611533096));
#182250=CARTESIAN_POINT('Ctrl Pts',(-8.06816498152606,2.66425108595449,
3.46795358061738));
#182251=CARTESIAN_POINT('Ctrl Pts',(-8.35893323744424,-1.5334140393396,
3.62662104590382));
#182252=CARTESIAN_POINT('Ctrl Pts',(-6.60599159799001,-5.33421058304081,
3.78528851119024));
#182253=CARTESIAN_POINT('Ctrl Pts',(-3.25969653764494,-7.84840872900535,
3.94395597647667));
#182254=CARTESIAN_POINT('Ctrl Pts',(0.905036893642654,-8.44833621522575,
4.1026234417631));
#182255=CARTESIAN_POINT('Ctrl Pts',(4.80404436523976,-6.99095285530132,
4.26129090704952));
#182256=CARTESIAN_POINT('Ctrl Pts',(8.54698316019777,-2.78734255264185,
4.47284752743144));
#182257=CARTESIAN_POINT('Ctrl Pts',(8.35257952803235,3.3010470592481,4.68440414781333));
#182258=CARTESIAN_POINT('Ctrl Pts',(4.38673881922155,7.2551398805805,4.89596076819524));
#182259=CARTESIAN_POINT('Ctrl Pts',(-0.957165854837313,8.93008003688911,
5.10751738857714));
#182260=CARTESIAN_POINT('Ctrl Pts',(-6.43896908919455,6.2737451428744,5.31907400895906));
#182261=CARTESIAN_POINT('Ctrl Pts',(-8.4225586316336,1.00636408820458,5.53063062934095));
#182262=CARTESIAN_POINT('Ctrl Pts',(-7.90176052552384,-3.12340509109876,
5.68929809462739));
#182263=CARTESIAN_POINT('Ctrl Pts',(-5.43569013465026,-6.53271861328957,
5.84796555991382));
#182264=CARTESIAN_POINT('Ctrl Pts',(-1.65468776311683,-8.32796088696628,
6.00663302520024));
#182265=CARTESIAN_POINT('Ctrl Pts',(2.52542173804131,-8.11451691537931,
6.16530049048667));
#182266=CARTESIAN_POINT('Ctrl Pts',(6.10752001228779,-5.90691781284157,
6.32396795577311));
#182267=CARTESIAN_POINT('Ctrl Pts',(8.16752607455826,-2.28993022775634,
6.48263542105952));
#182268=CARTESIAN_POINT('Ctrl Pts',(8.34826776562736,3.33565979134341,6.69419204144145));
#182269=CARTESIAN_POINT('Ctrl Pts',(4.29833574721033,7.88586113839222,6.90574866182333));
#182270=CARTESIAN_POINT('Ctrl Pts',(-1.27997205123254,8.38106220513736,
7.11730528220525));
#182271=CARTESIAN_POINT('Ctrl Pts',(-6.45618537530488,6.24340984473629,
7.32886190258714));
#182272=CARTESIAN_POINT('Ctrl Pts',(-8.9633486454374,0.691796206322683,
7.54041852296907));
#182273=CARTESIAN_POINT('Ctrl Pts',(-7.11170820944491,-4.62340447823024,
7.75197514335095));
#182274=CARTESIAN_POINT('Ctrl Pts',(-4.06600105329151,-7.46063765270232,
7.91064260863739));
#182275=CARTESIAN_POINT('Ctrl Pts',(0.0117368987423702,-8.4984117320148,
8.06931007392382));
#182276=CARTESIAN_POINT('Ctrl Pts',(4.06500630606157,-7.45443813195372,
8.22797753921025));
#182277=CARTESIAN_POINT('Ctrl Pts',(7.13780493916943,-4.61247009442929,
8.38664500449667));
#182278=CARTESIAN_POINT('Ctrl Pts',(8.47384110579392,-0.622491497167233,
8.5453124697831));
#182279=CARTESIAN_POINT('Ctrl Pts',(7.73823666162773,3.47447204539893,8.70397993506954));
#182280=CARTESIAN_POINT('Ctrl Pts',(4.27284971438061,7.90967485102876,8.91553655545142));
#182281=CARTESIAN_POINT('Ctrl Pts',(-1.75193518088393,8.80870133514469,
9.12709317583335));
#182282=CARTESIAN_POINT('Ctrl Pts',(-6.3522996305101,5.61505312017836,9.33864979621524));
#182283=CARTESIAN_POINT('Ctrl Pts',(-8.95713255407061,0.657474333040693,
9.55020641659717));
#182284=CARTESIAN_POINT('Ctrl Pts',(-7.32539921461132,-5.21140358034675,
9.76176303697903));
#182285=CARTESIAN_POINT('Ctrl Pts',(-2.49837894152679,-8.10619302078068,
9.97331965736098));
#182286=CARTESIAN_POINT('Ctrl Pts',(1.65789584672137,-8.33335827333214,
10.1319871226474));
#182287=CARTESIAN_POINT('Ctrl Pts',(5.45371364459879,-6.51767958742603,
10.2906545879339));
#182288=CARTESIAN_POINT('Ctrl Pts',(7.89702487857384,-3.11928232108554,
10.4493220532203));
#182289=CARTESIAN_POINT('Ctrl Pts',(8.43559070412863,1.03147912923697,10.6079895185067));
#182290=CARTESIAN_POINT('Ctrl Pts',(6.90514684855951,4.95100249950638,10.7666569837931));
#182291=CARTESIAN_POINT('Ctrl Pts',(3.71552607525479,7.62542645428566,10.9253244490795));
#182292=CARTESIAN_POINT('Ctrl Pts',(-1.78676051222955,8.8106576260014,11.1368810694615));
#182293=CARTESIAN_POINT('Ctrl Pts',(-6.98865629795398,5.64102643486689,
11.3484376898434));
#182294=CARTESIAN_POINT('Ctrl Pts',(-8.47479651957782,0.241570051858162,
11.5599943102253));
#182295=CARTESIAN_POINT('Ctrl Pts',(-7.29863731965333,-5.23377391238505,
11.7715509306072));
#182296=CARTESIAN_POINT('Ctrl Pts',(-2.28573880064005,-8.69457296627776,
11.9831075509891));
#182297=CARTESIAN_POINT('Ctrl Pts',(3.27512779064737,-7.82469172431395,
12.194664171371));
#182298=CARTESIAN_POINT('Ctrl Pts',(6.61191217838697,-5.33629985060691,
12.3533316366574));
#182299=CARTESIAN_POINT('Ctrl Pts',(8.36313795743936,-1.51031891548454,
12.5119991019438));
#182300=CARTESIAN_POINT('Ctrl Pts',(8.06188546056129,2.66438115746247,12.6706665672303));
#182301=CARTESIAN_POINT('Ctrl Pts',(5.8161235376237,6.19643822826732,12.8293340325167));
#182302=CARTESIAN_POINT('Ctrl Pts',(2.129895080009,8.22538909100614,12.9880014978031));
#182303=CARTESIAN_POINT('Ctrl Pts',(-2.03257114030819,8.23534560204998,
13.1466689630895));
#182304=CARTESIAN_POINT('Ctrl Pts',(-7.01664901574451,5.62021685707332,
13.3582255834715));
#182305=CARTESIAN_POINT('Ctrl Pts',(-8.98004044570451,-0.146183731344905,
13.5697822038533));
#182306=CARTESIAN_POINT('Ctrl Pts',(-6.66183439050809,-5.24409140763651,
13.7813388242353));
#182307=CARTESIAN_POINT('Ctrl Pts',(-2.25085857932651,-8.69460359911083,
13.9928954446172));
#182308=CARTESIAN_POINT('Ctrl Pts',(3.81535492978966,-8.14022528499111,
14.2044520649991));
#182309=CARTESIAN_POINT('Ctrl Pts',(7.52775656787826,-3.90962193573543,
14.416008685381));
#182310=CARTESIAN_POINT('Ctrl Pts',(8.49554099697729,0.138787315586332,
14.5746761506674));
#182311=CARTESIAN_POINT('Ctrl Pts',(7.38895437261531,4.19839171600769,14.7333436159538));
#182312=CARTESIAN_POINT('Ctrl Pts',(4.48303139811294,7.21078037489595,14.8920110812403));
#182313=CARTESIAN_POINT('Ctrl Pts',(0.495810896673869,8.48394432303586,
15.0506785465267));
#182314=CARTESIAN_POINT('Ctrl Pts',(-3.63442052989092,7.68013451459002,
15.2093460118131));
#182315=CARTESIAN_POINT('Ctrl Pts',(-6.83679903633618,5.02100005600181,
15.3680134770995));
#182316=CARTESIAN_POINT('Ctrl Pts',(-8.9882015129228,-0.180095790543731,
15.5795700974815));
#182317=CARTESIAN_POINT('Ctrl Pts',(-6.80134439463898,-5.86551025191433,
15.7911267178633));
#182318=CARTESIAN_POINT('Ctrl Pts',(-1.75530226611185,-8.2945431515416,
16.0026833382453));
#182319=CARTESIAN_POINT('Ctrl Pts',(3.84215607599829,-8.11790199358606,
16.2142399586272));
#182320=CARTESIAN_POINT('Ctrl Pts',(8.14470429666455,-3.80578413084255,
16.4257965790091));
#182321=CARTESIAN_POINT('Ctrl Pts',(8.28470525379816,1.82096718347887,16.637353199391));
#182322=CARTESIAN_POINT('Ctrl Pts',(6.43407764099153,5.5494255252217,16.7960206646774));
#182323=CARTESIAN_POINT('Ctrl Pts',(2.98354656274481,7.95748638890239,16.9546881299639));
#182324=CARTESIAN_POINT('Ctrl Pts',(-1.17761734855467,8.40869439995495,
17.1133555952503));
#182325=CARTESIAN_POINT('Ctrl Pts',(-5.05474248930127,6.83174341500656,
17.2720230605367));
#182326=CARTESIAN_POINT('Ctrl Pts',(-7.7110126626523,3.56843978045104,17.4306905258231));
#182327=CARTESIAN_POINT('Ctrl Pts',(-8.46620823782832,-0.524957807205056,
17.5893579911096));
#182328=CARTESIAN_POINT('Ctrl Pts',(-6.78588403939986,-5.89677697852795,
17.8009146114915));
#182329=CARTESIAN_POINT('Ctrl Pts',(-1.46429379529528,-8.86105748603732,
18.0124712318734));
#182330=CARTESIAN_POINT('Ctrl Pts',(3.96634324971134,-7.49324051153254,
18.2240278522553));
#182331=CARTESIAN_POINT('Ctrl Pts',(8.15098066334341,-3.77147322880607,
18.4355844726372));
#182332=CARTESIAN_POINT('Ctrl Pts',(8.69188026264128,2.29595697489877,18.6471410930191));
#182333=CARTESIAN_POINT('Ctrl Pts',(5.19446800099358,6.70594995599219,18.858697713401));
#182334=CARTESIAN_POINT('Ctrl Pts',(1.38480816870057,8.38306537527828,19.0173651786874));
#182335=CARTESIAN_POINT('Ctrl Pts',(-2.80733701627989,8.02134643302842,
19.1760326439739));
#182336=CARTESIAN_POINT('Ctrl Pts',(-6.29141345945949,5.70184538667814,
19.3347001092603));
#182337=CARTESIAN_POINT('Ctrl Pts',(-8.25801451366162,2.00707150191196,
19.4933675745467));
#182338=CARTESIAN_POINT('Ctrl Pts',(-8.20682568737216,-2.20033881195099,
19.6520350398332));
#182339=CARTESIAN_POINT('Ctrl Pts',(-6.16414657957517,-5.8271399134678,
19.8107025051195));
#182340=CARTESIAN_POINT('Ctrl Pts',(-1.43239137515728,-8.87515948471095,
20.0222591255015));
#182341=CARTESIAN_POINT('Ctrl Pts',(4.5527339820946,-7.74177688764536,20.2338157458833));
#182342=CARTESIAN_POINT('Ctrl Pts',(7.84612963947235,-3.21228607362366,
20.4453723662653));
#182343=CARTESIAN_POINT('Ctrl Pts',(8.67471728024408,2.32632246209199,20.6569289866471));
#182344=CARTESIAN_POINT('Ctrl Pts',(5.20278957783041,7.33151972918976,20.8684856070291));
#182345=CARTESIAN_POINT('Ctrl Pts',(-0.307935242075415,8.47687669559407,
21.080042227411));
#182346=CARTESIAN_POINT('Ctrl Pts',(-4.30752757465816,7.32384359089192,
21.2387096926974));
#182347=CARTESIAN_POINT('Ctrl Pts',(-7.29457162247705,4.36031702588079,
21.3973771579839));
#182348=CARTESIAN_POINT('Ctrl Pts',(-8.48365271897988,0.347218483372963,
21.5560446232702));
#182349=CARTESIAN_POINT('Ctrl Pts',(-7.62649503422331,-3.74962841020285,
21.7147120885567));
#182350=CARTESIAN_POINT('Ctrl Pts',(-4.89161787082002,-6.94734145959187,
21.8733795538431));
#182351=CARTESIAN_POINT('Ctrl Pts',(-0.999627257628274,-8.42336084775099,
22.0320470191296));
#182352=CARTESIAN_POINT('Ctrl Pts',(4.58626387344269,-7.73216558370512,
22.2436036395115));
#182353=CARTESIAN_POINT('Ctrl Pts',(8.45559914028475,-3.02743113358754,
22.4551602598934));
#182354=CARTESIAN_POINT('Ctrl Pts',(8.08239236753771,2.56036437941381,22.6667168802753));
#182355=CARTESIAN_POINT('Ctrl Pts',(5.17015725645673,7.343838916623,22.8782735006572));
#182356=CARTESIAN_POINT('Ctrl Pts',(-0.702331405317825,8.96252930415199,
23.0898301210391));
#182357=CARTESIAN_POINT('Ctrl Pts',(-5.66734195152509,6.31137844136298,
23.301386741421));
#182358=CARTESIAN_POINT('Ctrl Pts',(-7.99956771205129,2.86363321160307,
23.4600542067074));
#182359=CARTESIAN_POINT('Ctrl Pts',(-8.39441071908186,-1.32552193531339,
23.6187216719939));
#182360=CARTESIAN_POINT('Ctrl Pts',(-6.73632038848893,-5.16864699462819,
23.7773891372803));
#182361=CARTESIAN_POINT('Ctrl Pts',(-3.45344407495777,-7.76510552038876,
23.9360566025667));
#182362=CARTESIAN_POINT('Ctrl Pts',(0.695120786446635,-8.46819259597579,
24.0947240678531));
#182363=CARTESIAN_POINT('Ctrl Pts',(4.62909106859212,-7.10800805460281,
24.2533915331396));
#182364=CARTESIAN_POINT('Ctrl Pts',(8.47518615693812,-2.99856974838409,
24.4649481535214));
#182365=CARTESIAN_POINT('Ctrl Pts',(8.43192000758649,3.09276915974365,24.6765047739034));
#182366=CARTESIAN_POINT('Ctrl Pts',(4.56541761580388,7.144053060519,24.8880613942853));
#182367=CARTESIAN_POINT('Ctrl Pts',(-0.735279526212941,8.95108150494292,
25.0996180146672));
#182368=CARTESIAN_POINT('Ctrl Pts',(-6.28130928209251,6.43159036579426,
25.311174635049));
#182369=CARTESIAN_POINT('Ctrl Pts',(-8.39499320342797,1.2150521552657,25.522731255431));
#182370=CARTESIAN_POINT('Ctrl Pts',(-7.97683182846663,-2.92636852270024,
25.6813987207174));
#182371=CARTESIAN_POINT('Ctrl Pts',(-5.59611972016833,-6.39582549786784,
25.8400661860039));
#182372=CARTESIAN_POINT('Ctrl Pts',(-1.86082884370897,-8.28433703719686,
25.9987336512902));
#182373=CARTESIAN_POINT('Ctrl Pts',(2.32328994584553,-8.17468430883825,
26.1574011165767));
#182374=CARTESIAN_POINT('Ctrl Pts',(5.95906474753433,-6.05665139206334,
26.3160685818631));
#182375=CARTESIAN_POINT('Ctrl Pts',(8.10818867535513,-2.49189466680684,
26.4747360471496));
#182376=CARTESIAN_POINT('Ctrl Pts',(8.42846848557864,3.1274782042865,26.6862926675315));
#182377=CARTESIAN_POINT('Ctrl Pts',(4.49269251246894,7.77677375768411,26.8978492879134));
#182378=CARTESIAN_POINT('Ctrl Pts',(-1.07160968069293,8.41024285204944,
27.1094059082953));
#182379=CARTESIAN_POINT('Ctrl Pts',(-6.29927301456852,6.40169161844959,
27.3209625286772));
#182380=CARTESIAN_POINT('Ctrl Pts',(-8.94342240549927,0.91400033232656,
27.5325191490591));
#182381=CARTESIAN_POINT('Ctrl Pts',(-7.22424387033608,-4.44551044622881,
27.744075769441));
#182382=CARTESIAN_POINT('Ctrl Pts',(-4.24987783380582,-7.35744637411753,
27.9027432347274));
#182383=CARTESIAN_POINT('Ctrl Pts',(-0.199146880524199,-8.49608617197416,
28.0614107000139));
#182384=CARTESIAN_POINT('Ctrl Pts',(3.87877969046034,-7.55301213055581,
28.2200781653003));
#182385=CARTESIAN_POINT('Ctrl Pts',(7.02115294620548,-4.78816781531549,
28.3787456305867));
#182386=CARTESIAN_POINT('Ctrl Pts',(8.45578532500763,-0.832570289930731,
28.5374130958732));
#182387=CARTESIAN_POINT('Ctrl Pts',(7.82206971680332,3.28138506900459,28.6960805611595));
#182388=CARTESIAN_POINT('Ctrl Pts',(4.46780524230699,7.80121254982153,28.9076371815415));
#182389=CARTESIAN_POINT('Ctrl Pts',(-1.53281601878551,8.84946163008538,
29.1191938019234));
#182390=CARTESIAN_POINT('Ctrl Pts',(-6.21101134428347,5.77095054730025,
29.3307504223052));
#182391=CARTESIAN_POINT('Ctrl Pts',(-8.93805989346455,0.879534780801609,
29.5423070426872));
#182392=CARTESIAN_POINT('Ctrl Pts',(-7.45245972615058,-5.02802595068711,
29.7538636630691));
#182393=CARTESIAN_POINT('Ctrl Pts',(-2.69875727328044,-8.04170204655293,
29.965420283451));
#182394=CARTESIAN_POINT('Ctrl Pts',(1.45060083585998,-8.37193143577347,
30.1240877487374));
#182395=CARTESIAN_POINT('Ctrl Pts',(5.29030421332727,-6.6510015074487,30.2827552140239));
#182396=CARTESIAN_POINT('Ctrl Pts',(7.81719117206012,-3.31427915404184,
30.4414226793103));
#182397=CARTESIAN_POINT('Ctrl Pts',(8.45858844060299,0.821840199874878,
30.6000901445967));
#182398=CARTESIAN_POINT('Ctrl Pts',(7.02587515260265,4.77813322232961,30.7587576098831));
#182399=CARTESIAN_POINT('Ctrl Pts',(3.90359985326166,7.53088114441021,30.9174250751696));
#182400=CARTESIAN_POINT('Ctrl Pts',(-1.5675820833069,8.85228147670276,31.1289816955514));
#182401=CARTESIAN_POINT('Ctrl Pts',(-6.84652756348825,5.81270646189832,
31.3405383159334));
#182402=CARTESIAN_POINT('Ctrl Pts',(-8.46619265519094,0.451789844279516,
31.5520949363152));
#182403=CARTESIAN_POINT('Ctrl Pts',(-7.42626117055549,-5.05105346601071,
31.7636515566973));
#182404=CARTESIAN_POINT('Ctrl Pts',(-2.50078270766321,-8.63517728710487,
31.9752081770791));
#182405=CARTESIAN_POINT('Ctrl Pts',(3.07995689382489,-7.9035516166973,32.186764797461));
#182406=CARTESIAN_POINT('Ctrl Pts',(6.47746095574527,-5.49872515380471,
32.3454322627474));
#182407=CARTESIAN_POINT('Ctrl Pts',(8.32308565417483,-1.71737733620265,
32.5040997280339));
#182408=CARTESIAN_POINT('Ctrl Pts',(8.12551720871498,2.46351257807376,32.6627671933203));
#182409=CARTESIAN_POINT('Ctrl Pts',(5.96809149645942,6.05020855934091,32.8214346586068));
#182410=CARTESIAN_POINT('Ctrl Pts',(2.33334461335539,8.17000499789411,32.9801021238931));
#182411=CARTESIAN_POINT('Ctrl Pts',(-1.82759285385863,8.28324616235341,
33.1387695891796));
#182412=CARTESIAN_POINT('Ctrl Pts',(-6.87502803213741,5.79259790491315,
33.3503262095615));
#182413=CARTESIAN_POINT('Ctrl Pts',(-8.98090275711608,0.0766926138812347,
33.5618828299434));
#182414=CARTESIAN_POINT('Ctrl Pts',(-6.78991034249501,-5.07716945542322,
33.7734394503253));
#182415=CARTESIAN_POINT('Ctrl Pts',(-2.46591398666662,-8.63607343068368,
33.9849960707071));
#182416=CARTESIAN_POINT('Ctrl Pts',(3.61218801699627,-8.23239325230199,
34.1965526910891));
#182417=CARTESIAN_POINT('Ctrl Pts',(7.42842502431126,-4.09521236125845,
34.408109311471));
#182418=CARTESIAN_POINT('Ctrl Pts',(8.49636895854652,-0.072064349971219,
34.5667767767574));
#182419=CARTESIAN_POINT('Ctrl Pts',(7.49085836935161,4.01374894729953,34.7254442420439));
#182420=CARTESIAN_POINT('Ctrl Pts',(4.66057979270806,7.09731781219159,34.8841117073303));
#182421=CARTESIAN_POINT('Ctrl Pts',(0.706179398388318,8.46902889231848,
35.0427791726167));
#182422=CARTESIAN_POINT('Ctrl Pts',(-3.44272605335546,7.76795443291458,
35.2014466379032));
#182423=CARTESIAN_POINT('Ctrl Pts',(-6.71010243784006,5.18910280292371,
35.3601141031895));
#182424=CARTESIAN_POINT('Ctrl Pts',(-8.98990280754567,0.0429935060367458,
35.5716707235715));
#182425=CARTESIAN_POINT('Ctrl Pts',(-6.94479731857069,-5.69493514394782,
35.7832273439534));
#182426=CARTESIAN_POINT('Ctrl Pts',(-1.96058313627431,-8.24843293625886,
35.9947839643353));
#182427=CARTESIAN_POINT('Ctrl Pts',(3.63953484236017,-8.21074188006452,
36.2063405847172));
#182428=CARTESIAN_POINT('Ctrl Pts',(8.04775942311691,-4.00671551252553,
36.4178972050991));
#182429=CARTESIAN_POINT('Ctrl Pts',(8.32733986051514,1.61482923960804,36.629453825481));
#182430=CARTESIAN_POINT('Ctrl Pts',(6.56980030452289,5.3880611270642,36.7881212907674));
#182431=CARTESIAN_POINT('Ctrl Pts',(3.18008548698482,7.88100222161509,36.9467887560539));
#182432=CARTESIAN_POINT('Ctrl Pts',(-0.968600827556462,8.43532670193088,
37.1054562213403));
#182433=CARTESIAN_POINT('Ctrl Pts',(-4.8836627066618,6.95506853231466,37.2641236866267));
#182434=CARTESIAN_POINT('Ctrl Pts',(-7.62009080867894,3.75868259071931,
37.4227911519132));
#182435=CARTESIAN_POINT('Ctrl Pts',(-8.47662769221309,-0.314715098500337,
37.5814586171996));
#182436=CARTESIAN_POINT('Ctrl Pts',(-6.9301175785037,-5.72657587732783,
37.7930152375815));
#182437=CARTESIAN_POINT('Ctrl Pts',(-1.68372179686536,-8.82199393564511,
38.0045718579634));
#182438=CARTESIAN_POINT('Ctrl Pts',(3.7791841692025,-7.58935433047188,38.2161284783453));
#182439=CARTESIAN_POINT('Ctrl Pts',(8.05488525025052,-3.97257091756658,
38.4276850987272));
#182440=CARTESIAN_POINT('Ctrl Pts',(8.74617592240978,2.07956910559353,38.6392417191091));
#182441=CARTESIAN_POINT('Ctrl Pts',(5.3592704363355,6.57498920271645,38.850798339491));
#182442=CARTESIAN_POINT('Ctrl Pts',(1.59239971653258,8.34612136822109,39.0094658047774));
#182443=CARTESIAN_POINT('Ctrl Pts',(-2.60743035661901,8.08853798019237,
39.1681332700639));
#182444=CARTESIAN_POINT('Ctrl Pts',(-6.14799025189356,5.85620525545962,
39.3268007353503));
#182445=CARTESIAN_POINT('Ctrl Pts',(-8.20566812724701,2.21136842410207,
39.4854682006367));
#182446=CARTESIAN_POINT('Ctrl Pts',(-8.25889802781082,-1.99601656218376,
39.6441356659231));
#182447=CARTESIAN_POINT('Ctrl Pts',(-6.30684358297493,-5.67238809017028,
39.8028031312096));
#182448=CARTESIAN_POINT('Ctrl Pts',(-1.65217912795724,-8.83688322089987,
40.0143597515915));
#182449=CARTESIAN_POINT('Ctrl Pts',(4.35922714377091,-7.85236491757794,
40.2259163719734));
#182450=CARTESIAN_POINT('Ctrl Pts',(7.76400380301161,-3.4059913512846,40.4374729923552));
#182451=CARTESIAN_POINT('Ctrl Pts',(8.72977171603534,2.11035112616518,40.6490296127373));
#182452=CARTESIAN_POINT('Ctrl Pts',(5.38311238161584,7.2001598605569,40.8605862331191));
#182453=CARTESIAN_POINT('Ctrl Pts',(-0.097494630340501,8.48190765233122,
41.072142853501));
#182454=CARTESIAN_POINT('Ctrl Pts',(-4.12446686458516,7.42847574090534,
41.2308103187874));
#182455=CARTESIAN_POINT('Ctrl Pts',(-7.18412830183364,4.53998240794474,
41.3894777840739));
#182456=CARTESIAN_POINT('Ctrl Pts',(-8.47242456027463,0.557625503242588,
41.5481452493602));
#182457=CARTESIAN_POINT('Ctrl Pts',(-7.71719024518532,-3.55922947297612,
41.7068127146468));
#182458=CARTESIAN_POINT('Ctrl Pts',(-5.06250346381941,-6.82382132159638,
41.8654801799331));
#182459=CARTESIAN_POINT('Ctrl Pts',(-1.208337303577,-8.39596233831067,42.0241476452196));
#182460=CARTESIAN_POINT('Ctrl Pts',(4.39298520629619,-7.84358858612854,
42.2357042656015));
#182461=CARTESIAN_POINT('Ctrl Pts',(8.37787264113882,-3.23631674862855,
42.4472608859834));
#182462=CARTESIAN_POINT('Ctrl Pts',(8.14343672196345,2.35901896868263,42.6588175063653));
#182463=CARTESIAN_POINT('Ctrl Pts',(5.35079579724299,7.2132849954259,42.8703741267472));
#182464=CARTESIAN_POINT('Ctrl Pts',(-0.479718335406196,8.97719729348602,
43.0819307471292));
#182465=CARTESIAN_POINT('Ctrl Pts',(-5.50898591167253,6.45006487238597,
43.293487367511));
#182466=CARTESIAN_POINT('Ctrl Pts',(-7.92604612433575,3.06125326752493,
43.4521548327974));
#182467=CARTESIAN_POINT('Ctrl Pts',(-8.4247175354972,-1.11681430749398,
43.6108222980838));
#182468=CARTESIAN_POINT('Ctrl Pts',(-6.86250131878953,-4.99989997390344,
43.7694897633703));
#182469=CARTESIAN_POINT('Ctrl Pts',(-3.64506456463047,-7.67702051869797,
43.9281572286567));
#182470=CARTESIAN_POINT('Ctrl Pts',(0.484776453906018,-8.48283388042666,
44.0868246939431));
#182471=CARTESIAN_POINT('Ctrl Pts',(4.45128707980494,-7.22068595266879,
44.2454921592296));
#182472=CARTESIAN_POINT('Ctrl Pts',(8.39816984408708,-3.20795030561121,
44.4570487796115));
#182473=CARTESIAN_POINT('Ctrl Pts',(8.50606777116889,2.88258665185232,44.6686053999934));
#182474=CARTESIAN_POINT('Ctrl Pts',(4.74128497666517,7.02856665815852,44.8801620203753));
#182475=CARTESIAN_POINT('Ctrl Pts',(-0.51294065087776,8.96657071718121,
45.0917186407571));
#182476=CARTESIAN_POINT('Ctrl Pts',(-6.11978069739963,6.58547456624455,
45.3032752611392));
#182477=CARTESIAN_POINT('Ctrl Pts',(-8.36225853595016,1.4229922505889,45.5148318815209));
#182478=CARTESIAN_POINT('Ctrl Pts',(-8.04698931459037,-2.72753043001754,
45.6734993468075));
#182479=CARTESIAN_POINT('Ctrl Pts',(-5.75310580212732,-6.25499239713214,
45.8321668120938));
#182480=CARTESIAN_POINT('Ctrl Pts',(-2.06581869166397,-8.23561375568526,
45.9908342773804));
#182481=CARTESIAN_POINT('Ctrl Pts',(2.11971744252928,-8.22981305731506,
46.1495017426667));
#182482=CARTESIAN_POINT('Ctrl Pts',(5.80695827124323,-6.20266331091412,
46.3081692079531));
#182483=CARTESIAN_POINT('Ctrl Pts',(8.04382478280886,-2.69230981459282,
46.4668366732396));
#182484=CARTESIAN_POINT('Ctrl Pts',(8.50355374697948,2.9173373785056,46.6783932936214));
#182485=CARTESIAN_POINT('Ctrl Pts',(4.68413887105522,7.66296078718693,46.8899499140035));
#182486=CARTESIAN_POINT('Ctrl Pts',(-0.862418275557941,8.43416932904131,
47.1015065343852));
#182487=CARTESIAN_POINT('Ctrl Pts',(-6.13889939658387,6.55621610061593,
47.3130631547673));
#182488=CARTESIAN_POINT('Ctrl Pts',(-8.91715105499881,1.13527081630686,
47.524619775149));
#182489=CARTESIAN_POINT('Ctrl Pts',(-7.33336423065867,-4.26442109322725,
47.7361763955311));
#182490=CARTESIAN_POINT('Ctrl Pts',(-4.42895873448593,-7.25068884785307,
47.8948438608174));
#182491=CARTESIAN_POINT('Ctrl Pts',(-0.414139927621501,-8.48665355620754,
48.0535113261039));
#182492=CARTESIAN_POINT('Ctrl Pts',(3.69814652203495,-7.65047939402318,
48.2121787913904));
#182493=CARTESIAN_POINT('Ctrl Pts',(6.88569527407017,-4.95441811708111,
48.3708462566766));
#182494=CARTESIAN_POINT('Ctrl Pts',(8.97817226161953,0.247819711134177,
48.5824028770587));
#182495=CARTESIAN_POINT('Ctrl Pts',(6.20633671998026,7.37075419636882,48.8468486525359));
#182496=CARTESIAN_POINT('Ctrl Pts',(-2.85224887117413,9.20622344841131,
49.1641835831089));
#182497=CARTESIAN_POINT('Ctrl Pts',(-8.17586019302007,3.71558748174298,
49.4286293585863));
#182498=CARTESIAN_POINT('Ctrl Pts',(-8.26990206276113,-1.88382351173266,
49.6401859789681));
#182499=CARTESIAN_POINT('Ctrl Pts',(-6.38190782755159,-5.61929274005956,
49.7988534442546));
#182500=CARTESIAN_POINT('Ctrl Pts',(-2.91689738088643,-7.96447915796828,
49.957520909541));
#182501=CARTESIAN_POINT('Ctrl Pts',(2.65202034096889,-8.58081155893773,
50.1690775299229));
#182502=CARTESIAN_POINT('Ctrl Pts',(8.76699052457919,-3.99508362442263,
50.4335233054003));
#182503=CARTESIAN_POINT('Ctrl Pts',(8.10419147421929,5.22260796336014,50.7508582359731));
#182504=CARTESIAN_POINT('Ctrl Pts',(1.37159143871236,8.874804986452,51.0153040114506));
#182505=CARTESIAN_POINT('Ctrl Pts',(-4.02714773549846,7.45728686713406,
51.2268606318324));
#182506=CARTESIAN_POINT('Ctrl Pts',(-8.18910127503122,3.69908206285886,
51.4384172522143));
#182507=CARTESIAN_POINT('Ctrl Pts',(-8.66855129374023,-2.37337160374202,
51.6499738725964));
#182508=CARTESIAN_POINT('Ctrl Pts',(-5.13571306658545,-6.75184376042308,
51.8615304929781));
#182509=CARTESIAN_POINT('Ctrl Pts',(-1.3095180133245,-8.39509522717736,
52.0201979582646));
#182510=CARTESIAN_POINT('Ctrl Pts',(2.87827190579938,-7.99602505259151,
52.178865423551));
#182511=CARTESIAN_POINT('Ctrl Pts',(6.34208622339921,-5.64564105789136,
52.3375328888374));
#182512=CARTESIAN_POINT('Ctrl Pts',(8.27545483497107,-1.93349562876361,
52.4962003541239));
#182513=CARTESIAN_POINT('Ctrl Pts',(8.18696759196887,2.27328395429753,52.6548678194103));
#182514=CARTESIAN_POINT('Ctrl Pts',(6.11202192701451,5.88176726535637,52.8135352846966));
#182515=CARTESIAN_POINT('Ctrl Pts',(1.35337035089401,8.88755422499004,53.0250919050788));
#182516=CARTESIAN_POINT('Ctrl Pts',(-4.62145954539154,7.7009546273047,53.2366485254604));
#182517=CARTESIAN_POINT('Ctrl Pts',(-7.87440234716974,3.14233340779931,
53.4482051458425));
#182518=CARTESIAN_POINT('Ctrl Pts',(-8.6536742615346,-2.40342925122091,
53.6597617662243));
#182519=CARTESIAN_POINT('Ctrl Pts',(-5.13733632629595,-7.37753080297155,
53.8713183866063));
#182520=CARTESIAN_POINT('Ctrl Pts',(0.383360766010533,-8.4738005541894,
54.0828750069881));
#182521=CARTESIAN_POINT('Ctrl Pts',(4.37253465287558,-7.28521951823731,
54.2415424722746));
#182522=CARTESIAN_POINT('Ctrl Pts',(7.33308640359521,-4.29522760314234,
54.400209937561));
#182523=CARTESIAN_POINT('Ctrl Pts',(8.48640689467772,-0.271705983052308,
54.5588774028474));
#182524=CARTESIAN_POINT('Ctrl Pts',(7.59282381463648,3.81735056487313,54.7175448681339));
#182525=CARTESIAN_POINT('Ctrl Pts',(4.82959756664542,6.99059842741678,54.8762123334202));
#182526=CARTESIAN_POINT('Ctrl Pts',(0.924625456828362,8.43192329054703,
55.0348797987068));
#182527=CARTESIAN_POINT('Ctrl Pts',(-4.65489327796069,7.69104475199265,
55.2464364190885));
#182528=CARTESIAN_POINT('Ctrl Pts',(-8.48220639133452,2.95206214867202,
55.4579930394708));
#182529=CARTESIAN_POINT('Ctrl Pts',(-8.0592867972206,-2.63219080227642,
55.6695496598523));
#182530=CARTESIAN_POINT('Ctrl Pts',(-5.10459733409883,-7.38955899671512,
55.8811062802345));
#182531=CARTESIAN_POINT('Ctrl Pts',(0.782064028799498,-8.95592411694139,
56.0926629006161));
#182532=CARTESIAN_POINT('Ctrl Pts',(5.72328451496193,-6.26069301120408,
56.3042195209983));
#182533=CARTESIAN_POINT('Ctrl Pts',(8.0247353255809,-2.79232908323465,56.4628869862845));
#182534=CARTESIAN_POINT('Ctrl Pts',(8.38228205579894,1.40017400928179,56.6215544515712));
#182535=CARTESIAN_POINT('Ctrl Pts',(6.69005617785998,5.22839100197216,56.7802219168573));
#182536=CARTESIAN_POINT('Ctrl Pts',(3.38420314471914,7.79553133510935,56.9388893821439));
#182537=CARTESIAN_POINT('Ctrl Pts',(-0.770454432796781,8.46167115392818,
57.0975568474303));
#182538=CARTESIAN_POINT('Ctrl Pts',(-4.69216421046836,7.06653080710174,
57.2562243127168));
#182539=CARTESIAN_POINT('Ctrl Pts',(-8.50153577951395,2.92302759483824,
57.4677809330986));
#182540=CARTESIAN_POINT('Ctrl Pts',(-8.40406255692474,-3.16768505839187,
57.6793375534805));
#182541=CARTESIAN_POINT('Ctrl Pts',(-4.50165959757123,-7.18439927939594,
57.8908941738625));
#182542=CARTESIAN_POINT('Ctrl Pts',(0.814908966215111,-8.94418355505842,
58.1024507942443));
#182543=CARTESIAN_POINT('Ctrl Pts',(6.33829733768668,-6.37543628230751,
58.3140074146263));
#182544=CARTESIAN_POINT('Ctrl Pts',(8.40547390421308,-1.14029429149029,
58.5255640350081));
#182545=CARTESIAN_POINT('Ctrl Pts',(7.95047325203561,2.99724103451126,58.6842315002946));
#182546=CARTESIAN_POINT('Ctrl Pts',(5.53897960442787,6.44537389632009,58.8428989655811));
#182547=CARTESIAN_POINT('Ctrl Pts',(1.78703017219667,8.30056909465304,59.0015664308674));
#182548=CARTESIAN_POINT('Ctrl Pts',(-2.39594709235619,8.15368488796713,
59.1602338961539));
#182549=CARTESIAN_POINT('Ctrl Pts',(-6.01272886125954,6.00337991395397,
59.3189013614403));
#182550=CARTESIAN_POINT('Ctrl Pts',(-8.13004376622867,2.41963860624355,
59.4775688267267));
#182551=CARTESIAN_POINT('Ctrl Pts',(-8.40030228462738,-3.20236201225959,
59.6891254471087));
#182552=CARTESIAN_POINT('Ctrl Pts',(-4.42330658889043,-7.81644771686461,
59.9006820674905));
#182553=CARTESIAN_POINT('Ctrl Pts',(1.14641270476439,-8.40037320888529,
60.1122386878725));
#182554=CARTESIAN_POINT('Ctrl Pts',(6.35599428022148,-6.34537885390543,
60.3237953082543));
#182555=CARTESIAN_POINT('Ctrl Pts',(8.95120223150307,-0.834373742044771,
60.5353519286364));
#182556=CARTESIAN_POINT('Ctrl Pts',(7.1843957630033,4.50962527779835,60.7469085490181));
#182557=CARTESIAN_POINT('Ctrl Pts',(4.18423325505326,7.39497605253704,60.9055760143047));
#182558=CARTESIAN_POINT('Ctrl Pts',(0.123529587461397,8.49752200130453,
61.0642434795908));
#182559=CARTESIAN_POINT('Ctrl Pts',(-3.9458427790497,7.5181945235856,61.2229109448775));
#182560=CARTESIAN_POINT('Ctrl Pts',(-7.06348635765548,4.72549470392764,
61.3815784101638));
#182561=CARTESIAN_POINT('Ctrl Pts',(-8.46285978914737,0.757286563674393,
61.5402458754504));
#182562=CARTESIAN_POINT('Ctrl Pts',(-7.79255786233917,-3.35086624437824,
61.6989133407367));
#182563=CARTESIAN_POINT('Ctrl Pts',(-4.39820281557677,-7.84066406140013,
61.9104699611186));
#182564=CARTESIAN_POINT('Ctrl Pts',(1.61150952855133,-8.8354701702392,62.1220265815006));
#182565=CARTESIAN_POINT('Ctrl Pts',(6.26212293716273,-5.71544822897241,
62.3335832018824));
#182566=CARTESIAN_POINT('Ctrl Pts',(8.94553321178029,-0.799957278068402,
62.5451398222644));
#182567=CARTESIAN_POINT('Ctrl Pts',(7.40741858846125,5.09414868118294,62.7566964426463));
#182568=CARTESIAN_POINT('Ctrl Pts',(2.62708470693044,8.06540070723271,62.9682530630282));
#182569=CARTESIAN_POINT('Ctrl Pts',(-1.52504790634506,8.35869054539299,
63.1269205283146));
#182570=CARTESIAN_POINT('Ctrl Pts',(-5.34928412288214,6.6036580085824,63.285587993601));
#182571=CARTESIAN_POINT('Ctrl Pts',(-7.84637645075201,3.24458020775182,
63.4442554588875));
#182572=CARTESIAN_POINT('Ctrl Pts',(-8.45093966201039,-0.897083357716978,
63.6029229241739));
#182573=CARTESIAN_POINT('Ctrl Pts',(-6.98307478342027,-4.84046953501923,
63.7615903894603));
#182574=CARTESIAN_POINT('Ctrl Pts',(-3.83642553515746,-7.565322315593,63.9202578547468));
#182575=CARTESIAN_POINT('Ctrl Pts',(1.64629931106835,-8.83798051078726,
64.1318144751286));
#182576=CARTESIAN_POINT('Ctrl Pts',(6.89798558941472,-5.75154682655248,
64.3433710955106));
#182577=CARTESIAN_POINT('Ctrl Pts',(8.46987801939189,-0.376428578651072,
64.5549277158925));
#182578=CARTESIAN_POINT('Ctrl Pts',(7.38101614104786,5.11694213523958,64.7664843362744));
#182579=CARTESIAN_POINT('Ctrl Pts',(2.42383645377006,8.65709060689877,64.9780409566562));
#182580=CARTESIAN_POINT('Ctrl Pts',(-3.15017117937135,7.87582910976843,
65.1895975770382));
#182581=CARTESIAN_POINT('Ctrl Pts',(-6.52613937584308,5.44086239463559,
65.3482650423246));
#182582=CARTESIAN_POINT('Ctrl Pts',(-8.33803955603354,1.64323950891316,
65.506932507611));
#182583=CARTESIAN_POINT('Ctrl Pts',(-8.10327184848769,-2.53572661794554,
65.6655999728974));
#182584=CARTESIAN_POINT('Ctrl Pts',(-5.91401240716692,-6.10308094076339,
65.824267438184));
#182585=CARTESIAN_POINT('Ctrl Pts',(-2.26054470797334,-8.19044665287207,
65.9829349034703));
#182586=CARTESIAN_POINT('Ctrl Pts',(1.90123575674584,-8.26665381051419,
66.1416023687568));
#182587=CARTESIAN_POINT('Ctrl Pts',(6.92630597692818,-5.73118543101237,
66.3531589891386));
#182588=CARTESIAN_POINT('Ctrl Pts',(8.98122962787707,0.00323436894311558,
66.5647156095205));
#182589=CARTESIAN_POINT('Ctrl Pts',(6.74445809772123,5.13739399951818,66.7762722299025));
#182590=CARTESIAN_POINT('Ctrl Pts',(2.38896113849587,8.65767640701331,66.9878288502843));
#182591=CARTESIAN_POINT('Ctrl Pts',(-3.68530769393738,8.19992122716341,
67.1993854706664));
#182592=CARTESIAN_POINT('Ctrl Pts',(-7.46457547414581,4.02894224535407,
67.4109420910481));
#182593=CARTESIAN_POINT('Ctrl Pts',(-8.496673828314,-0.00355042726389536,
67.5696095563346));
#182594=CARTESIAN_POINT('Ctrl Pts',(-7.45484208877315,-4.0802535648032,
67.728277021621));
#182595=CARTESIAN_POINT('Ctrl Pts',(-4.59723391810387,-7.13851276063061,
67.8869444869076));
#182596=CARTESIAN_POINT('Ctrl Pts',(-0.630782818409487,-8.4749780387699,
68.0456119521938));
#182597=CARTESIAN_POINT('Ctrl Pts',(3.5117192503279,-7.73700889602476,68.2042794174804));
#182598=CARTESIAN_POINT('Ctrl Pts',(6.75601621638297,-5.12918195325416,
68.3629468827666));
#182599=CARTESIAN_POINT('Ctrl Pts',(8.98992942269384,0.0370122366584145,
68.5745035031487));
#182600=CARTESIAN_POINT('Ctrl Pts',(6.89384124450594,5.75651361375506,68.7860601235305));
#182601=CARTESIAN_POINT('Ctrl Pts',(1.8871000366735,8.26555416108259,68.9976167439125));
#182602=CARTESIAN_POINT('Ctrl Pts',(-3.7124607538397,8.1780273441093,69.2091733642944));
#182603=CARTESIAN_POINT('Ctrl Pts',(-8.08309778550766,3.93493724481097,
69.4207299846762));
#182604=CARTESIAN_POINT('Ctrl Pts',(-8.3126392144974,-1.68887297190101,
69.6322866050581));
#182605=CARTESIAN_POINT('Ctrl Pts',(-6.52159005094721,-5.4463145298152,
69.7909540703446));
#182606=CARTESIAN_POINT('Ctrl Pts',(-3.10982397965096,-7.90899074074696,
69.949621535631));
#182607=CARTESIAN_POINT('Ctrl Pts',(1.04363116001082,-8.42637277440925,
70.1082890009175));
#182608=CARTESIAN_POINT('Ctrl Pts',(4.94536470949391,-6.91133182619133,
70.2669564662039));
#182609=CARTESIAN_POINT('Ctrl Pts',(7.65323878179321,-3.69072010577144,
70.4256239314902));
#182610=CARTESIAN_POINT('Ctrl Pts',(8.47349126886064,0.390138875479095,
70.5842913967768));
#182611=CARTESIAN_POINT('Ctrl Pts',(6.87888050467731,5.78802245443554,70.7958480171586));
#182612=CARTESIAN_POINT('Ctrl Pts',(1.60514535686331,8.83662856937753,71.0074046375406));
#182613=CARTESIAN_POINT('Ctrl Pts',(-3.84657462269014,7.55542161697674,
71.2189612579225));
#182614=CARTESIAN_POINT('Ctrl Pts',(-8.08991946671398,3.90073058693897,
71.4305178783043));
#182615=CARTESIAN_POINT('Ctrl Pts',(-8.72732282085781,-2.15732179129917,
71.6420744986863));
#182616=CARTESIAN_POINT('Ctrl Pts',(-5.30054526426088,-6.62242270827973,
71.8536311190682));
#182617=CARTESIAN_POINT('Ctrl Pts',(-1.51806183608798,-8.35996214178644,
72.0122985843546));
#182618=CARTESIAN_POINT('Ctrl Pts',(2.67930960731952,-8.06501331367521,
72.1709660496411));
#182619=CARTESIAN_POINT('Ctrl Pts',(6.19986304949528,-5.80126040606293,
72.3296335149275));
#182620=CARTESIAN_POINT('Ctrl Pts',(8.22502286458498,-2.13825597127375,
72.4883009802139));
#182621=CARTESIAN_POINT('Ctrl Pts',(8.24080778333267,2.06943611364381,72.6469684455002));
#182622=CARTESIAN_POINT('Ctrl Pts',(6.25611342521144,5.72829009709764,72.8056359107867));
#182623=CARTESIAN_POINT('Ctrl Pts',(1.57347143249256,8.85123655665177,73.0171925311688));
#182624=CARTESIAN_POINT('Ctrl Pts',(-4.42893524361537,7.81325979970337,
73.2287491515504));
#182625=CARTESIAN_POINT('Ctrl Pts',(-7.79400736428803,3.3367621047398,73.4403057719326));
#182626=CARTESIAN_POINT('Ctrl Pts',(-8.71064532497189,-2.18795660659524,
73.6518623923142));
#182627=CARTESIAN_POINT('Ctrl Pts',(-5.31882267039395,-7.2477807866672,
73.8634190126964));
#182628=CARTESIAN_POINT('Ctrl Pts',(0.172973997260735,-8.48070413479266,
74.0749756330781));
#182629=CARTESIAN_POINT('Ctrl Pts',(4.19041193458728,-7.39147661626266,
74.2336430983647));
#182630=CARTESIAN_POINT('Ctrl Pts',(7.2242465776339,-4.47586875446305,74.392310563651));
#182631=CARTESIAN_POINT('Ctrl Pts',(8.47705154330805,-0.482204586819274,
74.5509780289375));
#182632=CARTESIAN_POINT('Ctrl Pts',(7.68520991709078,3.62776628958957,74.7096454942239));
#182633=CARTESIAN_POINT('Ctrl Pts',(5.00157560649177,6.86860394860821,74.8683129595104));
#182634=CARTESIAN_POINT('Ctrl Pts',(1.13357108105033,8.40638324309714,75.0269804247967));
#182635=CARTESIAN_POINT('Ctrl Pts',(-4.4626138658977,7.80418339191081,75.2385370451786));
#182636=CARTESIAN_POINT('Ctrl Pts',(-8.40634190449351,3.16163120470357,
75.4500936655605));
#182637=CARTESIAN_POINT('Ctrl Pts',(-8.1221205743362,-2.43139661802582,
75.6616502859425));
#182638=CARTESIAN_POINT('Ctrl Pts',(-5.286390561127,-7.26061780601531,75.8732069063243));
#182639=CARTESIAN_POINT('Ctrl Pts',(0.559590308740241,-8.97257263091493,
76.0847635267063));
#182640=CARTESIAN_POINT('Ctrl Pts',(5.56616896121972,-6.40078321151184,
76.2963201470882));
#182641=CARTESIAN_POINT('Ctrl Pts',(7.95297533448445,-2.99059560612457,
76.4549876123746));
#182642=CARTESIAN_POINT('Ctrl Pts',(8.41444502679094,1.19174435712809,76.6136550776611));
#182643=CARTESIAN_POINT('Ctrl Pts',(6.81773384888835,5.06077358683163,76.7723225429474));
#182644=CARTESIAN_POINT('Ctrl Pts',(3.57659993657919,7.70915511682669,76.9309900082339));
#182645=CARTESIAN_POINT('Ctrl Pts',(-0.560248715186514,8.47818377528005,
77.0896574735203));
#182646=CARTESIAN_POINT('Ctrl Pts',(-4.51537004133694,7.18078658751354,
77.2483249388068));
#182647=CARTESIAN_POINT('Ctrl Pts',(-8.42638581228697,3.13308523234964,
77.4598815591886));
#182648=CARTESIAN_POINT('Ctrl Pts',(-8.48007796028266,-2.95817069780082,
77.6714381795706));
#182649=CARTESIAN_POINT('Ctrl Pts',(-4.67854763394638,-7.07048259845802,
77.8829947999524));
#182650=CARTESIAN_POINT('Ctrl Pts',(0.592716464848895,-8.9616507007412,
78.0945514203345));
#182651=CARTESIAN_POINT('Ctrl Pts',(6.1781451636225,-6.53075212114861,78.3061080407161));
#182652=CARTESIAN_POINT('Ctrl Pts',(8.37459038114081,-1.34851717590935,
78.5176646610983));
#182653=CARTESIAN_POINT('Ctrl Pts',(8.02239891340539,2.79903455221292,78.6763321263845));
#182654=CARTESIAN_POINT('Ctrl Pts',(5.69721000697799,6.30594464438302,78.834999591671));
#182655=CARTESIAN_POINT('Ctrl Pts',(1.99245080097765,8.25366972546961,78.9936670569575));
#182656=CARTESIAN_POINT('Ctrl Pts',(-2.1928832509956,8.21062742846951,79.1523345222438));
#182657=CARTESIAN_POINT('Ctrl Pts',(-5.8619091670315,6.15073163678617,79.3110019875304));
#182658=CARTESIAN_POINT('Ctrl Pts',(-8.06749931598736,2.62063301745226,
79.4696694528166));
#182659=CARTESIAN_POINT('Ctrl Pts',(-8.47717932212457,-2.99293028171761,
79.6812260731989));
#182660=CARTESIAN_POINT('Ctrl Pts',(-4.6159024442474,-7.70428067472816,
79.8927826935804));
#182661=CARTESIAN_POINT('Ctrl Pts',(0.9376122747872,-8.42623375894427,80.1043393139626));
#182662=CARTESIAN_POINT('Ctrl Pts',(6.1965825040472,-6.50114308105391,80.3158959343442));
#182663=CARTESIAN_POINT('Ctrl Pts',(8.92774180300392,-1.05623256415178,
80.5274525547263));
#182664=CARTESIAN_POINT('Ctrl Pts',(7.29408571740519,4.32996260639319,80.7390091751082));
#182665=CARTESIAN_POINT('Ctrl Pts',(4.36644429853462,7.28887117035859,80.8976766403946));
#182666=CARTESIAN_POINT('Ctrl Pts',(0.334349638121285,8.49184020346127,
81.0563441056809));
#182667=CARTESIAN_POINT('Ctrl Pts',(-3.75807080042374,7.61379195870581,
81.2150115709676));
#182668=CARTESIAN_POINT('Ctrl Pts',(-6.94405264827288,4.89931347636055,
81.3736790362538));
#182669=CARTESIAN_POINT('Ctrl Pts',(-8.44146257576306,0.967051359691387,
81.5323465015405));
#182670=CARTESIAN_POINT('Ctrl Pts',(-7.87330702839439,-3.15646939827605,
81.6910139668267));
#182671=CARTESIAN_POINT('Ctrl Pts',(-4.59140730681298,-7.72911248938867,
81.9025705872088));
#182672=CARTESIAN_POINT('Ctrl Pts',(1.39176936212274,-8.87273769095279,
82.1141272075905));
#182673=CARTESIAN_POINT('Ctrl Pts',(6.11837120677715,-5.86907709220823,
82.3256838279725));
#182674=CARTESIAN_POINT('Ctrl Pts',(8.92292854133732,-1.02168602612884,
82.5372404483544));
#182675=CARTESIAN_POINT('Ctrl Pts',(7.5315442738682,4.90877192192126,82.7487970687363));
#182676=CARTESIAN_POINT('Ctrl Pts',(2.82641118483351,7.99772858003235,82.9603536891183));
#182677=CARTESIAN_POINT('Ctrl Pts',(-1.31716520482439,8.39395940980711,
83.1190211544045));
#182678=CARTESIAN_POINT('Ctrl Pts',(-5.18377337279622,6.73436213320326,
83.2776886196911));
#182679=CARTESIAN_POINT('Ctrl Pts',(-7.76344918945897,3.43828166591109,
83.4363560849775));
#182680=CARTESIAN_POINT('Ctrl Pts',(-8.47059776649664,-0.687104940933551,
83.595023550264));
#182681=CARTESIAN_POINT('Ctrl Pts',(-7.10103631969523,-4.66570058369135,
83.7536910155502));
#182682=CARTESIAN_POINT('Ctrl Pts',(-4.02297065806388,-7.46779550536667,
83.9123584808369));
#182683=CARTESIAN_POINT('Ctrl Pts',(1.42648614053484,-8.87611053454955,
84.1239151012184));
#182684=CARTESIAN_POINT('Ctrl Pts',(6.75314231344867,-5.92094291343086,
84.3354717216008));
#182685=CARTESIAN_POINT('Ctrl Pts',(8.45792928085866,-0.586484797924657,
84.5470283419822));
#182686=CARTESIAN_POINT('Ctrl Pts',(7.50571555451649,4.93221350962116,84.7585849623646));
#182687=CARTESIAN_POINT('Ctrl Pts',(2.63790774845381,8.59427970462494,84.9701415827459));
#182688=CARTESIAN_POINT('Ctrl Pts',(-2.95376983218562,7.95157257428289,
85.1816982031284));
#182689=CARTESIAN_POINT('Ctrl Pts',(-6.38911994199167,5.60112712917077,
85.3403656684144));
#182690=CARTESIAN_POINT('Ctrl Pts',(-8.29469668035499,1.84963420776674,
85.4990331337012));
#182691=CARTESIAN_POINT('Ctrl Pts',(-8.16369841062226,-2.3338706887604,
85.6577005989873));
#182692=CARTESIAN_POINT('Ctrl Pts',(-6.06363365034946,-5.95445099702591,
85.816368064274));
#182693=CARTESIAN_POINT('Ctrl Pts',(-2.46308694812765,-8.13183137037725,
85.9750355295601));
#182694=CARTESIAN_POINT('Ctrl Pts',(1.69552102660424,-8.31128576538918,
86.1337029948468));
#182695=CARTESIAN_POINT('Ctrl Pts',(6.78195922970113,-5.90129053151531,
86.3452596152285));
#182696=CARTESIAN_POINT('Ctrl Pts',(8.97854441794314,-0.219627468278469,
86.5568162356106));
#182697=CARTESIAN_POINT('Ctrl Pts',(6.86986101179065,4.96845467090943,86.7683728559925));
#182698=CARTESIAN_POINT('Ctrl Pts',(2.6030577079444,8.59573072280125,86.9799294763743));
#182699=CARTESIAN_POINT('Ctrl Pts',(-3.48069952566048,8.28884381218191,
87.1914860967563));
#182700=CARTESIAN_POINT('Ctrl Pts',(-7.36230256281513,4.21292815025172,
87.4030427171382));
#182701=CARTESIAN_POINT('Ctrl Pts',(-8.494145663744,0.207287706792954,87.5617101824246));
#182702=CARTESIAN_POINT('Ctrl Pts',(-7.55379430950297,-3.89401223050901,
87.720377647711));
#182703=CARTESIAN_POINT('Ctrl Pts',(-4.77295389438821,-7.0222386212301,
87.8790451129976));
#182704=CARTESIAN_POINT('Ctrl Pts',(-0.840887270071041,-8.45671616649546,
88.0377125782838));
#182705=CARTESIAN_POINT('Ctrl Pts',(3.31865127076786,-7.82176658391953,
88.1963800435704));
#182706=CARTESIAN_POINT('Ctrl Pts',(6.62666005930314,-5.29524683882204,
88.3550475088568));
#182707=CARTESIAN_POINT('Ctrl Pts',(8.9880797002516,-0.186075878621066,
88.5666041292387));
#182708=CARTESIAN_POINT('Ctrl Pts',(7.03456103716749,5.5836768445321,88.7781607496206));
#182709=CARTESIAN_POINT('Ctrl Pts',(2.09162098936609,8.21618243316483,88.9897173700025));
#182710=CARTESIAN_POINT('Ctrl Pts',(-3.50838750099007,8.26763044848369,
89.2012739903845));
#182711=CARTESIAN_POINT('Ctrl Pts',(-7.9829670674822,4.13430014998594,89.4128306107662));
#182712=CARTESIAN_POINT('Ctrl Pts',(-8.35198742516224,-1.48208254680695,
89.6243872311483));
#182713=CARTESIAN_POINT('Ctrl Pts',(-6.65472716473773,-5.28281034234522,
89.7830546964346));
#182714=CARTESIAN_POINT('Ctrl Pts',(-3.30512064670134,-7.82938804967445,
89.9417221617211));
#182715=CARTESIAN_POINT('Ctrl Pts',(0.834217223173009,-8.44967489055097,
90.1003896270074));
#182716=CARTESIAN_POINT('Ctrl Pts',(4.77234369383054,-7.03191832927506,
90.259057092294));
#182717=CARTESIAN_POINT('Ctrl Pts',(7.55930044505665,-3.87949165892316,
90.4177245575803));
#182718=CARTESIAN_POINT('Ctrl Pts',(8.48056307456161,0.179756958105245,
90.5763920228666));
#182719=CARTESIAN_POINT('Ctrl Pts',(7.02038676650769,5.61554721994126,90.7879486432487));
#182720=CARTESIAN_POINT('Ctrl Pts',(1.82392380713085,8.79407744083663,90.9995052636305));
#182721=CARTESIAN_POINT('Ctrl Pts',(-3.65790945473178,7.6485443425074,91.2110618840126));
#182722=CARTESIAN_POINT('Ctrl Pts',(-7.99063545451894,4.10027329854195,
91.4226185043941));
#182723=CARTESIAN_POINT('Ctrl Pts',(-8.77816746441304,-1.9400971359493,
91.6341751247764));
#182724=CARTESIAN_POINT('Ctrl Pts',(-5.46324238590482,-6.48885546606135,
91.8457317451582));
#182725=CARTESIAN_POINT('Ctrl Pts',(-1.72503906768333,-8.31971868293201,
92.0043992104447));
#182726=CARTESIAN_POINT('Ctrl Pts',(2.47835881636955,-8.12901453450982,
92.163066675731));
#182727=CARTESIAN_POINT('Ctrl Pts',(6.05400114093271,-5.95331792480741,
92.3217341410176));
#182728=CARTESIAN_POINT('Ctrl Pts',(8.16943141620118,-2.34169384342607,
92.4804016063039));
#182729=CARTESIAN_POINT('Ctrl Pts',(8.28962143227979,1.86431093847469,92.6390690715904));
#182730=CARTESIAN_POINT('Ctrl Pts',(6.39632924340885,5.57128663696691,92.7977365368768));
#182731=CARTESIAN_POINT('Ctrl Pts',(1.79262212165266,8.80946689523861,93.0092931572587));
#182732=CARTESIAN_POINT('Ctrl Pts',(-4.23369274768137,7.92075385661886,
93.2208497776406));
#182733=CARTESIAN_POINT('Ctrl Pts',(-7.7088088150833,3.52913570259757,93.4324063980225));
#182734=CARTESIAN_POINT('Ctrl Pts',(-8.76225529146867,-1.97113638965059,
93.6439630184044));
#182735=CARTESIAN_POINT('Ctrl Pts',(-5.49703181531362,-7.11356737986656,
93.8555196387864));
#182736=CARTESIAN_POINT('Ctrl Pts',(-0.0375200648321471,-8.48238506158333,
94.0670762591681));
#182737=CARTESIAN_POINT('Ctrl Pts',(4.00570910503058,-7.49318164401645,
94.2257437244544));
#182738=CARTESIAN_POINT('Ctrl Pts',(7.11095746815531,-4.65375385910643,
94.3844111897412));
#182739=CARTESIAN_POINT('Ctrl Pts',(8.46247611910779,-0.692405567907114,
94.5430786550272));
#182740=CARTESIAN_POINT('Ctrl Pts',(7.77286267026383,3.43594665169769,94.7017461203141));
#182741=CARTESIAN_POINT('Ctrl Pts',(5.17047444629095,6.74238192468996,94.8604135856003));
#182742=CARTESIAN_POINT('Ctrl Pts',(1.34181698677152,8.37566203695453,95.0190810508868));
#182743=CARTESIAN_POINT('Ctrl Pts',(-4.26758257056428,7.91252552958314,
95.2306376712688));
#182744=CARTESIAN_POINT('Ctrl Pts',(-8.32530750260123,3.36923491002623,
95.4421942916505));
#182745=CARTESIAN_POINT('Ctrl Pts',(-8.17994426503522,-2.22908354155261,
95.6537509120326));
#182746=CARTESIAN_POINT('Ctrl Pts',(-5.46494856849098,-7.12725858462383,
95.8653075324143));
#182747=CARTESIAN_POINT('Ctrl Pts',(0.336812665012069,-8.98358877145597,
96.0768641527964));
#182748=CARTESIAN_POINT('Ctrl Pts',(5.40557535339018,-6.5370633888607,96.2884207731781));
#182749=CARTESIAN_POINT('Ctrl Pts',(7.87642355379138,-3.1867425062301,96.4470882384646));
#182750=CARTESIAN_POINT('Ctrl Pts',(8.44121995650644,0.982039858335275,
96.605755703751));
#182751=CARTESIAN_POINT('Ctrl Pts',(6.94160524393157,4.89106892765923,96.7644231690373));
#182752=CARTESIAN_POINT('Ctrl Pts',(3.76605381086406,7.61608932442504,96.9230906343239));
#182753=CARTESIAN_POINT('Ctrl Pts',(-0.348317063116852,8.49309378863622,
97.0817580996103));
#182754=CARTESIAN_POINT('Ctrl Pts',(-4.33825713380984,7.2842007417435,97.2404255648969));
#182755=CARTESIAN_POINT('Ctrl Pts',(-8.34055300603935,3.35518593530714,
97.4519821852785));
#182756=CARTESIAN_POINT('Ctrl Pts',(-8.61567690191595,-4.30018024354439,
97.7164279607563));
#182757=CARTESIAN_POINT('Ctrl Pts',(-2.33198012360416,-8.68258067142632,
97.9808737362333));
#182758=CARTESIAN_POINT('Ctrl Pts',(3.21318317124227,-7.84533068859849,
98.1924303566154));
#182759=CARTESIAN_POINT('Ctrl Pts',(6.57877685610312,-5.38414191851868,
98.3510978219017));
#182760=CARTESIAN_POINT('Ctrl Pts',(8.34885206896818,-1.56744411886069,
98.5097652871882));
#182761=CARTESIAN_POINT('Ctrl Pts',(8.08427756212467,2.60563396349751,98.6684327524747));
#182762=CARTESIAN_POINT('Ctrl Pts',(5.85345793495883,6.15917312380028,98.8271060348031));
#182763=CARTESIAN_POINT('Ctrl Pts',(3.41624814820702,7.52225365430131,98.9328901620362));
#182764=CARTESIAN_POINT('Ctrl Pts',(2.10803039418863,7.87255331703859,98.9857851341739));
#182765=CARTESIAN_POINT('Ctrl Pts',(-5.31037376991254,4.57794244025904,
-5.5424415057459E-16));
#182766=CARTESIAN_POINT('Ctrl Pts',(-5.44331700421711,4.4462003696002,-1.29451042284116E-17));
#182767=CARTESIAN_POINT('Ctrl Pts',(-5.57062214561908,4.30929729963032,
-5.26815061343554E-17));
#182768=CARTESIAN_POINT('Ctrl Pts',(-5.69215510135391,4.1677062093632,-6.00214322687975E-16));
#182769=CARTESIAN_POINT('Ctrl Pts',(-5.81562375753537,4.02385994530381,
-2.0711506702255E-16));
#182770=CARTESIAN_POINT('Ctrl Pts',(-5.93313534079326,3.87517474031655,
-2.03905455560608E-15));
#182771=CARTESIAN_POINT('Ctrl Pts',(-6.0445238637167,3.72209865847224,-2.23432383705813E-15));
#182772=CARTESIAN_POINT('Ctrl Pts',(-6.15706744801159,3.56743522934661,
-2.43588381465624E-15));
#182773=CARTESIAN_POINT('Ctrl Pts',(-6.26336079465251,3.40828890743599,
-2.83121763992797E-15));
#182774=CARTESIAN_POINT('Ctrl Pts',(-6.36320004341494,3.24508007515358,
-8.46545056276682E-16));
#182775=CARTESIAN_POINT('Ctrl Pts',(-6.46313479819719,3.08171511763823,
3.73578344344788E-16));
#182776=CARTESIAN_POINT('Ctrl Pts',(-6.55660354150345,2.91427931386131,
-4.62227720763348E-16));
#182777=CARTESIAN_POINT('Ctrl Pts',(-6.6433625023191,2.74316055617857,-2.4980018054066E-16));
#182778=CARTESIAN_POINT('Ctrl Pts',(-6.69216088121534,2.64691323030984,
-1.28918032690918E-15));
#182779=CARTESIAN_POINT('Ctrl Pts',(-6.73883580575461,2.54950020323732,
-4.43215479361793E-15));
#182780=CARTESIAN_POINT('Ctrl Pts',(-6.78333763054534,2.45098684037426,
-3.88578058618805E-15));
#182781=CARTESIAN_POINT('Ctrl Pts',(-6.80155036661689,2.41066944022755,
-4.0530119472609E-15));
#182782=CARTESIAN_POINT('Ctrl Pts',(-6.81939896718112,2.37016796639514,
-4.21525031975438E-15));
#182783=CARTESIAN_POINT('Ctrl Pts',(-6.83688040508793,2.32948533314358,
-3.38618022510673E-15));
#182784=CARTESIAN_POINT('Ctrl Pts',(-6.84857336763547,2.30227358377367,
-2.8316328464711E-15));
#182785=CARTESIAN_POINT('Ctrl Pts',(-6.86010074485217,2.27498362189078,
-2.63071505109977E-15));
#182786=CARTESIAN_POINT('Ctrl Pts',(-6.87145407498761,2.24763530599042,
-2.83106871279415E-15));
#182787=CARTESIAN_POINT('Ctrl Pts',(-6.9466808909752,2.06642620669855,-4.158605907689E-15));
#182788=CARTESIAN_POINT('Ctrl Pts',(-7.01434821512689,1.88247767504642,
-3.52510701043973E-15));
#182789=CARTESIAN_POINT('Ctrl Pts',(-7.07427559886283,1.69624669194298,
-3.24740234702858E-15));
#182790=CARTESIAN_POINT('Ctrl Pts',(-7.09090024774233,1.64458375404096,
-3.17036340033011E-15));
#182791=CARTESIAN_POINT('Ctrl Pts',(-7.10692902931713,1.59274494156417,
-3.35064743386125E-15));
#182792=CARTESIAN_POINT('Ctrl Pts',(-7.12235757386584,1.54073952802914,
-3.30291349825984E-15));
#182793=CARTESIAN_POINT('Ctrl Pts',(-7.17736258705981,1.35533263831109,
-3.29727963165626E-15));
#182794=CARTESIAN_POINT('Ctrl Pts',(-7.22474203445627,1.1678103027789,-7.24618974341882E-15));
#182795=CARTESIAN_POINT('Ctrl Pts',(-7.2645811339778,0.978661458527771,
-5.93969318174459E-15));
#182796=CARTESIAN_POINT('Ctrl Pts',(-7.30481065710714,0.787658953549531,
-4.6203929395823E-15));
#182797=CARTESIAN_POINT('Ctrl Pts',(-7.33735147280739,0.594997259193497,
-3.65400968452058E-15));
#182798=CARTESIAN_POINT('Ctrl Pts',(-7.36224272937163,0.401157436213471,
-4.46864767411626E-15));
#182799=CARTESIAN_POINT('Ctrl Pts',(-7.38723762758615,0.206510507369071,
-5.28667763492113E-15));
#182800=CARTESIAN_POINT('Ctrl Pts',(-7.40451925616537,0.0106749153794845,
6.33680537375195E-16));
#182801=CARTESIAN_POINT('Ctrl Pts',(-7.41407644285483,-0.185874504306108,
-2.47024622979097E-15));
#182802=CARTESIAN_POINT('Ctrl Pts',(-7.41856230265033,-0.278128968746951,
-3.92713733649873E-15));
#182803=CARTESIAN_POINT('Ctrl Pts',(-7.42134566510405,-0.370540804922235,
-2.36763060747942E-15));
#182804=CARTESIAN_POINT('Ctrl Pts',(-7.42242141675543,-0.463061154024065,
-1.27675647831893E-15));
#182805=CARTESIAN_POINT('Ctrl Pts',(-7.42269559403654,-0.486641854765678,
-1.53461354303058E-15));
#182806=CARTESIAN_POINT('Ctrl Pts',(-7.42285872142643,-0.51022086257157,
5.6084351793085E-16));
#182807=CARTESIAN_POINT('Ctrl Pts',(-7.42291095902123,-0.533793942563365,
6.10622663543836E-16));
#182808=CARTESIAN_POINT('Ctrl Pts',(-7.42335282790941,-0.733194598119087,
1.18421068391936E-15));
#182809=CARTESIAN_POINT('Ctrl Pts',(-7.41586523167998,-0.932247529804568,
7.72423861470331E-16));
#182810=CARTESIAN_POINT('Ctrl Pts',(-7.40054244195954,-1.13044606574323,
2.22044604925031E-16));
#182811=CARTESIAN_POINT('Ctrl Pts',(-7.38505711727589,-1.33074697287766,
2.03079395727939E-16));
#182812=CARTESIAN_POINT('Ctrl Pts',(-7.36156964218886,-1.53017596445833,
1.52734294973599E-15));
#182813=CARTESIAN_POINT('Ctrl Pts',(-7.33012671706286,-1.72822631265957,
4.55191440096314E-15));
#182814=CARTESIAN_POINT('Ctrl Pts',(-7.30875088127035,-1.86286683051321,
7.77125758281482E-15));
#182815=CARTESIAN_POINT('Ctrl Pts',(-7.28369723421018,-1.99687051716647,
3.11416431501379E-15));
#182816=CARTESIAN_POINT('Ctrl Pts',(-7.25496680053326,-2.13007981682257,
3.77475828372553E-15));
#182817=CARTESIAN_POINT('Ctrl Pts',(-7.21283996301465,-2.32540184313392,
5.39452731674499E-15));
#182818=CARTESIAN_POINT('Ctrl Pts',(-7.1628105078922,-2.5190165641108,7.91946181298321E-15));
#182819=CARTESIAN_POINT('Ctrl Pts',(-7.10510958622245,-2.71054433168845,
7.43849426498855E-15));
#182820=CARTESIAN_POINT('Ctrl Pts',(-7.04813384283894,-2.89966500117753,
6.96357145964442E-15));
#182821=CARTESIAN_POINT('Ctrl Pts',(-6.98367793666496,-3.08675141819751,
4.05359569947312E-15));
#182822=CARTESIAN_POINT('Ctrl Pts',(-6.9119160153231,-3.27142605479363,
7.21644966006352E-15));
#182823=CARTESIAN_POINT('Ctrl Pts',(-6.90344888187215,-3.29321567195866,
7.50934034666217E-15));
#182824=CARTESIAN_POINT('Ctrl Pts',(-6.89487915416516,-3.31497377116827,
4.18261731543151E-15));
#182825=CARTESIAN_POINT('Ctrl Pts',(-6.88620977404331,-3.33669297006139,
4.6074255521944E-15));
#182826=CARTESIAN_POINT('Ctrl Pts',(-6.81144348703153,-3.52400323161249,
7.94999150818934E-15));
#182827=CARTESIAN_POINT('Ctrl Pts',(-6.72942390076641,-3.70803833235806,
5.973420582007E-15));
#182828=CARTESIAN_POINT('Ctrl Pts',(-6.64046121208781,-3.88843228962424,
5.32907051820075E-15));
#182829=CARTESIAN_POINT('Ctrl Pts',(-6.55004708816424,-4.07176939251072,
4.94538641220604E-15));
#182830=CARTESIAN_POINT('Ctrl Pts',(-6.45246134861859,-4.25134619449774,
4.35779931711698E-15));
#182831=CARTESIAN_POINT('Ctrl Pts',(-6.34797624592836,-4.42677407068446,
5.10702591327572E-15));
#182832=CARTESIAN_POINT('Ctrl Pts',(-6.24321137245675,-4.60267167502124,
4.46111568676177E-15));
#182833=CARTESIAN_POINT('Ctrl Pts',(-6.13150990586085,-4.77439874985371,
3.81014534070484E-15));
#182834=CARTESIAN_POINT('Ctrl Pts',(-6.01309583774504,-4.9415495441527,
3.21964677141295E-15));
#182835=CARTESIAN_POINT('Ctrl Pts',(-5.89542306846566,-5.10765393669139,
1.39687856458722E-15));
#182836=CARTESIAN_POINT('Ctrl Pts',(-5.77112118527314,-5.26923978164349,
3.32033915991433E-15));
#182837=CARTESIAN_POINT('Ctrl Pts',(-5.64036429125108,-5.42588572441345,
7.21644966006352E-16));
#182838=CARTESIAN_POINT('Ctrl Pts',(-5.61065088558373,-5.46148219891278,
6.16089719191022E-17));
#182839=CARTESIAN_POINT('Ctrl Pts',(-5.58060397387421,-5.49682346636191,
-5.43804932423255E-16));
#182840=CARTESIAN_POINT('Ctrl Pts',(-5.55022529123342,-5.53190436285383,
-3.88578058618805E-16));
#182841=CARTESIAN_POINT('Ctrl Pts',(-5.49592838736925,-5.59460570138167,
-1.3145331549245E-15));
#182842=CARTESIAN_POINT('Ctrl Pts',(-5.4405716751327,-5.65647532218303,
-2.98346659311989E-15));
#182843=CARTESIAN_POINT('Ctrl Pts',(-5.38418198249291,-5.71749394780626,
-1.0547118733939E-15));
#182844=CARTESIAN_POINT('Ctrl Pts',(-5.3532841852219,-5.75092809216853,
-2.12288582659533E-15));
#182845=CARTESIAN_POINT('Ctrl Pts',(-5.32207678287485,-5.78410615876794,
-9.2856319916077E-16));
#182846=CARTESIAN_POINT('Ctrl Pts',(-5.29056207773922,-5.81702691076677,
-9.43689570931383E-16));
#182847=CARTESIAN_POINT('Ctrl Pts',(-5.26481480858875,-5.84392290927611,
-9.56047699099551E-16));
#182848=CARTESIAN_POINT('Ctrl Pts',(-5.2388654098733,-5.87064385109954,
-1.61816256334409E-15));
#182849=CARTESIAN_POINT('Ctrl Pts',(-5.21273330931233,-5.89717117551002,
-1.55431223447522E-15));
#182850=CARTESIAN_POINT('Ctrl Pts',(-5.06794396085344,-6.04415032893814,
-1.2005386258731E-15));
#182851=CARTESIAN_POINT('Ctrl Pts',(-4.91743267615075,-6.18531130546595,
-6.78621530379578E-15));
#182852=CARTESIAN_POINT('Ctrl Pts',(-4.7616898899603,-6.32041813742794,
-7.21644966006352E-15));
#182853=CARTESIAN_POINT('Ctrl Pts',(-4.60415030900679,-6.45708368844242,
-7.65164760313445E-15));
#182854=CARTESIAN_POINT('Ctrl Pts',(-4.44125734847368,-6.5875551138735,
-5.31908651156807E-15));
#182855=CARTESIAN_POINT('Ctrl Pts',(-4.27347429869626,-6.71155865210133,
-5.55111512312578E-15));
#182856=CARTESIAN_POINT('Ctrl Pts',(-4.18666791907056,-6.775714704984,-5.67116040639858E-15));
#182857=CARTESIAN_POINT('Ctrl Pts',(-4.09855191061382,-6.83813894088107,
-6.05852963778292E-15));
#182858=CARTESIAN_POINT('Ctrl Pts',(-4.0091865085521,-6.89878969045305,
-6.99440505513849E-15));
#182859=CARTESIAN_POINT('Ctrl Pts',(-3.96288609764166,-6.9302129768975,
-7.47928416254308E-15));
#182860=CARTESIAN_POINT('Ctrl Pts',(-3.91625027173235,-6.96116016182333,
-5.96833885139656E-15));
#182861=CARTESIAN_POINT('Ctrl Pts',(-3.86928716320199,-6.99162514744697,
-6.43929354282591E-15));
#182862=CARTESIAN_POINT('Ctrl Pts',(-3.82791623921479,-7.01846248091889,
-6.85416877894764E-15));
#182863=CARTESIAN_POINT('Ctrl Pts',(-3.78628685685069,-7.04492822151511,
-6.98377421794483E-15));
#182864=CARTESIAN_POINT('Ctrl Pts',(-3.74443893455879,-7.07099713057179,
-6.99440505513849E-15));
#182865=CARTESIAN_POINT('Ctrl Pts',(-3.56475677190967,-7.18292904261593,
-7.04005061441867E-15));
#182866=CARTESIAN_POINT('Ctrl Pts',(-3.38092705064562,-7.28762890985193,
-5.99451951854587E-15));
#182867=CARTESIAN_POINT('Ctrl Pts',(-3.19343322407553,-7.3848264137291,
-4.88498130835069E-15));
#182868=CARTESIAN_POINT('Ctrl Pts',(-3.00594251740804,-7.48202230023705,
-3.77546156090279E-15));
#182869=CARTESIAN_POINT('Ctrl Pts',(-2.81478723729241,-7.57171655436551,
-2.84648883508677E-17));
#182870=CARTESIAN_POINT('Ctrl Pts',(-2.6204162358938,-7.65360035997005,
-1.33226762955019E-15));
#182871=CARTESIAN_POINT('Ctrl Pts',(-2.51614285898561,-7.6975282137293,
-2.03171309038931E-15));
#182872=CARTESIAN_POINT('Ctrl Pts',(-2.41094347454657,-7.73920755509353,
-2.1150680020794E-15));
#182873=CARTESIAN_POINT('Ctrl Pts',(-2.30488418583266,-7.77858539180668,
-2.22044604925031E-16));
#182874=CARTESIAN_POINT('Ctrl Pts',(-2.23785903866026,-7.80347057945064,
9.04037669818684E-16));
#182875=CARTESIAN_POINT('Ctrl Pts',(-2.17049042810051,-7.82743653127443,
2.51112873167852E-15));
#182876=CARTESIAN_POINT('Ctrl Pts',(-2.10279483963403,-7.85048474619609,
1.88737914186277E-15));
#182877=CARTESIAN_POINT('Ctrl Pts',(2.10803039481951,-7.87255331939627,
0.0142148672352196));
#182878=CARTESIAN_POINT('Ctrl Pts',(3.4162481492297,-7.52225365655416,0.0671098393728272));
#182879=CARTESIAN_POINT('Ctrl Pts',(5.85345793671154,-6.159173125645,0.172893966605912));
#182880=CARTESIAN_POINT('Ctrl Pts',(8.08427756454558,-2.60563396427805,
0.331567248934471));
#182881=CARTESIAN_POINT('Ctrl Pts',(8.34885207146841,1.56744411932978,0.490234714220902));
#182882=CARTESIAN_POINT('Ctrl Pts',(6.57877685807347,5.38414192013079,0.648902179507327));
#182883=CARTESIAN_POINT('Ctrl Pts',(3.21318317220485,7.84533069094777,0.807569644793758));
#182884=CARTESIAN_POINT('Ctrl Pts',(-2.33198012430219,8.68258067402656,
1.01912626517566));
#182885=CARTESIAN_POINT('Ctrl Pts',(-8.61567690449593,4.3001802448325,1.28357204065304));
#182886=CARTESIAN_POINT('Ctrl Pts',(-8.34055300853718,-3.3551859363116,
1.54801781613043));
#182887=CARTESIAN_POINT('Ctrl Pts',(-4.33825713510923,-7.28420074392475,
1.75957443651233));
#182888=CARTESIAN_POINT('Ctrl Pts',(-0.348317063221276,-8.49309379117966,
1.91824190179876));
#182889=CARTESIAN_POINT('Ctrl Pts',(3.76605381199188,-7.61608932670582,
2.07690936708519));
#182890=CARTESIAN_POINT('Ctrl Pts',(6.94160524601032,-4.89106892912396,
2.23557683237162));
#182891=CARTESIAN_POINT('Ctrl Pts',(8.44121995903425,-0.98203985862958,
2.39424429765805));
#182892=CARTESIAN_POINT('Ctrl Pts',(7.87642355615024,3.18674250718402,2.55291176294447));
#182893=CARTESIAN_POINT('Ctrl Pts',(5.40557535500932,6.53706339081806,2.7115792282309));
#182894=CARTESIAN_POINT('Ctrl Pts',(0.336812665113362,8.98358877414629,
2.92313584861281));
#182895=CARTESIAN_POINT('Ctrl Pts',(-5.46494857012726,7.12725858675843,
3.13469246899471));
#182896=CARTESIAN_POINT('Ctrl Pts',(-8.17994426748479,2.22908354222041,
3.34624908937662));
#182897=CARTESIAN_POINT('Ctrl Pts',(-8.32530750509452,-3.36923491103502,
3.55780570975852));
#182898=CARTESIAN_POINT('Ctrl Pts',(-4.2675825718424,-7.9125255319526,3.76936233014043));
#182899=CARTESIAN_POINT('Ctrl Pts',(1.34181698717311,-8.37566203946278,
3.98091895052233));
#182900=CARTESIAN_POINT('Ctrl Pts',(5.17047444783897,-6.74238192670933,
4.13958641580877));
#182901=CARTESIAN_POINT('Ctrl Pts',(7.77286267259136,-3.43594665272709,
4.29825388109519));
#182902=CARTESIAN_POINT('Ctrl Pts',(8.46247612164212,0.692405568114126,
4.45692134638163));
#182903=CARTESIAN_POINT('Ctrl Pts',(7.11095747028491,4.65375386049991,4.61558881166805));
#182904=CARTESIAN_POINT('Ctrl Pts',(4.00570910623038,7.49318164626026,4.77425627695448));
#182905=CARTESIAN_POINT('Ctrl Pts',(-0.0375200648430894,8.48238506412354,
4.93292374224091));
#182906=CARTESIAN_POINT('Ctrl Pts',(-5.49703181695961,7.11356738199704,
5.14448036262281));
#182907=CARTESIAN_POINT('Ctrl Pts',(-8.76225529409264,1.97113639024106,
5.35603698300472));
#182908=CARTESIAN_POINT('Ctrl Pts',(-7.7088088173919,-3.52913570365432,
5.56759360338662));
#182909=CARTESIAN_POINT('Ctrl Pts',(-4.23369274894941,-7.92075385899074,
5.77915022376853));
#182910=CARTESIAN_POINT('Ctrl Pts',(1.79262212218929,-8.80946689787677,
5.99070684415043));
#182911=CARTESIAN_POINT('Ctrl Pts',(6.39632924532418,-5.57128663863554,
6.20226346453234));
#182912=CARTESIAN_POINT('Ctrl Pts',(8.28962143476218,-1.86431093903326,
6.36093092981877));
#182913=CARTESIAN_POINT('Ctrl Pts',(8.16943141864774,2.34169384412702,6.51959839510519));
#182914=CARTESIAN_POINT('Ctrl Pts',(6.05400114274586,5.95331792659014,6.67826586039163));
#182915=CARTESIAN_POINT('Ctrl Pts',(2.47835881711179,8.12901453694417,6.83693332567804));
#182916=CARTESIAN_POINT('Ctrl Pts',(-1.7250390681998,8.31971868542347,6.99560079096449));
#182917=CARTESIAN_POINT('Ctrl Pts',(-5.46324238754078,6.48885546800465,
7.1542682562509));
#182918=CARTESIAN_POINT('Ctrl Pts',(-8.77816746704173,1.94009713653053,
7.36582487663282));
#182919=CARTESIAN_POINT('Ctrl Pts',(-7.99063545691195,-4.10027329976967,
7.57738149701471));
#182920=CARTESIAN_POINT('Ctrl Pts',(-3.65790945582747,-7.64854434479778,
7.78893811739663));
#182921=CARTESIAN_POINT('Ctrl Pts',(1.82392380767687,-8.79407744347022,
8.00049473777853));
#182922=CARTESIAN_POINT('Ctrl Pts',(7.02038676861,-5.61554722162305,8.21205135816044));
#182923=CARTESIAN_POINT('Ctrl Pts',(8.48056307710129,-0.179756958159142,
8.42360797854234));
#182924=CARTESIAN_POINT('Ctrl Pts',(7.55930044732043,3.87949166008483,8.58227544382877));
#182925=CARTESIAN_POINT('Ctrl Pts',(4.77234369525983,7.03191833138082,8.7409429091152));
#182926=CARTESIAN_POINT('Ctrl Pts',(0.834217223423008,8.44967489308136,
8.89961037440162));
#182927=CARTESIAN_POINT('Ctrl Pts',(-3.30512064769089,7.82938805201916,
9.05827783968807));
#182928=CARTESIAN_POINT('Ctrl Pts',(-6.65472716673046,5.28281034392745,
9.21694530497447));
#182929=CARTESIAN_POINT('Ctrl Pts',(-8.35198742766335,1.48208254725105,
9.37561277026092));
#182930=CARTESIAN_POINT('Ctrl Pts',(-7.98296706987295,-4.13430015122383,
9.58716939064281));
#182931=CARTESIAN_POINT('Ctrl Pts',(-3.50838750204087,-8.26763045095955,
9.79872601102473));
#182932=CARTESIAN_POINT('Ctrl Pts',(2.09162098999237,-8.21618243562534,
10.0102826314066));
#182933=CARTESIAN_POINT('Ctrl Pts',(7.03456103927407,-5.58367684620427,
10.2218392517885));
#182934=CARTESIAN_POINT('Ctrl Pts',(8.98807970294324,0.186075878676646,
10.4333958721704));
#182935=CARTESIAN_POINT('Ctrl Pts',(6.62666006128773,5.29524684040758,10.6449524925523));
#182936=CARTESIAN_POINT('Ctrl Pts',(3.31865127176191,7.82176658626181,10.8036199578387));
#182937=CARTESIAN_POINT('Ctrl Pts',(-0.840887270322603,8.45671616902799,
10.9622874231252));
#182938=CARTESIAN_POINT('Ctrl Pts',(-4.77295389581727,7.02223862333318,
11.1209548884116));
#182939=CARTESIAN_POINT('Ctrl Pts',(-7.5537943117649,3.89401223167548,11.279622353698));
#182940=CARTESIAN_POINT('Ctrl Pts',(-8.49414566628779,-0.207287706854769,
11.4382898189845));
#182941=CARTESIAN_POINT('Ctrl Pts',(-7.36230256501997,-4.21292815151322,
11.5969572842709));
#182942=CARTESIAN_POINT('Ctrl Pts',(-3.48069952670291,-8.28884381466413,
11.8085139046528));
#182943=CARTESIAN_POINT('Ctrl Pts',(2.60305770872397,-8.59573072537543,
12.0200705250347));
#182944=CARTESIAN_POINT('Ctrl Pts',(6.86986101384801,-4.96845467239725,
12.2316271454166));
#182945=CARTESIAN_POINT('Ctrl Pts',(8.97854442063184,0.219627468344228,
12.4431837657985));
#182946=CARTESIAN_POINT('Ctrl Pts',(6.78195923173225,5.90129053328225,12.6547403861804));
#182947=CARTESIAN_POINT('Ctrl Pts',(1.69552102711242,8.31128576787805,12.8662970065623));
#182948=CARTESIAN_POINT('Ctrl Pts',(-2.46308694886501,8.13183137281261,
13.0249644718488));
#182949=CARTESIAN_POINT('Ctrl Pts',(-6.06363365216522,5.95445099880917,
13.1836319371352));
#182950=CARTESIAN_POINT('Ctrl Pts',(-8.16369841306695,2.33387068945947,
13.3422994024216));
#182951=CARTESIAN_POINT('Ctrl Pts',(-8.29469668283903,-1.84963420832045,
13.500966867708));
#182952=CARTESIAN_POINT('Ctrl Pts',(-6.38911994390509,-5.60112713084813,
13.6596343329945));
#182953=CARTESIAN_POINT('Ctrl Pts',(-2.95376983307013,-7.95157257666414,
13.8183017982809));
#182954=CARTESIAN_POINT('Ctrl Pts',(2.63790774924367,-8.5942797071986,14.0298584186628));
#182955=CARTESIAN_POINT('Ctrl Pts',(7.50571555676396,-4.93221351109846,
14.2414150390447));
#182956=CARTESIAN_POINT('Ctrl Pts',(8.45792928339156,0.586484798099847,
14.4529716594266));
#182957=CARTESIAN_POINT('Ctrl Pts',(6.7531423154713,5.92094291520376,14.6645282798085));
#182958=CARTESIAN_POINT('Ctrl Pts',(1.4264861409623,8.87611053720761,14.8760849001904));
#182959=CARTESIAN_POINT('Ctrl Pts',(-4.02297065926845,7.46779550760314,
15.0876415205724));
#182960=CARTESIAN_POINT('Ctrl Pts',(-7.10103632182176,4.66570058508865,
15.2463089858587));
#182961=CARTESIAN_POINT('Ctrl Pts',(-8.47059776903331,0.687104941139273,
15.4049764511452));
#182962=CARTESIAN_POINT('Ctrl Pts',(-7.76344919178384,-3.4382816669407,
15.5636439164316));
#182963=CARTESIAN_POINT('Ctrl Pts',(-5.18377337434866,-6.73436213521994,
15.7223113817181));
#182964=CARTESIAN_POINT('Ctrl Pts',(-1.31716520521893,-8.39395941232081,
15.8809788470045));
#182965=CARTESIAN_POINT('Ctrl Pts',(2.82641118567979,-7.99772858242742,
16.0396463122909));
#182966=CARTESIAN_POINT('Ctrl Pts',(7.53154427612354,-4.90877192339148,
16.2512029326728));
#182967=CARTESIAN_POINT('Ctrl Pts',(8.92292854400946,1.02168602643451,16.4627595530547));
#182968=CARTESIAN_POINT('Ctrl Pts',(6.11837120860958,5.86907709396564,16.6743161734366));
#182969=CARTESIAN_POINT('Ctrl Pts',(1.39176936253974,8.87273769360992,16.8858727938185));
#182970=CARTESIAN_POINT('Ctrl Pts',(-4.59140730818783,7.72911249170335,
17.0974294142004));
#182971=CARTESIAN_POINT('Ctrl Pts',(-7.87330703075219,3.15646939922137,
17.3089860345823));
#182972=CARTESIAN_POINT('Ctrl Pts',(-8.441462578291,-0.967051359980911,
17.4676534998688));
#182973=CARTESIAN_POINT('Ctrl Pts',(-6.94405265035244,-4.89931347782761,
17.6263209651552));
#182974=CARTESIAN_POINT('Ctrl Pts',(-3.75807080154932,-7.61379196098583,
17.7849884304416));
#182975=CARTESIAN_POINT('Ctrl Pts',(0.334349638221215,-8.49184020600429,
17.943655895728));
#182976=CARTESIAN_POINT('Ctrl Pts',(4.36644429984199,-7.28887117254147,
18.1023233610145));
#182977=CARTESIAN_POINT('Ctrl Pts',(7.29408571958939,-4.32996260769013,
18.2609908263009));
#182978=CARTESIAN_POINT('Ctrl Pts',(8.92774180567757,1.05623256446788,18.4725474466828));
#182979=CARTESIAN_POINT('Ctrl Pts',(6.19658250590297,6.50114308300071,18.6841040670647));
#182980=CARTESIAN_POINT('Ctrl Pts',(0.937612275068185,8.4262337614676,18.8956606874466));
#182981=CARTESIAN_POINT('Ctrl Pts',(-4.61590244562942,7.70428067703549,
19.1072173078285));
#182982=CARTESIAN_POINT('Ctrl Pts',(-8.4771793246631,2.99293028261425,19.3187739282104));
#182983=CARTESIAN_POINT('Ctrl Pts',(-8.06749931840342,-2.6206330182368,
19.5303305485923));
#182984=CARTESIAN_POINT('Ctrl Pts',(-5.86190916878713,-6.1507316386279,
19.6889980138788));
#182985=CARTESIAN_POINT('Ctrl Pts',(-2.19288325165259,-8.21062743092827,
19.8476654791652));
#182986=CARTESIAN_POINT('Ctrl Pts',(1.99245080157417,-8.25366972794139,
20.0063329444516));
#182987=CARTESIAN_POINT('Ctrl Pts',(5.6972100086841,-6.30594464627148,20.165000409738));
#182988=CARTESIAN_POINT('Ctrl Pts',(8.02239891580781,-2.79903455305117,
20.3236678750245));
#182989=CARTESIAN_POINT('Ctrl Pts',(8.37459038364871,1.34851717631298,20.4823353403109));
#182990=CARTESIAN_POINT('Ctrl Pts',(6.17814516547287,6.53075212310415,20.6938919606928));
#182991=CARTESIAN_POINT('Ctrl Pts',(0.592716465026654,8.96165070342495,
20.9054485810747));
#182992=CARTESIAN_POINT('Ctrl Pts',(-4.67854763534728,7.07048260057551,
21.1170052014566));
#182993=CARTESIAN_POINT('Ctrl Pts',(-8.48007796282208,2.95817069868685,
21.3285618218385));
#182994=CARTESIAN_POINT('Ctrl Pts',(-8.4263858148105,-3.13308523328778,
21.5401184422205));
#182995=CARTESIAN_POINT('Ctrl Pts',(-4.51537004268918,-7.18078658966394,
21.7516750626023));
#182996=CARTESIAN_POINT('Ctrl Pts',(-0.560248715354337,-8.47818377781896,
21.9103425278888));
#182997=CARTESIAN_POINT('Ctrl Pts',(3.57659993765015,-7.70915511913537,
22.0690099931752));
#182998=CARTESIAN_POINT('Ctrl Pts',(6.81773385092994,-5.0607735883473,22.2276774584616));
#182999=CARTESIAN_POINT('Ctrl Pts',(8.41444502931074,-1.19174435748521,
22.386344923748));
#183000=CARTESIAN_POINT('Ctrl Pts',(7.95297533686621,2.99059560701983,22.5450123890345));
#183001=CARTESIAN_POINT('Ctrl Pts',(5.56616896288688,6.40078321342844,22.7036798543209));
#183002=CARTESIAN_POINT('Ctrl Pts',(0.559590308908195,8.97257263360188,
22.9152364747028));
#183003=CARTESIAN_POINT('Ctrl Pts',(-5.28639056270976,7.26061780818986,
23.1267930950847));
#183004=CARTESIAN_POINT('Ctrl Pts',(-8.12212057676843,2.4313966187543,23.3383497154666));
#183005=CARTESIAN_POINT('Ctrl Pts',(-8.40634190701105,-3.16163120565004,
23.5499063358486));
#183006=CARTESIAN_POINT('Ctrl Pts',(-4.46261386723436,-7.80418339424779,
23.7614629562304));
#183007=CARTESIAN_POINT('Ctrl Pts',(1.13357108138952,-8.4063832456146,23.9730195766124));
#183008=CARTESIAN_POINT('Ctrl Pts',(5.0015756079893,-6.8686039506653,24.1316870418987));
#183009=CARTESIAN_POINT('Ctrl Pts',(7.6852099193921,-3.6277662906763,24.2903545071852));
#183010=CARTESIAN_POINT('Ctrl Pts',(8.47705154584668,0.482204586963322,
24.4490219724716));
#183011=CARTESIAN_POINT('Ctrl Pts',(7.22424657979749,4.4758687558031,24.6076894377581));
#183012=CARTESIAN_POINT('Ctrl Pts',(4.19041193584253,7.39147661847597,24.7663569030444));
#183013=CARTESIAN_POINT('Ctrl Pts',(0.172973997312942,8.48070413733235,
24.9250243683309));
#183014=CARTESIAN_POINT('Ctrl Pts',(-5.31882267198645,7.24778078883794,
25.1365809887128));
#183015=CARTESIAN_POINT('Ctrl Pts',(-8.71064532758041,2.18795660725075,
25.3481376090947));
#183016=CARTESIAN_POINT('Ctrl Pts',(-7.79400736662216,-3.33676210573878,
25.5596942294766));
#183017=CARTESIAN_POINT('Ctrl Pts',(-4.42893524494197,-7.81325980204303,
25.7712508498586));
#183018=CARTESIAN_POINT('Ctrl Pts',(1.57347143296348,-8.85123655930249,
25.9828074702404));
#183019=CARTESIAN_POINT('Ctrl Pts',(6.25611342708481,-5.72829009881323,
26.1943640906224));
#183020=CARTESIAN_POINT('Ctrl Pts',(8.24080778580045,-2.06943611426375,
26.3530315559088));
#183021=CARTESIAN_POINT('Ctrl Pts',(8.22502286704817,2.13825597191375,26.5116990211952));
#183022=CARTESIAN_POINT('Ctrl Pts',(6.19986305135223,5.80126040779994,26.6703664864817));
#183023=CARTESIAN_POINT('Ctrl Pts',(2.67930960812223,8.06501331609031,26.829033951768));
#183024=CARTESIAN_POINT('Ctrl Pts',(-1.51806183654231,8.35996214429004,
26.9877014170545));
#183025=CARTESIAN_POINT('Ctrl Pts',(-5.30054526584808,6.62242271026307,
27.1463688823409));
#183026=CARTESIAN_POINT('Ctrl Pts',(-8.72732282347127,2.15732179194542,
27.3579255027229));
#183027=CARTESIAN_POINT('Ctrl Pts',(-8.08991946913675,-3.90073058810687,
27.5694821231047));
#183028=CARTESIAN_POINT('Ctrl Pts',(-3.84657462384231,-7.5554216192392,
27.7810387434866));
#183029=CARTESIAN_POINT('Ctrl Pts',(1.60514535734365,-8.83662857202387,
27.9925953638685));
#183030=CARTESIAN_POINT('Ctrl Pts',(6.87888050673705,-5.78802245616915,
28.2041519842505));
#183031=CARTESIAN_POINT('Ctrl Pts',(8.47349127139817,-0.390138875596302,
28.4157086046323));
#183032=CARTESIAN_POINT('Ctrl Pts',(7.65323878408526,3.69072010687644,28.5743760699188));
#183033=CARTESIAN_POINT('Ctrl Pts',(4.94536471097505,6.91133182826096,28.7330435352052));
#183034=CARTESIAN_POINT('Ctrl Pts',(1.04363116032353,8.42637277693261,28.8917110004916));
#183035=CARTESIAN_POINT('Ctrl Pts',(-3.10982398058202,7.90899074311553,
29.050378465778));
#183036=CARTESIAN_POINT('Ctrl Pts',(-6.52159005289998,5.44631453144641,
29.2090459310645));
#183037=CARTESIAN_POINT('Ctrl Pts',(-8.31263921698669,1.68887297240714,
29.3677133963509));
#183038=CARTESIAN_POINT('Ctrl Pts',(-8.08309778792846,-3.93493724598903,
29.5792700167329));
#183039=CARTESIAN_POINT('Ctrl Pts',(-3.71246075495181,-8.17802734655816,
29.7908266371147));
#183040=CARTESIAN_POINT('Ctrl Pts',(1.88710003723826,-8.26555416355795,
30.0023832574966));
#183041=CARTESIAN_POINT('Ctrl Pts',(6.89384124657026,-5.75651361547919,
30.2139398778785));
#183042=CARTESIAN_POINT('Ctrl Pts',(8.98992942538604,-0.0370122366697308,
30.4254964982604));
#183043=CARTESIAN_POINT('Ctrl Pts',(6.75601621840632,5.12918195478999,30.6370531186424));
#183044=CARTESIAN_POINT('Ctrl Pts',(3.51171925137983,7.73700889834157,30.7957205839287));
#183045=CARTESIAN_POINT('Ctrl Pts',(-0.63078281859802,8.47497804130793,
30.9543880492152));
#183046=CARTESIAN_POINT('Ctrl Pts',(-4.59723391948035,7.13851276276853,
31.1130555145016));
#183047=CARTESIAN_POINT('Ctrl Pts',(-7.45484209100556,4.0802535660253,31.2717229797881));
#183048=CARTESIAN_POINT('Ctrl Pts',(-8.49667383085844,0.00355042726519961,
31.4303904450745));
#183049=CARTESIAN_POINT('Ctrl Pts',(-7.46457547638134,-4.02894224656035,
31.5890579103609));
#183050=CARTESIAN_POINT('Ctrl Pts',(-3.68530769504133,-8.19992122961889,
31.8006145307429));
#183051=CARTESIAN_POINT('Ctrl Pts',(2.38896113921104,-8.6576764096061,32.0121711511247));
#183052=CARTESIAN_POINT('Ctrl Pts',(6.74445809974086,-5.13739400105683,
32.2237277715067));
#183053=CARTESIAN_POINT('Ctrl Pts',(8.98122963056665,-0.0032343689442986,
32.4352843918885));
#183054=CARTESIAN_POINT('Ctrl Pts',(6.92630597900252,5.73118543272851,32.6468410122704));
#183055=CARTESIAN_POINT('Ctrl Pts',(1.90123575731541,8.26665381298975,32.8583976326524));
#183056=CARTESIAN_POINT('Ctrl Pts',(-2.26054470865007,8.19044665532488,
33.0170650979387));
#183057=CARTESIAN_POINT('Ctrl Pts',(-5.91401240893771,6.10308094259127,
33.1757325632252));
#183058=CARTESIAN_POINT('Ctrl Pts',(-8.10327185091423,2.53572661870529,
33.3344000285116));
#183059=CARTESIAN_POINT('Ctrl Pts',(-8.33803955853058,-1.64323950940491,
33.4930674937981));
#183060=CARTESIAN_POINT('Ctrl Pts',(-6.52613937779765,-5.44086239626474,
33.6517349590845));
#183061=CARTESIAN_POINT('Ctrl Pts',(-3.1501711803149,-7.87582911212693,
33.810402424371));
#183062=CARTESIAN_POINT('Ctrl Pts',(2.4238364544957,-8.65709060949134,34.0219590447528));
#183063=CARTESIAN_POINT('Ctrl Pts',(7.38101614325807,-5.11694213677213,
34.2335156651348));
#183064=CARTESIAN_POINT('Ctrl Pts',(8.46987802192835,0.376428578763512,
34.4450722855166));
#183065=CARTESIAN_POINT('Ctrl Pts',(6.89798559148066,5.7515468282746,34.6566289058985));
#183066=CARTESIAN_POINT('Ctrl Pts',(1.64629931156174,8.83798051343387,34.8681855262805));
#183067=CARTESIAN_POINT('Ctrl Pts',(-3.83642553630601,7.56532231785874,
35.0797421466623));
#183068=CARTESIAN_POINT('Ctrl Pts',(-6.98307478551133,4.84046953646904,
35.2384096119488));
#183069=CARTESIAN_POINT('Ctrl Pts',(-8.45093966454115,0.897083357985828,
35.3970770772352));
#183070=CARTESIAN_POINT('Ctrl Pts',(-7.84637645310182,-3.24458020872331,
35.5557445425216));
#183071=CARTESIAN_POINT('Ctrl Pts',(-5.34928412448423,-6.60365801055984,
35.7144120078081));
#183072=CARTESIAN_POINT('Ctrl Pts',(-1.52504790680204,-8.35869054789607,
35.8730794730945));
#183073=CARTESIAN_POINT('Ctrl Pts',(2.62708470771682,-8.06540070964814,
36.0317469383809));
#183074=CARTESIAN_POINT('Ctrl Pts',(7.40741859067934,-5.09414868270878,
36.2433035587628));
#183075=CARTESIAN_POINT('Ctrl Pts',(8.94553321445923,0.799957278307623,
36.4548601791447));
#183076=CARTESIAN_POINT('Ctrl Pts',(6.26212293903824,5.71544823068376,36.6664167995266));
#183077=CARTESIAN_POINT('Ctrl Pts',(1.61150952903428,8.83547017288509,36.8779734199086));
#183078=CARTESIAN_POINT('Ctrl Pts',(-4.39820281689368,7.84066406374832,
37.0895300402904));
#183079=CARTESIAN_POINT('Ctrl Pts',(-7.79255786467272,3.35086624538187,
37.3010866606724));
#183080=CARTESIAN_POINT('Ctrl Pts',(-8.46285979168174,-0.757286563901003,
37.4597541259587));
#183081=CARTESIAN_POINT('Ctrl Pts',(-7.06348635977089,-4.72549470534256,
37.6184215912452));
#183082=CARTESIAN_POINT('Ctrl Pts',(-3.94584278023162,-7.51819452583688,
37.7770890565316));
#183083=CARTESIAN_POINT('Ctrl Pts',(0.123529587498059,-8.4975220038493,
37.9357565218181));
#183084=CARTESIAN_POINT('Ctrl Pts',(4.18423325630602,-7.39497605475173,
38.0944239871045));
#183085=CARTESIAN_POINT('Ctrl Pts',(7.18439576515461,-4.50962527914911,
38.2530914523909));
#183086=CARTESIAN_POINT('Ctrl Pts',(8.95120223418368,0.834373742294213,
38.4646480727728));
#183087=CARTESIAN_POINT('Ctrl Pts',(6.35599428212517,6.34537885580543,38.6762046931547));
#183088=CARTESIAN_POINT('Ctrl Pts',(1.14641270510795,8.40037321140093,38.8877613135367));
#183089=CARTESIAN_POINT('Ctrl Pts',(-4.42330659021481,7.81644771920545,
39.0993179339185));
#183090=CARTESIAN_POINT('Ctrl Pts',(-8.40030228714286,3.20236201321892,
39.3108745543005));
#183091=CARTESIAN_POINT('Ctrl Pts',(-8.13004376866344,-2.41963860696786,
39.5224311746824));
#183092=CARTESIAN_POINT('Ctrl Pts',(-6.01272886306041,-6.00337991575155,
39.6810986399688));
#183093=CARTESIAN_POINT('Ctrl Pts',(-2.39594709307398,-8.15368489040877,
39.8397661052552));
#183094=CARTESIAN_POINT('Ctrl Pts',(1.7870301727314,-8.3005690971389,39.9984335705416));
#183095=CARTESIAN_POINT('Ctrl Pts',(5.53897960608638,-6.44537389825049,
40.1571010358281));
#183096=CARTESIAN_POINT('Ctrl Pts',(7.95047325441626,-2.99724103540918,
40.3157685011145));
#183097=CARTESIAN_POINT('Ctrl Pts',(8.40547390673061,1.14029429183156,40.4744359664009));
#183098=CARTESIAN_POINT('Ctrl Pts',(6.33829733958424,6.3754362842165,40.6859925867828));
#183099=CARTESIAN_POINT('Ctrl Pts',(0.814908966460877,8.94418355773692,
40.8975492071648));
#183100=CARTESIAN_POINT('Ctrl Pts',(-4.50165959892069,7.18439928154756,
41.1091058275466));
#183101=CARTESIAN_POINT('Ctrl Pts',(-8.4040625594374,3.16768505934088,41.3206624479286));
#183102=CARTESIAN_POINT('Ctrl Pts',(-8.50153578206802,-2.92302759571368,
41.5322190683104));
#183103=CARTESIAN_POINT('Ctrl Pts',(-4.69216421186369,-7.06653080921752,
41.7437756886924));
#183104=CARTESIAN_POINT('Ctrl Pts',(-0.770454433048681,-8.46167115646284,
41.9024431539787));
#183105=CARTESIAN_POINT('Ctrl Pts',(3.38420314577333,-7.7955313374426,42.0611106192652));
#183106=CARTESIAN_POINT('Ctrl Pts',(6.69005617978553,-5.22839100354053,
42.2197780845516));
#183107=CARTESIAN_POINT('Ctrl Pts',(8.38228205845596,-1.40017400969653,
42.3784455498381));
#183108=CARTESIAN_POINT('Ctrl Pts',(8.02473532771008,2.79232908406186,42.5371130151245));
#183109=CARTESIAN_POINT('Ctrl Pts',(5.7232845171658,6.26069301309463,42.6957804804109));
#183110=CARTESIAN_POINT('Ctrl Pts',(0.782064027926499,8.95592411958767,
42.9073371007928));
#183111=CARTESIAN_POINT('Ctrl Pts',(-5.10459733350807,7.38955899899651,
43.1188937211747));
#183112=CARTESIAN_POINT('Ctrl Pts',(-8.05928680212849,2.63219080298456,
43.3304503415566));
#183113=CARTESIAN_POINT('Ctrl Pts',(-8.48220638770805,-2.95206214935692,
43.5420069619386));
#183114=CARTESIAN_POINT('Ctrl Pts',(-4.65489329170895,-7.69104475469404,
43.7535635823204));
#183115=CARTESIAN_POINT('Ctrl Pts',(0.92462547235416,-8.43192329258054,
43.9651202027024));
#183116=CARTESIAN_POINT('Ctrl Pts',(4.82959753593432,-6.99059843054699,
44.1237876679887));
#183117=CARTESIAN_POINT('Ctrl Pts',(7.59282387950186,-3.81735056399868,
44.2824551332753));
#183118=CARTESIAN_POINT('Ctrl Pts',(8.48640677810244,0.271705979293537,
44.4411225985615));
#183119=CARTESIAN_POINT('Ctrl Pts',(7.33308663060707,4.29522761167587,44.5997900638482));
#183120=CARTESIAN_POINT('Ctrl Pts',(4.37253423460613,7.28521950689286,44.7584575291344));
#183121=CARTESIAN_POINT('Ctrl Pts',(0.383361516135644,8.47380058090509,
44.917124994421));
#183122=CARTESIAN_POINT('Ctrl Pts',(-5.13733802342598,7.37753075052028,
45.1286816148028));
#183123=CARTESIAN_POINT('Ctrl Pts',(-8.65367101925888,2.40342935654577,
45.3402382351847));
#183124=CARTESIAN_POINT('Ctrl Pts',(-7.87440616908082,-3.1423335318712,
45.5517948555667));
#183125=CARTESIAN_POINT('Ctrl Pts',(-4.62145010432963,-7.70095432521442,
45.7633514759484));
#183126=CARTESIAN_POINT('Ctrl Pts',(1.35335143495645,-8.88755483745821,
45.9749080963306));
#183127=CARTESIAN_POINT('Ctrl Pts',(6.11204527800326,-5.88176651441044,
46.1864647167123));
#183128=CARTESIAN_POINT('Ctrl Pts',(8.18691835566083,-2.27328554229023,
46.3451321819989));
#183129=CARTESIAN_POINT('Ctrl Pts',(8.2755506768925,1.93349871892714,46.5037996472851));
#183130=CARTESIAN_POINT('Ctrl Pts',(6.34190383553277,5.64563517982648,46.6624671125717));
#183131=CARTESIAN_POINT('Ctrl Pts',(2.87861614074041,7.99603615249718,46.821134577858));
#183132=CARTESIAN_POINT('Ctrl Pts',(-1.31016046092372,8.39507451559495,
46.9798020431445));
#183133=CARTESIAN_POINT('Ctrl Pts',(-5.13456471748913,6.75188081050702,
47.1384695084309));
#183134=CARTESIAN_POINT('Ctrl Pts',(-8.67114696343998,2.37328761312805,
47.3500261288128));
#183135=CARTESIAN_POINT('Ctrl Pts',(-8.18413847504018,-3.69891909332623,
47.5615827491948));
#183136=CARTESIAN_POINT('Ctrl Pts',(-4.0329686081033,-7.45748897431712,
47.7731393695766));
#183137=CARTESIAN_POINT('Ctrl Pts',(1.38561984066132,-8.87412604512891,
47.9846959899586));
#183138=CARTESIAN_POINT('Ctrl Pts',(6.73265434236434,-5.95615549819381,
48.1962526103404));
#183139=CARTESIAN_POINT('Ctrl Pts',(8.46179816320036,-0.601240457908621,
48.4078092307224));
#183140=CARTESIAN_POINT('Ctrl Pts',(7.74120582594587,3.50169910810985,48.5664766960087));
#183141=CARTESIAN_POINT('Ctrl Pts',(5.1177835704526,6.78255791217336,48.7251441612953));
#183142=CARTESIAN_POINT('Ctrl Pts',(1.24779844848575,8.40530319096317,48.8838116265816));
#183143=CARTESIAN_POINT('Ctrl Pts',(-2.90429742469008,7.97020167864347,
49.0424790918682));
#183144=CARTESIAN_POINT('Ctrl Pts',(-7.56136164456266,4.84714368437679,
49.2540357122499));
#183145=CARTESIAN_POINT('Ctrl Pts',(-9.27805728479038,-2.6008240964781,
49.5184814877275));
#183146=CARTESIAN_POINT('Ctrl Pts',(-2.82248521115999,-9.21539207487178,
49.8358164183001));
#183147=CARTESIAN_POINT('Ctrl Pts',(4.66791625045747,-7.67208173557313,
50.1002621937777));
#183148=CARTESIAN_POINT('Ctrl Pts',(7.89643897624826,-3.09617872360307,
50.3118188141594));
#183149=CARTESIAN_POINT('Ctrl Pts',(8.43764997470094,1.05416382293544,50.470486279446));
#183150=CARTESIAN_POINT('Ctrl Pts',(6.8928911275569,4.94259754937307,50.6291537447324));
#183151=CARTESIAN_POINT('Ctrl Pts',(2.63608800317644,8.58571947985341,50.8407103651143));
#183152=CARTESIAN_POINT('Ctrl Pts',(-4.99930908329347,8.23575890671189,
51.1051561405917));
#183153=CARTESIAN_POINT('Ctrl Pts',(-9.63818235852632,0.24288735913145,
51.4224910711645));
#183154=CARTESIAN_POINT('Ctrl Pts',(-6.12768469299847,-6.5646711245724,
51.6869368466419));
#183155=CARTESIAN_POINT('Ctrl Pts',(-0.867116444760915,-8.43072686169507,
51.8984934670238));
#183156=CARTESIAN_POINT('Ctrl Pts',(4.68814972923802,-7.66588807412999,
52.1100500874056));
#183157=CARTESIAN_POINT('Ctrl Pts',(8.50145527199978,-2.91580736816088,
52.3216067077878));
#183158=CARTESIAN_POINT('Ctrl Pts',(8.0447532361429,2.69163301364258,52.5331633281694));
#183159=CARTESIAN_POINT('Ctrl Pts',(5.80643884209009,6.20304194060494,52.691830793456));
#183160=CARTESIAN_POINT('Ctrl Pts',(2.11999576383795,8.22961018578338,52.8504982587423));
#183161=CARTESIAN_POINT('Ctrl Pts',(-2.06596615843867,8.23572124922552,
53.0091657240289));
#183162=CARTESIAN_POINT('Ctrl Pts',(-5.75302831553045,6.25493591622287,
53.1678331893151));
#183163=CARTESIAN_POINT('Ctrl Pts',(-8.047029127633,2.72755944959616,53.3265006546018));
#183164=CARTESIAN_POINT('Ctrl Pts',(-8.36223966014006,-1.42300601179314,
53.485168119888));
#183165=CARTESIAN_POINT('Ctrl Pts',(-6.11979599351654,-6.58546341990916,
53.6967247402701));
#183166=CARTESIAN_POINT('Ctrl Pts',(-0.512933016603738,-8.96657628475243,
53.9082813606519));
#183167=CARTESIAN_POINT('Ctrl Pts',(4.74128188989137,-7.02856440921785,
54.1198379810338));
#183168=CARTESIAN_POINT('Ctrl Pts',(8.50607039726349,-2.8825885650715,54.3313946014157));
#183169=CARTESIAN_POINT('Ctrl Pts',(8.39816847567835,3.20795130586528,54.5429512217976));
#183170=CARTESIAN_POINT('Ctrl Pts',(4.45128768753787,7.22068551281421,54.7545078421795));
#183171=CARTESIAN_POINT('Ctrl Pts',(0.484776114812333,8.48283413024505,
54.913175307466));
#183172=CARTESIAN_POINT('Ctrl Pts',(-3.64506438395335,7.67702038850236,
55.0718427727524));
#183173=CARTESIAN_POINT('Ctrl Pts',(-6.86250141715301,4.99990004560204,
55.2305102380388));
#183174=CARTESIAN_POINT('Ctrl Pts',(-8.42471748741338,1.11681427094036,
55.3891777033253));
#183175=CARTESIAN_POINT('Ctrl Pts',(-7.92604615270924,-3.06125324948971,
55.5478451686116));
#183176=CARTESIAN_POINT('Ctrl Pts',(-5.50898590099322,-6.45006488330444,
55.7065126338981));
#183177=CARTESIAN_POINT('Ctrl Pts',(-0.479718345538541,-8.97719728889355,
55.91806925428));
#183178=CARTESIAN_POINT('Ctrl Pts',(5.35079580383119,-7.2132850012205,56.1296258746619));
#183179=CARTESIAN_POINT('Ctrl Pts',(8.14343672238523,-2.35901896791911,
56.3411824950438));
#183180=CARTESIAN_POINT('Ctrl Pts',(8.3778726453612,3.23631674834871,56.5527391154256));
#183181=CARTESIAN_POINT('Ctrl Pts',(4.39298520671649,7.84358858913003,56.7642957358077));
#183182=CARTESIAN_POINT('Ctrl Pts',(-1.20833730354274,8.39596234053631,
56.9758523561894));
#183183=CARTESIAN_POINT('Ctrl Pts',(-5.06250346555688,6.82382132380148,
57.134519821476));
#183184=CARTESIAN_POINT('Ctrl Pts',(-7.71719024737759,3.55922947395562,
57.2931872867624));
#183185=CARTESIAN_POINT('Ctrl Pts',(-8.47242456287475,-0.557625503363572,
57.4518547520488));
#183186=CARTESIAN_POINT('Ctrl Pts',(-7.18412830395208,-4.53998240932834,
57.6105222173352));
#183187=CARTESIAN_POINT('Ctrl Pts',(-4.12446686583729,-7.42847574311758,
57.7691896826217));
#183188=CARTESIAN_POINT('Ctrl Pts',(-0.0974946303616515,-8.48190765487712,
57.927857147908));
#183189=CARTESIAN_POINT('Ctrl Pts',(5.38311238322129,-7.20015986270839,
58.13941376829));
#183190=CARTESIAN_POINT('Ctrl Pts',(8.72977171865282,-2.1103511267997,58.3509703886718));
#183191=CARTESIAN_POINT('Ctrl Pts',(7.76400380533544,3.40599135230539,58.5625270090538));
#183192=CARTESIAN_POINT('Ctrl Pts',(4.35922714507761,7.85236491992856,58.7740836294357));
#183193=CARTESIAN_POINT('Ctrl Pts',(-1.65217912845243,8.83688322354667,
58.9856402498176));
#183194=CARTESIAN_POINT('Ctrl Pts',(-6.30684358486332,5.67238809186887,
59.1971968701995));
#183195=CARTESIAN_POINT('Ctrl Pts',(-8.25889803028424,1.99601656278161,
59.355864335486));
#183196=CARTESIAN_POINT('Ctrl Pts',(-8.20566812970426,-2.21136842476436,
59.5145318007724));
#183197=CARTESIAN_POINT('Ctrl Pts',(-6.14799025373477,-5.85620525721325,
59.6731992660588));
#183198=CARTESIAN_POINT('Ctrl Pts',(-2.60743035739999,-8.08853798261459,
59.8318667313452));
#183199=CARTESIAN_POINT('Ctrl Pts',(1.59239971700936,-8.34612137072049,
59.9905341966317));
#183200=CARTESIAN_POINT('Ctrl Pts',(5.35927043794044,-6.57498920468546,
60.149201661918));
#183201=CARTESIAN_POINT('Ctrl Pts',(8.74617592502894,-2.07956910621628,
60.3607582823));
#183202=CARTESIAN_POINT('Ctrl Pts',(8.05488525266272,3.97257091875613,60.5723149026819));
#183203=CARTESIAN_POINT('Ctrl Pts',(3.77918417033432,7.58935433274461,60.7838715230638));
#183204=CARTESIAN_POINT('Ctrl Pts',(-1.68372179736957,8.82199393828704,
60.9954281434456));
#183205=CARTESIAN_POINT('Ctrl Pts',(-6.9301175805791,5.72657587904268,61.2069847638278));
#183206=CARTESIAN_POINT('Ctrl Pts',(-8.47662769475153,0.314715098594593,
61.4185413842094));
#183207=CARTESIAN_POINT('Ctrl Pts',(-7.62009081096093,-3.7586825918449,
61.577208849496));
#183208=CARTESIAN_POINT('Ctrl Pts',(-4.88366270812431,-6.95506853439749,
61.7358763147823));
#183209=CARTESIAN_POINT('Ctrl Pts',(-0.968600827846532,-8.43532670445697,
61.8945437800688));
#183210=CARTESIAN_POINT('Ctrl Pts',(3.18008548793708,-7.8810022239752,62.0532112453553));
#183211=CARTESIAN_POINT('Ctrl Pts',(6.56980030649021,-5.38806112867788,
62.2118787106416));
#183212=CARTESIAN_POINT('Ctrl Pts',(8.32733986300889,-1.6148292400918,62.3705461759281));
#183213=CARTESIAN_POINT('Ctrl Pts',(8.04775942552698,4.00671551372531,62.5821027963099));
#183214=CARTESIAN_POINT('Ctrl Pts',(3.63953484345023,8.21074188252331,62.7936594166919));
#183215=CARTESIAN_POINT('Ctrl Pts',(-1.96058313686132,8.24843293872902,
63.0052160370739));
#183216=CARTESIAN_POINT('Ctrl Pts',(-6.94479732065039,5.69493514565335,
63.2167726574556));
#183217=CARTESIAN_POINT('Ctrl Pts',(-8.9899028102379,-0.0429935060496113,
63.4283292778377));
#183218=CARTESIAN_POINT('Ctrl Pts',(-6.71010243984948,-5.1891028044777,
63.6398858982195));
#183219=CARTESIAN_POINT('Ctrl Pts',(-3.44272605438647,-7.76795443524078,
63.798553363506));
#183220=CARTESIAN_POINT('Ctrl Pts',(0.706179398599664,-8.46902889485467,
63.9572208287924));
#183221=CARTESIAN_POINT('Ctrl Pts',(4.66057979410362,-7.09731781431708,
64.1158882940788));
#183222=CARTESIAN_POINT('Ctrl Pts',(7.49085837159483,-4.01374894850164,
64.2745557593653));
#183223=CARTESIAN_POINT('Ctrl Pts',(8.49636896109091,0.0720643499926889,
64.4332232246516));
#183224=CARTESIAN_POINT('Ctrl Pts',(7.42842502653588,4.0952123624847,64.5918906899381));
#183225=CARTESIAN_POINT('Ctrl Pts',(3.61218801807817,8.23239325476728,64.8034473103199));
#183226=CARTESIAN_POINT('Ctrl Pts',(-2.465913987405,8.63607343326995,65.0150039307019));
#183227=CARTESIAN_POINT('Ctrl Pts',(-6.78991034452835,5.07716945694371,
65.2265605510838));
#183228=CARTESIAN_POINT('Ctrl Pts',(-8.98090275980552,-0.076692613904169,
65.4381171714657));
#183229=CARTESIAN_POINT('Ctrl Pts',(-6.87502803419633,-5.79259790664771,
65.6496737918476));
#183230=CARTESIAN_POINT('Ctrl Pts',(-1.82759285440602,-8.28324616483398,
65.8612304122296));
#183231=CARTESIAN_POINT('Ctrl Pts',(2.33334461405416,-8.17000500034077,
66.0198978775159));
#183232=CARTESIAN_POINT('Ctrl Pts',(5.96809149824668,-6.05020856115271,
66.1785653428025));
#183233=CARTESIAN_POINT('Ctrl Pts',(8.1255172111483,-2.46351257881153,66.3372328080887));
#183234=CARTESIAN_POINT('Ctrl Pts',(8.32308565666732,1.71737733671682,66.4959002733753));
#183235=CARTESIAN_POINT('Ctrl Pts',(6.47746095768515,5.49872515545137,66.6545677386617));
#183236=CARTESIAN_POINT('Ctrl Pts',(3.07995689474727,7.90355161906414,66.8132352039482));
#183237=CARTESIAN_POINT('Ctrl Pts',(-2.50078270841206,8.63517728969084,
67.0247918243299));
#183238=CARTESIAN_POINT('Ctrl Pts',(-7.42626117277933,5.05105346752343,
67.2363484447121));
#183239=CARTESIAN_POINT('Ctrl Pts',(-8.46619265772629,-0.451789844414717,
67.4479050650937));
#183240=CARTESIAN_POINT('Ctrl Pts',(-6.84652756553861,-5.81270646363901,
67.6594616854758));
#183241=CARTESIAN_POINT('Ctrl Pts',(-1.56758208377637,-8.85228147935368,
67.8710183058576));
#183242=CARTESIAN_POINT('Ctrl Pts',(3.90359985443053,-7.53088114666553,
68.0825749262395));
#183243=CARTESIAN_POINT('Ctrl Pts',(7.02587515470665,-4.7781332237606,68.241242391526));
#183244=CARTESIAN_POINT('Ctrl Pts',(8.45858844313609,-0.821840200121001,
68.3999098568124));
#183245=CARTESIAN_POINT('Ctrl Pts',(7.81719117440107,3.31427915503444,68.5585773220988));
#183246=CARTESIAN_POINT('Ctrl Pts',(5.29030421491151,6.65100150944047,68.7172447873853));
#183247=CARTESIAN_POINT('Ctrl Pts',(1.45060083629443,8.37193143828057,68.8759122526716));
#183248=CARTESIAN_POINT('Ctrl Pts',(-2.69875727408849,8.04170204896118,
69.0345797179581));
#183249=CARTESIAN_POINT('Ctrl Pts',(-7.45245972838229,5.02802595219296,
69.24613633834));
#183250=CARTESIAN_POINT('Ctrl Pts',(-8.93805989614121,-0.879534781064867,
69.4576929587219));
#183251=CARTESIAN_POINT('Ctrl Pts',(-6.21101134614356,-5.77095054902837,
69.6692495791038));
#183252=CARTESIAN_POINT('Ctrl Pts',(-1.53281601924463,-8.84946163273552,
69.8808061994857));
#183253=CARTESIAN_POINT('Ctrl Pts',(4.46780524364497,-7.80121255215777,
70.0923628198677));
#183254=CARTESIAN_POINT('Ctrl Pts',(7.82206971914578,-3.28138506998721,
70.3039194402494));
#183255=CARTESIAN_POINT('Ctrl Pts',(8.45578532753984,0.832570290180003,
70.4625869055361));
#183256=CARTESIAN_POINT('Ctrl Pts',(7.02115294830815,4.78816781674929,70.6212543708223));
#183257=CARTESIAN_POINT('Ctrl Pts',(3.87877969162206,7.55301213281761,70.7799218361088));
#183258=CARTESIAN_POINT('Ctrl Pts',(-0.199146880583746,8.4960861745185,
70.9385893013953));
#183259=CARTESIAN_POINT('Ctrl Pts',(-4.24987783507853,7.35744637632085,
71.0972567666816));
#183260=CARTESIAN_POINT('Ctrl Pts',(-7.22424387249952,4.44551044756007,
71.2559242319681));
#183261=CARTESIAN_POINT('Ctrl Pts',(-8.94342240817753,-0.914000332600309,
71.4674808523501));
#183262=CARTESIAN_POINT('Ctrl Pts',(-6.29927301645491,-6.40169162036673,
71.6790374727318));
#183263=CARTESIAN_POINT('Ctrl Pts',(-1.07160968101382,-8.41024285456801,
71.8905940931139));
#183264=CARTESIAN_POINT('Ctrl Pts',(4.4926925138143,-7.776773760013,72.1021507134955));
#183265=CARTESIAN_POINT('Ctrl Pts',(8.42846848810263,-3.12747820522319,
72.3137073338779));
#183266=CARTESIAN_POINT('Ctrl Pts',(8.10818867778331,2.49189466755299,72.5252639542594));
#183267=CARTESIAN_POINT('Ctrl Pts',(5.9590647493189,6.05665139387714,72.6839314195461));
#183268=CARTESIAN_POINT('Ctrl Pts',(2.32328994654124,8.17468431128629,72.8425988848323));
#183269=CARTESIAN_POINT('Ctrl Pts',(-1.86082884426617,8.28433703967775,
73.0012663501188));
#183270=CARTESIAN_POINT('Ctrl Pts',(-5.59611972184407,6.39582549978325,
73.1599338154052));
#183271=CARTESIAN_POINT('Ctrl Pts',(-7.97683183085544,2.9263685235767,73.3186012806917));
#183272=CARTESIAN_POINT('Ctrl Pts',(-8.39499320594201,-1.21505215562958,
73.4772687459781));
#183273=CARTESIAN_POINT('Ctrl Pts',(-6.28130928397353,-6.43159036772032,
73.68882536636));
#183274=CARTESIAN_POINT('Ctrl Pts',(-0.735279526433169,-8.95108150762345,
73.900381986742));
#183275=CARTESIAN_POINT('Ctrl Pts',(4.56541761717103,-7.14405306265844,
74.1119386071238));
#183276=CARTESIAN_POINT('Ctrl Pts',(8.43192001011159,-3.09276916066988,
74.3234952275058));
#183277=CARTESIAN_POINT('Ctrl Pts',(8.47518615947612,2.998569749282,74.5350518478876));
#183278=CARTESIAN_POINT('Ctrl Pts',(4.62909106997849,7.10800805673135,74.7466084682696));
#183279=CARTESIAN_POINT('Ctrl Pts',(0.695120786654891,8.46819259851175,
74.9052759335559));
#183280=CARTESIAN_POINT('Ctrl Pts',(-3.45344407599199,7.76510552271418,
75.0639433988424));
#183281=CARTESIAN_POINT('Ctrl Pts',(-6.73632039050628,5.16864699617596,
75.2226108641288));
#183282=CARTESIAN_POINT('Ctrl Pts',(-8.39441072159572,1.3255219357103,75.3812783294153));
#183283=CARTESIAN_POINT('Ctrl Pts',(-7.99956771444687,-2.86363321246058,
75.5399457947017));
#183284=CARTESIAN_POINT('Ctrl Pts',(-5.66734195322239,-6.31137844325295,
75.6986132599881));
#183285=CARTESIAN_POINT('Ctrl Pts',(-0.702331405528227,-8.96252930683599,
75.91016988037));
#183286=CARTESIAN_POINT('Ctrl Pts',(5.17015725800501,-7.34383891882227,
76.1217265007519));
#183287=CARTESIAN_POINT('Ctrl Pts',(8.08239236995815,-2.56036438018052,
76.3332831211339));
#183288=CARTESIAN_POINT('Ctrl Pts',(8.4555991428169,3.0274311344942,76.5448397415157));
#183289=CARTESIAN_POINT('Ctrl Pts',(4.58626387481611,7.73216558602067,76.7563963618976));
#183290=CARTESIAN_POINT('Ctrl Pts',(-0.999627257927594,8.42336085027349,
76.9679529822796));
#183291=CARTESIAN_POINT('Ctrl Pts',(-4.89161787228477,6.94734146167241,
77.1266204475658));
#183292=CARTESIAN_POINT('Ctrl Pts',(-7.62649503650707,3.749628411326,77.2852879128524));
#183293=CARTESIAN_POINT('Ctrl Pts',(-8.48365272152047,-0.347218483476703,
77.4439553781389));
#183294=CARTESIAN_POINT('Ctrl Pts',(-7.29457162466165,-4.36031702718641,
77.6026228434252));
#183295=CARTESIAN_POINT('Ctrl Pts',(-4.30752757594821,-7.32384359308516,
77.7612903087117));
#183296=CARTESIAN_POINT('Ctrl Pts',(-0.307935242167678,-8.47687669813258,
77.919957773998));
#183297=CARTESIAN_POINT('Ctrl Pts',(5.20278957938838,-7.33151973138541,
78.1315143943802));
#183298=CARTESIAN_POINT('Ctrl Pts',(8.67471728284177,-2.32632246278883,
78.3430710147618));
#183299=CARTESIAN_POINT('Ctrl Pts',(7.84612964182211,3.21228607458539,78.5546276351438));
#183300=CARTESIAN_POINT('Ctrl Pts',(4.55273398345825,7.74177688996364,78.7661842555257));
#183301=CARTESIAN_POINT('Ctrl Pts',(-1.43239137558603,8.87515948736878,
78.9777408759076));
#183302=CARTESIAN_POINT('Ctrl Pts',(-6.16414658142105,5.82713991521296,
79.1892974962896));
#183303=CARTESIAN_POINT('Ctrl Pts',(-8.20682568982982,2.20033881260999,
79.3479649615759));
#183304=CARTESIAN_POINT('Ctrl Pts',(-8.25801451613462,-2.00707150251296,
79.5066324268624));
#183305=CARTESIAN_POINT('Ctrl Pts',(-6.29141346134359,-5.70184538838567,
79.6652998921488));
#183306=CARTESIAN_POINT('Ctrl Pts',(-2.80733701712054,-8.02134643543056,
79.8239673574353));
#183307=CARTESIAN_POINT('Ctrl Pts',(1.38480816911518,-8.38306537778871,
79.9826348227216));
#183308=CARTESIAN_POINT('Ctrl Pts',(5.19446800254897,-6.70594995800052,
80.1413022880081));
#183309=CARTESIAN_POINT('Ctrl Pts',(8.69188026524415,-2.29595697558664,
80.35285890839));
#183310=CARTESIAN_POINT('Ctrl Pts',(8.15098066578445,3.77147322993531,80.5644155287719));
#183311=CARTESIAN_POINT('Ctrl Pts',(3.96634325089928,7.49324051377649,80.7759721491538));
#183312=CARTESIAN_POINT('Ctrl Pts',(-1.4642937957338,8.86105748869096,80.9875287695356));
#183313=CARTESIAN_POINT('Ctrl Pts',(-6.78588404143214,5.89677698029374,
81.1990853899178));
#183314=CARTESIAN_POINT('Ctrl Pts',(-8.46620824036368,0.524957807362146,
81.4106420102994));
#183315=CARTESIAN_POINT('Ctrl Pts',(-7.71101266496146,-3.56843978151961,
81.5693094755861));
#183316=CARTESIAN_POINT('Ctrl Pts',(-5.05474249081517,-6.83174341705231,
81.7279769408722));
#183317=CARTESIAN_POINT('Ctrl Pts',(-1.1776173489075,-8.40869440247311,
81.886644406159));
#183318=CARTESIAN_POINT('Ctrl Pts',(2.98354656363832,-7.95748639128541,
82.0453118714451));
#183319=CARTESIAN_POINT('Ctrl Pts',(6.43407764291852,-5.54942552688341,
82.2039793367317));
#183320=CARTESIAN_POINT('Ctrl Pts',(8.2847052562792,-1.82096718402392,82.3626468020181));
#183321=CARTESIAN_POINT('Ctrl Pts',(8.14470429910349,3.80578413198247,82.5742034224));
#183322=CARTESIAN_POINT('Ctrl Pts',(3.84215607714871,8.1179019960172,82.785760042782));
#183323=CARTESIAN_POINT('Ctrl Pts',(-1.75530226663762,8.29454315402551,
82.9973166631638));
#183324=CARTESIAN_POINT('Ctrl Pts',(-6.80134439667575,5.8655102536708,83.2088732835457));
#183325=CARTESIAN_POINT('Ctrl Pts',(-8.98820151561447,0.180095790597725,
83.4204299039276));
#183326=CARTESIAN_POINT('Ctrl Pts',(-6.83679903838358,-5.02100005750552,
83.6319865243096));
#183327=CARTESIAN_POINT('Ctrl Pts',(-3.63442053097905,-7.68013451689011,
83.790653989596));
#183328=CARTESIAN_POINT('Ctrl Pts',(0.495810896822684,-8.48394432557652,
83.9493214548824));
#183329=CARTESIAN_POINT('Ctrl Pts',(4.48303139945561,-7.21078037705518,
84.1079889201689));
#183330=CARTESIAN_POINT('Ctrl Pts',(7.38895437482808,-4.19839171726494,
84.2666563854553));
#183331=CARTESIAN_POINT('Ctrl Pts',(8.49554099952146,-0.138787315627807,
84.4253238507417));
#183332=CARTESIAN_POINT('Ctrl Pts',(7.52775657013251,3.9096219369063,84.5839913160281));
#183333=CARTESIAN_POINT('Ctrl Pts',(3.81535493093217,8.14022528742885,84.7955479364101));
#183334=CARTESIAN_POINT('Ctrl Pts',(-2.25085858000059,8.69460360171458,
85.0071045567919));
#183335=CARTESIAN_POINT('Ctrl Pts',(-6.66183439250307,5.24409140920695,
85.2186611771738));
#183336=CARTESIAN_POINT('Ctrl Pts',(-8.98004044839375,0.146183731388637,
85.4302177975557));
#183337=CARTESIAN_POINT('Ctrl Pts',(-7.01664901784579,-5.62021685875639,
85.6417744179377));
#183338=CARTESIAN_POINT('Ctrl Pts',(-2.03257114091683,-8.2353456045162,
85.8533310383195));
#183339=CARTESIAN_POINT('Ctrl Pts',(2.12989508064693,-8.22538909346939,
86.0119985036061));
#183340=CARTESIAN_POINT('Ctrl Pts',(5.81612353936555,-6.19643823012284,
86.1706659688923));
#183341=CARTESIAN_POINT('Ctrl Pts',(8.06188546297556,-2.66438115826029,
86.3293334341789));
#183342=CARTESIAN_POINT('Ctrl Pts',(8.36313795994383,1.51031891593676,86.4880008994653));
#183343=CARTESIAN_POINT('Ctrl Pts',(6.6119121803671,5.33629985220495,86.6466683647516));
#183344=CARTESIAN_POINT('Ctrl Pts',(3.27512779162817,7.82469172665717,86.8053358300382));
#183345=CARTESIAN_POINT('Ctrl Pts',(-2.28573880132459,8.69457296888152,
87.0168924504199));
#183346=CARTESIAN_POINT('Ctrl Pts',(-7.29863732183906,5.2337739139524,87.2284490708019));
#183347=CARTESIAN_POINT('Ctrl Pts',(-8.47479652211573,-0.241570051930617,
87.440005691184));
#183348=CARTESIAN_POINT('Ctrl Pts',(-6.98865630004681,-5.64102643655628,
87.6515623115655));
#183349=CARTESIAN_POINT('Ctrl Pts',(-1.78676051276461,-8.81065762863984,
87.8631189319479));
#183350=CARTESIAN_POINT('Ctrl Pts',(3.71552607636741,-7.62542645656924,
88.0746755523293));
#183351=CARTESIAN_POINT('Ctrl Pts',(6.90514685062736,-4.9510025009891,88.2333430176163));
#183352=CARTESIAN_POINT('Ctrl Pts',(8.43559070665481,-1.03147912954588,
88.3920104829023));
#183353=CARTESIAN_POINT('Ctrl Pts',(7.89702488093872,3.11928232201967,88.5506779481889));
#183354=CARTESIAN_POINT('Ctrl Pts',(5.45371364623198,6.51767958937793,88.7093454134752));
#183355=CARTESIAN_POINT('Ctrl Pts',(1.6578958472177,8.33335827582775,88.8680128787618));
#183356=CARTESIAN_POINT('Ctrl Pts',(-2.49837894227512,8.10619302320815,
89.026680344048));
#183357=CARTESIAN_POINT('Ctrl Pts',(-7.32539921680512,5.21140358190732,
89.2382369644301));
#183358=CARTESIAN_POINT('Ctrl Pts',(-8.95713255675292,-0.657474333237619,
89.4497935848118));
#183359=CARTESIAN_POINT('Ctrl Pts',(-6.35229963241242,-5.61505312185985,
89.661350205194));
#183360=CARTESIAN_POINT('Ctrl Pts',(-1.75193518140865,-8.8087013377826,
89.8729068255757));
#183361=CARTESIAN_POINT('Ctrl Pts',(4.27284971566023,-7.90967485339745,
90.0844634459577));
#183362=CARTESIAN_POINT('Ctrl Pts',(7.73823666394516,-3.4744720464393,90.2960200663396));
#183363=CARTESIAN_POINT('Ctrl Pts',(8.47384110833154,0.622491497353808,
90.4546875316259));
#183364=CARTESIAN_POINT('Ctrl Pts',(7.13780494130685,4.61247009581071,90.6133549969124));
#183365=CARTESIAN_POINT('Ctrl Pts',(4.06500630727874,7.45443813418621,90.772022462199));
#183366=CARTESIAN_POINT('Ctrl Pts',(0.0117368987456195,8.4984117345598,
90.9306899274851));
#183367=CARTESIAN_POINT('Ctrl Pts',(-4.06600105450924,7.46063765493643,
91.0893573927718));
#183368=CARTESIAN_POINT('Ctrl Pts',(-7.11170821157464,4.62340447961477,
91.2480248580581));
#183369=CARTESIAN_POINT('Ctrl Pts',(-8.96334864812165,-0.691796206529803,
91.45958147844));
#183370=CARTESIAN_POINT('Ctrl Pts',(-6.45618537723826,-6.24340984660604,
91.671138098822));
#183371=CARTESIAN_POINT('Ctrl Pts',(-1.27997205161572,-8.38106220764725,
91.8826947192038));
#183372=CARTESIAN_POINT('Ctrl Pts',(4.29833574849777,-7.88586114075367,
92.0942513395859));
#183373=CARTESIAN_POINT('Ctrl Pts',(8.34826776812752,-3.335659792342,92.3058079599677));
#183374=CARTESIAN_POINT('Ctrl Pts',(8.1675260770041,2.28993022844238,92.5173645803496));
#183375=CARTESIAN_POINT('Ctrl Pts',(6.10752001411662,5.90691781461061,92.6760320456359));
#183376=CARTESIAN_POINT('Ctrl Pts',(2.52542173879755,8.11451691780934,92.8346995109225));
#183377=CARTESIAN_POINT('Ctrl Pts',(-1.65468776361244,8.32796088946025,
92.9933669762088));
#183378=CARTESIAN_POINT('Ctrl Pts',(-5.43569013627816,6.53271861524583,
93.1520344414954));
#183379=CARTESIAN_POINT('Ctrl Pts',(-7.9017605278901,3.12340509203412,93.3107019067816));
#183380=CARTESIAN_POINT('Ctrl Pts',(-8.4225586341559,-1.0063640885058,93.4693693720683));
#183381=CARTESIAN_POINT('Ctrl Pts',(-6.43896909112289,-6.27374514475321,
93.6809259924499));
#183382=CARTESIAN_POINT('Ctrl Pts',(-0.957165855123717,-8.93008003956348,
93.892482612832));
#183383=CARTESIAN_POINT('Ctrl Pts',(4.38673882053551,-7.255139882753,94.1040392332139));
#183384=CARTESIAN_POINT('Ctrl Pts',(8.35257953053373,-3.30104706023637,
94.3155958535957));
#183385=CARTESIAN_POINT('Ctrl Pts',(8.54698316275725,2.78734255347677,94.5271524739777));
#183386=CARTESIAN_POINT('Ctrl Pts',(4.80404436667829,6.99095285739496,94.7387090943597));
#183387=CARTESIAN_POINT('Ctrl Pts',(0.905036893913656,8.44833621775569,
94.8973765596459));
#183388=CARTESIAN_POINT('Ctrl Pts',(-3.259696538621,7.84840873135576,95.0560440249325));
#183389=CARTESIAN_POINT('Ctrl Pts',(-6.60599159996829,5.3342105846383,95.2147114902188));
#183390=CARTESIAN_POINT('Ctrl Pts',(-8.35893323994751,1.53341403979869,
95.3733789555053));
#183391=CARTESIAN_POINT('Ctrl Pts',(-8.06816498394215,-2.66425108675267,
95.5320464207917));
#183392=CARTESIAN_POINT('Ctrl Pts',(-5.82220414294444,-6.16880266698849,
95.6907138860781));
#183393=CARTESIAN_POINT('Ctrl Pts',(-0.924520356739141,-8.94234775723183,
95.9022705064601));
#183394=CARTESIAN_POINT('Ctrl Pts',(4.98635084039052,-7.46985905065529,
96.113827126842));
#183395=CARTESIAN_POINT('Ctrl Pts',(8.01635169065955,-2.76014623326642,
96.3253837472238));
#183396=CARTESIAN_POINT('Ctrl Pts',(8.52816518653268,2.81671375682173,96.5369403676058));
#183397=CARTESIAN_POINT('Ctrl Pts',(4.77662445525099,7.61591549636984,96.7484969879877));
#183398=CARTESIAN_POINT('Ctrl Pts',(-0.790185932557508,8.44565266194666,
96.9600536083696));
#183399=CARTESIAN_POINT('Ctrl Pts',(-4.71796379787996,7.06641305365506,
97.118721073656));
#183400=CARTESIAN_POINT('Ctrl Pts',(-7.5306283820057,3.93804937156272,97.2773885389424));
#183401=CARTESIAN_POINT('Ctrl Pts',(-8.49055988674188,-0.137227805231727,
97.4360560042289));
#183402=CARTESIAN_POINT('Ctrl Pts',(-7.39881793188242,-4.17677760456979,
97.5947234695152));
#183403=CARTESIAN_POINT('Ctrl Pts',(-4.49111326487404,-7.21691544666963,
97.7533909348017));
#183404=CARTESIAN_POINT('Ctrl Pts',(-0.512538772771953,-8.46270402734996,
97.9120584000882));
#183405=CARTESIAN_POINT('Ctrl Pts',(5.0068590599844,-7.4668239237907,98.12361502047));
#183406=CARTESIAN_POINT('Ctrl Pts',(9.54195894481759,-1.29323553776124,
98.3880607959474));
#183407=CARTESIAN_POINT('Ctrl Pts',(6.81343712599511,5.86535702163415,98.6525065714248));
#183408=CARTESIAN_POINT('Ctrl Pts',(1.75834181031916,8.29349105181592,98.8640631918067));
#183409=CARTESIAN_POINT('Ctrl Pts',(-2.40877456271746,8.15273538577312,
99.0227306570931));
#183410=CARTESIAN_POINT('Ctrl Pts',(-6.01967976731674,5.99363558096764,
99.1813981223796));
#183411=CARTESIAN_POINT('Ctrl Pts',(-8.14915213644516,2.39503477083037,
99.340065587666));
#183412=CARTESIAN_POINT('Ctrl Pts',(-8.304600130319,-1.79807814568109,99.4987486186825));
#183413=CARTESIAN_POINT('Ctrl Pts',(-7.05661567854373,-4.29650290335088,
99.6045424946037));
#183414=CARTESIAN_POINT('Ctrl Pts',(-6.1720159842572,-5.32232154063713,
99.6574472154292));
#183415=CARTESIAN_POINT('Ctrl Pts',(2.0091828425417,-7.50340179875822,-0.206423361386482));
#183416=CARTESIAN_POINT('Ctrl Pts',(3.2560570208879,-7.16952802062857,-0.153528389248873));
#183417=CARTESIAN_POINT('Ctrl Pts',(5.57898372095689,-5.87036363360852,
-0.0477442620157891));
#183418=CARTESIAN_POINT('Ctrl Pts',(7.70519809246894,-2.48345330685785,
0.110929020312771));
#183419=CARTESIAN_POINT('Ctrl Pts',(7.95736644885961,1.49394517220418,0.269596485599199));
#183420=CARTESIAN_POINT('Ctrl Pts',(6.27029174751694,5.13167437923139,0.428263950885628));
#183421=CARTESIAN_POINT('Ctrl Pts',(3.06251395397477,7.47745566527645,0.586931416172058));
#183422=CARTESIAN_POINT('Ctrl Pts',(-2.22263135598543,8.27544619949939,
0.79848803655396));
#183423=CARTESIAN_POINT('Ctrl Pts',(-8.21167961142144,4.09854069893237,
1.06293381203135));
#183424=CARTESIAN_POINT('Ctrl Pts',(-7.9494565368908,-3.19785807327113,
1.32737958750873));
#183425=CARTESIAN_POINT('Ctrl Pts',(-4.13483212757085,-6.94263763572355,
1.53893620789063));
#183426=CARTESIAN_POINT('Ctrl Pts',(-0.331984144492666,-8.09484453700046,
1.69760367317706));
#183427=CARTESIAN_POINT('Ctrl Pts',(3.58945996307169,-7.25896364686547,
1.85627113846349));
#183428=CARTESIAN_POINT('Ctrl Pts',(6.61610676689296,-4.66172205022977,
2.01493860374992));
#183429=CARTESIAN_POINT('Ctrl Pts',(8.04540311823364,-0.935991074654104,
2.17360606903635));
#183430=CARTESIAN_POINT('Ctrl Pts',(7.50709055642592,3.03731311691104,2.33227353432277));
#183431=CARTESIAN_POINT('Ctrl Pts',(5.15210277994162,6.23053426445669,2.49094099960921));
#183432=CARTESIAN_POINT('Ctrl Pts',(0.321019198565415,8.56233974321341,
2.70249761999111));
#183433=CARTESIAN_POINT('Ctrl Pts',(-5.20869192847317,6.79305464573205,
2.91405424037301));
#183434=CARTESIAN_POINT('Ctrl Pts',(-7.79637889262264,2.12455969260576,
3.12561086075492));
#183435=CARTESIAN_POINT('Ctrl Pts',(-7.93492590961988,-3.21124827819366,
3.33716748113683));
#183436=CARTESIAN_POINT('Ctrl Pts',(-4.06747156186517,-7.54149967621007,
3.54872410151873));
#183437=CARTESIAN_POINT('Ctrl Pts',(1.27889791109489,-7.98291927192884,
3.76028072190064));
#183438=CARTESIAN_POINT('Ctrl Pts',(4.92802597814904,-6.42622521871537,
3.91894818718706));
#183439=CARTESIAN_POINT('Ctrl Pts',(7.40838574129789,-3.27483184280127,
4.07761565247349));
#183440=CARTESIAN_POINT('Ctrl Pts',(8.06566255913872,0.659938011782959,
4.23628311775992));
#183441=CARTESIAN_POINT('Ctrl Pts',(6.77751790413037,4.4355349111222,4.39495058304635));
#183442=CARTESIAN_POINT('Ctrl Pts',(3.81787759238652,7.14181922457694,4.55361804833277));
#183443=CARTESIAN_POINT('Ctrl Pts',(-0.035760713279578,8.08463795235184,
4.71228551361921));
#183444=CARTESIAN_POINT('Ctrl Pts',(-5.23927076131497,6.78000543459735,
4.9238421340011));
#183445=CARTESIAN_POINT('Ctrl Pts',(-8.35138480077202,1.87870792817531,
5.13539875438302));
#183446=CARTESIAN_POINT('Ctrl Pts',(-7.34733543235467,-3.36365117040484,
5.34695537476492));
#183447=CARTESIAN_POINT('Ctrl Pts',(-4.03517086503427,-7.54934216915915,
5.55851199514683));
#183448=CARTESIAN_POINT('Ctrl Pts',(1.70856436411669,-8.39638260750436,
5.77006861552873));
#183449=CARTESIAN_POINT('Ctrl Pts',(6.09639927703859,-5.31004370370416,
5.98162523591064));
#183450=CARTESIAN_POINT('Ctrl Pts',(7.9009131931023,-1.77689162408361,6.14029270119706));
#183451=CARTESIAN_POINT('Ctrl Pts',(7.78635900127687,2.23188959023923,6.2989601664835));
#183452=CARTESIAN_POINT('Ctrl Pts',(5.77012326512224,5.67416118083297,6.45762763176992));
#183453=CARTESIAN_POINT('Ctrl Pts',(2.36214621252141,7.74783730563748,6.61629509705636));
#183454=CARTESIAN_POINT('Ctrl Pts',(-1.64415034387486,7.92959915502436,
6.77496256234278));
#183455=CARTESIAN_POINT('Ctrl Pts',(-5.20706575041264,6.18458685704297,
6.93363002762921));
#183456=CARTESIAN_POINT('Ctrl Pts',(-8.36655083678149,1.84912413462387,
7.14518664801111));
#183457=CARTESIAN_POINT('Ctrl Pts',(-7.61594695241928,-3.90800758085578,
7.35674326839301));
#183458=CARTESIAN_POINT('Ctrl Pts',(-3.48638659873253,-7.28989681825855,
7.56829988877493));
#183459=CARTESIAN_POINT('Ctrl Pts',(1.73839828376926,-8.3817147792673,7.77985650915683));
#183460=CARTESIAN_POINT('Ctrl Pts',(6.69119414888973,-5.35222886581472,
7.99141312953873));
#183461=CARTESIAN_POINT('Ctrl Pts',(8.08290140003575,-0.171327983243689,
8.20296974992065));
#183462=CARTESIAN_POINT('Ctrl Pts',(7.20483765210341,3.69757860246291,8.36163721520705));
#183463=CARTESIAN_POINT('Ctrl Pts',(4.54856395562032,6.70218498570296,8.52030468049351));
#183464=CARTESIAN_POINT('Ctrl Pts',(0.795099983554925,8.05346159237329,
8.67897214577991));
#183465=CARTESIAN_POINT('Ctrl Pts',(-3.1501403937012,7.46226059186625,8.83763961106636));
#183466=CARTESIAN_POINT('Ctrl Pts',(-6.34268067388839,5.03509433711445,
8.99630707635277));
#183467=CARTESIAN_POINT('Ctrl Pts',(-7.9603547852174,1.41258628551333,9.15497454163922));
#183468=CARTESIAN_POINT('Ctrl Pts',(-7.60863814334965,-3.94043888084814,
9.36653116202111));
#183469=CARTESIAN_POINT('Ctrl Pts',(-3.34387587171949,-7.87995338746789,
9.57808778240303));
#183470=CARTESIAN_POINT('Ctrl Pts',(1.99354289033037,-7.83091781855655,
9.7896444027849));
#183471=CARTESIAN_POINT('Ctrl Pts',(6.70470377450696,-5.32185292264324,
10.0012010231668));
#183472=CARTESIAN_POINT('Ctrl Pts',(8.56662008808325,0.177350603561869,
10.2127576435487));
#183473=CARTESIAN_POINT('Ctrl Pts',(6.31592966174266,5.04694767443379,10.4243142639306));
#183474=CARTESIAN_POINT('Ctrl Pts',(3.16303655392699,7.45499650389469,10.5829817292171));
#183475=CARTESIAN_POINT('Ctrl Pts',(-0.801457265604823,8.06017269618677,
10.7416491945035));
#183476=CARTESIAN_POINT('Ctrl Pts',(-4.54914554329267,6.69295916838177,
10.9003166597899));
#183477=CARTESIAN_POINT('Ctrl Pts',(-7.1995897044865,3.71141829062658,11.0589841250764));
#183478=CARTESIAN_POINT('Ctrl Pts',(-8.09584708868326,-0.19756778892084,
11.2176515903628));
#183479=CARTESIAN_POINT('Ctrl Pts',(-7.01707718806656,-4.01537993934193,
11.3763190556492));
#183480=CARTESIAN_POINT('Ctrl Pts',(-3.31748621190696,-7.90017203635101,
11.5878756760311));
#183481=CARTESIAN_POINT('Ctrl Pts',(2.48099785437956,-8.19266872763073,
11.799432296413));
#183482=CARTESIAN_POINT('Ctrl Pts',(6.54772669008474,-4.73547910232167,
12.0109889167949));
#183483=CARTESIAN_POINT('Ctrl Pts',(8.55753192423801,0.209328927245312,
12.2225455371769));
#183484=CARTESIAN_POINT('Ctrl Pts',(6.46394670622404,5.62457340153279,12.4341021575587));
#183485=CARTESIAN_POINT('Ctrl Pts',(1.61601643183833,7.92156166501164,12.6456587779407));
#183486=CARTESIAN_POINT('Ctrl Pts',(-2.34759045671714,7.75052205739014,
12.8043262432271));
#183487=CARTESIAN_POINT('Ctrl Pts',(-5.77930409700375,5.67524112221684,
12.9629937085135));
#183488=CARTESIAN_POINT('Ctrl Pts',(-7.78089482178619,2.2244332707425,13.1216611737999));
#183489=CARTESIAN_POINT('Ctrl Pts',(-7.90575045796466,-1.7629030992477,
13.2803286390864));
#183490=CARTESIAN_POINT('Ctrl Pts',(-6.08952802662705,-5.33848494682565,
13.4389961043728));
#183491=CARTESIAN_POINT('Ctrl Pts',(-2.81526475330063,-7.57871576781822,
13.5976635696592));
#183492=CARTESIAN_POINT('Ctrl Pts',(2.51421374331843,-8.19128574907772,
13.8092201900411));
#183493=CARTESIAN_POINT('Ctrl Pts',(7.15376540808352,-4.70093732358155,
14.020776810423));
#183494=CARTESIAN_POINT('Ctrl Pts',(8.06132892646283,0.558983967522269,
14.2323334308049));
#183495=CARTESIAN_POINT('Ctrl Pts',(6.43648104260328,5.64330426455488,14.4438900511868));
#183496=CARTESIAN_POINT('Ctrl Pts',(1.35959684764904,8.45990126313526,14.6554466715687));
#183497=CARTESIAN_POINT('Ctrl Pts',(-3.83432973476785,7.11762346613171,
14.8670032919507));
#183498=CARTESIAN_POINT('Ctrl Pts',(-6.76806196776461,4.44692144242042,
15.0256707572371));
#183499=CARTESIAN_POINT('Ctrl Pts',(-8.07340337475109,0.654885936253715,
15.1843382225235));
#183500=CARTESIAN_POINT('Ctrl Pts',(-7.39941366756805,-3.27705736597523,
15.3430056878099));
#183501=CARTESIAN_POINT('Ctrl Pts',(-4.94070130533272,-6.4185814828846,
15.5016731530964));
#183502=CARTESIAN_POINT('Ctrl Pts',(-1.25540207466762,-8.00035866355257,
15.6603406183828));
#183503=CARTESIAN_POINT('Ctrl Pts',(2.69387807414514,-7.62270747452594,
15.8190080836692));
#183504=CARTESIAN_POINT('Ctrl Pts',(7.17838299420069,-4.67859493424099,
16.0305647040511));
#183505=CARTESIAN_POINT('Ctrl Pts',(8.50452392902259,0.973778195903384,
16.2421213244331));
#183506=CARTESIAN_POINT('Ctrl Pts',(5.83147495731057,5.59387048105627,16.4536779448149));
#183507=CARTESIAN_POINT('Ctrl Pts',(1.32650797202072,8.45668657538519,16.6652345651969));
#183508=CARTESIAN_POINT('Ctrl Pts',(-4.37611184800845,7.36668704804644,
16.8767911855787));
#183509=CARTESIAN_POINT('Ctrl Pts',(-7.50412016787103,3.00845954380391,
17.0883478059607));
#183510=CARTESIAN_POINT('Ctrl Pts',(-8.04563436084246,-0.921705400977682,
17.247015271247));
#183511=CARTESIAN_POINT('Ctrl Pts',(-6.61843941011529,-4.66958000419504,
17.4056827365335));
#183512=CARTESIAN_POINT('Ctrl Pts',(-3.58185128358946,-7.25677400681142,
17.5643502018199));
#183513=CARTESIAN_POINT('Ctrl Pts',(0.31867166534931,-8.09364973362753,
17.7230176671064));
#183514=CARTESIAN_POINT('Ctrl Pts',(4.16169756931217,-6.94708906349569,
17.8816851323928));
#183515=CARTESIAN_POINT('Ctrl Pts',(6.95205909546775,-4.12692653843969,
18.0403525976792));
#183516=CARTESIAN_POINT('Ctrl Pts',(8.50911149226834,1.00670481387645,18.2519092180611));
#183517=CARTESIAN_POINT('Ctrl Pts',(5.90601885240856,6.19629829407277,18.4634658384431));
#183518=CARTESIAN_POINT('Ctrl Pts',(0.893646742785605,8.03111963773931,
18.6750224588249));
#183519=CARTESIAN_POINT('Ctrl Pts',(-4.39945838513347,7.34301962081084,
18.8865790792069));
#183520=CARTESIAN_POINT('Ctrl Pts',(-8.07967631497109,2.85258893208078,
19.0981356995887));
#183521=CARTESIAN_POINT('Ctrl Pts',(-7.68920659426301,-2.4977490408958,
19.3096923199707));
#183522=CARTESIAN_POINT('Ctrl Pts',(-5.58703866671401,-5.86231797595484,
19.4683597852571));
#183523=CARTESIAN_POINT('Ctrl Pts',(-2.09005686812911,-7.82562329331867,
19.6270272505435));
#183524=CARTESIAN_POINT('Ctrl Pts',(1.89902288646746,-7.8666472960441,19.7856947158299));
#183525=CARTESIAN_POINT('Ctrl Pts',(5.43006240703896,-6.01025289789105,
19.9443621811164));
#183526=CARTESIAN_POINT('Ctrl Pts',(7.6462209924854,-2.66778515788588,20.1030296464028));
#183527=CARTESIAN_POINT('Ctrl Pts',(7.98189786707622,1.28528392198672,20.2616971116892));
#183528=CARTESIAN_POINT('Ctrl Pts',(5.88844605642552,6.22451893809486,20.4732537320711));
#183529=CARTESIAN_POINT('Ctrl Pts',(0.564923425653677,8.54143036951552,
20.684810352453));
#183530=CARTESIAN_POINT('Ctrl Pts',(-4.4591660822607,6.73894093959792,20.8963669728349));
#183531=CARTESIAN_POINT('Ctrl Pts',(-8.082439033227,2.8194592581385,21.1079235932168));
#183532=CARTESIAN_POINT('Ctrl Pts',(-8.03126456115619,-2.98617188367512,
21.3194802135988));
#183533=CARTESIAN_POINT('Ctrl Pts',(-4.30364004228442,-6.84407266961708,
21.5310368339806));
#183534=CARTESIAN_POINT('Ctrl Pts',(-0.533978119676184,-8.08063366836214,
21.6897042992671));
#183535=CARTESIAN_POINT('Ctrl Pts',(3.4088897612777,-7.34766549567967,21.8483717645535));
#183536=CARTESIAN_POINT('Ctrl Pts',(6.49804381946639,-4.82346909640559,
22.00703922984));
#183537=CARTESIAN_POINT('Ctrl Pts',(8.01988369045738,-1.13586232989786,
22.1657066951263));
#183538=CARTESIAN_POINT('Ctrl Pts',(7.58005275125885,2.85036373164785,22.3243741604128));
#183539=CARTESIAN_POINT('Ctrl Pts',(5.30516600064393,6.1006443943378,22.4830416256992));
#183540=CARTESIAN_POINT('Ctrl Pts',(0.533350586535182,8.55184015998767,
22.6945982460811));
#183541=CARTESIAN_POINT('Ctrl Pts',(-5.03850667602932,6.92016052629867,
22.9061548664631));
#183542=CARTESIAN_POINT('Ctrl Pts',(-7.74126660981814,2.31738611635783,
23.1177114868449));
#183543=CARTESIAN_POINT('Ctrl Pts',(-8.01216053127736,-3.01337930821458,
23.3292681072269));
#183544=CARTESIAN_POINT('Ctrl Pts',(-4.25335765412606,-7.43823780449522,
23.5408247276087));
#183545=CARTESIAN_POINT('Ctrl Pts',(1.08041685410531,-8.01219993147444,
23.7523813479907));
#183546=CARTESIAN_POINT('Ctrl Pts',(4.76704696570923,-6.5465285717915,23.9110488132771));
#183547=CARTESIAN_POINT('Ctrl Pts',(7.3248431091507,-3.45765687529476,24.0697162785635));
#183548=CARTESIAN_POINT('Ctrl Pts',(8.07955452782502,0.459593554771575,
24.22838374385));
#183549=CARTESIAN_POINT('Ctrl Pts',(6.88549477943484,4.26599100834977,24.3870512091364));
#183550=CARTESIAN_POINT('Ctrl Pts',(3.99391953046181,7.04488324237925,24.5457186744228));
#183551=CARTESIAN_POINT('Ctrl Pts',(0.164863081889657,8.08303584581827,
24.7043861397092));
#183552=CARTESIAN_POINT('Ctrl Pts',(-5.06941801282327,6.90792544700635,
24.9159427600911));
#183553=CARTESIAN_POINT('Ctrl Pts',(-8.30219487472764,2.08536123877397,
25.127499380473));
#183554=CARTESIAN_POINT('Ctrl Pts',(-7.42853894049362,-3.18029815365528,
25.339056000855));
#183555=CARTESIAN_POINT('Ctrl Pts',(-4.22125825449852,-7.44688861088727,
25.5506126212369));
#183556=CARTESIAN_POINT('Ctrl Pts',(1.49968985936297,-8.43619364973677,
25.7621692416187));
#183557=CARTESIAN_POINT('Ctrl Pts',(5.96275831201656,-5.45968512215048,
25.9737258620007));
#183558=CARTESIAN_POINT('Ctrl Pts',(7.85438846261605,-1.97239828454699,
26.1323933272871));
#183559=CARTESIAN_POINT('Ctrl Pts',(7.83934371373296,2.03799111354809,26.2910607925735));
#183560=CARTESIAN_POINT('Ctrl Pts',(5.9091455699583,5.52923378387345,26.44972825786));
#183561=CARTESIAN_POINT('Ctrl Pts',(2.55367422961529,7.68683716296529,26.6083957231464));
#183562=CARTESIAN_POINT('Ctrl Pts',(-1.4468784716737,7.96795555978871,26.7670631884328));
#183563=CARTESIAN_POINT('Ctrl Pts',(-5.05199765166073,6.31189100414194,
26.9257306537192));
#183564=CARTESIAN_POINT('Ctrl Pts',(-8.31809034695746,2.05616291912584,
27.1372872741011));
#183565=CARTESIAN_POINT('Ctrl Pts',(-7.71057544278213,-3.71782161692833,
27.3488438944831));
#183566=CARTESIAN_POINT('Ctrl Pts',(-3.66620507739025,-7.20114070596396,
27.5604005148649));
#183567=CARTESIAN_POINT('Ctrl Pts',(1.52987856327207,-8.42227064488995,
27.7719571352469));
#183568=CARTESIAN_POINT('Ctrl Pts',(6.5563232503647,-5.51661657239854,27.9835137556287));
#183569=CARTESIAN_POINT('Ctrl Pts',(8.07616119803516,-0.371844892266704,
28.1950703760107));
#183570=CARTESIAN_POINT('Ctrl Pts',(7.29437113081824,3.51765872711467,28.353737841297));
#183571=CARTESIAN_POINT('Ctrl Pts',(4.71347185117461,6.58725289852531,28.5124053065836));
#183572=CARTESIAN_POINT('Ctrl Pts',(0.994694301570285,8.03125213463683,
28.6710727718699));
#183573=CARTESIAN_POINT('Ctrl Pts',(-2.96400137325586,7.53813063698705,
28.8297402371564));
#183574=CARTESIAN_POINT('Ctrl Pts',(-6.21578648608584,5.19093165760762,
28.9884077024428));
#183575=CARTESIAN_POINT('Ctrl Pts',(-7.92285164960296,1.60968011074781,
29.1470751677293));
#183576=CARTESIAN_POINT('Ctrl Pts',(-7.70407363670064,-3.75042429205407,
29.3586317881111));
#183577=CARTESIAN_POINT('Ctrl Pts',(-3.53837993550241,-7.79455185794337,
29.5701884084931));
#183578=CARTESIAN_POINT('Ctrl Pts',(1.79861211977617,-7.87797445915938,
29.7817450288749));
#183579=CARTESIAN_POINT('Ctrl Pts',(6.57058246686297,-5.48658521124823,
29.9933016492569));
#183580=CARTESIAN_POINT('Ctrl Pts',(8.56838307527957,-0.0352766976527707,
30.2048582696387));
#183581=CARTESIAN_POINT('Ctrl Pts',(6.43922018549342,4.88866972941389,30.4164148900207));
#183582=CARTESIAN_POINT('Ctrl Pts',(3.34705139215976,7.3742131846592,30.575082355307));
#183583=CARTESIAN_POINT('Ctrl Pts',(-0.601204811662946,8.07757825188831,
30.7337498205936));
#183584=CARTESIAN_POINT('Ctrl Pts',(-4.38166524394992,6.80378110271389,
30.8924172858799));
#183585=CARTESIAN_POINT('Ctrl Pts',(-7.10527744757138,3.88892659148757,
31.0510847511664));
#183586=CARTESIAN_POINT('Ctrl Pts',(-8.09825670521013,0.00338394435035205,
31.2097522164528));
#183587=CARTESIAN_POINT('Ctrl Pts',(-7.11455442523969,-3.84002130864605,
31.3684196817392));
#183588=CARTESIAN_POINT('Ctrl Pts',(-3.51250010842368,-7.81541911598213,
31.5799763021212));
#183589=CARTESIAN_POINT('Ctrl Pts',(2.27694047685335,-8.25170971974905,
31.791532922503));
#183590=CARTESIAN_POINT('Ctrl Pts',(6.42820403801672,-4.89649670501255,
32.003089542885));
#183591=CARTESIAN_POINT('Ctrl Pts',(8.56009122212236,-0.00308270630504298,
32.2146461632669));
#183592=CARTESIAN_POINT('Ctrl Pts',(6.60152489708165,5.46244469110179,32.4262027836487));
#183593=CARTESIAN_POINT('Ctrl Pts',(1.81208500248022,7.87902254498234,32.6377594040307));
#183594=CARTESIAN_POINT('Ctrl Pts',(-2.15454561498722,7.80638881349754,
32.796426869317));
#183595=CARTESIAN_POINT('Ctrl Pts',(-5.6366987363262,5.8169016664238,32.9550943346036));
#183596=CARTESIAN_POINT('Ctrl Pts',(-7.72330171866522,2.41682398327808,
33.1137617998899));
#183597=CARTESIAN_POINT('Ctrl Pts',(-7.94706094494807,-1.56618644427357,
33.2724292651764));
#183598=CARTESIAN_POINT('Ctrl Pts',(-6.22012248880763,-5.18573517823562,
33.4310967304628));
#183599=CARTESIAN_POINT('Ctrl Pts',(-3.00245665437853,-7.50652398644883,
33.5897641957493));
#183600=CARTESIAN_POINT('Ctrl Pts',(2.31018045539937,-8.25115138835942,
33.8013208161311));
#183601=CARTESIAN_POINT('Ctrl Pts',(7.03491326880379,-4.87700384811648,
34.0128774365131));
#183602=CARTESIAN_POINT('Ctrl Pts',(8.07271737727317,0.358777484306035,
34.2244340568949));
#183603=CARTESIAN_POINT('Ctrl Pts',(6.57453247949466,5.48185132142458,34.4359906772769));
#183604=CARTESIAN_POINT('Ctrl Pts',(1.56910276939402,8.42355919248004,34.6475472976587));
#183605=CARTESIAN_POINT('Ctrl Pts',(-3.65653189023152,7.21057715139873,
34.8591039180407));
#183606=CARTESIAN_POINT('Ctrl Pts',(-6.65563176020345,4.61349531127234,
35.0177713833271));
#183607=CARTESIAN_POINT('Ctrl Pts',(-8.05466705749516,0.855018265212991,
35.1764388486135));
#183608=CARTESIAN_POINT('Ctrl Pts',(-7.4784523906474,-3.09243875355764,
35.3351063139));
#183609=CARTESIAN_POINT('Ctrl Pts',(-5.09845109881096,-6.29400619907375,
35.4937737791864));
#183610=CARTESIAN_POINT('Ctrl Pts',(-1.45353695844748,-7.96674358976034,
35.6524412444728));
#183611=CARTESIAN_POINT('Ctrl Pts',(2.50389820451343,-7.68720639127034,
35.8111087097592));
#183612=CARTESIAN_POINT('Ctrl Pts',(7.06007768032758,-4.85527920081592,
36.0226653301412));
#183613=CARTESIAN_POINT('Ctrl Pts',(8.52606864495294,0.762446519885064,
36.234221950523));
#183614=CARTESIAN_POINT('Ctrl Pts',(5.96848603223279,5.44744542144437,36.445778570905));
#183615=CARTESIAN_POINT('Ctrl Pts',(1.53594431289278,8.42116656418975,36.6573351912868));
#183616=CARTESIAN_POINT('Ctrl Pts',(-4.19196689926189,7.47300786066947,
36.8688918116688));
#183617=CARTESIAN_POINT('Ctrl Pts',(-7.42715740707066,3.19374093676189,
37.0804484320506));
#183618=CARTESIAN_POINT('Ctrl Pts',(-8.06602823852491,-0.721776675903932,
37.2391158973371));
#183619=CARTESIAN_POINT('Ctrl Pts',(-6.73227275918578,-4.50391175944539,
37.3977833626235));
#183620=CARTESIAN_POINT('Ctrl Pts',(-3.76081845541284,-7.16565922641535,
37.5564508279099));
#183621=CARTESIAN_POINT('Ctrl Pts',(0.11773716752723,-8.09906510656189,
37.7151182931964));
#183622=CARTESIAN_POINT('Ctrl Pts',(3.98803057509151,-7.04821858675621,
37.8737857584828));
#183623=CARTESIAN_POINT('Ctrl Pts',(6.8475126074327,-4.29816465617636,38.0324532237692));
#183624=CARTESIAN_POINT('Ctrl Pts',(8.53147183894502,0.795249163107236,
38.2440098441512));
#183625=CARTESIAN_POINT('Ctrl Pts',(6.05795565866709,6.04783799979448,38.455566464533));
#183626=CARTESIAN_POINT('Ctrl Pts',(1.09265632186101,8.0064717134872,38.667123084915));
#183627=CARTESIAN_POINT('Ctrl Pts',(-4.21589353275059,7.44992704357874,
38.8786797052968));
#183628=CARTESIAN_POINT('Ctrl Pts',(-8.00640411493513,3.05220020943656,
39.0902363256788));
#183629=CARTESIAN_POINT('Ctrl Pts',(-7.7488182757015,-2.30617944893889,
39.3017929460607));
#183630=CARTESIAN_POINT('Ctrl Pts',(-5.73078628192673,-5.72187571565837,
39.4604604113471));
#183631=CARTESIAN_POINT('Ctrl Pts',(-2.28359885268831,-7.77135084273937,
39.6191278766335));
#183632=CARTESIAN_POINT('Ctrl Pts',(1.70323462649298,-7.91134750916685,
39.7777953419201));
#183633=CARTESIAN_POINT('Ctrl Pts',(5.27925157867091,-6.14314417949359,
39.9364628072063));
#183634=CARTESIAN_POINT('Ctrl Pts',(7.57766799383721,-2.85669754957289,
40.0951302724929));
#183635=CARTESIAN_POINT('Ctrl Pts',(8.01133323235648,1.08682480680852,40.2537977377792));
#183636=CARTESIAN_POINT('Ctrl Pts',(6.04108854261124,6.07648600676953,40.4653543581612));
#183637=CARTESIAN_POINT('Ctrl Pts',(0.776697109145226,8.52478227491935,
40.6769109785431));
#183638=CARTESIAN_POINT('Ctrl Pts',(-4.29057249427801,6.84751595893862,
40.8884675989249));
#183639=CARTESIAN_POINT('Ctrl Pts',(-8.0099880644816,3.01914929094193,41.1000242193069));
#183640=CARTESIAN_POINT('Ctrl Pts',(-8.1028906748984,-2.78596404872365,
41.3115808396888));
#183641=CARTESIAN_POINT('Ctrl Pts',(-4.47214416453986,-6.73517445149922,
41.5231374600707));
#183642=CARTESIAN_POINT('Ctrl Pts',(-0.734327091130077,-8.06489533954312,
41.681804925357));
#183643=CARTESIAN_POINT('Ctrl Pts',(3.22551463815378,-7.42999145087132,
41.8404723906437));
#183644=CARTESIAN_POINT('Ctrl Pts',(6.3763530758844,-4.98322677141116,41.9991398559298));
#183645=CARTESIAN_POINT('Ctrl Pts',(7.98922887192849,-1.33451851727022,
42.1578073212165));
#183646=CARTESIAN_POINT('Ctrl Pts',(7.64844784780906,2.66139411472179,42.3164747865027));
#183647=CARTESIAN_POINT('Ctrl Pts',(5.45491425699232,5.96712315687812,42.4751422517893));
#183648=CARTESIAN_POINT('Ctrl Pts',(0.745392301050544,8.53597231064671,
42.686698872171));
#183649=CARTESIAN_POINT('Ctrl Pts',(-4.86523790443101,7.04305554190294,
42.8982554925532));
#183650=CARTESIAN_POINT('Ctrl Pts',(-7.68137917069536,2.50876487011254,
43.1098121129349));
#183651=CARTESIAN_POINT('Ctrl Pts',(-8.0844676542436,-2.81363714450263,
43.3213687333169));
#183652=CARTESIAN_POINT('Ctrl Pts',(-4.43662091331696,-7.33040434346995,
43.5329253536988));
#183653=CARTESIAN_POINT('Ctrl Pts',(0.881268903615611,-8.03654238132135,
43.7444819740807));
#183654=CARTESIAN_POINT('Ctrl Pts',(4.60313310919397,-6.66280261436008,
43.9031494393671));
#183655=CARTESIAN_POINT('Ctrl Pts',(7.23678913863202,-3.63835136153705,
44.0618169046536));
#183656=CARTESIAN_POINT('Ctrl Pts',(8.08847108433317,0.25896542723205,44.2204843699399));
#183657=CARTESIAN_POINT('Ctrl Pts',(6.98923121663487,4.09382029945987,44.3791518352265));
#183658=CARTESIAN_POINT('Ctrl Pts',(4.16750194123697,6.94360862792613,44.5378193005128));
#183659=CARTESIAN_POINT('Ctrl Pts',(0.365385329643911,8.0764560037248,44.6964867657992));
#183660=CARTESIAN_POINT('Ctrl Pts',(-4.89644335222612,7.03159130944993,
44.9080433861812));
#183661=CARTESIAN_POINT('Ctrl Pts',(-8.24789214596878,2.29073026570201,
45.119600006563));
#183662=CARTESIAN_POINT('Ctrl Pts',(-7.50516776655695,-2.99498652073261,
45.331156626945));
#183663=CARTESIAN_POINT('Ctrl Pts',(-4.40474590883526,-7.33984924479369,
45.5427132473268));
#183664=CARTESIAN_POINT('Ctrl Pts',(1.28989149763967,-8.47080892925094,
45.7542698677089));
#183665=CARTESIAN_POINT('Ctrl Pts',(5.82544565561335,-5.60596488249478,
45.9658264880906));
#183666=CARTESIAN_POINT('Ctrl Pts',(7.80302595916402,-2.1666890188074,46.1244939533772));
#183667=CARTESIAN_POINT('Ctrl Pts',(7.88750222646596,1.84283512310428,46.2831614186634));
#183668=CARTESIAN_POINT('Ctrl Pts',(6.04452592653096,5.3809059710111,46.4418288839501));
#183669=CARTESIAN_POINT('Ctrl Pts',(2.7436350891584,7.62109440424651,46.6004963492363));
#183670=CARTESIAN_POINT('Ctrl Pts',(-1.24872578950165,8.00142147857247,
46.7591638145229));
#183671=CARTESIAN_POINT('Ctrl Pts',(-4.89380008924511,6.43527869080786,
46.9178312798092));
#183672=CARTESIAN_POINT('Ctrl Pts',(-8.2645486264883,2.26200189733122,47.1293879001912));
#183673=CARTESIAN_POINT('Ctrl Pts',(-7.80037642979242,-3.52547325528354,
47.3409445205731));
#183674=CARTESIAN_POINT('Ctrl Pts',(-3.84385887026274,-7.10780021600436,
47.5525011409549));
#183675=CARTESIAN_POINT('Ctrl Pts',(1.32064680707816,-8.4580098257796,47.7640577613369));
#183676=CARTESIAN_POINT('Ctrl Pts',(6.41695377006199,-5.67686569600247,
47.9756143817187));
#183677=CARTESIAN_POINT('Ctrl Pts',(8.06501639081381,-0.573047720393685,
48.1871710021008));
#183678=CARTESIAN_POINT('Ctrl Pts',(7.37821331433221,3.33750110294794,48.345838467387));
#183679=CARTESIAN_POINT('Ctrl Pts',(4.87780582617054,6.46451731396927,48.5045059326737));
#183680=CARTESIAN_POINT('Ctrl Pts',(1.18928799120203,8.01117052161392,48.6631733979599));
#183681=CARTESIAN_POINT('Ctrl Pts',(-2.7681121532524,7.5964713334689,48.8218408632464));
#183682=CARTESIAN_POINT('Ctrl Pts',(-7.20680219784448,4.6198565020302,49.0333974836283));
#183683=CARTESIAN_POINT('Ctrl Pts',(-8.84300034502869,-2.47886897833852,
49.2978432591057));
#183684=CARTESIAN_POINT('Ctrl Pts',(-2.6901361923085,-8.78327356646699,
49.6151781896785));
#183685=CARTESIAN_POINT('Ctrl Pts',(4.44903321313057,-7.31233051837037,
49.8796239651559));
#183686=CARTESIAN_POINT('Ctrl Pts',(7.52616743441877,-2.95099595536838,
50.0911805855378));
#183687=CARTESIAN_POINT('Ctrl Pts',(8.0420005338647,1.00473307760414,50.2498480508243));
#183688=CARTESIAN_POINT('Ctrl Pts',(6.56967689983475,4.71083444441478,50.4085155161107));
#183689=CARTESIAN_POINT('Ctrl Pts',(2.51247932687687,8.18312691894298,50.6200721364926));
#183690=CARTESIAN_POINT('Ctrl Pts',(-4.76488672051435,7.84957633027501,
50.8845179119699));
#183691=CARTESIAN_POINT('Ctrl Pts',(-9.18623881118053,0.231498139607691,
51.201852842543));
#183692=CARTESIAN_POINT('Ctrl Pts',(-5.84035172354906,-6.25684744528986,
51.4662986180201));
#183693=CARTESIAN_POINT('Ctrl Pts',(-0.82645652908081,-8.03540205221921,
51.6778552384022));
#183694=CARTESIAN_POINT('Ctrl Pts',(4.46831792482671,-7.30642728360933,
51.8894118587839));
#183695=CARTESIAN_POINT('Ctrl Pts',(8.10281394002393,-2.77908238451519,
52.100968479166));
#183696=CARTESIAN_POINT('Ctrl Pts',(7.66752709745631,2.56541977891761,52.3125250995478));
#183697=CARTESIAN_POINT('Ctrl Pts',(5.53416939644934,5.9121753980673,52.4711925648344));
#183698=CARTESIAN_POINT('Ctrl Pts',(2.02058714401458,7.84371592872507,52.6298600301206));
#183699=CARTESIAN_POINT('Ctrl Pts',(-1.9690910382543,7.84954043858405,52.7885274954072));
#183700=CARTESIAN_POINT('Ctrl Pts',(-5.48326334033245,5.96163601576004,
52.9471949606936));
#183701=CARTESIAN_POINT('Ctrl Pts',(-7.66969627022757,2.59966159008363,
53.10586242598));
#183702=CARTESIAN_POINT('Ctrl Pts',(-7.97012628075206,-1.35627990505007,
53.2645298912664));
#183703=CARTESIAN_POINT('Ctrl Pts',(-5.83283293269671,-6.27666477010184,
53.4760865116484));
#183704=CARTESIAN_POINT('Ctrl Pts',(-0.488881099089476,-8.5461249856449,
53.6876431320301));
#183705=CARTESIAN_POINT('Ctrl Pts',(4.51895866787966,-6.69898833214349,
53.8991997524122));
#183706=CARTESIAN_POINT('Ctrl Pts',(8.10721265766993,-2.74742124273045,
54.1107563727939));
#183707=CARTESIAN_POINT('Ctrl Pts',(8.00437035992183,3.05752741482916,54.322312993176));
#183708=CARTESIAN_POINT('Ctrl Pts',(4.24256256977924,6.8821006942729,54.5338696135578));
#183709=CARTESIAN_POINT('Ctrl Pts',(0.462044501231383,8.08506596133534,
54.6925370788443));
#183710=CARTESIAN_POINT('Ctrl Pts',(-3.47414384450845,7.31703759316164,
54.8512045441307));
#183711=CARTESIAN_POINT('Ctrl Pts',(-6.54071219188587,4.76544997203763,
55.0098720094171));
#183712=CARTESIAN_POINT('Ctrl Pts',(-8.02967446321915,1.06444578645232,
55.1685394747036));
#183713=CARTESIAN_POINT('Ctrl Pts',(-7.5543863021864,-2.91770816998886,
55.3272069399899));
#183714=CARTESIAN_POINT('Ctrl Pts',(-5.25066430696669,-6.14761519979205,
55.4858744052765));
#183715=CARTESIAN_POINT('Ctrl Pts',(-0.457223895574364,-8.55624796078953,
55.6974310256582));
#183716=CARTESIAN_POINT('Ctrl Pts',(5.09989189407407,-6.8750471997139,55.9089876460403));
#183717=CARTESIAN_POINT('Ctrl Pts',(7.76158322107178,-2.24840232248137,
56.1205442664221));
#183718=CARTESIAN_POINT('Ctrl Pts',(7.98502622041197,3.08456277470767,56.332100886804));
#183719=CARTESIAN_POINT('Ctrl Pts',(4.18699394779361,7.47579525227161,56.5436575071859));
#183720=CARTESIAN_POINT('Ctrl Pts',(-1.15167721691652,8.00226767255704,
56.7552141275679));
#183721=CARTESIAN_POINT('Ctrl Pts',(-4.8251178580258,6.50384584493907,56.9138815928542));
#183722=CARTESIAN_POINT('Ctrl Pts',(-7.35532384910833,3.39233381516429,
57.0725490581407));
#183723=CARTESIAN_POINT('Ctrl Pts',(-8.07514450849003,-0.531477912593235,
57.2312165234271));
#183724=CARTESIAN_POINT('Ctrl Pts',(-6.84725768774057,-4.32709831161835,
57.3898839887136));
#183725=CARTESIAN_POINT('Ctrl Pts',(-3.93106668757571,-7.08014744283938,
57.5485514539999));
#183726=CARTESIAN_POINT('Ctrl Pts',(-0.0929230143189289,-8.08418292927951,
57.7072189192864));
#183727=CARTESIAN_POINT('Ctrl Pts',(5.1306931182878,-6.86253751144311,57.9187755396683));
#183728=CARTESIAN_POINT('Ctrl Pts',(8.32042441111236,-2.01139475318977,
58.1303321600502));
#183729=CARTESIAN_POINT('Ctrl Pts',(7.39994227476214,3.24628117493691,58.3418887804322));
#183730=CARTESIAN_POINT('Ctrl Pts',(4.1548188338062,7.48416005256301,58.5534454008139));
#183731=CARTESIAN_POINT('Ctrl Pts',(-1.57470687607251,8.42251335556041,
58.765002021196));
#183732=CARTESIAN_POINT('Ctrl Pts',(-6.01110968439643,5.40640441353625,
58.9765586415778));
#183733=CARTESIAN_POINT('Ctrl Pts',(-7.87163043831221,1.90242144573692,
59.1352261068644));
#183734=CARTESIAN_POINT('Ctrl Pts',(-7.82089653845082,-2.10767525387386,
59.2938935721506));
#183735=CARTESIAN_POINT('Ctrl Pts',(-5.85970513720944,-5.58160221698454,
59.4525610374372));
#183736=CARTESIAN_POINT('Ctrl Pts',(-2.48516546539594,-7.70925873547831,
59.6112285027235));
#183737=CARTESIAN_POINT('Ctrl Pts',(1.51773057814824,-7.9547637932697,59.7698959680101));
#183738=CARTESIAN_POINT('Ctrl Pts',(5.10796914452118,-6.26668170080252,
59.9285634332964));
#183739=CARTESIAN_POINT('Ctrl Pts',(8.33605940863296,-1.98205613085918,
60.1401200536783));
#183740=CARTESIAN_POINT('Ctrl Pts',(7.67718401407479,3.78629328607396,60.3516766740603));
#183741=CARTESIAN_POINT('Ctrl Pts',(3.60197462640998,7.23348228222562,60.5632332944421));
#183742=CARTESIAN_POINT('Ctrl Pts',(-1.60477047921222,8.40832224306274,
60.7747899148241));
#183743=CARTESIAN_POINT('Ctrl Pts',(-6.60515776903126,5.45805128377708,
60.9863465352058));
#183744=CARTESIAN_POINT('Ctrl Pts',(-8.0791505515113,0.299957807979901,
61.1979031555879));
#183745=CARTESIAN_POINT('Ctrl Pts',(-7.26277749771403,-3.58243438645558,
61.3565706208743));
#183746=CARTESIAN_POINT('Ctrl Pts',(-4.65466311398428,-6.62893874886922,
61.5152380861607));
#183747=CARTESIAN_POINT('Ctrl Pts',(-0.923182212819831,-8.03978620397445,
61.6739055514471));
#183748=CARTESIAN_POINT('Ctrl Pts',(3.03096825163476,-7.51145452615722,
61.8325730167336));
#183749=CARTESIAN_POINT('Ctrl Pts',(6.26173611498402,-5.1354098123582,61.9912404820199));
#183750=CARTESIAN_POINT('Ctrl Pts',(7.93686296833665,-1.53910835953809,
62.1499079473065));
#183751=CARTESIAN_POINT('Ctrl Pts',(7.67039232375798,3.81883680847582,62.3614645676883));
#183752=CARTESIAN_POINT('Ctrl Pts',(3.46887358942421,7.82573237816946,62.5730211880701));
#183753=CARTESIAN_POINT('Ctrl Pts',(-1.86864952689433,7.86165606486387,
62.7845778084522));
#183754=CARTESIAN_POINT('Ctrl Pts',(-6.61914916211397,5.42789421450165,
62.996134428834));
#183755=CARTESIAN_POINT('Ctrl Pts',(-8.56835770814106,-0.0409774996166555,
63.207691049216));
#183756=CARTESIAN_POINT('Ctrl Pts',(-6.39545934772782,-4.94578083340884,
63.4192476695978));
#183757=CARTESIAN_POINT('Ctrl Pts',(-3.28129335186214,-7.40370765586983,
63.5779151348843));
#183758=CARTESIAN_POINT('Ctrl Pts',(0.673065974242905,-8.07190806657644,
63.7365826001707));
#183759=CARTESIAN_POINT('Ctrl Pts',(4.44204077020023,-6.76451782461722,
63.8952500654571));
#183760=CARTESIAN_POINT('Ctrl Pts',(7.13960489047256,-3.82554043879892,
64.0539175307436));
#183761=CARTESIAN_POINT('Ctrl Pts',(8.09796613107626,0.0686851840087504,
64.21258499603));
#183762=CARTESIAN_POINT('Ctrl Pts',(7.08009910440649,3.90318395573866,64.3712524613163));
#183763=CARTESIAN_POINT('Ctrl Pts',(3.44280908273089,7.84636849695452,64.5828090816984));
#183764=CARTESIAN_POINT('Ctrl Pts',(-2.35028493272838,8.23111972754161,
64.7943657020802));
#183765=CARTESIAN_POINT('Ctrl Pts',(-6.47152498377083,4.83909614711294,
65.0059223224622));
#183766=CARTESIAN_POINT('Ctrl Pts',(-8.55977967864248,-0.073096424218834,
65.2174789428439));
#183767=CARTESIAN_POINT('Ctrl Pts',(-6.55265142392936,-5.52097747564786,
65.429035563226));
#183768=CARTESIAN_POINT('Ctrl Pts',(-1.74189528540399,-7.89483686565093,
65.6405921836078));
#183769=CARTESIAN_POINT('Ctrl Pts',(2.22393186351381,-7.78690568717823,
65.7992596488943));
#183770=CARTESIAN_POINT('Ctrl Pts',(5.68824200564854,-5.76650852129091,
65.9579271141807));
#183771=CARTESIAN_POINT('Ctrl Pts',(7.74450397277799,-2.34799612847024,
66.1165945794671));
#183772=CARTESIAN_POINT('Ctrl Pts',(7.93280824578086,1.63684787827589,66.2752620447535));
#183773=CARTESIAN_POINT('Ctrl Pts',(6.17372664616111,5.24088469755259,66.4339295100401));
#183774=CARTESIAN_POINT('Ctrl Pts',(2.93553478351249,7.53294655864104,66.5925969753264));
#183775=CARTESIAN_POINT('Ctrl Pts',(-2.38351862620874,8.23026560498812,
66.8041535957083));
#183776=CARTESIAN_POINT('Ctrl Pts',(-7.0780367158128,4.81420476130172,67.0157102160903));
#183777=CARTESIAN_POINT('Ctrl Pts',(-8.06920482330742,-0.430604988459075,
67.2272668364721));
#183778=CARTESIAN_POINT('Ctrl Pts',(-6.52548736938242,-5.54014312325638,
67.4388234568541));
#183779=CARTESIAN_POINT('Ctrl Pts',(-1.49407666736653,-8.43718957249187,
67.6503800772358));
#183780=CARTESIAN_POINT('Ctrl Pts',(3.72055634062224,-7.17775095951435,
67.8619366976179));
#183781=CARTESIAN_POINT('Ctrl Pts',(6.69642517933677,-4.55408200761746,
68.0206041629042));
#183782=CARTESIAN_POINT('Ctrl Pts',(8.06195717757933,-0.783303330659765,
68.1792716281907));
#183783=CARTESIAN_POINT('Ctrl Pts',(7.45063563745237,3.15886944991555,68.3379390934771));
#183784=CARTESIAN_POINT('Ctrl Pts',(5.04223681335312,6.33912971621593,68.4966065587636));
#183785=CARTESIAN_POINT('Ctrl Pts',(1.38258078195735,7.97936360218798,68.6552740240499));
#183786=CARTESIAN_POINT('Ctrl Pts',(-2.57220997600818,7.66461898334663,
68.8139414893365));
#183787=CARTESIAN_POINT('Ctrl Pts',(-7.10300679619978,4.79225702808968,
69.0254981097182));
#183788=CARTESIAN_POINT('Ctrl Pts',(-8.51894575764623,-0.838292557771904,
69.2370547301004));
#183789=CARTESIAN_POINT('Ctrl Pts',(-5.91977111059251,-5.50034518323783,
69.4486113504821));
#183790=CARTESIAN_POINT('Ctrl Pts',(-1.4609408167016,-8.43450195116639,
69.6601679708642));
#183791=CARTESIAN_POINT('Ctrl Pts',(4.25830560195405,-7.4354062680194,69.8717245912458));
#183792=CARTESIAN_POINT('Ctrl Pts',(7.45528542258912,-3.1275177998348,70.0832812116279));
#183793=CARTESIAN_POINT('Ctrl Pts',(8.05928550274226,0.793530276579739,
70.2419486769142));
#183794=CARTESIAN_POINT('Ctrl Pts',(6.69192440169235,4.56364606898694,70.4006161422007));
#183795=CARTESIAN_POINT('Ctrl Pts',(3.69690001887922,7.19884420265474,70.5592836074872));
#183796=CARTESIAN_POINT('Ctrl Pts',(-0.189808693744583,8.09769660463547,
70.7179510727736));
#183797=CARTESIAN_POINT('Ctrl Pts',(-4.05059701706489,7.01244871067912,
70.87661853806));
#183798=CARTESIAN_POINT('Ctrl Pts',(-6.88549219908465,4.23705623008454,
71.0352860033464));
#183799=CARTESIAN_POINT('Ctrl Pts',(-8.52405681638749,-0.871141986781069,
71.2468426237284));
#183800=CARTESIAN_POINT('Ctrl Pts',(-6.00389410714868,-6.10151020520986,
71.4583992441102));
#183801=CARTESIAN_POINT('Ctrl Pts',(-1.02136088278692,-8.01587855968927,
71.6699558644921));
#183802=CARTESIAN_POINT('Ctrl Pts',(4.28202588432986,-7.41211343410654,
71.881512484874));
#183803=CARTESIAN_POINT('Ctrl Pts',(8.03324957591474,-2.98082777449497,
72.0930691052561));
#183804=CARTESIAN_POINT('Ctrl Pts',(7.72798799084106,2.37504735404791,72.3046257256377));
#183805=CARTESIAN_POINT('Ctrl Pts',(5.67963852957239,5.77264924345462,72.4632931909244));
#183806=CARTESIAN_POINT('Ctrl Pts',(2.21434866893366,7.79136558077833,72.6219606562107));
#183807=CARTESIAN_POINT('Ctrl Pts',(-1.77357280805547,7.89587658833466,
72.7806281214972));
#183808=CARTESIAN_POINT('Ctrl Pts',(-5.33371233999737,6.09591915260571,
72.9392955867835));
#183809=CARTESIAN_POINT('Ctrl Pts',(-7.60279059153105,2.78914831729824,
73.09796305207));
#183810=CARTESIAN_POINT('Ctrl Pts',(-8.00134398160658,-1.15807720319577,
73.2566305173565));
#183811=CARTESIAN_POINT('Ctrl Pts',(-5.98677271118669,-6.13000697183332,
73.4681871377381));
#183812=CARTESIAN_POINT('Ctrl Pts',(-0.700801569375949,-8.53135677336813,
73.6797437581205));
#183813=CARTESIAN_POINT('Ctrl Pts',(4.35134083834832,-6.80906161266702,
73.891300378502));
#183814=CARTESIAN_POINT('Ctrl Pts',(8.03653925277048,-2.94774627008737,
74.1028569988843));
#183815=CARTESIAN_POINT('Ctrl Pts',(8.07777661119743,2.85796395878713,74.3144136192658));
#183816=CARTESIAN_POINT('Ctrl Pts',(4.41202858232987,6.77470679138646,74.5259702396479));
#183817=CARTESIAN_POINT('Ctrl Pts',(0.662525911141174,8.07111098496528,
74.6846377049342));
#183818=CARTESIAN_POINT('Ctrl Pts',(-3.29150879522989,7.40099233156405,
74.8433051702208));
#183819=CARTESIAN_POINT('Ctrl Pts',(-6.42044791371609,4.92628421743445,
75.0019726355071));
#183820=CARTESIAN_POINT('Ctrl Pts',(-8.00078881050586,1.26336695010976,
75.1606401007937));
#183821=CARTESIAN_POINT('Ctrl Pts',(-7.62446036789397,-2.72935472465092,
75.3193075660799));
#183822=CARTESIAN_POINT('Ctrl Pts',(-5.40159489313535,-6.01543189895851,
75.4779750313666));
#183823=CARTESIAN_POINT('Ctrl Pts',(-0.669398417230296,-8.54226777437611,
75.6895316517482));
#183824=CARTESIAN_POINT('Ctrl Pts',(4.92772366164841,-6.99947931981837,
75.9010882721302));
#183825=CARTESIAN_POINT('Ctrl Pts',(7.70340129645059,-2.44030645666002,
76.1126448925122));
#183826=CARTESIAN_POINT('Ctrl Pts',(8.05910804839823,2.88547200616767,76.324201512894));
#183827=CARTESIAN_POINT('Ctrl Pts',(4.37120959512461,7.36959697986436,76.535758133276));
#183828=CARTESIAN_POINT('Ctrl Pts',(-0.952753784053995,8.02838144008641,
76.7473147536578));
#183829=CARTESIAN_POINT('Ctrl Pts',(-4.66224525292312,6.62157400594119,
76.9059822189443));
#183830=CARTESIAN_POINT('Ctrl Pts',(-7.26888142302682,3.57380476508172,
77.0646496842306));
#183831=CARTESIAN_POINT('Ctrl Pts',(-8.08584616808648,-0.330937078198273,
77.2233171495173));
#183832=CARTESIAN_POINT('Ctrl Pts',(-6.95252221598853,-4.15585761030523,
77.3819846148034));
#183833=CARTESIAN_POINT('Ctrl Pts',(-4.10554350669663,-6.98042159394269,
77.5406520800901));
#183834=CARTESIAN_POINT('Ctrl Pts',(-0.293495865475981,-8.07938787888673,
77.6993195453763));
#183835=CARTESIAN_POINT('Ctrl Pts',(4.95882582241272,-6.98773779080956,
77.9108761657584));
#183836=CARTESIAN_POINT('Ctrl Pts',(8.26795153021402,-2.21723898760715,
78.1224327861402));
#183837=CARTESIAN_POINT('Ctrl Pts',(7.47821715258361,3.06165892211683,78.3339894065222));
#183838=CARTESIAN_POINT('Ctrl Pts',(4.33925195229646,7.37875760061446,78.5455460269039));
#183839=CARTESIAN_POINT('Ctrl Pts',(-1.36522518019884,8.45899480892892,
78.757102647286));
#183840=CARTESIAN_POINT('Ctrl Pts',(-5.87510387930802,5.55389977654387,
78.9686592676679));
#183841=CARTESIAN_POINT('Ctrl Pts',(-7.82199981947996,2.09716283073475,
79.1273267329542));
#183842=CARTESIAN_POINT('Ctrl Pts',(-7.87078835298228,-1.9129580088188,
79.2859941982408));
#183843=CARTESIAN_POINT('Ctrl Pts',(-5.99640309405961,-5.43448042937297,
79.4446616635271));
#183844=CARTESIAN_POINT('Ctrl Pts',(-2.67569831151025,-7.64521786391511,
79.6033291288137));
#183845=CARTESIAN_POINT('Ctrl Pts',(1.31987319558362,-7.9899754606719,79.7619965940999));
#183846=CARTESIAN_POINT('Ctrl Pts',(4.95089445223432,-6.39150157970637,
79.9206640593866));
#183847=CARTESIAN_POINT('Ctrl Pts',(8.28430972403062,-2.18829736701093,
80.1322206797682));
#183848=CARTESIAN_POINT('Ctrl Pts',(7.76877342178239,3.59462525934789,80.3437773001502));
#183849=CARTESIAN_POINT('Ctrl Pts',(3.78035763949229,7.14187533173929,80.5553339205322));
#183850=CARTESIAN_POINT('Ctrl Pts',(-1.39563166549146,8.44555406639563,
80.766890540914));
#183851=CARTESIAN_POINT('Ctrl Pts',(-6.4676874778603,5.62027149334128,80.978447161296));
#183852=CARTESIAN_POINT('Ctrl Pts',(-8.06921967526007,0.500342035960366,
81.1900037816779));
#183853=CARTESIAN_POINT('Ctrl Pts',(-7.3494359394134,-3.40111224263743,
81.3486712469643));
#183854=CARTESIAN_POINT('Ctrl Pts',(-4.81772080277898,-6.51139646369471,
81.5073387122507));
#183855=CARTESIAN_POINT('Ctrl Pts',(-1.12239775020272,-8.01440271598737,
81.6660061775372));
#183856=CARTESIAN_POINT('Ctrl Pts',(2.84364522462193,-7.58435227804134,
81.8246736428235));
#183857=CARTESIAN_POINT('Ctrl Pts',(6.13237761632933,-5.28920768029616,
81.9833411081101));
#183858=CARTESIAN_POINT('Ctrl Pts',(7.8962275389091,-1.73558029901443,82.1420085733965));
#183859=CARTESIAN_POINT('Ctrl Pts',(7.76279135991085,3.62732729053053,82.3535651937783));
#183860=CARTESIAN_POINT('Ctrl Pts',(3.66199372055804,7.73724584233487,82.5651218141603));
#183861=CARTESIAN_POINT('Ctrl Pts',(-1.67299447212423,7.90560412826337,
82.7766784345421));
#183862=CARTESIAN_POINT('Ctrl Pts',(-6.48242288232662,5.59047089329887,
82.9882350549241));
#183863=CARTESIAN_POINT('Ctrl Pts',(-8.56673618884236,0.171650927506622,
83.199791675306));
#183864=CARTESIAN_POINT('Ctrl Pts',(-6.51621502212827,-4.78556058429354,
83.4113482956879));
#183865=CARTESIAN_POINT('Ctrl Pts',(-3.46399909193418,-7.32000569710434,
83.5700157609743));
#183866=CARTESIAN_POINT('Ctrl Pts',(0.47256185180701,-8.08612409855068,
83.7286832262607));
#183867=CARTESIAN_POINT('Ctrl Pts',(4.27281778882183,-6.87266001976035,
83.8873506915472));
#183868=CARTESIAN_POINT('Ctrl Pts',(7.04247926913745,-4.00152513233574,
84.0460181568335));
#183869=CARTESIAN_POINT('Ctrl Pts',(8.09717699341311,-0.132279446258024,
84.2046856221201));
#183870=CARTESIAN_POINT('Ctrl Pts',(7.17477289734989,3.72629604191705,84.3633530874064));
#183871=CARTESIAN_POINT('Ctrl Pts',(3.63644930560508,7.75852237335814,84.5749097077883));
#183872=CARTESIAN_POINT('Ctrl Pts',(-2.14531367813232,8.28690536066105,
84.7864663281702));
#183873=CARTESIAN_POINT('Ctrl Pts',(-6.34945463507768,4.99819097010746,
84.9980229485521));
#183874=CARTESIAN_POINT('Ctrl Pts',(-8.5589578018338,0.139329037041669,
85.209579568934));
#183875=CARTESIAN_POINT('Ctrl Pts',(-6.68763166481757,-5.35667953921688,
85.421136189316));
#183876=CARTESIAN_POINT('Ctrl Pts',(-1.93726194489959,-7.84918240821281,
85.6326928096978));
#183877=CARTESIAN_POINT('Ctrl Pts',(2.03002227243321,-7.83969276744859,
85.7913602749844));
#183878=CARTESIAN_POINT('Ctrl Pts',(5.54339996904871,-5.90588134185714,
85.9500277402706));
#183879=CARTESIAN_POINT('Ctrl Pts',(7.68385597786112,-2.53944578898081,
86.1086952055573));
#183880=CARTESIAN_POINT('Ctrl Pts',(7.97098245842279,1.43949862398741,86.2673626708435));
#183881=CARTESIAN_POINT('Ctrl Pts',(6.30187332299991,5.08607567142123,86.42603013613));
#183882=CARTESIAN_POINT('Ctrl Pts',(3.1215539312156,7.45778448167187,86.5846976014164));
#183883=CARTESIAN_POINT('Ctrl Pts',(-2.17855833266883,8.28687616423068,
86.7962542217983));
#183884=CARTESIAN_POINT('Ctrl Pts',(-6.95639726875433,4.98835727202873,
87.0078108421803));
#183885=CARTESIAN_POINT('Ctrl Pts',(-8.07740524430385,-0.230242602195722,
87.2193674625621));
#183886=CARTESIAN_POINT('Ctrl Pts',(-6.66095155220817,-5.37651333610082,
87.4309240829441));
#183887=CARTESIAN_POINT('Ctrl Pts',(-1.70297761113879,-8.39751750376825,
87.6424807033259));
#183888=CARTESIAN_POINT('Ctrl Pts',(3.54130152107833,-7.26786294981969,
87.8540373237079));
#183889=CARTESIAN_POINT('Ctrl Pts',(6.58135794038168,-4.71884527984714,
88.0127047889942));
#183890=CARTESIAN_POINT('Ctrl Pts',(8.04003782685793,-0.983112091085808,
88.1713722542807));
#183891=CARTESIAN_POINT('Ctrl Pts',(7.52672586548044,2.97301620405819,88.3300397195672));
#183892=CARTESIAN_POINT('Ctrl Pts',(5.19798382085618,6.21205938792148,88.4887071848536));
#183893=CARTESIAN_POINT('Ctrl Pts',(1.58015553245196,7.94259917204825,88.64737465014));
#183894=CARTESIAN_POINT('Ctrl Pts',(-2.3812275749546,7.726085914409,88.8060421154264));
#183895=CARTESIAN_POINT('Ctrl Pts',(-6.98190427298533,4.96703590615213,
89.0175987358083));
#183896=CARTESIAN_POINT('Ctrl Pts',(-8.5371240830427,-0.626644735768,89.2291553561904));
#183897=CARTESIAN_POINT('Ctrl Pts',(-6.05443425459705,-5.35175793485983,
89.440711976572));
#183898=CARTESIAN_POINT('Ctrl Pts',(-1.66978527272744,-8.3956529452519,
89.6522685969541));
#183899=CARTESIAN_POINT('Ctrl Pts',(4.0724917242945,-7.53878266868651,89.863825217336));
#183900=CARTESIAN_POINT('Ctrl Pts',(7.37538337916467,-3.31155074412213,
90.0753818377178));
#183901=CARTESIAN_POINT('Ctrl Pts',(8.07649463078164,0.593302278366084,
90.2340493030044));
#183902=CARTESIAN_POINT('Ctrl Pts',(6.80310647167449,4.39618698146572,90.3927167682906));
#183903=CARTESIAN_POINT('Ctrl Pts',(3.87439429122061,7.10489243267192,90.5513842335773));
#183904=CARTESIAN_POINT('Ctrl Pts',(0.0111865443886908,8.09991311695225,
90.7100516988636));
#183905=CARTESIAN_POINT('Ctrl Pts',(-3.87534239380638,7.11080125199156,
90.86871916415));
#183906=CARTESIAN_POINT('Ctrl Pts',(-6.7782334424462,4.40660864160255,91.0273866294365));
#183907=CARTESIAN_POINT('Ctrl Pts',(-8.54304869596879,-0.659357223743514,
91.2389432498183));
#183908=CARTESIAN_POINT('Ctrl Pts',(-6.15344869793795,-5.95065041452155,
91.4504998702001));
#183909=CARTESIAN_POINT('Ctrl Pts',(-1.21995294344862,-7.98806622108564,
91.6620564905823));
#183910=CARTESIAN_POINT('Ctrl Pts',(4.09678269278692,-7.51608560370173,
91.8736131109638));
#183911=CARTESIAN_POINT('Ctrl Pts',(7.95680954405873,-3.17924752878318,
92.0851697313462));
#183912=CARTESIAN_POINT('Ctrl Pts',(7.78454300291698,2.18255321977839,92.2967263517278));
#183913=CARTESIAN_POINT('Ctrl Pts',(5.82113258565889,5.6299368142819,92.4553938170143));
#183914=CARTESIAN_POINT('Ctrl Pts',(2.40700230900052,7.73401949366712,92.6140612823008));
#183915=CARTESIAN_POINT('Ctrl Pts',(-1.57709787894137,7.93745487426641,
92.772728747587));
#183916=CARTESIAN_POINT('Ctrl Pts',(-5.18080545044434,6.22639321954773,
92.9313962128737));
#183917=CARTESIAN_POINT('Ctrl Pts',(-7.53123945343747,2.97694565346133,
93.0900636781598));
#183918=CARTESIAN_POINT('Ctrl Pts',(-8.02761684064636,-0.959174718232218,
93.2487311434466));
#183919=CARTESIAN_POINT('Ctrl Pts',(-6.13703969987023,-5.97956326165626,
93.4602877638282));
#183920=CARTESIAN_POINT('Ctrl Pts',(-0.912283436855274,-8.51134008414109,
93.6718443842103));
#183921=CARTESIAN_POINT('Ctrl Pts',(4.18104046060788,-6.91493946600112,
93.8834010045922));
#183922=CARTESIAN_POINT('Ctrl Pts',(7.96091912382044,-3.14625782064091,
94.094957624974));
#183923=CARTESIAN_POINT('Ctrl Pts',(8.14620698463648,2.65664140730353,94.306514245356));
#183924=CARTESIAN_POINT('Ctrl Pts',(4.57877815237362,6.6631404217957,94.5180708657379));
#183925=CARTESIAN_POINT('Ctrl Pts',(0.86259885226857,8.05218568880823,94.6767383310243));
#183926=CARTESIAN_POINT('Ctrl Pts',(-3.1068462643541,7.48038937343908,94.8354057963108));
#183927=CARTESIAN_POINT('Ctrl Pts',(-6.29623036425301,5.08408437159998,
94.9940732615971));
#183928=CARTESIAN_POINT('Ctrl Pts',(-7.96697490175043,1.46151079550249,
95.1527407268836));
#183929=CARTESIAN_POINT('Ctrl Pts',(-7.68984104611083,-2.53932181665002,
95.31140819217));
#183930=CARTESIAN_POINT('Ctrl Pts',(-5.54919544733642,-5.87954163659009,
95.4700756574564));
#183931=CARTESIAN_POINT('Ctrl Pts',(-0.881168716971856,-8.52303255684783,
95.6816322778383));
#183932=CARTESIAN_POINT('Ctrl Pts',(4.75253610195871,-7.11959024768543,
95.8931888982204));
#183933=CARTESIAN_POINT('Ctrl Pts',(7.64045732748193,-2.63072034844158,
96.104745518602));
#183934=CARTESIAN_POINT('Ctrl Pts',(8.12827140123375,2.68463536695919,96.3163021389842));
#183935=CARTESIAN_POINT('Ctrl Pts',(4.55264398669978,7.25879796759945,96.5278587593658));
#183936=CARTESIAN_POINT('Ctrl Pts',(-0.753133361840499,8.0496279674861,
96.739415379748));
#183937=CARTESIAN_POINT('Ctrl Pts',(-4.49673398340393,6.73506221760718,
96.8980828450341));
#183938=CARTESIAN_POINT('Ctrl Pts',(-7.17751004723008,3.75339048709656,
97.0567503103208));
#183939=CARTESIAN_POINT('Ctrl Pts',(-8.0924294497543,-0.130793062789233,
97.2154177756071));
#183940=CARTESIAN_POINT('Ctrl Pts',(-7.05188031461038,-3.98092452596377,
97.3740852408936));
#183941=CARTESIAN_POINT('Ctrl Pts',(-4.28052068787601,-6.87850741011934,
97.5327527061801));
#183942=CARTESIAN_POINT('Ctrl Pts',(-0.488505341726331,-8.06587977813096,
97.6914201714664));
#183943=CARTESIAN_POINT('Ctrl Pts',(4.77208267160989,-7.11669744080927,
97.9029767918484));
#183944=CARTESIAN_POINT('Ctrl Pts',(9.09452740495533,-1.23259449210053,
98.1674225673258));
#183945=CARTESIAN_POINT('Ctrl Pts',(6.49394857205468,5.59032484645831,98.4318683428031));
#183946=CARTESIAN_POINT('Ctrl Pts',(1.67589148870856,7.90460136012811,98.6434249631851));
#183947=CARTESIAN_POINT('Ctrl Pts',(-2.29582483006711,7.77044586128011,
98.8020924284714));
#183948=CARTESIAN_POINT('Ctrl Pts',(-5.73741125166451,5.7125883020101,98.960759893758));
#183949=CARTESIAN_POINT('Ctrl Pts',(-7.76703063392476,2.28272931010332,
99.1194273590443));
#183950=CARTESIAN_POINT('Ctrl Pts',(-7.91518952336318,-1.71376454947224,
99.2781103900609));
#183951=CARTESIAN_POINT('Ctrl Pts',(-6.72572425074295,-4.09503579149403,
99.383904265982));
#183952=CARTESIAN_POINT('Ctrl Pts',(-5.88260427835266,-5.07275281619164,
99.4368089868075));
#183953=CARTESIAN_POINT('Ctrl Pts',(1.9103352902639,-7.13425027812016,-0.427061590008181));
#183954=CARTESIAN_POINT('Ctrl Pts',(3.0958658925461,-6.81680238470299,-0.374166617870574));
#183955=CARTESIAN_POINT('Ctrl Pts',(5.30450950520224,-5.58155414157205,
-0.26838249063749));
#183956=CARTESIAN_POINT('Ctrl Pts',(7.32611862039227,-2.36127264943766,
-0.10970920830893));
#183957=CARTESIAN_POINT('Ctrl Pts',(7.56588082625083,1.42044622507859,0.0489582569774992));
#183958=CARTESIAN_POINT('Ctrl Pts',(5.96180663696039,4.879206838332,0.207625722263927));
#183959=CARTESIAN_POINT('Ctrl Pts',(2.91184473574469,7.10958063960511,0.366293187550357));
#183960=CARTESIAN_POINT('Ctrl Pts',(-2.1132825876687,7.86831172497225,0.577849807932259));
#183961=CARTESIAN_POINT('Ctrl Pts',(-7.80768231834692,3.89690115303222,
0.842295583409641));
#183962=CARTESIAN_POINT('Ctrl Pts',(-7.55836006524443,-3.04053021023064,
1.10674135888703));
#183963=CARTESIAN_POINT('Ctrl Pts',(-3.93140712003248,-6.60107452752234,
1.31829797926893));
#183964=CARTESIAN_POINT('Ctrl Pts',(-0.315651225764061,-7.69659528282126,
1.47696544455536));
#183965=CARTESIAN_POINT('Ctrl Pts',(3.41286611415151,-6.90183796702513,
1.63563290984179));
#183966=CARTESIAN_POINT('Ctrl Pts',(6.29060828777561,-4.43237517133558,
1.79430037512822));
#183967=CARTESIAN_POINT('Ctrl Pts',(7.64958627743303,-0.889942290678628,
1.95296784041465));
#183968=CARTESIAN_POINT('Ctrl Pts',(7.13775755670161,2.88788372663806,2.11163530570107));
#183969=CARTESIAN_POINT('Ctrl Pts',(4.89863020487389,5.92400513809533,2.27030277098751));
#183970=CARTESIAN_POINT('Ctrl Pts',(0.305225732017479,8.14109071228054,
2.4818593913694));
#183971=CARTESIAN_POINT('Ctrl Pts',(-4.95243528681909,6.45885070470568,
2.69341601175132));
#183972=CARTESIAN_POINT('Ctrl Pts',(-7.41281351776048,2.02003584299111,
2.90497263213322));
#183973=CARTESIAN_POINT('Ctrl Pts',(-7.54454431414525,-3.05326164535232,
3.11652925251513));
#183974=CARTESIAN_POINT('Ctrl Pts',(-3.86736055188791,-7.17047382046754,
3.32808587289703));
#183975=CARTESIAN_POINT('Ctrl Pts',(1.21597883501667,-7.59017650439491,
3.53964249327894));
#183976=CARTESIAN_POINT('Ctrl Pts',(4.68557750845913,-6.1100685107214,3.69830995856536));
#183977=CARTESIAN_POINT('Ctrl Pts',(7.0439088100044,-3.11371703287544,3.85697742385179));
#183978=CARTESIAN_POINT('Ctrl Pts',(7.66884899663536,0.627470455451795,
4.01564488913822));
#183979=CARTESIAN_POINT('Ctrl Pts',(6.44407833797578,4.21731596174447,4.17431235442465));
#183980=CARTESIAN_POINT('Ctrl Pts',(3.63004607854268,6.79045680289362,4.33297981971107));
#183981=CARTESIAN_POINT('Ctrl Pts',(-0.0340013617160748,7.68689084058012,
4.49164728499751));
#183982=CARTESIAN_POINT('Ctrl Pts',(-4.98150970567032,6.4464434871977,4.70320390537941));
#183983=CARTESIAN_POINT('Ctrl Pts',(-7.94051430745141,1.78627946610955,
4.91476052576132));
#183984=CARTESIAN_POINT('Ctrl Pts',(-6.98586204731743,-3.19816663715534,
5.12631714614322));
#183985=CARTESIAN_POINT('Ctrl Pts',(-3.83664898111913,-7.17793047932758,
5.33787376652512));
#183986=CARTESIAN_POINT('Ctrl Pts',(1.62450660604406,-7.98329831713192,
5.54943038690703));
#183987=CARTESIAN_POINT('Ctrl Pts',(5.79646930875302,-5.0488007687728,5.76098700728893));
#183988=CARTESIAN_POINT('Ctrl Pts',(7.51220495144241,-1.68947230913394,
5.91965447257537));
#183989=CARTESIAN_POINT('Ctrl Pts',(7.40328658390602,2.12208533635141,6.07832193786179));
#183990=CARTESIAN_POINT('Ctrl Pts',(5.48624538749858,5.39500443507579,6.23698940314823));
#183991=CARTESIAN_POINT('Ctrl Pts',(2.24593360793106,7.36666007433078,6.39565686843465));
#183992=CARTESIAN_POINT('Ctrl Pts',(-1.56326161954992,7.53947962462525,
6.55432433372108));
#183993=CARTESIAN_POINT('Ctrl Pts',(-4.95088911328448,5.88031824608128,
6.7129917990075));
#183994=CARTESIAN_POINT('Ctrl Pts',(-7.95493420652126,1.7581511327172,6.92454841938941));
#183995=CARTESIAN_POINT('Ctrl Pts',(-7.2412584479266,-3.71574186194191,
7.13610503977132));
#183996=CARTESIAN_POINT('Ctrl Pts',(-3.31486374163761,-6.93124929171932,
7.34766166015322));
#183997=CARTESIAN_POINT('Ctrl Pts',(1.65287275986168,-7.96935211506437,
7.55921828053513));
#183998=CARTESIAN_POINT('Ctrl Pts',(6.36200152916944,-5.08891051000637,
7.77077490091703));
#183999=CARTESIAN_POINT('Ctrl Pts',(7.68523972297024,-0.162899008328246,
7.98233152129894));
#184000=CARTESIAN_POINT('Ctrl Pts',(6.85037485688638,3.515665544841,8.14099898658536));
#184001=CARTESIAN_POINT('Ctrl Pts',(4.32478421598083,6.3724516400251,8.2996664518718));
#184002=CARTESIAN_POINT('Ctrl Pts',(0.755982743686845,7.65724829166524,
8.45833391715822));
#184003=CARTESIAN_POINT('Ctrl Pts',(-2.99516013971152,7.09513313171334,
8.61700138244464));
#184004=CARTESIAN_POINT('Ctrl Pts',(-6.0306341810463,4.78737833030146,8.77566884773109));
#184005=CARTESIAN_POINT('Ctrl Pts',(-7.56872214277144,1.34309002377562,
8.93433631301751));
#184006=CARTESIAN_POINT('Ctrl Pts',(-7.23430921682634,-3.74657761047246,
9.14589293339943));
#184007=CARTESIAN_POINT('Ctrl Pts',(-3.17936424139809,-7.4922763239762,
9.3574495537813));
#184008=CARTESIAN_POINT('Ctrl Pts',(1.89546479066837,-7.44565320148777,
9.56900617416324));
#184009=CARTESIAN_POINT('Ctrl Pts',(6.37484650973986,-5.0600289990822,9.78056279454512));
#184010=CARTESIAN_POINT('Ctrl Pts',(8.14516047322325,0.168625328447077,
9.99211941492704));
#184011=CARTESIAN_POINT('Ctrl Pts',(6.00519926219761,4.79864850846001,10.203676035309));
#184012=CARTESIAN_POINT('Ctrl Pts',(3.00742183609204,7.08822642152758,10.3623435005954));
#184013=CARTESIAN_POINT('Ctrl Pts',(-0.762027260887039,7.66362922334555,
10.5210109658818));
#184014=CARTESIAN_POINT('Ctrl Pts',(-4.32533719076805,6.36367971343036,
10.6796784311683));
#184015=CARTESIAN_POINT('Ctrl Pts',(-6.84538509720808,3.52882434957768,
10.8383458964547));
#184016=CARTESIAN_POINT('Ctrl Pts',(-7.69754851107875,-0.187847870986907,
10.9970133617411));
#184017=CARTESIAN_POINT('Ctrl Pts',(-6.67185181111312,-3.81783172717063,
11.1556808270275));
#184018=CARTESIAN_POINT('Ctrl Pts',(-3.154272897111,-7.51150025803788,11.3672374474094));
#184019=CARTESIAN_POINT('Ctrl Pts',(2.35893800003516,-7.78960672988603,
11.5787940677913));
#184020=CARTESIAN_POINT('Ctrl Pts',(6.22559236632147,-4.5025035322461,11.7903506881733));
#184021=CARTESIAN_POINT('Ctrl Pts',(8.13651942784416,0.199030386146407,
12.0019073085552));
#184022=CARTESIAN_POINT('Ctrl Pts',(6.14593418071584,5.34785626978331,12.213463928937));
#184023=CARTESIAN_POINT('Ctrl Pts',(1.53651183656423,7.53183756214526,12.425020549319));
#184024=CARTESIAN_POINT('Ctrl Pts',(-2.23209396456929,7.36921274196765,
12.5836880146054));
#184025=CARTESIAN_POINT('Ctrl Pts',(-5.49497454184229,5.39603124562451,
12.7423554798918));
#184026=CARTESIAN_POINT('Ctrl Pts',(-7.39809123050544,2.11499585202551,
12.9010229451783));
#184027=CARTESIAN_POINT('Ctrl Pts',(-7.51680423309027,-1.67617199017493,
13.0596904104647));
#184028=CARTESIAN_POINT('Ctrl Pts',(-5.78993610934901,-5.07584276280316,
13.2183578757511));
#184029=CARTESIAN_POINT('Ctrl Pts',(-2.67675967353113,-7.2058589589723,
13.3770253410375));
#184030=CARTESIAN_POINT('Ctrl Pts',(2.39051973739319,-7.78829179095684,
13.5885819614195));
#184031=CARTESIAN_POINT('Ctrl Pts',(6.80181525940307,-4.46966113606466,
13.8001385818013));
#184032=CARTESIAN_POINT('Ctrl Pts',(7.66472856953409,0.531483136944698,
14.0116952021832));
#184033=CARTESIAN_POINT('Ctrl Pts',(6.11981976973525,5.36566561390598,14.2232518225652));
#184034=CARTESIAN_POINT('Ctrl Pts',(1.29270755433579,8.04369198906295,14.4348084429471));
#184035=CARTESIAN_POINT('Ctrl Pts',(-3.64568881026725,6.76745142466027,
14.646365063329));
#184036=CARTESIAN_POINT('Ctrl Pts',(-6.43508761370743,4.22814229975222,
14.8050325286154));
#184037=CARTESIAN_POINT('Ctrl Pts',(-7.67620898046891,0.62266693136815,
14.9636999939018));
#184038=CARTESIAN_POINT('Ctrl Pts',(-7.03537814335224,-3.11583306500975,
15.1223674591882));
#184039=CARTESIAN_POINT('Ctrl Pts',(-4.6976292363168,-6.10280083054923,
15.2810349244747));
#184040=CARTESIAN_POINT('Ctrl Pts',(-1.19363894411629,-7.60675791478432,
15.4397023897611));
#184041=CARTESIAN_POINT('Ctrl Pts',(2.56134496261047,-7.24768636662445,
15.5983698550475));
#184042=CARTESIAN_POINT('Ctrl Pts',(6.82522171227787,-4.4484179450905,15.8099264754294));
#184043=CARTESIAN_POINT('Ctrl Pts',(8.08611931403569,0.925870365372249,
16.0214830958114));
#184044=CARTESIAN_POINT('Ctrl Pts',(5.54457870601156,5.31866386814692,16.2330397161932));
#184045=CARTESIAN_POINT('Ctrl Pts',(1.26124658150169,8.04063545716044,16.4445963365752));
#184046=CARTESIAN_POINT('Ctrl Pts',(-4.16081638782906,7.00426160438954,
16.656152956957));
#184047=CARTESIAN_POINT('Ctrl Pts',(-7.13493330498989,2.86044968838645,
16.867709577339));
#184048=CARTESIAN_POINT('Ctrl Pts',(-7.6498061433939,-0.876359441974459,
17.0263770426254));
#184049=CARTESIAN_POINT('Ctrl Pts',(-6.29282616987816,-4.43984653056245,
17.1850445079118));
#184050=CARTESIAN_POINT('Ctrl Pts',(-3.40563176562958,-6.89975605263704,
17.3437119731982));
#184051=CARTESIAN_POINT('Ctrl Pts',(0.302993692477398,-7.69545926125072,
17.5023794384847));
#184052=CARTESIAN_POINT('Ctrl Pts',(3.95695083878236,-6.60530695444992,
17.6610469037711));
#184053=CARTESIAN_POINT('Ctrl Pts',(6.6100324713461,-3.92389046918924,17.8197143690576));
#184054=CARTESIAN_POINT('Ctrl Pts',(8.0904811788591,0.957177063285023,18.0312709894394));
#184055=CARTESIAN_POINT('Ctrl Pts',(5.61545519891417,5.89145350514484,18.2428276098214));
#184056=CARTESIAN_POINT('Ctrl Pts',(0.84968121050301,7.63600551401102,18.4543842302032));
#184057=CARTESIAN_POINT('Ctrl Pts',(-4.18301432463752,6.98175856458619,
18.6659408505852));
#184058=CARTESIAN_POINT('Ctrl Pts',(-7.68217330527907,2.71224758154732,
18.877497470967));
#184059=CARTESIAN_POINT('Ctrl Pts',(-7.31091387012258,-2.37486506355482,
19.089054091349));
#184060=CARTESIAN_POINT('Ctrl Pts',(-5.31216816464087,-5.57390431328177,
19.2477215566354));
#184061=CARTESIAN_POINT('Ctrl Pts',(-1.98723048460563,-7.44061915570909,
19.4063890219218));
#184062=CARTESIAN_POINT('Ctrl Pts',(1.80559497136075,-7.4796248641468,19.5650564872083));
#184063=CARTESIAN_POINT('Ctrl Pts',(5.16291480539385,-5.71456114951061,
19.7237239524947));
#184064=CARTESIAN_POINT('Ctrl Pts',(7.27004306916297,-2.53653576272058,
19.8823914177811));
#184065=CARTESIAN_POINT('Ctrl Pts',(7.58920535050375,1.22205066766044,20.0410588830675));
#184066=CARTESIAN_POINT('Ctrl Pts',(5.59874694737816,5.91828575308559,20.2526155034494));
#184067=CARTESIAN_POINT('Ctrl Pts',(0.537130386280701,8.1212100356061,20.4641721238314));
#184068=CARTESIAN_POINT('Ctrl Pts',(-4.23978452917413,6.40739927862032,
20.6757287442132));
#184069=CARTESIAN_POINT('Ctrl Pts',(-7.68480010363191,2.68074781759015,
20.8872853645952));
#184070=CARTESIAN_POINT('Ctrl Pts',(-7.63614330750188,-2.83925853406245,
21.0988419849771));
#184071=CARTESIAN_POINT('Ctrl Pts',(-4.09191004187968,-6.50735874957023,
21.310398605359));
#184072=CARTESIAN_POINT('Ctrl Pts',(-0.507707523998028,-7.68308355890531,
21.4690660706454));
#184073=CARTESIAN_POINT('Ctrl Pts',(3.24117958490524,-6.98617587222398,
21.6277335359318));
#184074=CARTESIAN_POINT('Ctrl Pts',(6.17835378800283,-4.58616460446389,
21.7864010012183));
#184075=CARTESIAN_POINT('Ctrl Pts',(7.62532235160403,-1.07998030231049,
21.9450684665047));
#184076=CARTESIAN_POINT('Ctrl Pts',(7.20713016565148,2.71013185627586,22.1037359317911));
#184077=CARTESIAN_POINT('Ctrl Pts',(5.04416303840098,5.80050557524718,22.2624033970775));
#184078=CARTESIAN_POINT('Ctrl Pts',(0.50711086416215,8.13110768637341,22.4739600174594));
#184079=CARTESIAN_POINT('Ctrl Pts',(-4.79062278934888,6.57970324440751,
22.6855166378414));
#184080=CARTESIAN_POINT('Ctrl Pts',(-7.36041264286785,2.20337561396134,
22.8970732582232));
#184081=CARTESIAN_POINT('Ctrl Pts',(-7.61797915554366,-2.86512741077909,
23.1086298786052));
#184082=CARTESIAN_POINT('Ctrl Pts',(-4.04410144101776,-7.07229221474271,
23.320186498987));
#184083=CARTESIAN_POINT('Ctrl Pts',(1.0272626268211,-7.61801661733424,23.531743119369));
#184084=CARTESIAN_POINT('Ctrl Pts',(4.53251832342916,-6.22445319291774,
23.6904105846554));
#184085=CARTESIAN_POINT('Ctrl Pts',(6.96447629890928,-3.28754745991319,
23.8490780499418));
#184086=CARTESIAN_POINT('Ctrl Pts',(7.68205750980338,0.436982522579811,
24.0077455152283));
#184087=CARTESIAN_POINT('Ctrl Pts',(6.54674297907218,4.05611326089645,24.1664129805147));
#184088=CARTESIAN_POINT('Ctrl Pts',(3.79742712508109,6.69828986628251,24.3250804458011));
#184089=CARTESIAN_POINT('Ctrl Pts',(0.156752166466377,7.68536755430423,
24.4837479110876));
#184090=CARTESIAN_POINT('Ctrl Pts',(-4.8200133536601,6.56807010517477,24.6953045314694));
#184091=CARTESIAN_POINT('Ctrl Pts',(-7.89374442187484,1.98276587029716,
24.9068611518514));
#184092=CARTESIAN_POINT('Ctrl Pts',(-7.06307051436508,-3.02383420157176,
25.1184177722332));
#184093=CARTESIAN_POINT('Ctrl Pts',(-4.01358126405507,-7.08051741973153,
25.3299743926152));
#184094=CARTESIAN_POINT('Ctrl Pts',(1.42590828576246,-8.02115074017103,
25.541531012997));
#184095=CARTESIAN_POINT('Ctrl Pts',(5.66940319694829,-5.19108014548771,
25.753087633379));
#184096=CARTESIAN_POINT('Ctrl Pts',(7.46796913943167,-1.87536045483022,
25.9117550986654));
#184097=CARTESIAN_POINT('Ctrl Pts',(7.45366456041774,1.93772625518244,26.0704225639519));
#184098=CARTESIAN_POINT('Ctrl Pts',(5.61842808856437,5.25720715994694,26.2290900292382));
#184099=CARTESIAN_POINT('Ctrl Pts',(2.42803885110833,7.30866100984028,26.3877574945247));
#184100=CARTESIAN_POINT('Ctrl Pts',(-1.37569510680508,7.57594897528736,
26.5464249598111));
#184101=CARTESIAN_POINT('Ctrl Pts',(-4.80345003747338,6.00135929802082,
26.7050924250976));
#184102=CARTESIAN_POINT('Ctrl Pts',(-7.90885787044363,1.95500404630625,
26.9166490454794));
#184103=CARTESIAN_POINT('Ctrl Pts',(-7.33123141642751,-3.53491264574978,
27.1282056658614));
#184104=CARTESIAN_POINT('Ctrl Pts',(-3.4858355309382,-6.84685979268871,
27.3397622862433));
#184105=CARTESIAN_POINT('Ctrl Pts',(1.45461176920048,-8.00791271775603,
27.5513189066251));
#184106=CARTESIAN_POINT('Ctrl Pts',(6.23376599399237,-5.24521068862792,
27.7628755270071));
#184107=CARTESIAN_POINT('Ctrl Pts',(7.67883112467215,-0.353550908937111,
27.974432147389));
#184108=CARTESIAN_POINT('Ctrl Pts',(6.93550347755123,3.34459734735289,28.1330996126754));
#184109=CARTESIAN_POINT('Ctrl Pts',(4.48157899137418,6.26317396878968,28.2917670779619));
#184110=CARTESIAN_POINT('Ctrl Pts',(0.94575744281704,7.63613149234103,28.4504345432483));
#184111=CARTESIAN_POINT('Ctrl Pts',(-2.8181787659297,7.16727053085858,28.6091020085347));
#184112=CARTESIAN_POINT('Ctrl Pts',(-5.90998291927167,4.93554878376881,
28.7677694738211));
#184113=CARTESIAN_POINT('Ctrl Pts',(-7.53306408221923,1.53048724908849,
28.9264369391076));
#184114=CARTESIAN_POINT('Ctrl Pts',(-7.32504948547284,-3.56591133811914,
29.1379935594895));
#184115=CARTESIAN_POINT('Ctrl Pts',(-3.36429911605302,-7.41107636932855,
29.3495501798714));
#184116=CARTESIAN_POINT('Ctrl Pts',(1.71012420231409,-7.49039475476082,
29.5611068002533));
#184117=CARTESIAN_POINT('Ctrl Pts',(6.24732368715564,-5.21665680701726,
29.7726634206352));
#184118=CARTESIAN_POINT('Ctrl Pts',(8.14683672517312,-0.0335411586358248,
29.984220041017));
#184119=CARTESIAN_POINT('Ctrl Pts',(6.1224241525805,4.64815750403779,30.195776661399));
#184120=CARTESIAN_POINT('Ctrl Pts',(3.18238353293971,7.01141747097681,30.3544441266854));
#184121=CARTESIAN_POINT('Ctrl Pts',(-0.571626804727882,7.68017846246866,
30.5131115919718));
#184122=CARTESIAN_POINT('Ctrl Pts',(-4.16609656841948,6.46904944265926,
30.6717790572583));
#184123=CARTESIAN_POINT('Ctrl Pts',(-6.7557128041372,3.69759961694983,30.8304465225447));
#184124=CARTESIAN_POINT('Ctrl Pts',(-7.69983957956182,0.00321746143552028,
30.9891139878311));
#184125=CARTESIAN_POINT('Ctrl Pts',(-6.76453337409805,-3.65110037073176,
31.1477814531175));
#184126=CARTESIAN_POINT('Ctrl Pts',(-3.33969252180603,-7.43091700234533,
31.3593380734995));
#184127=CARTESIAN_POINT('Ctrl Pts',(2.16491981449567,-7.84574302989205,
31.5708946938813));
#184128=CARTESIAN_POINT('Ctrl Pts',(6.11194997629257,-4.65559940896827,
31.7824513142633));
#184129=CARTESIAN_POINT('Ctrl Pts',(8.1389528136781,-0.00293104366579359,
31.9940079346452));
#184130=CARTESIAN_POINT('Ctrl Pts',(6.27674381516078,5.19370394947507,32.2055645550271));
#184131=CARTESIAN_POINT('Ctrl Pts',(1.72293424764504,7.49139127697494,32.417121175409));
#184132=CARTESIAN_POINT('Ctrl Pts',(-2.04854652132436,7.42233097167019,
32.5757886406954));
#184133=CARTESIAN_POINT('Ctrl Pts',(-5.3593850637147,5.53072239025633,32.7344561059818));
#184134=CARTESIAN_POINT('Ctrl Pts',(-7.34333158641618,2.29792134785086,
32.8931235712683));
#184135=CARTESIAN_POINT('Ctrl Pts',(-7.55608233136559,-1.48913337914222,
33.0517910365546));
#184136=CARTESIAN_POINT('Ctrl Pts',(-5.91410559981757,-4.93060796020649,
33.2104585018412));
#184137=CARTESIAN_POINT('Ctrl Pts',(-2.85474212844216,-7.13721886077074,
33.3691259671275));
#184138=CARTESIAN_POINT('Ctrl Pts',(2.19652445630305,-7.84521216722752,
33.5806825875095));
#184139=CARTESIAN_POINT('Ctrl Pts',(6.6888103943495,-4.63706555946082,33.7922392078914));
#184140=CARTESIAN_POINT('Ctrl Pts',(7.67555673261799,0.341126389848561,
34.0037958282733));
#184141=CARTESIAN_POINT('Ctrl Pts',(6.25107936750864,5.21215581457453,34.2153524486552));
#184142=CARTESIAN_POINT('Ctrl Pts',(1.49190622722631,8.00913787152622,34.4269090690371));
#184143=CARTESIAN_POINT('Ctrl Pts',(-3.47663824415704,6.85583198493872,
34.638465689419));
#184144=CARTESIAN_POINT('Ctrl Pts',(-6.32818873489555,4.38652108607564,
34.7971331547054));
#184145=CARTESIAN_POINT('Ctrl Pts',(-7.65839445044915,0.812953172440143,
34.9558006199919));
#184146=CARTESIAN_POINT('Ctrl Pts',(-7.11052832819302,-2.94029729839196,
35.1144680852783));
#184147=CARTESIAN_POINT('Ctrl Pts',(-4.84761807313768,-5.98435438758767,
35.2731355505647));
#184148=CARTESIAN_POINT('Ctrl Pts',(-1.38202601009292,-7.57479663162461,
35.4318030158511));
#184149=CARTESIAN_POINT('Ctrl Pts',(2.38071170131004,-7.30901207289255,
35.5904704811375));
#184150=CARTESIAN_POINT('Ctrl Pts',(6.71273676997582,-4.61640971892303,
35.8020271015195));
#184151=CARTESIAN_POINT('Ctrl Pts',(8.10660407544666,0.724935761462476,
36.0135837219014));
#184152=CARTESIAN_POINT('Ctrl Pts',(5.67484912542736,5.179442612205,36.2251403422833));
#184153=CARTESIAN_POINT('Ctrl Pts',(1.46037909675127,8.00686295549433,36.4366969626652));
#184154=CARTESIAN_POINT('Ctrl Pts',(-3.9857309816301,7.10535165759066,36.648253583047));
#184155=CARTESIAN_POINT('Ctrl Pts',(-7.06175694946863,3.03661562814189,
36.859810203429));
#184156=CARTESIAN_POINT('Ctrl Pts',(-7.66919668536809,-0.686266787906841,
37.0184776687154));
#184157=CARTESIAN_POINT('Ctrl Pts',(-6.40105915860065,-4.28232881354824,
37.1771451340019));
#184158=CARTESIAN_POINT('Ctrl Pts',(-3.57579413059405,-6.81312392699381,
37.3358125992882));
#184159=CARTESIAN_POINT('Ctrl Pts',(0.111944747556397,-7.70060820927449,
37.4944800645747));
#184160=CARTESIAN_POINT('Ctrl Pts',(3.79182789387702,-6.7014611187607,37.6531475298611));
#184161=CARTESIAN_POINT('Ctrl Pts',(6.51062944971077,-4.08670403320362,
37.8118149951476));
#184162=CARTESIAN_POINT('Ctrl Pts',(8.11174144370636,0.756124583920268,
38.0233716155295));
#184163=CARTESIAN_POINT('Ctrl Pts',(5.759917035209,5.75029714378351,38.2349282359114));
#184164=CARTESIAN_POINT('Ctrl Pts',(1.03889993861408,7.61257021557348,38.4464848562933));
#184165=CARTESIAN_POINT('Ctrl Pts',(-4.00848047528635,7.08340636795202,
38.6580414766752));
#184166=CARTESIAN_POINT('Ctrl Pts',(-7.61250594272741,2.90203840565421,
38.8695980970571));
#184167=CARTESIAN_POINT('Ctrl Pts',(-7.36759278273956,-2.19272029090994,
39.081154717439));
#184168=CARTESIAN_POINT('Ctrl Pts',(-5.44884370079305,-5.44037151556518,
39.2398221827254));
#184169=CARTESIAN_POINT('Ctrl Pts',(-2.17125061230263,-7.38901679506997,
39.3984896480118));
#184170=CARTESIAN_POINT('Ctrl Pts',(1.61943908025456,-7.5221259211948,39.5571571132983));
#184171=CARTESIAN_POINT('Ctrl Pts',(5.01952355125543,-5.84091446073667,
39.7158245785847));
#184172=CARTESIAN_POINT('Ctrl Pts',(7.20486273325817,-2.71615406373658,
39.8744920438711));
#184173=CARTESIAN_POINT('Ctrl Pts',(7.61719255798237,1.03335532178548,40.0331595091576));
#184174=CARTESIAN_POINT('Ctrl Pts',(5.74387974563822,5.77753572932256,40.2447161295394));
#184175=CARTESIAN_POINT('Ctrl Pts',(0.738485251829574,8.10538099210179,
40.4562727499214));
#184176=CARTESIAN_POINT('Ctrl Pts',(-4.07948538963533,6.51063263632969,
40.6678293703032));
#184177=CARTESIAN_POINT('Ctrl Pts',(-7.61591356952583,2.870613522543,40.8793859906852));
#184178=CARTESIAN_POINT('Ctrl Pts',(-7.70424556772878,-2.64890050173359,
41.0909426110671));
#184179=CARTESIAN_POINT('Ctrl Pts',(-4.25212411721605,-6.40381809378092,
41.302499231449));
#184180=CARTESIAN_POINT('Ctrl Pts',(-0.698199749211469,-7.66811952262341,
41.4611666967354));
#184181=CARTESIAN_POINT('Ctrl Pts',(3.06682613053423,-7.06445156430003,
41.6198341620219));
#184182=CARTESIAN_POINT('Ctrl Pts',(6.06264997198326,-4.7380625392818,41.7785016273082));
#184183=CARTESIAN_POINT('Ctrl Pts',(7.59617568540101,-1.2688630248439,41.9371690925948));
#184184=CARTESIAN_POINT('Ctrl Pts',(7.27216036790802,2.5304591453817,42.0958365578811));
#184185=CARTESIAN_POINT('Ctrl Pts',(5.18654399681884,5.67355330066163,42.2545040231676));
#184186=CARTESIAN_POINT('Ctrl Pts',(0.708720574174565,8.1160205017057,42.4660606435494));
#184187=CARTESIAN_POINT('Ctrl Pts',(-4.62587847535394,6.69655208480938,
42.6776172639315));
#184188=CARTESIAN_POINT('Ctrl Pts',(-7.30347153926227,2.38533893724051,
42.8891738843132));
#184189=CARTESIAN_POINT('Ctrl Pts',(-7.68672892077909,-2.67521213964834,
43.1007305046952));
#184190=CARTESIAN_POINT('Ctrl Pts',(-4.21834853492501,-6.96976393224585,
43.3122871250771));
#184191=CARTESIAN_POINT('Ctrl Pts',(0.837912334877082,-7.64116147006215,
43.523843745459));
#184192=CARTESIAN_POINT('Ctrl Pts',(4.37666868245361,-6.33500679817317,
43.6825112107454));
#184193=CARTESIAN_POINT('Ctrl Pts',(6.88075439776222,-3.45935215907542,
43.8411786760319));
#184194=CARTESIAN_POINT('Ctrl Pts',(7.69053539056388,0.246224875170558,
43.9998461413183));
#184195=CARTESIAN_POINT('Ctrl Pts',(6.64537580266269,3.89241298724387,44.1585136066047));
#184196=CARTESIAN_POINT('Ctrl Pts',(3.96246964786781,6.60199774895939,44.3171810718911));
#184197=CARTESIAN_POINT('Ctrl Pts',(0.347409143152186,7.67911142654452,
44.4758485371776));
#184198=CARTESIAN_POINT('Ctrl Pts',(-4.65554868102627,6.68565186837957,
44.6874051575595));
#184199=CARTESIAN_POINT('Ctrl Pts',(-7.84211327267865,2.17803117485824,
44.8989617779414));
#184200=CARTESIAN_POINT('Ctrl Pts',(-7.13592936403309,-2.84763950959403,
45.1105183983233));
#184201=CARTESIAN_POINT('Ctrl Pts',(-4.18804171334091,-6.97874416437295,
45.3220750187052));
#184202=CARTESIAN_POINT('Ctrl Pts',(1.22643156032289,-8.0540630210437,45.5336316390871));
#184203=CARTESIAN_POINT('Ctrl Pts',(5.53884603322342,-5.33016325057911,
45.745188259469));
#184204=CARTESIAN_POINT('Ctrl Pts',(7.41913356266724,-2.06009249532456,
45.9038557247554));
#184205=CARTESIAN_POINT('Ctrl Pts',(7.49945377603941,1.7521715272814,46.0625231900418));
#184206=CARTESIAN_POINT('Ctrl Pts',(5.74714801752916,5.11617676219574,46.2211906553283));
#184207=CARTESIAN_POINT('Ctrl Pts',(2.6086540375764,7.2461526559958,46.3798581206147));
#184208=CARTESIAN_POINT('Ctrl Pts',(-1.18729111807959,7.60776844155002,
46.5385255859012));
#184209=CARTESIAN_POINT('Ctrl Pts',(-4.6530354610011,6.11867657110869,46.6971930511876));
#184210=CARTESIAN_POINT('Ctrl Pts',(-7.85795028953664,2.1507161815344,46.9087496715695));
#184211=CARTESIAN_POINT('Ctrl Pts',(-7.41661438454468,-3.35202741724084,
47.1203062919514));
#184212=CARTESIAN_POINT('Ctrl Pts',(-3.65474913242218,-6.75811145769161,
47.3318629123333));
#184213=CARTESIAN_POINT('Ctrl Pts',(1.25567377349499,-8.04189360643028,
47.5434195327152));
#184214=CARTESIAN_POINT('Ctrl Pts',(6.10125319775964,-5.39757589381113,
47.754976153097));
#184215=CARTESIAN_POINT('Ctrl Pts',(7.66823461842726,-0.544854982878747,
47.9665327734791));
#184216=CARTESIAN_POINT('Ctrl Pts',(7.01522080271856,3.17330309778602,48.1252002387653));
#184217=CARTESIAN_POINT('Ctrl Pts',(4.63782808188847,6.14647671576517,48.283867704052));
#184218=CARTESIAN_POINT('Ctrl Pts',(1.13077753391832,7.61703785226467,48.4425351693382));
#184219=CARTESIAN_POINT('Ctrl Pts',(-2.63192688181473,7.22274098829433,
48.6012026346247));
#184220=CARTESIAN_POINT('Ctrl Pts',(-6.85224275112629,4.39256931968361,
48.8127592550066));
#184221=CARTESIAN_POINT('Ctrl Pts',(-8.40794340526699,-2.35691386019897,
49.077205030484));
#184222=CARTESIAN_POINT('Ctrl Pts',(-2.55778717345702,-8.35115505806219,
49.3945399610569));
#184223=CARTESIAN_POINT('Ctrl Pts',(4.23015017580366,-6.95257930116764,
49.6589857365342));
#184224=CARTESIAN_POINT('Ctrl Pts',(7.1558958925893,-2.80581318713367,49.8705423569161));
#184225=CARTESIAN_POINT('Ctrl Pts',(7.64635109302848,0.955302332272822,
50.0292098222026));
#184226=CARTESIAN_POINT('Ctrl Pts',(6.24646267211259,4.47907133945649,50.1878772874891));
#184227=CARTESIAN_POINT('Ctrl Pts',(2.3888706505773,7.78053435803256,50.3994339078708));
#184228=CARTESIAN_POINT('Ctrl Pts',(-4.53046435773524,7.46339375383813,
50.6638796833484));
#184229=CARTESIAN_POINT('Ctrl Pts',(-8.73429526383473,0.220108920083938,
50.9812146139211));
#184230=CARTESIAN_POINT('Ctrl Pts',(-5.55301875409966,-5.94902376600732,
51.2456603893986));
#184231=CARTESIAN_POINT('Ctrl Pts',(-0.785796613400711,-7.64007724274336,
51.4572170097804));
#184232=CARTESIAN_POINT('Ctrl Pts',(4.24848612041541,-6.94696649308868,
51.6687736301623));
#184233=CARTESIAN_POINT('Ctrl Pts',(7.70417260804807,-2.64235740086951,
51.8803302505443));
#184234=CARTESIAN_POINT('Ctrl Pts',(7.29030095876973,2.43920654419265,52.0918868709261));
#184235=CARTESIAN_POINT('Ctrl Pts',(5.26189995080857,5.62130885552968,52.2505543362126));
#184236=CARTESIAN_POINT('Ctrl Pts',(1.92117852419122,7.45782167166676,52.409221801499));
#184237=CARTESIAN_POINT('Ctrl Pts',(-1.87221591806992,7.46335962794256,
52.5678892667854));
#184238=CARTESIAN_POINT('Ctrl Pts',(-5.21349836513446,5.66833611529721,
52.7265567320719));
#184239=CARTESIAN_POINT('Ctrl Pts',(-7.29236341282212,2.47176373057108,
52.8852241973583));
#184240=CARTESIAN_POINT('Ctrl Pts',(-7.5780129013641,-1.28955379830699,
53.0438916626446));
#184241=CARTESIAN_POINT('Ctrl Pts',(-5.54586987187687,-5.96786612029453,
53.2554482830267));
#184242=CARTESIAN_POINT('Ctrl Pts',(-0.464829181575225,-8.12567368653735,
53.4670049034085));
#184243=CARTESIAN_POINT('Ctrl Pts',(4.29663544586798,-6.36941225506916,
53.6785615237905));
#184244=CARTESIAN_POINT('Ctrl Pts',(7.70835491807636,-2.61225392038938,
53.8901181441723));
#184245=CARTESIAN_POINT('Ctrl Pts',(7.61057224416527,2.90710352379302,54.1016747645543));
#184246=CARTESIAN_POINT('Ctrl Pts',(4.03383745202061,6.54351587573162,54.3132313849361));
#184247=CARTESIAN_POINT('Ctrl Pts',(0.439312887650428,7.68729779242562,
54.4718988502226));
#184248=CARTESIAN_POINT('Ctrl Pts',(-3.30322330506354,6.95705479782095,
54.630566315509));
#184249=CARTESIAN_POINT('Ctrl Pts',(-6.21892296661873,4.53099989847321,
54.7892337807954));
#184250=CARTESIAN_POINT('Ctrl Pts',(-7.63463143902492,1.0120773019643,54.9479012460819));
#184251=CARTESIAN_POINT('Ctrl Pts',(-7.18272645166355,-2.77416309048803,
55.1065687113683));
#184252=CARTESIAN_POINT('Ctrl Pts',(-4.99234271294018,-5.84516551627964,
55.2652361766548));
#184253=CARTESIAN_POINT('Ctrl Pts',(-0.434729445610179,-8.13529863268552,
55.4767927970366));
#184254=CARTESIAN_POINT('Ctrl Pts',(4.84898798431694,-6.53680939820729,
55.6883494174187));
#184255=CARTESIAN_POINT('Ctrl Pts',(7.37972971975833,-2.13778567704362,
55.8999060378003));
#184256=CARTESIAN_POINT('Ctrl Pts',(7.59217979546274,2.93280880106663,56.1114626581825));
#184257=CARTESIAN_POINT('Ctrl Pts',(3.98100268887075,7.10800191541319,56.3230192785642));
#184258=CARTESIAN_POINT('Ctrl Pts',(-1.0950171302903,7.60857300457776,56.5345758989462));
#184259=CARTESIAN_POINT('Ctrl Pts',(-4.58773225049471,6.18387036607666,
56.6932433642326));
#184260=CARTESIAN_POINT('Ctrl Pts',(-6.99345745083907,3.22543815637297,
56.851910829519));
#184261=CARTESIAN_POINT('Ctrl Pts',(-7.6778644541053,-0.505330321822897,
57.0105782948054));
#184262=CARTESIAN_POINT('Ctrl Pts',(-6.5103870715291,-4.11421421390834,
57.1692457600919));
#184263=CARTESIAN_POINT('Ctrl Pts',(-3.73766650931412,-6.73181914256119,
57.3279132253782));
#184264=CARTESIAN_POINT('Ctrl Pts',(-0.0883513982762259,-7.68645820368191,
57.4865806906648));
#184265=CARTESIAN_POINT('Ctrl Pts',(4.87827385335432,-6.52491516017783,
57.6981373110465));
#184266=CARTESIAN_POINT('Ctrl Pts',(7.91107710357185,-1.91243837957983,
57.9096939314286));
#184267=CARTESIAN_POINT('Ctrl Pts',(7.03588074418887,3.08657099756842,58.1212505518105));
#184268=CARTESIAN_POINT('Ctrl Pts',(3.95041052253477,7.11595518519746,58.3328071721923));
#184269=CARTESIAN_POINT('Ctrl Pts',(-1.49723462369259,8.00814348757412,
58.5443637925744));
#184270=CARTESIAN_POINT('Ctrl Pts',(-5.71537578392953,5.14042073520366,
58.7559204129561));
#184271=CARTESIAN_POINT('Ctrl Pts',(-7.48436284634017,1.80882632869221,
58.9145878782426));
#184272=CARTESIAN_POINT('Ctrl Pts',(-7.43612494719741,-2.00398208298336,
59.073255343529));
#184273=CARTESIAN_POINT('Ctrl Pts',(-5.5714200206841,-5.30699917675582,
59.2319228088155));
#184274=CARTESIAN_POINT('Ctrl Pts',(-2.36290057339191,-7.32997948834203,
59.3905902741018));
#184275=CARTESIAN_POINT('Ctrl Pts',(1.4430614392871,-7.56340621581888,59.5492577393884));
#184276=CARTESIAN_POINT('Ctrl Pts',(4.85666785110194,-5.95837419691958,
59.7079252046747));
#184277=CARTESIAN_POINT('Ctrl Pts',(7.92594289223697,-1.8845431555021,59.9194818250565));
#184278=CARTESIAN_POINT('Ctrl Pts',(7.29948277548688,3.60001565339179,60.1310384454387));
#184279=CARTESIAN_POINT('Ctrl Pts',(3.42476508248566,6.87761023170662,60.3425950658204));
#184280=CARTESIAN_POINT('Ctrl Pts',(-1.52581916105486,7.99465054783844,
60.5541516862024));
#184281=CARTESIAN_POINT('Ctrl Pts',(-6.28019795748342,5.18952668851147,
60.7657083065843));
#184282=CARTESIAN_POINT('Ctrl Pts',(-7.68167340827104,0.285200517365215,
60.9772649269661));
#184283=CARTESIAN_POINT('Ctrl Pts',(-6.90546418446714,-3.40618618106626,
61.1359323922526));
#184284=CARTESIAN_POINT('Ctrl Pts',(-4.42566351984426,-6.30280896334092,
61.294599857539));
#184285=CARTESIAN_POINT('Ctrl Pts',(-0.877763597793129,-7.64424570349199,
61.4532673228255));
#184286=CARTESIAN_POINT('Ctrl Pts',(2.88185101533245,-7.1419068283392,61.6119347881118));
#184287=CARTESIAN_POINT('Ctrl Pts',(5.95367192347783,-4.88275849603854,
61.7706022533983));
#184288=CARTESIAN_POINT('Ctrl Pts',(7.54638607366438,-1.46338747898439,
61.9292697186847));
#184289=CARTESIAN_POINT('Ctrl Pts',(7.29302522198898,3.63095810322632,62.1408263390666));
#184290=CARTESIAN_POINT('Ctrl Pts',(3.29821233539819,7.44072287381559,62.3523829594485));
#184291=CARTESIAN_POINT('Ctrl Pts',(-1.77671591692733,7.47487919099873,
62.5639395798305));
#184292=CARTESIAN_POINT('Ctrl Pts',(-6.29350100357757,5.16085328334994,
62.7754962002123));
#184293=CARTESIAN_POINT('Ctrl Pts',(-8.14681260604421,-0.0389614931836734,
62.9870528205943));
#184294=CARTESIAN_POINT('Ctrl Pts',(-6.08081625560616,-4.70245886234001,
63.1986094409762));
#184295=CARTESIAN_POINT('Ctrl Pts',(-3.1198606493378,-7.03946087649886,
63.3572769062625));
#184296=CARTESIAN_POINT('Ctrl Pts',(0.639952549886159,-7.67478723829821,
63.515944371549));
#184297=CARTESIAN_POINT('Ctrl Pts',(4.22350174629681,-6.43171783491736,
63.6746118368354));
#184298=CARTESIAN_POINT('Ctrl Pts',(6.78835140935033,-3.6373319290962,63.8332793021219));
#184299=CARTESIAN_POINT('Ctrl Pts',(7.69956330106161,0.0653060180248196,
63.9919467674083));
#184300=CARTESIAN_POINT('Ctrl Pts',(6.73177318227711,3.71115554899262,64.1506142326947));
#184301=CARTESIAN_POINT('Ctrl Pts',(3.27343014738359,7.46034373914179,64.3621708530767));
#184302=CARTESIAN_POINT('Ctrl Pts',(-2.23465587805173,7.82616602181326,
64.5737274734585));
#184303=CARTESIAN_POINT('Ctrl Pts',(-6.15313962301333,4.60102283728218,
64.7852840938405));
#184304=CARTESIAN_POINT('Ctrl Pts',(-8.13865659747939,-0.0695002345335011,
64.9968407142223));
#184305=CARTESIAN_POINT('Ctrl Pts',(-6.23027481366242,-5.24935704464801,
65.2083973346043));
#184306=CARTESIAN_POINT('Ctrl Pts',(-1.65619771640194,-7.50642756646789,
65.4199539549862));
#184307=CARTESIAN_POINT('Ctrl Pts',(2.11451911297346,-7.40380637401568,
65.5786214202726));
#184308=CARTESIAN_POINT('Ctrl Pts',(5.40839251305042,-5.48280848142911,
65.737288885559));
#184309=CARTESIAN_POINT('Ctrl Pts',(7.36349073440769,-2.23247967812894,
65.8959563508455));
#184310=CARTESIAN_POINT('Ctrl Pts',(7.54253083489441,1.55631841983495,66.0546238161318));
#184311=CARTESIAN_POINT('Ctrl Pts',(5.86999233463708,4.98304423965384,66.2132912814184));
#184312=CARTESIAN_POINT('Ctrl Pts',(2.79111267227769,7.16234149821795,66.3719587467047));
#184313=CARTESIAN_POINT('Ctrl Pts',(-2.26625454400543,7.82535392028544,
66.5835153670866));
#184314=CARTESIAN_POINT('Ctrl Pts',(-6.72981225884627,4.57735605508002,
66.7950719874686));
#184315=CARTESIAN_POINT('Ctrl Pts',(-7.67221698888851,-0.409420132503432,
67.0066286078505));
#184316=CARTESIAN_POINT('Ctrl Pts',(-6.20444717322626,-5.26757978287376,
67.2181852282322));
#184317=CARTESIAN_POINT('Ctrl Pts',(-1.42057125095667,-8.02209766563004,
67.4297418486144));
#184318=CARTESIAN_POINT('Ctrl Pts',(3.53751282681393,-6.82462077236317,
67.6412984689961));
#184319=CARTESIAN_POINT('Ctrl Pts',(6.36697520396691,-4.33003079147432,
67.7999659342826));
#184320=CARTESIAN_POINT('Ctrl Pts',(7.66532591202258,-0.744766461198532,
67.9586333995689));
#184321=CARTESIAN_POINT('Ctrl Pts',(7.08408010050368,3.00345974479668,68.1173008648555));
#184322=CARTESIAN_POINT('Ctrl Pts',(4.79416941179473,6.02725792299139,68.2759683301418));
#184323=CARTESIAN_POINT('Ctrl Pts',(1.31456072762026,7.5867957660954,68.4346357954283));
#184324=CARTESIAN_POINT('Ctrl Pts',(-2.44566267792787,7.28753591773205,
68.5933032607148));
#184325=CARTESIAN_POINT('Ctrl Pts',(-6.75355386401727,4.55648810398642,
68.8048598810967));
#184326=CARTESIAN_POINT('Ctrl Pts',(-8.09983161915125,-0.797050334478962,
69.0164165014784));
#184327=CARTESIAN_POINT('Ctrl Pts',(-5.62853087504148,-5.22973981744729,
69.2279731218606));
#184328=CARTESIAN_POINT('Ctrl Pts',(-1.38906561415854,-8.0195422695973,
69.4395297422423));
#184329=CARTESIAN_POINT('Ctrl Pts',(4.04880596026311,-7.06959998388101,
69.6510863626243));
#184330=CARTESIAN_POINT('Ctrl Pts',(7.08850112603248,-2.97365052968238,
69.8626429830061));
#184331=CARTESIAN_POINT('Ctrl Pts',(7.66278567794466,0.754490262979475,
70.0213104482926));
#184332=CARTESIAN_POINT('Ctrl Pts',(6.36269585507655,4.33912432122458,70.1799779135791));
#184333=CARTESIAN_POINT('Ctrl Pts',(3.51502034613637,6.84467627249188,70.3386453788654));
#184334=CARTESIAN_POINT('Ctrl Pts',(-0.180470506905408,7.69930703475246,
70.4973128441519));
#184335=CARTESIAN_POINT('Ctrl Pts',(-3.85131619905127,6.66745104503739,
70.6559803094382));
#184336=CARTESIAN_POINT('Ctrl Pts',(-6.54674052566976,4.02860201260901,
70.8146477747248));
#184337=CARTESIAN_POINT('Ctrl Pts',(-8.10469122459747,-0.828283640961824,
71.0262043951065));
#184338=CARTESIAN_POINT('Ctrl Pts',(-5.70851519784241,-5.80132879005301,
71.2377610154887));
#184339=CARTESIAN_POINT('Ctrl Pts',(-0.971112084560053,-7.6215142648105,
71.4493176358703));
#184340=CARTESIAN_POINT('Ctrl Pts',(4.07135925484543,-7.0474531082001,71.6608742562524));
#184341=CARTESIAN_POINT('Ctrl Pts',(7.63803066372684,-2.83417734376672,
71.8724308766342));
#184342=CARTESIAN_POINT('Ctrl Pts',(7.34778730389881,2.25820004054282,72.0839874970162));
#184343=CARTESIAN_POINT('Ctrl Pts',(5.40021230982589,5.48864709303213,72.2426549623026));
#184344=CARTESIAN_POINT('Ctrl Pts',(2.10540739132609,7.40804685027035,72.401322427589));
#184345=CARTESIAN_POINT('Ctrl Pts',(-1.68631677184475,7.50741613699158,
72.5599898928755));
#184346=CARTESIAN_POINT('Ctrl Pts',(-5.07130495815068,5.79601280542814,
72.7186573581618));
#184347=CARTESIAN_POINT('Ctrl Pts',(-7.22874935220666,2.6519281110198,72.8773248234484));
#184348=CARTESIAN_POINT('Ctrl Pts',(-7.60769475727116,-1.10110225076198,
73.0359922887348));
#184349=CARTESIAN_POINT('Ctrl Pts',(-5.69223613839982,-5.82842357594631,
73.2475489091166));
#184350=CARTESIAN_POINT('Ctrl Pts',(-0.666323612318729,-8.11163203911284,
73.4591055294986));
#184351=CARTESIAN_POINT('Ctrl Pts',(4.1372640595256,-6.47407016267561,73.6706621498805));
#184352=CARTESIAN_POINT('Ctrl Pts',(7.64115849542936,-2.80272337950486,
73.8822187702623));
#184353=CARTESIAN_POINT('Ctrl Pts',(7.68036706291875,2.71735816829225,74.0937753906443));
#184354=CARTESIAN_POINT('Ctrl Pts',(4.19496609468124,6.44140552604157,74.3053320110261));
#184355=CARTESIAN_POINT('Ctrl Pts',(0.629931035627467,7.67402937141879,
74.4639994763127));
#184356=CARTESIAN_POINT('Ctrl Pts',(-3.1295735144678,7.03687914041394,74.622666941599));
#184357=CARTESIAN_POINT('Ctrl Pts',(-6.10457543692591,4.68392143869292,
74.7813344068855));
#184358=CARTESIAN_POINT('Ctrl Pts',(-7.60716689941602,1.20121196450923,
74.9400018721718));
#184359=CARTESIAN_POINT('Ctrl Pts',(-7.24935302134104,-2.59507623684127,
75.0986693374583));
#184360=CARTESIAN_POINT('Ctrl Pts',(-5.13584783304834,-5.71948535466407,
75.2573368027448));
#184361=CARTESIAN_POINT('Ctrl Pts',(-0.636465428932352,-8.12200624191624,
75.4688934231266));
#184362=CARTESIAN_POINT('Ctrl Pts',(4.6852900652918,-6.65511972081445,75.6804500435086));
#184363=CARTESIAN_POINT('Ctrl Pts',(7.32441022294305,-2.32024853313952,
75.8920066638904));
#184364=CARTESIAN_POINT('Ctrl Pts',(7.66261695397957,2.74351287784116,76.1035632842725));
#184365=CARTESIAN_POINT('Ctrl Pts',(4.1561553154331,7.00702837370805,76.3151199046541));
#184366=CARTESIAN_POINT('Ctrl Pts',(-0.905880310180398,7.63340202989932,
76.5266765250363));
#184367=CARTESIAN_POINT('Ctrl Pts',(-4.43287263356147,6.29580655020996,
76.6853439903225));
#184368=CARTESIAN_POINT('Ctrl Pts',(-6.91126780954659,3.39798111883746,
76.844011455609));
#184369=CARTESIAN_POINT('Ctrl Pts',(-7.68803961465247,-0.314655672919856,
77.0026789208954));
#184370=CARTESIAN_POINT('Ctrl Pts',(-6.61047280731541,-3.95139819342403,
77.1613463861817));
#184371=CARTESIAN_POINT('Ctrl Pts',(-3.90355943744507,-6.63699959480023,
77.3200138514683));
#184372=CARTESIAN_POINT('Ctrl Pts',(-0.279056488784278,-7.68189905964088,
77.4786813167547));
#184373=CARTESIAN_POINT('Ctrl Pts',(4.71486206543706,-6.64395585023371,
77.6902379371367));
#184374=CARTESIAN_POINT('Ctrl Pts',(7.86118577758629,-2.10815551242545,
77.9017945575185));
#184375=CARTESIAN_POINT('Ctrl Pts',(7.1103046633451,2.91103176964826,78.1133511779004));
#184376=CARTESIAN_POINT('Ctrl Pts',(4.12576992113469,7.01573831126531,78.3249077982824));
#184377=CARTESIAN_POINT('Ctrl Pts',(-1.29805898481169,8.04283013048902,
78.5364644186642));
#184378=CARTESIAN_POINT('Ctrl Pts',(-5.58606117719495,5.28065963787479,
78.7480210390462));
#184379=CARTESIAN_POINT('Ctrl Pts',(-7.43717394913015,1.9939868488595,78.9066885043326));
#184380=CARTESIAN_POINT('Ctrl Pts',(-7.48356218982991,-1.81884451512464,
79.065355969619));
#184381=CARTESIAN_POINT('Ctrl Pts',(-5.70139272677566,-5.16711547036028,
79.2240234349055));
#184382=CARTESIAN_POINT('Ctrl Pts',(-2.54405960589992,-7.26908929239964,
79.3826909001919));
#184383=CARTESIAN_POINT('Ctrl Pts',(1.25493822205205,-7.59688554355514,
79.5413583654783));
#184384=CARTESIAN_POINT('Ctrl Pts',(4.70732090191969,-6.07705320141218,
79.7000258307647));
#184385=CARTESIAN_POINT('Ctrl Pts',(7.87673918281708,-2.08063775843527,
79.9115824511467));
#184386=CARTESIAN_POINT('Ctrl Pts',(7.38656617778034,3.41777728876049,80.1231390715286));
#184387=CARTESIAN_POINT('Ctrl Pts',(3.59437202808532,6.79051014970209,80.3346956919104));
#184388=CARTESIAN_POINT('Ctrl Pts',(-1.32696953524914,8.03005064410032,
80.5462523122924));
#184389=CARTESIAN_POINT('Ctrl Pts',(-6.14949091428842,5.34376600638882,
80.7578089326743));
#184390=CARTESIAN_POINT('Ctrl Pts',(-7.67223111015648,0.475726264558584,
80.969365553056));
#184391=CARTESIAN_POINT('Ctrl Pts',(-6.98785921386535,-3.23378470375526,
81.1280330183426));
#184392=CARTESIAN_POINT('Ctrl Pts',(-4.58069911474279,-6.19104951033711,
81.2867004836291));
#184393=CARTESIAN_POINT('Ctrl Pts',(-1.06717815149796,-7.62011102950162,
81.4453679489154));
#184394=CARTESIAN_POINT('Ctrl Pts',(2.70374388560553,-7.21121816479727,
81.6040354142019));
#184395=CARTESIAN_POINT('Ctrl Pts',(5.83067758974013,-5.0289898337089,81.7627028794884));
#184396=CARTESIAN_POINT('Ctrl Pts',(7.50774982153899,-1.65019341400493,
81.9213703447746));
#184397=CARTESIAN_POINT('Ctrl Pts',(7.38087842071822,3.44887044907858,82.1329269651568));
#184398=CARTESIAN_POINT('Ctrl Pts',(3.48183136396736,7.35658968865254,82.3444835855383));
#184399=CARTESIAN_POINT('Ctrl Pts',(-1.59068667761081,7.51666510250124,
82.5560402059206));
#184400=CARTESIAN_POINT('Ctrl Pts',(-6.16350136797752,5.31543153292694,
82.7675968263023));
#184401=CARTESIAN_POINT('Ctrl Pts',(-8.14527086207023,0.163206064415523,
82.9791534466843));
#184402=CARTESIAN_POINT('Ctrl Pts',(-6.19563100587296,-4.55012111108156,
83.1907100670662));
#184403=CARTESIAN_POINT('Ctrl Pts',(-3.29357765288929,-6.95987687731857,
83.3493775323525));
#184404=CARTESIAN_POINT('Ctrl Pts',(0.449312806791323,-7.68830387152485,
83.508044997639));
#184405=CARTESIAN_POINT('Ctrl Pts',(4.06260417818805,-6.5345396624655,83.6667124629256));
#184406=CARTESIAN_POINT('Ctrl Pts',(6.69600416344681,-3.80465854740654,
83.8253799282118));
#184407=CARTESIAN_POINT('Ctrl Pts',(7.69881298730476,-0.125771576888246,
83.9840473934985));
#184408=CARTESIAN_POINT('Ctrl Pts',(6.82178922456726,3.54297014692783,84.1427148587846));
#184409=CARTESIAN_POINT('Ctrl Pts',(3.45754368027798,7.3768194592874,84.3542714791668));
#184410=CARTESIAN_POINT('Ctrl Pts',(-2.03976877626405,7.87920711960751,
84.5658280995486));
#184411=CARTESIAN_POINT('Ctrl Pts',(-6.0370748776523,4.75229053100797,84.7773847199304));
#184412=CARTESIAN_POINT('Ctrl Pts',(-8.13787515527384,0.132474342694702,
84.9889413403124));
#184413=CARTESIAN_POINT('Ctrl Pts',(-6.35861431178935,-5.09314221967737,
85.2004979606943));
#184414=CARTESIAN_POINT('Ctrl Pts',(-1.84195274888236,-7.46301921190938,
85.4120545810761));
#184415=CARTESIAN_POINT('Ctrl Pts',(1.93014946421949,-7.45399644142782,
85.5707220463626));
#184416=CARTESIAN_POINT('Ctrl Pts',(5.27067639873185,-5.61532445359144,
85.7293895116489));
#184417=CARTESIAN_POINT('Ctrl Pts',(7.30582649274669,-2.41451041970134,
85.8880569769355));
#184418=CARTESIAN_POINT('Ctrl Pts',(7.57882695690173,1.36867833203807,86.046724442222));
#184419=CARTESIAN_POINT('Ctrl Pts',(5.99183446563274,4.8358514906375,86.2053919075083));
#184420=CARTESIAN_POINT('Ctrl Pts',(2.96798007080302,7.09087723668659,86.3640593727949));
#184421=CARTESIAN_POINT('Ctrl Pts',(-2.07137786401307,7.87917935957984,
86.5756159931766));
#184422=CARTESIAN_POINT('Ctrl Pts',(-6.6141572156696,4.74294063010507,86.7871726135587));
#184423=CARTESIAN_POINT('Ctrl Pts',(-7.68001396649197,-0.218915152460824,
86.9987292339403));
#184424=CARTESIAN_POINT('Ctrl Pts',(-6.33324680436952,-5.11200023564539,
87.2102858543225));
#184425=CARTESIAN_POINT('Ctrl Pts',(-1.61919470951296,-7.98437737889667,
87.4218424747043));
#184426=CARTESIAN_POINT('Ctrl Pts',(3.36707696578925,-6.91029944307013,
87.633399095086));
#184427=CARTESIAN_POINT('Ctrl Pts',(6.25756903013603,-4.4866880587052,87.7920665603727));
#184428=CARTESIAN_POINT('Ctrl Pts',(7.64448494706102,-0.934745052625723,
87.9507340256589));
#184429=CARTESIAN_POINT('Ctrl Pts',(7.1564268500222,2.82675008609669,88.1094014909455));
#184430=CARTESIAN_POINT('Ctrl Pts',(4.94225399548035,5.90643918646504,88.2680689562319));
#184431=CARTESIAN_POINT('Ctrl Pts',(1.50241521768622,7.55184006826877,88.4267364215184));
#184432=CARTESIAN_POINT('Ctrl Pts',(-2.26407620763408,7.34597880560986,
88.5854038868047));
#184433=CARTESIAN_POINT('Ctrl Pts',(-6.63840932916552,4.72266823039694,
88.7969605071868));
#184434=CARTESIAN_POINT('Ctrl Pts',(-8.11711560933248,-0.595815138298367,
89.0085171275685));
#184435=CARTESIAN_POINT('Ctrl Pts',(-5.75656887678168,-5.08846274785982,
89.2200737479506));
#184436=CARTESIAN_POINT('Ctrl Pts',(-1.58763536404624,-7.98260455272119,
89.4316303683323));
#184437=CARTESIAN_POINT('Ctrl Pts',(3.87213373292876,-7.16789048397557,
89.6431869887142));
#184438=CARTESIAN_POINT('Ctrl Pts',(7.01253009438418,-3.14862944180495,
89.8547436090961));
#184439=CARTESIAN_POINT('Ctrl Pts',(7.67914815323174,0.564113059378357,
90.0134110743827));
#184440=CARTESIAN_POINT('Ctrl Pts',(6.46840800204212,4.17990386712071,90.172078539669));
#184441=CARTESIAN_POINT('Ctrl Pts',(3.68378227516248,6.75534673115761,90.3307460049555));
#184442=CARTESIAN_POINT('Ctrl Pts',(0.0106361900317569,7.70141449934472,
90.489413470242));
#184443=CARTESIAN_POINT('Ctrl Pts',(-3.6846837331035,6.76096484904669,90.6480809355283));
#184444=CARTESIAN_POINT('Ctrl Pts',(-6.44475867331778,4.18981280359029,
90.8067484008148));
#184445=CARTESIAN_POINT('Ctrl Pts',(-8.12274874381592,-0.626918240957216,
91.0183050211967));
#184446=CARTESIAN_POINT('Ctrl Pts',(-5.85071201863764,-5.65789098243707,
91.2298616415786));
#184447=CARTESIAN_POINT('Ctrl Pts',(-1.1599338352815,-7.59507023452402,
91.4414182619603));
#184448=CARTESIAN_POINT('Ctrl Pts',(3.89522963707608,-7.14631006664979,
91.6529748823425));
#184449=CARTESIAN_POINT('Ctrl Pts',(7.56535131998991,-3.02283526522436,
91.8645315027241));
#184450=CARTESIAN_POINT('Ctrl Pts',(7.40155992882987,2.0751762111144,92.0760881231063));
#184451=CARTESIAN_POINT('Ctrl Pts',(5.53474515720112,5.35295581395318,92.2347555883925));
#184452=CARTESIAN_POINT('Ctrl Pts',(2.28858287920351,7.35352206952492,92.393423053679));
#184453=CARTESIAN_POINT('Ctrl Pts',(-1.49950799427032,7.54694885907257,
92.5520905189655));
#184454=CARTESIAN_POINT('Ctrl Pts',(-4.9259207646105,5.92006782384962,92.710757984252));
#184455=CARTESIAN_POINT('Ctrl Pts',(-7.16071837898484,2.83048621488856,
92.8694254495382));
#184456=CARTESIAN_POINT('Ctrl Pts',(-7.63267504713682,-0.911985347958647,
93.028092914825));
#184457=CARTESIAN_POINT('Ctrl Pts',(-5.83511030861758,-5.68538137855928,
93.2396495352064));
#184458=CARTESIAN_POINT('Ctrl Pts',(-0.867401018586824,-8.0926001287187,
93.4512061555888));
#184459=CARTESIAN_POINT('Ctrl Pts',(3.97534210068024,-6.57473904924924,
93.6627627759704));
#184460=CARTESIAN_POINT('Ctrl Pts',(7.56925871710715,-2.99146858104545,
93.8743193963525));
#184461=CARTESIAN_POINT('Ctrl Pts',(7.74543080651569,2.52594026113027,94.0858760167343));
#184462=CARTESIAN_POINT('Ctrl Pts',(4.35351193806897,6.33532798619646,94.2974326371162));
#184463=CARTESIAN_POINT('Ctrl Pts',(0.820160810623469,7.65603515986074,
94.4561001024026));
#184464=CARTESIAN_POINT('Ctrl Pts',(-2.95399599008719,7.11237001552241,
94.614767567689));
#184465=CARTESIAN_POINT('Ctrl Pts',(-5.98646912853775,4.83395815856167,
94.7734350329756));
#184466=CARTESIAN_POINT('Ctrl Pts',(-7.57501656355332,1.38960755120628,
94.9321024982618));
#184467=CARTESIAN_POINT('Ctrl Pts',(-7.31151710827953,-2.41439254654737,
95.0907699635484));
#184468=CARTESIAN_POINT('Ctrl Pts',(-5.27618675172836,-5.5902806061917,
95.2494374288348));
#184469=CARTESIAN_POINT('Ctrl Pts',(-0.837817077204601,-8.10371735646381,
95.4609940492167));
#184470=CARTESIAN_POINT('Ctrl Pts',(4.51872136352693,-6.76932144471558,
95.6725506695986));
#184471=CARTESIAN_POINT('Ctrl Pts',(7.2645629643043,-2.50129446361673,95.8841072899803));
#184472=CARTESIAN_POINT('Ctrl Pts',(7.72837761593481,2.55255697709665,96.0956639103624));
#184473=CARTESIAN_POINT('Ctrl Pts',(4.32866351814856,6.90168043882907,96.3072205307442));
#184474=CARTESIAN_POINT('Ctrl Pts',(-0.71608079112348,7.65360327302554,
96.5187771511263));
#184475=CARTESIAN_POINT('Ctrl Pts',(-4.27550416892791,6.40371138155931,
96.6774446164126));
#184476=CARTESIAN_POINT('Ctrl Pts',(-6.82439171245445,3.5687316026304,96.836112081699));
#184477=CARTESIAN_POINT('Ctrl Pts',(-7.69429901276673,-0.124358320346745,
96.9947795469856));
#184478=CARTESIAN_POINT('Ctrl Pts',(-6.70494269733832,-3.78507144735772,
97.1534470122718));
#184479=CARTESIAN_POINT('Ctrl Pts',(-4.069928110878,-6.54009937356905,97.3121144775584));
#184480=CARTESIAN_POINT('Ctrl Pts',(-0.464471910680699,-7.66905552891195,
97.4707819428448));
#184481=CARTESIAN_POINT('Ctrl Pts',(4.53730628323536,-6.76657095782785,
97.6823385632266));
#184482=CARTESIAN_POINT('Ctrl Pts',(8.64709586509307,-1.17195344643985,
97.9467843387042));
#184483=CARTESIAN_POINT('Ctrl Pts',(6.17446001811424,5.31529267128248,98.2112301141812));
#184484=CARTESIAN_POINT('Ctrl Pts',(1.59344116709797,7.51571166844028,98.4227867345635));
#184485=CARTESIAN_POINT('Ctrl Pts',(-2.18287509741676,7.38815633678711,
98.5814541998497));
#184486=CARTESIAN_POINT('Ctrl Pts',(-5.45514273601227,5.43154102305253,
98.7401216651363));
#184487=CARTESIAN_POINT('Ctrl Pts',(-7.38490913140437,2.17042384937628,
98.8987891304226));
#184488=CARTESIAN_POINT('Ctrl Pts',(-7.52577891640735,-1.62945095326339,
99.0574721614392));
#184489=CARTESIAN_POINT('Ctrl Pts',(-6.39483282294218,-3.89356867963719,
99.1632660373603));
#184490=CARTESIAN_POINT('Ctrl Pts',(-5.59319257244812,-4.82318409174615,
99.2161707581859));
#184491=CARTESIAN_POINT('Ctrl Pts',(1.81148773798609,-6.76509875748211,
-0.647699818629882));
#184492=CARTESIAN_POINT('Ctrl Pts',(2.9356747642043,-6.4640767487774,-0.594804846492275));
#184493=CARTESIAN_POINT('Ctrl Pts',(5.03003528944759,-5.29274464953558,
-0.48902071925919));
#184494=CARTESIAN_POINT('Ctrl Pts',(6.94703914831561,-2.23909199201746,
-0.330347436930631));
#184495=CARTESIAN_POINT('Ctrl Pts',(7.17439520364204,1.34694727795299,-0.171679971644201));
#184496=CARTESIAN_POINT('Ctrl Pts',(5.65332152640384,4.62673929743261,-0.0130125063577741));
#184497=CARTESIAN_POINT('Ctrl Pts',(2.76117551751462,6.7417056139338,0.145654958928656));
#184498=CARTESIAN_POINT('Ctrl Pts',(-2.00393381935195,7.46117725044506,
0.35721157931056));
#184499=CARTESIAN_POINT('Ctrl Pts',(-7.40368502527241,3.69526160713211,
0.621657354787942));
#184500=CARTESIAN_POINT('Ctrl Pts',(-7.16726359359808,-2.88320234719017,
0.886103130265323));
#184501=CARTESIAN_POINT('Ctrl Pts',(-3.72798211249409,-6.25951141932115,
1.09765975064723));
#184502=CARTESIAN_POINT('Ctrl Pts',(-0.299318307035459,-7.29834602864205,
1.25632721593366));
#184503=CARTESIAN_POINT('Ctrl Pts',(3.23627226523133,-6.5447122871848,1.41499468122009));
#184504=CARTESIAN_POINT('Ctrl Pts',(5.96510980865824,-4.20302829244138,
1.57366214650652));
#184505=CARTESIAN_POINT('Ctrl Pts',(7.25376943663242,-0.843893506703157,
1.73232961179295));
#184506=CARTESIAN_POINT('Ctrl Pts',(6.76842455697729,2.73845433636508,1.89099707707937));
#184507=CARTESIAN_POINT('Ctrl Pts',(4.64515762980617,5.61747601173395,2.0496645423658));
#184508=CARTESIAN_POINT('Ctrl Pts',(0.28943226546954,7.71984168134768,2.26122116274771));
#184509=CARTESIAN_POINT('Ctrl Pts',(-4.696178645165,6.1246467636793,2.47277778312961));
#184510=CARTESIAN_POINT('Ctrl Pts',(-7.02924814289832,1.91551199337645,
2.68433440351152));
#184511=CARTESIAN_POINT('Ctrl Pts',(-7.15416271867062,-2.89527501251096,
2.89589102389342));
#184512=CARTESIAN_POINT('Ctrl Pts',(-3.66724954191068,-6.79944796472502,
3.10744764427533));
#184513=CARTESIAN_POINT('Ctrl Pts',(1.15305975893845,-7.19743373686098,
3.31900426465724));
#184514=CARTESIAN_POINT('Ctrl Pts',(4.4431290387692,-5.79391180272745,3.47767172994366));
#184515=CARTESIAN_POINT('Ctrl Pts',(6.67943187871092,-2.95260222294961,
3.63633919523009));
#184516=CARTESIAN_POINT('Ctrl Pts',(7.27203543413197,0.595002899120626,
3.79500666051652));
#184517=CARTESIAN_POINT('Ctrl Pts',(6.11063877182122,3.99909701236675,3.95367412580295));
#184518=CARTESIAN_POINT('Ctrl Pts',(3.44221456469882,6.4390943812103,4.11234159108937));
#184519=CARTESIAN_POINT('Ctrl Pts',(-0.0322420101525694,7.2891437288084,
4.27100905637581));
#184520=CARTESIAN_POINT('Ctrl Pts',(-4.72374865002565,6.11288153979805,
4.4825656767577));
#184521=CARTESIAN_POINT('Ctrl Pts',(-7.52964381413083,1.69385100404379,
4.69412229713962));
#184522=CARTESIAN_POINT('Ctrl Pts',(-6.6243886622802,-3.03268210390586,
4.90567891752152));
#184523=CARTESIAN_POINT('Ctrl Pts',(-3.63812709720399,-6.806518789496,5.11723553790342));
#184524=CARTESIAN_POINT('Ctrl Pts',(1.54044884797145,-7.57021402675952,
5.32879215828533));
#184525=CARTESIAN_POINT('Ctrl Pts',(5.49653934046743,-4.78755783384142,
5.54034877866723));
#184526=CARTESIAN_POINT('Ctrl Pts',(7.12349670978252,-1.60205299418428,
5.69901624395365));
#184527=CARTESIAN_POINT('Ctrl Pts',(7.02021416653516,2.01228108246361,5.85768370924009));
#184528=CARTESIAN_POINT('Ctrl Pts',(5.20236750987495,5.11584768931862,6.01635117452652));
#184529=CARTESIAN_POINT('Ctrl Pts',(2.12972100334069,6.98548284302409,6.17501863981295));
#184530=CARTESIAN_POINT('Ctrl Pts',(-1.482372895225,7.14936009422613,6.33368610509938));
#184531=CARTESIAN_POINT('Ctrl Pts',(-4.69471247615635,5.5760496351196,6.4923535703858));
#184532=CARTESIAN_POINT('Ctrl Pts',(-7.54331757626103,1.66717813081053,
6.70391019076773));
#184533=CARTESIAN_POINT('Ctrl Pts',(-6.86656994343393,-3.52347614302802,
6.91546681114959));
#184534=CARTESIAN_POINT('Ctrl Pts',(-3.14334088454267,-6.57260176518009,
7.12702343153154));
#184535=CARTESIAN_POINT('Ctrl Pts',(1.56734723595408,-7.55698945086143,
7.33858005191341));
#184536=CARTESIAN_POINT('Ctrl Pts',(6.03280890944917,-4.82559215419803,
7.55013667229535));
#184537=CARTESIAN_POINT('Ctrl Pts',(7.28757804590471,-0.154470033412791,
7.76169329267723));
#184538=CARTESIAN_POINT('Ctrl Pts',(6.49591206166936,3.33375248721907,7.92036075796366));
#184539=CARTESIAN_POINT('Ctrl Pts',(4.10100447634132,6.04271829434726,8.0790282232501));
#184540=CARTESIAN_POINT('Ctrl Pts',(0.71686550381877,7.26103499095718,8.23769568853653));
#184541=CARTESIAN_POINT('Ctrl Pts',(-2.84017988572185,6.72800567156045,
8.39636315382295));
#184542=CARTESIAN_POINT('Ctrl Pts',(-5.71858768820421,4.53966232348845,
8.55503061910938));
#184543=CARTESIAN_POINT('Ctrl Pts',(-7.1770895003255,1.27359376203791,8.7136980843958));
#184544=CARTESIAN_POINT('Ctrl Pts',(-6.85998029030304,-3.55271634009679,
8.92525470477772));
#184545=CARTESIAN_POINT('Ctrl Pts',(-3.0148526110767,-7.10459926048452,
9.13681132515961));
#184546=CARTESIAN_POINT('Ctrl Pts',(1.79738669100636,-7.06038858441899,
9.34836794554153));
#184547=CARTESIAN_POINT('Ctrl Pts',(6.04498924497277,-4.79820507552116,
9.55992456592342));
#184548=CARTESIAN_POINT('Ctrl Pts',(7.72370085836326,0.15990005333229,9.77148118630533));
#184549=CARTESIAN_POINT('Ctrl Pts',(5.69446886265255,4.55034934248621,9.98303780668723));
#184550=CARTESIAN_POINT('Ctrl Pts',(2.85180711825711,6.72145633916047,10.1417052719737));
#184551=CARTESIAN_POINT('Ctrl Pts',(-0.722597256169256,7.26708575050433,
10.3003727372601));
#184552=CARTESIAN_POINT('Ctrl Pts',(-4.10152883824344,6.03440025847895,
10.4590402025466));
#184553=CARTESIAN_POINT('Ctrl Pts',(-6.49118048992967,3.34623040852877,
10.617707667833));
#184554=CARTESIAN_POINT('Ctrl Pts',(-7.29924993347423,-0.178127953052982,
10.7763751331194));
#184555=CARTESIAN_POINT('Ctrl Pts',(-6.32662643415969,-3.62028351499932,
10.9350425984058));
#184556=CARTESIAN_POINT('Ctrl Pts',(-2.99105958231506,-7.12282847972478,
11.1465992187878));
#184557=CARTESIAN_POINT('Ctrl Pts',(2.23687814569076,-7.38654473214131,
11.3581558391696));
#184558=CARTESIAN_POINT('Ctrl Pts',(5.90345804255817,-4.26952796217054,
11.5697124595516));
#184559=CARTESIAN_POINT('Ctrl Pts',(7.71550693145034,0.188731845047503,
11.7812690799335));
#184560=CARTESIAN_POINT('Ctrl Pts',(5.82792165520761,5.07113913803384,11.9928257003154));
#184561=CARTESIAN_POINT('Ctrl Pts',(1.45700724129014,7.14211345927886,12.2043823206973));
#184562=CARTESIAN_POINT('Ctrl Pts',(-2.11659747242143,6.98790342654516,
12.3630497859837));
#184563=CARTESIAN_POINT('Ctrl Pts',(-5.21064498668082,5.11682136903217,
12.5217172512701));
#184564=CARTESIAN_POINT('Ctrl Pts',(-7.01528763922469,2.00555843330852,
12.6803847165566));
#184565=CARTESIAN_POINT('Ctrl Pts',(-7.12785800821589,-1.58944088110218,
12.839052181843));
#184566=CARTESIAN_POINT('Ctrl Pts',(-5.49034419207099,-4.81320057878068,
12.9977196471294));
#184567=CARTESIAN_POINT('Ctrl Pts',(-2.53825459376162,-6.83300215012639,
13.1563871124158));
#184568=CARTESIAN_POINT('Ctrl Pts',(2.26682573146794,-7.38529783283597,
13.3679437327978));
#184569=CARTESIAN_POINT('Ctrl Pts',(6.44986511072266,-4.23838494854773,
13.5795003531797));
#184570=CARTESIAN_POINT('Ctrl Pts',(7.26812821260535,0.503982306367112,
13.7910569735616));
#184571=CARTESIAN_POINT('Ctrl Pts',(5.80315849686722,5.08802696325712,14.0026135939435));
#184572=CARTESIAN_POINT('Ctrl Pts',(1.22581826102254,7.62748271499059,14.2141702143254));
#184573=CARTESIAN_POINT('Ctrl Pts',(-3.45704788576664,6.41727938318885,
14.4257268347073));
#184574=CARTESIAN_POINT('Ctrl Pts',(-6.10211325965028,4.009363157084,14.5843942999937));
#184575=CARTESIAN_POINT('Ctrl Pts',(-7.27901458618669,0.590447926482588,
14.7430617652802));
#184576=CARTESIAN_POINT('Ctrl Pts',(-6.67134261913644,-2.95460876404428,
14.9017292305666));
#184577=CARTESIAN_POINT('Ctrl Pts',(-4.45455716730087,-5.78702017821389,
15.060396695853));
#184578=CARTESIAN_POINT('Ctrl Pts',(-1.13187581356497,-7.21315716601607,
15.2190641611394));
#184579=CARTESIAN_POINT('Ctrl Pts',(2.42881185107581,-6.87266525872296,
15.3777316264259));
#184580=CARTESIAN_POINT('Ctrl Pts',(6.47206043035504,-4.21824095594001,
15.5892882468078));
#184581=CARTESIAN_POINT('Ctrl Pts',(7.66771469904878,0.877962534841119,
15.8008448671897));
#184582=CARTESIAN_POINT('Ctrl Pts',(5.25768245471256,5.04345725523755,16.0124014875716));
#184583=CARTESIAN_POINT('Ctrl Pts',(1.19598519098265,7.62458433893572,16.2239581079535));
#184584=CARTESIAN_POINT('Ctrl Pts',(-3.94552092764966,6.6418361607326,16.4355147283354));
#184585=CARTESIAN_POINT('Ctrl Pts',(-6.76574644210875,2.71243983296901,
16.6470713487173));
#184586=CARTESIAN_POINT('Ctrl Pts',(-7.25397792594533,-0.831013482971238,
16.8057388140037));
#184587=CARTESIAN_POINT('Ctrl Pts',(-5.96721292964101,-4.21011305692988,
16.9644062792902));
#184588=CARTESIAN_POINT('Ctrl Pts',(-3.22941224766971,-6.54273809846264,
17.1230737445766));
#184589=CARTESIAN_POINT('Ctrl Pts',(0.287315719605487,-7.29726878887394,
17.281741209863));
#184590=CARTESIAN_POINT('Ctrl Pts',(3.75220410825254,-6.26352484540415,
17.4404086751494));
#184591=CARTESIAN_POINT('Ctrl Pts',(6.26800584722447,-3.7208543999388,17.5990761404359));
#184592=CARTESIAN_POINT('Ctrl Pts',(7.67185086544985,0.9076493126936,17.8106327608178));
#184593=CARTESIAN_POINT('Ctrl Pts',(5.32489154541977,5.58660871621691,18.0221893811997));
#184594=CARTESIAN_POINT('Ctrl Pts',(0.805715678220419,7.24089139028274,
18.2337460015816));
#184595=CARTESIAN_POINT('Ctrl Pts',(-3.96657026414156,6.62049750836153,
18.4453026219635));
#184596=CARTESIAN_POINT('Ctrl Pts',(-7.28467029558708,2.57190623101386,
18.6568592423454));
#184597=CARTESIAN_POINT('Ctrl Pts',(-6.93262114598217,-2.25198108621383,
18.8684158627273));
#184598=CARTESIAN_POINT('Ctrl Pts',(-5.03729766256775,-5.28549065060871,
19.0270833280137));
#184599=CARTESIAN_POINT('Ctrl Pts',(-1.88440410108215,-7.0556150180995,
19.1857507933002));
#184600=CARTESIAN_POINT('Ctrl Pts',(1.71216705625404,-7.09260243224952,
19.3444182585866));
#184601=CARTESIAN_POINT('Ctrl Pts',(4.89576720374872,-5.41886940113016,
19.503085723873));
#184602=CARTESIAN_POINT('Ctrl Pts',(6.89386514584056,-2.40528636755529,
19.6617531891595));
#184603=CARTESIAN_POINT('Ctrl Pts',(7.19651283393127,1.15881741333419,19.8204206544458));
#184604=CARTESIAN_POINT('Ctrl Pts',(5.3090478383308,5.6120525680763,20.0319772748278));
#184605=CARTESIAN_POINT('Ctrl Pts',(0.509337346907726,7.7009897016967,20.2435338952097));
#184606=CARTESIAN_POINT('Ctrl Pts',(-4.02040297608755,6.07585761764272,
20.4550905155916));
#184607=CARTESIAN_POINT('Ctrl Pts',(-7.28716117403683,2.5420363770418,20.6666471359734));
#184608=CARTESIAN_POINT('Ctrl Pts',(-7.24102205384756,-2.69234518444979,
20.8782037563553));
#184609=CARTESIAN_POINT('Ctrl Pts',(-3.88018004147492,-6.17064482952338,
21.0897603767373));
#184610=CARTESIAN_POINT('Ctrl Pts',(-0.481436928319875,-7.28553344944846,
21.2484278420237));
#184611=CARTESIAN_POINT('Ctrl Pts',(3.07346940853279,-6.62468624876828,
21.4070953073102));
#184612=CARTESIAN_POINT('Ctrl Pts',(5.85866375653926,-4.34886011252219,
21.5657627725966));
#184613=CARTESIAN_POINT('Ctrl Pts',(7.23076101275068,-1.02409827472313,
21.724430237883));
#184614=CARTESIAN_POINT('Ctrl Pts',(6.83420758004411,2.56989998090389,21.8830977031693));
#184615=CARTESIAN_POINT('Ctrl Pts',(4.78316007615802,5.50036675615653,22.0417651684559));
#184616=CARTESIAN_POINT('Ctrl Pts',(0.480871141789132,7.7103752127592,22.2533217888377));
#184617=CARTESIAN_POINT('Ctrl Pts',(-4.54273890266845,6.23924596251632,
22.4648784092197));
#184618=CARTESIAN_POINT('Ctrl Pts',(-6.97955867591758,2.08936511156489,
22.6764350296014));
#184619=CARTESIAN_POINT('Ctrl Pts',(-7.22379777980997,-2.71687551334363,
22.8879916499834));
#184620=CARTESIAN_POINT('Ctrl Pts',(-3.83484522790946,-6.70634662499014,
23.0995482703654));
#184621=CARTESIAN_POINT('Ctrl Pts',(0.974108399536885,-7.22383330319408,
23.3111048907473));
#184622=CARTESIAN_POINT('Ctrl Pts',(4.29798968114909,-5.90237781404394,
23.4697723560337));
#184623=CARTESIAN_POINT('Ctrl Pts',(6.60410948866788,-3.11743804453164,
23.6284398213202));
#184624=CARTESIAN_POINT('Ctrl Pts',(7.28456049178172,0.414371490388069,
23.7871072866066));
#184625=CARTESIAN_POINT('Ctrl Pts',(6.20799117870954,3.84623551344313,23.9457747518929));
#184626=CARTESIAN_POINT('Ctrl Pts',(3.60093471970036,6.35169649018581,24.1044422171794));
#184627=CARTESIAN_POINT('Ctrl Pts',(0.148641251043096,7.28769926279015,
24.2631096824659));
#184628=CARTESIAN_POINT('Ctrl Pts',(-4.57060869449693,6.22821476334319,
24.4746663028478));
#184629=CARTESIAN_POINT('Ctrl Pts',(-7.48529396902207,1.88017050182036,
24.6862229232297));
#184630=CARTESIAN_POINT('Ctrl Pts',(-6.69760208823655,-2.86737024948825,
24.8977795436115));
#184631=CARTESIAN_POINT('Ctrl Pts',(-3.80590427361161,-6.71414622857579,
25.1093361639936));
#184632=CARTESIAN_POINT('Ctrl Pts',(1.35212671216194,-7.60610783060528,
25.3208927843753));
#184633=CARTESIAN_POINT('Ctrl Pts',(5.37604808188003,-4.92247516882494,
25.5324494047574));
#184634=CARTESIAN_POINT('Ctrl Pts',(7.08154981624727,-1.77832262511345,
25.6911168700437));
#184635=CARTESIAN_POINT('Ctrl Pts',(7.06798540710253,1.83746139681678,25.8497843353302));
#184636=CARTESIAN_POINT('Ctrl Pts',(5.32771060717042,4.98518053602045,26.0084518006166));
#184637=CARTESIAN_POINT('Ctrl Pts',(2.30240347260139,6.93048485671525,26.167119265903));
#184638=CARTESIAN_POINT('Ctrl Pts',(-1.30451174193647,7.18394239078603,
26.3257867311895));
#184639=CARTESIAN_POINT('Ctrl Pts',(-4.55490242328604,5.69082759189972,
26.4844541964758));
#184640=CARTESIAN_POINT('Ctrl Pts',(-7.49962539392981,1.85384517348665,
26.6960108168578));
#184641=CARTESIAN_POINT('Ctrl Pts',(-6.9518873900729,-3.35200367457123,
26.9075674372397));
#184642=CARTESIAN_POINT('Ctrl Pts',(-3.30546598448613,-6.49257887941348,
27.1191240576216));
#184643=CARTESIAN_POINT('Ctrl Pts',(1.3793449751289,-7.5935547906221,27.3306806780035));
#184644=CARTESIAN_POINT('Ctrl Pts',(5.91120873762003,-4.97380480485731,
27.5422372983854));
#184645=CARTESIAN_POINT('Ctrl Pts',(7.28150105130914,-0.33525692560751,
27.7537939187673));
#184646=CARTESIAN_POINT('Ctrl Pts',(6.57663582428421,3.17153596759111,27.9124613840537));
#184647=CARTESIAN_POINT('Ctrl Pts',(4.24968613157374,5.93909503905403,28.0711288493402));
#184648=CARTESIAN_POINT('Ctrl Pts',(0.896820584063796,7.24101085004523,
28.2297963146266));
#184649=CARTESIAN_POINT('Ctrl Pts',(-2.67235615860355,6.79641042473009,
28.388463779913));
#184650=CARTESIAN_POINT('Ctrl Pts',(-5.60417935245751,4.68016590993002,
28.5471312451994));
#184651=CARTESIAN_POINT('Ctrl Pts',(-7.14327651483552,1.45129438742917,
28.7057987104858));
#184652=CARTESIAN_POINT('Ctrl Pts',(-6.94602533424502,-3.3813983841842,
28.9173553308678));
#184653=CARTESIAN_POINT('Ctrl Pts',(-3.19021829660363,-7.02760088071376,
29.1289119512497));
#184654=CARTESIAN_POINT('Ctrl Pts',(1.621636284852,-7.10281505036224,29.3404685716316));
#184655=CARTESIAN_POINT('Ctrl Pts',(5.92406490744834,-4.9467284027863,29.5520251920136));
#184656=CARTESIAN_POINT('Ctrl Pts',(7.72529037506664,-0.0318056196188755,
29.7635818123952));
#184657=CARTESIAN_POINT('Ctrl Pts',(5.80562811966761,4.4076452786617,29.9751384327773));
#184658=CARTESIAN_POINT('Ctrl Pts',(3.01771567371964,6.64862175729444,30.1338058980636));
#184659=CARTESIAN_POINT('Ctrl Pts',(-0.542048797792806,7.28277867304903,
30.2924733633502));
#184660=CARTESIAN_POINT('Ctrl Pts',(-3.95052789288905,6.13431778260462,
30.4511408286365));
#184661=CARTESIAN_POINT('Ctrl Pts',(-6.40614816070303,3.5062726424121,30.609808293923));
#184662=CARTESIAN_POINT('Ctrl Pts',(-7.30142245391351,0.00305097852067317,
30.7684757592094));
#184663=CARTESIAN_POINT('Ctrl Pts',(-6.41451232295641,-3.46217943281746,
30.9271432244959));
#184664=CARTESIAN_POINT('Ctrl Pts',(-3.16688493518839,-7.04641488870857,
31.1386998448778));
#184665=CARTESIAN_POINT('Ctrl Pts',(2.05289915213799,-7.43977634003499,
31.3502564652597));
#184666=CARTESIAN_POINT('Ctrl Pts',(5.79569591456842,-4.41470211292401,
31.5618130856415));
#184667=CARTESIAN_POINT('Ctrl Pts',(7.71781440523383,-0.00277938102652562,
31.7733697060235));
#184668=CARTESIAN_POINT('Ctrl Pts',(5.95196273323992,4.92496320784834,31.9849263264054));
#184669=CARTESIAN_POINT('Ctrl Pts',(1.63378349280986,7.10376000896753,32.1964829467872));
#184670=CARTESIAN_POINT('Ctrl Pts',(-1.94254742766151,7.03827312984283,
32.3551504120736));
#184671=CARTESIAN_POINT('Ctrl Pts',(-5.08207139110319,5.24454311408885,
32.5138178773602));
#184672=CARTESIAN_POINT('Ctrl Pts',(-6.96336145416715,2.17901871242365,
32.6724853426466));
#184673=CARTESIAN_POINT('Ctrl Pts',(-7.16510371778309,-1.4120803140109,
32.831152807933));
#184674=CARTESIAN_POINT('Ctrl Pts',(-5.60808871082753,-4.67548074217737,
32.9898202732195));
#184675=CARTESIAN_POINT('Ctrl Pts',(-2.70702760250579,-6.76791373509264,
33.1484877385058));
#184676=CARTESIAN_POINT('Ctrl Pts',(2.08286845720673,-7.43927294609562,
33.3600443588877));
#184677=CARTESIAN_POINT('Ctrl Pts',(6.34270751989519,-4.39712727080515,
33.5716009792697));
#184678=CARTESIAN_POINT('Ctrl Pts',(7.27839608796281,0.323475295391082,
33.7831575996516));
#184679=CARTESIAN_POINT('Ctrl Pts',(5.92762625552265,4.94246030772449,33.9947142200335));
#184680=CARTESIAN_POINT('Ctrl Pts',(1.41470968505858,7.5947165505724,34.2062708404153));
#184681=CARTESIAN_POINT('Ctrl Pts',(-3.29674459808255,6.5010868184787,34.4178274607972));
#184682=CARTESIAN_POINT('Ctrl Pts',(-6.00074570958766,4.15954686087893,
34.5764949260837));
#184683=CARTESIAN_POINT('Ctrl Pts',(-7.26212184340316,0.770888079667298,
34.7351623913702));
#184684=CARTESIAN_POINT('Ctrl Pts',(-6.74260426573862,-2.78815584322628,
34.8938298566566));
#184685=CARTESIAN_POINT('Ctrl Pts',(-4.59678504746441,-5.67470257610159,
35.0524973219429));
#184686=CARTESIAN_POINT('Ctrl Pts',(-1.31051506173837,-7.18284967348886,
35.2111647872294));
#184687=CARTESIAN_POINT('Ctrl Pts',(2.25752519810666,-6.93081775451478,
35.3698322525159));
#184688=CARTESIAN_POINT('Ctrl Pts',(6.36539585962406,-4.37754023703014,
35.5813888728977));
#184689=CARTESIAN_POINT('Ctrl Pts',(7.68713950594037,0.687425003039892,
35.7929454932797));
#184690=CARTESIAN_POINT('Ctrl Pts',(5.38121221862192,4.91143980296563,36.0045021136616));
#184691=CARTESIAN_POINT('Ctrl Pts',(1.38481388060976,7.59255934679895,36.2160587340434));
#184692=CARTESIAN_POINT('Ctrl Pts',(-3.77949506399831,6.73769545451185,
36.4276153544254));
#184693=CARTESIAN_POINT('Ctrl Pts',(-6.69635649186656,2.87949031952191,
36.6391719748073));
#184694=CARTESIAN_POINT('Ctrl Pts',(-7.27236513221127,-0.650756899909756,
36.7978394400936));
#184695=CARTESIAN_POINT('Ctrl Pts',(-6.06984555801552,-4.06074586765109,
36.9565069053802));
#184696=CARTESIAN_POINT('Ctrl Pts',(-3.39076980577527,-6.46058862757227,
37.1151743706665));
#184697=CARTESIAN_POINT('Ctrl Pts',(0.106152327585571,-7.30215131198709,
37.273841835953));
#184698=CARTESIAN_POINT('Ctrl Pts',(3.59562521266251,-6.35470365076517,
37.4325093012393));
#184699=CARTESIAN_POINT('Ctrl Pts',(6.17374629198885,-3.87524341023087,
37.5911767665259));
#184700=CARTESIAN_POINT('Ctrl Pts',(7.6920110484677,0.717000004733298,37.8027333869076));
#184701=CARTESIAN_POINT('Ctrl Pts',(5.4618784117509,5.45275628777254,38.0142900072896));
#184702=CARTESIAN_POINT('Ctrl Pts',(0.985143555367147,7.21866871765976,
38.2258466276716));
#184703=CARTESIAN_POINT('Ctrl Pts',(-3.80106741782214,6.71688569232528,
38.4374032480534));
#184704=CARTESIAN_POINT('Ctrl Pts',(-7.21860777051966,2.75187660187186,
38.6489598684354));
#184705=CARTESIAN_POINT('Ctrl Pts',(-6.98636728977761,-2.079261132881,38.8605164888174));
#184706=CARTESIAN_POINT('Ctrl Pts',(-5.16690111965938,-5.15886731547199,
39.0191839541036));
#184707=CARTESIAN_POINT('Ctrl Pts',(-2.05890237191696,-7.00668274740058,
39.1778514193902));
#184708=CARTESIAN_POINT('Ctrl Pts',(1.53564353401614,-7.13290433322274,
39.3365188846766));
#184709=CARTESIAN_POINT('Ctrl Pts',(4.75979552383996,-5.53868474197975,
39.4951863499629));
#184710=CARTESIAN_POINT('Ctrl Pts',(6.83205747267912,-2.57561057790029,
39.6538538152494));
#184711=CARTESIAN_POINT('Ctrl Pts',(7.22305188360824,0.979885836762448,
39.8125212805359));
#184712=CARTESIAN_POINT('Ctrl Pts',(5.44667094866521,5.4785854518756,40.0240779009177));
#184713=CARTESIAN_POINT('Ctrl Pts',(0.70027339451393,7.68597970928423,40.2356345212996));
#184714=CARTESIAN_POINT('Ctrl Pts',(-3.86839828499266,6.17374931372075,
40.4471911416815));
#184715=CARTESIAN_POINT('Ctrl Pts',(-7.22183907457001,2.72207775414406,
40.6587477620636));
#184716=CARTESIAN_POINT('Ctrl Pts',(-7.30560046055917,-2.51183695474356,
40.8703043824454));
#184717=CARTESIAN_POINT('Ctrl Pts',(-4.0321040698922,-6.07246173606261,
41.0818610028273));
#184718=CARTESIAN_POINT('Ctrl Pts',(-0.662072407292881,-7.27134370570371,
41.2405284681137));
#184719=CARTESIAN_POINT('Ctrl Pts',(2.90813762291469,-6.69891167772874,
41.3991959334001));
#184720=CARTESIAN_POINT('Ctrl Pts',(5.74894686808211,-4.49289830715243,
41.5578633986865));
#184721=CARTESIAN_POINT('Ctrl Pts',(7.20312249887356,-1.2032075324176,41.716530863973));
#184722=CARTESIAN_POINT('Ctrl Pts',(6.895872888007,2.39952417604162,41.8751983292594));
#184723=CARTESIAN_POINT('Ctrl Pts',(4.91817373664537,5.37998344444512,42.0338657945458));
#184724=CARTESIAN_POINT('Ctrl Pts',(0.672048847298596,7.69606869276473,
42.2454224149276));
#184725=CARTESIAN_POINT('Ctrl Pts',(-4.38651904627686,6.35004862771582,
42.4569790353096));
#184726=CARTESIAN_POINT('Ctrl Pts',(-6.92556390782915,2.26191300436849,
42.6685356556916));
#184727=CARTESIAN_POINT('Ctrl Pts',(-7.28899018731462,-2.53678713479404,
42.8800922760735));
#184728=CARTESIAN_POINT('Ctrl Pts',(-4.00007615653303,-6.60912352102177,
43.0916488964554));
#184729=CARTESIAN_POINT('Ctrl Pts',(0.79455576613854,-7.24578055880295,
43.3032055168372));
#184730=CARTESIAN_POINT('Ctrl Pts',(4.15020425571326,-6.00721098198628,
43.4618729821236));
#184731=CARTESIAN_POINT('Ctrl Pts',(6.52471965689241,-3.28035295661377,
43.6205404474101));
#184732=CARTESIAN_POINT('Ctrl Pts',(7.2925996967946,0.233484323109056,43.7792079126966));
#184733=CARTESIAN_POINT('Ctrl Pts',(6.30152038869049,3.69100567502789,43.937875377983));
#184734=CARTESIAN_POINT('Ctrl Pts',(3.75743735449865,6.26038686999263,44.0965428432694));
#184735=CARTESIAN_POINT('Ctrl Pts',(0.329432956660445,7.28176684936425,
44.2552103085558));
#184736=CARTESIAN_POINT('Ctrl Pts',(-4.41465400982639,6.33971242730919,
44.4667669289379));
#184737=CARTESIAN_POINT('Ctrl Pts',(-7.43633439938857,2.06533208401449,
44.6783235493196));
#184738=CARTESIAN_POINT('Ctrl Pts',(-6.76669096150921,-2.70029249845544,
44.8898801697016));
#184739=CARTESIAN_POINT('Ctrl Pts',(-3.97133751784657,-6.61763908395221,
45.1014367900834));
#184740=CARTESIAN_POINT('Ctrl Pts',(1.16297162300613,-7.63731711283647,
45.3129934104654));
#184741=CARTESIAN_POINT('Ctrl Pts',(5.25224641083348,-5.05436161866343,
45.5245500308472));
#184742=CARTESIAN_POINT('Ctrl Pts',(7.03524116617045,-1.95349597184172,
45.6832174961336));
#184743=CARTESIAN_POINT('Ctrl Pts',(7.11140532561285,1.66150793145855,45.8418849614201));
#184744=CARTESIAN_POINT('Ctrl Pts',(5.44977010852736,4.85144755338035,46.0005524267066));
#184745=CARTESIAN_POINT('Ctrl Pts',(2.47367298599438,6.87121090774512,46.159219891993));
#184746=CARTESIAN_POINT('Ctrl Pts',(-1.12585644665751,7.21411540452755,
46.3178873572794));
#184747=CARTESIAN_POINT('Ctrl Pts',(-4.41227083275708,5.80207445140952,
46.4765548225659));
#184748=CARTESIAN_POINT('Ctrl Pts',(-7.45135195258497,2.03943046573758,
46.6881114429478));
#184749=CARTESIAN_POINT('Ctrl Pts',(-7.03285233929692,-3.17858157919814,
46.8996680633297));
#184750=CARTESIAN_POINT('Ctrl Pts',(-3.46563939458162,-6.40842269937884,
47.1112246837114));
#184751=CARTESIAN_POINT('Ctrl Pts',(1.19070073991183,-7.62577738708096,
47.3227813040936));
#184752=CARTESIAN_POINT('Ctrl Pts',(5.78555262545727,-5.11828609161979,
47.5343379244752));
#184753=CARTESIAN_POINT('Ctrl Pts',(7.2714528460407,-0.516662245363808,
47.7458945448574));
#184754=CARTESIAN_POINT('Ctrl Pts',(6.65222829110491,3.00910509262411,47.9045620101436));
#184755=CARTESIAN_POINT('Ctrl Pts',(4.39785033760639,5.82843611756107,48.0632294754302));
#184756=CARTESIAN_POINT('Ctrl Pts',(1.0722670766346,7.22290518291542,48.2218969407165));
#184757=CARTESIAN_POINT('Ctrl Pts',(-2.49574161037706,6.84901064311975,
48.3805644060031));
#184758=CARTESIAN_POINT('Ctrl Pts',(-6.49768330440811,4.16528213733704,
48.592121026385));
#184759=CARTESIAN_POINT('Ctrl Pts',(-7.97288646550528,-2.23495874205941,
48.8565668018623));
#184760=CARTESIAN_POINT('Ctrl Pts',(-2.42543815460554,-7.91903654965738,
49.173901732435));
#184761=CARTESIAN_POINT('Ctrl Pts',(4.01126713847677,-6.59282808396492,
49.4383475079127));
#184762=CARTESIAN_POINT('Ctrl Pts',(6.78562435075981,-2.66063041889896,
49.6499041282944));
#184763=CARTESIAN_POINT('Ctrl Pts',(7.25070165219227,0.905871586941507,
49.8085715935808));
#184764=CARTESIAN_POINT('Ctrl Pts',(5.92324844439043,4.24730823449819,49.9672390588673));
#184765=CARTESIAN_POINT('Ctrl Pts',(2.26526197427776,7.37794179712212,50.1787956792492));
#184766=CARTESIAN_POINT('Ctrl Pts',(-4.29604199495613,7.07721117740128,
50.4432414547267));
#184767=CARTESIAN_POINT('Ctrl Pts',(-8.28235171648892,0.208719700560167,
50.7605763852993));
#184768=CARTESIAN_POINT('Ctrl Pts',(-5.26568578465025,-5.64120008672477,
51.0250221607768));
#184769=CARTESIAN_POINT('Ctrl Pts',(-0.745136697720609,-7.2447524332675,
51.2365787811588));
#184770=CARTESIAN_POINT('Ctrl Pts',(4.0286543160041,-6.58750570256803,51.4481354015405));
#184771=CARTESIAN_POINT('Ctrl Pts',(7.3055312760722,-2.50563241722382,51.6596920219226));
#184772=CARTESIAN_POINT('Ctrl Pts',(6.91307482008316,2.31299330946768,51.8712486423043));
#184773=CARTESIAN_POINT('Ctrl Pts',(4.98963050516779,5.33044231299205,52.0299161075908));
#184774=CARTESIAN_POINT('Ctrl Pts',(1.82176990436786,7.07192741460845,52.1885835728774));
#184775=CARTESIAN_POINT('Ctrl Pts',(-1.77534079788555,7.07717881730109,
52.3472510381637));
#184776=CARTESIAN_POINT('Ctrl Pts',(-4.94373338993647,5.37503621483437,
52.5059185034503));
#184777=CARTESIAN_POINT('Ctrl Pts',(-6.91503055541669,2.34386587105855,
52.6645859687366));
#184778=CARTESIAN_POINT('Ctrl Pts',(-7.18589952197611,-1.22282769156393,
52.823253434023));
#184779=CARTESIAN_POINT('Ctrl Pts',(-5.25890681105704,-5.65906747048718,
53.034810054405));
#184780=CARTESIAN_POINT('Ctrl Pts',(-0.440777264060952,-7.70522238742984,
53.2463666747867));
#184781=CARTESIAN_POINT('Ctrl Pts',(4.07431222385627,-6.0398361779948,53.4579232951687));
#184782=CARTESIAN_POINT('Ctrl Pts',(7.30949717848282,-2.47708659804833,
53.6694799155507));
#184783=CARTESIAN_POINT('Ctrl Pts',(7.21677412840871,2.75667963275689,53.8810365359325));
#184784=CARTESIAN_POINT('Ctrl Pts',(3.82511233426199,6.2049310571903,54.0925931563145));
#184785=CARTESIAN_POINT('Ctrl Pts',(0.416581274069471,7.28952962351591,
54.2512606216008));
#184786=CARTESIAN_POINT('Ctrl Pts',(-3.13230276561864,6.59707200248025,
54.4099280868873));
#184787=CARTESIAN_POINT('Ctrl Pts',(-5.89713374135158,4.29654982490879,
54.5685955521736));
#184788=CARTESIAN_POINT('Ctrl Pts',(-7.23958841483069,0.959708817476291,
54.7272630174602));
#184789=CARTESIAN_POINT('Ctrl Pts',(-6.81106660114069,-2.6306180109872,
54.8859304827466));
#184790=CARTESIAN_POINT('Ctrl Pts',(-4.73402111891364,-5.54271583276722,
55.0445979480329));
#184791=CARTESIAN_POINT('Ctrl Pts',(-0.412234995645997,-7.71434930458152,
55.2561545684149));
#184792=CARTESIAN_POINT('Ctrl Pts',(4.5980840745598,-6.19857159670066,55.4677111887967));
#184793=CARTESIAN_POINT('Ctrl Pts',(6.99787621844488,-2.02716903160589,
55.6792678091788));
#184794=CARTESIAN_POINT('Ctrl Pts',(7.19933337051351,2.7810548274256,55.8908244295606));
#184795=CARTESIAN_POINT('Ctrl Pts',(3.77501142994787,6.74020857855475,56.1023810499424));
#184796=CARTESIAN_POINT('Ctrl Pts',(-1.03835704366409,7.2148783365985,56.3139376703245));
#184797=CARTESIAN_POINT('Ctrl Pts',(-4.35034664296364,5.86389488721425,
56.4726051356107));
#184798=CARTESIAN_POINT('Ctrl Pts',(-6.63159105256981,3.05854249758164,
56.6312726008973));
#184799=CARTESIAN_POINT('Ctrl Pts',(-7.28058439972057,-0.479182731052562,
56.7899400661836));
#184800=CARTESIAN_POINT('Ctrl Pts',(-6.17351645531762,-3.90133011619834,
56.9486075314703));
#184801=CARTESIAN_POINT('Ctrl Pts',(-3.54426633105253,-6.383490842283,57.1072749967566));
#184802=CARTESIAN_POINT('Ctrl Pts',(-0.0837797822335151,-7.28873347808429,
57.265942462043));
#184803=CARTESIAN_POINT('Ctrl Pts',(4.62585458842083,-6.18729280891253,
57.4774990824248));
#184804=CARTESIAN_POINT('Ctrl Pts',(7.50172979603139,-1.81348200596989,
57.6890557028069));
#184805=CARTESIAN_POINT('Ctrl Pts',(6.67181921361558,2.92686082019994,57.9006123231887));
#184806=CARTESIAN_POINT('Ctrl Pts',(3.74600221126334,6.7477503178319,58.1121689435707));
#184807=CARTESIAN_POINT('Ctrl Pts',(-1.41976237131267,7.59377361958786,
58.3237255639525));
#184808=CARTESIAN_POINT('Ctrl Pts',(-5.41964188346264,4.87443705687105,
58.5352821843343));
#184809=CARTESIAN_POINT('Ctrl Pts',(-7.09709525436815,1.7152312116475,58.6939496496209));
#184810=CARTESIAN_POINT('Ctrl Pts',(-7.05135335594398,-1.90028891209286,
58.8526171149072));
#184811=CARTESIAN_POINT('Ctrl Pts',(-5.28313490415875,-5.03239613652711,
59.0112845801937));
#184812=CARTESIAN_POINT('Ctrl Pts',(-2.24063568138787,-6.95070024120576,
59.16995204548));
#184813=CARTESIAN_POINT('Ctrl Pts',(1.36839230042598,-7.17204863836807,
59.3286195107666));
#184814=CARTESIAN_POINT('Ctrl Pts',(4.6053665576827,-5.65006669303664,59.4872869760529));
#184815=CARTESIAN_POINT('Ctrl Pts',(7.51582637584101,-1.78703018014501,
59.6988435964349));
#184816=CARTESIAN_POINT('Ctrl Pts',(6.92178153689894,3.41373802070961,59.9104002168167));
#184817=CARTESIAN_POINT('Ctrl Pts',(3.24755553856133,6.52173818118763,60.1219568371987));
#184818=CARTESIAN_POINT('Ctrl Pts',(-1.44686784289751,7.58097885261414,
60.3335134575804));
#184819=CARTESIAN_POINT('Ctrl Pts',(-5.95523814593559,4.92100209324587,
60.5450700779626));
#184820=CARTESIAN_POINT('Ctrl Pts',(-7.2841962650308,0.270443226750529,
60.7566266983443));
#184821=CARTESIAN_POINT('Ctrl Pts',(-6.54815087122025,-3.22993797567694,
60.9152941636308));
#184822=CARTESIAN_POINT('Ctrl Pts',(-4.19666392570424,-5.97667917781263,
61.0739616289173));
#184823=CARTESIAN_POINT('Ctrl Pts',(-0.832344982766427,-7.24870520300951,
61.2326290942037));
#184824=CARTESIAN_POINT('Ctrl Pts',(2.73273377903013,-6.7723591305212,61.3912965594901));
#184825=CARTESIAN_POINT('Ctrl Pts',(5.64560773197164,-4.63010717971888,
61.5499640247765));
#184826=CARTESIAN_POINT('Ctrl Pts',(7.15590917899213,-1.38766659843069,
61.7086314900631));
#184827=CARTESIAN_POINT('Ctrl Pts',(6.91565812021998,3.44307939797683,61.9201881104448));
#184828=CARTESIAN_POINT('Ctrl Pts',(3.12755108137218,7.05571336946174,62.131744730827));
#184829=CARTESIAN_POINT('Ctrl Pts',(-1.68478230696036,7.08810231713357,
62.3433013512086));
#184830=CARTESIAN_POINT('Ctrl Pts',(-5.96785284504113,4.89381235219824,
62.5548579715907));
#184831=CARTESIAN_POINT('Ctrl Pts',(-7.72526750394742,-0.0369454867507081,
62.7664145919723));
#184832=CARTESIAN_POINT('Ctrl Pts',(-5.76617316348448,-4.45913689127116,
62.9779712123546));
#184833=CARTESIAN_POINT('Ctrl Pts',(-2.95842794681348,-6.6752140971279,
63.1366386776407));
#184834=CARTESIAN_POINT('Ctrl Pts',(0.60683912552941,-7.27766641001998,
63.2953061429274));
#184835=CARTESIAN_POINT('Ctrl Pts',(4.00496272239341,-6.09891784521749,
63.4539736082136));
#184836=CARTESIAN_POINT('Ctrl Pts',(6.43709792822806,-3.44912341939349,
63.6126410735002));
#184837=CARTESIAN_POINT('Ctrl Pts',(7.30116047104696,0.0619268520408896,
63.7713085387865));
#184838=CARTESIAN_POINT('Ctrl Pts',(6.38344726014772,3.51912714224657,63.929976004073));
#184839=CARTESIAN_POINT('Ctrl Pts',(3.10405121203629,7.07431898132906,64.1415326244549));
#184840=CARTESIAN_POINT('Ctrl Pts',(-2.1190268233751,7.42121231608492,64.3530892448369));
#184841=CARTESIAN_POINT('Ctrl Pts',(-5.83475426225583,4.36294952745141,
64.5646458652188));
#184842=CARTESIAN_POINT('Ctrl Pts',(-7.71753351631633,-0.0659040448481696,
64.7762024856005));
#184843=CARTESIAN_POINT('Ctrl Pts',(-5.90789820339546,-4.97773661364814,
64.9877591059827));
#184844=CARTESIAN_POINT('Ctrl Pts',(-1.5705001473999,-7.11801826728487,
65.1993157263643));
#184845=CARTESIAN_POINT('Ctrl Pts',(2.00510636243311,-7.02070706085311,
65.3579831916509));
#184846=CARTESIAN_POINT('Ctrl Pts',(5.12854302045228,-5.1991084415673,65.5166506569372));
#184847=CARTESIAN_POINT('Ctrl Pts',(6.98247749603737,-2.11696322778764,
65.6753181222237));
#184848=CARTESIAN_POINT('Ctrl Pts',(7.15225342400797,1.47578896139401,65.8339855875101));
#184849=CARTESIAN_POINT('Ctrl Pts',(5.56625802311303,4.72520378175507,65.9926530527966));
#184850=CARTESIAN_POINT('Ctrl Pts',(2.64669056104292,6.79173643779485,66.151320518083));
#184851=CARTESIAN_POINT('Ctrl Pts',(-2.14899046180211,7.42044223558275,
66.3628771384648));
#184852=CARTESIAN_POINT('Ctrl Pts',(-6.38158780187974,4.34050734885831,
66.574433758847));
#184853=CARTESIAN_POINT('Ctrl Pts',(-7.27522915446962,-0.388235276547787,
66.7859903792287));
#184854=CARTESIAN_POINT('Ctrl Pts',(-5.88340697707009,-4.99501644249114,
66.9975469996106));
#184855=CARTESIAN_POINT('Ctrl Pts',(-1.34706583454681,-7.60700575876824,
67.2091036199925));
#184856=CARTESIAN_POINT('Ctrl Pts',(3.35446931300563,-6.47149058521199,
67.4206602403744));
#184857=CARTESIAN_POINT('Ctrl Pts',(6.03752522859704,-4.10597957533119,
67.5793277056609));
#184858=CARTESIAN_POINT('Ctrl Pts',(7.26869464646582,-0.706229591737301,
67.7379951709472));
#184859=CARTESIAN_POINT('Ctrl Pts',(6.71752456355499,2.84805003967782,67.8966626362337));
#184860=CARTESIAN_POINT('Ctrl Pts',(4.54610201023635,5.71538612976684,68.0553301015202));
#184861=CARTESIAN_POINT('Ctrl Pts',(1.24654067328318,7.19422793000284,68.2139975668065));
#184862=CARTESIAN_POINT('Ctrl Pts',(-2.31911537984757,6.91045285211747,
68.372665032093));
#184863=CARTESIAN_POINT('Ctrl Pts',(-6.40410093183477,4.32071917988316,
68.584221652475));
#184864=CARTESIAN_POINT('Ctrl Pts',(-7.68071748065629,-0.755808111186017,
68.7957782728568));
#184865=CARTESIAN_POINT('Ctrl Pts',(-5.33729063949043,-4.95913445165674,
69.0073348932388));
#184866=CARTESIAN_POINT('Ctrl Pts',(-1.31719041161549,-7.6045825880282,
69.2188915136204));
#184867=CARTESIAN_POINT('Ctrl Pts',(3.83930631857219,-6.70379369974262,
69.4304481340026));
#184868=CARTESIAN_POINT('Ctrl Pts',(6.72171682947581,-2.81978325952998,
69.6420047543843));
#184869=CARTESIAN_POINT('Ctrl Pts',(7.26628585314707,0.715450249379216,
69.8006722196709));
#184870=CARTESIAN_POINT('Ctrl Pts',(6.03346730846074,4.11460257346222,69.9593396849572));
#184871=CARTESIAN_POINT('Ctrl Pts',(3.33314067339355,6.49050834232903,70.1180071502437));
#184872=CARTESIAN_POINT('Ctrl Pts',(-0.171132320066243,7.30091746486942,
70.2766746155301));
#184873=CARTESIAN_POINT('Ctrl Pts',(-3.65203538103765,6.32245337939566,
70.4353420808165));
#184874=CARTESIAN_POINT('Ctrl Pts',(-6.20798885225487,3.82014779513346,
70.5940095461031));
#184875=CARTESIAN_POINT('Ctrl Pts',(-7.68532563280746,-0.785425295142584,
70.805566166485));
#184876=CARTESIAN_POINT('Ctrl Pts',(-5.41313628853616,-5.50114737489614,
71.0171227868668));
#184877=CARTESIAN_POINT('Ctrl Pts',(-0.920863286333173,-7.22714996993175,
71.2286794072488));
#184878=CARTESIAN_POINT('Ctrl Pts',(3.86069262536099,-6.68279278229367,
71.4402360276305));
#184879=CARTESIAN_POINT('Ctrl Pts',(7.24281175153894,-2.68752691303847,
71.6517926480126));
#184880=CARTESIAN_POINT('Ctrl Pts',(6.96758661695657,2.14135272703773,71.8633492683943));
#184881=CARTESIAN_POINT('Ctrl Pts',(5.12078609007939,5.20464494260962,72.0220167336809));
#184882=CARTESIAN_POINT('Ctrl Pts',(1.99646611371851,7.02472811976237,72.1806841989672));
#184883=CARTESIAN_POINT('Ctrl Pts',(-1.59906073563403,7.11895568564848,
72.3393516642537));
#184884=CARTESIAN_POINT('Ctrl Pts',(-4.80889757630398,5.49610645825061,
72.4980191295401));
#184885=CARTESIAN_POINT('Ctrl Pts',(-6.85470811288226,2.51470790474134,
72.6566865948267));
#184886=CARTESIAN_POINT('Ctrl Pts',(-7.21404553293573,-1.04412729832816,
72.815354060113));
#184887=CARTESIAN_POINT('Ctrl Pts',(-5.39769956561297,-5.52684018005931,
73.026910680495));
#184888=CARTESIAN_POINT('Ctrl Pts',(-0.631845655261508,-7.69190730485752,
73.2384673008768));
#184889=CARTESIAN_POINT('Ctrl Pts',(3.92318728070288,-6.13907871268419,
73.4500239212587));
#184890=CARTESIAN_POINT('Ctrl Pts',(7.24577773808827,-2.65770048892236,
73.6615805416405));
#184891=CARTESIAN_POINT('Ctrl Pts',(7.28295751464004,2.5767523777974,73.8731371620225));
#184892=CARTESIAN_POINT('Ctrl Pts',(3.97790360703262,6.10810426069667,74.0846937824044));
#184893=CARTESIAN_POINT('Ctrl Pts',(0.597336160113752,7.27694775787233,
74.2433612476908));
#184894=CARTESIAN_POINT('Ctrl Pts',(-2.96763823370572,6.6727659492638,74.4020287129772));
#184895=CARTESIAN_POINT('Ctrl Pts',(-5.78870296013572,4.4415586599514,74.5606961782637));
#184896=CARTESIAN_POINT('Ctrl Pts',(-7.21354498832617,1.13905697890869,
74.7193636435501));
#184897=CARTESIAN_POINT('Ctrl Pts',(-6.87424567478813,-2.4607977490316,
74.8780311088366));
#184898=CARTESIAN_POINT('Ctrl Pts',(-4.87010077296131,-5.42353881036963,
75.0366985741231));
#184899=CARTESIAN_POINT('Ctrl Pts',(-0.603532440634412,-7.70174470945635,
75.2482551945048));
#184900=CARTESIAN_POINT('Ctrl Pts',(4.44285646893518,-6.31076012181055,
75.4598118148867));
#184901=CARTESIAN_POINT('Ctrl Pts',(6.94541914943549,-2.20019060961902,
75.6713684352688));
#184902=CARTESIAN_POINT('Ctrl Pts',(7.26612585956091,2.60155374951464,75.8829250556504));
#184903=CARTESIAN_POINT('Ctrl Pts',(3.9411010357416,6.64445976755175,76.0944816760327));
#184904=CARTESIAN_POINT('Ctrl Pts',(-0.859006836306801,7.23842261971224,
76.3060382964143));
#184905=CARTESIAN_POINT('Ctrl Pts',(-4.20350001419982,5.97003909447874,
76.4647057617009));
#184906=CARTESIAN_POINT('Ctrl Pts',(-6.55365419606634,3.22215747259319,
76.6233732269872));
#184907=CARTESIAN_POINT('Ctrl Pts',(-7.29023306121847,-0.298374267641428,
76.7820406922739));
#184908=CARTESIAN_POINT('Ctrl Pts',(-6.2684233986423,-3.74693877654286,
76.9407081575602));
#184909=CARTESIAN_POINT('Ctrl Pts',(-3.70157536819349,-6.29357759565777,
77.0993756228467));
#184910=CARTESIAN_POINT('Ctrl Pts',(-0.264617112092581,-7.28441024039501,
77.258043088133));
#184911=CARTESIAN_POINT('Ctrl Pts',(4.47089830846142,-6.30017390965787,
77.4695997085149));
#184912=CARTESIAN_POINT('Ctrl Pts',(7.45442002495854,-1.99907203724375,
77.6811563288968));
#184913=CARTESIAN_POINT('Ctrl Pts',(6.7423921741066,2.76040461717969,77.8927129492787));
#184914=CARTESIAN_POINT('Ctrl Pts',(3.9122878899729,6.65271902191615,78.1042695696606));
#184915=CARTESIAN_POINT('Ctrl Pts',(-1.23089278942452,7.62666545204912,
78.3158261900425));
#184916=CARTESIAN_POINT('Ctrl Pts',(-5.29701847508189,5.00741949920571,
78.5273828104243));
#184917=CARTESIAN_POINT('Ctrl Pts',(-7.05234807878031,1.89081086698427,
78.6860502757109));
#184918=CARTESIAN_POINT('Ctrl Pts',(-7.09633602667755,-1.72473102143047,
78.8447177409972));
#184919=CARTESIAN_POINT('Ctrl Pts',(-5.40638235949169,-4.89975051134758,
79.0033852062838));
#184920=CARTESIAN_POINT('Ctrl Pts',(-2.4124209002896,-6.89296072088419,
79.1620526715701));
#184921=CARTESIAN_POINT('Ctrl Pts',(1.19000324852048,-7.20379562643837,
79.3207201368566));
#184922=CARTESIAN_POINT('Ctrl Pts',(4.46374735160504,-5.762604823118,79.479387602143));
#184923=CARTESIAN_POINT('Ctrl Pts',(7.46916864160353,-1.97297814985959,
79.6909442225248));
#184924=CARTESIAN_POINT('Ctrl Pts',(7.00435893377828,3.24092931817309,79.9025008429068));
#184925=CARTESIAN_POINT('Ctrl Pts',(3.40838641667833,6.43914496766489,80.1140574632888));
#184926=CARTESIAN_POINT('Ctrl Pts',(-1.25830740500682,7.61454722180501,
80.3256140836704));
#184927=CARTESIAN_POINT('Ctrl Pts',(-5.83129435071655,5.06726051943635,
80.5371707040526));
#184928=CARTESIAN_POINT('Ctrl Pts',(-7.27524254505289,0.45111049315681,
80.7487273244343));
#184929=CARTESIAN_POINT('Ctrl Pts',(-6.62628248831729,-3.06645716487308,
80.9073947897209));
#184930=CARTESIAN_POINT('Ctrl Pts',(-4.3436774267066,-5.87070255697951,
81.0660622550072));
#184931=CARTESIAN_POINT('Ctrl Pts',(-1.01195855279319,-7.2258193430159,
81.2247297202939));
#184932=CARTESIAN_POINT('Ctrl Pts',(2.56384254658913,-6.83808405155319,
81.3833971855802));
#184933=CARTESIAN_POINT('Ctrl Pts',(5.52897756315095,-4.76877198712165,
81.5420646508666));
#184934=CARTESIAN_POINT('Ctrl Pts',(7.11927210416887,-1.56480652899543,
81.700732116153));
#184935=CARTESIAN_POINT('Ctrl Pts',(6.99896548152559,3.27041360762663,81.9122887365349));
#184936=CARTESIAN_POINT('Ctrl Pts',(3.30166900737668,6.97593353497021,82.1238453569169));
#184937=CARTESIAN_POINT('Ctrl Pts',(-1.50837888309741,7.12772607673909,
82.3354019772986));
#184938=CARTESIAN_POINT('Ctrl Pts',(-5.84457985362841,5.040392172555,82.5469585976806));
#184939=CARTESIAN_POINT('Ctrl Pts',(-7.72380553529811,0.15476120132443,
82.7585152180625));
#184940=CARTESIAN_POINT('Ctrl Pts',(-5.87504698961766,-4.31468163786957,
82.9700718384444));
#184941=CARTESIAN_POINT('Ctrl Pts',(-3.1231562138444,-6.59974805753279,
83.1287393037308));
#184942=CARTESIAN_POINT('Ctrl Pts',(0.426063761775637,-7.29048364449903,
83.2874067690173));
#184943=CARTESIAN_POINT('Ctrl Pts',(3.85239056755428,-6.19641930517066,
83.4460742343038));
#184944=CARTESIAN_POINT('Ctrl Pts',(6.34952905775618,-3.60779196247734,
83.6047416995901));
#184945=CARTESIAN_POINT('Ctrl Pts',(7.30044898119642,-0.119263707518461,
83.7634091648767));
#184946=CARTESIAN_POINT('Ctrl Pts',(6.46880555178464,3.35964425193858,83.9220766301628));
#184947=CARTESIAN_POINT('Ctrl Pts',(3.27863805495089,6.99511654521669,84.1336332505451));
#184948=CARTESIAN_POINT('Ctrl Pts',(-1.93422387439578,7.47150887855398,
84.3451898709266));
#184949=CARTESIAN_POINT('Ctrl Pts',(-5.72469512022691,4.50639009190849,
84.5567464913088));
#184950=CARTESIAN_POINT('Ctrl Pts',(-7.71679250871388,0.12561964834773,
84.7683031116905));
#184951=CARTESIAN_POINT('Ctrl Pts',(-6.02959695876113,-4.82960490013786,
84.9798597320726));
#184952=CARTESIAN_POINT('Ctrl Pts',(-1.74664355286513,-7.07685601560598,
85.1914163524544));
#184953=CARTESIAN_POINT('Ctrl Pts',(1.83027665600578,-7.06830011540703,
85.3500838177409));
#184954=CARTESIAN_POINT('Ctrl Pts',(4.99795282841499,-5.32476756532573,
85.5087512830274));
#184955=CARTESIAN_POINT('Ctrl Pts',(6.92779700763227,-2.28957505042186,
85.6674187483137));
#184956=CARTESIAN_POINT('Ctrl Pts',(7.18667145538067,1.2978580400887,85.8260862136001));
#184957=CARTESIAN_POINT('Ctrl Pts',(5.68179560826557,4.5856273098538,85.9847536788866));
#184958=CARTESIAN_POINT('Ctrl Pts',(2.81440621039045,6.72396999170129,86.1434211441729));
#184959=CARTESIAN_POINT('Ctrl Pts',(-1.96419739535731,7.47148255492902,
86.3549777645549));
#184960=CARTESIAN_POINT('Ctrl Pts',(-6.27191716258488,4.49752398818139,
86.5665343849368));
#184961=CARTESIAN_POINT('Ctrl Pts',(-7.28262268868008,-0.207587702725921,
86.7780910053187));
#184962=CARTESIAN_POINT('Ctrl Pts',(-6.0055420565309,-4.84748713518995,
86.9896476257005));
#184963=CARTESIAN_POINT('Ctrl Pts',(-1.53541180788712,-7.57123725402508,
87.2012042460826));
#184964=CARTESIAN_POINT('Ctrl Pts',(3.19285241050017,-6.55273593632057,
87.4127608664643));
#184965=CARTESIAN_POINT('Ctrl Pts',(5.93378011989038,-4.25453083756324,
87.5714283317508));
#184966=CARTESIAN_POINT('Ctrl Pts',(7.24893206726411,-0.886378014165637,
87.7300957970374));
#184967=CARTESIAN_POINT('Ctrl Pts',(6.78612783456396,2.68048396813518,87.8887632623237));
#184968=CARTESIAN_POINT('Ctrl Pts',(4.68652417010452,5.60081898500862,88.0474307276101));
#184969=CARTESIAN_POINT('Ctrl Pts',(1.42467490292049,7.16108096448926,88.2060981928966));
#184970=CARTESIAN_POINT('Ctrl Pts',(-2.14692484031357,6.96587169681071,
88.3647656581829));
#184971=CARTESIAN_POINT('Ctrl Pts',(-6.2949143853457,4.47830055464174,88.5763222785649));
#184972=CARTESIAN_POINT('Ctrl Pts',(-7.69710713562227,-0.564985540828742,
88.7878788989468));
#184973=CARTESIAN_POINT('Ctrl Pts',(-5.45870349896631,-4.82516756085981,
88.9994355193286));
#184974=CARTESIAN_POINT('Ctrl Pts',(-1.50548545536504,-7.56955616019048,
89.2109921397107));
#184975=CARTESIAN_POINT('Ctrl Pts',(3.67177574156303,-6.79699829926463,
89.4225487600925));
#184976=CARTESIAN_POINT('Ctrl Pts',(6.64967680960369,-2.98570813948777,
89.6341053804744));
#184977=CARTESIAN_POINT('Ctrl Pts',(7.28180167568186,0.534923840390631,
89.7927728457607));
#184978=CARTESIAN_POINT('Ctrl Pts',(6.13370953240971,3.96362075277572,89.9514403110474));
#184979=CARTESIAN_POINT('Ctrl Pts',(3.49317025910436,6.40580102964331,90.1101077763336));
#184980=CARTESIAN_POINT('Ctrl Pts',(0.0100858356748187,7.30291588173718,
90.2687752416203));
#184981=CARTESIAN_POINT('Ctrl Pts',(-3.49402507240063,6.41112844610182,
90.4274427069065));
#184982=CARTESIAN_POINT('Ctrl Pts',(-6.11128390418936,3.97301696557805,
90.586110172193));
#184983=CARTESIAN_POINT('Ctrl Pts',(-7.70244879166303,-0.594479258170914,
90.7976667925749));
#184984=CARTESIAN_POINT('Ctrl Pts',(-5.54797533933734,-5.3651315503526,
91.0092234129566));
#184985=CARTESIAN_POINT('Ctrl Pts',(-1.0999147271144,-7.2020742479624,91.2207800333388));
#184986=CARTESIAN_POINT('Ctrl Pts',(3.69367658136524,-6.77653452959786,
91.4323366537205));
#184987=CARTESIAN_POINT('Ctrl Pts',(7.17389309592108,-2.86642300166554,
91.6438932741026));
#184988=CARTESIAN_POINT('Ctrl Pts',(7.01857685474278,1.96779920245041,91.8554498944844));
#184989=CARTESIAN_POINT('Ctrl Pts',(5.24835772874336,5.07597481362446,92.0141173597708));
#184990=CARTESIAN_POINT('Ctrl Pts',(2.17016344940649,6.97302464538271,92.1727848250574));
#184991=CARTESIAN_POINT('Ctrl Pts',(-1.42191810959926,7.15644284387873,
92.3314522903436));
#184992=CARTESIAN_POINT('Ctrl Pts',(-4.67103607877668,5.6137424281515,92.4901197556303));
#184993=CARTESIAN_POINT('Ctrl Pts',(-6.7901973045322,2.68402677631578,92.6487872209163));
#184994=CARTESIAN_POINT('Ctrl Pts',(-7.23773325362728,-0.864795977685073,
92.8074546862032));
#184995=CARTESIAN_POINT('Ctrl Pts',(-5.53318091736492,-5.39119949546233,
93.0190113065847));
#184996=CARTESIAN_POINT('Ctrl Pts',(-0.822518600318388,-7.67386017329631,
93.2305679269669));
#184997=CARTESIAN_POINT('Ctrl Pts',(3.7696437407526,-6.23453863249735,93.4421245473486));
#184998=CARTESIAN_POINT('Ctrl Pts',(7.17759831039387,-2.83667934145,93.6536811677308));
#184999=CARTESIAN_POINT('Ctrl Pts',(7.34465462839491,2.39523911495703,93.8652377881125));
#185000=CARTESIAN_POINT('Ctrl Pts',(4.12824572376432,6.00751555059719,94.0767944084945));
#185001=CARTESIAN_POINT('Ctrl Pts',(0.77772276897837,7.25988463091326,94.2354618737807));
#185002=CARTESIAN_POINT('Ctrl Pts',(-2.80114571582029,6.74435065760574,
94.3941293390673));
#185003=CARTESIAN_POINT('Ctrl Pts',(-5.67670789282248,4.58383194552335,
94.5527968043538));
#185004=CARTESIAN_POINT('Ctrl Pts',(-7.18305822535622,1.31770430691009,
94.7114642696399));
#185005=CARTESIAN_POINT('Ctrl Pts',(-6.93319317044822,-2.28946327644473,
94.8701317349268));
#185006=CARTESIAN_POINT('Ctrl Pts',(-5.00317805612032,-5.3010195757933,
95.0287992002129));
#185007=CARTESIAN_POINT('Ctrl Pts',(-0.794465437437333,-7.68440215607981,
95.240355820595));
#185008=CARTESIAN_POINT('Ctrl Pts',(4.28490662509514,-6.41905264174572,
95.4519124409768));
#185009=CARTESIAN_POINT('Ctrl Pts',(6.88866860112665,-2.37186857879187,
95.6634690613587));
#185010=CARTESIAN_POINT('Ctrl Pts',(7.32848383063589,2.42047858723411,95.8750256817408));
#185011=CARTESIAN_POINT('Ctrl Pts',(4.10468304959734,6.54456291005869,96.0865823021226));
#185012=CARTESIAN_POINT('Ctrl Pts',(-0.679028220406464,7.25757857856497,
96.2981389225044));
#185013=CARTESIAN_POINT('Ctrl Pts',(-4.05427435445187,6.07236054551145,
96.4568063877909));
#185014=CARTESIAN_POINT('Ctrl Pts',(-6.47127337767883,3.38407271816423,
96.6154738530771));
#185015=CARTESIAN_POINT('Ctrl Pts',(-7.29616857577915,-0.117923577904248,
96.7741413183638));
#185016=CARTESIAN_POINT('Ctrl Pts',(-6.35800508006628,-3.58921836875169,
96.9328087836501));
#185017=CARTESIAN_POINT('Ctrl Pts',(-3.85933553387998,-6.20169133701876,
97.0914762489367));
#185018=CARTESIAN_POINT('Ctrl Pts',(-0.440438479635075,-7.27223127969294,
97.2501437142229));
#185019=CARTESIAN_POINT('Ctrl Pts',(4.30252989486086,-6.41644447484644,
97.461700334605));
#185020=CARTESIAN_POINT('Ctrl Pts',(8.19966432523079,-1.11131240077915,
97.7261461100822));
#185021=CARTESIAN_POINT('Ctrl Pts',(5.85497146417381,5.04026049610663,97.9905918855599));
#185022=CARTESIAN_POINT('Ctrl Pts',(1.51099084548737,7.12682197675247,98.2021485059416));
#185023=CARTESIAN_POINT('Ctrl Pts',(-2.06992536476643,7.0058668122941,98.3608159712281));
#185024=CARTESIAN_POINT('Ctrl Pts',(-5.17287422036002,5.15049374409499,
98.5194834365144));
#185025=CARTESIAN_POINT('Ctrl Pts',(-7.00278762888398,2.05811838864922,
98.6781509018009));
#185026=CARTESIAN_POINT('Ctrl Pts',(-7.13636830945152,-1.54513735705454,
98.8368339328175));
#185027=CARTESIAN_POINT('Ctrl Pts',(-6.06394139514141,-3.69210156778035,
98.9426278087385));
#185028=CARTESIAN_POINT('Ctrl Pts',(-5.30378086654358,-4.57361536730065,
98.9955325295642));
#185029=CARTESIAN_POINT('Ctrl Pts',(2.10208451021625,-7.84862588447231,
-3.290770433928E-15));
#185030=CARTESIAN_POINT('Ctrl Pts',(2.29962771051048,-7.78108676365297,
-5.16703836131539E-15));
#185031=CARTESIAN_POINT('Ctrl Pts',(2.49411343411202,-7.70593369986541,
-3.15384150650199E-16));
#185032=CARTESIAN_POINT('Ctrl Pts',(2.68517636753987,-7.62347406731538,
-1.58206781009085E-15));
#185033=CARTESIAN_POINT('Ctrl Pts',(2.88113552763045,-7.53890130353552,
-2.88121182275299E-15));
#185034=CARTESIAN_POINT('Ctrl Pts',(3.07349491021749,-7.44664244674981,
-5.00442052337E-15));
#185035=CARTESIAN_POINT('Ctrl Pts',(3.26183706294806,-7.3469783482138,-5.12090370108353E-15));
#185036=CARTESIAN_POINT('Ctrl Pts',(3.44701891521803,-7.24898657046175,
-5.23543234108555E-15));
#185037=CARTESIAN_POINT('Ctrl Pts',(3.62831770409081,-7.14383543019674,
-3.83143952960435E-15));
#185038=CARTESIAN_POINT('Ctrl Pts',(3.80530588214224,-7.03174992031122,
-3.38618022510673E-15));
#185039=CARTESIAN_POINT('Ctrl Pts',(3.98682476188306,-6.91679514528841,
-2.92952277466898E-15));
#185040=CARTESIAN_POINT('Ctrl Pts',(4.16381029498468,-6.79454614842656,
-2.24677972717022E-15));
#185041=CARTESIAN_POINT('Ctrl Pts',(4.33575872179093,-6.66520704214514,
-3.27515792264421E-15));
#185042=CARTESIAN_POINT('Ctrl Pts',(4.42173293519406,-6.60053748900443,
-3.78934702038121E-15));
#185043=CARTESIAN_POINT('Ctrl Pts',(4.50644714130402,-6.53409484017392,
-2.34365924677727E-15));
#185044=CARTESIAN_POINT('Ctrl Pts',(4.58983358603305,-6.46590148664305,
-2.80331313717852E-15));
#185045=CARTESIAN_POINT('Ctrl Pts',(4.63152680839756,-6.43180480987762,
-3.03314008237915E-15));
#185046=CARTESIAN_POINT('Ctrl Pts',(4.67288803734242,-6.3972704267277,2.90312324695387E-16));
#185047=CARTESIAN_POINT('Ctrl Pts',(4.71390847258368,-6.36230096370932,
-1.38777878078145E-16));
#185048=CARTESIAN_POINT('Ctrl Pts',(4.73461573528928,-6.34464825346536,
-3.55384150073381E-16));
#185049=CARTESIAN_POINT('Ctrl Pts',(4.75523615107994,-6.32688467152668,
1.18624335832746E-15));
#185050=CARTESIAN_POINT('Ctrl Pts',(4.77576856551071,-6.30901054537397,
7.49400541621981E-16));
#185051=CARTESIAN_POINT('Ctrl Pts',(4.79591021739563,-6.29147659056661,
3.20871496867989E-16));
#185052=CARTESIAN_POINT('Ctrl Pts',(4.81596202834693,-6.27384070654854,
1.48999836866843E-15));
#185053=CARTESIAN_POINT('Ctrl Pts',(4.83591612347545,-6.25610961852038,
1.33226762955019E-15));
#185054=CARTESIAN_POINT('Ctrl Pts',(4.98978344512459,-6.11938404879417,
-1.0694073052437E-16));
#185055=CARTESIAN_POINT('Ctrl Pts',(5.13797274440312,-5.97688834344088,
-6.37152335888765E-16));
#185056=CARTESIAN_POINT('Ctrl Pts',(5.28010241489011,-5.82886074576049,
3.13638004456607E-15));
#185057=CARTESIAN_POINT('Ctrl Pts',(5.32388371551095,-5.78326266105362,
5.08932056714925E-15));
#185058=CARTESIAN_POINT('Ctrl Pts',(5.36708977798512,-5.73713940061267,
3.61201614627145E-15));
#185059=CARTESIAN_POINT('Ctrl Pts',(5.40970872589629,-5.69049723734325,
2.96984659087229E-15));
#185060=CARTESIAN_POINT('Ctrl Pts',(5.54848269366366,-5.53862305040551,
1.23002056944179E-15));
#185061=CARTESIAN_POINT('Ctrl Pts',(5.68103508731973,-5.38124932257935,
1.45242263650514E-15));
#185062=CARTESIAN_POINT('Ctrl Pts',(5.80714429668145,-5.21882934647248,
1.88737914186277E-15));
#185063=CARTESIAN_POINT('Ctrl Pts',(5.93327032734641,-5.05638770568561,
4.98380169643257E-15));
#185064=CARTESIAN_POINT('Ctrl Pts',(6.05295174788962,-4.88889779050302,
3.62171887105232E-16));
#185065=CARTESIAN_POINT('Ctrl Pts',(6.16592022815171,-4.71679013773437,
1.30451205393456E-15));
#185066=CARTESIAN_POINT('Ctrl Pts',(6.27792279739088,-4.5461540518891,3.75006097235274E-15));
#185067=CARTESIAN_POINT('Ctrl Pts',(6.38332694768264,-4.37097818866154,
-2.53100327216846E-15));
#185068=CARTESIAN_POINT('Ctrl Pts',(6.48182164283881,-4.19166967163302,
-2.4980018054066E-15));
#185069=CARTESIAN_POINT('Ctrl Pts',(6.52326227113616,-4.11622746032462,
-3.45241306837116E-15));
#185070=CARTESIAN_POINT('Ctrl Pts',(6.56347915093949,-4.04005358422469,
-2.64250873965109E-15));
#185071=CARTESIAN_POINT('Ctrl Pts',(6.60244631812086,-3.96317813022292,
-8.32667268468867E-16));
#185072=CARTESIAN_POINT('Ctrl Pts',(6.61905364025482,-3.9304147675987,9.32549959876183E-17));
#185073=CARTESIAN_POINT('Ctrl Pts',(6.63543635568491,-3.89751882078441,
-2.52119858109353E-16));
#185074=CARTESIAN_POINT('Ctrl Pts',(6.65157567526072,-3.86452741946229,
-7.7715611723761E-16));
#185075=CARTESIAN_POINT('Ctrl Pts',(6.74048447841371,-3.68278332596983,
-3.66949276078462E-15));
#185076=CARTESIAN_POINT('Ctrl Pts',(6.82211074143566,-3.49795239268472,
-5.08282477872157E-15));
#185077=CARTESIAN_POINT('Ctrl Pts',(6.89625206046576,-3.31046675549432,
-4.88498130835069E-15));
#185078=CARTESIAN_POINT('Ctrl Pts',(6.9699232370716,-3.12416999588444,-4.68839239630173E-15));
#185079=CARTESIAN_POINT('Ctrl Pts',(7.03620429877872,-2.93525142177202,
-7.13421723312083E-15));
#185080=CARTESIAN_POINT('Ctrl Pts',(7.09484826120896,-2.74411884411799,
-5.49560397189452E-15));
#185081=CARTESIAN_POINT('Ctrl Pts',(7.13726862362652,-2.60586227212168,
-4.31030602266199E-15));
#185082=CARTESIAN_POINT('Ctrl Pts',(7.17569194887325,-2.46644687839578,
-7.62442829405664E-15));
#185083=CARTESIAN_POINT('Ctrl Pts',(7.21000787802524,-2.32602464360175,
-9.10382880192628E-15));
#185084=CARTESIAN_POINT('Ctrl Pts',(7.25913415483096,-2.12499783923887,
-1.13420163587531E-14));
#185085=CARTESIAN_POINT('Ctrl Pts',(7.29984486455965,-1.92190694651327,
-8.44330237013337E-15));
#185086=CARTESIAN_POINT('Ctrl Pts',(7.33208917201402,-1.71725913517378,
-9.43689570931383E-15));
#185087=CARTESIAN_POINT('Ctrl Pts',(7.36433347946838,-1.51261132383428,
-1.04304890484943E-14));
#185088=CARTESIAN_POINT('Ctrl Pts',(7.38811133250517,-1.30640578628499,
-2.38941095831012E-14));
#185089=CARTESIAN_POINT('Ctrl Pts',(7.40331446894898,-1.09916311536333,
-1.06026298851702E-14));
#185090=CARTESIAN_POINT('Ctrl Pts',(7.40617088924807,-1.06022561228647,
-9.55573486110841E-15));
#185091=CARTESIAN_POINT('Ctrl Pts',(7.40872267048525,-1.0212752751884,-1.0646464482034E-14));
#185092=CARTESIAN_POINT('Ctrl Pts',(7.41096959872409,-0.982324841880129,
-1.04360964314765E-14));
#185093=CARTESIAN_POINT('Ctrl Pts',(7.42235430710878,-0.784971265113983,
-9.37020617843963E-15));
#185094=CARTESIAN_POINT('Ctrl Pts',(7.42592266440482,-0.587537835352548,
-1.293591650313E-14));
#185095=CARTESIAN_POINT('Ctrl Pts',(7.42170473423292,-0.390466204597829,
-1.06026298851702E-14));
#185096=CARTESIAN_POINT('Ctrl Pts',(7.41749426002231,-0.193742933913072,
-8.27346777709736E-15));
#185097=CARTESIAN_POINT('Ctrl Pts',(7.40552490615871,0.00262049832885516,
-6.9361844842518E-15));
#185098=CARTESIAN_POINT('Ctrl Pts',(7.3857749724574,0.198180275996753,-7.7715611723761E-15));
#185099=CARTESIAN_POINT('Ctrl Pts',(7.36615089037624,0.3924938968305,-8.60161462695303E-15));
#185100=CARTESIAN_POINT('Ctrl Pts',(7.33884495154307,0.586014712140499,
-6.51498341349402E-15));
#185101=CARTESIAN_POINT('Ctrl Pts',(7.3037865412977,0.778293044380834,-5.38458166943201E-15));
#185102=CARTESIAN_POINT('Ctrl Pts',(7.26872813105233,0.97057137662117,-4.25417992536999E-15));
#185103=CARTESIAN_POINT('Ctrl Pts',(7.22591719058655,1.16160786872303,-3.07562274669201E-15));
#185104=CARTESIAN_POINT('Ctrl Pts',(7.17523488235407,1.35092889849934,-3.49720252756924E-15));
#185105=CARTESIAN_POINT('Ctrl Pts',(7.15288410775808,1.43441901192123,-2.89610734490173E-15));
#185106=CARTESIAN_POINT('Ctrl Pts',(7.12900186354509,1.51757513502465,-7.5026934907553E-15));
#185107=CARTESIAN_POINT('Ctrl Pts',(7.10360232537748,1.60035343100048,-3.33066907387547E-15));
#185108=CARTESIAN_POINT('Ctrl Pts',(7.09112003500542,1.64103380558275,-1.28037903052207E-15));
#185109=CARTESIAN_POINT('Ctrl Pts',(7.07827076461064,1.68162450295897,-1.8855884437478E-15));
#185110=CARTESIAN_POINT('Ctrl Pts',(7.06505739175309,1.72211611694885,-4.44089209850063E-16));
#185111=CARTESIAN_POINT('Ctrl Pts',(7.0544290607665,1.7546860202056,7.15397557075437E-16));
#185112=CARTESIAN_POINT('Ctrl Pts',(7.04356771062853,1.78718385328651,1.24968543471361E-16));
#185113=CARTESIAN_POINT('Ctrl Pts',(7.0324785567182,1.8195956752456,3.33066907387547E-16));
#185114=CARTESIAN_POINT('Ctrl Pts',(6.96943089491119,2.00387389935086,1.51621535828537E-15));
#185115=CARTESIAN_POINT('Ctrl Pts',(6.89898792830898,2.1854825028391,1.33828956628801E-15));
#185116=CARTESIAN_POINT('Ctrl Pts',(6.82139528078071,2.36395748737489,1.4432899320127E-15));
#185117=CARTESIAN_POINT('Ctrl Pts',(6.74433218910303,2.54121441227158,1.54757368914425E-15));
#185118=CARTESIAN_POINT('Ctrl Pts',(6.66021621392354,2.71538095692703,1.6559467280731E-15));
#185119=CARTESIAN_POINT('Ctrl Pts',(6.56924627918247,2.88597335464335,1.77635683940025E-15));
#185120=CARTESIAN_POINT('Ctrl Pts',(6.50266459558114,3.01083140892107,1.86448604337962E-15));
#185121=CARTESIAN_POINT('Ctrl Pts',(6.43241042807166,3.13377426257987,2.03877470991558E-15));
#185122=CARTESIAN_POINT('Ctrl Pts',(6.3585495483742,3.25459937292915,0.));
#185123=CARTESIAN_POINT('Ctrl Pts',(6.34340397157949,3.27937522172788,-7.56577460625889E-16));
#185124=CARTESIAN_POINT('Ctrl Pts',(6.32810731413255,3.30406089503788,2.43515525521077E-15));
#185125=CARTESIAN_POINT('Ctrl Pts',(6.31266697535328,3.32864399987372,1.77635683940025E-15));
#185126=CARTESIAN_POINT('Ctrl Pts',(6.21101507324467,3.49048755797315,1.06570322610702E-15));
#185127=CARTESIAN_POINT('Ctrl Pts',(6.10306202439148,3.64801466098077,-3.81869933772724E-15));
#185128=CARTESIAN_POINT('Ctrl Pts',(5.98901561316641,3.80076293866515,-2.77555756156289E-15));
#185129=CARTESIAN_POINT('Ctrl Pts',(5.8769084671812,3.95091385776383,-1.13531658097703E-15));
#185130=CARTESIAN_POINT('Ctrl Pts',(5.75891294518698,4.09644756264395,-7.79843788104419E-16));
#185131=CARTESIAN_POINT('Ctrl Pts',(5.63519336749352,4.23688737897504,1.77635683940025E-15));
#185132=CARTESIAN_POINT('Ctrl Pts',(5.57235559782876,4.30821743841185,-1.38140305958728E-15));
#185133=CARTESIAN_POINT('Ctrl Pts',(5.50804072164468,4.37823279464964,-1.50833598234392E-15));
#185134=CARTESIAN_POINT('Ctrl Pts',(5.44226749982665,4.44686660289082,-6.66133814775094E-16));
#185135=CARTESIAN_POINT('Ctrl Pts',(5.39900343271652,4.49201229598133,-4.7094403649886E-16));
#185136=CARTESIAN_POINT('Ctrl Pts',(5.35510834142393,4.53656016442929,-5.35226817025197E-16));
#185137=CARTESIAN_POINT('Ctrl Pts',(5.31059519289858,4.58050191706158,-5.55111512312578E-16));
#185138=CARTESIAN_POINT('Origin',(0.,0.,100.));
#185139=CARTESIAN_POINT('',(-4.,4.89858719658941E-16,100.));
#185140=CARTESIAN_POINT('Origin',(0.,0.,100.));
#185141=CARTESIAN_POINT('Origin',(0.,0.,0.));
#185142=CARTESIAN_POINT('',(-4.,-4.89858719658941E-16,0.));
#185143=CARTESIAN_POINT('Origin',(0.,0.,0.));
#185144=CARTESIAN_POINT('Origin',(0.,0.,0.));
#185145=CARTESIAN_POINT('Origin',(0.,0.,0.));
#289354=UNCERTAINTY_MEASURE_WITH_UNIT(LENGTH_MEASURE(0.01),#289388,
'DISTANCE_ACCURACY_VALUE',
'Maximum model space distance between geometric entities at asserted c
onnectivities');
#289368=UNCERTAINTY_MEASURE_WITH_UNIT(LENGTH_MEASURE(0.01),#289388,
'DISTANCE_ACCURACY_VALUE',
'Maximum model space distance between geometric entities at asserted c
onnectivities');
#289373=(
GEOMETRIC_REPRESENTATION_CONTEXT(3)
GLOBAL_UNCERTAINTY_ASSIGNED_CONTEXT((#289354))
GLOBAL_UNIT_ASSIGNED_CONTEXT((#289388,#289390,#289391))
REPRESENTATION_CONTEXT('','3D')
);
#289387=(
GEOMETRIC_REPRESENTATION_CONTEXT(3)
GLOBAL_UNCERTAINTY_ASSIGNED_CONTEXT((#289368))
GLOBAL_UNIT_ASSIGNED_CONTEXT((#289388,#289390,#289391))
REPRESENTATION_CONTEXT('','3D')
);
#289388=(
LENGTH_UNIT()
NAMED_UNIT(*)
SI_UNIT(.MILLI.,.METRE.)
);
#289390=(
NAMED_UNIT(*)
PLANE_ANGLE_UNIT()
SI_UNIT($,.RADIAN.)
);
#289391=(
NAMED_UNIT(*)
SI_UNIT($,.STERADIAN.)
SOLID_ANGLE_UNIT()
);
#289396=SHAPE_DEFINITION_REPRESENTATION(#289414,#289457);
#289414=PRODUCT_DEFINITION_SHAPE('',$,#289476);
#289457=SHAPE_REPRESENTATION('',(#17450),#289373);
#289471=PRODUCT_DEFINITION_CONTEXT('part definition',#289527,'design');
#289476=PRODUCT_DEFINITION('Quill','Quill',#289494,#289471);
#289494=PRODUCT_DEFINITION_FORMATION('',$,#289533);
#289527=APPLICATION_CONTEXT(
'Core Data for Automotive Mechanical Design Process');
#289528=PRODUCT_CONTEXT('part definition',#289527,'mechanical');
#289533=PRODUCT('Quill','Quill',$,(#289528));
#289551=PRESENTATION_STYLE_ASSIGNMENT((#289558));
#289558=SURFACE_STYLE_USAGE(.BOTH.,#289565);
#289565=SURFACE_SIDE_STYLE('',(#289572));
#289572=SURFACE_STYLE_FILL_AREA(#289579);
#289579=FILL_AREA_STYLE('Opaque(169,212,242)',(#289586));
#289586=FILL_AREA_STYLE_COLOUR('Opaque(169,212,242)',#289593);
#289593=COLOUR_RGB('Opaque(169,212,242)',0.662745098039216,0.831372549019608,
0.949019607843137);
ENDSEC;
END-ISO-10303-21;
